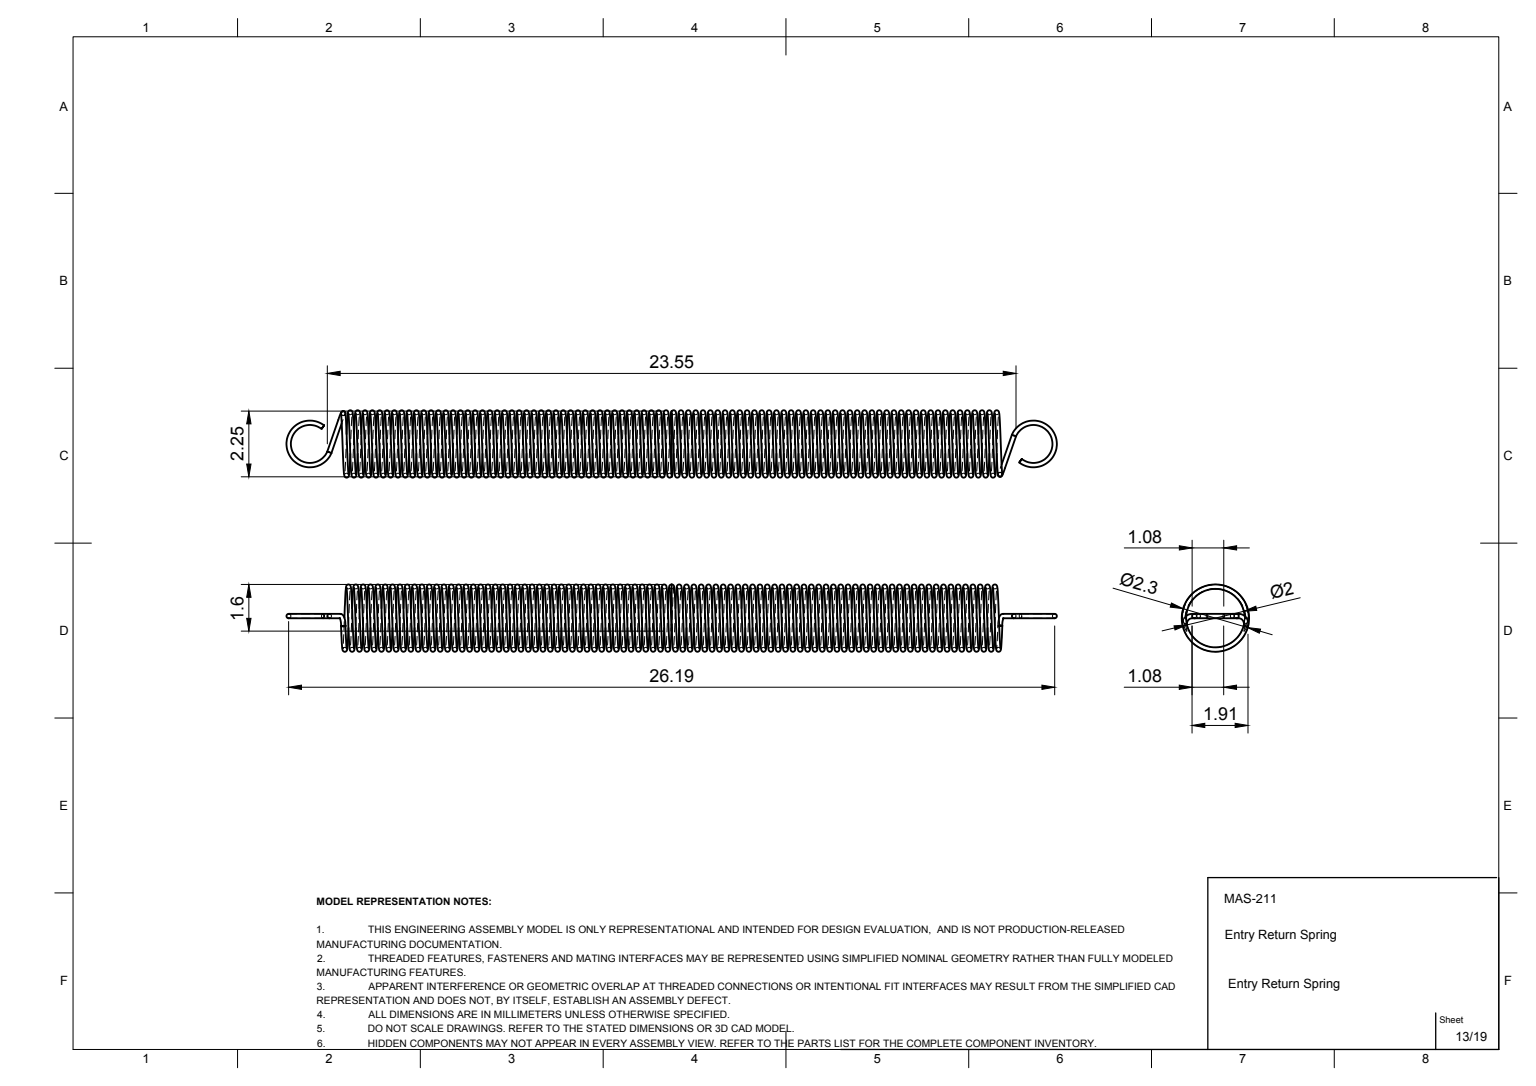
ISO-10303-21;
HEADER;
FILE_DESCRIPTION(
 (''),
 '2;1');
FILE_NAME ( 'Entry Return Spring.step', '2026-10-05T20:07:59+06:00', ( '' ), ( '' ), 'STEP AP214', 'Unspecified', '' );
FILE_SCHEMA (('AUTOMOTIVE_DESIGN { 1 0 10303 214 3 1 1 }'));
ENDSEC;
DATA;
#10=MECHANICAL_DESIGN_GEOMETRIC_PRESENTATION_REPRESENTATION('',(#331),#196741);
#19=(
BOUNDED_CURVE()
B_SPLINE_CURVE(3,(#132841,#132842,#132843,#132844,#132845,#132846,#132847,
#132848,#132849,#132850,#132851,#132852,#132853,#132854,#132855,#132856,
#132857,#132858,#132859,#132860,#132861,#132862,#132863,#132864,#132865,
#132866,#132867,#132868,#132869,#132870,#132871,#132872,#132873,#132874,
#132875,#132876,#132877,#132878,#132879,#132880,#132881,#132882,#132883,
#132884,#132885,#132886,#132887,#132888,#132889,#132890,#132891,#132892,
#132893,#132894,#132895,#132896,#132897,#132898,#132899,#132900,#132901,
#132902,#132903,#132904,#132905,#132906,#132907,#132908,#132909,#132910,
#132911,#132912,#132913,#132914,#132915,#132916,#132917,#132918,#132919,
#132920,#132921,#132922,#132923,#132924,#132925,#132926,#132927,#132928,
#132929,#132930,#132931,#132932,#132933,#132934,#132935,#132936,#132937,
#132938,#132939,#132940,#132941,#132942,#132943,#132944,#132945,#132946,
#132947,#132948,#132949,#132950,#132951,#132952,#132953,#132954,#132955,
#132956,#132957,#132958,#132959,#132960,#132961,#132962,#132963,#132964,
#132965,#132966,#132967,#132968,#132969,#132970,#132971,#132972,#132973,
#132974,#132975,#132976,#132977,#132978,#132979,#132980,#132981,#132982,
#132983,#132984,#132985,#132986,#132987,#132988,#132989,#132990,#132991,
#132992,#132993,#132994,#132995,#132996,#132997,#132998,#132999,#133000,
#133001,#133002,#133003,#133004,#133005,#133006,#133007,#133008,#133009,
#133010,#133011,#133012,#133013,#133014,#133015,#133016,#133017,#133018,
#133019,#133020,#133021,#133022,#133023,#133024,#133025,#133026,#133027,
#133028,#133029,#133030,#133031,#133032,#133033,#133034,#133035,#133036,
#133037,#133038,#133039,#133040,#133041,#133042,#133043,#133044,#133045,
#133046,#133047,#133048,#133049,#133050,#133051,#133052,#133053,#133054,
#133055,#133056,#133057,#133058,#133059,#133060,#133061,#133062,#133063,
#133064,#133065,#133066,#133067,#133068,#133069,#133070,#133071,#133072,
#133073,#133074,#133075,#133076,#133077,#133078,#133079,#133080,#133081,
#133082,#133083,#133084,#133085,#133086,#133087,#133088,#133089,#133090,
#133091,#133092,#133093,#133094,#133095,#133096,#133097,#133098,#133099,
#133100,#133101,#133102,#133103,#133104,#133105,#133106,#133107,#133108,
#133109,#133110,#133111,#133112,#133113,#133114,#133115,#133116,#133117,
#133118,#133119,#133120,#133121,#133122,#133123,#133124,#133125,#133126,
#133127,#133128,#133129,#133130,#133131,#133132,#133133,#133134,#133135,
#133136,#133137,#133138,#133139,#133140,#133141,#133142,#133143,#133144,
#133145,#133146,#133147,#133148,#133149,#133150,#133151,#133152,#133153,
#133154,#133155,#133156,#133157,#133158,#133159,#133160,#133161,#133162,
#133163,#133164,#133165,#133166,#133167,#133168,#133169,#133170,#133171,
#133172,#133173,#133174,#133175,#133176,#133177,#133178,#133179,#133180,
#133181,#133182,#133183,#133184,#133185,#133186,#133187,#133188,#133189,
#133190,#133191,#133192,#133193,#133194,#133195,#133196,#133197,#133198,
#133199,#133200,#133201,#133202,#133203,#133204,#133205,#133206,#133207,
#133208,#133209,#133210,#133211,#133212,#133213,#133214,#133215,#133216,
#133217,#133218,#133219,#133220,#133221,#133222,#133223,#133224,#133225,
#133226,#133227,#133228,#133229,#133230,#133231,#133232,#133233,#133234,
#133235,#133236,#133237,#133238,#133239,#133240,#133241,#133242,#133243,
#133244,#133245,#133246,#133247,#133248,#133249,#133250,#133251,#133252,
#133253,#133254,#133255,#133256,#133257,#133258,#133259,#133260,#133261,
#133262,#133263,#133264,#133265,#133266,#133267,#133268,#133269,#133270,
#133271,#133272,#133273,#133274,#133275,#133276,#133277,#133278,#133279,
#133280,#133281,#133282,#133283,#133284,#133285,#133286,#133287,#133288,
#133289,#133290,#133291,#133292,#133293,#133294,#133295,#133296,#133297,
#133298,#133299,#133300,#133301,#133302,#133303,#133304,#133305,#133306,
#133307,#133308,#133309,#133310,#133311,#133312,#133313,#133314,#133315,
#133316,#133317,#133318,#133319,#133320,#133321,#133322,#133323,#133324,
#133325,#133326,#133327,#133328,#133329,#133330,#133331,#133332,#133333,
#133334,#133335,#133336,#133337,#133338,#133339,#133340,#133341,#133342,
#133343,#133344,#133345,#133346,#133347,#133348,#133349,#133350,#133351,
#133352,#133353,#133354,#133355,#133356,#133357,#133358,#133359,#133360,
#133361,#133362,#133363,#133364,#133365,#133366,#133367,#133368,#133369,
#133370,#133371,#133372,#133373,#133374,#133375,#133376,#133377,#133378,
#133379,#133380,#133381,#133382,#133383,#133384,#133385,#133386,#133387,
#133388,#133389,#133390,#133391,#133392,#133393,#133394,#133395,#133396,
#133397,#133398,#133399,#133400,#133401,#133402,#133403,#133404,#133405,
#133406,#133407,#133408,#133409,#133410,#133411,#133412,#133413,#133414,
#133415,#133416,#133417,#133418,#133419,#133420,#133421,#133422,#133423,
#133424,#133425,#133426,#133427,#133428,#133429,#133430,#133431,#133432,
#133433,#133434,#133435,#133436,#133437,#133438,#133439,#133440,#133441,
#133442,#133443,#133444,#133445,#133446,#133447,#133448,#133449,#133450,
#133451,#133452,#133453,#133454,#133455,#133456,#133457,#133458,#133459,
#133460,#133461,#133462,#133463,#133464,#133465,#133466,#133467,#133468,
#133469,#133470,#133471,#133472,#133473,#133474,#133475,#133476,#133477,
#133478,#133479,#133480,#133481,#133482,#133483,#133484,#133485,#133486,
#133487,#133488,#133489,#133490,#133491,#133492,#133493,#133494,#133495,
#133496,#133497,#133498,#133499,#133500,#133501,#133502,#133503,#133504,
#133505,#133506,#133507,#133508,#133509,#133510,#133511,#133512,#133513,
#133514,#133515,#133516,#133517,#133518,#133519,#133520,#133521,#133522,
#133523,#133524,#133525,#133526,#133527,#133528,#133529,#133530,#133531,
#133532,#133533,#133534,#133535,#133536,#133537,#133538,#133539,#133540,
#133541,#133542,#133543,#133544,#133545,#133546,#133547,#133548,#133549,
#133550,#133551,#133552,#133553,#133554,#133555,#133556,#133557,#133558,
#133559,#133560,#133561,#133562,#133563,#133564,#133565,#133566,#133567,
#133568,#133569,#133570,#133571,#133572,#133573,#133574,#133575,#133576,
#133577,#133578,#133579,#133580,#133581,#133582,#133583,#133584,#133585,
#133586,#133587,#133588,#133589,#133590,#133591,#133592,#133593,#133594,
#133595,#133596,#133597,#133598,#133599,#133600,#133601,#133602,#133603,
#133604,#133605,#133606,#133607,#133608,#133609,#133610,#133611,#133612,
#133613,#133614,#133615,#133616,#133617,#133618,#133619,#133620,#133621,
#133622,#133623,#133624,#133625,#133626,#133627,#133628,#133629,#133630,
#133631,#133632,#133633,#133634,#133635,#133636,#133637,#133638,#133639,
#133640,#133641,#133642,#133643,#133644,#133645,#133646,#133647,#133648,
#133649,#133650,#133651,#133652,#133653,#133654,#133655,#133656,#133657,
#133658,#133659,#133660,#133661,#133662,#133663,#133664,#133665,#133666,
#133667,#133668,#133669,#133670,#133671,#133672,#133673,#133674,#133675,
#133676,#133677,#133678,#133679,#133680,#133681,#133682,#133683,#133684,
#133685,#133686,#133687,#133688,#133689,#133690,#133691,#133692,#133693,
#133694,#133695,#133696,#133697,#133698,#133699,#133700,#133701,#133702,
#133703,#133704,#133705,#133706,#133707,#133708,#133709,#133710,#133711,
#133712,#133713,#133714,#133715,#133716,#133717,#133718,#133719,#133720,
#133721,#133722,#133723,#133724,#133725,#133726,#133727,#133728,#133729,
#133730,#133731,#133732,#133733,#133734,#133735,#133736,#133737,#133738,
#133739,#133740,#133741,#133742,#133743,#133744,#133745,#133746,#133747,
#133748,#133749,#133750,#133751,#133752,#133753,#133754,#133755,#133756,
#133757,#133758,#133759,#133760,#133761,#133762,#133763,#133764,#133765,
#133766,#133767,#133768,#133769,#133770,#133771,#133772,#133773,#133774,
#133775,#133776,#133777,#133778,#133779,#133780,#133781,#133782,#133783,
#133784,#133785,#133786,#133787,#133788,#133789,#133790,#133791,#133792,
#133793,#133794,#133795,#133796,#133797,#133798,#133799,#133800,#133801,
#133802,#133803,#133804,#133805,#133806,#133807,#133808,#133809,#133810,
#133811,#133812,#133813,#133814,#133815,#133816,#133817,#133818,#133819,
#133820,#133821,#133822,#133823,#133824,#133825,#133826,#133827,#133828,
#133829,#133830,#133831,#133832,#133833,#133834,#133835,#133836,#133837,
#133838,#133839,#133840,#133841,#133842,#133843,#133844,#133845,#133846,
#133847,#133848,#133849,#133850,#133851,#133852,#133853,#133854,#133855,
#133856,#133857,#133858,#133859,#133860,#133861,#133862,#133863,#133864,
#133865,#133866,#133867,#133868,#133869,#133870,#133871,#133872,#133873,
#133874,#133875,#133876,#133877,#133878,#133879,#133880,#133881,#133882,
#133883,#133884,#133885,#133886,#133887,#133888,#133889,#133890,#133891,
#133892,#133893,#133894,#133895,#133896,#133897,#133898),.UNSPECIFIED.,
 .F.,.F.)
B_SPLINE_CURVE_WITH_KNOTS((4,1,1,1,1,1,1,1,1,1,1,1,1,1,1,1,1,1,1,1,1,1,
1,1,1,1,1,1,1,1,1,1,1,1,1,1,1,1,1,1,1,1,1,1,1,1,1,1,1,1,1,1,1,1,1,1,1,1,
1,1,1,1,1,1,1,1,1,1,1,1,1,1,1,1,1,1,1,1,1,1,1,1,1,1,1,1,1,1,1,1,1,1,1,1,
1,1,1,1,1,1,1,1,1,1,1,1,1,1,1,1,1,1,1,1,1,1,1,1,1,1,1,1,1,1,1,1,1,1,1,1,
1,1,1,1,1,1,1,1,1,1,1,1,1,1,1,1,1,1,1,1,1,1,1,1,1,1,1,1,1,1,1,1,1,1,1,1,
1,1,1,1,1,1,1,1,1,1,1,1,1,1,1,1,1,1,1,1,1,1,1,1,1,1,1,1,1,1,1,1,1,1,1,1,
1,1,1,1,1,1,1,1,1,1,1,1,1,1,1,1,1,1,1,1,1,1,1,1,1,1,1,1,1,1,1,1,1,1,1,1,
1,1,1,1,1,1,1,1,1,1,1,1,1,1,1,1,1,1,1,1,1,1,1,1,1,1,1,1,1,1,1,1,1,1,1,1,
1,1,1,1,1,1,1,1,1,1,1,1,1,1,1,1,1,1,1,1,1,1,1,1,1,1,1,1,1,1,1,1,1,1,1,1,
1,1,1,1,1,1,1,1,1,1,1,1,1,1,1,1,1,1,1,1,1,1,1,1,1,1,1,1,1,1,1,1,1,1,1,1,
1,1,1,1,1,1,1,1,1,1,1,1,1,1,1,1,1,1,1,1,1,1,1,1,1,1,1,1,1,1,1,1,1,1,1,1,
1,1,1,1,1,1,1,1,1,1,1,1,1,1,1,1,1,1,1,1,1,1,1,1,1,1,1,1,1,1,1,1,1,1,1,1,
1,1,1,1,1,1,1,1,1,1,1,1,1,1,1,1,1,1,1,1,1,1,1,1,1,1,1,1,1,1,1,1,1,1,1,1,
1,1,1,1,1,1,1,1,1,1,1,1,1,1,1,1,1,1,1,1,1,1,1,1,1,1,1,1,1,1,1,1,1,1,1,1,
1,1,1,1,1,1,1,1,1,1,1,1,1,1,1,1,1,1,1,1,1,1,1,1,1,1,1,1,1,1,1,1,1,1,1,1,
1,1,1,1,1,1,1,1,1,1,1,1,1,1,1,1,1,1,1,1,1,1,1,1,1,1,1,1,1,1,1,1,1,1,1,1,
1,1,1,1,1,1,1,1,1,1,1,1,1,1,1,1,1,1,1,1,1,1,1,1,1,1,1,1,1,1,1,1,1,1,1,1,
1,1,1,1,1,1,1,1,1,1,1,1,1,1,1,1,1,1,1,1,1,1,1,1,1,1,1,1,1,1,1,1,1,1,1,1,
1,1,1,1,1,1,1,1,1,1,1,1,1,1,1,1,1,1,1,1,1,1,1,1,1,1,1,1,1,1,1,1,1,1,1,1,
1,1,1,1,1,1,1,1,1,1,1,1,1,1,1,1,1,1,1,1,1,1,1,1,1,1,1,1,1,1,1,1,1,1,1,1,
1,1,1,1,1,1,1,1,1,1,1,1,1,1,1,1,1,1,1,1,1,1,1,1,1,1,1,1,1,1,1,1,1,1,1,1,
1,1,1,1,1,1,1,1,1,1,1,1,1,1,1,1,1,1,1,1,1,1,1,1,1,1,1,1,1,1,1,1,1,1,1,1,
1,1,1,1,1,1,1,1,1,1,1,1,1,1,1,1,1,1,1,1,1,1,1,1,1,1,1,1,1,1,1,1,1,1,1,1,
1,1,1,1,1,1,1,1,1,1,1,1,1,1,1,1,1,1,1,1,1,1,1,1,1,1,1,1,1,1,1,1,1,1,1,1,
1,1,1,1,1,1,1,1,1,1,1,1,1,1,1,1,1,1,1,1,1,1,1,1,1,1,1,1,1,1,1,1,1,1,1,1,
1,1,1,1,1,1,1,1,1,1,1,1,1,1,1,1,1,1,1,1,1,1,1,1,1,1,1,1,1,1,1,1,1,1,1,1,
1,1,1,1,1,1,1,1,1,1,1,1,1,1,1,1,1,1,1,1,1,1,1,1,1,1,1,1,1,1,1,1,1,1,1,1,
1,1,1,1,1,1,1,1,1,1,1,1,1,1,1,1,1,1,1,1,1,1,1,1,1,1,1,1,1,1,1,1,1,1,1,1,
1,1,1,1,1,1,1,1,1,1,1,1,1,1,1,1,1,1,1,1,1,1,1,1,1,1,1,1,1,1,1,1,1,1,1,1,
1,1,1,1,1,1,1,1,1,1,1,1,1,1,1,1,1,1,1,1,1,1,1,1,1,4),(0.,0.01797683372391,
0.286633051710584,0.555289278308216,0.823945516665782,1.09260176953922,
1.36125803873948,1.62991432588463,1.89857063164012,2.16722695661301,2.43588330050525,
2.70453966304674,2.9731960431531,3.24185243981471,3.51050885133453,3.77916527610465,
4.04782171198515,4.31647815691489,4.58513460847725,4.85379106430677,5.12244752187208,
5.39110397865606,5.65976043217153,5.92841687990537,6.19707331956994,6.46572974881596,
6.73438616570634,7.00304256821933,7.2716989549161,7.5403553242696,7.809011675483,
8.07766800769526,8.34632432089157,8.61498061505147,8.8836368910788,9.15229314997201,
9.4209493936865,9.68960562442157,9.95826184531348,10.226918059948,10.4955742727586,
10.7642304884925,11.0328867113173,11.3015429448574,11.5701991918227,11.8388554546081,
12.1075117346518,12.3761680332469,12.6448243507434,12.9134806874637,13.1821370428496,
13.450793416388,13.7194498067883,13.9881062128412,14.2567626326955,14.5254190645885,
14.7940755062772,15.0627319555912,15.3313884100611,15.6000448672586,15.8687013246492,
16.1373577797,16.4060142299691,16.6746706729765,16.9433271065265,17.2119835283531,
17.4806399366567,17.7492963295502,18.0179527057767,18.286609063996,18.555265403637,
18.8239217240786,19.0925780255742,19.3612343083975,19.6298905737625,19.898546823017,
20.1672030584666,20.4358592827168,20.7045154992928,20.973171712245,21.2418279262962,
21.5104841459723,21.7791403749736,22.0477966165324,22.316452872948,22.585109146262,
22.8537654375589,23.1224217478187,23.3910780770929,23.6597344254327,23.9283907920352,
24.197047176159,24.4657035763222,24.7343599911301,25.0030164185931,25.2716728568073,
25.5403293034427,25.8089857562333,26.0776422126729,26.3462986702843,26.6149551265448,
26.8836115789212,27.1522680250308,27.4209244624423,27.6895808890659,27.9582373027346,
28.2268937018004,28.4955500845261,28.7642064498512,29.0328627966379,29.3015191245544,
29.5701754332357,29.838831723217,30.1074879950829,30.3761442503694,30.6448004907916,
30.9134567190168,31.1821129380756,31.450769151893,31.7194253649682,31.9880815819663,
32.2567378070174,32.5253940433706,32.7940502938785,33.0627065604467,33.3313628447765,
33.6000191476151,33.8686754696427,34.1373318106287,34.405988170366,34.6746445478242,
34.9433009420458,35.2119573513747,35.480613774244,35.7492702085419,36.0179266522368,
36.2865831029275,36.5552395582669,36.8238960157264,37.0925524727952,37.3612089269773,
37.6298653757534,37.8985218168153,38.1671782477952,38.4358346667239,38.7044910715485,
38.9731474607866,39.2418038328672,39.5104601869391,39.7791165220837,40.0477728382212,
40.3164291352602,40.5850854140292,40.8537416754418,41.1223979213679,41.3910541539077,
41.6597103761025,41.9283665914244,42.1970228042084,42.4656790192,42.7343352406829,
43.0029914723808,43.2716477171096,43.540303977354,43.8089602546436,44.0776165503516,
44.3462728649052,44.614929198697,44.883585551232,45.1522419220568,45.4208983099307,
45.6895547136931,45.9582111315299,46.2268675617156,46.4955240020317,46.7641804503338,
47.0328369041642,47.3014933611089,47.5701498186329,47.8388062742058,48.107462725373,
48.3761191696448,48.6447756048012,48.9134320285537,49.1820884390673,49.4507448344197,
49.7194012133072,49.9880575743413,50.2567139168934,50.5253702402807,50.7940265446884,
51.0626828303152,51.3313390982961,51.5999953498901,51.8686515873141,52.1373078130706,
52.4059640305862,52.6746202437936,52.9432764573682,53.211932675918,53.480588903259,
53.7492451427202,54.0179013967021,54.2865576673334,54.5552139557853,54.823870263115,
55.0925265894471,55.3611829348992,55.6298392987282,55.8984956802486,56.1671520780245,
56.4358084907065,56.7044649163381,56.9731213530494,57.2417777985307,57.5104342505384,
57.7790907065743,58.0477471641719,58.3164036208043,58.5850600739368,58.8537165211707,
59.1223729600609,59.39102938849,59.6596858042645,59.9283422056975,60.1969985910129,
60.4656549590995,60.7343113087676,61.0029676396243,61.2716239512389,61.540280244075,
61.808936518638,62.0775927763821,62.3462490189291,62.6149052488546,62.8835614690812,
63.1522176834332,63.4208738963055,63.6895301124163,63.9581863359981,64.2268425704115,
64.4954988186027,64.7641550825741,65.0328113641112,65.3014676640435,65.5701239831253,
65.8387803211949,66.1074366781083,66.3760930528907,66.6447494446373,66.9134058517341,
67.1820622726558,67.4507187053199,67.7193751477252,67.988031597487,68.256688052277,
68.5253445095709,68.7940009668648,69.0626574216546,69.3313138714164,69.5999703138218,
69.8686267464858,70.1372831674076,70.4059395745042,70.6745959662509,70.9432523410334,
71.2119086979469,71.4805650360164,71.7492213550982,72.0178776550306,72.2865339365675,
72.5551902005389,72.8238464487301,73.0925026831433,73.3611589067251,73.6298151228357,
73.8984713357081,74.1671275500599,74.4357837702864,74.7044400002118,74.9730962427587,
75.2417525005027,75.5104087750655,75.7790650679015,76.047721379516,76.3163777103726,
76.5850340600405,76.853690428127,77.1223468134422,77.391003214875,77.6596596306495,
77.9283160590784,78.1969724979684,78.4656289452021,78.7342853983344,79.0029418549666,
79.2715983125641,79.5402547685998,79.8089112206075,80.0775676660886,80.3462241027997,
80.6148805284312,80.8835369411131,81.1521933388889,81.4208497204091,81.689506084238,
81.9581624296899,82.2268187560219,82.4954750633515,82.7641313518033,83.0327876224345,
83.3014438764161,83.5701001158772,83.838756343218,84.1074125617677,84.3760687753422,
84.6447249885494,84.913381206065,85.1820374318212,85.4506936692451,85.719349920839,
85.9880061888197,86.2566624744465,86.5253187788541,86.7939751022413,87.0626314447932,
87.3312878058273,87.5999441847146,87.8686005800667,88.1372569905802,88.4059134143327,
88.6745698494889,88.9432262937606,89.2118827449277,89.4805392005005,89.7491956580243,
90.0178521149689,90.2865085687992,90.5551650171012,90.8238214574172,91.0924778876028,
91.3611343054394,91.6297907092016,91.8984470970753,92.1671034679,92.4357598204347,
92.7044161542264,92.9730724687798,93.2417287644878,93.5103850417773,93.7790413020216,
94.0476975467502,94.3163537784479,94.5850099999307,94.8536662149221,95.1223224277061,
95.390978643028,95.6596348652226,95.9282910977624,96.1969473436883,96.4656036051009,
96.7342598838697,97.0029161809086,97.2715724970461,97.5402288321905,97.8088851862623,
98.0775415583427,98.3461979475807,98.6148543524051,98.8835107713336,99.1521672023136,
99.4208236433754,99.6894800921513,99.9581365463333,100.226793003402,100.495449460861,
100.7641059162,101.032762366891,101.301418810586,101.570075244884,101.838731667753,
102.107388077082,102.376044471303,102.644700848761,102.913357208498,103.182013549484,
103.450669871511,103.71932617435,103.98798245868,104.256638725248,104.525294975755,
104.793951212108,105.062607437159,105.331263654157,105.599919867233,105.86857608105,
106.137232300108,106.405888528334,106.674544768756,106.943201024042,107.211857295908,
107.480513585889,107.74916989457,108.017826222487,108.286482569273,108.555138934598,
108.823795317324,109.09245171639,109.361108130058,109.629764556682,109.898420994093,
110.167077440202,110.435733892579,110.704390348839,110.97304680645,111.24170326289,
111.51035971568,111.779016162316,112.04767260053,112.316329027993,112.5849854428,
112.853641842963,113.122298227087,113.39095459369,113.659610942029,113.928267271303,
114.196923581563,114.46557987286,114.734236146174,115.002892402589,115.271548644148,
115.540204873149,115.808861092825,116.077517306876,116.346173519828,116.614829736404,
116.883485960654,117.152142196103,117.420798445358,117.689454710722,117.958110993546,
118.226767295041,118.495423615483,118.764079955123,119.032736313343,119.301392689569,
119.570049082462,119.838705490766,120.107361912592,120.376018346142,120.644674789149,
120.913331239418,121.181987694469,121.45064415186,121.719300609057,121.987957063527,
122.256613512841,122.525269954529,122.793926386422,123.062582806276,123.331239212329,
123.599895602729,123.868551976268,124.137208331653,124.405864668374,124.67452098587,
124.943177284465,125.211833564508,125.480489827294,125.749146074259,126.017802307799,
126.286458530624,126.555114746357,126.823770959168,127.092427173802,127.361083394694,
127.629739625429,127.898395869143,128.167052128037,128.435708404064,128.704364698224,
128.97302101142,129.241677343633,129.510333694846,129.7789900642,130.047646450897,
130.31630285341,130.5849592703,130.853615699547,131.122272139211,131.390928586945,
131.659585040461,131.928241497245,132.19689795481,132.46555441064,132.734210862202,
133.002867307132,133.271523743013,133.540180167783,133.808836579303,134.077492975965,
134.346149356071,134.614805718613,134.883462062505,135.152118387478,135.420774693234,
135.689430980379,135.958087249579,136.226743502453,136.49539974081,136.76405596741,
137.032712185392,137.301368398783,137.570024612174,137.838680830155,138.107337056755,
138.375993295112,138.644649547986,138.913305817186,139.181962104332,139.450618410087,
139.71927473506,139.987931078952,140.256587441494,140.525243821601,140.793900218262,
141.062556629782,141.331213054552,141.599869490433,141.868525935363,142.137182386925,
142.405838842755,142.67449530032,142.943151757104,143.21180821062,143.480464658354,
143.749121098019,144.017777527265,144.286433944155,144.555090346668,144.823746733365,
145.092403102719,145.361059453932,145.629715786145,145.898372099341,146.167028393501,
146.435684669529,146.704340928422,146.972997172137,147.241653402872,147.510309623764,
147.778965838398,148.047622051209,148.316278266943,148.584934489768,148.853590723308,
149.122246970274,149.390903233059,149.659559513103,149.928215811698,150.196872129195,
150.465528465915,150.734184821301,151.00284119484,151.27149758524,151.540153991293,
151.808810411148,152.077466843041,152.34612328473,152.614779734044,152.883436188514,
153.152092645711,153.420749103102,153.689405558153,153.958062008422,154.22671845143,
154.49537488498,154.764031306806,155.03268771511,155.301344108004,155.57000048423,
155.838656842449,156.107313182091,156.375969502532,156.644625804028,156.913282086851,
157.181938352216,157.450594601471,157.719250836921,157.987907061171,158.256563277747,
158.525219490699,158.793875704751,159.062531924427,159.331188153428,159.599844394987,
159.868500651403,160.137156924717,160.405813216014,160.674469526274,160.943125855548,
161.211782203888,161.480438570491,161.749094954615,162.017751354778,162.286407769586,
162.555064197049,162.823720635263,163.092377081899,163.361033534689,163.629689991129,
163.898346448741,164.167002905001,164.435659357378,164.704315803488,164.972972240899,
165.241628667523,165.510285081192,165.778941480257,166.047597862983,166.316254228308,
166.584910575095,166.853566903012,167.122223211693,167.390879501675,167.659535773541,
167.928192028827,168.19684826925,168.465504497475,168.734160716534,169.002816930351,
169.271473143427,169.540129360425,169.808785585476,170.077441821829,170.346098072337,
170.614754338905,170.883410623235,171.152066926074,171.420723248102,171.689379589088,
171.958035948825,172.226692326284,172.495348720505,172.764005129834,173.032661552704,
173.301317987002,173.569974430697,173.838630881388,174.107287336727,174.375943794187,
174.644600251255,174.913256705437,175.181913154214,175.450569595276,175.719226026256,
175.987882445184,176.256538850009,176.525195239247,176.793851611328,177.0625079654,
177.331164300545,177.599820616682,177.868476913721,178.137133192491,178.405789453903,
178.674445699829,178.943101932369,179.211758154564,179.480414369886,179.74907058267,
180.017726797662,180.286383019145,180.555039250843,180.823695495572,181.092351755816,
181.361008033106,181.629664328814,181.898320643368,182.16697697716,182.435633329695,
182.70428970052,182.972946088394,183.241602492156,183.510258909993,183.778915340179,
184.047571780495,184.316228228797,184.584884682628,184.853541139572,185.122197597096,
185.39085405267,185.659510503837,185.928166948109,186.196823383265,186.465479807018,
186.734136217531,187.002792612884,187.271448991771,187.540105352806,187.808761695358,
188.077418018745,188.346074323153,188.61473060878,188.883386876761,189.152043128355,
189.420699365779,189.689355591536,189.958011809051,190.226668022259,190.495324235834,
190.763980454383,191.032636681725,191.301292921186,191.569949175168,191.838605445799,
192.107261734251,192.375918041581,192.644574367913,192.913230713365,193.181887077194,
193.450543458715,193.719199856491,193.987856269173,194.256512694805,194.525169131516,
194.793825576997,195.062482029005,195.331138485041,195.599794942639,195.868451399271,
196.137107852404,196.405764299638,196.674420738528,196.943077166957,197.211733582732,
197.480389984165,197.749046369481,198.017702737567,198.286359087236,198.555015418092,
198.823671729707,199.092328022543,199.360984297106,199.62964055485,199.898296797397,
200.166953027323,200.43560924755,200.704265461902,200.972921674774,201.241577890885,
201.510234114467,201.77889034888,202.047546597072,202.316202861043,202.584859142581,
202.853515442513,203.122171761595,203.390828099665,203.659484456579,203.928140831361,
204.196797223108,204.465453630205,204.734110051127,205.002766483791,205.271422926197,
205.540079375959,205.808735830749,206.077392288043,206.346048745337,206.614705200127,
206.883361649889,207.152018092295,207.420674524959,207.689330945881,207.957987352978,
208.226643744725,208.495300119508,208.763956476421,209.032612814491,209.301269133573,
209.569925433505,209.838581715043,210.107237979014,210.375894227206,210.644550461619,
210.913206685201,211.181862901312,211.450519114184,211.719175328536,211.987831548763,
212.256487778689,212.525144021236,212.79380027898,213.062456553543,213.331112846379,
213.599769157994,213.868425488851,214.137081838519,214.405738206606,214.674394591921,
214.943050993354,215.211707409129,215.480363837558,215.749020276448,216.017676723682,
216.286333176815,216.554989633447,216.823646091045,217.092302547081,217.360958999089,
217.62961544457,217.898271881281,218.166928306913,218.435584719595,218.704241117371,
218.972897498892,219.241553862721,219.510210208173,219.778866534505,220.047522841835,
220.316179130287,220.584835400918,220.8534916549,221.122147894361,221.390804121702,
221.659460340252,221.928116553827,222.196772767034,222.46542898455,222.734085210306,
223.00274144773,223.271397699324,223.540053967305,223.808710252932,224.07736655734,
224.346022880728,224.61467922328,224.883335584314,225.151991963201,225.420648358554,
225.689304769068,225.95796119282,226.226617627977,226.495274072249,226.763930523416,
227.032586978989,227.301243436513,227.569899893458,227.838556347288,228.10721279559,
228.375869235907,228.644525666093,228.913182083929,229.181838487692,229.450494875566,
229.719151246391,229.987807598926,230.256463932718,230.525120247271,230.79377654298,
231.062432820269,231.331089080514,231.599745325243,231.868401556941,232.137057778424,
232.405713993415,232.674370206199,232.943026421521,233.211682643716,233.480338876256,
233.748995122182,234.017651383595,234.286307662364,234.554963959403,234.823620275541,
235.092276610685,235.360932964757,235.629589336838,235.898245726076,236.166902130901,
236.43555854983,236.70421498081,236.972871421872,237.241527870648,237.51018432483,
237.778840781899,238.047497239359,238.316153694698,238.584810145389,238.853466589084,
239.122123023382,239.390779446251,239.65943585558,239.928092249802,240.19674862726,
240.465404986998,240.734061327984,241.002717650011,241.27137395285,241.54003023718,
241.808686503748,242.077342754256,242.345998990609,242.614655215661,242.883311432659,
243.151967645734,243.420623859552,243.68928007861,243.957936306836,244.226592547258,
244.495248802545,244.763905074411,245.032561364392,245.301217673074,245.56987400099,
245.838530347777,246.107186713102,246.375843095828,246.644499494894,246.913155908563,
247.181812335186,247.450468772598,247.719125218708,247.987781671084,248.256438127345,
248.525094584956,248.793751041396,249.062407494187,249.331063940822,249.599720379036,
249.8683768065,250.137033221308,250.405689621471,250.674346005595,250.943002372197,
251.211658720537,251.480315049812,251.748971360071,252.017627651368,252.286283924683,
252.554940181098,252.823596422657,253.092252651658,253.360908871335,253.629565085386,
253.898221298338,254.166877514914,254.435533739165,254.704189974614,254.972846223869,
255.241502489234,255.510158772057,255.778815073553,256.047471393995,256.316127733635,
256.584784091854,256.85344046808,257.122096860973,257.390753269276,257.659409691102,
257.928066124652,258.196722567659,258.465379017928,258.734035472978,259.002691930368,
259.271348387566,259.540004842035,259.808661291349,260.077317733037,260.345974164929,
260.614630584783,260.883286990836,261.151943381235,261.420599754774,261.689256110159,
261.957912446879,262.226568764375,262.49522506297,262.763881343014,263.032537605798,
263.301193852763,263.569850086303,263.838506309127,264.107162524861,264.375818737671,
264.644474952305,264.913131173196,265.181787403931,265.450443647645,265.719099906538,
265.987756182565,266.256412476724,266.52506878992,266.793725122132,267.062381473345,
267.331037842698,267.599694229394,267.868350631907,268.137007048797,268.405663478042,
268.674319917706,268.94297636544,269.211632818955,269.480289275739,269.748945733304,
270.017602189133,270.286258640695,270.554915085624,270.823571521504,271.092227946274,
271.360884357793,271.629540754454,271.89819713456,272.166853497101,272.435509840993,
272.704166165965,272.97282247172,273.241478758865,273.510135028065,273.778791280938,
274.047447519295,274.316103745894,274.584759963875,274.853416177266,275.122072390656,
275.390728608637,275.659384835237,275.928041073593,276.196697326466,276.465353595666,
276.734009882811,277.002666188566,277.271322513539,277.53997885743,277.808635219972,
278.077291600077,278.345947996739,278.614604408258,278.883260833028,279.151917268908,
279.420573713837,279.689230165399,279.957886621228,280.226543078793,280.495199535576,
280.763855989092,281.032512436825,281.301168876489,281.569825305735,281.838481722625,
282.107138125138,282.375794511834,282.644450881187,282.9131072324,283.140531716307),
 .UNSPECIFIED.)
CURVE()
GEOMETRIC_REPRESENTATION_ITEM()
RATIONAL_B_SPLINE_CURVE((1.,1.,1.,1.,1.,1.,1.,1.,1.,1.,1.,1.,1.,1.,1.,1.,
1.,1.,1.,1.,1.,1.,1.,1.,1.,1.,1.,1.,1.,1.,1.,1.,1.,1.,1.,1.,1.,1.,1.,1.,
1.,1.,1.,1.,1.,1.,1.,1.,1.,1.,1.,1.,1.,1.,1.,1.,1.,1.,1.,1.,1.,1.,1.,1.,
1.,1.,1.,1.,1.,1.,1.,1.,1.,1.,1.,1.,1.,1.,1.,1.,1.,1.,1.,1.,1.,1.,1.,1.,
1.,1.,1.,1.,1.,1.,1.,1.,1.,1.,1.,1.,1.,1.,1.,1.,1.,1.,1.,1.,1.,1.,1.,1.,
1.,1.,1.,1.,1.,1.,1.,1.,1.,1.,1.,1.,1.,1.,1.,1.,1.,1.,1.,1.,1.,1.,1.,1.,
1.,1.,1.,1.,1.,1.,1.,1.,1.,1.,1.,1.,1.,1.,1.,1.,1.,1.,1.,1.,1.,1.,1.,1.,
1.,1.,1.,1.,1.,1.,1.,1.,1.,1.,1.,1.,1.,1.,1.,1.,1.,1.,1.,1.,1.,1.,1.,1.,
1.,1.,1.,1.,1.,1.,1.,1.,1.,1.,1.,1.,1.,1.,1.,1.,1.,1.,1.,1.,1.,1.,1.,1.,
1.,1.,1.,1.,1.,1.,1.,1.,1.,1.,1.,1.,1.,1.,1.,1.,1.,1.,1.,1.,1.,1.,1.,1.,
1.,1.,1.,1.,1.,1.,1.,1.,1.,1.,1.,1.,1.,1.,1.,1.,1.,1.,1.,1.,1.,1.,1.,1.,
1.,1.,1.,1.,1.,1.,1.,1.,1.,1.,1.,1.,1.,1.,1.,1.,1.,1.,1.,1.,1.,1.,1.,1.,
1.,1.,1.,1.,1.,1.,1.,1.,1.,1.,1.,1.,1.,1.,1.,1.,1.,1.,1.,1.,1.,1.,1.,1.,
1.,1.,1.,1.,1.,1.,1.,1.,1.,1.,1.,1.,1.,1.,1.,1.,1.,1.,1.,1.,1.,1.,1.,1.,
1.,1.,1.,1.,1.,1.,1.,1.,1.,1.,1.,1.,1.,1.,1.,1.,1.,1.,1.,1.,1.,1.,1.,1.,
1.,1.,1.,1.,1.,1.,1.,1.,1.,1.,1.,1.,1.,1.,1.,1.,1.,1.,1.,1.,1.,1.,1.,1.,
1.,1.,1.,1.,1.,1.,1.,1.,1.,1.,1.,1.,1.,1.,1.,1.,1.,1.,1.,1.,1.,1.,1.,1.,
1.,1.,1.,1.,1.,1.,1.,1.,1.,1.,1.,1.,1.,1.,1.,1.,1.,1.,1.,1.,1.,1.,1.,1.,
1.,1.,1.,1.,1.,1.,1.,1.,1.,1.,1.,1.,1.,1.,1.,1.,1.,1.,1.,1.,1.,1.,1.,1.,
1.,1.,1.,1.,1.,1.,1.,1.,1.,1.,1.,1.,1.,1.,1.,1.,1.,1.,1.,1.,1.,1.,1.,1.,
1.,1.,1.,1.,1.,1.,1.,1.,1.,1.,1.,1.,1.,1.,1.,1.,1.,1.,1.,1.,1.,1.,1.,1.,
1.,1.,1.,1.,1.,1.,1.,1.,1.,1.,1.,1.,1.,1.,1.,1.,1.,1.,1.,1.,1.,1.,1.,1.,
1.,1.,1.,1.,1.,1.,1.,1.,1.,1.,1.,1.,1.,1.,1.,1.,1.,1.,1.,1.,1.,1.,1.,1.,
1.,1.,1.,1.,1.,1.,1.,1.,1.,1.,1.,1.,1.,1.,1.,1.,1.,1.,1.,1.,1.,1.,1.,1.,
1.,1.,1.,1.,1.,1.,1.,1.,1.,1.,1.,1.,1.,1.,1.,1.,1.,1.,1.,1.,1.,1.,1.,1.,
1.,1.,1.,1.,1.,1.,1.,1.,1.,1.,1.,1.,1.,1.,1.,1.,1.,1.,1.,1.,1.,1.,1.,1.,
1.,1.,1.,1.,1.,1.,1.,1.,1.,1.,1.,1.,1.,1.,1.,1.,1.,1.,1.,1.,1.,1.,1.,1.,
1.,1.,1.,1.,1.,1.,1.,1.,1.,1.,1.,1.,1.,1.,1.,1.,1.,1.,1.,1.,1.,1.,1.,1.,
1.,1.,1.,1.,1.,1.,1.,1.,1.,1.,1.,1.,1.,1.,1.,1.,1.,1.,1.,1.,1.,1.,1.,1.,
1.,1.,1.,1.,1.,1.,1.,1.,1.,1.,1.,1.,1.,1.,1.,1.,1.,1.,1.,1.,1.,1.,1.,1.,
1.,1.,1.,1.,1.,1.,1.,1.,1.,1.,1.,1.,1.,1.,1.,1.,1.,1.,1.,1.,1.,1.,1.,1.,
1.,1.,1.,1.,1.,1.,1.,1.,1.,1.,1.,1.,1.,1.,1.,1.,1.,1.,1.,1.,1.,1.,1.,1.,
1.,1.,1.,1.,1.,1.,1.,1.,1.,1.,1.,1.,1.,1.,1.,1.,1.,1.,1.,1.,1.,1.,1.,1.,
1.,1.,1.,1.,1.,1.,1.,1.,1.,1.,1.,1.,1.,1.,1.,1.,1.,1.,1.,1.,1.,1.,1.,1.,
1.,1.,1.,1.,1.,1.,1.,1.,1.,1.,1.,1.,1.,1.,1.,1.,1.,1.,1.,1.,1.,1.,1.,1.,
1.,1.,1.,1.,1.,1.,1.,1.,1.,1.,1.,1.,1.,1.,1.,1.,1.,1.,1.,1.,1.,1.,1.,1.,
1.,1.,1.,1.,1.,1.,1.,1.,1.,1.,1.,1.,1.,1.,1.,1.,1.,1.,1.,1.,1.,1.,1.,1.,
1.,1.,1.,1.,1.,1.,1.,1.,1.,1.,1.,1.,1.,1.,1.,1.,1.,1.,1.,1.,1.,1.,1.,1.,
1.,1.,1.,1.,1.,1.,1.,1.,1.,1.,1.,1.,1.,1.,1.,1.,1.,1.,1.,1.,1.,1.,1.,1.,
1.,1.,1.,1.,1.,1.,1.,1.,1.,1.,1.,1.,1.,1.,1.,1.,1.,1.,1.,1.,1.,1.,1.,1.,
1.,1.,1.,1.,1.,1.,1.,1.,1.,1.,1.,1.,1.,1.,1.,1.,1.,1.,1.,1.,1.,1.,1.,1.,
1.,1.,1.,1.,1.,1.,1.,1.,1.,1.,1.,1.,1.,1.,1.,1.,1.,1.,1.,1.,1.,1.,1.,1.,
1.,1.,1.,1.,1.,1.,1.,1.,1.,1.,1.,1.,1.,1.,1.,1.,1.,1.,1.,1.,1.,1.,1.,1.,
1.,1.,1.,1.,1.,1.,1.,1.,1.,1.,1.,1.,1.,1.,1.,1.,1.,1.,1.,1.,1.,1.,1.,1.,
1.,1.,1.,1.,1.,1.,1.,1.,1.,1.))
REPRESENTATION_ITEM('')
) ;
#20=(
BOUNDED_CURVE()
B_SPLINE_CURVE(3,(#134125,#134126,#134127,#134128,#134129,#134130,#134131),
 .UNSPECIFIED.,.F.,.F.)
B_SPLINE_CURVE_WITH_KNOTS((4,1,1,1,4),(0.,0.0911446219616379,0.182289243923276,
0.273433865884915,0.364578487846551),.UNSPECIFIED.)
CURVE()
GEOMETRIC_REPRESENTATION_ITEM()
RATIONAL_B_SPLINE_CURVE((1.,1.,1.,1.,1.,1.,1.))
REPRESENTATION_ITEM('')
) ;
#21=(
BOUNDED_CURVE()
B_SPLINE_CURVE(3,(#134347,#134348,#134349,#134350,#134351,#134352,#134353,
#134354,#134355,#134356,#134357,#134358,#134359,#134360,#134361,#134362,
#134363,#134364,#134365),.UNSPECIFIED.,.F.,.F.)
B_SPLINE_CURVE_WITH_KNOTS((4,1,1,1,1,1,1,1,1,1,1,1,1,1,1,1,4),(0.,0.226732296973331,
0.464902013928651,0.70307173088397,0.9298040278573,1.15653632483063,1.39470604178595,
1.63287575874127,1.8596080557146,2.08634035268793,2.32451006964325,2.56267978659857,
2.7894120835719,3.01614438054523,3.25431409750055,3.49248381445586,3.7192161114292),
 .UNSPECIFIED.)
CURVE()
GEOMETRIC_REPRESENTATION_ITEM()
RATIONAL_B_SPLINE_CURVE((1.,1.,1.,1.,1.,1.,1.,1.,1.,1.,1.,1.,1.,1.,1.,1.,
1.,1.,1.))
REPRESENTATION_ITEM('')
) ;
#22=(
BOUNDED_CURVE()
B_SPLINE_CURVE(3,(#152830,#152831,#152832,#152833,#152834,#152835,#152836,
#152837,#152838,#152839,#152840,#152841,#152842,#152843,#152844,#152845,
#152846,#152847,#152848,#152849,#152850,#152851,#152852,#152853,#152854,
#152855,#152856,#152857,#152858,#152859,#152860,#152861,#152862,#152863,
#152864,#152865,#152866,#152867,#152868,#152869,#152870,#152871,#152872,
#152873,#152874,#152875,#152876,#152877,#152878,#152879,#152880,#152881,
#152882,#152883,#152884,#152885,#152886,#152887,#152888,#152889,#152890,
#152891,#152892,#152893,#152894,#152895,#152896,#152897,#152898,#152899,
#152900,#152901,#152902,#152903,#152904,#152905,#152906,#152907,#152908,
#152909,#152910,#152911,#152912,#152913,#152914,#152915,#152916,#152917,
#152918,#152919,#152920,#152921,#152922,#152923,#152924,#152925,#152926,
#152927,#152928,#152929,#152930,#152931,#152932,#152933,#152934,#152935,
#152936,#152937,#152938,#152939,#152940,#152941,#152942,#152943,#152944,
#152945,#152946,#152947,#152948,#152949,#152950,#152951,#152952,#152953,
#152954,#152955,#152956,#152957,#152958,#152959,#152960,#152961,#152962,
#152963,#152964,#152965,#152966,#152967,#152968,#152969,#152970,#152971,
#152972,#152973,#152974,#152975,#152976,#152977,#152978,#152979,#152980,
#152981,#152982,#152983,#152984,#152985,#152986,#152987,#152988,#152989,
#152990,#152991,#152992,#152993,#152994,#152995,#152996,#152997,#152998,
#152999,#153000,#153001,#153002,#153003,#153004,#153005,#153006,#153007,
#153008,#153009,#153010,#153011,#153012,#153013,#153014,#153015,#153016,
#153017,#153018,#153019,#153020,#153021,#153022,#153023,#153024,#153025,
#153026,#153027,#153028,#153029,#153030,#153031,#153032,#153033,#153034,
#153035,#153036,#153037,#153038,#153039,#153040,#153041,#153042,#153043,
#153044,#153045,#153046,#153047,#153048,#153049,#153050,#153051,#153052,
#153053,#153054,#153055,#153056,#153057,#153058,#153059,#153060,#153061,
#153062,#153063,#153064,#153065,#153066,#153067,#153068,#153069,#153070,
#153071,#153072,#153073,#153074,#153075,#153076,#153077,#153078,#153079,
#153080,#153081,#153082,#153083,#153084,#153085,#153086,#153087,#153088,
#153089,#153090,#153091,#153092,#153093,#153094,#153095,#153096,#153097,
#153098,#153099,#153100,#153101,#153102,#153103,#153104,#153105,#153106,
#153107,#153108,#153109,#153110,#153111,#153112,#153113,#153114,#153115,
#153116,#153117,#153118,#153119,#153120,#153121,#153122,#153123,#153124,
#153125,#153126,#153127,#153128,#153129,#153130,#153131,#153132,#153133,
#153134,#153135,#153136,#153137,#153138,#153139,#153140,#153141,#153142,
#153143,#153144,#153145,#153146,#153147,#153148,#153149,#153150,#153151,
#153152,#153153,#153154,#153155,#153156,#153157,#153158,#153159,#153160,
#153161,#153162,#153163,#153164,#153165,#153166,#153167,#153168,#153169,
#153170,#153171,#153172,#153173,#153174,#153175,#153176,#153177,#153178,
#153179,#153180,#153181,#153182,#153183,#153184,#153185,#153186,#153187,
#153188,#153189,#153190,#153191,#153192,#153193,#153194,#153195,#153196,
#153197,#153198,#153199,#153200,#153201,#153202,#153203,#153204,#153205,
#153206,#153207,#153208,#153209,#153210,#153211,#153212,#153213,#153214,
#153215,#153216,#153217,#153218,#153219,#153220,#153221,#153222,#153223,
#153224,#153225,#153226,#153227,#153228,#153229,#153230,#153231,#153232,
#153233,#153234,#153235,#153236,#153237,#153238,#153239,#153240,#153241,
#153242,#153243,#153244,#153245,#153246,#153247,#153248,#153249,#153250,
#153251,#153252,#153253,#153254,#153255,#153256,#153257,#153258,#153259,
#153260,#153261,#153262,#153263,#153264,#153265,#153266,#153267,#153268,
#153269,#153270,#153271,#153272,#153273,#153274,#153275,#153276,#153277,
#153278,#153279,#153280,#153281,#153282,#153283,#153284,#153285,#153286,
#153287,#153288,#153289,#153290,#153291,#153292,#153293,#153294,#153295,
#153296,#153297,#153298,#153299,#153300,#153301,#153302,#153303,#153304,
#153305,#153306,#153307,#153308,#153309,#153310,#153311,#153312,#153313,
#153314,#153315,#153316,#153317,#153318,#153319,#153320,#153321,#153322,
#153323,#153324,#153325,#153326,#153327,#153328,#153329,#153330,#153331,
#153332,#153333,#153334,#153335,#153336,#153337,#153338,#153339,#153340,
#153341,#153342,#153343,#153344,#153345,#153346,#153347,#153348,#153349,
#153350,#153351,#153352,#153353,#153354,#153355,#153356,#153357,#153358,
#153359,#153360,#153361,#153362,#153363,#153364,#153365,#153366,#153367,
#153368,#153369,#153370,#153371,#153372,#153373,#153374,#153375,#153376,
#153377,#153378,#153379,#153380,#153381,#153382,#153383,#153384,#153385,
#153386,#153387,#153388,#153389,#153390,#153391,#153392,#153393,#153394,
#153395,#153396,#153397,#153398,#153399,#153400,#153401,#153402,#153403,
#153404,#153405,#153406,#153407,#153408,#153409,#153410,#153411,#153412,
#153413,#153414,#153415,#153416,#153417,#153418,#153419,#153420,#153421,
#153422,#153423,#153424,#153425,#153426,#153427,#153428,#153429,#153430,
#153431,#153432,#153433,#153434,#153435,#153436,#153437,#153438,#153439,
#153440,#153441,#153442,#153443,#153444,#153445,#153446,#153447,#153448,
#153449,#153450,#153451,#153452,#153453,#153454,#153455,#153456,#153457,
#153458,#153459,#153460,#153461,#153462,#153463,#153464,#153465,#153466,
#153467,#153468,#153469,#153470,#153471,#153472,#153473,#153474,#153475,
#153476,#153477,#153478,#153479,#153480,#153481,#153482,#153483,#153484,
#153485,#153486,#153487,#153488,#153489,#153490,#153491,#153492,#153493,
#153494,#153495,#153496,#153497,#153498,#153499,#153500,#153501,#153502,
#153503,#153504,#153505,#153506,#153507,#153508,#153509,#153510,#153511,
#153512,#153513,#153514,#153515,#153516,#153517,#153518,#153519,#153520,
#153521,#153522,#153523,#153524,#153525,#153526,#153527,#153528,#153529,
#153530,#153531,#153532,#153533,#153534,#153535,#153536,#153537,#153538,
#153539,#153540,#153541,#153542,#153543,#153544,#153545,#153546,#153547,
#153548,#153549,#153550,#153551,#153552,#153553,#153554,#153555,#153556,
#153557,#153558,#153559,#153560,#153561,#153562,#153563,#153564,#153565,
#153566,#153567,#153568,#153569,#153570,#153571,#153572,#153573,#153574,
#153575,#153576,#153577,#153578,#153579,#153580,#153581,#153582,#153583,
#153584,#153585,#153586,#153587,#153588,#153589,#153590,#153591,#153592,
#153593,#153594,#153595,#153596,#153597,#153598,#153599,#153600,#153601,
#153602,#153603,#153604,#153605,#153606,#153607,#153608,#153609,#153610,
#153611,#153612,#153613,#153614,#153615,#153616,#153617,#153618,#153619,
#153620,#153621,#153622,#153623,#153624,#153625,#153626,#153627,#153628,
#153629,#153630,#153631,#153632,#153633,#153634,#153635,#153636,#153637,
#153638,#153639,#153640,#153641,#153642,#153643,#153644,#153645,#153646,
#153647,#153648,#153649,#153650,#153651,#153652,#153653,#153654,#153655,
#153656,#153657,#153658,#153659,#153660,#153661,#153662,#153663,#153664,
#153665,#153666,#153667,#153668,#153669,#153670,#153671,#153672,#153673,
#153674,#153675,#153676,#153677,#153678,#153679,#153680,#153681,#153682,
#153683,#153684,#153685,#153686,#153687,#153688,#153689,#153690,#153691,
#153692,#153693,#153694,#153695,#153696,#153697,#153698,#153699,#153700,
#153701,#153702,#153703,#153704,#153705,#153706,#153707,#153708,#153709,
#153710,#153711,#153712,#153713,#153714,#153715,#153716,#153717,#153718,
#153719,#153720,#153721,#153722,#153723,#153724,#153725,#153726,#153727,
#153728,#153729,#153730,#153731,#153732,#153733,#153734,#153735,#153736,
#153737,#153738,#153739,#153740,#153741,#153742,#153743,#153744,#153745,
#153746,#153747,#153748,#153749,#153750,#153751,#153752,#153753,#153754,
#153755,#153756,#153757,#153758,#153759,#153760,#153761,#153762,#153763,
#153764,#153765,#153766,#153767,#153768,#153769,#153770,#153771,#153772,
#153773,#153774,#153775,#153776,#153777,#153778,#153779,#153780,#153781,
#153782,#153783,#153784,#153785,#153786,#153787,#153788,#153789,#153790,
#153791,#153792,#153793,#153794,#153795,#153796,#153797,#153798,#153799,
#153800,#153801,#153802,#153803,#153804,#153805,#153806,#153807,#153808,
#153809,#153810,#153811,#153812,#153813,#153814,#153815,#153816,#153817,
#153818,#153819,#153820,#153821,#153822,#153823,#153824,#153825,#153826,
#153827,#153828,#153829,#153830,#153831,#153832,#153833,#153834,#153835,
#153836,#153837,#153838,#153839,#153840,#153841,#153842,#153843,#153844,
#153845,#153846,#153847,#153848,#153849,#153850,#153851,#153852,#153853,
#153854,#153855,#153856,#153857,#153858,#153859,#153860,#153861,#153862,
#153863,#153864,#153865,#153866,#153867,#153868,#153869,#153870,#153871,
#153872,#153873,#153874,#153875,#153876,#153877,#153878,#153879,#153880,
#153881,#153882,#153883,#153884,#153885,#153886,#153887),.UNSPECIFIED.,
 .F.,.F.)
B_SPLINE_CURVE_WITH_KNOTS((4,1,1,1,1,1,1,1,1,1,1,1,1,1,1,1,1,1,1,1,1,1,
1,1,1,1,1,1,1,1,1,1,1,1,1,1,1,1,1,1,1,1,1,1,1,1,1,1,1,1,1,1,1,1,1,1,1,1,
1,1,1,1,1,1,1,1,1,1,1,1,1,1,1,1,1,1,1,1,1,1,1,1,1,1,1,1,1,1,1,1,1,1,1,1,
1,1,1,1,1,1,1,1,1,1,1,1,1,1,1,1,1,1,1,1,1,1,1,1,1,1,1,1,1,1,1,1,1,1,1,1,
1,1,1,1,1,1,1,1,1,1,1,1,1,1,1,1,1,1,1,1,1,1,1,1,1,1,1,1,1,1,1,1,1,1,1,1,
1,1,1,1,1,1,1,1,1,1,1,1,1,1,1,1,1,1,1,1,1,1,1,1,1,1,1,1,1,1,1,1,1,1,1,1,
1,1,1,1,1,1,1,1,1,1,1,1,1,1,1,1,1,1,1,1,1,1,1,1,1,1,1,1,1,1,1,1,1,1,1,1,
1,1,1,1,1,1,1,1,1,1,1,1,1,1,1,1,1,1,1,1,1,1,1,1,1,1,1,1,1,1,1,1,1,1,1,1,
1,1,1,1,1,1,1,1,1,1,1,1,1,1,1,1,1,1,1,1,1,1,1,1,1,1,1,1,1,1,1,1,1,1,1,1,
1,1,1,1,1,1,1,1,1,1,1,1,1,1,1,1,1,1,1,1,1,1,1,1,1,1,1,1,1,1,1,1,1,1,1,1,
1,1,1,1,1,1,1,1,1,1,1,1,1,1,1,1,1,1,1,1,1,1,1,1,1,1,1,1,1,1,1,1,1,1,1,1,
1,1,1,1,1,1,1,1,1,1,1,1,1,1,1,1,1,1,1,1,1,1,1,1,1,1,1,1,1,1,1,1,1,1,1,1,
1,1,1,1,1,1,1,1,1,1,1,1,1,1,1,1,1,1,1,1,1,1,1,1,1,1,1,1,1,1,1,1,1,1,1,1,
1,1,1,1,1,1,1,1,1,1,1,1,1,1,1,1,1,1,1,1,1,1,1,1,1,1,1,1,1,1,1,1,1,1,1,1,
1,1,1,1,1,1,1,1,1,1,1,1,1,1,1,1,1,1,1,1,1,1,1,1,1,1,1,1,1,1,1,1,1,1,1,1,
1,1,1,1,1,1,1,1,1,1,1,1,1,1,1,1,1,1,1,1,1,1,1,1,1,1,1,1,1,1,1,1,1,1,1,1,
1,1,1,1,1,1,1,1,1,1,1,1,1,1,1,1,1,1,1,1,1,1,1,1,1,1,1,1,1,1,1,1,1,1,1,1,
1,1,1,1,1,1,1,1,1,1,1,1,1,1,1,1,1,1,1,1,1,1,1,1,1,1,1,1,1,1,1,1,1,1,1,1,
1,1,1,1,1,1,1,1,1,1,1,1,1,1,1,1,1,1,1,1,1,1,1,1,1,1,1,1,1,1,1,1,1,1,1,1,
1,1,1,1,1,1,1,1,1,1,1,1,1,1,1,1,1,1,1,1,1,1,1,1,1,1,1,1,1,1,1,1,1,1,1,1,
1,1,1,1,1,1,1,1,1,1,1,1,1,1,1,1,1,1,1,1,1,1,1,1,1,1,1,1,1,1,1,1,1,1,1,1,
1,1,1,1,1,1,1,1,1,1,1,1,1,1,1,1,1,1,1,1,1,1,1,1,1,1,1,1,1,1,1,1,1,1,1,1,
1,1,1,1,1,1,1,1,1,1,1,1,1,1,1,1,1,1,1,1,1,1,1,1,1,1,1,1,1,1,1,1,1,1,1,1,
1,1,1,1,1,1,1,1,1,1,1,1,1,1,1,1,1,1,1,1,1,1,1,1,1,1,1,1,1,1,1,1,1,1,1,1,
1,1,1,1,1,1,1,1,1,1,1,1,1,1,1,1,1,1,1,1,1,1,1,1,1,1,1,1,1,1,1,1,1,1,1,1,
1,1,1,1,1,1,1,1,1,1,1,1,1,1,1,1,1,1,1,1,1,1,1,1,1,1,1,1,1,1,1,1,1,1,1,1,
1,1,1,1,1,1,1,1,1,1,1,1,1,1,1,1,1,1,1,1,1,1,1,1,1,1,1,1,1,1,1,1,1,1,1,1,
1,1,1,1,1,1,1,1,1,1,1,1,1,1,1,1,1,1,1,1,1,1,1,1,1,1,1,1,1,1,1,1,1,1,1,1,
1,1,1,1,1,1,1,1,1,1,1,1,1,1,1,1,1,1,1,1,1,1,1,1,1,1,1,1,1,1,1,1,1,1,1,1,
1,1,1,1,1,1,1,1,1,1,1,1,1,1,1,1,1,1,1,1,1,1,1,1,1,4),(0.,0.01797683372391,
0.286633051710584,0.555289278308216,0.823945516665782,1.09260176953922,
1.36125803873948,1.62991432588463,1.89857063164012,2.16722695661301,2.43588330050525,
2.70453966304674,2.9731960431531,3.24185243981471,3.51050885133453,3.77916527610465,
4.04782171198515,4.31647815691489,4.58513460847725,4.85379106430677,5.12244752187208,
5.39110397865606,5.65976043217153,5.92841687990537,6.19707331956994,6.46572974881596,
6.73438616570634,7.00304256821933,7.2716989549161,7.5403553242696,7.809011675483,
8.07766800769526,8.34632432089157,8.61498061505147,8.8836368910788,9.15229314997201,
9.4209493936865,9.68960562442157,9.95826184531348,10.226918059948,10.4955742727586,
10.7642304884925,11.0328867113173,11.3015429448574,11.5701991918227,11.8388554546081,
12.1075117346518,12.3761680332469,12.6448243507434,12.9134806874637,13.1821370428496,
13.450793416388,13.7194498067883,13.9881062128412,14.2567626326955,14.5254190645885,
14.7940755062772,15.0627319555912,15.3313884100611,15.6000448672586,15.8687013246492,
16.1373577797,16.4060142299691,16.6746706729765,16.9433271065265,17.2119835283531,
17.4806399366567,17.7492963295502,18.0179527057767,18.286609063996,18.555265403637,
18.8239217240786,19.0925780255742,19.3612343083975,19.6298905737625,19.898546823017,
20.1672030584666,20.4358592827168,20.7045154992928,20.973171712245,21.2418279262962,
21.5104841459723,21.7791403749736,22.0477966165324,22.316452872948,22.585109146262,
22.8537654375589,23.1224217478187,23.3910780770929,23.6597344254327,23.9283907920352,
24.197047176159,24.4657035763222,24.7343599911301,25.0030164185931,25.2716728568073,
25.5403293034427,25.8089857562333,26.0776422126729,26.3462986702843,26.6149551265448,
26.8836115789212,27.1522680250308,27.4209244624423,27.6895808890659,27.9582373027346,
28.2268937018004,28.4955500845261,28.7642064498512,29.0328627966379,29.3015191245544,
29.5701754332357,29.838831723217,30.1074879950829,30.3761442503694,30.6448004907916,
30.9134567190168,31.1821129380756,31.450769151893,31.7194253649682,31.9880815819663,
32.2567378070174,32.5253940433706,32.7940502938785,33.0627065604467,33.3313628447765,
33.6000191476151,33.8686754696427,34.1373318106287,34.405988170366,34.6746445478242,
34.9433009420458,35.2119573513747,35.480613774244,35.7492702085419,36.0179266522368,
36.2865831029275,36.5552395582669,36.8238960157264,37.0925524727952,37.3612089269773,
37.6298653757534,37.8985218168153,38.1671782477952,38.4358346667239,38.7044910715485,
38.9731474607866,39.2418038328672,39.5104601869391,39.7791165220837,40.0477728382212,
40.3164291352602,40.5850854140292,40.8537416754418,41.1223979213679,41.3910541539077,
41.6597103761025,41.9283665914244,42.1970228042084,42.4656790192,42.7343352406829,
43.0029914723808,43.2716477171096,43.540303977354,43.8089602546436,44.0776165503516,
44.3462728649052,44.614929198697,44.883585551232,45.1522419220568,45.4208983099307,
45.6895547136931,45.9582111315299,46.2268675617156,46.4955240020317,46.7641804503338,
47.0328369041642,47.3014933611089,47.5701498186329,47.8388062742058,48.107462725373,
48.3761191696448,48.6447756048012,48.9134320285537,49.1820884390673,49.4507448344197,
49.7194012133072,49.9880575743413,50.2567139168934,50.5253702402807,50.7940265446884,
51.0626828303152,51.3313390982961,51.5999953498901,51.8686515873141,52.1373078130706,
52.4059640305862,52.6746202437936,52.9432764573682,53.211932675918,53.480588903259,
53.7492451427202,54.0179013967021,54.2865576673334,54.5552139557853,54.823870263115,
55.0925265894471,55.3611829348992,55.6298392987282,55.8984956802486,56.1671520780245,
56.4358084907065,56.7044649163381,56.9731213530494,57.2417777985307,57.5104342505384,
57.7790907065743,58.0477471641719,58.3164036208043,58.5850600739368,58.8537165211707,
59.1223729600609,59.39102938849,59.6596858042645,59.9283422056975,60.1969985910129,
60.4656549590995,60.7343113087676,61.0029676396243,61.2716239512389,61.540280244075,
61.808936518638,62.0775927763821,62.3462490189291,62.6149052488546,62.8835614690812,
63.1522176834332,63.4208738963055,63.6895301124163,63.9581863359981,64.2268425704115,
64.4954988186027,64.7641550825741,65.0328113641112,65.3014676640435,65.5701239831253,
65.8387803211949,66.1074366781083,66.3760930528907,66.6447494446373,66.9134058517341,
67.1820622726558,67.4507187053199,67.7193751477252,67.988031597487,68.256688052277,
68.5253445095709,68.7940009668648,69.0626574216546,69.3313138714164,69.5999703138218,
69.8686267464858,70.1372831674076,70.4059395745042,70.6745959662509,70.9432523410334,
71.2119086979469,71.4805650360164,71.7492213550982,72.0178776550306,72.2865339365675,
72.5551902005389,72.8238464487301,73.0925026831433,73.3611589067251,73.6298151228357,
73.8984713357081,74.1671275500599,74.4357837702864,74.7044400002118,74.9730962427587,
75.2417525005027,75.5104087750655,75.7790650679015,76.047721379516,76.3163777103726,
76.5850340600405,76.853690428127,77.1223468134422,77.391003214875,77.6596596306495,
77.9283160590784,78.1969724979684,78.4656289452021,78.7342853983344,79.0029418549666,
79.2715983125641,79.5402547685998,79.8089112206075,80.0775676660886,80.3462241027997,
80.6148805284312,80.8835369411131,81.1521933388889,81.4208497204091,81.689506084238,
81.9581624296899,82.2268187560219,82.4954750633515,82.7641313518033,83.0327876224345,
83.3014438764161,83.5701001158772,83.838756343218,84.1074125617677,84.3760687753422,
84.6447249885494,84.913381206065,85.1820374318212,85.4506936692451,85.719349920839,
85.9880061888197,86.2566624744465,86.5253187788541,86.7939751022413,87.0626314447932,
87.3312878058273,87.5999441847146,87.8686005800667,88.1372569905802,88.4059134143327,
88.6745698494889,88.9432262937606,89.2118827449277,89.4805392005005,89.7491956580243,
90.0178521149689,90.2865085687992,90.5551650171012,90.8238214574172,91.0924778876028,
91.3611343054394,91.6297907092016,91.8984470970753,92.1671034679,92.4357598204347,
92.7044161542264,92.9730724687798,93.2417287644878,93.5103850417773,93.7790413020216,
94.0476975467502,94.3163537784479,94.5850099999307,94.8536662149221,95.1223224277061,
95.390978643028,95.6596348652226,95.9282910977624,96.1969473436883,96.4656036051009,
96.7342598838697,97.0029161809086,97.2715724970461,97.5402288321905,97.8088851862623,
98.0775415583427,98.3461979475807,98.6148543524051,98.8835107713336,99.1521672023136,
99.4208236433754,99.6894800921513,99.9581365463333,100.226793003402,100.495449460861,
100.7641059162,101.032762366891,101.301418810586,101.570075244884,101.838731667753,
102.107388077082,102.376044471303,102.644700848761,102.913357208498,103.182013549484,
103.450669871511,103.71932617435,103.98798245868,104.256638725248,104.525294975755,
104.793951212108,105.062607437159,105.331263654157,105.599919867233,105.86857608105,
106.137232300108,106.405888528334,106.674544768756,106.943201024042,107.211857295908,
107.480513585889,107.74916989457,108.017826222487,108.286482569273,108.555138934598,
108.823795317324,109.09245171639,109.361108130058,109.629764556682,109.898420994093,
110.167077440202,110.435733892579,110.704390348839,110.97304680645,111.24170326289,
111.51035971568,111.779016162316,112.04767260053,112.316329027993,112.5849854428,
112.853641842963,113.122298227087,113.39095459369,113.659610942029,113.928267271303,
114.196923581563,114.46557987286,114.734236146174,115.002892402589,115.271548644148,
115.540204873149,115.808861092825,116.077517306876,116.346173519828,116.614829736404,
116.883485960654,117.152142196103,117.420798445358,117.689454710722,117.958110993546,
118.226767295041,118.495423615483,118.764079955123,119.032736313343,119.301392689569,
119.570049082462,119.838705490766,120.107361912592,120.376018346142,120.644674789149,
120.913331239418,121.181987694469,121.45064415186,121.719300609057,121.987957063527,
122.256613512841,122.525269954529,122.793926386422,123.062582806276,123.331239212329,
123.599895602729,123.868551976268,124.137208331653,124.405864668374,124.67452098587,
124.943177284465,125.211833564508,125.480489827294,125.749146074259,126.017802307799,
126.286458530624,126.555114746357,126.823770959168,127.092427173802,127.361083394694,
127.629739625429,127.898395869143,128.167052128037,128.435708404064,128.704364698224,
128.97302101142,129.241677343633,129.510333694846,129.7789900642,130.047646450897,
130.31630285341,130.5849592703,130.853615699547,131.122272139211,131.390928586945,
131.659585040461,131.928241497245,132.19689795481,132.46555441064,132.734210862202,
133.002867307132,133.271523743013,133.540180167783,133.808836579303,134.077492975965,
134.346149356071,134.614805718613,134.883462062505,135.152118387478,135.420774693234,
135.689430980379,135.958087249579,136.226743502453,136.49539974081,136.76405596741,
137.032712185392,137.301368398783,137.570024612174,137.838680830155,138.107337056755,
138.375993295112,138.644649547986,138.913305817186,139.181962104332,139.450618410087,
139.71927473506,139.987931078952,140.256587441494,140.525243821601,140.793900218262,
141.062556629782,141.331213054552,141.599869490433,141.868525935363,142.137182386925,
142.405838842755,142.67449530032,142.943151757104,143.21180821062,143.480464658354,
143.749121098019,144.017777527265,144.286433944155,144.555090346668,144.823746733365,
145.092403102719,145.361059453932,145.629715786145,145.898372099341,146.167028393501,
146.435684669529,146.704340928422,146.972997172137,147.241653402872,147.510309623764,
147.778965838398,148.047622051209,148.316278266943,148.584934489768,148.853590723308,
149.122246970274,149.390903233059,149.659559513103,149.928215811698,150.196872129195,
150.465528465915,150.734184821301,151.00284119484,151.27149758524,151.540153991293,
151.808810411148,152.077466843041,152.34612328473,152.614779734044,152.883436188514,
153.152092645711,153.420749103102,153.689405558153,153.958062008422,154.22671845143,
154.49537488498,154.764031306806,155.03268771511,155.301344108004,155.57000048423,
155.838656842449,156.107313182091,156.375969502532,156.644625804028,156.913282086851,
157.181938352216,157.450594601471,157.719250836921,157.987907061171,158.256563277747,
158.525219490699,158.793875704751,159.062531924427,159.331188153428,159.599844394987,
159.868500651403,160.137156924717,160.405813216014,160.674469526274,160.943125855548,
161.211782203888,161.480438570491,161.749094954615,162.017751354778,162.286407769586,
162.555064197049,162.823720635263,163.092377081899,163.361033534689,163.629689991129,
163.898346448741,164.167002905001,164.435659357378,164.704315803488,164.972972240899,
165.241628667523,165.510285081192,165.778941480257,166.047597862983,166.316254228308,
166.584910575095,166.853566903012,167.122223211693,167.390879501675,167.659535773541,
167.928192028827,168.19684826925,168.465504497475,168.734160716534,169.002816930351,
169.271473143427,169.540129360425,169.808785585476,170.077441821829,170.346098072337,
170.614754338905,170.883410623235,171.152066926074,171.420723248102,171.689379589088,
171.958035948825,172.226692326284,172.495348720505,172.764005129834,173.032661552704,
173.301317987002,173.569974430697,173.838630881388,174.107287336727,174.375943794187,
174.644600251255,174.913256705437,175.181913154214,175.450569595276,175.719226026256,
175.987882445184,176.256538850009,176.525195239247,176.793851611328,177.0625079654,
177.331164300545,177.599820616682,177.868476913721,178.137133192491,178.405789453903,
178.674445699829,178.943101932369,179.211758154564,179.480414369886,179.74907058267,
180.017726797662,180.286383019145,180.555039250843,180.823695495572,181.092351755816,
181.361008033106,181.629664328814,181.898320643368,182.16697697716,182.435633329695,
182.70428970052,182.972946088394,183.241602492156,183.510258909993,183.778915340179,
184.047571780495,184.316228228797,184.584884682628,184.853541139572,185.122197597096,
185.39085405267,185.659510503837,185.928166948109,186.196823383265,186.465479807018,
186.734136217531,187.002792612884,187.271448991771,187.540105352806,187.808761695358,
188.077418018745,188.346074323153,188.61473060878,188.883386876761,189.152043128355,
189.420699365779,189.689355591536,189.958011809051,190.226668022259,190.495324235834,
190.763980454383,191.032636681725,191.301292921186,191.569949175168,191.838605445799,
192.107261734251,192.375918041581,192.644574367913,192.913230713365,193.181887077194,
193.450543458715,193.719199856491,193.987856269173,194.256512694805,194.525169131516,
194.793825576997,195.062482029005,195.331138485041,195.599794942639,195.868451399271,
196.137107852404,196.405764299638,196.674420738528,196.943077166957,197.211733582732,
197.480389984165,197.749046369481,198.017702737567,198.286359087236,198.555015418092,
198.823671729707,199.092328022543,199.360984297106,199.62964055485,199.898296797397,
200.166953027323,200.43560924755,200.704265461902,200.972921674774,201.241577890885,
201.510234114467,201.77889034888,202.047546597072,202.316202861043,202.584859142581,
202.853515442513,203.122171761595,203.390828099665,203.659484456579,203.928140831361,
204.196797223108,204.465453630205,204.734110051127,205.002766483791,205.271422926197,
205.540079375959,205.808735830749,206.077392288043,206.346048745337,206.614705200127,
206.883361649889,207.152018092295,207.420674524959,207.689330945881,207.957987352978,
208.226643744725,208.495300119508,208.763956476421,209.032612814491,209.301269133573,
209.569925433505,209.838581715043,210.107237979014,210.375894227206,210.644550461619,
210.913206685201,211.181862901312,211.450519114184,211.719175328536,211.987831548763,
212.256487778689,212.525144021236,212.79380027898,213.062456553543,213.331112846379,
213.599769157994,213.868425488851,214.137081838519,214.405738206606,214.674394591921,
214.943050993354,215.211707409129,215.480363837558,215.749020276448,216.017676723682,
216.286333176815,216.554989633447,216.823646091045,217.092302547081,217.360958999089,
217.62961544457,217.898271881281,218.166928306913,218.435584719595,218.704241117371,
218.972897498892,219.241553862721,219.510210208173,219.778866534505,220.047522841835,
220.316179130287,220.584835400918,220.8534916549,221.122147894361,221.390804121702,
221.659460340252,221.928116553827,222.196772767034,222.46542898455,222.734085210306,
223.00274144773,223.271397699324,223.540053967305,223.808710252932,224.07736655734,
224.346022880728,224.61467922328,224.883335584314,225.151991963201,225.420648358554,
225.689304769068,225.95796119282,226.226617627977,226.495274072249,226.763930523416,
227.032586978989,227.301243436513,227.569899893458,227.838556347288,228.10721279559,
228.375869235907,228.644525666093,228.913182083929,229.181838487692,229.450494875566,
229.719151246391,229.987807598926,230.256463932718,230.525120247271,230.79377654298,
231.062432820269,231.331089080514,231.599745325243,231.868401556941,232.137057778424,
232.405713993415,232.674370206199,232.943026421521,233.211682643716,233.480338876256,
233.748995122182,234.017651383595,234.286307662364,234.554963959403,234.823620275541,
235.092276610685,235.360932964757,235.629589336838,235.898245726076,236.166902130901,
236.43555854983,236.70421498081,236.972871421872,237.241527870648,237.51018432483,
237.778840781899,238.047497239359,238.316153694698,238.584810145389,238.853466589084,
239.122123023382,239.390779446251,239.65943585558,239.928092249802,240.19674862726,
240.465404986998,240.734061327984,241.002717650011,241.27137395285,241.54003023718,
241.808686503748,242.077342754256,242.345998990609,242.614655215661,242.883311432659,
243.151967645734,243.420623859552,243.68928007861,243.957936306836,244.226592547258,
244.495248802545,244.763905074411,245.032561364392,245.301217673074,245.56987400099,
245.838530347777,246.107186713102,246.375843095828,246.644499494894,246.913155908563,
247.181812335186,247.450468772598,247.719125218708,247.987781671084,248.256438127345,
248.525094584956,248.793751041396,249.062407494187,249.331063940822,249.599720379036,
249.8683768065,250.137033221308,250.405689621471,250.674346005595,250.943002372197,
251.211658720537,251.480315049812,251.748971360071,252.017627651368,252.286283924683,
252.554940181098,252.823596422657,253.092252651658,253.360908871335,253.629565085386,
253.898221298338,254.166877514914,254.435533739165,254.704189974614,254.972846223869,
255.241502489234,255.510158772057,255.778815073553,256.047471393995,256.316127733635,
256.584784091854,256.85344046808,257.122096860973,257.390753269276,257.659409691102,
257.928066124652,258.196722567659,258.465379017928,258.734035472978,259.002691930368,
259.271348387566,259.540004842035,259.808661291349,260.077317733037,260.345974164929,
260.614630584783,260.883286990836,261.151943381235,261.420599754774,261.689256110159,
261.957912446879,262.226568764375,262.49522506297,262.763881343014,263.032537605798,
263.301193852763,263.569850086303,263.838506309127,264.107162524861,264.375818737671,
264.644474952305,264.913131173196,265.181787403931,265.450443647645,265.719099906538,
265.987756182565,266.256412476724,266.52506878992,266.793725122132,267.062381473345,
267.331037842698,267.599694229394,267.868350631907,268.137007048797,268.405663478042,
268.674319917706,268.94297636544,269.211632818955,269.480289275739,269.748945733304,
270.017602189133,270.286258640695,270.554915085624,270.823571521504,271.092227946274,
271.360884357793,271.629540754454,271.89819713456,272.166853497101,272.435509840993,
272.704166165965,272.97282247172,273.241478758865,273.510135028065,273.778791280938,
274.047447519295,274.316103745894,274.584759963875,274.853416177266,275.122072390656,
275.390728608637,275.659384835237,275.928041073593,276.196697326466,276.465353595666,
276.734009882811,277.002666188566,277.271322513539,277.53997885743,277.808635219972,
278.077291600077,278.345947996739,278.614604408258,278.883260833028,279.151917268908,
279.420573713837,279.689230165399,279.957886621228,280.226543078793,280.495199535576,
280.763855989092,281.032512436825,281.301168876489,281.569825305735,281.838481722625,
282.107138125138,282.375794511834,282.644450881187,282.9131072324,283.140531716307),
 .UNSPECIFIED.)
CURVE()
GEOMETRIC_REPRESENTATION_ITEM()
RATIONAL_B_SPLINE_CURVE((1.,1.,1.,1.,1.,1.,1.,1.,1.,1.,1.,1.,1.,1.,1.,1.,
1.,1.,1.,1.,1.,1.,1.,1.,1.,1.,1.,1.,1.,1.,1.,1.,1.,1.,1.,1.,1.,1.,1.,1.,
1.,1.,1.,1.,1.,1.,1.,1.,1.,1.,1.,1.,1.,1.,1.,1.,1.,1.,1.,1.,1.,1.,1.,1.,
1.,1.,1.,1.,1.,1.,1.,1.,1.,1.,1.,1.,1.,1.,1.,1.,1.,1.,1.,1.,1.,1.,1.,1.,
1.,1.,1.,1.,1.,1.,1.,1.,1.,1.,1.,1.,1.,1.,1.,1.,1.,1.,1.,1.,1.,1.,1.,1.,
1.,1.,1.,1.,1.,1.,1.,1.,1.,1.,1.,1.,1.,1.,1.,1.,1.,1.,1.,1.,1.,1.,1.,1.,
1.,1.,1.,1.,1.,1.,1.,1.,1.,1.,1.,1.,1.,1.,1.,1.,1.,1.,1.,1.,1.,1.,1.,1.,
1.,1.,1.,1.,1.,1.,1.,1.,1.,1.,1.,1.,1.,1.,1.,1.,1.,1.,1.,1.,1.,1.,1.,1.,
1.,1.,1.,1.,1.,1.,1.,1.,1.,1.,1.,1.,1.,1.,1.,1.,1.,1.,1.,1.,1.,1.,1.,1.,
1.,1.,1.,1.,1.,1.,1.,1.,1.,1.,1.,1.,1.,1.,1.,1.,1.,1.,1.,1.,1.,1.,1.,1.,
1.,1.,1.,1.,1.,1.,1.,1.,1.,1.,1.,1.,1.,1.,1.,1.,1.,1.,1.,1.,1.,1.,1.,1.,
1.,1.,1.,1.,1.,1.,1.,1.,1.,1.,1.,1.,1.,1.,1.,1.,1.,1.,1.,1.,1.,1.,1.,1.,
1.,1.,1.,1.,1.,1.,1.,1.,1.,1.,1.,1.,1.,1.,1.,1.,1.,1.,1.,1.,1.,1.,1.,1.,
1.,1.,1.,1.,1.,1.,1.,1.,1.,1.,1.,1.,1.,1.,1.,1.,1.,1.,1.,1.,1.,1.,1.,1.,
1.,1.,1.,1.,1.,1.,1.,1.,1.,1.,1.,1.,1.,1.,1.,1.,1.,1.,1.,1.,1.,1.,1.,1.,
1.,1.,1.,1.,1.,1.,1.,1.,1.,1.,1.,1.,1.,1.,1.,1.,1.,1.,1.,1.,1.,1.,1.,1.,
1.,1.,1.,1.,1.,1.,1.,1.,1.,1.,1.,1.,1.,1.,1.,1.,1.,1.,1.,1.,1.,1.,1.,1.,
1.,1.,1.,1.,1.,1.,1.,1.,1.,1.,1.,1.,1.,1.,1.,1.,1.,1.,1.,1.,1.,1.,1.,1.,
1.,1.,1.,1.,1.,1.,1.,1.,1.,1.,1.,1.,1.,1.,1.,1.,1.,1.,1.,1.,1.,1.,1.,1.,
1.,1.,1.,1.,1.,1.,1.,1.,1.,1.,1.,1.,1.,1.,1.,1.,1.,1.,1.,1.,1.,1.,1.,1.,
1.,1.,1.,1.,1.,1.,1.,1.,1.,1.,1.,1.,1.,1.,1.,1.,1.,1.,1.,1.,1.,1.,1.,1.,
1.,1.,1.,1.,1.,1.,1.,1.,1.,1.,1.,1.,1.,1.,1.,1.,1.,1.,1.,1.,1.,1.,1.,1.,
1.,1.,1.,1.,1.,1.,1.,1.,1.,1.,1.,1.,1.,1.,1.,1.,1.,1.,1.,1.,1.,1.,1.,1.,
1.,1.,1.,1.,1.,1.,1.,1.,1.,1.,1.,1.,1.,1.,1.,1.,1.,1.,1.,1.,1.,1.,1.,1.,
1.,1.,1.,1.,1.,1.,1.,1.,1.,1.,1.,1.,1.,1.,1.,1.,1.,1.,1.,1.,1.,1.,1.,1.,
1.,1.,1.,1.,1.,1.,1.,1.,1.,1.,1.,1.,1.,1.,1.,1.,1.,1.,1.,1.,1.,1.,1.,1.,
1.,1.,1.,1.,1.,1.,1.,1.,1.,1.,1.,1.,1.,1.,1.,1.,1.,1.,1.,1.,1.,1.,1.,1.,
1.,1.,1.,1.,1.,1.,1.,1.,1.,1.,1.,1.,1.,1.,1.,1.,1.,1.,1.,1.,1.,1.,1.,1.,
1.,1.,1.,1.,1.,1.,1.,1.,1.,1.,1.,1.,1.,1.,1.,1.,1.,1.,1.,1.,1.,1.,1.,1.,
1.,1.,1.,1.,1.,1.,1.,1.,1.,1.,1.,1.,1.,1.,1.,1.,1.,1.,1.,1.,1.,1.,1.,1.,
1.,1.,1.,1.,1.,1.,1.,1.,1.,1.,1.,1.,1.,1.,1.,1.,1.,1.,1.,1.,1.,1.,1.,1.,
1.,1.,1.,1.,1.,1.,1.,1.,1.,1.,1.,1.,1.,1.,1.,1.,1.,1.,1.,1.,1.,1.,1.,1.,
1.,1.,1.,1.,1.,1.,1.,1.,1.,1.,1.,1.,1.,1.,1.,1.,1.,1.,1.,1.,1.,1.,1.,1.,
1.,1.,1.,1.,1.,1.,1.,1.,1.,1.,1.,1.,1.,1.,1.,1.,1.,1.,1.,1.,1.,1.,1.,1.,
1.,1.,1.,1.,1.,1.,1.,1.,1.,1.,1.,1.,1.,1.,1.,1.,1.,1.,1.,1.,1.,1.,1.,1.,
1.,1.,1.,1.,1.,1.,1.,1.,1.,1.,1.,1.,1.,1.,1.,1.,1.,1.,1.,1.,1.,1.,1.,1.,
1.,1.,1.,1.,1.,1.,1.,1.,1.,1.,1.,1.,1.,1.,1.,1.,1.,1.,1.,1.,1.,1.,1.,1.,
1.,1.,1.,1.,1.,1.,1.,1.,1.,1.,1.,1.,1.,1.,1.,1.,1.,1.,1.,1.,1.,1.,1.,1.,
1.,1.,1.,1.,1.,1.,1.,1.,1.,1.,1.,1.,1.,1.,1.,1.,1.,1.,1.,1.,1.,1.,1.,1.,
1.,1.,1.,1.,1.,1.,1.,1.,1.,1.,1.,1.,1.,1.,1.,1.,1.,1.,1.,1.,1.,1.,1.,1.,
1.,1.,1.,1.,1.,1.,1.,1.,1.,1.,1.,1.,1.,1.,1.,1.,1.,1.,1.,1.,1.,1.,1.,1.,
1.,1.,1.,1.,1.,1.,1.,1.,1.,1.,1.,1.,1.,1.,1.,1.,1.,1.,1.,1.,1.,1.,1.,1.,
1.,1.,1.,1.,1.,1.,1.,1.,1.,1.,1.,1.,1.,1.,1.,1.,1.,1.,1.,1.,1.,1.,1.,1.,
1.,1.,1.,1.,1.,1.,1.,1.,1.,1.,1.,1.,1.,1.,1.,1.,1.,1.,1.,1.,1.,1.,1.,1.,
1.,1.,1.,1.,1.,1.,1.,1.,1.,1.))
REPRESENTATION_ITEM('')
) ;
#23=(
BOUNDED_CURVE()
B_SPLINE_CURVE(3,(#154112,#154113,#154114,#154115,#154116,#154117,#154118),
 .UNSPECIFIED.,.F.,.F.)
B_SPLINE_CURVE_WITH_KNOTS((4,1,1,1,4),(0.,0.0911446219616379,0.182289243923276,
0.273433865884915,0.364578487846551),.UNSPECIFIED.)
CURVE()
GEOMETRIC_REPRESENTATION_ITEM()
RATIONAL_B_SPLINE_CURVE((1.,1.,1.,1.,1.,1.,1.))
REPRESENTATION_ITEM('')
) ;
#24=(
BOUNDED_CURVE()
B_SPLINE_CURVE(3,(#154334,#154335,#154336,#154337,#154338,#154339,#154340,
#154341,#154342,#154343,#154344,#154345,#154346,#154347,#154348,#154349,
#154350,#154351,#154352),.UNSPECIFIED.,.F.,.F.)
B_SPLINE_CURVE_WITH_KNOTS((4,1,1,1,1,1,1,1,1,1,1,1,1,1,1,1,4),(0.,0.226732296973331,
0.464902013928651,0.70307173088397,0.9298040278573,1.15653632483063,1.39470604178595,
1.63287575874127,1.8596080557146,2.08634035268793,2.32451006964325,2.56267978659857,
2.7894120835719,3.01614438054523,3.25431409750055,3.49248381445586,3.7192161114292),
 .UNSPECIFIED.)
CURVE()
GEOMETRIC_REPRESENTATION_ITEM()
RATIONAL_B_SPLINE_CURVE((1.,1.,1.,1.,1.,1.,1.,1.,1.,1.,1.,1.,1.,1.,1.,1.,
1.,1.,1.))
REPRESENTATION_ITEM('')
) ;
#43=(
BOUNDED_SURFACE()
B_SPLINE_SURFACE(2,3,((#114380,#114381,#114382,#114383,#114384,#114385,
#114386,#114387,#114388,#114389,#114390,#114391,#114392,#114393,#114394,
#114395,#114396,#114397,#114398,#114399,#114400,#114401,#114402,#114403,
#114404,#114405,#114406,#114407,#114408,#114409,#114410,#114411,#114412,
#114413,#114414,#114415,#114416,#114417,#114418,#114419,#114420,#114421,
#114422,#114423,#114424,#114425,#114426,#114427,#114428,#114429,#114430,
#114431,#114432,#114433,#114434,#114435,#114436,#114437,#114438,#114439,
#114440,#114441,#114442,#114443,#114444,#114445,#114446,#114447,#114448,
#114449,#114450,#114451,#114452,#114453,#114454,#114455,#114456,#114457,
#114458,#114459,#114460,#114461,#114462,#114463,#114464,#114465,#114466,
#114467,#114468,#114469,#114470,#114471,#114472,#114473,#114474,#114475,
#114476,#114477,#114478,#114479,#114480,#114481,#114482,#114483,#114484,
#114485,#114486,#114487,#114488,#114489,#114490,#114491,#114492,#114493,
#114494,#114495,#114496,#114497,#114498,#114499,#114500,#114501,#114502,
#114503,#114504,#114505,#114506,#114507,#114508,#114509,#114510,#114511,
#114512,#114513,#114514,#114515,#114516,#114517,#114518,#114519,#114520,
#114521,#114522,#114523,#114524,#114525,#114526,#114527,#114528,#114529,
#114530,#114531,#114532,#114533,#114534,#114535,#114536,#114537,#114538,
#114539,#114540,#114541,#114542,#114543,#114544,#114545,#114546,#114547,
#114548,#114549,#114550,#114551,#114552,#114553,#114554,#114555,#114556,
#114557,#114558,#114559,#114560,#114561,#114562,#114563,#114564,#114565,
#114566,#114567,#114568,#114569,#114570,#114571,#114572,#114573,#114574,
#114575,#114576,#114577,#114578,#114579,#114580,#114581,#114582,#114583,
#114584,#114585,#114586,#114587,#114588,#114589,#114590,#114591,#114592,
#114593,#114594,#114595,#114596,#114597,#114598,#114599,#114600,#114601,
#114602,#114603,#114604,#114605,#114606,#114607,#114608,#114609,#114610,
#114611,#114612,#114613,#114614,#114615,#114616,#114617,#114618,#114619,
#114620,#114621,#114622,#114623,#114624,#114625,#114626,#114627,#114628,
#114629,#114630,#114631,#114632,#114633,#114634,#114635,#114636,#114637,
#114638,#114639,#114640,#114641,#114642,#114643,#114644,#114645,#114646,
#114647,#114648,#114649,#114650,#114651,#114652,#114653,#114654,#114655,
#114656,#114657,#114658,#114659,#114660,#114661,#114662,#114663,#114664,
#114665,#114666,#114667,#114668,#114669,#114670,#114671,#114672,#114673,
#114674,#114675,#114676,#114677,#114678,#114679,#114680,#114681,#114682,
#114683,#114684,#114685,#114686,#114687,#114688,#114689,#114690,#114691,
#114692,#114693,#114694,#114695,#114696,#114697,#114698,#114699,#114700,
#114701,#114702,#114703,#114704,#114705,#114706,#114707,#114708,#114709,
#114710,#114711,#114712,#114713,#114714,#114715,#114716,#114717,#114718,
#114719,#114720,#114721,#114722,#114723,#114724,#114725,#114726,#114727,
#114728,#114729,#114730,#114731,#114732,#114733,#114734,#114735,#114736,
#114737,#114738,#114739,#114740,#114741,#114742,#114743,#114744,#114745,
#114746,#114747,#114748,#114749,#114750,#114751,#114752,#114753,#114754,
#114755,#114756,#114757,#114758,#114759,#114760,#114761,#114762,#114763,
#114764,#114765,#114766,#114767,#114768,#114769,#114770,#114771,#114772,
#114773,#114774,#114775,#114776,#114777,#114778,#114779,#114780,#114781,
#114782,#114783,#114784,#114785,#114786,#114787,#114788,#114789,#114790,
#114791,#114792,#114793,#114794,#114795,#114796,#114797,#114798,#114799,
#114800,#114801,#114802,#114803,#114804,#114805,#114806,#114807,#114808,
#114809,#114810,#114811,#114812,#114813,#114814,#114815,#114816,#114817,
#114818,#114819,#114820,#114821,#114822,#114823,#114824,#114825,#114826,
#114827,#114828,#114829,#114830,#114831,#114832,#114833,#114834,#114835,
#114836,#114837,#114838,#114839,#114840,#114841,#114842,#114843,#114844,
#114845,#114846,#114847,#114848,#114849,#114850,#114851,#114852,#114853,
#114854,#114855,#114856,#114857,#114858,#114859,#114860,#114861,#114862,
#114863,#114864,#114865,#114866,#114867,#114868,#114869,#114870,#114871,
#114872,#114873,#114874,#114875,#114876,#114877,#114878,#114879,#114880,
#114881,#114882,#114883,#114884,#114885,#114886,#114887,#114888,#114889,
#114890,#114891,#114892,#114893,#114894,#114895,#114896,#114897,#114898,
#114899,#114900,#114901,#114902,#114903,#114904,#114905,#114906,#114907,
#114908,#114909,#114910,#114911,#114912,#114913,#114914,#114915,#114916,
#114917,#114918,#114919,#114920,#114921,#114922,#114923,#114924,#114925,
#114926,#114927,#114928,#114929,#114930,#114931,#114932,#114933,#114934,
#114935,#114936,#114937,#114938,#114939,#114940,#114941,#114942,#114943,
#114944,#114945,#114946,#114947,#114948,#114949,#114950,#114951,#114952,
#114953,#114954,#114955,#114956,#114957,#114958,#114959,#114960,#114961,
#114962,#114963,#114964,#114965,#114966,#114967,#114968,#114969,#114970,
#114971,#114972,#114973,#114974,#114975,#114976,#114977,#114978,#114979,
#114980,#114981,#114982,#114983,#114984,#114985,#114986,#114987,#114988,
#114989,#114990,#114991,#114992,#114993,#114994,#114995,#114996,#114997,
#114998,#114999,#115000,#115001,#115002,#115003,#115004,#115005,#115006,
#115007,#115008,#115009,#115010,#115011,#115012,#115013,#115014,#115015,
#115016,#115017,#115018,#115019,#115020,#115021,#115022,#115023,#115024,
#115025,#115026,#115027,#115028,#115029,#115030,#115031,#115032,#115033,
#115034,#115035,#115036,#115037,#115038,#115039,#115040,#115041,#115042,
#115043,#115044,#115045,#115046,#115047,#115048,#115049,#115050,#115051,
#115052,#115053,#115054,#115055,#115056,#115057,#115058,#115059,#115060,
#115061,#115062,#115063,#115064,#115065,#115066,#115067,#115068,#115069,
#115070,#115071,#115072,#115073,#115074,#115075,#115076,#115077,#115078,
#115079,#115080,#115081,#115082,#115083,#115084,#115085,#115086,#115087,
#115088,#115089,#115090,#115091,#115092,#115093,#115094,#115095,#115096,
#115097,#115098,#115099,#115100,#115101,#115102,#115103,#115104,#115105,
#115106,#115107,#115108,#115109,#115110,#115111,#115112,#115113,#115114,
#115115,#115116,#115117,#115118,#115119,#115120,#115121,#115122,#115123,
#115124,#115125,#115126,#115127,#115128,#115129,#115130,#115131,#115132,
#115133,#115134,#115135,#115136,#115137,#115138,#115139,#115140,#115141,
#115142,#115143,#115144,#115145,#115146,#115147,#115148,#115149,#115150,
#115151,#115152,#115153,#115154,#115155,#115156,#115157,#115158,#115159,
#115160,#115161,#115162,#115163,#115164,#115165,#115166,#115167,#115168,
#115169,#115170,#115171,#115172,#115173,#115174,#115175,#115176,#115177,
#115178,#115179,#115180,#115181,#115182,#115183,#115184,#115185,#115186,
#115187,#115188,#115189,#115190,#115191,#115192,#115193,#115194,#115195,
#115196,#115197,#115198,#115199,#115200,#115201,#115202,#115203,#115204,
#115205,#115206,#115207,#115208,#115209,#115210,#115211,#115212,#115213,
#115214,#115215,#115216,#115217,#115218,#115219,#115220,#115221,#115222,
#115223,#115224,#115225,#115226,#115227,#115228,#115229,#115230,#115231,
#115232,#115233,#115234,#115235,#115236,#115237,#115238,#115239,#115240,
#115241,#115242,#115243,#115244,#115245,#115246,#115247,#115248,#115249,
#115250,#115251,#115252,#115253,#115254,#115255,#115256,#115257,#115258,
#115259,#115260,#115261,#115262,#115263,#115264,#115265,#115266,#115267,
#115268,#115269,#115270,#115271,#115272,#115273,#115274,#115275,#115276,
#115277,#115278,#115279,#115280,#115281,#115282,#115283,#115284,#115285,
#115286,#115287,#115288,#115289,#115290,#115291,#115292,#115293,#115294,
#115295,#115296,#115297,#115298,#115299,#115300,#115301,#115302,#115303,
#115304,#115305,#115306,#115307,#115308,#115309,#115310,#115311,#115312,
#115313,#115314,#115315,#115316,#115317,#115318,#115319,#115320,#115321,
#115322,#115323,#115324,#115325,#115326,#115327,#115328,#115329,#115330,
#115331,#115332,#115333,#115334,#115335,#115336,#115337,#115338,#115339,
#115340,#115341,#115342,#115343,#115344,#115345,#115346,#115347,#115348,
#115349,#115350,#115351,#115352,#115353,#115354,#115355,#115356,#115357,
#115358,#115359,#115360,#115361,#115362,#115363,#115364,#115365,#115366,
#115367,#115368,#115369,#115370,#115371,#115372,#115373,#115374,#115375,
#115376,#115377,#115378,#115379,#115380,#115381,#115382,#115383,#115384,
#115385,#115386,#115387,#115388,#115389,#115390,#115391,#115392,#115393,
#115394,#115395,#115396,#115397,#115398,#115399,#115400,#115401,#115402,
#115403,#115404,#115405,#115406,#115407,#115408,#115409,#115410,#115411,
#115412,#115413,#115414,#115415,#115416,#115417,#115418,#115419,#115420,
#115421,#115422,#115423,#115424,#115425,#115426,#115427,#115428,#115429,
#115430,#115431,#115432,#115433,#115434,#115435,#115436,#115437,#115438,
#115439,#115440,#115441,#115442,#115443,#115444,#115445,#115446,#115447,
#115448,#115449,#115450,#115451,#115452,#115453,#115454,#115455,#115456,
#115457,#115458,#115459,#115460,#115461,#115462,#115463,#115464,#115465,
#115466,#115467,#115468,#115469,#115470,#115471,#115472,#115473,#115474,
#115475,#115476,#115477,#115478,#115479,#115480,#115481,#115482,#115483,
#115484,#115485,#115486,#115487,#115488,#115489,#115490,#115491,#115492,
#115493,#115494,#115495,#115496,#115497,#115498,#115499,#115500,#115501,
#115502,#115503,#115504,#115505,#115506,#115507,#115508,#115509,#115510,
#115511,#115512,#115513,#115514,#115515,#115516,#115517,#115518,#115519,
#115520,#115521,#115522,#115523,#115524,#115525,#115526,#115527,#115528,
#115529,#115530,#115531,#115532,#115533,#115534,#115535,#115536,#115537,
#115538,#115539,#115540,#115541,#115542,#115543,#115544,#115545,#115546,
#115547,#115548,#115549,#115550,#115551,#115552,#115553,#115554,#115555,
#115556,#115557,#115558,#115559,#115560,#115561,#115562,#115563,#115564,
#115565,#115566,#115567,#115568,#115569,#115570,#115571,#115572,#115573,
#115574,#115575,#115576,#115577,#115578,#115579,#115580,#115581,#115582,
#115583,#115584,#115585,#115586,#115587,#115588,#115589,#115590,#115591,
#115592,#115593,#115594,#115595,#115596,#115597,#115598,#115599,#115600,
#115601,#115602,#115603,#115604,#115605,#115606,#115607,#115608,#115609,
#115610,#115611,#115612,#115613,#115614,#115615,#115616,#115617,#115618,
#115619,#115620,#115621,#115622,#115623,#115624,#115625,#115626,#115627,
#115628,#115629,#115630,#115631,#115632,#115633,#115634,#115635,#115636,
#115637,#115638,#115639,#115640,#115641,#115642,#115643,#115644,#115645,
#115646,#115647,#115648,#115649,#115650,#115651,#115652,#115653,#115654,
#115655,#115656,#115657,#115658,#115659,#115660,#115661,#115662,#115663,
#115664,#115665,#115666,#115667,#115668,#115669,#115670,#115671,#115672,
#115673,#115674,#115675,#115676,#115677,#115678,#115679,#115680,#115681,
#115682,#115683,#115684,#115685,#115686,#115687,#115688,#115689,#115690,
#115691,#115692,#115693,#115694,#115695,#115696,#115697,#115698,#115699,
#115700,#115701,#115702,#115703,#115704,#115705,#115706,#115707,#115708,
#115709,#115710,#115711,#115712,#115713,#115714,#115715,#115716,#115717,
#115718,#115719,#115720,#115721,#115722,#115723,#115724,#115725,#115726,
#115727,#115728,#115729,#115730,#115731,#115732,#115733,#115734,#115735,
#115736,#115737,#115738,#115739,#115740,#115741,#115742,#115743,#115744,
#115745,#115746,#115747,#115748,#115749,#115750,#115751,#115752,#115753,
#115754,#115755,#115756,#115757,#115758,#115759,#115760,#115761,#115762,
#115763,#115764,#115765,#115766,#115767,#115768,#115769,#115770,#115771,
#115772,#115773,#115774,#115775,#115776,#115777,#115778,#115779,#115780,
#115781,#115782,#115783,#115784,#115785,#115786,#115787,#115788,#115789,
#115790,#115791,#115792,#115793,#115794,#115795,#115796,#115797,#115798,
#115799,#115800,#115801,#115802,#115803,#115804,#115805,#115806,#115807,
#115808,#115809,#115810,#115811,#115812,#115813,#115814,#115815,#115816,
#115817,#115818,#115819,#115820,#115821,#115822,#115823,#115824,#115825,
#115826,#115827,#115828,#115829,#115830,#115831,#115832,#115833,#115834,
#115835,#115836,#115837,#115838,#115839,#115840,#115841,#115842,#115843,
#115844,#115845,#115846,#115847,#115848,#115849,#115850,#115851,#115852,
#115853,#115854,#115855,#115856,#115857,#115858,#115859,#115860,#115861,
#115862,#115863,#115864,#115865,#115866,#115867,#115868,#115869,#115870,
#115871,#115872,#115873,#115874,#115875,#115876,#115877,#115878,#115879,
#115880,#115881,#115882,#115883,#115884,#115885,#115886,#115887,#115888,
#115889,#115890,#115891,#115892,#115893,#115894,#115895,#115896,#115897,
#115898,#115899,#115900,#115901,#115902,#115903,#115904,#115905,#115906,
#115907,#115908,#115909,#115910,#115911,#115912,#115913,#115914,#115915,
#115916,#115917,#115918,#115919,#115920,#115921,#115922,#115923,#115924,
#115925,#115926,#115927,#115928,#115929,#115930,#115931,#115932,#115933,
#115934,#115935,#115936,#115937,#115938,#115939,#115940,#115941,#115942,
#115943,#115944,#115945,#115946,#115947,#115948,#115949,#115950,#115951,
#115952,#115953,#115954,#115955,#115956,#115957,#115958,#115959,#115960,
#115961,#115962,#115963,#115964,#115965,#115966,#115967,#115968,#115969,
#115970,#115971,#115972,#115973,#115974,#115975,#115976,#115977,#115978,
#115979,#115980,#115981,#115982,#115983,#115984,#115985,#115986,#115987,
#115988,#115989,#115990,#115991,#115992,#115993,#115994,#115995,#115996,
#115997,#115998,#115999,#116000,#116001,#116002,#116003,#116004,#116005,
#116006,#116007,#116008,#116009,#116010,#116011,#116012,#116013,#116014,
#116015,#116016,#116017,#116018,#116019,#116020,#116021,#116022,#116023,
#116024,#116025,#116026,#116027,#116028,#116029,#116030,#116031,#116032,
#116033,#116034,#116035,#116036,#116037,#116038,#116039,#116040,#116041,
#116042,#116043,#116044,#116045,#116046,#116047,#116048,#116049,#116050,
#116051,#116052,#116053,#116054,#116055,#116056,#116057,#116058,#116059,
#116060,#116061,#116062,#116063,#116064,#116065,#116066,#116067,#116068,
#116069,#116070,#116071,#116072,#116073,#116074,#116075,#116076,#116077,
#116078,#116079,#116080,#116081,#116082,#116083,#116084,#116085,#116086,
#116087,#116088,#116089,#116090,#116091,#116092,#116093,#116094,#116095,
#116096,#116097,#116098,#116099,#116100,#116101,#116102,#116103,#116104,
#116105,#116106,#116107,#116108,#116109,#116110,#116111,#116112,#116113,
#116114,#116115,#116116,#116117,#116118,#116119,#116120,#116121,#116122,
#116123,#116124,#116125,#116126,#116127,#116128,#116129,#116130,#116131,
#116132,#116133,#116134,#116135,#116136,#116137,#116138,#116139,#116140,
#116141,#116142,#116143,#116144,#116145,#116146,#116147,#116148,#116149,
#116150,#116151,#116152,#116153,#116154,#116155,#116156,#116157,#116158,
#116159,#116160,#116161,#116162,#116163,#116164,#116165,#116166,#116167,
#116168,#116169,#116170,#116171,#116172,#116173,#116174,#116175,#116176,
#116177,#116178,#116179,#116180,#116181,#116182,#116183,#116184,#116185,
#116186,#116187,#116188,#116189,#116190,#116191,#116192,#116193,#116194,
#116195,#116196,#116197,#116198,#116199,#116200,#116201,#116202,#116203,
#116204,#116205,#116206,#116207,#116208,#116209,#116210,#116211,#116212,
#116213,#116214,#116215,#116216,#116217,#116218,#116219,#116220,#116221,
#116222,#116223,#116224,#116225,#116226,#116227,#116228,#116229,#116230,
#116231,#116232,#116233,#116234,#116235,#116236,#116237,#116238,#116239,
#116240,#116241,#116242,#116243,#116244,#116245,#116246,#116247,#116248,
#116249,#116250,#116251,#116252,#116253,#116254,#116255,#116256,#116257,
#116258,#116259,#116260,#116261,#116262,#116263,#116264,#116265,#116266,
#116267,#116268,#116269,#116270,#116271,#116272,#116273,#116274,#116275,
#116276,#116277,#116278,#116279,#116280,#116281,#116282,#116283,#116284,
#116285,#116286,#116287,#116288,#116289,#116290,#116291,#116292,#116293,
#116294,#116295,#116296,#116297,#116298,#116299,#116300,#116301,#116302,
#116303,#116304,#116305,#116306,#116307,#116308,#116309,#116310,#116311,
#116312,#116313,#116314,#116315,#116316,#116317,#116318,#116319,#116320,
#116321,#116322,#116323,#116324,#116325,#116326,#116327,#116328,#116329,
#116330,#116331,#116332,#116333,#116334,#116335,#116336,#116337,#116338,
#116339,#116340,#116341,#116342,#116343,#116344,#116345,#116346,#116347,
#116348,#116349,#116350,#116351,#116352,#116353,#116354,#116355,#116356,
#116357,#116358,#116359,#116360,#116361,#116362,#116363,#116364,#116365,
#116366,#116367,#116368,#116369,#116370,#116371,#116372,#116373,#116374,
#116375,#116376,#116377,#116378,#116379,#116380,#116381,#116382,#116383,
#116384,#116385,#116386,#116387,#116388,#116389,#116390,#116391,#116392,
#116393,#116394,#116395,#116396,#116397,#116398,#116399,#116400,#116401,
#116402,#116403,#116404,#116405,#116406,#116407,#116408,#116409,#116410,
#116411,#116412,#116413,#116414,#116415,#116416,#116417,#116418,#116419,
#116420,#116421,#116422,#116423,#116424,#116425,#116426,#116427,#116428,
#116429,#116430),(#116431,#116432,#116433,#116434,#116435,#116436,#116437,
#116438,#116439,#116440,#116441,#116442,#116443,#116444,#116445,#116446,
#116447,#116448,#116449,#116450,#116451,#116452,#116453,#116454,#116455,
#116456,#116457,#116458,#116459,#116460,#116461,#116462,#116463,#116464,
#116465,#116466,#116467,#116468,#116469,#116470,#116471,#116472,#116473,
#116474,#116475,#116476,#116477,#116478,#116479,#116480,#116481,#116482,
#116483,#116484,#116485,#116486,#116487,#116488,#116489,#116490,#116491,
#116492,#116493,#116494,#116495,#116496,#116497,#116498,#116499,#116500,
#116501,#116502,#116503,#116504,#116505,#116506,#116507,#116508,#116509,
#116510,#116511,#116512,#116513,#116514,#116515,#116516,#116517,#116518,
#116519,#116520,#116521,#116522,#116523,#116524,#116525,#116526,#116527,
#116528,#116529,#116530,#116531,#116532,#116533,#116534,#116535,#116536,
#116537,#116538,#116539,#116540,#116541,#116542,#116543,#116544,#116545,
#116546,#116547,#116548,#116549,#116550,#116551,#116552,#116553,#116554,
#116555,#116556,#116557,#116558,#116559,#116560,#116561,#116562,#116563,
#116564,#116565,#116566,#116567,#116568,#116569,#116570,#116571,#116572,
#116573,#116574,#116575,#116576,#116577,#116578,#116579,#116580,#116581,
#116582,#116583,#116584,#116585,#116586,#116587,#116588,#116589,#116590,
#116591,#116592,#116593,#116594,#116595,#116596,#116597,#116598,#116599,
#116600,#116601,#116602,#116603,#116604,#116605,#116606,#116607,#116608,
#116609,#116610,#116611,#116612,#116613,#116614,#116615,#116616,#116617,
#116618,#116619,#116620,#116621,#116622,#116623,#116624,#116625,#116626,
#116627,#116628,#116629,#116630,#116631,#116632,#116633,#116634,#116635,
#116636,#116637,#116638,#116639,#116640,#116641,#116642,#116643,#116644,
#116645,#116646,#116647,#116648,#116649,#116650,#116651,#116652,#116653,
#116654,#116655,#116656,#116657,#116658,#116659,#116660,#116661,#116662,
#116663,#116664,#116665,#116666,#116667,#116668,#116669,#116670,#116671,
#116672,#116673,#116674,#116675,#116676,#116677,#116678,#116679,#116680,
#116681,#116682,#116683,#116684,#116685,#116686,#116687,#116688,#116689,
#116690,#116691,#116692,#116693,#116694,#116695,#116696,#116697,#116698,
#116699,#116700,#116701,#116702,#116703,#116704,#116705,#116706,#116707,
#116708,#116709,#116710,#116711,#116712,#116713,#116714,#116715,#116716,
#116717,#116718,#116719,#116720,#116721,#116722,#116723,#116724,#116725,
#116726,#116727,#116728,#116729,#116730,#116731,#116732,#116733,#116734,
#116735,#116736,#116737,#116738,#116739,#116740,#116741,#116742,#116743,
#116744,#116745,#116746,#116747,#116748,#116749,#116750,#116751,#116752,
#116753,#116754,#116755,#116756,#116757,#116758,#116759,#116760,#116761,
#116762,#116763,#116764,#116765,#116766,#116767,#116768,#116769,#116770,
#116771,#116772,#116773,#116774,#116775,#116776,#116777,#116778,#116779,
#116780,#116781,#116782,#116783,#116784,#116785,#116786,#116787,#116788,
#116789,#116790,#116791,#116792,#116793,#116794,#116795,#116796,#116797,
#116798,#116799,#116800,#116801,#116802,#116803,#116804,#116805,#116806,
#116807,#116808,#116809,#116810,#116811,#116812,#116813,#116814,#116815,
#116816,#116817,#116818,#116819,#116820,#116821,#116822,#116823,#116824,
#116825,#116826,#116827,#116828,#116829,#116830,#116831,#116832,#116833,
#116834,#116835,#116836,#116837,#116838,#116839,#116840,#116841,#116842,
#116843,#116844,#116845,#116846,#116847,#116848,#116849,#116850,#116851,
#116852,#116853,#116854,#116855,#116856,#116857,#116858,#116859,#116860,
#116861,#116862,#116863,#116864,#116865,#116866,#116867,#116868,#116869,
#116870,#116871,#116872,#116873,#116874,#116875,#116876,#116877,#116878,
#116879,#116880,#116881,#116882,#116883,#116884,#116885,#116886,#116887,
#116888,#116889,#116890,#116891,#116892,#116893,#116894,#116895,#116896,
#116897,#116898,#116899,#116900,#116901,#116902,#116903,#116904,#116905,
#116906,#116907,#116908,#116909,#116910,#116911,#116912,#116913,#116914,
#116915,#116916,#116917,#116918,#116919,#116920,#116921,#116922,#116923,
#116924,#116925,#116926,#116927,#116928,#116929,#116930,#116931,#116932,
#116933,#116934,#116935,#116936,#116937,#116938,#116939,#116940,#116941,
#116942,#116943,#116944,#116945,#116946,#116947,#116948,#116949,#116950,
#116951,#116952,#116953,#116954,#116955,#116956,#116957,#116958,#116959,
#116960,#116961,#116962,#116963,#116964,#116965,#116966,#116967,#116968,
#116969,#116970,#116971,#116972,#116973,#116974,#116975,#116976,#116977,
#116978,#116979,#116980,#116981,#116982,#116983,#116984,#116985,#116986,
#116987,#116988,#116989,#116990,#116991,#116992,#116993,#116994,#116995,
#116996,#116997,#116998,#116999,#117000,#117001,#117002,#117003,#117004,
#117005,#117006,#117007,#117008,#117009,#117010,#117011,#117012,#117013,
#117014,#117015,#117016,#117017,#117018,#117019,#117020,#117021,#117022,
#117023,#117024,#117025,#117026,#117027,#117028,#117029,#117030,#117031,
#117032,#117033,#117034,#117035,#117036,#117037,#117038,#117039,#117040,
#117041,#117042,#117043,#117044,#117045,#117046,#117047,#117048,#117049,
#117050,#117051,#117052,#117053,#117054,#117055,#117056,#117057,#117058,
#117059,#117060,#117061,#117062,#117063,#117064,#117065,#117066,#117067,
#117068,#117069,#117070,#117071,#117072,#117073,#117074,#117075,#117076,
#117077,#117078,#117079,#117080,#117081,#117082,#117083,#117084,#117085,
#117086,#117087,#117088,#117089,#117090,#117091,#117092,#117093,#117094,
#117095,#117096,#117097,#117098,#117099,#117100,#117101,#117102,#117103,
#117104,#117105,#117106,#117107,#117108,#117109,#117110,#117111,#117112,
#117113,#117114,#117115,#117116,#117117,#117118,#117119,#117120,#117121,
#117122,#117123,#117124,#117125,#117126,#117127,#117128,#117129,#117130,
#117131,#117132,#117133,#117134,#117135,#117136,#117137,#117138,#117139,
#117140,#117141,#117142,#117143,#117144,#117145,#117146,#117147,#117148,
#117149,#117150,#117151,#117152,#117153,#117154,#117155,#117156,#117157,
#117158,#117159,#117160,#117161,#117162,#117163,#117164,#117165,#117166,
#117167,#117168,#117169,#117170,#117171,#117172,#117173,#117174,#117175,
#117176,#117177,#117178,#117179,#117180,#117181,#117182,#117183,#117184,
#117185,#117186,#117187,#117188,#117189,#117190,#117191,#117192,#117193,
#117194,#117195,#117196,#117197,#117198,#117199,#117200,#117201,#117202,
#117203,#117204,#117205,#117206,#117207,#117208,#117209,#117210,#117211,
#117212,#117213,#117214,#117215,#117216,#117217,#117218,#117219,#117220,
#117221,#117222,#117223,#117224,#117225,#117226,#117227,#117228,#117229,
#117230,#117231,#117232,#117233,#117234,#117235,#117236,#117237,#117238,
#117239,#117240,#117241,#117242,#117243,#117244,#117245,#117246,#117247,
#117248,#117249,#117250,#117251,#117252,#117253,#117254,#117255,#117256,
#117257,#117258,#117259,#117260,#117261,#117262,#117263,#117264,#117265,
#117266,#117267,#117268,#117269,#117270,#117271,#117272,#117273,#117274,
#117275,#117276,#117277,#117278,#117279,#117280,#117281,#117282,#117283,
#117284,#117285,#117286,#117287,#117288,#117289,#117290,#117291,#117292,
#117293,#117294,#117295,#117296,#117297,#117298,#117299,#117300,#117301,
#117302,#117303,#117304,#117305,#117306,#117307,#117308,#117309,#117310,
#117311,#117312,#117313,#117314,#117315,#117316,#117317,#117318,#117319,
#117320,#117321,#117322,#117323,#117324,#117325,#117326,#117327,#117328,
#117329,#117330,#117331,#117332,#117333,#117334,#117335,#117336,#117337,
#117338,#117339,#117340,#117341,#117342,#117343,#117344,#117345,#117346,
#117347,#117348,#117349,#117350,#117351,#117352,#117353,#117354,#117355,
#117356,#117357,#117358,#117359,#117360,#117361,#117362,#117363,#117364,
#117365,#117366,#117367,#117368,#117369,#117370,#117371,#117372,#117373,
#117374,#117375,#117376,#117377,#117378,#117379,#117380,#117381,#117382,
#117383,#117384,#117385,#117386,#117387,#117388,#117389,#117390,#117391,
#117392,#117393,#117394,#117395,#117396,#117397,#117398,#117399,#117400,
#117401,#117402,#117403,#117404,#117405,#117406,#117407,#117408,#117409,
#117410,#117411,#117412,#117413,#117414,#117415,#117416,#117417,#117418,
#117419,#117420,#117421,#117422,#117423,#117424,#117425,#117426,#117427,
#117428,#117429,#117430,#117431,#117432,#117433,#117434,#117435,#117436,
#117437,#117438,#117439,#117440,#117441,#117442,#117443,#117444,#117445,
#117446,#117447,#117448,#117449,#117450,#117451,#117452,#117453,#117454,
#117455,#117456,#117457,#117458,#117459,#117460,#117461,#117462,#117463,
#117464,#117465,#117466,#117467,#117468,#117469,#117470,#117471,#117472,
#117473,#117474,#117475,#117476,#117477,#117478,#117479,#117480,#117481,
#117482,#117483,#117484,#117485,#117486,#117487,#117488,#117489,#117490,
#117491,#117492,#117493,#117494,#117495,#117496,#117497,#117498,#117499,
#117500,#117501,#117502,#117503,#117504,#117505,#117506,#117507,#117508,
#117509,#117510,#117511,#117512,#117513,#117514,#117515,#117516,#117517,
#117518,#117519,#117520,#117521,#117522,#117523,#117524,#117525,#117526,
#117527,#117528,#117529,#117530,#117531,#117532,#117533,#117534,#117535,
#117536,#117537,#117538,#117539,#117540,#117541,#117542,#117543,#117544,
#117545,#117546,#117547,#117548,#117549,#117550,#117551,#117552,#117553,
#117554,#117555,#117556,#117557,#117558,#117559,#117560,#117561,#117562,
#117563,#117564,#117565,#117566,#117567,#117568,#117569,#117570,#117571,
#117572,#117573,#117574,#117575,#117576,#117577,#117578,#117579,#117580,
#117581,#117582,#117583,#117584,#117585,#117586,#117587,#117588,#117589,
#117590,#117591,#117592,#117593,#117594,#117595,#117596,#117597,#117598,
#117599,#117600,#117601,#117602,#117603,#117604,#117605,#117606,#117607,
#117608,#117609,#117610,#117611,#117612,#117613,#117614,#117615,#117616,
#117617,#117618,#117619,#117620,#117621,#117622,#117623,#117624,#117625,
#117626,#117627,#117628,#117629,#117630,#117631,#117632,#117633,#117634,
#117635,#117636,#117637,#117638,#117639,#117640,#117641,#117642,#117643,
#117644,#117645,#117646,#117647,#117648,#117649,#117650,#117651,#117652,
#117653,#117654,#117655,#117656,#117657,#117658,#117659,#117660,#117661,
#117662,#117663,#117664,#117665,#117666,#117667,#117668,#117669,#117670,
#117671,#117672,#117673,#117674,#117675,#117676,#117677,#117678,#117679,
#117680,#117681,#117682,#117683,#117684,#117685,#117686,#117687,#117688,
#117689,#117690,#117691,#117692,#117693,#117694,#117695,#117696,#117697,
#117698,#117699,#117700,#117701,#117702,#117703,#117704,#117705,#117706,
#117707,#117708,#117709,#117710,#117711,#117712,#117713,#117714,#117715,
#117716,#117717,#117718,#117719,#117720,#117721,#117722,#117723,#117724,
#117725,#117726,#117727,#117728,#117729,#117730,#117731,#117732,#117733,
#117734,#117735,#117736,#117737,#117738,#117739,#117740,#117741,#117742,
#117743,#117744,#117745,#117746,#117747,#117748,#117749,#117750,#117751,
#117752,#117753,#117754,#117755,#117756,#117757,#117758,#117759,#117760,
#117761,#117762,#117763,#117764,#117765,#117766,#117767,#117768,#117769,
#117770,#117771,#117772,#117773,#117774,#117775,#117776,#117777,#117778,
#117779,#117780,#117781,#117782,#117783,#117784,#117785,#117786,#117787,
#117788,#117789,#117790,#117791,#117792,#117793,#117794,#117795,#117796,
#117797,#117798,#117799,#117800,#117801,#117802,#117803,#117804,#117805,
#117806,#117807,#117808,#117809,#117810,#117811,#117812,#117813,#117814,
#117815,#117816,#117817,#117818,#117819,#117820,#117821,#117822,#117823,
#117824,#117825,#117826,#117827,#117828,#117829,#117830,#117831,#117832,
#117833,#117834,#117835,#117836,#117837,#117838,#117839,#117840,#117841,
#117842,#117843,#117844,#117845,#117846,#117847,#117848,#117849,#117850,
#117851,#117852,#117853,#117854,#117855,#117856,#117857,#117858,#117859,
#117860,#117861,#117862,#117863,#117864,#117865,#117866,#117867,#117868,
#117869,#117870,#117871,#117872,#117873,#117874,#117875,#117876,#117877,
#117878,#117879,#117880,#117881,#117882,#117883,#117884,#117885,#117886,
#117887,#117888,#117889,#117890,#117891,#117892,#117893,#117894,#117895,
#117896,#117897,#117898,#117899,#117900,#117901,#117902,#117903,#117904,
#117905,#117906,#117907,#117908,#117909,#117910,#117911,#117912,#117913,
#117914,#117915,#117916,#117917,#117918,#117919,#117920,#117921,#117922,
#117923,#117924,#117925,#117926,#117927,#117928,#117929,#117930,#117931,
#117932,#117933,#117934,#117935,#117936,#117937,#117938,#117939,#117940,
#117941,#117942,#117943,#117944,#117945,#117946,#117947,#117948,#117949,
#117950,#117951,#117952,#117953,#117954,#117955,#117956,#117957,#117958,
#117959,#117960,#117961,#117962,#117963,#117964,#117965,#117966,#117967,
#117968,#117969,#117970,#117971,#117972,#117973,#117974,#117975,#117976,
#117977,#117978,#117979,#117980,#117981,#117982,#117983,#117984,#117985,
#117986,#117987,#117988,#117989,#117990,#117991,#117992,#117993,#117994,
#117995,#117996,#117997,#117998,#117999,#118000,#118001,#118002,#118003,
#118004,#118005,#118006,#118007,#118008,#118009,#118010,#118011,#118012,
#118013,#118014,#118015,#118016,#118017,#118018,#118019,#118020,#118021,
#118022,#118023,#118024,#118025,#118026,#118027,#118028,#118029,#118030,
#118031,#118032,#118033,#118034,#118035,#118036,#118037,#118038,#118039,
#118040,#118041,#118042,#118043,#118044,#118045,#118046,#118047,#118048,
#118049,#118050,#118051,#118052,#118053,#118054,#118055,#118056,#118057,
#118058,#118059,#118060,#118061,#118062,#118063,#118064,#118065,#118066,
#118067,#118068,#118069,#118070,#118071,#118072,#118073,#118074,#118075,
#118076,#118077,#118078,#118079,#118080,#118081,#118082,#118083,#118084,
#118085,#118086,#118087,#118088,#118089,#118090,#118091,#118092,#118093,
#118094,#118095,#118096,#118097,#118098,#118099,#118100,#118101,#118102,
#118103,#118104,#118105,#118106,#118107,#118108,#118109,#118110,#118111,
#118112,#118113,#118114,#118115,#118116,#118117,#118118,#118119,#118120,
#118121,#118122,#118123,#118124,#118125,#118126,#118127,#118128,#118129,
#118130,#118131,#118132,#118133,#118134,#118135,#118136,#118137,#118138,
#118139,#118140,#118141,#118142,#118143,#118144,#118145,#118146,#118147,
#118148,#118149,#118150,#118151,#118152,#118153,#118154,#118155,#118156,
#118157,#118158,#118159,#118160,#118161,#118162,#118163,#118164,#118165,
#118166,#118167,#118168,#118169,#118170,#118171,#118172,#118173,#118174,
#118175,#118176,#118177,#118178,#118179,#118180,#118181,#118182,#118183,
#118184,#118185,#118186,#118187,#118188,#118189,#118190,#118191,#118192,
#118193,#118194,#118195,#118196,#118197,#118198,#118199,#118200,#118201,
#118202,#118203,#118204,#118205,#118206,#118207,#118208,#118209,#118210,
#118211,#118212,#118213,#118214,#118215,#118216,#118217,#118218,#118219,
#118220,#118221,#118222,#118223,#118224,#118225,#118226,#118227,#118228,
#118229,#118230,#118231,#118232,#118233,#118234,#118235,#118236,#118237,
#118238,#118239,#118240,#118241,#118242,#118243,#118244,#118245,#118246,
#118247,#118248,#118249,#118250,#118251,#118252,#118253,#118254,#118255,
#118256,#118257,#118258,#118259,#118260,#118261,#118262,#118263,#118264,
#118265,#118266,#118267,#118268,#118269,#118270,#118271,#118272,#118273,
#118274,#118275,#118276,#118277,#118278,#118279,#118280,#118281,#118282,
#118283,#118284,#118285,#118286,#118287,#118288,#118289,#118290,#118291,
#118292,#118293,#118294,#118295,#118296,#118297,#118298,#118299,#118300,
#118301,#118302,#118303,#118304,#118305,#118306,#118307,#118308,#118309,
#118310,#118311,#118312,#118313,#118314,#118315,#118316,#118317,#118318,
#118319,#118320,#118321,#118322,#118323,#118324,#118325,#118326,#118327,
#118328,#118329,#118330,#118331,#118332,#118333,#118334,#118335,#118336,
#118337,#118338,#118339,#118340,#118341,#118342,#118343,#118344,#118345,
#118346,#118347,#118348,#118349,#118350,#118351,#118352,#118353,#118354,
#118355,#118356,#118357,#118358,#118359,#118360,#118361,#118362,#118363,
#118364,#118365,#118366,#118367,#118368,#118369,#118370,#118371,#118372,
#118373,#118374,#118375,#118376,#118377,#118378,#118379,#118380,#118381,
#118382,#118383,#118384,#118385,#118386,#118387,#118388,#118389,#118390,
#118391,#118392,#118393,#118394,#118395,#118396,#118397,#118398,#118399,
#118400,#118401,#118402,#118403,#118404,#118405,#118406,#118407,#118408,
#118409,#118410,#118411,#118412,#118413,#118414,#118415,#118416,#118417,
#118418,#118419,#118420,#118421,#118422,#118423,#118424,#118425,#118426,
#118427,#118428,#118429,#118430,#118431,#118432,#118433,#118434,#118435,
#118436,#118437,#118438,#118439,#118440,#118441,#118442,#118443,#118444,
#118445,#118446,#118447,#118448,#118449,#118450,#118451,#118452,#118453,
#118454,#118455,#118456,#118457,#118458,#118459,#118460,#118461,#118462,
#118463,#118464,#118465,#118466,#118467,#118468,#118469,#118470,#118471,
#118472,#118473,#118474,#118475,#118476,#118477,#118478,#118479,#118480,
#118481),(#118482,#118483,#118484,#118485,#118486,#118487,#118488,#118489,
#118490,#118491,#118492,#118493,#118494,#118495,#118496,#118497,#118498,
#118499,#118500,#118501,#118502,#118503,#118504,#118505,#118506,#118507,
#118508,#118509,#118510,#118511,#118512,#118513,#118514,#118515,#118516,
#118517,#118518,#118519,#118520,#118521,#118522,#118523,#118524,#118525,
#118526,#118527,#118528,#118529,#118530,#118531,#118532,#118533,#118534,
#118535,#118536,#118537,#118538,#118539,#118540,#118541,#118542,#118543,
#118544,#118545,#118546,#118547,#118548,#118549,#118550,#118551,#118552,
#118553,#118554,#118555,#118556,#118557,#118558,#118559,#118560,#118561,
#118562,#118563,#118564,#118565,#118566,#118567,#118568,#118569,#118570,
#118571,#118572,#118573,#118574,#118575,#118576,#118577,#118578,#118579,
#118580,#118581,#118582,#118583,#118584,#118585,#118586,#118587,#118588,
#118589,#118590,#118591,#118592,#118593,#118594,#118595,#118596,#118597,
#118598,#118599,#118600,#118601,#118602,#118603,#118604,#118605,#118606,
#118607,#118608,#118609,#118610,#118611,#118612,#118613,#118614,#118615,
#118616,#118617,#118618,#118619,#118620,#118621,#118622,#118623,#118624,
#118625,#118626,#118627,#118628,#118629,#118630,#118631,#118632,#118633,
#118634,#118635,#118636,#118637,#118638,#118639,#118640,#118641,#118642,
#118643,#118644,#118645,#118646,#118647,#118648,#118649,#118650,#118651,
#118652,#118653,#118654,#118655,#118656,#118657,#118658,#118659,#118660,
#118661,#118662,#118663,#118664,#118665,#118666,#118667,#118668,#118669,
#118670,#118671,#118672,#118673,#118674,#118675,#118676,#118677,#118678,
#118679,#118680,#118681,#118682,#118683,#118684,#118685,#118686,#118687,
#118688,#118689,#118690,#118691,#118692,#118693,#118694,#118695,#118696,
#118697,#118698,#118699,#118700,#118701,#118702,#118703,#118704,#118705,
#118706,#118707,#118708,#118709,#118710,#118711,#118712,#118713,#118714,
#118715,#118716,#118717,#118718,#118719,#118720,#118721,#118722,#118723,
#118724,#118725,#118726,#118727,#118728,#118729,#118730,#118731,#118732,
#118733,#118734,#118735,#118736,#118737,#118738,#118739,#118740,#118741,
#118742,#118743,#118744,#118745,#118746,#118747,#118748,#118749,#118750,
#118751,#118752,#118753,#118754,#118755,#118756,#118757,#118758,#118759,
#118760,#118761,#118762,#118763,#118764,#118765,#118766,#118767,#118768,
#118769,#118770,#118771,#118772,#118773,#118774,#118775,#118776,#118777,
#118778,#118779,#118780,#118781,#118782,#118783,#118784,#118785,#118786,
#118787,#118788,#118789,#118790,#118791,#118792,#118793,#118794,#118795,
#118796,#118797,#118798,#118799,#118800,#118801,#118802,#118803,#118804,
#118805,#118806,#118807,#118808,#118809,#118810,#118811,#118812,#118813,
#118814,#118815,#118816,#118817,#118818,#118819,#118820,#118821,#118822,
#118823,#118824,#118825,#118826,#118827,#118828,#118829,#118830,#118831,
#118832,#118833,#118834,#118835,#118836,#118837,#118838,#118839,#118840,
#118841,#118842,#118843,#118844,#118845,#118846,#118847,#118848,#118849,
#118850,#118851,#118852,#118853,#118854,#118855,#118856,#118857,#118858,
#118859,#118860,#118861,#118862,#118863,#118864,#118865,#118866,#118867,
#118868,#118869,#118870,#118871,#118872,#118873,#118874,#118875,#118876,
#118877,#118878,#118879,#118880,#118881,#118882,#118883,#118884,#118885,
#118886,#118887,#118888,#118889,#118890,#118891,#118892,#118893,#118894,
#118895,#118896,#118897,#118898,#118899,#118900,#118901,#118902,#118903,
#118904,#118905,#118906,#118907,#118908,#118909,#118910,#118911,#118912,
#118913,#118914,#118915,#118916,#118917,#118918,#118919,#118920,#118921,
#118922,#118923,#118924,#118925,#118926,#118927,#118928,#118929,#118930,
#118931,#118932,#118933,#118934,#118935,#118936,#118937,#118938,#118939,
#118940,#118941,#118942,#118943,#118944,#118945,#118946,#118947,#118948,
#118949,#118950,#118951,#118952,#118953,#118954,#118955,#118956,#118957,
#118958,#118959,#118960,#118961,#118962,#118963,#118964,#118965,#118966,
#118967,#118968,#118969,#118970,#118971,#118972,#118973,#118974,#118975,
#118976,#118977,#118978,#118979,#118980,#118981,#118982,#118983,#118984,
#118985,#118986,#118987,#118988,#118989,#118990,#118991,#118992,#118993,
#118994,#118995,#118996,#118997,#118998,#118999,#119000,#119001,#119002,
#119003,#119004,#119005,#119006,#119007,#119008,#119009,#119010,#119011,
#119012,#119013,#119014,#119015,#119016,#119017,#119018,#119019,#119020,
#119021,#119022,#119023,#119024,#119025,#119026,#119027,#119028,#119029,
#119030,#119031,#119032,#119033,#119034,#119035,#119036,#119037,#119038,
#119039,#119040,#119041,#119042,#119043,#119044,#119045,#119046,#119047,
#119048,#119049,#119050,#119051,#119052,#119053,#119054,#119055,#119056,
#119057,#119058,#119059,#119060,#119061,#119062,#119063,#119064,#119065,
#119066,#119067,#119068,#119069,#119070,#119071,#119072,#119073,#119074,
#119075,#119076,#119077,#119078,#119079,#119080,#119081,#119082,#119083,
#119084,#119085,#119086,#119087,#119088,#119089,#119090,#119091,#119092,
#119093,#119094,#119095,#119096,#119097,#119098,#119099,#119100,#119101,
#119102,#119103,#119104,#119105,#119106,#119107,#119108,#119109,#119110,
#119111,#119112,#119113,#119114,#119115,#119116,#119117,#119118,#119119,
#119120,#119121,#119122,#119123,#119124,#119125,#119126,#119127,#119128,
#119129,#119130,#119131,#119132,#119133,#119134,#119135,#119136,#119137,
#119138,#119139,#119140,#119141,#119142,#119143,#119144,#119145,#119146,
#119147,#119148,#119149,#119150,#119151,#119152,#119153,#119154,#119155,
#119156,#119157,#119158,#119159,#119160,#119161,#119162,#119163,#119164,
#119165,#119166,#119167,#119168,#119169,#119170,#119171,#119172,#119173,
#119174,#119175,#119176,#119177,#119178,#119179,#119180,#119181,#119182,
#119183,#119184,#119185,#119186,#119187,#119188,#119189,#119190,#119191,
#119192,#119193,#119194,#119195,#119196,#119197,#119198,#119199,#119200,
#119201,#119202,#119203,#119204,#119205,#119206,#119207,#119208,#119209,
#119210,#119211,#119212,#119213,#119214,#119215,#119216,#119217,#119218,
#119219,#119220,#119221,#119222,#119223,#119224,#119225,#119226,#119227,
#119228,#119229,#119230,#119231,#119232,#119233,#119234,#119235,#119236,
#119237,#119238,#119239,#119240,#119241,#119242,#119243,#119244,#119245,
#119246,#119247,#119248,#119249,#119250,#119251,#119252,#119253,#119254,
#119255,#119256,#119257,#119258,#119259,#119260,#119261,#119262,#119263,
#119264,#119265,#119266,#119267,#119268,#119269,#119270,#119271,#119272,
#119273,#119274,#119275,#119276,#119277,#119278,#119279,#119280,#119281,
#119282,#119283,#119284,#119285,#119286,#119287,#119288,#119289,#119290,
#119291,#119292,#119293,#119294,#119295,#119296,#119297,#119298,#119299,
#119300,#119301,#119302,#119303,#119304,#119305,#119306,#119307,#119308,
#119309,#119310,#119311,#119312,#119313,#119314,#119315,#119316,#119317,
#119318,#119319,#119320,#119321,#119322,#119323,#119324,#119325,#119326,
#119327,#119328,#119329,#119330,#119331,#119332,#119333,#119334,#119335,
#119336,#119337,#119338,#119339,#119340,#119341,#119342,#119343,#119344,
#119345,#119346,#119347,#119348,#119349,#119350,#119351,#119352,#119353,
#119354,#119355,#119356,#119357,#119358,#119359,#119360,#119361,#119362,
#119363,#119364,#119365,#119366,#119367,#119368,#119369,#119370,#119371,
#119372,#119373,#119374,#119375,#119376,#119377,#119378,#119379,#119380,
#119381,#119382,#119383,#119384,#119385,#119386,#119387,#119388,#119389,
#119390,#119391,#119392,#119393,#119394,#119395,#119396,#119397,#119398,
#119399,#119400,#119401,#119402,#119403,#119404,#119405,#119406,#119407,
#119408,#119409,#119410,#119411,#119412,#119413,#119414,#119415,#119416,
#119417,#119418,#119419,#119420,#119421,#119422,#119423,#119424,#119425,
#119426,#119427,#119428,#119429,#119430,#119431,#119432,#119433,#119434,
#119435,#119436,#119437,#119438,#119439,#119440,#119441,#119442,#119443,
#119444,#119445,#119446,#119447,#119448,#119449,#119450,#119451,#119452,
#119453,#119454,#119455,#119456,#119457,#119458,#119459,#119460,#119461,
#119462,#119463,#119464,#119465,#119466,#119467,#119468,#119469,#119470,
#119471,#119472,#119473,#119474,#119475,#119476,#119477,#119478,#119479,
#119480,#119481,#119482,#119483,#119484,#119485,#119486,#119487,#119488,
#119489,#119490,#119491,#119492,#119493,#119494,#119495,#119496,#119497,
#119498,#119499,#119500,#119501,#119502,#119503,#119504,#119505,#119506,
#119507,#119508,#119509,#119510,#119511,#119512,#119513,#119514,#119515,
#119516,#119517,#119518,#119519,#119520,#119521,#119522,#119523,#119524,
#119525,#119526,#119527,#119528,#119529,#119530,#119531,#119532,#119533,
#119534,#119535,#119536,#119537,#119538,#119539,#119540,#119541,#119542,
#119543,#119544,#119545,#119546,#119547,#119548,#119549,#119550,#119551,
#119552,#119553,#119554,#119555,#119556,#119557,#119558,#119559,#119560,
#119561,#119562,#119563,#119564,#119565,#119566,#119567,#119568,#119569,
#119570,#119571,#119572,#119573,#119574,#119575,#119576,#119577,#119578,
#119579,#119580,#119581,#119582,#119583,#119584,#119585,#119586,#119587,
#119588,#119589,#119590,#119591,#119592,#119593,#119594,#119595,#119596,
#119597,#119598,#119599,#119600,#119601,#119602,#119603,#119604,#119605,
#119606,#119607,#119608,#119609,#119610,#119611,#119612,#119613,#119614,
#119615,#119616,#119617,#119618,#119619,#119620,#119621,#119622,#119623,
#119624,#119625,#119626,#119627,#119628,#119629,#119630,#119631,#119632,
#119633,#119634,#119635,#119636,#119637,#119638,#119639,#119640,#119641,
#119642,#119643,#119644,#119645,#119646,#119647,#119648,#119649,#119650,
#119651,#119652,#119653,#119654,#119655,#119656,#119657,#119658,#119659,
#119660,#119661,#119662,#119663,#119664,#119665,#119666,#119667,#119668,
#119669,#119670,#119671,#119672,#119673,#119674,#119675,#119676,#119677,
#119678,#119679,#119680,#119681,#119682,#119683,#119684,#119685,#119686,
#119687,#119688,#119689,#119690,#119691,#119692,#119693,#119694,#119695,
#119696,#119697,#119698,#119699,#119700,#119701,#119702,#119703,#119704,
#119705,#119706,#119707,#119708,#119709,#119710,#119711,#119712,#119713,
#119714,#119715,#119716,#119717,#119718,#119719,#119720,#119721,#119722,
#119723,#119724,#119725,#119726,#119727,#119728,#119729,#119730,#119731,
#119732,#119733,#119734,#119735,#119736,#119737,#119738,#119739,#119740,
#119741,#119742,#119743,#119744,#119745,#119746,#119747,#119748,#119749,
#119750,#119751,#119752,#119753,#119754,#119755,#119756,#119757,#119758,
#119759,#119760,#119761,#119762,#119763,#119764,#119765,#119766,#119767,
#119768,#119769,#119770,#119771,#119772,#119773,#119774,#119775,#119776,
#119777,#119778,#119779,#119780,#119781,#119782,#119783,#119784,#119785,
#119786,#119787,#119788,#119789,#119790,#119791,#119792,#119793,#119794,
#119795,#119796,#119797,#119798,#119799,#119800,#119801,#119802,#119803,
#119804,#119805,#119806,#119807,#119808,#119809,#119810,#119811,#119812,
#119813,#119814,#119815,#119816,#119817,#119818,#119819,#119820,#119821,
#119822,#119823,#119824,#119825,#119826,#119827,#119828,#119829,#119830,
#119831,#119832,#119833,#119834,#119835,#119836,#119837,#119838,#119839,
#119840,#119841,#119842,#119843,#119844,#119845,#119846,#119847,#119848,
#119849,#119850,#119851,#119852,#119853,#119854,#119855,#119856,#119857,
#119858,#119859,#119860,#119861,#119862,#119863,#119864,#119865,#119866,
#119867,#119868,#119869,#119870,#119871,#119872,#119873,#119874,#119875,
#119876,#119877,#119878,#119879,#119880,#119881,#119882,#119883,#119884,
#119885,#119886,#119887,#119888,#119889,#119890,#119891,#119892,#119893,
#119894,#119895,#119896,#119897,#119898,#119899,#119900,#119901,#119902,
#119903,#119904,#119905,#119906,#119907,#119908,#119909,#119910,#119911,
#119912,#119913,#119914,#119915,#119916,#119917,#119918,#119919,#119920,
#119921,#119922,#119923,#119924,#119925,#119926,#119927,#119928,#119929,
#119930,#119931,#119932,#119933,#119934,#119935,#119936,#119937,#119938,
#119939,#119940,#119941,#119942,#119943,#119944,#119945,#119946,#119947,
#119948,#119949,#119950,#119951,#119952,#119953,#119954,#119955,#119956,
#119957,#119958,#119959,#119960,#119961,#119962,#119963,#119964,#119965,
#119966,#119967,#119968,#119969,#119970,#119971,#119972,#119973,#119974,
#119975,#119976,#119977,#119978,#119979,#119980,#119981,#119982,#119983,
#119984,#119985,#119986,#119987,#119988,#119989,#119990,#119991,#119992,
#119993,#119994,#119995,#119996,#119997,#119998,#119999,#120000,#120001,
#120002,#120003,#120004,#120005,#120006,#120007,#120008,#120009,#120010,
#120011,#120012,#120013,#120014,#120015,#120016,#120017,#120018,#120019,
#120020,#120021,#120022,#120023,#120024,#120025,#120026,#120027,#120028,
#120029,#120030,#120031,#120032,#120033,#120034,#120035,#120036,#120037,
#120038,#120039,#120040,#120041,#120042,#120043,#120044,#120045,#120046,
#120047,#120048,#120049,#120050,#120051,#120052,#120053,#120054,#120055,
#120056,#120057,#120058,#120059,#120060,#120061,#120062,#120063,#120064,
#120065,#120066,#120067,#120068,#120069,#120070,#120071,#120072,#120073,
#120074,#120075,#120076,#120077,#120078,#120079,#120080,#120081,#120082,
#120083,#120084,#120085,#120086,#120087,#120088,#120089,#120090,#120091,
#120092,#120093,#120094,#120095,#120096,#120097,#120098,#120099,#120100,
#120101,#120102,#120103,#120104,#120105,#120106,#120107,#120108,#120109,
#120110,#120111,#120112,#120113,#120114,#120115,#120116,#120117,#120118,
#120119,#120120,#120121,#120122,#120123,#120124,#120125,#120126,#120127,
#120128,#120129,#120130,#120131,#120132,#120133,#120134,#120135,#120136,
#120137,#120138,#120139,#120140,#120141,#120142,#120143,#120144,#120145,
#120146,#120147,#120148,#120149,#120150,#120151,#120152,#120153,#120154,
#120155,#120156,#120157,#120158,#120159,#120160,#120161,#120162,#120163,
#120164,#120165,#120166,#120167,#120168,#120169,#120170,#120171,#120172,
#120173,#120174,#120175,#120176,#120177,#120178,#120179,#120180,#120181,
#120182,#120183,#120184,#120185,#120186,#120187,#120188,#120189,#120190,
#120191,#120192,#120193,#120194,#120195,#120196,#120197,#120198,#120199,
#120200,#120201,#120202,#120203,#120204,#120205,#120206,#120207,#120208,
#120209,#120210,#120211,#120212,#120213,#120214,#120215,#120216,#120217,
#120218,#120219,#120220,#120221,#120222,#120223,#120224,#120225,#120226,
#120227,#120228,#120229,#120230,#120231,#120232,#120233,#120234,#120235,
#120236,#120237,#120238,#120239,#120240,#120241,#120242,#120243,#120244,
#120245,#120246,#120247,#120248,#120249,#120250,#120251,#120252,#120253,
#120254,#120255,#120256,#120257,#120258,#120259,#120260,#120261,#120262,
#120263,#120264,#120265,#120266,#120267,#120268,#120269,#120270,#120271,
#120272,#120273,#120274,#120275,#120276,#120277,#120278,#120279,#120280,
#120281,#120282,#120283,#120284,#120285,#120286,#120287,#120288,#120289,
#120290,#120291,#120292,#120293,#120294,#120295,#120296,#120297,#120298,
#120299,#120300,#120301,#120302,#120303,#120304,#120305,#120306,#120307,
#120308,#120309,#120310,#120311,#120312,#120313,#120314,#120315,#120316,
#120317,#120318,#120319,#120320,#120321,#120322,#120323,#120324,#120325,
#120326,#120327,#120328,#120329,#120330,#120331,#120332,#120333,#120334,
#120335,#120336,#120337,#120338,#120339,#120340,#120341,#120342,#120343,
#120344,#120345,#120346,#120347,#120348,#120349,#120350,#120351,#120352,
#120353,#120354,#120355,#120356,#120357,#120358,#120359,#120360,#120361,
#120362,#120363,#120364,#120365,#120366,#120367,#120368,#120369,#120370,
#120371,#120372,#120373,#120374,#120375,#120376,#120377,#120378,#120379,
#120380,#120381,#120382,#120383,#120384,#120385,#120386,#120387,#120388,
#120389,#120390,#120391,#120392,#120393,#120394,#120395,#120396,#120397,
#120398,#120399,#120400,#120401,#120402,#120403,#120404,#120405,#120406,
#120407,#120408,#120409,#120410,#120411,#120412,#120413,#120414,#120415,
#120416,#120417,#120418,#120419,#120420,#120421,#120422,#120423,#120424,
#120425,#120426,#120427,#120428,#120429,#120430,#120431,#120432,#120433,
#120434,#120435,#120436,#120437,#120438,#120439,#120440,#120441,#120442,
#120443,#120444,#120445,#120446,#120447,#120448,#120449,#120450,#120451,
#120452,#120453,#120454,#120455,#120456,#120457,#120458,#120459,#120460,
#120461,#120462,#120463,#120464,#120465,#120466,#120467,#120468,#120469,
#120470,#120471,#120472,#120473,#120474,#120475,#120476,#120477,#120478,
#120479,#120480,#120481,#120482,#120483,#120484,#120485,#120486,#120487,
#120488,#120489,#120490,#120491,#120492,#120493,#120494,#120495,#120496,
#120497,#120498,#120499,#120500,#120501,#120502,#120503,#120504,#120505,
#120506,#120507,#120508,#120509,#120510,#120511,#120512,#120513,#120514,
#120515,#120516,#120517,#120518,#120519,#120520,#120521,#120522,#120523,
#120524,#120525,#120526,#120527,#120528,#120529,#120530,#120531,#120532),
(#120533,#120534,#120535,#120536,#120537,#120538,#120539,#120540,#120541,
#120542,#120543,#120544,#120545,#120546,#120547,#120548,#120549,#120550,
#120551,#120552,#120553,#120554,#120555,#120556,#120557,#120558,#120559,
#120560,#120561,#120562,#120563,#120564,#120565,#120566,#120567,#120568,
#120569,#120570,#120571,#120572,#120573,#120574,#120575,#120576,#120577,
#120578,#120579,#120580,#120581,#120582,#120583,#120584,#120585,#120586,
#120587,#120588,#120589,#120590,#120591,#120592,#120593,#120594,#120595,
#120596,#120597,#120598,#120599,#120600,#120601,#120602,#120603,#120604,
#120605,#120606,#120607,#120608,#120609,#120610,#120611,#120612,#120613,
#120614,#120615,#120616,#120617,#120618,#120619,#120620,#120621,#120622,
#120623,#120624,#120625,#120626,#120627,#120628,#120629,#120630,#120631,
#120632,#120633,#120634,#120635,#120636,#120637,#120638,#120639,#120640,
#120641,#120642,#120643,#120644,#120645,#120646,#120647,#120648,#120649,
#120650,#120651,#120652,#120653,#120654,#120655,#120656,#120657,#120658,
#120659,#120660,#120661,#120662,#120663,#120664,#120665,#120666,#120667,
#120668,#120669,#120670,#120671,#120672,#120673,#120674,#120675,#120676,
#120677,#120678,#120679,#120680,#120681,#120682,#120683,#120684,#120685,
#120686,#120687,#120688,#120689,#120690,#120691,#120692,#120693,#120694,
#120695,#120696,#120697,#120698,#120699,#120700,#120701,#120702,#120703,
#120704,#120705,#120706,#120707,#120708,#120709,#120710,#120711,#120712,
#120713,#120714,#120715,#120716,#120717,#120718,#120719,#120720,#120721,
#120722,#120723,#120724,#120725,#120726,#120727,#120728,#120729,#120730,
#120731,#120732,#120733,#120734,#120735,#120736,#120737,#120738,#120739,
#120740,#120741,#120742,#120743,#120744,#120745,#120746,#120747,#120748,
#120749,#120750,#120751,#120752,#120753,#120754,#120755,#120756,#120757,
#120758,#120759,#120760,#120761,#120762,#120763,#120764,#120765,#120766,
#120767,#120768,#120769,#120770,#120771,#120772,#120773,#120774,#120775,
#120776,#120777,#120778,#120779,#120780,#120781,#120782,#120783,#120784,
#120785,#120786,#120787,#120788,#120789,#120790,#120791,#120792,#120793,
#120794,#120795,#120796,#120797,#120798,#120799,#120800,#120801,#120802,
#120803,#120804,#120805,#120806,#120807,#120808,#120809,#120810,#120811,
#120812,#120813,#120814,#120815,#120816,#120817,#120818,#120819,#120820,
#120821,#120822,#120823,#120824,#120825,#120826,#120827,#120828,#120829,
#120830,#120831,#120832,#120833,#120834,#120835,#120836,#120837,#120838,
#120839,#120840,#120841,#120842,#120843,#120844,#120845,#120846,#120847,
#120848,#120849,#120850,#120851,#120852,#120853,#120854,#120855,#120856,
#120857,#120858,#120859,#120860,#120861,#120862,#120863,#120864,#120865,
#120866,#120867,#120868,#120869,#120870,#120871,#120872,#120873,#120874,
#120875,#120876,#120877,#120878,#120879,#120880,#120881,#120882,#120883,
#120884,#120885,#120886,#120887,#120888,#120889,#120890,#120891,#120892,
#120893,#120894,#120895,#120896,#120897,#120898,#120899,#120900,#120901,
#120902,#120903,#120904,#120905,#120906,#120907,#120908,#120909,#120910,
#120911,#120912,#120913,#120914,#120915,#120916,#120917,#120918,#120919,
#120920,#120921,#120922,#120923,#120924,#120925,#120926,#120927,#120928,
#120929,#120930,#120931,#120932,#120933,#120934,#120935,#120936,#120937,
#120938,#120939,#120940,#120941,#120942,#120943,#120944,#120945,#120946,
#120947,#120948,#120949,#120950,#120951,#120952,#120953,#120954,#120955,
#120956,#120957,#120958,#120959,#120960,#120961,#120962,#120963,#120964,
#120965,#120966,#120967,#120968,#120969,#120970,#120971,#120972,#120973,
#120974,#120975,#120976,#120977,#120978,#120979,#120980,#120981,#120982,
#120983,#120984,#120985,#120986,#120987,#120988,#120989,#120990,#120991,
#120992,#120993,#120994,#120995,#120996,#120997,#120998,#120999,#121000,
#121001,#121002,#121003,#121004,#121005,#121006,#121007,#121008,#121009,
#121010,#121011,#121012,#121013,#121014,#121015,#121016,#121017,#121018,
#121019,#121020,#121021,#121022,#121023,#121024,#121025,#121026,#121027,
#121028,#121029,#121030,#121031,#121032,#121033,#121034,#121035,#121036,
#121037,#121038,#121039,#121040,#121041,#121042,#121043,#121044,#121045,
#121046,#121047,#121048,#121049,#121050,#121051,#121052,#121053,#121054,
#121055,#121056,#121057,#121058,#121059,#121060,#121061,#121062,#121063,
#121064,#121065,#121066,#121067,#121068,#121069,#121070,#121071,#121072,
#121073,#121074,#121075,#121076,#121077,#121078,#121079,#121080,#121081,
#121082,#121083,#121084,#121085,#121086,#121087,#121088,#121089,#121090,
#121091,#121092,#121093,#121094,#121095,#121096,#121097,#121098,#121099,
#121100,#121101,#121102,#121103,#121104,#121105,#121106,#121107,#121108,
#121109,#121110,#121111,#121112,#121113,#121114,#121115,#121116,#121117,
#121118,#121119,#121120,#121121,#121122,#121123,#121124,#121125,#121126,
#121127,#121128,#121129,#121130,#121131,#121132,#121133,#121134,#121135,
#121136,#121137,#121138,#121139,#121140,#121141,#121142,#121143,#121144,
#121145,#121146,#121147,#121148,#121149,#121150,#121151,#121152,#121153,
#121154,#121155,#121156,#121157,#121158,#121159,#121160,#121161,#121162,
#121163,#121164,#121165,#121166,#121167,#121168,#121169,#121170,#121171,
#121172,#121173,#121174,#121175,#121176,#121177,#121178,#121179,#121180,
#121181,#121182,#121183,#121184,#121185,#121186,#121187,#121188,#121189,
#121190,#121191,#121192,#121193,#121194,#121195,#121196,#121197,#121198,
#121199,#121200,#121201,#121202,#121203,#121204,#121205,#121206,#121207,
#121208,#121209,#121210,#121211,#121212,#121213,#121214,#121215,#121216,
#121217,#121218,#121219,#121220,#121221,#121222,#121223,#121224,#121225,
#121226,#121227,#121228,#121229,#121230,#121231,#121232,#121233,#121234,
#121235,#121236,#121237,#121238,#121239,#121240,#121241,#121242,#121243,
#121244,#121245,#121246,#121247,#121248,#121249,#121250,#121251,#121252,
#121253,#121254,#121255,#121256,#121257,#121258,#121259,#121260,#121261,
#121262,#121263,#121264,#121265,#121266,#121267,#121268,#121269,#121270,
#121271,#121272,#121273,#121274,#121275,#121276,#121277,#121278,#121279,
#121280,#121281,#121282,#121283,#121284,#121285,#121286,#121287,#121288,
#121289,#121290,#121291,#121292,#121293,#121294,#121295,#121296,#121297,
#121298,#121299,#121300,#121301,#121302,#121303,#121304,#121305,#121306,
#121307,#121308,#121309,#121310,#121311,#121312,#121313,#121314,#121315,
#121316,#121317,#121318,#121319,#121320,#121321,#121322,#121323,#121324,
#121325,#121326,#121327,#121328,#121329,#121330,#121331,#121332,#121333,
#121334,#121335,#121336,#121337,#121338,#121339,#121340,#121341,#121342,
#121343,#121344,#121345,#121346,#121347,#121348,#121349,#121350,#121351,
#121352,#121353,#121354,#121355,#121356,#121357,#121358,#121359,#121360,
#121361,#121362,#121363,#121364,#121365,#121366,#121367,#121368,#121369,
#121370,#121371,#121372,#121373,#121374,#121375,#121376,#121377,#121378,
#121379,#121380,#121381,#121382,#121383,#121384,#121385,#121386,#121387,
#121388,#121389,#121390,#121391,#121392,#121393,#121394,#121395,#121396,
#121397,#121398,#121399,#121400,#121401,#121402,#121403,#121404,#121405,
#121406,#121407,#121408,#121409,#121410,#121411,#121412,#121413,#121414,
#121415,#121416,#121417,#121418,#121419,#121420,#121421,#121422,#121423,
#121424,#121425,#121426,#121427,#121428,#121429,#121430,#121431,#121432,
#121433,#121434,#121435,#121436,#121437,#121438,#121439,#121440,#121441,
#121442,#121443,#121444,#121445,#121446,#121447,#121448,#121449,#121450,
#121451,#121452,#121453,#121454,#121455,#121456,#121457,#121458,#121459,
#121460,#121461,#121462,#121463,#121464,#121465,#121466,#121467,#121468,
#121469,#121470,#121471,#121472,#121473,#121474,#121475,#121476,#121477,
#121478,#121479,#121480,#121481,#121482,#121483,#121484,#121485,#121486,
#121487,#121488,#121489,#121490,#121491,#121492,#121493,#121494,#121495,
#121496,#121497,#121498,#121499,#121500,#121501,#121502,#121503,#121504,
#121505,#121506,#121507,#121508,#121509,#121510,#121511,#121512,#121513,
#121514,#121515,#121516,#121517,#121518,#121519,#121520,#121521,#121522,
#121523,#121524,#121525,#121526,#121527,#121528,#121529,#121530,#121531,
#121532,#121533,#121534,#121535,#121536,#121537,#121538,#121539,#121540,
#121541,#121542,#121543,#121544,#121545,#121546,#121547,#121548,#121549,
#121550,#121551,#121552,#121553,#121554,#121555,#121556,#121557,#121558,
#121559,#121560,#121561,#121562,#121563,#121564,#121565,#121566,#121567,
#121568,#121569,#121570,#121571,#121572,#121573,#121574,#121575,#121576,
#121577,#121578,#121579,#121580,#121581,#121582,#121583,#121584,#121585,
#121586,#121587,#121588,#121589,#121590,#121591,#121592,#121593,#121594,
#121595,#121596,#121597,#121598,#121599,#121600,#121601,#121602,#121603,
#121604,#121605,#121606,#121607,#121608,#121609,#121610,#121611,#121612,
#121613,#121614,#121615,#121616,#121617,#121618,#121619,#121620,#121621,
#121622,#121623,#121624,#121625,#121626,#121627,#121628,#121629,#121630,
#121631,#121632,#121633,#121634,#121635,#121636,#121637,#121638,#121639,
#121640,#121641,#121642,#121643,#121644,#121645,#121646,#121647,#121648,
#121649,#121650,#121651,#121652,#121653,#121654,#121655,#121656,#121657,
#121658,#121659,#121660,#121661,#121662,#121663,#121664,#121665,#121666,
#121667,#121668,#121669,#121670,#121671,#121672,#121673,#121674,#121675,
#121676,#121677,#121678,#121679,#121680,#121681,#121682,#121683,#121684,
#121685,#121686,#121687,#121688,#121689,#121690,#121691,#121692,#121693,
#121694,#121695,#121696,#121697,#121698,#121699,#121700,#121701,#121702,
#121703,#121704,#121705,#121706,#121707,#121708,#121709,#121710,#121711,
#121712,#121713,#121714,#121715,#121716,#121717,#121718,#121719,#121720,
#121721,#121722,#121723,#121724,#121725,#121726,#121727,#121728,#121729,
#121730,#121731,#121732,#121733,#121734,#121735,#121736,#121737,#121738,
#121739,#121740,#121741,#121742,#121743,#121744,#121745,#121746,#121747,
#121748,#121749,#121750,#121751,#121752,#121753,#121754,#121755,#121756,
#121757,#121758,#121759,#121760,#121761,#121762,#121763,#121764,#121765,
#121766,#121767,#121768,#121769,#121770,#121771,#121772,#121773,#121774,
#121775,#121776,#121777,#121778,#121779,#121780,#121781,#121782,#121783,
#121784,#121785,#121786,#121787,#121788,#121789,#121790,#121791,#121792,
#121793,#121794,#121795,#121796,#121797,#121798,#121799,#121800,#121801,
#121802,#121803,#121804,#121805,#121806,#121807,#121808,#121809,#121810,
#121811,#121812,#121813,#121814,#121815,#121816,#121817,#121818,#121819,
#121820,#121821,#121822,#121823,#121824,#121825,#121826,#121827,#121828,
#121829,#121830,#121831,#121832,#121833,#121834,#121835,#121836,#121837,
#121838,#121839,#121840,#121841,#121842,#121843,#121844,#121845,#121846,
#121847,#121848,#121849,#121850,#121851,#121852,#121853,#121854,#121855,
#121856,#121857,#121858,#121859,#121860,#121861,#121862,#121863,#121864,
#121865,#121866,#121867,#121868,#121869,#121870,#121871,#121872,#121873,
#121874,#121875,#121876,#121877,#121878,#121879,#121880,#121881,#121882,
#121883,#121884,#121885,#121886,#121887,#121888,#121889,#121890,#121891,
#121892,#121893,#121894,#121895,#121896,#121897,#121898,#121899,#121900,
#121901,#121902,#121903,#121904,#121905,#121906,#121907,#121908,#121909,
#121910,#121911,#121912,#121913,#121914,#121915,#121916,#121917,#121918,
#121919,#121920,#121921,#121922,#121923,#121924,#121925,#121926,#121927,
#121928,#121929,#121930,#121931,#121932,#121933,#121934,#121935,#121936,
#121937,#121938,#121939,#121940,#121941,#121942,#121943,#121944,#121945,
#121946,#121947,#121948,#121949,#121950,#121951,#121952,#121953,#121954,
#121955,#121956,#121957,#121958,#121959,#121960,#121961,#121962,#121963,
#121964,#121965,#121966,#121967,#121968,#121969,#121970,#121971,#121972,
#121973,#121974,#121975,#121976,#121977,#121978,#121979,#121980,#121981,
#121982,#121983,#121984,#121985,#121986,#121987,#121988,#121989,#121990,
#121991,#121992,#121993,#121994,#121995,#121996,#121997,#121998,#121999,
#122000,#122001,#122002,#122003,#122004,#122005,#122006,#122007,#122008,
#122009,#122010,#122011,#122012,#122013,#122014,#122015,#122016,#122017,
#122018,#122019,#122020,#122021,#122022,#122023,#122024,#122025,#122026,
#122027,#122028,#122029,#122030,#122031,#122032,#122033,#122034,#122035,
#122036,#122037,#122038,#122039,#122040,#122041,#122042,#122043,#122044,
#122045,#122046,#122047,#122048,#122049,#122050,#122051,#122052,#122053,
#122054,#122055,#122056,#122057,#122058,#122059,#122060,#122061,#122062,
#122063,#122064,#122065,#122066,#122067,#122068,#122069,#122070,#122071,
#122072,#122073,#122074,#122075,#122076,#122077,#122078,#122079,#122080,
#122081,#122082,#122083,#122084,#122085,#122086,#122087,#122088,#122089,
#122090,#122091,#122092,#122093,#122094,#122095,#122096,#122097,#122098,
#122099,#122100,#122101,#122102,#122103,#122104,#122105,#122106,#122107,
#122108,#122109,#122110,#122111,#122112,#122113,#122114,#122115,#122116,
#122117,#122118,#122119,#122120,#122121,#122122,#122123,#122124,#122125,
#122126,#122127,#122128,#122129,#122130,#122131,#122132,#122133,#122134,
#122135,#122136,#122137,#122138,#122139,#122140,#122141,#122142,#122143,
#122144,#122145,#122146,#122147,#122148,#122149,#122150,#122151,#122152,
#122153,#122154,#122155,#122156,#122157,#122158,#122159,#122160,#122161,
#122162,#122163,#122164,#122165,#122166,#122167,#122168,#122169,#122170,
#122171,#122172,#122173,#122174,#122175,#122176,#122177,#122178,#122179,
#122180,#122181,#122182,#122183,#122184,#122185,#122186,#122187,#122188,
#122189,#122190,#122191,#122192,#122193,#122194,#122195,#122196,#122197,
#122198,#122199,#122200,#122201,#122202,#122203,#122204,#122205,#122206,
#122207,#122208,#122209,#122210,#122211,#122212,#122213,#122214,#122215,
#122216,#122217,#122218,#122219,#122220,#122221,#122222,#122223,#122224,
#122225,#122226,#122227,#122228,#122229,#122230,#122231,#122232,#122233,
#122234,#122235,#122236,#122237,#122238,#122239,#122240,#122241,#122242,
#122243,#122244,#122245,#122246,#122247,#122248,#122249,#122250,#122251,
#122252,#122253,#122254,#122255,#122256,#122257,#122258,#122259,#122260,
#122261,#122262,#122263,#122264,#122265,#122266,#122267,#122268,#122269,
#122270,#122271,#122272,#122273,#122274,#122275,#122276,#122277,#122278,
#122279,#122280,#122281,#122282,#122283,#122284,#122285,#122286,#122287,
#122288,#122289,#122290,#122291,#122292,#122293,#122294,#122295,#122296,
#122297,#122298,#122299,#122300,#122301,#122302,#122303,#122304,#122305,
#122306,#122307,#122308,#122309,#122310,#122311,#122312,#122313,#122314,
#122315,#122316,#122317,#122318,#122319,#122320,#122321,#122322,#122323,
#122324,#122325,#122326,#122327,#122328,#122329,#122330,#122331,#122332,
#122333,#122334,#122335,#122336,#122337,#122338,#122339,#122340,#122341,
#122342,#122343,#122344,#122345,#122346,#122347,#122348,#122349,#122350,
#122351,#122352,#122353,#122354,#122355,#122356,#122357,#122358,#122359,
#122360,#122361,#122362,#122363,#122364,#122365,#122366,#122367,#122368,
#122369,#122370,#122371,#122372,#122373,#122374,#122375,#122376,#122377,
#122378,#122379,#122380,#122381,#122382,#122383,#122384,#122385,#122386,
#122387,#122388,#122389,#122390,#122391,#122392,#122393,#122394,#122395,
#122396,#122397,#122398,#122399,#122400,#122401,#122402,#122403,#122404,
#122405,#122406,#122407,#122408,#122409,#122410,#122411,#122412,#122413,
#122414,#122415,#122416,#122417,#122418,#122419,#122420,#122421,#122422,
#122423,#122424,#122425,#122426,#122427,#122428,#122429,#122430,#122431,
#122432,#122433,#122434,#122435,#122436,#122437,#122438,#122439,#122440,
#122441,#122442,#122443,#122444,#122445,#122446,#122447,#122448,#122449,
#122450,#122451,#122452,#122453,#122454,#122455,#122456,#122457,#122458,
#122459,#122460,#122461,#122462,#122463,#122464,#122465,#122466,#122467,
#122468,#122469,#122470,#122471,#122472,#122473,#122474,#122475,#122476,
#122477,#122478,#122479,#122480,#122481,#122482,#122483,#122484,#122485,
#122486,#122487,#122488,#122489,#122490,#122491,#122492,#122493,#122494,
#122495,#122496,#122497,#122498,#122499,#122500,#122501,#122502,#122503,
#122504,#122505,#122506,#122507,#122508,#122509,#122510,#122511,#122512,
#122513,#122514,#122515,#122516,#122517,#122518,#122519,#122520,#122521,
#122522,#122523,#122524,#122525,#122526,#122527,#122528,#122529,#122530,
#122531,#122532,#122533,#122534,#122535,#122536,#122537,#122538,#122539,
#122540,#122541,#122542,#122543,#122544,#122545,#122546,#122547,#122548,
#122549,#122550,#122551,#122552,#122553,#122554,#122555,#122556,#122557,
#122558,#122559,#122560,#122561,#122562,#122563,#122564,#122565,#122566,
#122567,#122568,#122569,#122570,#122571,#122572,#122573,#122574,#122575,
#122576,#122577,#122578,#122579,#122580,#122581,#122582,#122583),(#122584,
#122585,#122586,#122587,#122588,#122589,#122590,#122591,#122592,#122593,
#122594,#122595,#122596,#122597,#122598,#122599,#122600,#122601,#122602,
#122603,#122604,#122605,#122606,#122607,#122608,#122609,#122610,#122611,
#122612,#122613,#122614,#122615,#122616,#122617,#122618,#122619,#122620,
#122621,#122622,#122623,#122624,#122625,#122626,#122627,#122628,#122629,
#122630,#122631,#122632,#122633,#122634,#122635,#122636,#122637,#122638,
#122639,#122640,#122641,#122642,#122643,#122644,#122645,#122646,#122647,
#122648,#122649,#122650,#122651,#122652,#122653,#122654,#122655,#122656,
#122657,#122658,#122659,#122660,#122661,#122662,#122663,#122664,#122665,
#122666,#122667,#122668,#122669,#122670,#122671,#122672,#122673,#122674,
#122675,#122676,#122677,#122678,#122679,#122680,#122681,#122682,#122683,
#122684,#122685,#122686,#122687,#122688,#122689,#122690,#122691,#122692,
#122693,#122694,#122695,#122696,#122697,#122698,#122699,#122700,#122701,
#122702,#122703,#122704,#122705,#122706,#122707,#122708,#122709,#122710,
#122711,#122712,#122713,#122714,#122715,#122716,#122717,#122718,#122719,
#122720,#122721,#122722,#122723,#122724,#122725,#122726,#122727,#122728,
#122729,#122730,#122731,#122732,#122733,#122734,#122735,#122736,#122737,
#122738,#122739,#122740,#122741,#122742,#122743,#122744,#122745,#122746,
#122747,#122748,#122749,#122750,#122751,#122752,#122753,#122754,#122755,
#122756,#122757,#122758,#122759,#122760,#122761,#122762,#122763,#122764,
#122765,#122766,#122767,#122768,#122769,#122770,#122771,#122772,#122773,
#122774,#122775,#122776,#122777,#122778,#122779,#122780,#122781,#122782,
#122783,#122784,#122785,#122786,#122787,#122788,#122789,#122790,#122791,
#122792,#122793,#122794,#122795,#122796,#122797,#122798,#122799,#122800,
#122801,#122802,#122803,#122804,#122805,#122806,#122807,#122808,#122809,
#122810,#122811,#122812,#122813,#122814,#122815,#122816,#122817,#122818,
#122819,#122820,#122821,#122822,#122823,#122824,#122825,#122826,#122827,
#122828,#122829,#122830,#122831,#122832,#122833,#122834,#122835,#122836,
#122837,#122838,#122839,#122840,#122841,#122842,#122843,#122844,#122845,
#122846,#122847,#122848,#122849,#122850,#122851,#122852,#122853,#122854,
#122855,#122856,#122857,#122858,#122859,#122860,#122861,#122862,#122863,
#122864,#122865,#122866,#122867,#122868,#122869,#122870,#122871,#122872,
#122873,#122874,#122875,#122876,#122877,#122878,#122879,#122880,#122881,
#122882,#122883,#122884,#122885,#122886,#122887,#122888,#122889,#122890,
#122891,#122892,#122893,#122894,#122895,#122896,#122897,#122898,#122899,
#122900,#122901,#122902,#122903,#122904,#122905,#122906,#122907,#122908,
#122909,#122910,#122911,#122912,#122913,#122914,#122915,#122916,#122917,
#122918,#122919,#122920,#122921,#122922,#122923,#122924,#122925,#122926,
#122927,#122928,#122929,#122930,#122931,#122932,#122933,#122934,#122935,
#122936,#122937,#122938,#122939,#122940,#122941,#122942,#122943,#122944,
#122945,#122946,#122947,#122948,#122949,#122950,#122951,#122952,#122953,
#122954,#122955,#122956,#122957,#122958,#122959,#122960,#122961,#122962,
#122963,#122964,#122965,#122966,#122967,#122968,#122969,#122970,#122971,
#122972,#122973,#122974,#122975,#122976,#122977,#122978,#122979,#122980,
#122981,#122982,#122983,#122984,#122985,#122986,#122987,#122988,#122989,
#122990,#122991,#122992,#122993,#122994,#122995,#122996,#122997,#122998,
#122999,#123000,#123001,#123002,#123003,#123004,#123005,#123006,#123007,
#123008,#123009,#123010,#123011,#123012,#123013,#123014,#123015,#123016,
#123017,#123018,#123019,#123020,#123021,#123022,#123023,#123024,#123025,
#123026,#123027,#123028,#123029,#123030,#123031,#123032,#123033,#123034,
#123035,#123036,#123037,#123038,#123039,#123040,#123041,#123042,#123043,
#123044,#123045,#123046,#123047,#123048,#123049,#123050,#123051,#123052,
#123053,#123054,#123055,#123056,#123057,#123058,#123059,#123060,#123061,
#123062,#123063,#123064,#123065,#123066,#123067,#123068,#123069,#123070,
#123071,#123072,#123073,#123074,#123075,#123076,#123077,#123078,#123079,
#123080,#123081,#123082,#123083,#123084,#123085,#123086,#123087,#123088,
#123089,#123090,#123091,#123092,#123093,#123094,#123095,#123096,#123097,
#123098,#123099,#123100,#123101,#123102,#123103,#123104,#123105,#123106,
#123107,#123108,#123109,#123110,#123111,#123112,#123113,#123114,#123115,
#123116,#123117,#123118,#123119,#123120,#123121,#123122,#123123,#123124,
#123125,#123126,#123127,#123128,#123129,#123130,#123131,#123132,#123133,
#123134,#123135,#123136,#123137,#123138,#123139,#123140,#123141,#123142,
#123143,#123144,#123145,#123146,#123147,#123148,#123149,#123150,#123151,
#123152,#123153,#123154,#123155,#123156,#123157,#123158,#123159,#123160,
#123161,#123162,#123163,#123164,#123165,#123166,#123167,#123168,#123169,
#123170,#123171,#123172,#123173,#123174,#123175,#123176,#123177,#123178,
#123179,#123180,#123181,#123182,#123183,#123184,#123185,#123186,#123187,
#123188,#123189,#123190,#123191,#123192,#123193,#123194,#123195,#123196,
#123197,#123198,#123199,#123200,#123201,#123202,#123203,#123204,#123205,
#123206,#123207,#123208,#123209,#123210,#123211,#123212,#123213,#123214,
#123215,#123216,#123217,#123218,#123219,#123220,#123221,#123222,#123223,
#123224,#123225,#123226,#123227,#123228,#123229,#123230,#123231,#123232,
#123233,#123234,#123235,#123236,#123237,#123238,#123239,#123240,#123241,
#123242,#123243,#123244,#123245,#123246,#123247,#123248,#123249,#123250,
#123251,#123252,#123253,#123254,#123255,#123256,#123257,#123258,#123259,
#123260,#123261,#123262,#123263,#123264,#123265,#123266,#123267,#123268,
#123269,#123270,#123271,#123272,#123273,#123274,#123275,#123276,#123277,
#123278,#123279,#123280,#123281,#123282,#123283,#123284,#123285,#123286,
#123287,#123288,#123289,#123290,#123291,#123292,#123293,#123294,#123295,
#123296,#123297,#123298,#123299,#123300,#123301,#123302,#123303,#123304,
#123305,#123306,#123307,#123308,#123309,#123310,#123311,#123312,#123313,
#123314,#123315,#123316,#123317,#123318,#123319,#123320,#123321,#123322,
#123323,#123324,#123325,#123326,#123327,#123328,#123329,#123330,#123331,
#123332,#123333,#123334,#123335,#123336,#123337,#123338,#123339,#123340,
#123341,#123342,#123343,#123344,#123345,#123346,#123347,#123348,#123349,
#123350,#123351,#123352,#123353,#123354,#123355,#123356,#123357,#123358,
#123359,#123360,#123361,#123362,#123363,#123364,#123365,#123366,#123367,
#123368,#123369,#123370,#123371,#123372,#123373,#123374,#123375,#123376,
#123377,#123378,#123379,#123380,#123381,#123382,#123383,#123384,#123385,
#123386,#123387,#123388,#123389,#123390,#123391,#123392,#123393,#123394,
#123395,#123396,#123397,#123398,#123399,#123400,#123401,#123402,#123403,
#123404,#123405,#123406,#123407,#123408,#123409,#123410,#123411,#123412,
#123413,#123414,#123415,#123416,#123417,#123418,#123419,#123420,#123421,
#123422,#123423,#123424,#123425,#123426,#123427,#123428,#123429,#123430,
#123431,#123432,#123433,#123434,#123435,#123436,#123437,#123438,#123439,
#123440,#123441,#123442,#123443,#123444,#123445,#123446,#123447,#123448,
#123449,#123450,#123451,#123452,#123453,#123454,#123455,#123456,#123457,
#123458,#123459,#123460,#123461,#123462,#123463,#123464,#123465,#123466,
#123467,#123468,#123469,#123470,#123471,#123472,#123473,#123474,#123475,
#123476,#123477,#123478,#123479,#123480,#123481,#123482,#123483,#123484,
#123485,#123486,#123487,#123488,#123489,#123490,#123491,#123492,#123493,
#123494,#123495,#123496,#123497,#123498,#123499,#123500,#123501,#123502,
#123503,#123504,#123505,#123506,#123507,#123508,#123509,#123510,#123511,
#123512,#123513,#123514,#123515,#123516,#123517,#123518,#123519,#123520,
#123521,#123522,#123523,#123524,#123525,#123526,#123527,#123528,#123529,
#123530,#123531,#123532,#123533,#123534,#123535,#123536,#123537,#123538,
#123539,#123540,#123541,#123542,#123543,#123544,#123545,#123546,#123547,
#123548,#123549,#123550,#123551,#123552,#123553,#123554,#123555,#123556,
#123557,#123558,#123559,#123560,#123561,#123562,#123563,#123564,#123565,
#123566,#123567,#123568,#123569,#123570,#123571,#123572,#123573,#123574,
#123575,#123576,#123577,#123578,#123579,#123580,#123581,#123582,#123583,
#123584,#123585,#123586,#123587,#123588,#123589,#123590,#123591,#123592,
#123593,#123594,#123595,#123596,#123597,#123598,#123599,#123600,#123601,
#123602,#123603,#123604,#123605,#123606,#123607,#123608,#123609,#123610,
#123611,#123612,#123613,#123614,#123615,#123616,#123617,#123618,#123619,
#123620,#123621,#123622,#123623,#123624,#123625,#123626,#123627,#123628,
#123629,#123630,#123631,#123632,#123633,#123634,#123635,#123636,#123637,
#123638,#123639,#123640,#123641,#123642,#123643,#123644,#123645,#123646,
#123647,#123648,#123649,#123650,#123651,#123652,#123653,#123654,#123655,
#123656,#123657,#123658,#123659,#123660,#123661,#123662,#123663,#123664,
#123665,#123666,#123667,#123668,#123669,#123670,#123671,#123672,#123673,
#123674,#123675,#123676,#123677,#123678,#123679,#123680,#123681,#123682,
#123683,#123684,#123685,#123686,#123687,#123688,#123689,#123690,#123691,
#123692,#123693,#123694,#123695,#123696,#123697,#123698,#123699,#123700,
#123701,#123702,#123703,#123704,#123705,#123706,#123707,#123708,#123709,
#123710,#123711,#123712,#123713,#123714,#123715,#123716,#123717,#123718,
#123719,#123720,#123721,#123722,#123723,#123724,#123725,#123726,#123727,
#123728,#123729,#123730,#123731,#123732,#123733,#123734,#123735,#123736,
#123737,#123738,#123739,#123740,#123741,#123742,#123743,#123744,#123745,
#123746,#123747,#123748,#123749,#123750,#123751,#123752,#123753,#123754,
#123755,#123756,#123757,#123758,#123759,#123760,#123761,#123762,#123763,
#123764,#123765,#123766,#123767,#123768,#123769,#123770,#123771,#123772,
#123773,#123774,#123775,#123776,#123777,#123778,#123779,#123780,#123781,
#123782,#123783,#123784,#123785,#123786,#123787,#123788,#123789,#123790,
#123791,#123792,#123793,#123794,#123795,#123796,#123797,#123798,#123799,
#123800,#123801,#123802,#123803,#123804,#123805,#123806,#123807,#123808,
#123809,#123810,#123811,#123812,#123813,#123814,#123815,#123816,#123817,
#123818,#123819,#123820,#123821,#123822,#123823,#123824,#123825,#123826,
#123827,#123828,#123829,#123830,#123831,#123832,#123833,#123834,#123835,
#123836,#123837,#123838,#123839,#123840,#123841,#123842,#123843,#123844,
#123845,#123846,#123847,#123848,#123849,#123850,#123851,#123852,#123853,
#123854,#123855,#123856,#123857,#123858,#123859,#123860,#123861,#123862,
#123863,#123864,#123865,#123866,#123867,#123868,#123869,#123870,#123871,
#123872,#123873,#123874,#123875,#123876,#123877,#123878,#123879,#123880,
#123881,#123882,#123883,#123884,#123885,#123886,#123887,#123888,#123889,
#123890,#123891,#123892,#123893,#123894,#123895,#123896,#123897,#123898,
#123899,#123900,#123901,#123902,#123903,#123904,#123905,#123906,#123907,
#123908,#123909,#123910,#123911,#123912,#123913,#123914,#123915,#123916,
#123917,#123918,#123919,#123920,#123921,#123922,#123923,#123924,#123925,
#123926,#123927,#123928,#123929,#123930,#123931,#123932,#123933,#123934,
#123935,#123936,#123937,#123938,#123939,#123940,#123941,#123942,#123943,
#123944,#123945,#123946,#123947,#123948,#123949,#123950,#123951,#123952,
#123953,#123954,#123955,#123956,#123957,#123958,#123959,#123960,#123961,
#123962,#123963,#123964,#123965,#123966,#123967,#123968,#123969,#123970,
#123971,#123972,#123973,#123974,#123975,#123976,#123977,#123978,#123979,
#123980,#123981,#123982,#123983,#123984,#123985,#123986,#123987,#123988,
#123989,#123990,#123991,#123992,#123993,#123994,#123995,#123996,#123997,
#123998,#123999,#124000,#124001,#124002,#124003,#124004,#124005,#124006,
#124007,#124008,#124009,#124010,#124011,#124012,#124013,#124014,#124015,
#124016,#124017,#124018,#124019,#124020,#124021,#124022,#124023,#124024,
#124025,#124026,#124027,#124028,#124029,#124030,#124031,#124032,#124033,
#124034,#124035,#124036,#124037,#124038,#124039,#124040,#124041,#124042,
#124043,#124044,#124045,#124046,#124047,#124048,#124049,#124050,#124051,
#124052,#124053,#124054,#124055,#124056,#124057,#124058,#124059,#124060,
#124061,#124062,#124063,#124064,#124065,#124066,#124067,#124068,#124069,
#124070,#124071,#124072,#124073,#124074,#124075,#124076,#124077,#124078,
#124079,#124080,#124081,#124082,#124083,#124084,#124085,#124086,#124087,
#124088,#124089,#124090,#124091,#124092,#124093,#124094,#124095,#124096,
#124097,#124098,#124099,#124100,#124101,#124102,#124103,#124104,#124105,
#124106,#124107,#124108,#124109,#124110,#124111,#124112,#124113,#124114,
#124115,#124116,#124117,#124118,#124119,#124120,#124121,#124122,#124123,
#124124,#124125,#124126,#124127,#124128,#124129,#124130,#124131,#124132,
#124133,#124134,#124135,#124136,#124137,#124138,#124139,#124140,#124141,
#124142,#124143,#124144,#124145,#124146,#124147,#124148,#124149,#124150,
#124151,#124152,#124153,#124154,#124155,#124156,#124157,#124158,#124159,
#124160,#124161,#124162,#124163,#124164,#124165,#124166,#124167,#124168,
#124169,#124170,#124171,#124172,#124173,#124174,#124175,#124176,#124177,
#124178,#124179,#124180,#124181,#124182,#124183,#124184,#124185,#124186,
#124187,#124188,#124189,#124190,#124191,#124192,#124193,#124194,#124195,
#124196,#124197,#124198,#124199,#124200,#124201,#124202,#124203,#124204,
#124205,#124206,#124207,#124208,#124209,#124210,#124211,#124212,#124213,
#124214,#124215,#124216,#124217,#124218,#124219,#124220,#124221,#124222,
#124223,#124224,#124225,#124226,#124227,#124228,#124229,#124230,#124231,
#124232,#124233,#124234,#124235,#124236,#124237,#124238,#124239,#124240,
#124241,#124242,#124243,#124244,#124245,#124246,#124247,#124248,#124249,
#124250,#124251,#124252,#124253,#124254,#124255,#124256,#124257,#124258,
#124259,#124260,#124261,#124262,#124263,#124264,#124265,#124266,#124267,
#124268,#124269,#124270,#124271,#124272,#124273,#124274,#124275,#124276,
#124277,#124278,#124279,#124280,#124281,#124282,#124283,#124284,#124285,
#124286,#124287,#124288,#124289,#124290,#124291,#124292,#124293,#124294,
#124295,#124296,#124297,#124298,#124299,#124300,#124301,#124302,#124303,
#124304,#124305,#124306,#124307,#124308,#124309,#124310,#124311,#124312,
#124313,#124314,#124315,#124316,#124317,#124318,#124319,#124320,#124321,
#124322,#124323,#124324,#124325,#124326,#124327,#124328,#124329,#124330,
#124331,#124332,#124333,#124334,#124335,#124336,#124337,#124338,#124339,
#124340,#124341,#124342,#124343,#124344,#124345,#124346,#124347,#124348,
#124349,#124350,#124351,#124352,#124353,#124354,#124355,#124356,#124357,
#124358,#124359,#124360,#124361,#124362,#124363,#124364,#124365,#124366,
#124367,#124368,#124369,#124370,#124371,#124372,#124373,#124374,#124375,
#124376,#124377,#124378,#124379,#124380,#124381,#124382,#124383,#124384,
#124385,#124386,#124387,#124388,#124389,#124390,#124391,#124392,#124393,
#124394,#124395,#124396,#124397,#124398,#124399,#124400,#124401,#124402,
#124403,#124404,#124405,#124406,#124407,#124408,#124409,#124410,#124411,
#124412,#124413,#124414,#124415,#124416,#124417,#124418,#124419,#124420,
#124421,#124422,#124423,#124424,#124425,#124426,#124427,#124428,#124429,
#124430,#124431,#124432,#124433,#124434,#124435,#124436,#124437,#124438,
#124439,#124440,#124441,#124442,#124443,#124444,#124445,#124446,#124447,
#124448,#124449,#124450,#124451,#124452,#124453,#124454,#124455,#124456,
#124457,#124458,#124459,#124460,#124461,#124462,#124463,#124464,#124465,
#124466,#124467,#124468,#124469,#124470,#124471,#124472,#124473,#124474,
#124475,#124476,#124477,#124478,#124479,#124480,#124481,#124482,#124483,
#124484,#124485,#124486,#124487,#124488,#124489,#124490,#124491,#124492,
#124493,#124494,#124495,#124496,#124497,#124498,#124499,#124500,#124501,
#124502,#124503,#124504,#124505,#124506,#124507,#124508,#124509,#124510,
#124511,#124512,#124513,#124514,#124515,#124516,#124517,#124518,#124519,
#124520,#124521,#124522,#124523,#124524,#124525,#124526,#124527,#124528,
#124529,#124530,#124531,#124532,#124533,#124534,#124535,#124536,#124537,
#124538,#124539,#124540,#124541,#124542,#124543,#124544,#124545,#124546,
#124547,#124548,#124549,#124550,#124551,#124552,#124553,#124554,#124555,
#124556,#124557,#124558,#124559,#124560,#124561,#124562,#124563,#124564,
#124565,#124566,#124567,#124568,#124569,#124570,#124571,#124572,#124573,
#124574,#124575,#124576,#124577,#124578,#124579,#124580,#124581,#124582,
#124583,#124584,#124585,#124586,#124587,#124588,#124589,#124590,#124591,
#124592,#124593,#124594,#124595,#124596,#124597,#124598,#124599,#124600,
#124601,#124602,#124603,#124604,#124605,#124606,#124607,#124608,#124609,
#124610,#124611,#124612,#124613,#124614,#124615,#124616,#124617,#124618,
#124619,#124620,#124621,#124622,#124623,#124624,#124625,#124626,#124627,
#124628,#124629,#124630,#124631,#124632,#124633,#124634),(#124635,#124636,
#124637,#124638,#124639,#124640,#124641,#124642,#124643,#124644,#124645,
#124646,#124647,#124648,#124649,#124650,#124651,#124652,#124653,#124654,
#124655,#124656,#124657,#124658,#124659,#124660,#124661,#124662,#124663,
#124664,#124665,#124666,#124667,#124668,#124669,#124670,#124671,#124672,
#124673,#124674,#124675,#124676,#124677,#124678,#124679,#124680,#124681,
#124682,#124683,#124684,#124685,#124686,#124687,#124688,#124689,#124690,
#124691,#124692,#124693,#124694,#124695,#124696,#124697,#124698,#124699,
#124700,#124701,#124702,#124703,#124704,#124705,#124706,#124707,#124708,
#124709,#124710,#124711,#124712,#124713,#124714,#124715,#124716,#124717,
#124718,#124719,#124720,#124721,#124722,#124723,#124724,#124725,#124726,
#124727,#124728,#124729,#124730,#124731,#124732,#124733,#124734,#124735,
#124736,#124737,#124738,#124739,#124740,#124741,#124742,#124743,#124744,
#124745,#124746,#124747,#124748,#124749,#124750,#124751,#124752,#124753,
#124754,#124755,#124756,#124757,#124758,#124759,#124760,#124761,#124762,
#124763,#124764,#124765,#124766,#124767,#124768,#124769,#124770,#124771,
#124772,#124773,#124774,#124775,#124776,#124777,#124778,#124779,#124780,
#124781,#124782,#124783,#124784,#124785,#124786,#124787,#124788,#124789,
#124790,#124791,#124792,#124793,#124794,#124795,#124796,#124797,#124798,
#124799,#124800,#124801,#124802,#124803,#124804,#124805,#124806,#124807,
#124808,#124809,#124810,#124811,#124812,#124813,#124814,#124815,#124816,
#124817,#124818,#124819,#124820,#124821,#124822,#124823,#124824,#124825,
#124826,#124827,#124828,#124829,#124830,#124831,#124832,#124833,#124834,
#124835,#124836,#124837,#124838,#124839,#124840,#124841,#124842,#124843,
#124844,#124845,#124846,#124847,#124848,#124849,#124850,#124851,#124852,
#124853,#124854,#124855,#124856,#124857,#124858,#124859,#124860,#124861,
#124862,#124863,#124864,#124865,#124866,#124867,#124868,#124869,#124870,
#124871,#124872,#124873,#124874,#124875,#124876,#124877,#124878,#124879,
#124880,#124881,#124882,#124883,#124884,#124885,#124886,#124887,#124888,
#124889,#124890,#124891,#124892,#124893,#124894,#124895,#124896,#124897,
#124898,#124899,#124900,#124901,#124902,#124903,#124904,#124905,#124906,
#124907,#124908,#124909,#124910,#124911,#124912,#124913,#124914,#124915,
#124916,#124917,#124918,#124919,#124920,#124921,#124922,#124923,#124924,
#124925,#124926,#124927,#124928,#124929,#124930,#124931,#124932,#124933,
#124934,#124935,#124936,#124937,#124938,#124939,#124940,#124941,#124942,
#124943,#124944,#124945,#124946,#124947,#124948,#124949,#124950,#124951,
#124952,#124953,#124954,#124955,#124956,#124957,#124958,#124959,#124960,
#124961,#124962,#124963,#124964,#124965,#124966,#124967,#124968,#124969,
#124970,#124971,#124972,#124973,#124974,#124975,#124976,#124977,#124978,
#124979,#124980,#124981,#124982,#124983,#124984,#124985,#124986,#124987,
#124988,#124989,#124990,#124991,#124992,#124993,#124994,#124995,#124996,
#124997,#124998,#124999,#125000,#125001,#125002,#125003,#125004,#125005,
#125006,#125007,#125008,#125009,#125010,#125011,#125012,#125013,#125014,
#125015,#125016,#125017,#125018,#125019,#125020,#125021,#125022,#125023,
#125024,#125025,#125026,#125027,#125028,#125029,#125030,#125031,#125032,
#125033,#125034,#125035,#125036,#125037,#125038,#125039,#125040,#125041,
#125042,#125043,#125044,#125045,#125046,#125047,#125048,#125049,#125050,
#125051,#125052,#125053,#125054,#125055,#125056,#125057,#125058,#125059,
#125060,#125061,#125062,#125063,#125064,#125065,#125066,#125067,#125068,
#125069,#125070,#125071,#125072,#125073,#125074,#125075,#125076,#125077,
#125078,#125079,#125080,#125081,#125082,#125083,#125084,#125085,#125086,
#125087,#125088,#125089,#125090,#125091,#125092,#125093,#125094,#125095,
#125096,#125097,#125098,#125099,#125100,#125101,#125102,#125103,#125104,
#125105,#125106,#125107,#125108,#125109,#125110,#125111,#125112,#125113,
#125114,#125115,#125116,#125117,#125118,#125119,#125120,#125121,#125122,
#125123,#125124,#125125,#125126,#125127,#125128,#125129,#125130,#125131,
#125132,#125133,#125134,#125135,#125136,#125137,#125138,#125139,#125140,
#125141,#125142,#125143,#125144,#125145,#125146,#125147,#125148,#125149,
#125150,#125151,#125152,#125153,#125154,#125155,#125156,#125157,#125158,
#125159,#125160,#125161,#125162,#125163,#125164,#125165,#125166,#125167,
#125168,#125169,#125170,#125171,#125172,#125173,#125174,#125175,#125176,
#125177,#125178,#125179,#125180,#125181,#125182,#125183,#125184,#125185,
#125186,#125187,#125188,#125189,#125190,#125191,#125192,#125193,#125194,
#125195,#125196,#125197,#125198,#125199,#125200,#125201,#125202,#125203,
#125204,#125205,#125206,#125207,#125208,#125209,#125210,#125211,#125212,
#125213,#125214,#125215,#125216,#125217,#125218,#125219,#125220,#125221,
#125222,#125223,#125224,#125225,#125226,#125227,#125228,#125229,#125230,
#125231,#125232,#125233,#125234,#125235,#125236,#125237,#125238,#125239,
#125240,#125241,#125242,#125243,#125244,#125245,#125246,#125247,#125248,
#125249,#125250,#125251,#125252,#125253,#125254,#125255,#125256,#125257,
#125258,#125259,#125260,#125261,#125262,#125263,#125264,#125265,#125266,
#125267,#125268,#125269,#125270,#125271,#125272,#125273,#125274,#125275,
#125276,#125277,#125278,#125279,#125280,#125281,#125282,#125283,#125284,
#125285,#125286,#125287,#125288,#125289,#125290,#125291,#125292,#125293,
#125294,#125295,#125296,#125297,#125298,#125299,#125300,#125301,#125302,
#125303,#125304,#125305,#125306,#125307,#125308,#125309,#125310,#125311,
#125312,#125313,#125314,#125315,#125316,#125317,#125318,#125319,#125320,
#125321,#125322,#125323,#125324,#125325,#125326,#125327,#125328,#125329,
#125330,#125331,#125332,#125333,#125334,#125335,#125336,#125337,#125338,
#125339,#125340,#125341,#125342,#125343,#125344,#125345,#125346,#125347,
#125348,#125349,#125350,#125351,#125352,#125353,#125354,#125355,#125356,
#125357,#125358,#125359,#125360,#125361,#125362,#125363,#125364,#125365,
#125366,#125367,#125368,#125369,#125370,#125371,#125372,#125373,#125374,
#125375,#125376,#125377,#125378,#125379,#125380,#125381,#125382,#125383,
#125384,#125385,#125386,#125387,#125388,#125389,#125390,#125391,#125392,
#125393,#125394,#125395,#125396,#125397,#125398,#125399,#125400,#125401,
#125402,#125403,#125404,#125405,#125406,#125407,#125408,#125409,#125410,
#125411,#125412,#125413,#125414,#125415,#125416,#125417,#125418,#125419,
#125420,#125421,#125422,#125423,#125424,#125425,#125426,#125427,#125428,
#125429,#125430,#125431,#125432,#125433,#125434,#125435,#125436,#125437,
#125438,#125439,#125440,#125441,#125442,#125443,#125444,#125445,#125446,
#125447,#125448,#125449,#125450,#125451,#125452,#125453,#125454,#125455,
#125456,#125457,#125458,#125459,#125460,#125461,#125462,#125463,#125464,
#125465,#125466,#125467,#125468,#125469,#125470,#125471,#125472,#125473,
#125474,#125475,#125476,#125477,#125478,#125479,#125480,#125481,#125482,
#125483,#125484,#125485,#125486,#125487,#125488,#125489,#125490,#125491,
#125492,#125493,#125494,#125495,#125496,#125497,#125498,#125499,#125500,
#125501,#125502,#125503,#125504,#125505,#125506,#125507,#125508,#125509,
#125510,#125511,#125512,#125513,#125514,#125515,#125516,#125517,#125518,
#125519,#125520,#125521,#125522,#125523,#125524,#125525,#125526,#125527,
#125528,#125529,#125530,#125531,#125532,#125533,#125534,#125535,#125536,
#125537,#125538,#125539,#125540,#125541,#125542,#125543,#125544,#125545,
#125546,#125547,#125548,#125549,#125550,#125551,#125552,#125553,#125554,
#125555,#125556,#125557,#125558,#125559,#125560,#125561,#125562,#125563,
#125564,#125565,#125566,#125567,#125568,#125569,#125570,#125571,#125572,
#125573,#125574,#125575,#125576,#125577,#125578,#125579,#125580,#125581,
#125582,#125583,#125584,#125585,#125586,#125587,#125588,#125589,#125590,
#125591,#125592,#125593,#125594,#125595,#125596,#125597,#125598,#125599,
#125600,#125601,#125602,#125603,#125604,#125605,#125606,#125607,#125608,
#125609,#125610,#125611,#125612,#125613,#125614,#125615,#125616,#125617,
#125618,#125619,#125620,#125621,#125622,#125623,#125624,#125625,#125626,
#125627,#125628,#125629,#125630,#125631,#125632,#125633,#125634,#125635,
#125636,#125637,#125638,#125639,#125640,#125641,#125642,#125643,#125644,
#125645,#125646,#125647,#125648,#125649,#125650,#125651,#125652,#125653,
#125654,#125655,#125656,#125657,#125658,#125659,#125660,#125661,#125662,
#125663,#125664,#125665,#125666,#125667,#125668,#125669,#125670,#125671,
#125672,#125673,#125674,#125675,#125676,#125677,#125678,#125679,#125680,
#125681,#125682,#125683,#125684,#125685,#125686,#125687,#125688,#125689,
#125690,#125691,#125692,#125693,#125694,#125695,#125696,#125697,#125698,
#125699,#125700,#125701,#125702,#125703,#125704,#125705,#125706,#125707,
#125708,#125709,#125710,#125711,#125712,#125713,#125714,#125715,#125716,
#125717,#125718,#125719,#125720,#125721,#125722,#125723,#125724,#125725,
#125726,#125727,#125728,#125729,#125730,#125731,#125732,#125733,#125734,
#125735,#125736,#125737,#125738,#125739,#125740,#125741,#125742,#125743,
#125744,#125745,#125746,#125747,#125748,#125749,#125750,#125751,#125752,
#125753,#125754,#125755,#125756,#125757,#125758,#125759,#125760,#125761,
#125762,#125763,#125764,#125765,#125766,#125767,#125768,#125769,#125770,
#125771,#125772,#125773,#125774,#125775,#125776,#125777,#125778,#125779,
#125780,#125781,#125782,#125783,#125784,#125785,#125786,#125787,#125788,
#125789,#125790,#125791,#125792,#125793,#125794,#125795,#125796,#125797,
#125798,#125799,#125800,#125801,#125802,#125803,#125804,#125805,#125806,
#125807,#125808,#125809,#125810,#125811,#125812,#125813,#125814,#125815,
#125816,#125817,#125818,#125819,#125820,#125821,#125822,#125823,#125824,
#125825,#125826,#125827,#125828,#125829,#125830,#125831,#125832,#125833,
#125834,#125835,#125836,#125837,#125838,#125839,#125840,#125841,#125842,
#125843,#125844,#125845,#125846,#125847,#125848,#125849,#125850,#125851,
#125852,#125853,#125854,#125855,#125856,#125857,#125858,#125859,#125860,
#125861,#125862,#125863,#125864,#125865,#125866,#125867,#125868,#125869,
#125870,#125871,#125872,#125873,#125874,#125875,#125876,#125877,#125878,
#125879,#125880,#125881,#125882,#125883,#125884,#125885,#125886,#125887,
#125888,#125889,#125890,#125891,#125892,#125893,#125894,#125895,#125896,
#125897,#125898,#125899,#125900,#125901,#125902,#125903,#125904,#125905,
#125906,#125907,#125908,#125909,#125910,#125911,#125912,#125913,#125914,
#125915,#125916,#125917,#125918,#125919,#125920,#125921,#125922,#125923,
#125924,#125925,#125926,#125927,#125928,#125929,#125930,#125931,#125932,
#125933,#125934,#125935,#125936,#125937,#125938,#125939,#125940,#125941,
#125942,#125943,#125944,#125945,#125946,#125947,#125948,#125949,#125950,
#125951,#125952,#125953,#125954,#125955,#125956,#125957,#125958,#125959,
#125960,#125961,#125962,#125963,#125964,#125965,#125966,#125967,#125968,
#125969,#125970,#125971,#125972,#125973,#125974,#125975,#125976,#125977,
#125978,#125979,#125980,#125981,#125982,#125983,#125984,#125985,#125986,
#125987,#125988,#125989,#125990,#125991,#125992,#125993,#125994,#125995,
#125996,#125997,#125998,#125999,#126000,#126001,#126002,#126003,#126004,
#126005,#126006,#126007,#126008,#126009,#126010,#126011,#126012,#126013,
#126014,#126015,#126016,#126017,#126018,#126019,#126020,#126021,#126022,
#126023,#126024,#126025,#126026,#126027,#126028,#126029,#126030,#126031,
#126032,#126033,#126034,#126035,#126036,#126037,#126038,#126039,#126040,
#126041,#126042,#126043,#126044,#126045,#126046,#126047,#126048,#126049,
#126050,#126051,#126052,#126053,#126054,#126055,#126056,#126057,#126058,
#126059,#126060,#126061,#126062,#126063,#126064,#126065,#126066,#126067,
#126068,#126069,#126070,#126071,#126072,#126073,#126074,#126075,#126076,
#126077,#126078,#126079,#126080,#126081,#126082,#126083,#126084,#126085,
#126086,#126087,#126088,#126089,#126090,#126091,#126092,#126093,#126094,
#126095,#126096,#126097,#126098,#126099,#126100,#126101,#126102,#126103,
#126104,#126105,#126106,#126107,#126108,#126109,#126110,#126111,#126112,
#126113,#126114,#126115,#126116,#126117,#126118,#126119,#126120,#126121,
#126122,#126123,#126124,#126125,#126126,#126127,#126128,#126129,#126130,
#126131,#126132,#126133,#126134,#126135,#126136,#126137,#126138,#126139,
#126140,#126141,#126142,#126143,#126144,#126145,#126146,#126147,#126148,
#126149,#126150,#126151,#126152,#126153,#126154,#126155,#126156,#126157,
#126158,#126159,#126160,#126161,#126162,#126163,#126164,#126165,#126166,
#126167,#126168,#126169,#126170,#126171,#126172,#126173,#126174,#126175,
#126176,#126177,#126178,#126179,#126180,#126181,#126182,#126183,#126184,
#126185,#126186,#126187,#126188,#126189,#126190,#126191,#126192,#126193,
#126194,#126195,#126196,#126197,#126198,#126199,#126200,#126201,#126202,
#126203,#126204,#126205,#126206,#126207,#126208,#126209,#126210,#126211,
#126212,#126213,#126214,#126215,#126216,#126217,#126218,#126219,#126220,
#126221,#126222,#126223,#126224,#126225,#126226,#126227,#126228,#126229,
#126230,#126231,#126232,#126233,#126234,#126235,#126236,#126237,#126238,
#126239,#126240,#126241,#126242,#126243,#126244,#126245,#126246,#126247,
#126248,#126249,#126250,#126251,#126252,#126253,#126254,#126255,#126256,
#126257,#126258,#126259,#126260,#126261,#126262,#126263,#126264,#126265,
#126266,#126267,#126268,#126269,#126270,#126271,#126272,#126273,#126274,
#126275,#126276,#126277,#126278,#126279,#126280,#126281,#126282,#126283,
#126284,#126285,#126286,#126287,#126288,#126289,#126290,#126291,#126292,
#126293,#126294,#126295,#126296,#126297,#126298,#126299,#126300,#126301,
#126302,#126303,#126304,#126305,#126306,#126307,#126308,#126309,#126310,
#126311,#126312,#126313,#126314,#126315,#126316,#126317,#126318,#126319,
#126320,#126321,#126322,#126323,#126324,#126325,#126326,#126327,#126328,
#126329,#126330,#126331,#126332,#126333,#126334,#126335,#126336,#126337,
#126338,#126339,#126340,#126341,#126342,#126343,#126344,#126345,#126346,
#126347,#126348,#126349,#126350,#126351,#126352,#126353,#126354,#126355,
#126356,#126357,#126358,#126359,#126360,#126361,#126362,#126363,#126364,
#126365,#126366,#126367,#126368,#126369,#126370,#126371,#126372,#126373,
#126374,#126375,#126376,#126377,#126378,#126379,#126380,#126381,#126382,
#126383,#126384,#126385,#126386,#126387,#126388,#126389,#126390,#126391,
#126392,#126393,#126394,#126395,#126396,#126397,#126398,#126399,#126400,
#126401,#126402,#126403,#126404,#126405,#126406,#126407,#126408,#126409,
#126410,#126411,#126412,#126413,#126414,#126415,#126416,#126417,#126418,
#126419,#126420,#126421,#126422,#126423,#126424,#126425,#126426,#126427,
#126428,#126429,#126430,#126431,#126432,#126433,#126434,#126435,#126436,
#126437,#126438,#126439,#126440,#126441,#126442,#126443,#126444,#126445,
#126446,#126447,#126448,#126449,#126450,#126451,#126452,#126453,#126454,
#126455,#126456,#126457,#126458,#126459,#126460,#126461,#126462,#126463,
#126464,#126465,#126466,#126467,#126468,#126469,#126470,#126471,#126472,
#126473,#126474,#126475,#126476,#126477,#126478,#126479,#126480,#126481,
#126482,#126483,#126484,#126485,#126486,#126487,#126488,#126489,#126490,
#126491,#126492,#126493,#126494,#126495,#126496,#126497,#126498,#126499,
#126500,#126501,#126502,#126503,#126504,#126505,#126506,#126507,#126508,
#126509,#126510,#126511,#126512,#126513,#126514,#126515,#126516,#126517,
#126518,#126519,#126520,#126521,#126522,#126523,#126524,#126525,#126526,
#126527,#126528,#126529,#126530,#126531,#126532,#126533,#126534,#126535,
#126536,#126537,#126538,#126539,#126540,#126541,#126542,#126543,#126544,
#126545,#126546,#126547,#126548,#126549,#126550,#126551,#126552,#126553,
#126554,#126555,#126556,#126557,#126558,#126559,#126560,#126561,#126562,
#126563,#126564,#126565,#126566,#126567,#126568,#126569,#126570,#126571,
#126572,#126573,#126574,#126575,#126576,#126577,#126578,#126579,#126580,
#126581,#126582,#126583,#126584,#126585,#126586,#126587,#126588,#126589,
#126590,#126591,#126592,#126593,#126594,#126595,#126596,#126597,#126598,
#126599,#126600,#126601,#126602,#126603,#126604,#126605,#126606,#126607,
#126608,#126609,#126610,#126611,#126612,#126613,#126614,#126615,#126616,
#126617,#126618,#126619,#126620,#126621,#126622,#126623,#126624,#126625,
#126626,#126627,#126628,#126629,#126630,#126631,#126632,#126633,#126634,
#126635,#126636,#126637,#126638,#126639,#126640,#126641,#126642,#126643,
#126644,#126645,#126646,#126647,#126648,#126649,#126650,#126651,#126652,
#126653,#126654,#126655,#126656,#126657,#126658,#126659,#126660,#126661,
#126662,#126663,#126664,#126665,#126666,#126667,#126668,#126669,#126670,
#126671,#126672,#126673,#126674,#126675,#126676,#126677,#126678,#126679,
#126680,#126681,#126682,#126683,#126684,#126685),(#126686,#126687,#126688,
#126689,#126690,#126691,#126692,#126693,#126694,#126695,#126696,#126697,
#126698,#126699,#126700,#126701,#126702,#126703,#126704,#126705,#126706,
#126707,#126708,#126709,#126710,#126711,#126712,#126713,#126714,#126715,
#126716,#126717,#126718,#126719,#126720,#126721,#126722,#126723,#126724,
#126725,#126726,#126727,#126728,#126729,#126730,#126731,#126732,#126733,
#126734,#126735,#126736,#126737,#126738,#126739,#126740,#126741,#126742,
#126743,#126744,#126745,#126746,#126747,#126748,#126749,#126750,#126751,
#126752,#126753,#126754,#126755,#126756,#126757,#126758,#126759,#126760,
#126761,#126762,#126763,#126764,#126765,#126766,#126767,#126768,#126769,
#126770,#126771,#126772,#126773,#126774,#126775,#126776,#126777,#126778,
#126779,#126780,#126781,#126782,#126783,#126784,#126785,#126786,#126787,
#126788,#126789,#126790,#126791,#126792,#126793,#126794,#126795,#126796,
#126797,#126798,#126799,#126800,#126801,#126802,#126803,#126804,#126805,
#126806,#126807,#126808,#126809,#126810,#126811,#126812,#126813,#126814,
#126815,#126816,#126817,#126818,#126819,#126820,#126821,#126822,#126823,
#126824,#126825,#126826,#126827,#126828,#126829,#126830,#126831,#126832,
#126833,#126834,#126835,#126836,#126837,#126838,#126839,#126840,#126841,
#126842,#126843,#126844,#126845,#126846,#126847,#126848,#126849,#126850,
#126851,#126852,#126853,#126854,#126855,#126856,#126857,#126858,#126859,
#126860,#126861,#126862,#126863,#126864,#126865,#126866,#126867,#126868,
#126869,#126870,#126871,#126872,#126873,#126874,#126875,#126876,#126877,
#126878,#126879,#126880,#126881,#126882,#126883,#126884,#126885,#126886,
#126887,#126888,#126889,#126890,#126891,#126892,#126893,#126894,#126895,
#126896,#126897,#126898,#126899,#126900,#126901,#126902,#126903,#126904,
#126905,#126906,#126907,#126908,#126909,#126910,#126911,#126912,#126913,
#126914,#126915,#126916,#126917,#126918,#126919,#126920,#126921,#126922,
#126923,#126924,#126925,#126926,#126927,#126928,#126929,#126930,#126931,
#126932,#126933,#126934,#126935,#126936,#126937,#126938,#126939,#126940,
#126941,#126942,#126943,#126944,#126945,#126946,#126947,#126948,#126949,
#126950,#126951,#126952,#126953,#126954,#126955,#126956,#126957,#126958,
#126959,#126960,#126961,#126962,#126963,#126964,#126965,#126966,#126967,
#126968,#126969,#126970,#126971,#126972,#126973,#126974,#126975,#126976,
#126977,#126978,#126979,#126980,#126981,#126982,#126983,#126984,#126985,
#126986,#126987,#126988,#126989,#126990,#126991,#126992,#126993,#126994,
#126995,#126996,#126997,#126998,#126999,#127000,#127001,#127002,#127003,
#127004,#127005,#127006,#127007,#127008,#127009,#127010,#127011,#127012,
#127013,#127014,#127015,#127016,#127017,#127018,#127019,#127020,#127021,
#127022,#127023,#127024,#127025,#127026,#127027,#127028,#127029,#127030,
#127031,#127032,#127033,#127034,#127035,#127036,#127037,#127038,#127039,
#127040,#127041,#127042,#127043,#127044,#127045,#127046,#127047,#127048,
#127049,#127050,#127051,#127052,#127053,#127054,#127055,#127056,#127057,
#127058,#127059,#127060,#127061,#127062,#127063,#127064,#127065,#127066,
#127067,#127068,#127069,#127070,#127071,#127072,#127073,#127074,#127075,
#127076,#127077,#127078,#127079,#127080,#127081,#127082,#127083,#127084,
#127085,#127086,#127087,#127088,#127089,#127090,#127091,#127092,#127093,
#127094,#127095,#127096,#127097,#127098,#127099,#127100,#127101,#127102,
#127103,#127104,#127105,#127106,#127107,#127108,#127109,#127110,#127111,
#127112,#127113,#127114,#127115,#127116,#127117,#127118,#127119,#127120,
#127121,#127122,#127123,#127124,#127125,#127126,#127127,#127128,#127129,
#127130,#127131,#127132,#127133,#127134,#127135,#127136,#127137,#127138,
#127139,#127140,#127141,#127142,#127143,#127144,#127145,#127146,#127147,
#127148,#127149,#127150,#127151,#127152,#127153,#127154,#127155,#127156,
#127157,#127158,#127159,#127160,#127161,#127162,#127163,#127164,#127165,
#127166,#127167,#127168,#127169,#127170,#127171,#127172,#127173,#127174,
#127175,#127176,#127177,#127178,#127179,#127180,#127181,#127182,#127183,
#127184,#127185,#127186,#127187,#127188,#127189,#127190,#127191,#127192,
#127193,#127194,#127195,#127196,#127197,#127198,#127199,#127200,#127201,
#127202,#127203,#127204,#127205,#127206,#127207,#127208,#127209,#127210,
#127211,#127212,#127213,#127214,#127215,#127216,#127217,#127218,#127219,
#127220,#127221,#127222,#127223,#127224,#127225,#127226,#127227,#127228,
#127229,#127230,#127231,#127232,#127233,#127234,#127235,#127236,#127237,
#127238,#127239,#127240,#127241,#127242,#127243,#127244,#127245,#127246,
#127247,#127248,#127249,#127250,#127251,#127252,#127253,#127254,#127255,
#127256,#127257,#127258,#127259,#127260,#127261,#127262,#127263,#127264,
#127265,#127266,#127267,#127268,#127269,#127270,#127271,#127272,#127273,
#127274,#127275,#127276,#127277,#127278,#127279,#127280,#127281,#127282,
#127283,#127284,#127285,#127286,#127287,#127288,#127289,#127290,#127291,
#127292,#127293,#127294,#127295,#127296,#127297,#127298,#127299,#127300,
#127301,#127302,#127303,#127304,#127305,#127306,#127307,#127308,#127309,
#127310,#127311,#127312,#127313,#127314,#127315,#127316,#127317,#127318,
#127319,#127320,#127321,#127322,#127323,#127324,#127325,#127326,#127327,
#127328,#127329,#127330,#127331,#127332,#127333,#127334,#127335,#127336,
#127337,#127338,#127339,#127340,#127341,#127342,#127343,#127344,#127345,
#127346,#127347,#127348,#127349,#127350,#127351,#127352,#127353,#127354,
#127355,#127356,#127357,#127358,#127359,#127360,#127361,#127362,#127363,
#127364,#127365,#127366,#127367,#127368,#127369,#127370,#127371,#127372,
#127373,#127374,#127375,#127376,#127377,#127378,#127379,#127380,#127381,
#127382,#127383,#127384,#127385,#127386,#127387,#127388,#127389,#127390,
#127391,#127392,#127393,#127394,#127395,#127396,#127397,#127398,#127399,
#127400,#127401,#127402,#127403,#127404,#127405,#127406,#127407,#127408,
#127409,#127410,#127411,#127412,#127413,#127414,#127415,#127416,#127417,
#127418,#127419,#127420,#127421,#127422,#127423,#127424,#127425,#127426,
#127427,#127428,#127429,#127430,#127431,#127432,#127433,#127434,#127435,
#127436,#127437,#127438,#127439,#127440,#127441,#127442,#127443,#127444,
#127445,#127446,#127447,#127448,#127449,#127450,#127451,#127452,#127453,
#127454,#127455,#127456,#127457,#127458,#127459,#127460,#127461,#127462,
#127463,#127464,#127465,#127466,#127467,#127468,#127469,#127470,#127471,
#127472,#127473,#127474,#127475,#127476,#127477,#127478,#127479,#127480,
#127481,#127482,#127483,#127484,#127485,#127486,#127487,#127488,#127489,
#127490,#127491,#127492,#127493,#127494,#127495,#127496,#127497,#127498,
#127499,#127500,#127501,#127502,#127503,#127504,#127505,#127506,#127507,
#127508,#127509,#127510,#127511,#127512,#127513,#127514,#127515,#127516,
#127517,#127518,#127519,#127520,#127521,#127522,#127523,#127524,#127525,
#127526,#127527,#127528,#127529,#127530,#127531,#127532,#127533,#127534,
#127535,#127536,#127537,#127538,#127539,#127540,#127541,#127542,#127543,
#127544,#127545,#127546,#127547,#127548,#127549,#127550,#127551,#127552,
#127553,#127554,#127555,#127556,#127557,#127558,#127559,#127560,#127561,
#127562,#127563,#127564,#127565,#127566,#127567,#127568,#127569,#127570,
#127571,#127572,#127573,#127574,#127575,#127576,#127577,#127578,#127579,
#127580,#127581,#127582,#127583,#127584,#127585,#127586,#127587,#127588,
#127589,#127590,#127591,#127592,#127593,#127594,#127595,#127596,#127597,
#127598,#127599,#127600,#127601,#127602,#127603,#127604,#127605,#127606,
#127607,#127608,#127609,#127610,#127611,#127612,#127613,#127614,#127615,
#127616,#127617,#127618,#127619,#127620,#127621,#127622,#127623,#127624,
#127625,#127626,#127627,#127628,#127629,#127630,#127631,#127632,#127633,
#127634,#127635,#127636,#127637,#127638,#127639,#127640,#127641,#127642,
#127643,#127644,#127645,#127646,#127647,#127648,#127649,#127650,#127651,
#127652,#127653,#127654,#127655,#127656,#127657,#127658,#127659,#127660,
#127661,#127662,#127663,#127664,#127665,#127666,#127667,#127668,#127669,
#127670,#127671,#127672,#127673,#127674,#127675,#127676,#127677,#127678,
#127679,#127680,#127681,#127682,#127683,#127684,#127685,#127686,#127687,
#127688,#127689,#127690,#127691,#127692,#127693,#127694,#127695,#127696,
#127697,#127698,#127699,#127700,#127701,#127702,#127703,#127704,#127705,
#127706,#127707,#127708,#127709,#127710,#127711,#127712,#127713,#127714,
#127715,#127716,#127717,#127718,#127719,#127720,#127721,#127722,#127723,
#127724,#127725,#127726,#127727,#127728,#127729,#127730,#127731,#127732,
#127733,#127734,#127735,#127736,#127737,#127738,#127739,#127740,#127741,
#127742,#127743,#127744,#127745,#127746,#127747,#127748,#127749,#127750,
#127751,#127752,#127753,#127754,#127755,#127756,#127757,#127758,#127759,
#127760,#127761,#127762,#127763,#127764,#127765,#127766,#127767,#127768,
#127769,#127770,#127771,#127772,#127773,#127774,#127775,#127776,#127777,
#127778,#127779,#127780,#127781,#127782,#127783,#127784,#127785,#127786,
#127787,#127788,#127789,#127790,#127791,#127792,#127793,#127794,#127795,
#127796,#127797,#127798,#127799,#127800,#127801,#127802,#127803,#127804,
#127805,#127806,#127807,#127808,#127809,#127810,#127811,#127812,#127813,
#127814,#127815,#127816,#127817,#127818,#127819,#127820,#127821,#127822,
#127823,#127824,#127825,#127826,#127827,#127828,#127829,#127830,#127831,
#127832,#127833,#127834,#127835,#127836,#127837,#127838,#127839,#127840,
#127841,#127842,#127843,#127844,#127845,#127846,#127847,#127848,#127849,
#127850,#127851,#127852,#127853,#127854,#127855,#127856,#127857,#127858,
#127859,#127860,#127861,#127862,#127863,#127864,#127865,#127866,#127867,
#127868,#127869,#127870,#127871,#127872,#127873,#127874,#127875,#127876,
#127877,#127878,#127879,#127880,#127881,#127882,#127883,#127884,#127885,
#127886,#127887,#127888,#127889,#127890,#127891,#127892,#127893,#127894,
#127895,#127896,#127897,#127898,#127899,#127900,#127901,#127902,#127903,
#127904,#127905,#127906,#127907,#127908,#127909,#127910,#127911,#127912,
#127913,#127914,#127915,#127916,#127917,#127918,#127919,#127920,#127921,
#127922,#127923,#127924,#127925,#127926,#127927,#127928,#127929,#127930,
#127931,#127932,#127933,#127934,#127935,#127936,#127937,#127938,#127939,
#127940,#127941,#127942,#127943,#127944,#127945,#127946,#127947,#127948,
#127949,#127950,#127951,#127952,#127953,#127954,#127955,#127956,#127957,
#127958,#127959,#127960,#127961,#127962,#127963,#127964,#127965,#127966,
#127967,#127968,#127969,#127970,#127971,#127972,#127973,#127974,#127975,
#127976,#127977,#127978,#127979,#127980,#127981,#127982,#127983,#127984,
#127985,#127986,#127987,#127988,#127989,#127990,#127991,#127992,#127993,
#127994,#127995,#127996,#127997,#127998,#127999,#128000,#128001,#128002,
#128003,#128004,#128005,#128006,#128007,#128008,#128009,#128010,#128011,
#128012,#128013,#128014,#128015,#128016,#128017,#128018,#128019,#128020,
#128021,#128022,#128023,#128024,#128025,#128026,#128027,#128028,#128029,
#128030,#128031,#128032,#128033,#128034,#128035,#128036,#128037,#128038,
#128039,#128040,#128041,#128042,#128043,#128044,#128045,#128046,#128047,
#128048,#128049,#128050,#128051,#128052,#128053,#128054,#128055,#128056,
#128057,#128058,#128059,#128060,#128061,#128062,#128063,#128064,#128065,
#128066,#128067,#128068,#128069,#128070,#128071,#128072,#128073,#128074,
#128075,#128076,#128077,#128078,#128079,#128080,#128081,#128082,#128083,
#128084,#128085,#128086,#128087,#128088,#128089,#128090,#128091,#128092,
#128093,#128094,#128095,#128096,#128097,#128098,#128099,#128100,#128101,
#128102,#128103,#128104,#128105,#128106,#128107,#128108,#128109,#128110,
#128111,#128112,#128113,#128114,#128115,#128116,#128117,#128118,#128119,
#128120,#128121,#128122,#128123,#128124,#128125,#128126,#128127,#128128,
#128129,#128130,#128131,#128132,#128133,#128134,#128135,#128136,#128137,
#128138,#128139,#128140,#128141,#128142,#128143,#128144,#128145,#128146,
#128147,#128148,#128149,#128150,#128151,#128152,#128153,#128154,#128155,
#128156,#128157,#128158,#128159,#128160,#128161,#128162,#128163,#128164,
#128165,#128166,#128167,#128168,#128169,#128170,#128171,#128172,#128173,
#128174,#128175,#128176,#128177,#128178,#128179,#128180,#128181,#128182,
#128183,#128184,#128185,#128186,#128187,#128188,#128189,#128190,#128191,
#128192,#128193,#128194,#128195,#128196,#128197,#128198,#128199,#128200,
#128201,#128202,#128203,#128204,#128205,#128206,#128207,#128208,#128209,
#128210,#128211,#128212,#128213,#128214,#128215,#128216,#128217,#128218,
#128219,#128220,#128221,#128222,#128223,#128224,#128225,#128226,#128227,
#128228,#128229,#128230,#128231,#128232,#128233,#128234,#128235,#128236,
#128237,#128238,#128239,#128240,#128241,#128242,#128243,#128244,#128245,
#128246,#128247,#128248,#128249,#128250,#128251,#128252,#128253,#128254,
#128255,#128256,#128257,#128258,#128259,#128260,#128261,#128262,#128263,
#128264,#128265,#128266,#128267,#128268,#128269,#128270,#128271,#128272,
#128273,#128274,#128275,#128276,#128277,#128278,#128279,#128280,#128281,
#128282,#128283,#128284,#128285,#128286,#128287,#128288,#128289,#128290,
#128291,#128292,#128293,#128294,#128295,#128296,#128297,#128298,#128299,
#128300,#128301,#128302,#128303,#128304,#128305,#128306,#128307,#128308,
#128309,#128310,#128311,#128312,#128313,#128314,#128315,#128316,#128317,
#128318,#128319,#128320,#128321,#128322,#128323,#128324,#128325,#128326,
#128327,#128328,#128329,#128330,#128331,#128332,#128333,#128334,#128335,
#128336,#128337,#128338,#128339,#128340,#128341,#128342,#128343,#128344,
#128345,#128346,#128347,#128348,#128349,#128350,#128351,#128352,#128353,
#128354,#128355,#128356,#128357,#128358,#128359,#128360,#128361,#128362,
#128363,#128364,#128365,#128366,#128367,#128368,#128369,#128370,#128371,
#128372,#128373,#128374,#128375,#128376,#128377,#128378,#128379,#128380,
#128381,#128382,#128383,#128384,#128385,#128386,#128387,#128388,#128389,
#128390,#128391,#128392,#128393,#128394,#128395,#128396,#128397,#128398,
#128399,#128400,#128401,#128402,#128403,#128404,#128405,#128406,#128407,
#128408,#128409,#128410,#128411,#128412,#128413,#128414,#128415,#128416,
#128417,#128418,#128419,#128420,#128421,#128422,#128423,#128424,#128425,
#128426,#128427,#128428,#128429,#128430,#128431,#128432,#128433,#128434,
#128435,#128436,#128437,#128438,#128439,#128440,#128441,#128442,#128443,
#128444,#128445,#128446,#128447,#128448,#128449,#128450,#128451,#128452,
#128453,#128454,#128455,#128456,#128457,#128458,#128459,#128460,#128461,
#128462,#128463,#128464,#128465,#128466,#128467,#128468,#128469,#128470,
#128471,#128472,#128473,#128474,#128475,#128476,#128477,#128478,#128479,
#128480,#128481,#128482,#128483,#128484,#128485,#128486,#128487,#128488,
#128489,#128490,#128491,#128492,#128493,#128494,#128495,#128496,#128497,
#128498,#128499,#128500,#128501,#128502,#128503,#128504,#128505,#128506,
#128507,#128508,#128509,#128510,#128511,#128512,#128513,#128514,#128515,
#128516,#128517,#128518,#128519,#128520,#128521,#128522,#128523,#128524,
#128525,#128526,#128527,#128528,#128529,#128530,#128531,#128532,#128533,
#128534,#128535,#128536,#128537,#128538,#128539,#128540,#128541,#128542,
#128543,#128544,#128545,#128546,#128547,#128548,#128549,#128550,#128551,
#128552,#128553,#128554,#128555,#128556,#128557,#128558,#128559,#128560,
#128561,#128562,#128563,#128564,#128565,#128566,#128567,#128568,#128569,
#128570,#128571,#128572,#128573,#128574,#128575,#128576,#128577,#128578,
#128579,#128580,#128581,#128582,#128583,#128584,#128585,#128586,#128587,
#128588,#128589,#128590,#128591,#128592,#128593,#128594,#128595,#128596,
#128597,#128598,#128599,#128600,#128601,#128602,#128603,#128604,#128605,
#128606,#128607,#128608,#128609,#128610,#128611,#128612,#128613,#128614,
#128615,#128616,#128617,#128618,#128619,#128620,#128621,#128622,#128623,
#128624,#128625,#128626,#128627,#128628,#128629,#128630,#128631,#128632,
#128633,#128634,#128635,#128636,#128637,#128638,#128639,#128640,#128641,
#128642,#128643,#128644,#128645,#128646,#128647,#128648,#128649,#128650,
#128651,#128652,#128653,#128654,#128655,#128656,#128657,#128658,#128659,
#128660,#128661,#128662,#128663,#128664,#128665,#128666,#128667,#128668,
#128669,#128670,#128671,#128672,#128673,#128674,#128675,#128676,#128677,
#128678,#128679,#128680,#128681,#128682,#128683,#128684,#128685,#128686,
#128687,#128688,#128689,#128690,#128691,#128692,#128693,#128694,#128695,
#128696,#128697,#128698,#128699,#128700,#128701,#128702,#128703,#128704,
#128705,#128706,#128707,#128708,#128709,#128710,#128711,#128712,#128713,
#128714,#128715,#128716,#128717,#128718,#128719,#128720,#128721,#128722,
#128723,#128724,#128725,#128726,#128727,#128728,#128729,#128730,#128731,
#128732,#128733,#128734,#128735,#128736),(#128737,#128738,#128739,#128740,
#128741,#128742,#128743,#128744,#128745,#128746,#128747,#128748,#128749,
#128750,#128751,#128752,#128753,#128754,#128755,#128756,#128757,#128758,
#128759,#128760,#128761,#128762,#128763,#128764,#128765,#128766,#128767,
#128768,#128769,#128770,#128771,#128772,#128773,#128774,#128775,#128776,
#128777,#128778,#128779,#128780,#128781,#128782,#128783,#128784,#128785,
#128786,#128787,#128788,#128789,#128790,#128791,#128792,#128793,#128794,
#128795,#128796,#128797,#128798,#128799,#128800,#128801,#128802,#128803,
#128804,#128805,#128806,#128807,#128808,#128809,#128810,#128811,#128812,
#128813,#128814,#128815,#128816,#128817,#128818,#128819,#128820,#128821,
#128822,#128823,#128824,#128825,#128826,#128827,#128828,#128829,#128830,
#128831,#128832,#128833,#128834,#128835,#128836,#128837,#128838,#128839,
#128840,#128841,#128842,#128843,#128844,#128845,#128846,#128847,#128848,
#128849,#128850,#128851,#128852,#128853,#128854,#128855,#128856,#128857,
#128858,#128859,#128860,#128861,#128862,#128863,#128864,#128865,#128866,
#128867,#128868,#128869,#128870,#128871,#128872,#128873,#128874,#128875,
#128876,#128877,#128878,#128879,#128880,#128881,#128882,#128883,#128884,
#128885,#128886,#128887,#128888,#128889,#128890,#128891,#128892,#128893,
#128894,#128895,#128896,#128897,#128898,#128899,#128900,#128901,#128902,
#128903,#128904,#128905,#128906,#128907,#128908,#128909,#128910,#128911,
#128912,#128913,#128914,#128915,#128916,#128917,#128918,#128919,#128920,
#128921,#128922,#128923,#128924,#128925,#128926,#128927,#128928,#128929,
#128930,#128931,#128932,#128933,#128934,#128935,#128936,#128937,#128938,
#128939,#128940,#128941,#128942,#128943,#128944,#128945,#128946,#128947,
#128948,#128949,#128950,#128951,#128952,#128953,#128954,#128955,#128956,
#128957,#128958,#128959,#128960,#128961,#128962,#128963,#128964,#128965,
#128966,#128967,#128968,#128969,#128970,#128971,#128972,#128973,#128974,
#128975,#128976,#128977,#128978,#128979,#128980,#128981,#128982,#128983,
#128984,#128985,#128986,#128987,#128988,#128989,#128990,#128991,#128992,
#128993,#128994,#128995,#128996,#128997,#128998,#128999,#129000,#129001,
#129002,#129003,#129004,#129005,#129006,#129007,#129008,#129009,#129010,
#129011,#129012,#129013,#129014,#129015,#129016,#129017,#129018,#129019,
#129020,#129021,#129022,#129023,#129024,#129025,#129026,#129027,#129028,
#129029,#129030,#129031,#129032,#129033,#129034,#129035,#129036,#129037,
#129038,#129039,#129040,#129041,#129042,#129043,#129044,#129045,#129046,
#129047,#129048,#129049,#129050,#129051,#129052,#129053,#129054,#129055,
#129056,#129057,#129058,#129059,#129060,#129061,#129062,#129063,#129064,
#129065,#129066,#129067,#129068,#129069,#129070,#129071,#129072,#129073,
#129074,#129075,#129076,#129077,#129078,#129079,#129080,#129081,#129082,
#129083,#129084,#129085,#129086,#129087,#129088,#129089,#129090,#129091,
#129092,#129093,#129094,#129095,#129096,#129097,#129098,#129099,#129100,
#129101,#129102,#129103,#129104,#129105,#129106,#129107,#129108,#129109,
#129110,#129111,#129112,#129113,#129114,#129115,#129116,#129117,#129118,
#129119,#129120,#129121,#129122,#129123,#129124,#129125,#129126,#129127,
#129128,#129129,#129130,#129131,#129132,#129133,#129134,#129135,#129136,
#129137,#129138,#129139,#129140,#129141,#129142,#129143,#129144,#129145,
#129146,#129147,#129148,#129149,#129150,#129151,#129152,#129153,#129154,
#129155,#129156,#129157,#129158,#129159,#129160,#129161,#129162,#129163,
#129164,#129165,#129166,#129167,#129168,#129169,#129170,#129171,#129172,
#129173,#129174,#129175,#129176,#129177,#129178,#129179,#129180,#129181,
#129182,#129183,#129184,#129185,#129186,#129187,#129188,#129189,#129190,
#129191,#129192,#129193,#129194,#129195,#129196,#129197,#129198,#129199,
#129200,#129201,#129202,#129203,#129204,#129205,#129206,#129207,#129208,
#129209,#129210,#129211,#129212,#129213,#129214,#129215,#129216,#129217,
#129218,#129219,#129220,#129221,#129222,#129223,#129224,#129225,#129226,
#129227,#129228,#129229,#129230,#129231,#129232,#129233,#129234,#129235,
#129236,#129237,#129238,#129239,#129240,#129241,#129242,#129243,#129244,
#129245,#129246,#129247,#129248,#129249,#129250,#129251,#129252,#129253,
#129254,#129255,#129256,#129257,#129258,#129259,#129260,#129261,#129262,
#129263,#129264,#129265,#129266,#129267,#129268,#129269,#129270,#129271,
#129272,#129273,#129274,#129275,#129276,#129277,#129278,#129279,#129280,
#129281,#129282,#129283,#129284,#129285,#129286,#129287,#129288,#129289,
#129290,#129291,#129292,#129293,#129294,#129295,#129296,#129297,#129298,
#129299,#129300,#129301,#129302,#129303,#129304,#129305,#129306,#129307,
#129308,#129309,#129310,#129311,#129312,#129313,#129314,#129315,#129316,
#129317,#129318,#129319,#129320,#129321,#129322,#129323,#129324,#129325,
#129326,#129327,#129328,#129329,#129330,#129331,#129332,#129333,#129334,
#129335,#129336,#129337,#129338,#129339,#129340,#129341,#129342,#129343,
#129344,#129345,#129346,#129347,#129348,#129349,#129350,#129351,#129352,
#129353,#129354,#129355,#129356,#129357,#129358,#129359,#129360,#129361,
#129362,#129363,#129364,#129365,#129366,#129367,#129368,#129369,#129370,
#129371,#129372,#129373,#129374,#129375,#129376,#129377,#129378,#129379,
#129380,#129381,#129382,#129383,#129384,#129385,#129386,#129387,#129388,
#129389,#129390,#129391,#129392,#129393,#129394,#129395,#129396,#129397,
#129398,#129399,#129400,#129401,#129402,#129403,#129404,#129405,#129406,
#129407,#129408,#129409,#129410,#129411,#129412,#129413,#129414,#129415,
#129416,#129417,#129418,#129419,#129420,#129421,#129422,#129423,#129424,
#129425,#129426,#129427,#129428,#129429,#129430,#129431,#129432,#129433,
#129434,#129435,#129436,#129437,#129438,#129439,#129440,#129441,#129442,
#129443,#129444,#129445,#129446,#129447,#129448,#129449,#129450,#129451,
#129452,#129453,#129454,#129455,#129456,#129457,#129458,#129459,#129460,
#129461,#129462,#129463,#129464,#129465,#129466,#129467,#129468,#129469,
#129470,#129471,#129472,#129473,#129474,#129475,#129476,#129477,#129478,
#129479,#129480,#129481,#129482,#129483,#129484,#129485,#129486,#129487,
#129488,#129489,#129490,#129491,#129492,#129493,#129494,#129495,#129496,
#129497,#129498,#129499,#129500,#129501,#129502,#129503,#129504,#129505,
#129506,#129507,#129508,#129509,#129510,#129511,#129512,#129513,#129514,
#129515,#129516,#129517,#129518,#129519,#129520,#129521,#129522,#129523,
#129524,#129525,#129526,#129527,#129528,#129529,#129530,#129531,#129532,
#129533,#129534,#129535,#129536,#129537,#129538,#129539,#129540,#129541,
#129542,#129543,#129544,#129545,#129546,#129547,#129548,#129549,#129550,
#129551,#129552,#129553,#129554,#129555,#129556,#129557,#129558,#129559,
#129560,#129561,#129562,#129563,#129564,#129565,#129566,#129567,#129568,
#129569,#129570,#129571,#129572,#129573,#129574,#129575,#129576,#129577,
#129578,#129579,#129580,#129581,#129582,#129583,#129584,#129585,#129586,
#129587,#129588,#129589,#129590,#129591,#129592,#129593,#129594,#129595,
#129596,#129597,#129598,#129599,#129600,#129601,#129602,#129603,#129604,
#129605,#129606,#129607,#129608,#129609,#129610,#129611,#129612,#129613,
#129614,#129615,#129616,#129617,#129618,#129619,#129620,#129621,#129622,
#129623,#129624,#129625,#129626,#129627,#129628,#129629,#129630,#129631,
#129632,#129633,#129634,#129635,#129636,#129637,#129638,#129639,#129640,
#129641,#129642,#129643,#129644,#129645,#129646,#129647,#129648,#129649,
#129650,#129651,#129652,#129653,#129654,#129655,#129656,#129657,#129658,
#129659,#129660,#129661,#129662,#129663,#129664,#129665,#129666,#129667,
#129668,#129669,#129670,#129671,#129672,#129673,#129674,#129675,#129676,
#129677,#129678,#129679,#129680,#129681,#129682,#129683,#129684,#129685,
#129686,#129687,#129688,#129689,#129690,#129691,#129692,#129693,#129694,
#129695,#129696,#129697,#129698,#129699,#129700,#129701,#129702,#129703,
#129704,#129705,#129706,#129707,#129708,#129709,#129710,#129711,#129712,
#129713,#129714,#129715,#129716,#129717,#129718,#129719,#129720,#129721,
#129722,#129723,#129724,#129725,#129726,#129727,#129728,#129729,#129730,
#129731,#129732,#129733,#129734,#129735,#129736,#129737,#129738,#129739,
#129740,#129741,#129742,#129743,#129744,#129745,#129746,#129747,#129748,
#129749,#129750,#129751,#129752,#129753,#129754,#129755,#129756,#129757,
#129758,#129759,#129760,#129761,#129762,#129763,#129764,#129765,#129766,
#129767,#129768,#129769,#129770,#129771,#129772,#129773,#129774,#129775,
#129776,#129777,#129778,#129779,#129780,#129781,#129782,#129783,#129784,
#129785,#129786,#129787,#129788,#129789,#129790,#129791,#129792,#129793,
#129794,#129795,#129796,#129797,#129798,#129799,#129800,#129801,#129802,
#129803,#129804,#129805,#129806,#129807,#129808,#129809,#129810,#129811,
#129812,#129813,#129814,#129815,#129816,#129817,#129818,#129819,#129820,
#129821,#129822,#129823,#129824,#129825,#129826,#129827,#129828,#129829,
#129830,#129831,#129832,#129833,#129834,#129835,#129836,#129837,#129838,
#129839,#129840,#129841,#129842,#129843,#129844,#129845,#129846,#129847,
#129848,#129849,#129850,#129851,#129852,#129853,#129854,#129855,#129856,
#129857,#129858,#129859,#129860,#129861,#129862,#129863,#129864,#129865,
#129866,#129867,#129868,#129869,#129870,#129871,#129872,#129873,#129874,
#129875,#129876,#129877,#129878,#129879,#129880,#129881,#129882,#129883,
#129884,#129885,#129886,#129887,#129888,#129889,#129890,#129891,#129892,
#129893,#129894,#129895,#129896,#129897,#129898,#129899,#129900,#129901,
#129902,#129903,#129904,#129905,#129906,#129907,#129908,#129909,#129910,
#129911,#129912,#129913,#129914,#129915,#129916,#129917,#129918,#129919,
#129920,#129921,#129922,#129923,#129924,#129925,#129926,#129927,#129928,
#129929,#129930,#129931,#129932,#129933,#129934,#129935,#129936,#129937,
#129938,#129939,#129940,#129941,#129942,#129943,#129944,#129945,#129946,
#129947,#129948,#129949,#129950,#129951,#129952,#129953,#129954,#129955,
#129956,#129957,#129958,#129959,#129960,#129961,#129962,#129963,#129964,
#129965,#129966,#129967,#129968,#129969,#129970,#129971,#129972,#129973,
#129974,#129975,#129976,#129977,#129978,#129979,#129980,#129981,#129982,
#129983,#129984,#129985,#129986,#129987,#129988,#129989,#129990,#129991,
#129992,#129993,#129994,#129995,#129996,#129997,#129998,#129999,#130000,
#130001,#130002,#130003,#130004,#130005,#130006,#130007,#130008,#130009,
#130010,#130011,#130012,#130013,#130014,#130015,#130016,#130017,#130018,
#130019,#130020,#130021,#130022,#130023,#130024,#130025,#130026,#130027,
#130028,#130029,#130030,#130031,#130032,#130033,#130034,#130035,#130036,
#130037,#130038,#130039,#130040,#130041,#130042,#130043,#130044,#130045,
#130046,#130047,#130048,#130049,#130050,#130051,#130052,#130053,#130054,
#130055,#130056,#130057,#130058,#130059,#130060,#130061,#130062,#130063,
#130064,#130065,#130066,#130067,#130068,#130069,#130070,#130071,#130072,
#130073,#130074,#130075,#130076,#130077,#130078,#130079,#130080,#130081,
#130082,#130083,#130084,#130085,#130086,#130087,#130088,#130089,#130090,
#130091,#130092,#130093,#130094,#130095,#130096,#130097,#130098,#130099,
#130100,#130101,#130102,#130103,#130104,#130105,#130106,#130107,#130108,
#130109,#130110,#130111,#130112,#130113,#130114,#130115,#130116,#130117,
#130118,#130119,#130120,#130121,#130122,#130123,#130124,#130125,#130126,
#130127,#130128,#130129,#130130,#130131,#130132,#130133,#130134,#130135,
#130136,#130137,#130138,#130139,#130140,#130141,#130142,#130143,#130144,
#130145,#130146,#130147,#130148,#130149,#130150,#130151,#130152,#130153,
#130154,#130155,#130156,#130157,#130158,#130159,#130160,#130161,#130162,
#130163,#130164,#130165,#130166,#130167,#130168,#130169,#130170,#130171,
#130172,#130173,#130174,#130175,#130176,#130177,#130178,#130179,#130180,
#130181,#130182,#130183,#130184,#130185,#130186,#130187,#130188,#130189,
#130190,#130191,#130192,#130193,#130194,#130195,#130196,#130197,#130198,
#130199,#130200,#130201,#130202,#130203,#130204,#130205,#130206,#130207,
#130208,#130209,#130210,#130211,#130212,#130213,#130214,#130215,#130216,
#130217,#130218,#130219,#130220,#130221,#130222,#130223,#130224,#130225,
#130226,#130227,#130228,#130229,#130230,#130231,#130232,#130233,#130234,
#130235,#130236,#130237,#130238,#130239,#130240,#130241,#130242,#130243,
#130244,#130245,#130246,#130247,#130248,#130249,#130250,#130251,#130252,
#130253,#130254,#130255,#130256,#130257,#130258,#130259,#130260,#130261,
#130262,#130263,#130264,#130265,#130266,#130267,#130268,#130269,#130270,
#130271,#130272,#130273,#130274,#130275,#130276,#130277,#130278,#130279,
#130280,#130281,#130282,#130283,#130284,#130285,#130286,#130287,#130288,
#130289,#130290,#130291,#130292,#130293,#130294,#130295,#130296,#130297,
#130298,#130299,#130300,#130301,#130302,#130303,#130304,#130305,#130306,
#130307,#130308,#130309,#130310,#130311,#130312,#130313,#130314,#130315,
#130316,#130317,#130318,#130319,#130320,#130321,#130322,#130323,#130324,
#130325,#130326,#130327,#130328,#130329,#130330,#130331,#130332,#130333,
#130334,#130335,#130336,#130337,#130338,#130339,#130340,#130341,#130342,
#130343,#130344,#130345,#130346,#130347,#130348,#130349,#130350,#130351,
#130352,#130353,#130354,#130355,#130356,#130357,#130358,#130359,#130360,
#130361,#130362,#130363,#130364,#130365,#130366,#130367,#130368,#130369,
#130370,#130371,#130372,#130373,#130374,#130375,#130376,#130377,#130378,
#130379,#130380,#130381,#130382,#130383,#130384,#130385,#130386,#130387,
#130388,#130389,#130390,#130391,#130392,#130393,#130394,#130395,#130396,
#130397,#130398,#130399,#130400,#130401,#130402,#130403,#130404,#130405,
#130406,#130407,#130408,#130409,#130410,#130411,#130412,#130413,#130414,
#130415,#130416,#130417,#130418,#130419,#130420,#130421,#130422,#130423,
#130424,#130425,#130426,#130427,#130428,#130429,#130430,#130431,#130432,
#130433,#130434,#130435,#130436,#130437,#130438,#130439,#130440,#130441,
#130442,#130443,#130444,#130445,#130446,#130447,#130448,#130449,#130450,
#130451,#130452,#130453,#130454,#130455,#130456,#130457,#130458,#130459,
#130460,#130461,#130462,#130463,#130464,#130465,#130466,#130467,#130468,
#130469,#130470,#130471,#130472,#130473,#130474,#130475,#130476,#130477,
#130478,#130479,#130480,#130481,#130482,#130483,#130484,#130485,#130486,
#130487,#130488,#130489,#130490,#130491,#130492,#130493,#130494,#130495,
#130496,#130497,#130498,#130499,#130500,#130501,#130502,#130503,#130504,
#130505,#130506,#130507,#130508,#130509,#130510,#130511,#130512,#130513,
#130514,#130515,#130516,#130517,#130518,#130519,#130520,#130521,#130522,
#130523,#130524,#130525,#130526,#130527,#130528,#130529,#130530,#130531,
#130532,#130533,#130534,#130535,#130536,#130537,#130538,#130539,#130540,
#130541,#130542,#130543,#130544,#130545,#130546,#130547,#130548,#130549,
#130550,#130551,#130552,#130553,#130554,#130555,#130556,#130557,#130558,
#130559,#130560,#130561,#130562,#130563,#130564,#130565,#130566,#130567,
#130568,#130569,#130570,#130571,#130572,#130573,#130574,#130575,#130576,
#130577,#130578,#130579,#130580,#130581,#130582,#130583,#130584,#130585,
#130586,#130587,#130588,#130589,#130590,#130591,#130592,#130593,#130594,
#130595,#130596,#130597,#130598,#130599,#130600,#130601,#130602,#130603,
#130604,#130605,#130606,#130607,#130608,#130609,#130610,#130611,#130612,
#130613,#130614,#130615,#130616,#130617,#130618,#130619,#130620,#130621,
#130622,#130623,#130624,#130625,#130626,#130627,#130628,#130629,#130630,
#130631,#130632,#130633,#130634,#130635,#130636,#130637,#130638,#130639,
#130640,#130641,#130642,#130643,#130644,#130645,#130646,#130647,#130648,
#130649,#130650,#130651,#130652,#130653,#130654,#130655,#130656,#130657,
#130658,#130659,#130660,#130661,#130662,#130663,#130664,#130665,#130666,
#130667,#130668,#130669,#130670,#130671,#130672,#130673,#130674,#130675,
#130676,#130677,#130678,#130679,#130680,#130681,#130682,#130683,#130684,
#130685,#130686,#130687,#130688,#130689,#130690,#130691,#130692,#130693,
#130694,#130695,#130696,#130697,#130698,#130699,#130700,#130701,#130702,
#130703,#130704,#130705,#130706,#130707,#130708,#130709,#130710,#130711,
#130712,#130713,#130714,#130715,#130716,#130717,#130718,#130719,#130720,
#130721,#130722,#130723,#130724,#130725,#130726,#130727,#130728,#130729,
#130730,#130731,#130732,#130733,#130734,#130735,#130736,#130737,#130738,
#130739,#130740,#130741,#130742,#130743,#130744,#130745,#130746,#130747,
#130748,#130749,#130750,#130751,#130752,#130753,#130754,#130755,#130756,
#130757,#130758,#130759,#130760,#130761,#130762,#130763,#130764,#130765,
#130766,#130767,#130768,#130769,#130770,#130771,#130772,#130773,#130774,
#130775,#130776,#130777,#130778,#130779,#130780,#130781,#130782,#130783,
#130784,#130785,#130786,#130787),(#130788,#130789,#130790,#130791,#130792,
#130793,#130794,#130795,#130796,#130797,#130798,#130799,#130800,#130801,
#130802,#130803,#130804,#130805,#130806,#130807,#130808,#130809,#130810,
#130811,#130812,#130813,#130814,#130815,#130816,#130817,#130818,#130819,
#130820,#130821,#130822,#130823,#130824,#130825,#130826,#130827,#130828,
#130829,#130830,#130831,#130832,#130833,#130834,#130835,#130836,#130837,
#130838,#130839,#130840,#130841,#130842,#130843,#130844,#130845,#130846,
#130847,#130848,#130849,#130850,#130851,#130852,#130853,#130854,#130855,
#130856,#130857,#130858,#130859,#130860,#130861,#130862,#130863,#130864,
#130865,#130866,#130867,#130868,#130869,#130870,#130871,#130872,#130873,
#130874,#130875,#130876,#130877,#130878,#130879,#130880,#130881,#130882,
#130883,#130884,#130885,#130886,#130887,#130888,#130889,#130890,#130891,
#130892,#130893,#130894,#130895,#130896,#130897,#130898,#130899,#130900,
#130901,#130902,#130903,#130904,#130905,#130906,#130907,#130908,#130909,
#130910,#130911,#130912,#130913,#130914,#130915,#130916,#130917,#130918,
#130919,#130920,#130921,#130922,#130923,#130924,#130925,#130926,#130927,
#130928,#130929,#130930,#130931,#130932,#130933,#130934,#130935,#130936,
#130937,#130938,#130939,#130940,#130941,#130942,#130943,#130944,#130945,
#130946,#130947,#130948,#130949,#130950,#130951,#130952,#130953,#130954,
#130955,#130956,#130957,#130958,#130959,#130960,#130961,#130962,#130963,
#130964,#130965,#130966,#130967,#130968,#130969,#130970,#130971,#130972,
#130973,#130974,#130975,#130976,#130977,#130978,#130979,#130980,#130981,
#130982,#130983,#130984,#130985,#130986,#130987,#130988,#130989,#130990,
#130991,#130992,#130993,#130994,#130995,#130996,#130997,#130998,#130999,
#131000,#131001,#131002,#131003,#131004,#131005,#131006,#131007,#131008,
#131009,#131010,#131011,#131012,#131013,#131014,#131015,#131016,#131017,
#131018,#131019,#131020,#131021,#131022,#131023,#131024,#131025,#131026,
#131027,#131028,#131029,#131030,#131031,#131032,#131033,#131034,#131035,
#131036,#131037,#131038,#131039,#131040,#131041,#131042,#131043,#131044,
#131045,#131046,#131047,#131048,#131049,#131050,#131051,#131052,#131053,
#131054,#131055,#131056,#131057,#131058,#131059,#131060,#131061,#131062,
#131063,#131064,#131065,#131066,#131067,#131068,#131069,#131070,#131071,
#131072,#131073,#131074,#131075,#131076,#131077,#131078,#131079,#131080,
#131081,#131082,#131083,#131084,#131085,#131086,#131087,#131088,#131089,
#131090,#131091,#131092,#131093,#131094,#131095,#131096,#131097,#131098,
#131099,#131100,#131101,#131102,#131103,#131104,#131105,#131106,#131107,
#131108,#131109,#131110,#131111,#131112,#131113,#131114,#131115,#131116,
#131117,#131118,#131119,#131120,#131121,#131122,#131123,#131124,#131125,
#131126,#131127,#131128,#131129,#131130,#131131,#131132,#131133,#131134,
#131135,#131136,#131137,#131138,#131139,#131140,#131141,#131142,#131143,
#131144,#131145,#131146,#131147,#131148,#131149,#131150,#131151,#131152,
#131153,#131154,#131155,#131156,#131157,#131158,#131159,#131160,#131161,
#131162,#131163,#131164,#131165,#131166,#131167,#131168,#131169,#131170,
#131171,#131172,#131173,#131174,#131175,#131176,#131177,#131178,#131179,
#131180,#131181,#131182,#131183,#131184,#131185,#131186,#131187,#131188,
#131189,#131190,#131191,#131192,#131193,#131194,#131195,#131196,#131197,
#131198,#131199,#131200,#131201,#131202,#131203,#131204,#131205,#131206,
#131207,#131208,#131209,#131210,#131211,#131212,#131213,#131214,#131215,
#131216,#131217,#131218,#131219,#131220,#131221,#131222,#131223,#131224,
#131225,#131226,#131227,#131228,#131229,#131230,#131231,#131232,#131233,
#131234,#131235,#131236,#131237,#131238,#131239,#131240,#131241,#131242,
#131243,#131244,#131245,#131246,#131247,#131248,#131249,#131250,#131251,
#131252,#131253,#131254,#131255,#131256,#131257,#131258,#131259,#131260,
#131261,#131262,#131263,#131264,#131265,#131266,#131267,#131268,#131269,
#131270,#131271,#131272,#131273,#131274,#131275,#131276,#131277,#131278,
#131279,#131280,#131281,#131282,#131283,#131284,#131285,#131286,#131287,
#131288,#131289,#131290,#131291,#131292,#131293,#131294,#131295,#131296,
#131297,#131298,#131299,#131300,#131301,#131302,#131303,#131304,#131305,
#131306,#131307,#131308,#131309,#131310,#131311,#131312,#131313,#131314,
#131315,#131316,#131317,#131318,#131319,#131320,#131321,#131322,#131323,
#131324,#131325,#131326,#131327,#131328,#131329,#131330,#131331,#131332,
#131333,#131334,#131335,#131336,#131337,#131338,#131339,#131340,#131341,
#131342,#131343,#131344,#131345,#131346,#131347,#131348,#131349,#131350,
#131351,#131352,#131353,#131354,#131355,#131356,#131357,#131358,#131359,
#131360,#131361,#131362,#131363,#131364,#131365,#131366,#131367,#131368,
#131369,#131370,#131371,#131372,#131373,#131374,#131375,#131376,#131377,
#131378,#131379,#131380,#131381,#131382,#131383,#131384,#131385,#131386,
#131387,#131388,#131389,#131390,#131391,#131392,#131393,#131394,#131395,
#131396,#131397,#131398,#131399,#131400,#131401,#131402,#131403,#131404,
#131405,#131406,#131407,#131408,#131409,#131410,#131411,#131412,#131413,
#131414,#131415,#131416,#131417,#131418,#131419,#131420,#131421,#131422,
#131423,#131424,#131425,#131426,#131427,#131428,#131429,#131430,#131431,
#131432,#131433,#131434,#131435,#131436,#131437,#131438,#131439,#131440,
#131441,#131442,#131443,#131444,#131445,#131446,#131447,#131448,#131449,
#131450,#131451,#131452,#131453,#131454,#131455,#131456,#131457,#131458,
#131459,#131460,#131461,#131462,#131463,#131464,#131465,#131466,#131467,
#131468,#131469,#131470,#131471,#131472,#131473,#131474,#131475,#131476,
#131477,#131478,#131479,#131480,#131481,#131482,#131483,#131484,#131485,
#131486,#131487,#131488,#131489,#131490,#131491,#131492,#131493,#131494,
#131495,#131496,#131497,#131498,#131499,#131500,#131501,#131502,#131503,
#131504,#131505,#131506,#131507,#131508,#131509,#131510,#131511,#131512,
#131513,#131514,#131515,#131516,#131517,#131518,#131519,#131520,#131521,
#131522,#131523,#131524,#131525,#131526,#131527,#131528,#131529,#131530,
#131531,#131532,#131533,#131534,#131535,#131536,#131537,#131538,#131539,
#131540,#131541,#131542,#131543,#131544,#131545,#131546,#131547,#131548,
#131549,#131550,#131551,#131552,#131553,#131554,#131555,#131556,#131557,
#131558,#131559,#131560,#131561,#131562,#131563,#131564,#131565,#131566,
#131567,#131568,#131569,#131570,#131571,#131572,#131573,#131574,#131575,
#131576,#131577,#131578,#131579,#131580,#131581,#131582,#131583,#131584,
#131585,#131586,#131587,#131588,#131589,#131590,#131591,#131592,#131593,
#131594,#131595,#131596,#131597,#131598,#131599,#131600,#131601,#131602,
#131603,#131604,#131605,#131606,#131607,#131608,#131609,#131610,#131611,
#131612,#131613,#131614,#131615,#131616,#131617,#131618,#131619,#131620,
#131621,#131622,#131623,#131624,#131625,#131626,#131627,#131628,#131629,
#131630,#131631,#131632,#131633,#131634,#131635,#131636,#131637,#131638,
#131639,#131640,#131641,#131642,#131643,#131644,#131645,#131646,#131647,
#131648,#131649,#131650,#131651,#131652,#131653,#131654,#131655,#131656,
#131657,#131658,#131659,#131660,#131661,#131662,#131663,#131664,#131665,
#131666,#131667,#131668,#131669,#131670,#131671,#131672,#131673,#131674,
#131675,#131676,#131677,#131678,#131679,#131680,#131681,#131682,#131683,
#131684,#131685,#131686,#131687,#131688,#131689,#131690,#131691,#131692,
#131693,#131694,#131695,#131696,#131697,#131698,#131699,#131700,#131701,
#131702,#131703,#131704,#131705,#131706,#131707,#131708,#131709,#131710,
#131711,#131712,#131713,#131714,#131715,#131716,#131717,#131718,#131719,
#131720,#131721,#131722,#131723,#131724,#131725,#131726,#131727,#131728,
#131729,#131730,#131731,#131732,#131733,#131734,#131735,#131736,#131737,
#131738,#131739,#131740,#131741,#131742,#131743,#131744,#131745,#131746,
#131747,#131748,#131749,#131750,#131751,#131752,#131753,#131754,#131755,
#131756,#131757,#131758,#131759,#131760,#131761,#131762,#131763,#131764,
#131765,#131766,#131767,#131768,#131769,#131770,#131771,#131772,#131773,
#131774,#131775,#131776,#131777,#131778,#131779,#131780,#131781,#131782,
#131783,#131784,#131785,#131786,#131787,#131788,#131789,#131790,#131791,
#131792,#131793,#131794,#131795,#131796,#131797,#131798,#131799,#131800,
#131801,#131802,#131803,#131804,#131805,#131806,#131807,#131808,#131809,
#131810,#131811,#131812,#131813,#131814,#131815,#131816,#131817,#131818,
#131819,#131820,#131821,#131822,#131823,#131824,#131825,#131826,#131827,
#131828,#131829,#131830,#131831,#131832,#131833,#131834,#131835,#131836,
#131837,#131838,#131839,#131840,#131841,#131842,#131843,#131844,#131845,
#131846,#131847,#131848,#131849,#131850,#131851,#131852,#131853,#131854,
#131855,#131856,#131857,#131858,#131859,#131860,#131861,#131862,#131863,
#131864,#131865,#131866,#131867,#131868,#131869,#131870,#131871,#131872,
#131873,#131874,#131875,#131876,#131877,#131878,#131879,#131880,#131881,
#131882,#131883,#131884,#131885,#131886,#131887,#131888,#131889,#131890,
#131891,#131892,#131893,#131894,#131895,#131896,#131897,#131898,#131899,
#131900,#131901,#131902,#131903,#131904,#131905,#131906,#131907,#131908,
#131909,#131910,#131911,#131912,#131913,#131914,#131915,#131916,#131917,
#131918,#131919,#131920,#131921,#131922,#131923,#131924,#131925,#131926,
#131927,#131928,#131929,#131930,#131931,#131932,#131933,#131934,#131935,
#131936,#131937,#131938,#131939,#131940,#131941,#131942,#131943,#131944,
#131945,#131946,#131947,#131948,#131949,#131950,#131951,#131952,#131953,
#131954,#131955,#131956,#131957,#131958,#131959,#131960,#131961,#131962,
#131963,#131964,#131965,#131966,#131967,#131968,#131969,#131970,#131971,
#131972,#131973,#131974,#131975,#131976,#131977,#131978,#131979,#131980,
#131981,#131982,#131983,#131984,#131985,#131986,#131987,#131988,#131989,
#131990,#131991,#131992,#131993,#131994,#131995,#131996,#131997,#131998,
#131999,#132000,#132001,#132002,#132003,#132004,#132005,#132006,#132007,
#132008,#132009,#132010,#132011,#132012,#132013,#132014,#132015,#132016,
#132017,#132018,#132019,#132020,#132021,#132022,#132023,#132024,#132025,
#132026,#132027,#132028,#132029,#132030,#132031,#132032,#132033,#132034,
#132035,#132036,#132037,#132038,#132039,#132040,#132041,#132042,#132043,
#132044,#132045,#132046,#132047,#132048,#132049,#132050,#132051,#132052,
#132053,#132054,#132055,#132056,#132057,#132058,#132059,#132060,#132061,
#132062,#132063,#132064,#132065,#132066,#132067,#132068,#132069,#132070,
#132071,#132072,#132073,#132074,#132075,#132076,#132077,#132078,#132079,
#132080,#132081,#132082,#132083,#132084,#132085,#132086,#132087,#132088,
#132089,#132090,#132091,#132092,#132093,#132094,#132095,#132096,#132097,
#132098,#132099,#132100,#132101,#132102,#132103,#132104,#132105,#132106,
#132107,#132108,#132109,#132110,#132111,#132112,#132113,#132114,#132115,
#132116,#132117,#132118,#132119,#132120,#132121,#132122,#132123,#132124,
#132125,#132126,#132127,#132128,#132129,#132130,#132131,#132132,#132133,
#132134,#132135,#132136,#132137,#132138,#132139,#132140,#132141,#132142,
#132143,#132144,#132145,#132146,#132147,#132148,#132149,#132150,#132151,
#132152,#132153,#132154,#132155,#132156,#132157,#132158,#132159,#132160,
#132161,#132162,#132163,#132164,#132165,#132166,#132167,#132168,#132169,
#132170,#132171,#132172,#132173,#132174,#132175,#132176,#132177,#132178,
#132179,#132180,#132181,#132182,#132183,#132184,#132185,#132186,#132187,
#132188,#132189,#132190,#132191,#132192,#132193,#132194,#132195,#132196,
#132197,#132198,#132199,#132200,#132201,#132202,#132203,#132204,#132205,
#132206,#132207,#132208,#132209,#132210,#132211,#132212,#132213,#132214,
#132215,#132216,#132217,#132218,#132219,#132220,#132221,#132222,#132223,
#132224,#132225,#132226,#132227,#132228,#132229,#132230,#132231,#132232,
#132233,#132234,#132235,#132236,#132237,#132238,#132239,#132240,#132241,
#132242,#132243,#132244,#132245,#132246,#132247,#132248,#132249,#132250,
#132251,#132252,#132253,#132254,#132255,#132256,#132257,#132258,#132259,
#132260,#132261,#132262,#132263,#132264,#132265,#132266,#132267,#132268,
#132269,#132270,#132271,#132272,#132273,#132274,#132275,#132276,#132277,
#132278,#132279,#132280,#132281,#132282,#132283,#132284,#132285,#132286,
#132287,#132288,#132289,#132290,#132291,#132292,#132293,#132294,#132295,
#132296,#132297,#132298,#132299,#132300,#132301,#132302,#132303,#132304,
#132305,#132306,#132307,#132308,#132309,#132310,#132311,#132312,#132313,
#132314,#132315,#132316,#132317,#132318,#132319,#132320,#132321,#132322,
#132323,#132324,#132325,#132326,#132327,#132328,#132329,#132330,#132331,
#132332,#132333,#132334,#132335,#132336,#132337,#132338,#132339,#132340,
#132341,#132342,#132343,#132344,#132345,#132346,#132347,#132348,#132349,
#132350,#132351,#132352,#132353,#132354,#132355,#132356,#132357,#132358,
#132359,#132360,#132361,#132362,#132363,#132364,#132365,#132366,#132367,
#132368,#132369,#132370,#132371,#132372,#132373,#132374,#132375,#132376,
#132377,#132378,#132379,#132380,#132381,#132382,#132383,#132384,#132385,
#132386,#132387,#132388,#132389,#132390,#132391,#132392,#132393,#132394,
#132395,#132396,#132397,#132398,#132399,#132400,#132401,#132402,#132403,
#132404,#132405,#132406,#132407,#132408,#132409,#132410,#132411,#132412,
#132413,#132414,#132415,#132416,#132417,#132418,#132419,#132420,#132421,
#132422,#132423,#132424,#132425,#132426,#132427,#132428,#132429,#132430,
#132431,#132432,#132433,#132434,#132435,#132436,#132437,#132438,#132439,
#132440,#132441,#132442,#132443,#132444,#132445,#132446,#132447,#132448,
#132449,#132450,#132451,#132452,#132453,#132454,#132455,#132456,#132457,
#132458,#132459,#132460,#132461,#132462,#132463,#132464,#132465,#132466,
#132467,#132468,#132469,#132470,#132471,#132472,#132473,#132474,#132475,
#132476,#132477,#132478,#132479,#132480,#132481,#132482,#132483,#132484,
#132485,#132486,#132487,#132488,#132489,#132490,#132491,#132492,#132493,
#132494,#132495,#132496,#132497,#132498,#132499,#132500,#132501,#132502,
#132503,#132504,#132505,#132506,#132507,#132508,#132509,#132510,#132511,
#132512,#132513,#132514,#132515,#132516,#132517,#132518,#132519,#132520,
#132521,#132522,#132523,#132524,#132525,#132526,#132527,#132528,#132529,
#132530,#132531,#132532,#132533,#132534,#132535,#132536,#132537,#132538,
#132539,#132540,#132541,#132542,#132543,#132544,#132545,#132546,#132547,
#132548,#132549,#132550,#132551,#132552,#132553,#132554,#132555,#132556,
#132557,#132558,#132559,#132560,#132561,#132562,#132563,#132564,#132565,
#132566,#132567,#132568,#132569,#132570,#132571,#132572,#132573,#132574,
#132575,#132576,#132577,#132578,#132579,#132580,#132581,#132582,#132583,
#132584,#132585,#132586,#132587,#132588,#132589,#132590,#132591,#132592,
#132593,#132594,#132595,#132596,#132597,#132598,#132599,#132600,#132601,
#132602,#132603,#132604,#132605,#132606,#132607,#132608,#132609,#132610,
#132611,#132612,#132613,#132614,#132615,#132616,#132617,#132618,#132619,
#132620,#132621,#132622,#132623,#132624,#132625,#132626,#132627,#132628,
#132629,#132630,#132631,#132632,#132633,#132634,#132635,#132636,#132637,
#132638,#132639,#132640,#132641,#132642,#132643,#132644,#132645,#132646,
#132647,#132648,#132649,#132650,#132651,#132652,#132653,#132654,#132655,
#132656,#132657,#132658,#132659,#132660,#132661,#132662,#132663,#132664,
#132665,#132666,#132667,#132668,#132669,#132670,#132671,#132672,#132673,
#132674,#132675,#132676,#132677,#132678,#132679,#132680,#132681,#132682,
#132683,#132684,#132685,#132686,#132687,#132688,#132689,#132690,#132691,
#132692,#132693,#132694,#132695,#132696,#132697,#132698,#132699,#132700,
#132701,#132702,#132703,#132704,#132705,#132706,#132707,#132708,#132709,
#132710,#132711,#132712,#132713,#132714,#132715,#132716,#132717,#132718,
#132719,#132720,#132721,#132722,#132723,#132724,#132725,#132726,#132727,
#132728,#132729,#132730,#132731,#132732,#132733,#132734,#132735,#132736,
#132737,#132738,#132739,#132740,#132741,#132742,#132743,#132744,#132745,
#132746,#132747,#132748,#132749,#132750,#132751,#132752,#132753,#132754,
#132755,#132756,#132757,#132758,#132759,#132760,#132761,#132762,#132763,
#132764,#132765,#132766,#132767,#132768,#132769,#132770,#132771,#132772,
#132773,#132774,#132775,#132776,#132777,#132778,#132779,#132780,#132781,
#132782,#132783,#132784,#132785,#132786,#132787,#132788,#132789,#132790,
#132791,#132792,#132793,#132794,#132795,#132796,#132797,#132798,#132799,
#132800,#132801,#132802,#132803,#132804,#132805,#132806,#132807,#132808,
#132809,#132810,#132811,#132812,#132813,#132814,#132815,#132816,#132817,
#132818,#132819,#132820,#132821,#132822,#132823,#132824,#132825,#132826,
#132827,#132828,#132829,#132830,#132831,#132832,#132833,#132834,#132835,
#132836,#132837,#132838)),.UNSPECIFIED.,.T.,.F.,.F.)
B_SPLINE_SURFACE_WITH_KNOTS((3,2,2,2,3),(4,1,1,1,1,1,1,1,1,1,1,1,1,1,1,
1,1,1,1,1,1,1,1,1,1,1,1,1,1,1,1,1,1,1,1,1,1,1,1,1,1,1,1,1,1,1,1,1,1,1,1,
1,1,1,1,1,1,1,1,1,1,1,1,1,1,1,1,1,1,1,1,1,1,1,1,1,1,1,1,1,1,1,1,1,1,1,1,
1,1,1,1,1,1,1,1,1,1,1,1,1,1,1,1,1,1,1,1,1,1,1,1,1,1,1,1,1,1,1,1,1,1,1,1,
1,1,1,1,1,1,1,1,1,1,1,1,1,1,1,1,1,1,1,1,1,1,1,1,1,1,1,1,1,1,1,1,1,1,1,1,
1,1,1,1,1,1,1,1,1,1,1,1,1,1,1,1,1,1,1,1,1,1,1,1,1,1,1,1,1,1,1,1,1,1,1,1,
1,1,1,1,1,1,1,1,1,1,1,1,1,1,1,1,1,1,1,1,1,1,1,1,1,1,1,1,1,1,1,1,1,1,1,1,
1,1,1,1,1,1,1,1,1,1,1,1,1,1,1,1,1,1,1,1,1,1,1,1,1,1,1,1,1,1,1,1,1,1,1,1,
1,1,1,1,1,1,1,1,1,1,1,1,1,1,1,1,1,1,1,1,1,1,1,1,1,1,1,1,1,1,1,1,1,1,1,1,
1,1,1,1,1,1,1,1,1,1,1,1,1,1,1,1,1,1,1,1,1,1,1,1,1,1,1,1,1,1,1,1,1,1,1,1,
1,1,1,1,1,1,1,1,1,1,1,1,1,1,1,1,1,1,1,1,1,1,1,1,1,1,1,1,1,1,1,1,1,1,1,1,
1,1,1,1,1,1,1,1,1,1,1,1,1,1,1,1,1,1,1,1,1,1,1,1,1,1,1,1,1,1,1,1,1,1,1,1,
1,1,1,1,1,1,1,1,1,1,1,1,1,1,1,1,1,1,1,1,1,1,1,1,1,1,1,1,1,1,1,1,1,1,1,1,
1,1,1,1,1,1,1,1,1,1,1,1,1,1,1,1,1,1,1,1,1,1,1,1,1,1,1,1,1,1,1,1,1,1,1,1,
1,1,1,1,1,1,1,1,1,1,1,1,1,1,1,1,1,1,1,1,1,1,1,1,1,1,1,1,1,1,1,1,1,1,1,1,
1,1,1,1,1,1,1,1,1,1,1,1,1,1,1,1,1,1,1,1,1,1,1,1,1,1,1,1,1,1,1,1,1,1,1,1,
1,1,1,1,1,1,1,1,1,1,1,1,1,1,1,1,1,1,1,1,1,1,1,1,1,1,1,1,1,1,1,1,1,1,1,1,
1,1,1,1,1,1,1,1,1,1,1,1,1,1,1,1,1,1,1,1,1,1,1,1,1,1,1,1,1,1,1,1,1,1,1,1,
1,1,1,1,1,1,1,1,1,1,1,1,1,1,1,1,1,1,1,1,1,1,1,1,1,1,1,1,1,1,1,1,1,1,1,1,
1,1,1,1,1,1,1,1,1,1,1,1,1,1,1,1,1,1,1,1,1,1,1,1,1,1,1,1,1,1,1,1,1,1,1,1,
1,1,1,1,1,1,1,1,1,1,1,1,1,1,1,1,1,1,1,1,1,1,1,1,1,1,1,1,1,1,1,1,1,1,1,1,
1,1,1,1,1,1,1,1,1,1,1,1,1,1,1,1,1,1,1,1,1,1,1,1,1,1,1,1,1,1,1,1,1,1,1,1,
1,1,1,1,1,1,1,1,1,1,1,1,1,1,1,1,1,1,1,1,1,1,1,1,1,1,1,1,1,1,1,1,1,1,1,1,
1,1,1,1,1,1,1,1,1,1,1,1,1,1,1,1,1,1,1,1,1,1,1,1,1,1,1,1,1,1,1,1,1,1,1,1,
1,1,1,1,1,1,1,1,1,1,1,1,1,1,1,1,1,1,1,1,1,1,1,1,1,1,1,1,1,1,1,1,1,1,1,1,
1,1,1,1,1,1,1,1,1,1,1,1,1,1,1,1,1,1,1,1,1,1,1,1,1,1,1,1,1,1,1,1,1,1,1,1,
1,1,1,1,1,1,1,1,1,1,1,1,1,1,1,1,1,1,1,1,1,1,1,1,1,1,1,1,1,1,1,1,1,1,1,1,
1,1,1,1,1,1,1,1,1,1,1,1,1,1,1,1,1,1,1,1,1,1,1,1,1,1,1,1,1,1,1,1,1,1,1,1,
1,1,1,1,1,1,1,1,1,1,1,1,1,1,1,1,1,1,1,1,1,1,1,1,1,1,1,1,1,1,1,1,1,1,1,1,
1,1,1,1,1,1,1,1,1,1,1,1,1,1,1,1,1,1,1,1,1,1,1,1,1,1,1,1,1,1,1,1,1,1,1,1,
1,1,1,1,1,1,1,1,1,1,1,1,1,1,1,1,1,1,1,1,1,1,1,1,1,1,1,1,1,1,1,1,1,1,1,1,
1,1,1,1,1,1,1,1,1,1,1,1,1,1,1,1,1,1,1,1,1,1,1,1,1,1,1,1,1,1,1,1,1,1,1,1,
1,1,1,1,1,1,1,1,1,1,1,1,1,1,1,1,1,1,1,1,1,1,1,1,1,1,1,1,1,1,1,1,1,1,1,1,
1,1,1,1,1,1,1,1,1,1,1,1,1,1,1,1,1,1,1,1,1,1,1,1,1,1,1,1,1,1,1,1,1,1,1,1,
1,1,1,1,1,1,1,1,1,1,1,1,1,1,1,1,1,1,1,1,1,1,1,1,1,1,1,1,1,1,1,1,1,1,1,1,
1,1,1,1,1,1,1,1,1,1,1,1,1,1,1,1,1,1,1,1,1,1,1,1,1,1,1,1,1,1,1,1,1,1,1,1,
1,1,1,1,1,1,1,1,1,1,1,1,1,1,1,1,1,1,1,1,1,1,1,1,1,1,1,1,1,1,1,1,1,1,1,1,
1,1,1,1,1,1,1,1,1,1,1,1,1,1,1,1,1,1,1,1,1,1,1,1,1,1,1,1,1,1,1,1,1,1,1,1,
1,1,1,1,1,1,1,1,1,1,1,1,1,1,1,1,1,1,1,1,1,1,1,1,1,1,1,1,1,1,1,1,1,1,1,1,
1,1,1,1,1,1,1,1,1,1,1,1,1,1,1,1,1,1,1,1,1,1,1,1,1,1,1,1,1,1,1,1,1,1,1,1,
1,1,1,1,1,1,1,1,1,1,1,1,1,1,1,1,1,1,1,1,1,1,1,1,1,1,1,1,1,1,1,1,1,1,1,1,
1,1,1,1,1,1,1,1,1,1,1,1,1,1,1,1,1,1,1,1,1,1,1,1,1,1,1,1,1,1,1,1,1,1,1,1,
1,1,1,1,1,1,1,1,1,1,1,1,1,1,1,1,1,1,1,1,1,1,1,1,1,1,1,1,1,1,1,1,1,1,1,1,
1,1,1,1,1,1,1,1,1,1,1,1,1,1,1,1,1,1,1,1,1,1,1,1,1,1,1,1,1,1,1,1,1,1,1,1,
1,1,1,1,1,1,1,1,1,1,1,1,1,1,1,1,1,1,1,1,1,1,1,1,1,1,1,1,1,1,1,1,1,1,1,1,
1,1,1,1,1,1,1,1,1,1,1,1,1,1,1,1,1,1,1,1,1,1,1,1,1,1,1,1,1,1,1,1,1,1,1,1,
1,1,1,1,1,1,1,1,1,1,1,1,1,1,1,1,1,1,1,1,1,1,1,1,1,1,1,1,1,1,1,1,1,1,1,1,
1,1,1,1,1,1,1,1,1,1,1,1,1,1,1,1,1,1,1,1,1,1,1,1,1,1,1,1,1,1,1,1,1,1,1,1,
1,1,1,1,1,1,1,1,1,1,1,1,1,1,1,1,1,1,1,1,1,1,1,1,1,1,1,1,1,1,1,1,1,1,1,1,
1,1,1,1,1,1,1,1,1,1,1,1,1,1,1,1,1,1,1,1,1,1,1,1,1,1,1,1,1,1,1,1,1,1,1,1,
1,1,1,1,1,1,1,1,1,1,1,1,1,1,1,1,1,1,1,1,1,1,1,1,1,1,1,1,1,1,1,1,1,1,1,1,
1,1,1,1,1,1,1,1,1,1,1,1,1,1,1,1,1,1,1,1,1,1,1,1,1,1,1,1,1,1,1,1,1,1,1,1,
1,1,1,1,1,1,1,1,1,1,1,1,1,1,1,1,1,1,1,1,1,1,1,1,1,1,1,1,1,1,1,1,1,1,1,1,
1,1,1,1,1,1,1,1,1,1,1,1,1,1,1,1,1,1,1,1,1,1,1,1,1,1,1,1,1,1,1,1,1,1,1,1,
1,1,1,1,1,1,1,1,1,1,1,1,1,1,1,1,1,1,1,1,1,1,1,1,1,1,1,1,1,1,1,1,1,1,1,1,
1,1,1,1,1,1,1,1,1,1,1,1,1,1,1,1,1,1,1,1,1,1,1,1,1,1,1,1,1,1,1,1,1,1,1,1,
1,1,1,1,1,1,1,1,1,1,1,1,1,1,1,1,1,1,1,1,1,1,1,1,1,1,1,1,1,1,1,1,1,1,1,1,
1,1,1,1,1,1,1,1,1,1,1,1,1,1,1,1,1,4),(0.,0.117809724509617,0.235619449019234,
0.353429173528852,0.471238898038469),(0.,0.01797683372391,0.286633051710584,
0.555289278308216,0.823945516665782,1.09260176953922,1.36125803873948,1.62991432588463,
1.89857063164012,2.16722695661301,2.43588330050525,2.70453966304674,2.9731960431531,
3.24185243981471,3.51050885133453,3.77916527610465,4.04782171198515,4.31647815691489,
4.58513460847725,4.85379106430677,5.12244752187208,5.39110397865606,5.65976043217153,
5.92841687990537,6.19707331956994,6.46572974881596,6.73438616570634,7.00304256821933,
7.2716989549161,7.5403553242696,7.809011675483,8.07766800769526,8.34632432089157,
8.61498061505147,8.8836368910788,9.15229314997201,9.4209493936865,9.68960562442157,
9.95826184531348,10.226918059948,10.4955742727586,10.7642304884925,11.0328867113173,
11.3015429448574,11.5701991918227,11.8388554546081,12.1075117346518,12.3761680332469,
12.6448243507434,12.9134806874637,13.1821370428496,13.450793416388,13.7194498067883,
13.9881062128412,14.2567626326955,14.5254190645885,14.7940755062772,15.0627319555912,
15.3313884100611,15.6000448672586,15.8687013246492,16.1373577797,16.4060142299691,
16.6746706729765,16.9433271065265,17.2119835283531,17.4806399366567,17.7492963295502,
18.0179527057767,18.286609063996,18.555265403637,18.8239217240786,19.0925780255742,
19.3612343083975,19.6298905737625,19.898546823017,20.1672030584666,20.4358592827168,
20.7045154992928,20.973171712245,21.2418279262962,21.5104841459723,21.7791403749736,
22.0477966165324,22.316452872948,22.585109146262,22.8537654375589,23.1224217478187,
23.3910780770929,23.6597344254327,23.9283907920352,24.197047176159,24.4657035763222,
24.7343599911301,25.0030164185931,25.2716728568073,25.5403293034427,25.8089857562333,
26.0776422126729,26.3462986702843,26.6149551265448,26.8836115789212,27.1522680250308,
27.4209244624423,27.6895808890659,27.9582373027346,28.2268937018004,28.4955500845261,
28.7642064498512,29.0328627966379,29.3015191245544,29.5701754332357,29.838831723217,
30.1074879950829,30.3761442503694,30.6448004907916,30.9134567190168,31.1821129380756,
31.450769151893,31.7194253649682,31.9880815819663,32.2567378070174,32.5253940433706,
32.7940502938785,33.0627065604467,33.3313628447765,33.6000191476151,33.8686754696427,
34.1373318106287,34.405988170366,34.6746445478242,34.9433009420458,35.2119573513747,
35.480613774244,35.7492702085419,36.0179266522368,36.2865831029275,36.5552395582669,
36.8238960157264,37.0925524727952,37.3612089269773,37.6298653757534,37.8985218168153,
38.1671782477952,38.4358346667239,38.7044910715485,38.9731474607866,39.2418038328672,
39.5104601869391,39.7791165220837,40.0477728382212,40.3164291352602,40.5850854140292,
40.8537416754418,41.1223979213679,41.3910541539077,41.6597103761025,41.9283665914244,
42.1970228042084,42.4656790192,42.7343352406829,43.0029914723808,43.2716477171096,
43.540303977354,43.8089602546436,44.0776165503516,44.3462728649052,44.614929198697,
44.883585551232,45.1522419220568,45.4208983099307,45.6895547136931,45.9582111315299,
46.2268675617156,46.4955240020317,46.7641804503338,47.0328369041642,47.3014933611089,
47.5701498186329,47.8388062742058,48.107462725373,48.3761191696448,48.6447756048012,
48.9134320285537,49.1820884390673,49.4507448344197,49.7194012133072,49.9880575743413,
50.2567139168934,50.5253702402807,50.7940265446884,51.0626828303152,51.3313390982961,
51.5999953498901,51.8686515873141,52.1373078130706,52.4059640305862,52.6746202437936,
52.9432764573682,53.211932675918,53.480588903259,53.7492451427202,54.0179013967021,
54.2865576673334,54.5552139557853,54.823870263115,55.0925265894471,55.3611829348992,
55.6298392987282,55.8984956802486,56.1671520780245,56.4358084907065,56.7044649163381,
56.9731213530494,57.2417777985307,57.5104342505384,57.7790907065743,58.0477471641719,
58.3164036208043,58.5850600739368,58.8537165211707,59.1223729600609,59.39102938849,
59.6596858042645,59.9283422056975,60.1969985910129,60.4656549590995,60.7343113087676,
61.0029676396243,61.2716239512389,61.540280244075,61.808936518638,62.0775927763821,
62.3462490189291,62.6149052488546,62.8835614690812,63.1522176834332,63.4208738963055,
63.6895301124163,63.9581863359981,64.2268425704115,64.4954988186027,64.7641550825741,
65.0328113641112,65.3014676640435,65.5701239831253,65.8387803211949,66.1074366781083,
66.3760930528907,66.6447494446373,66.9134058517341,67.1820622726558,67.4507187053199,
67.7193751477252,67.988031597487,68.256688052277,68.5253445095709,68.7940009668648,
69.0626574216546,69.3313138714164,69.5999703138218,69.8686267464858,70.1372831674076,
70.4059395745042,70.6745959662509,70.9432523410334,71.2119086979469,71.4805650360164,
71.7492213550982,72.0178776550306,72.2865339365675,72.5551902005389,72.8238464487301,
73.0925026831433,73.3611589067251,73.6298151228357,73.8984713357081,74.1671275500599,
74.4357837702864,74.7044400002118,74.9730962427587,75.2417525005027,75.5104087750655,
75.7790650679015,76.047721379516,76.3163777103726,76.5850340600405,76.853690428127,
77.1223468134422,77.391003214875,77.6596596306495,77.9283160590784,78.1969724979684,
78.4656289452021,78.7342853983344,79.0029418549666,79.2715983125641,79.5402547685998,
79.8089112206075,80.0775676660886,80.3462241027997,80.6148805284312,80.8835369411131,
81.1521933388889,81.4208497204091,81.689506084238,81.9581624296899,82.2268187560219,
82.4954750633515,82.7641313518033,83.0327876224345,83.3014438764161,83.5701001158772,
83.838756343218,84.1074125617677,84.3760687753422,84.6447249885494,84.913381206065,
85.1820374318212,85.4506936692451,85.719349920839,85.9880061888197,86.2566624744465,
86.5253187788541,86.7939751022413,87.0626314447932,87.3312878058273,87.5999441847146,
87.8686005800667,88.1372569905802,88.4059134143327,88.6745698494889,88.9432262937606,
89.2118827449277,89.4805392005005,89.7491956580243,90.0178521149689,90.2865085687992,
90.5551650171012,90.8238214574172,91.0924778876028,91.3611343054394,91.6297907092016,
91.8984470970753,92.1671034679,92.4357598204347,92.7044161542264,92.9730724687798,
93.2417287644878,93.5103850417773,93.7790413020216,94.0476975467502,94.3163537784479,
94.5850099999307,94.8536662149221,95.1223224277061,95.390978643028,95.6596348652226,
95.9282910977624,96.1969473436883,96.4656036051009,96.7342598838697,97.0029161809086,
97.2715724970461,97.5402288321905,97.8088851862623,98.0775415583427,98.3461979475807,
98.6148543524051,98.8835107713336,99.1521672023136,99.4208236433754,99.6894800921513,
99.9581365463333,100.226793003402,100.495449460861,100.7641059162,101.032762366891,
101.301418810586,101.570075244884,101.838731667753,102.107388077082,102.376044471303,
102.644700848761,102.913357208498,103.182013549484,103.450669871511,103.71932617435,
103.98798245868,104.256638725248,104.525294975755,104.793951212108,105.062607437159,
105.331263654157,105.599919867233,105.86857608105,106.137232300108,106.405888528334,
106.674544768756,106.943201024042,107.211857295908,107.480513585889,107.74916989457,
108.017826222487,108.286482569273,108.555138934598,108.823795317324,109.09245171639,
109.361108130058,109.629764556682,109.898420994093,110.167077440202,110.435733892579,
110.704390348839,110.97304680645,111.24170326289,111.51035971568,111.779016162316,
112.04767260053,112.316329027993,112.5849854428,112.853641842963,113.122298227087,
113.39095459369,113.659610942029,113.928267271303,114.196923581563,114.46557987286,
114.734236146174,115.002892402589,115.271548644148,115.540204873149,115.808861092825,
116.077517306876,116.346173519828,116.614829736404,116.883485960654,117.152142196103,
117.420798445358,117.689454710722,117.958110993546,118.226767295041,118.495423615483,
118.764079955123,119.032736313343,119.301392689569,119.570049082462,119.838705490766,
120.107361912592,120.376018346142,120.644674789149,120.913331239418,121.181987694469,
121.45064415186,121.719300609057,121.987957063527,122.256613512841,122.525269954529,
122.793926386422,123.062582806276,123.331239212329,123.599895602729,123.868551976268,
124.137208331653,124.405864668374,124.67452098587,124.943177284465,125.211833564508,
125.480489827294,125.749146074259,126.017802307799,126.286458530624,126.555114746357,
126.823770959168,127.092427173802,127.361083394694,127.629739625429,127.898395869143,
128.167052128037,128.435708404064,128.704364698224,128.97302101142,129.241677343633,
129.510333694846,129.7789900642,130.047646450897,130.31630285341,130.5849592703,
130.853615699547,131.122272139211,131.390928586945,131.659585040461,131.928241497245,
132.19689795481,132.46555441064,132.734210862202,133.002867307132,133.271523743013,
133.540180167783,133.808836579303,134.077492975965,134.346149356071,134.614805718613,
134.883462062505,135.152118387478,135.420774693234,135.689430980379,135.958087249579,
136.226743502453,136.49539974081,136.76405596741,137.032712185392,137.301368398783,
137.570024612174,137.838680830155,138.107337056755,138.375993295112,138.644649547986,
138.913305817186,139.181962104332,139.450618410087,139.71927473506,139.987931078952,
140.256587441494,140.525243821601,140.793900218262,141.062556629782,141.331213054552,
141.599869490433,141.868525935363,142.137182386925,142.405838842755,142.67449530032,
142.943151757104,143.21180821062,143.480464658354,143.749121098019,144.017777527265,
144.286433944155,144.555090346668,144.823746733365,145.092403102719,145.361059453932,
145.629715786145,145.898372099341,146.167028393501,146.435684669529,146.704340928422,
146.972997172137,147.241653402872,147.510309623764,147.778965838398,148.047622051209,
148.316278266943,148.584934489768,148.853590723308,149.122246970274,149.390903233059,
149.659559513103,149.928215811698,150.196872129195,150.465528465915,150.734184821301,
151.00284119484,151.27149758524,151.540153991293,151.808810411148,152.077466843041,
152.34612328473,152.614779734044,152.883436188514,153.152092645711,153.420749103102,
153.689405558153,153.958062008422,154.22671845143,154.49537488498,154.764031306806,
155.03268771511,155.301344108004,155.57000048423,155.838656842449,156.107313182091,
156.375969502532,156.644625804028,156.913282086851,157.181938352216,157.450594601471,
157.719250836921,157.987907061171,158.256563277747,158.525219490699,158.793875704751,
159.062531924427,159.331188153428,159.599844394987,159.868500651403,160.137156924717,
160.405813216014,160.674469526274,160.943125855548,161.211782203888,161.480438570491,
161.749094954615,162.017751354778,162.286407769586,162.555064197049,162.823720635263,
163.092377081899,163.361033534689,163.629689991129,163.898346448741,164.167002905001,
164.435659357378,164.704315803488,164.972972240899,165.241628667523,165.510285081192,
165.778941480257,166.047597862983,166.316254228308,166.584910575095,166.853566903012,
167.122223211693,167.390879501675,167.659535773541,167.928192028827,168.19684826925,
168.465504497475,168.734160716534,169.002816930351,169.271473143427,169.540129360425,
169.808785585476,170.077441821829,170.346098072337,170.614754338905,170.883410623235,
171.152066926074,171.420723248102,171.689379589088,171.958035948825,172.226692326284,
172.495348720505,172.764005129834,173.032661552704,173.301317987002,173.569974430697,
173.838630881388,174.107287336727,174.375943794187,174.644600251255,174.913256705437,
175.181913154214,175.450569595276,175.719226026256,175.987882445184,176.256538850009,
176.525195239247,176.793851611328,177.0625079654,177.331164300545,177.599820616682,
177.868476913721,178.137133192491,178.405789453903,178.674445699829,178.943101932369,
179.211758154564,179.480414369886,179.74907058267,180.017726797662,180.286383019145,
180.555039250843,180.823695495572,181.092351755816,181.361008033106,181.629664328814,
181.898320643368,182.16697697716,182.435633329695,182.70428970052,182.972946088394,
183.241602492156,183.510258909993,183.778915340179,184.047571780495,184.316228228797,
184.584884682628,184.853541139572,185.122197597096,185.39085405267,185.659510503837,
185.928166948109,186.196823383265,186.465479807018,186.734136217531,187.002792612884,
187.271448991771,187.540105352806,187.808761695358,188.077418018745,188.346074323153,
188.61473060878,188.883386876761,189.152043128355,189.420699365779,189.689355591536,
189.958011809051,190.226668022259,190.495324235834,190.763980454383,191.032636681725,
191.301292921186,191.569949175168,191.838605445799,192.107261734251,192.375918041581,
192.644574367913,192.913230713365,193.181887077194,193.450543458715,193.719199856491,
193.987856269173,194.256512694805,194.525169131516,194.793825576997,195.062482029005,
195.331138485041,195.599794942639,195.868451399271,196.137107852404,196.405764299638,
196.674420738528,196.943077166957,197.211733582732,197.480389984165,197.749046369481,
198.017702737567,198.286359087236,198.555015418092,198.823671729707,199.092328022543,
199.360984297106,199.62964055485,199.898296797397,200.166953027323,200.43560924755,
200.704265461902,200.972921674774,201.241577890885,201.510234114467,201.77889034888,
202.047546597072,202.316202861043,202.584859142581,202.853515442513,203.122171761595,
203.390828099665,203.659484456579,203.928140831361,204.196797223108,204.465453630205,
204.734110051127,205.002766483791,205.271422926197,205.540079375959,205.808735830749,
206.077392288043,206.346048745337,206.614705200127,206.883361649889,207.152018092295,
207.420674524959,207.689330945881,207.957987352978,208.226643744725,208.495300119508,
208.763956476421,209.032612814491,209.301269133573,209.569925433505,209.838581715043,
210.107237979014,210.375894227206,210.644550461619,210.913206685201,211.181862901312,
211.450519114184,211.719175328536,211.987831548763,212.256487778689,212.525144021236,
212.79380027898,213.062456553543,213.331112846379,213.599769157994,213.868425488851,
214.137081838519,214.405738206606,214.674394591921,214.943050993354,215.211707409129,
215.480363837558,215.749020276448,216.017676723682,216.286333176815,216.554989633447,
216.823646091045,217.092302547081,217.360958999089,217.62961544457,217.898271881281,
218.166928306913,218.435584719595,218.704241117371,218.972897498892,219.241553862721,
219.510210208173,219.778866534505,220.047522841835,220.316179130287,220.584835400918,
220.8534916549,221.122147894361,221.390804121702,221.659460340252,221.928116553827,
222.196772767034,222.46542898455,222.734085210306,223.00274144773,223.271397699324,
223.540053967305,223.808710252932,224.07736655734,224.346022880728,224.61467922328,
224.883335584314,225.151991963201,225.420648358554,225.689304769068,225.95796119282,
226.226617627977,226.495274072249,226.763930523416,227.032586978989,227.301243436513,
227.569899893458,227.838556347288,228.10721279559,228.375869235907,228.644525666093,
228.913182083929,229.181838487692,229.450494875566,229.719151246391,229.987807598926,
230.256463932718,230.525120247271,230.79377654298,231.062432820269,231.331089080514,
231.599745325243,231.868401556941,232.137057778424,232.405713993415,232.674370206199,
232.943026421521,233.211682643716,233.480338876256,233.748995122182,234.017651383595,
234.286307662364,234.554963959403,234.823620275541,235.092276610685,235.360932964757,
235.629589336838,235.898245726076,236.166902130901,236.43555854983,236.70421498081,
236.972871421872,237.241527870648,237.51018432483,237.778840781899,238.047497239359,
238.316153694698,238.584810145389,238.853466589084,239.122123023382,239.390779446251,
239.65943585558,239.928092249802,240.19674862726,240.465404986998,240.734061327984,
241.002717650011,241.27137395285,241.54003023718,241.808686503748,242.077342754256,
242.345998990609,242.614655215661,242.883311432659,243.151967645734,243.420623859552,
243.68928007861,243.957936306836,244.226592547258,244.495248802545,244.763905074411,
245.032561364392,245.301217673074,245.56987400099,245.838530347777,246.107186713102,
246.375843095828,246.644499494894,246.913155908563,247.181812335186,247.450468772598,
247.719125218708,247.987781671084,248.256438127345,248.525094584956,248.793751041396,
249.062407494187,249.331063940822,249.599720379036,249.8683768065,250.137033221308,
250.405689621471,250.674346005595,250.943002372197,251.211658720537,251.480315049812,
251.748971360071,252.017627651368,252.286283924683,252.554940181098,252.823596422657,
253.092252651658,253.360908871335,253.629565085386,253.898221298338,254.166877514914,
254.435533739165,254.704189974614,254.972846223869,255.241502489234,255.510158772057,
255.778815073553,256.047471393995,256.316127733635,256.584784091854,256.85344046808,
257.122096860973,257.390753269276,257.659409691102,257.928066124652,258.196722567659,
258.465379017928,258.734035472978,259.002691930368,259.271348387566,259.540004842035,
259.808661291349,260.077317733037,260.345974164929,260.614630584783,260.883286990836,
261.151943381235,261.420599754774,261.689256110159,261.957912446879,262.226568764375,
262.49522506297,262.763881343014,263.032537605798,263.301193852763,263.569850086303,
263.838506309127,264.107162524861,264.375818737671,264.644474952305,264.913131173196,
265.181787403931,265.450443647645,265.719099906538,265.987756182565,266.256412476724,
266.52506878992,266.793725122132,267.062381473345,267.331037842698,267.599694229394,
267.868350631907,268.137007048797,268.405663478042,268.674319917706,268.94297636544,
269.211632818955,269.480289275739,269.748945733304,270.017602189133,270.286258640695,
270.554915085624,270.823571521504,271.092227946274,271.360884357793,271.629540754454,
271.89819713456,272.166853497101,272.435509840993,272.704166165965,272.97282247172,
273.241478758865,273.510135028065,273.778791280938,274.047447519295,274.316103745894,
274.584759963875,274.853416177266,275.122072390656,275.390728608637,275.659384835237,
275.928041073593,276.196697326466,276.465353595666,276.734009882811,277.002666188566,
277.271322513539,277.53997885743,277.808635219972,278.077291600077,278.345947996739,
278.614604408258,278.883260833028,279.151917268908,279.420573713837,279.689230165399,
279.957886621228,280.226543078793,280.495199535576,280.763855989092,281.032512436825,
281.301168876489,281.569825305735,281.838481722625,282.107138125138,282.375794511834,
282.644450881187,282.9131072324,283.181763564612,283.450419877808,283.719076171967,
283.987732447994,284.256388706887,284.525044950601,284.793701181336,285.062357402228,
285.331013616862,285.599669829672,285.868326045405,286.136982268229,286.405638501769,
286.674294748734,286.942951011519,287.211607291562,287.480263590157,287.748919907653,
288.017576244373,288.286232599758,288.554888973296,288.823545363696,289.092201769749,
289.360858189603,289.629514621495,289.898171063183,290.166827512497,290.435483966966,
290.704140424163,290.972796881554,291.241453336604,291.510109786873,291.77876622988,
292.047422663429,292.316079085255,292.584735493559,292.853391886452,293.122048262678,
293.390704620897,293.659360960537,293.928017280978,294.196673582474,294.465329865297,
294.733986130661,295.002642379915,295.271298615364,295.539954839614,295.808611056189,
296.077267269141,296.345923483192,296.614579702867,296.883235931868,297.151892173427,
297.420548429842,297.689204703155,297.957860994452,298.226517304711,298.495173633985,
298.763829982324,299.032486348927,299.30114273305,299.569799133212,299.83845554802,
300.107111975482,300.375768413696,300.644424860331,300.913081313121,301.181737769561,
301.450394227172,301.719050683432,301.987707135808,302.256363581917,302.525020019328,
302.793676445951,303.062332859619,303.330989258684,303.59964564141,303.868302006734,
304.136958353521,304.405614681437,304.674270990118,304.942927280098,305.211583551964,
305.48023980725,305.748896047671,306.017552275896,306.286208494954,306.554864708772,
306.823520921846,307.092177138844,307.360833363895,307.629489600247,307.898145850755,
308.166802117323,308.435458401652,308.70411470449,308.972771026517,309.241427367503,
309.51008372724,309.778740104698,310.047396498919,310.316052908247,310.584709331116,
310.853365765414,311.122022209108,311.390678659798,311.659335115137,311.927991572596,
312.196648029665,312.465304483846,312.733960932622,313.002617373684,313.271273804663,
313.539930223591,313.808586628416,314.077243017653,314.345899389733,314.614555743805,
314.883212078949,315.151868395086,315.420524692125,315.689180970894,315.957837232306,
316.226493478231,316.495149710771,316.763805932965,317.032462148286,317.30111836107,
317.569774576061,317.838430797543,318.107087029241,318.375743273969,318.644399534213,
318.913055811502,319.18171210721,319.450368421763,319.719024755555,319.987681108089,
320.256337478914,320.524993866787,320.793650270549,321.062306688385,321.33096311857,
321.599619558886,321.868276007188,322.136932461018,322.405588917962,322.674245375486,
322.942901831059,323.211558282225,323.480214726497,323.748871161653,324.017527585405,
324.286183995918,324.55484039127,324.823496770157,325.09215313119,325.360809473742,
325.629465797129,325.898122101536,326.166778387163,326.435434655143,326.704090906737,
326.97274714416,327.241403369916,327.510059587432,327.778715800638,328.047372014213,
328.316028232762,328.584684460102,328.853340699563,329.121996953545,329.390653224175,
329.659309512627,329.927965819956,330.196622146288,330.46527849174,330.733934855568,
331.002591237088,331.271247634863,331.539904047545,331.808560473176,332.077216909887,
332.345873355368,332.614529807375,332.883186263411,333.151842721008,333.42049917764,
333.689155630772,333.957812078005,334.226468516895,334.495124945324,334.763781361098,
335.03243776253,335.301094147845,335.569750515931,335.838406865599,336.107063196455,
336.375719508069,336.644375800905,336.913032075468,337.181688333211,337.450344575758,
337.719000805683,337.987657025909,338.256313240261,338.524969453133,338.793625669243,
339.062281892824,339.330938127237,339.599594375428,339.868250639399,340.136906920936,
340.405563220868,340.674219539949,340.942875878019,341.211532234932,341.480188609714,
341.74884500146,342.017501408557,342.286157829478,342.554814262142,342.823470704547,
343.092127154308,343.360783609098,343.629440066391,343.898096523685,344.166752978475,
344.435409428236,344.704065870641,344.972722303305,345.241378724226,345.510035131323,
345.778691523069,346.047347897851,346.316004254764,346.584660592834,346.853316911915,
347.121973211847,347.390629493384,347.659285757355,347.927942005546,348.196598239959,
348.46525446354,348.733910679651,349.002566892523,349.271223106874,349.5398793271,
349.808535557025,350.077191799572,350.345848057315,350.614504331878,350.883160624714,
351.151816936328,351.420473267184,351.689129616852,351.957785984938,352.226442370253,
352.495098771685,352.76375518746,353.032411615888,353.301068054778,353.569724502012,
353.838380955144,354.107037411776,354.375693869373,354.644350325408,354.913006777416,
355.181663222896,355.450319659607,355.718976085238,355.98763249792,356.256288895695,
356.524945277215,356.793601641044,357.062257986496,357.330914312827,357.599570620156,
357.868226908608,358.136883179239,358.40553943322,358.674195672681,358.942851900021,
359.211508118571,359.480164332145,359.748820545352,360.017476762867,360.286132988623,
360.554789226047,360.82344547764,361.09210174562,361.360758031247,361.629414335654,
361.898070659041,362.166727001593,362.435383362626,362.704039741513,362.972696136865,
363.241352547378,363.510008971131,363.778665406287,364.047321850558,364.315978301725,
364.584634757297,364.853291214821,365.121947671765,365.390604125595,365.659260573897,
365.927917014213,366.196573444398,366.465229862234,366.733886265996,367.002542653869,
367.271199024694,367.539855377228,367.808511711019,368.077168025573,368.34582432128,
368.614480598569,368.883136858813,369.151793103542,369.420449335239,369.689105556722,
369.957761771713,370.226417984496,370.495074199818,370.763730422012,371.032386654551,
371.301042900477,371.569699161889,371.838355440658,372.107011737697,372.375668053834,
372.644324388978,372.912980743049,373.18163711513,373.450293504367,373.718949909191,
373.98760632812,374.256262759099,374.524919200161,374.793575648936,375.062232103118,
375.330888560186,375.599545017646,375.868201472985,376.136857923675,376.40551436737,
376.674170801667,376.942827224536,377.211483633864,377.480140028085,377.748796405543,
378.01745276528,378.286109106266,378.554765428293,378.823421731131,379.092078015461,
379.360734282028,379.629390532536,379.898046768888,380.166702993939,380.435359210937,
380.704015424011,380.972671637828,381.241327856887,381.509984085112,381.778640325533,
382.047296580819,382.315952852685,382.584609142666,382.853265451347,383.121921779263,
383.390578126049,383.659234491374,383.927890874099,384.196547273165,384.465203686833,
384.733860113456,385.002516550867,385.271172996977,385.539829449352,385.808485905613,
386.077142363224,386.345798819663,386.614455272453,386.883111719088,387.151768157302,
387.420424584764,387.689080999572,387.957737399735,388.226393783858,388.49505015046,
388.7637064988,389.032362828074,389.301019138333,389.56967542963,389.838331702943,
390.106987959358,390.375644200917,390.644300429918,390.912956649593,391.181612863644,
391.450269076596,391.718925293171,391.987581517421,392.25623775287,392.524894002124,
392.793550267489,393.062206550312,393.330862851807,393.599519172248,393.868175511888,
394.136831870107,394.405488246334,394.674144639227,394.94280104753,395.211457469356,
395.480113902905,395.748770345913,396.017426796181,396.286083251232,396.554739708622,
396.823396165819,397.092052620289,397.360709069602,397.629365511291,397.898021943183,
398.166678363037,398.43533476909,398.703991159489,398.972647533028,399.241303888413,
399.509960225133,399.778616542629,400.047272841224,400.315929121267,400.584585384052,
400.853241631017,401.121897864557,401.390554087381,401.659210303115,401.927866515925,
402.196522730559,402.465178951451,402.733835182185,403.002491425899,403.271147684792,
403.539803960819,403.808460254978,404.077116568174,404.345772900386,404.614429251599,
404.883085620952,405.151742007649,405.420398410161,405.689054827051,405.957711256297,
406.226367695961,406.495024143695,406.76368059721,407.032337053993,407.300993511558,
407.569649967387,407.838306418949,408.106962863879,408.375619299759,408.644275724528,
408.912932136048,409.181588532709,409.450244912815,409.718901275356,409.987557619248,
410.25621394422,410.524870249975,410.79352653712,411.06218280632,411.330839059193,
411.599495297549,411.868151524149,412.13680774213,412.40546395552,412.674120168911,
412.942776386892,413.211432613491,413.480088851848,413.748745104721,414.017401373921,
414.286057661065,414.55471396682,414.823370291793,415.092026635685,415.360682998226,
415.629339378332,415.897995774993,416.166652186512,416.435308611282,416.703965047162,
416.972621492092,417.241277943654,417.509934399483,417.778590857048,418.047247313831,
418.315903767346,418.58456021508,418.853216654744,419.121873083989,419.390529500879,
419.659185903392,419.927842290088,420.196498659441,420.465155010654,420.733811342866,
421.002467656062,421.271123950222,421.539780226249,421.808436485141,422.077092728855,
422.34574895959,422.614405180482,422.883061395116,423.151717607926,423.42037382366,
423.689030046484,423.957686280024,424.226342526988,424.494998789773,424.763655069817,
425.032311368411,425.300967685907,425.569624022627,425.838280378013,426.106936751551,
426.375593141951,426.644249548003,426.912905967857,427.18156239975,427.450218841438,
427.718875290752,427.987531745221,428.256188202418,428.524844659809,428.793501114859,
429.062157565128,429.330814008135,429.599470441684,429.868126863511,430.136783271814,
430.405439664707,430.674096040933,430.942752399152,431.211408738792,431.480065059233,
431.748721360729,432.017377643552,432.286033908916,432.554690158171,432.823346393619,
433.092002617869,433.360658834445,433.629315047397,433.897971261447,434.166627481123,
434.435283710124,434.703939951682,434.972596208097,435.241252481411,435.509908772707,
435.778565082967,436.047221412241,436.31587776058,436.584534127182,436.853190511305,
437.121846911468,437.390503326275,437.659159753738,437.927816191952,438.196472638587,
438.465129091377,438.733785547816,439.002442005427,439.271098461688,439.539754914064,
439.808411360173,440.077067797584,440.345724224207,440.614380637875,440.883037036941,
441.151693419666,441.420349784991,441.689006131777,441.957662459693,442.226318768374,
442.494975058355,442.763631330221,443.032287585506,443.300943825928,443.569600054153,
443.838256273211,444.106912487028,444.375568700103,444.644224917101,444.912881142151,
445.181537378504,445.450193629011,445.718849895579,445.987506179909,446.256162482747,
446.524818804774,446.79347514576,447.062131505496,447.330787882954,447.599444277176,
447.868100686504,448.136757109373,448.40541354367,448.674069987365,448.942726438055,
449.211382893394,449.480039350853,449.748695807921,450.017352262103,450.286008710879,
450.55466515194,450.82332158292,451.091978001848,451.360634406672,451.62929079591,
451.89794716799,452.166603522061,452.435259857205,452.703916173343,452.972572470381,
453.24122874915,453.509885010562,453.778541256488,454.047197489028,454.315853711222,
454.584509926543,454.853166139327,455.121822354318,455.3904785758,455.659134807498,
455.927791052226,456.19644731247,456.465103589759,456.733759885467,457.00241620002,
457.271072533811,457.539728886346,457.80838525717,458.077041645044,458.345698048806,
458.614354466642,458.883010896827,459.151667337143,459.420323785445,459.688980239275,
459.957636696219,460.226293153743,460.494949609316,460.763606060482,461.032262504754,
461.300918939909,461.569575363662,461.838231774175,462.106888169527,462.375544548414,
462.644200909447,462.912857251999,463.181513575386,463.450169879794,463.71882616542,
463.987482433401,464.256138684994,464.524794922418,464.793451148174,465.062107365689,
465.330763578896,465.59941979247,465.86807601102,466.13673223836,466.405388477821,
466.674044731802,466.942701002433,467.211357290885,467.480013598214,467.748669924546,
468.017326269997,468.285982633826,468.554639015346,468.823295413121,469.091951825803,
469.360608251434,469.629264688145,469.897921133626,470.166577585633,470.435234041669,
470.703890499266,470.972546955898,471.24120340903,471.509859856263,471.778516295153,
472.047172723582,472.315829139356,472.584485540789,472.853141926103,473.12179829419,
473.390454643857,473.659110974714,473.927767286328,474.196423579164,474.465079853726,
474.73373611147,475.002392354016,475.271048583941,475.539704804167,475.808361018519,
476.077017231391,476.345673447501,476.614329671083,476.882985905496,477.151642153686,
477.420298417658,477.688954699194,477.957610999126,478.226267318208,478.494923656277,
478.76358001319,479.032236387973,479.300892779719,479.569549186815,479.838205607737,
480.106862040401,480.375518482806,480.644174932567,480.912831387357,481.18148784465,
481.450144301944,481.718800756733,481.987457206495,482.2561136489,482.524770081563,
482.793426502485,483.062082909582,483.330739301328,483.59939567611,483.868052033023,
484.136708371092,484.405364690174,484.674020990106,484.942677271643,485.211333535614,
485.479989783805,485.748646018218,486.017302241799,486.28595845791,486.554614670781,
486.823270885133,487.091927105359,487.360583335284,487.629239577831,487.897895835574,
488.166552110137,488.435208402973,488.703864714587,488.972521045443,489.241177395111,
489.509833763197,489.778490148512,490.047146549945,490.315802965719,490.584459394147,
490.853115833037,491.12177228027,491.390428733402,491.659085190034,491.927741647632,
492.196398103667,492.465054555674,492.733711001155,493.002367437866,493.271023863497,
493.539680276179,493.808336673954,494.076993055474,494.345649419303,494.614305764754,
494.882962091086,495.151618398416,495.420274686867,495.688930957498,495.95758721148,
496.22624345094,496.494899678281,496.76355589683,497.032212110404,497.300868323611,
497.569524541126,497.838180766882,498.106837004306,498.3754932559,498.64414952388,
498.912805809507,499.181462113914,499.450118437301,499.718774779852,499.987431140886,
500.256087519773,500.524743915125,500.793400325638,501.06205674939,501.330713184546,
501.599369628818,501.868026079984,502.136682535557,502.40533899308,502.673995450025,
502.942651903855,503.211308352156,503.479964792472,503.748621222657,504.017277640494,
504.285934044256,504.554590432129,504.823246802954,505.091903155488,505.360559489279,
505.629215803832,505.89787209954,506.166528376829,506.435184637073,506.703840881801,
506.972497113499,507.241153334981,507.509809549972,507.778465762756,508.047121978078,
508.315778200272,508.584434432811,508.853090678737,509.121746940149,509.390403218918,
509.659059515956,509.927715832093,510.196372167238,510.465028521309,510.733684893389,
511.002341282627,511.270997687451,511.53965410638,511.808310537359,512.076966978421,
512.345623427198,512.614279881382,512.882936338452,513.151592795914,513.420249251254,
513.688905701946,513.957562145643,514.226218579942,514.494875002812,514.763531412143,
515.032187806366,515.300844183826,515.569500543564,515.838156884552,516.106813206581,
516.375469509421,516.644125793752,516.912782060321,517.181438310831,517.450094547186,
517.718750772238,517.987406989238,518.256063202315,518.524719416134,518.793375635194,
519.062031863421,519.330688103845,519.599344359133,519.868000631,520.136656920983,
520.405313229665,520.673969557583,520.942625904371,521.211282269698,521.479938652425,
521.748595051492,522.017251465163,522.285907891788,522.554564329201,522.823220775312,
523.091877227689,523.360533683951,523.629190141564,523.897846598005,524.166503050797,
524.435159497434,524.70381593565,524.972472363114,525.241128777924,525.509785178088,
525.778441562214,526.047097928818,526.315754277159,526.584410606435,526.853066916696,
527.121723207994,527.390379481309,527.659035737726,527.927691979287,528.19634820829,
528.465004427967,528.73366064202,529.002316854973,529.270973071551,529.539629295803,
529.808285531254,530.07694178051,530.345598045876,530.614254328701,530.882910630198,
531.151566950641,531.420223290284,531.688879648504,531.957536024733,532.226192417628,
532.494848825933,532.76350524776,533.032161681312,533.30081812432,533.569474574591,
533.838131029643,534.106787487035,534.375443944235,534.644100398706,534.912756848021,
535.181413289711,535.450069721605,535.718726141461,535.987382547516,536.256038937917,
536.524695311458,536.793351666845,537.062008003567,537.330664321065,537.599320619661,
537.867976899706,538.136633162493,538.40528940946,538.673945643001,538.942601865828,
539.211258081563,539.479914294375,539.748570509011,540.017226729904,540.285882960641,
540.554539204357,540.823195463252,541.09185173928,541.360508033441,541.629164346639,
541.897820678853,542.166477030068,542.435133399423,542.703789786121,542.972446188636,
543.241102605527,543.509759034775,543.778415474441,544.047071922176,544.315728375693,
544.584384832479,544.853041290046,545.121697745877,545.390354197441,545.659010642372,
545.927667078254,546.196323503025,546.464979914547,546.733636311202,547.002292691334,
547.270949053789,547.539605397955,547.808261722147,548.076918029812,548.345574313508,
548.614230583738,548.882886864851,549.151542935882,549.420199787641,549.68885445376,
549.957511414581),.UNSPECIFIED.)
GEOMETRIC_REPRESENTATION_ITEM()
RATIONAL_B_SPLINE_SURFACE(((1.,1.,1.,1.,1.,1.,1.,1.,1.,1.,1.,1.,1.,1.,1.,
1.,1.,1.,1.,1.,1.,1.,1.,1.,1.,1.,1.,1.,1.,1.,1.,1.,1.,1.,1.,1.,1.,1.,1.,
1.,1.,1.,1.,1.,1.,1.,1.,1.,1.,1.,1.,1.,1.,1.,1.,1.,1.,1.,1.,1.,1.,1.,1.,
1.,1.,1.,1.,1.,1.,1.,1.,1.,1.,1.,1.,1.,1.,1.,1.,1.,1.,1.,1.,1.,1.,1.,1.,
1.,1.,1.,1.,1.,1.,1.,1.,1.,1.,1.,1.,1.,1.,1.,1.,1.,1.,1.,1.,1.,1.,1.,1.,
1.,1.,1.,1.,1.,1.,1.,1.,1.,1.,1.,1.,1.,1.,1.,1.,1.,1.,1.,1.,1.,1.,1.,1.,
1.,1.,1.,1.,1.,1.,1.,1.,1.,1.,1.,1.,1.,1.,1.,1.,1.,1.,1.,1.,1.,1.,1.,1.,
1.,1.,1.,1.,1.,1.,1.,1.,1.,1.,1.,1.,1.,1.,1.,1.,1.,1.,1.,1.,1.,1.,1.,1.,
1.,1.,1.,1.,1.,1.,1.,1.,1.,1.,1.,1.,1.,1.,1.,1.,1.,1.,1.,1.,1.,1.,1.,1.,
1.,1.,1.,1.,1.,1.,1.,1.,1.,1.,1.,1.,1.,1.,1.,1.,1.,1.,1.,1.,1.,1.,1.,1.,
1.,1.,1.,1.,1.,1.,1.,1.,1.,1.,1.,1.,1.,1.,1.,1.,1.,1.,1.,1.,1.,1.,1.,1.,
1.,1.,1.,1.,1.,1.,1.,1.,1.,1.,1.,1.,1.,1.,1.,1.,1.,1.,1.,1.,1.,1.,1.,1.,
1.,1.,1.,1.,1.,1.,1.,1.,1.,1.,1.,1.,1.,1.,1.,1.,1.,1.,1.,1.,1.,1.,1.,1.,
1.,1.,1.,1.,1.,1.,1.,1.,1.,1.,1.,1.,1.,1.,1.,1.,1.,1.,1.,1.,1.,1.,1.,1.,
1.,1.,1.,1.,1.,1.,1.,1.,1.,1.,1.,1.,1.,1.,1.,1.,1.,1.,1.,1.,1.,1.,1.,1.,
1.,1.,1.,1.,1.,1.,1.,1.,1.,1.,1.,1.,1.,1.,1.,1.,1.,1.,1.,1.,1.,1.,1.,1.,
1.,1.,1.,1.,1.,1.,1.,1.,1.,1.,1.,1.,1.,1.,1.,1.,1.,1.,1.,1.,1.,1.,1.,1.,
1.,1.,1.,1.,1.,1.,1.,1.,1.,1.,1.,1.,1.,1.,1.,1.,1.,1.,1.,1.,1.,1.,1.,1.,
1.,1.,1.,1.,1.,1.,1.,1.,1.,1.,1.,1.,1.,1.,1.,1.,1.,1.,1.,1.,1.,1.,1.,1.,
1.,1.,1.,1.,1.,1.,1.,1.,1.,1.,1.,1.,1.,1.,1.,1.,1.,1.,1.,1.,1.,1.,1.,1.,
1.,1.,1.,1.,1.,1.,1.,1.,1.,1.,1.,1.,1.,1.,1.,1.,1.,1.,1.,1.,1.,1.,1.,1.,
1.,1.,1.,1.,1.,1.,1.,1.,1.,1.,1.,1.,1.,1.,1.,1.,1.,1.,1.,1.,1.,1.,1.,1.,
1.,1.,1.,1.,1.,1.,1.,1.,1.,1.,1.,1.,1.,1.,1.,1.,1.,1.,1.,1.,1.,1.,1.,1.,
1.,1.,1.,1.,1.,1.,1.,1.,1.,1.,1.,1.,1.,1.,1.,1.,1.,1.,1.,1.,1.,1.,1.,1.,
1.,1.,1.,1.,1.,1.,1.,1.,1.,1.,1.,1.,1.,1.,1.,1.,1.,1.,1.,1.,1.,1.,1.,1.,
1.,1.,1.,1.,1.,1.,1.,1.,1.,1.,1.,1.,1.,1.,1.,1.,1.,1.,1.,1.,1.,1.,1.,1.,
1.,1.,1.,1.,1.,1.,1.,1.,1.,1.,1.,1.,1.,1.,1.,1.,1.,1.,1.,1.,1.,1.,1.,1.,
1.,1.,1.,1.,1.,1.,1.,1.,1.,1.,1.,1.,1.,1.,1.,1.,1.,1.,1.,1.,1.,1.,1.,1.,
1.,1.,1.,1.,1.,1.,1.,1.,1.,1.,1.,1.,1.,1.,1.,1.,1.,1.,1.,1.,1.,1.,1.,1.,
1.,1.,1.,1.,1.,1.,1.,1.,1.,1.,1.,1.,1.,1.,1.,1.,1.,1.,1.,1.,1.,1.,1.,1.,
1.,1.,1.,1.,1.,1.,1.,1.,1.,1.,1.,1.,1.,1.,1.,1.,1.,1.,1.,1.,1.,1.,1.,1.,
1.,1.,1.,1.,1.,1.,1.,1.,1.,1.,1.,1.,1.,1.,1.,1.,1.,1.,1.,1.,1.,1.,1.,1.,
1.,1.,1.,1.,1.,1.,1.,1.,1.,1.,1.,1.,1.,1.,1.,1.,1.,1.,1.,1.,1.,1.,1.,1.,
1.,1.,1.,1.,1.,1.,1.,1.,1.,1.,1.,1.,1.,1.,1.,1.,1.,1.,1.,1.,1.,1.,1.,1.,
1.,1.,1.,1.,1.,1.,1.,1.,1.,1.,1.,1.,1.,1.,1.,1.,1.,1.,1.,1.,1.,1.,1.,1.,
1.,1.,1.,1.,1.,1.,1.,1.,1.,1.,1.,1.,1.,1.,1.,1.,1.,1.,1.,1.,1.,1.,1.,1.,
1.,1.,1.,1.,1.,1.,1.,1.,1.,1.,1.,1.,1.,1.,1.,1.,1.,1.,1.,1.,1.,1.,1.,1.,
1.,1.,1.,1.,1.,1.,1.,1.,1.,1.,1.,1.,1.,1.,1.,1.,1.,1.,1.,1.,1.,1.,1.,1.,
1.,1.,1.,1.,1.,1.,1.,1.,1.,1.,1.,1.,1.,1.,1.,1.,1.,1.,1.,1.,1.,1.,1.,1.,
1.,1.,1.,1.,1.,1.,1.,1.,1.,1.,1.,1.,1.,1.,1.,1.,1.,1.,1.,1.,1.,1.,1.,1.,
1.,1.,1.,1.,1.,1.,1.,1.,1.,1.,1.,1.,1.,1.,1.,1.,1.,1.,1.,1.,1.,1.,1.,1.,
1.,1.,1.,1.,1.,1.,1.,1.,1.,1.,1.,1.,1.,1.,1.,1.,1.,1.,1.,1.,1.,1.,1.,1.,
1.,1.,1.,1.,1.,1.,1.,1.,1.,1.,1.,1.,1.,1.,1.,1.,1.,1.,1.,1.,1.,1.,1.,1.,
1.,1.,1.,1.,1.,1.,1.,1.,1.,1.,1.,1.,1.,1.,1.,1.,1.,1.,1.,1.,1.,1.,1.,1.,
1.,1.,1.,1.,1.,1.,1.,1.,1.,1.,1.,1.,1.,1.,1.,1.,1.,1.,1.,1.,1.,1.,1.,1.,
1.,1.,1.,1.,1.,1.,1.,1.,1.,1.,1.,1.,1.,1.,1.,1.,1.,1.,1.,1.,1.,1.,1.,1.,
1.,1.,1.,1.,1.,1.,1.,1.,1.,1.,1.,1.,1.,1.,1.,1.,1.,1.,1.,1.,1.,1.,1.,1.,
1.,1.,1.,1.,1.,1.,1.,1.,1.,1.,1.,1.,1.,1.,1.,1.,1.,1.,1.,1.,1.,1.,1.,1.,
1.,1.,1.,1.,1.,1.,1.,1.,1.,1.,1.,1.,1.,1.,1.,1.,1.,1.,1.,1.,1.,1.,1.,1.,
1.,1.,1.,1.,1.,1.,1.,1.,1.,1.,1.,1.,1.,1.,1.,1.,1.,1.,1.,1.,1.,1.,1.,1.,
1.,1.,1.,1.,1.,1.,1.,1.,1.,1.,1.,1.,1.,1.,1.,1.,1.,1.,1.,1.,1.,1.,1.,1.,
1.,1.,1.,1.,1.,1.,1.,1.,1.,1.,1.,1.,1.,1.,1.,1.,1.,1.,1.,1.,1.,1.,1.,1.,
1.,1.,1.,1.,1.,1.,1.,1.,1.,1.,1.,1.,1.,1.,1.,1.,1.,1.,1.,1.,1.,1.,1.,1.,
1.,1.,1.,1.,1.,1.,1.,1.,1.,1.,1.,1.,1.,1.,1.,1.,1.,1.,1.,1.,1.,1.,1.,1.,
1.,1.,1.,1.,1.,1.,1.,1.,1.,1.,1.,1.,1.,1.,1.,1.,1.,1.,1.,1.,1.,1.,1.,1.,
1.,1.,1.,1.,1.,1.,1.,1.,1.,1.,1.,1.,1.,1.,1.,1.,1.,1.,1.,1.,1.,1.,1.,1.,
1.,1.,1.,1.,1.,1.,1.,1.,1.,1.,1.,1.,1.,1.,1.,1.,1.,1.,1.,1.,1.,1.,1.,1.,
1.,1.,1.,1.,1.,1.,1.,1.,1.,1.,1.,1.,1.,1.,1.,1.,1.,1.,1.,1.,1.,1.,1.,1.,
1.,1.,1.,1.,1.,1.,1.,1.,1.,1.,1.,1.,1.,1.,1.,1.,1.,1.,1.,1.,1.,1.,1.,1.,
1.,1.,1.,1.,1.,1.,1.,1.,1.,1.,1.,1.,1.,1.,1.,1.,1.,1.,1.,1.,1.,1.,1.,1.,
1.,1.,1.,1.,1.,1.,1.,1.,1.,1.,1.,1.,1.,1.,1.,1.,1.,1.,1.,1.,1.,1.,1.,1.,
1.,1.,1.,1.,1.,1.,1.,1.,1.,1.,1.,1.,1.,1.,1.,1.,1.,1.,1.,1.,1.,1.,1.,1.,
1.,1.,1.,1.,1.,1.,1.,1.,1.,1.,1.,1.,1.,1.,1.,1.,1.,1.,1.,1.,1.,1.,1.,1.,
1.,1.,1.,1.,1.,1.,1.,1.,1.,1.,1.,1.,1.,1.,1.,1.,1.,1.,1.,1.,1.,1.,1.,1.,
1.,1.,1.,1.,1.,1.,1.,1.,1.,1.,1.,1.,1.,1.,1.,1.,1.,1.,1.,1.,1.,1.,1.,1.,
1.,1.,1.,1.,1.,1.,1.,1.,1.,1.,1.,1.,1.,1.,1.,1.,1.,1.,1.,1.,1.,1.,1.,1.,
1.,1.,1.,1.,1.,1.,1.,1.,1.,1.,1.,1.,1.,1.,1.,1.,1.,1.,1.,1.,1.,1.,1.,1.,
1.,1.,1.,1.,1.,1.,1.,1.,1.,1.,1.,1.,1.,1.,1.,1.,1.,1.,1.,1.,1.,1.,1.,1.,
1.,1.,1.,1.,1.,1.,1.,1.,1.,1.,1.,1.,1.,1.,1.,1.,1.,1.,1.,1.,1.,1.,1.,1.,
1.,1.,1.,1.,1.,1.,1.,1.,1.,1.,1.,1.,1.,1.,1.,1.,1.,1.,1.,1.,1.,1.,1.,1.,
1.,1.,1.,1.,1.,1.,1.,1.,1.,1.,1.,1.,1.,1.,1.,1.,1.,1.,1.,1.,1.,1.,1.,1.,
1.,1.,1.,1.,1.,1.,1.,1.,1.,1.,1.,1.,1.,1.,1.,1.,1.,1.,1.,1.,1.,1.,1.,1.,
1.,1.,1.,1.,1.,1.,1.,1.,1.,1.,1.,1.,1.,1.,1.,1.,1.,1.,1.,1.,1.,1.,1.,1.,
1.,1.,1.,1.,1.,1.,1.,1.,1.,1.,1.,1.,1.,1.,1.,1.,1.,1.,1.,1.,1.,1.,1.,1.,
1.,1.,1.,1.,1.,1.,1.,1.,1.,1.,1.,1.,1.,1.,1.,1.,1.,1.,1.,1.,1.,1.,1.,1.,
1.,1.,1.,1.,1.,1.,1.,1.,1.,1.,1.,1.,1.,1.,1.,1.,1.,1.,1.,1.,1.,1.,1.,1.,
1.,1.,1.,1.,1.,1.,1.,1.,1.,1.,1.,1.,1.,1.,1.,1.,1.,1.,1.,1.,1.,1.,1.,1.,
1.,1.,1.,1.,1.,1.,1.,1.,1.,1.,1.,1.,1.,1.,1.,1.,1.,1.,1.,1.,1.,1.,1.,1.,
1.,1.,1.,1.,1.,1.,1.,1.,1.,1.,1.,1.,1.,1.,1.,1.,1.,1.,1.,1.,1.,1.,1.,1.,
1.,1.,1.,1.,1.,1.,1.,1.,1.,1.,1.,1.,1.,1.,1.,1.,1.,1.,1.,1.,1.,1.,1.,1.,
1.,1.,1.,1.,1.,1.,1.,1.,1.,1.,1.,1.,1.,1.,1.,1.,1.,1.,1.,1.,1.,1.,1.,1.,
1.,1.,1.,1.,1.,1.,1.,1.,1.,1.,1.,1.,1.,1.,1.,1.,1.,1.,1.,1.,1.,1.,1.,1.,
1.,1.,1.,1.,1.,1.,1.,1.,1.,1.,1.,1.,1.,1.,1.,1.,1.,1.,1.,1.,1.,1.,1.,1.,
1.,1.,1.,1.,1.,1.,1.,1.,1.,1.,1.,1.,1.,1.,1.,1.,1.,1.,1.,1.,1.,1.,1.,1.,
1.,1.,1.,1.,1.,1.,1.,1.,1.,1.,1.,1.,1.,1.,1.,1.,1.,1.,1.,1.,1.,1.,1.,1.,
1.,1.,1.,1.,1.,1.,1.,1.,1.,1.,1.,1.,1.,1.,1.,1.,1.,1.,1.,1.),(0.707106781186548,
0.707106781186548,0.707106781186548,0.707106781186547,0.707106781186547,
0.707106781186548,0.707106781186547,0.707106781186547,0.707106781186547,
0.707106781186547,0.707106781186547,0.707106781186548,0.707106781186548,
0.707106781186548,0.707106781186547,0.707106781186548,0.707106781186547,
0.707106781186547,0.707106781186548,0.707106781186547,0.707106781186548,
0.707106781186547,0.707106781186548,0.707106781186547,0.707106781186548,
0.707106781186547,0.707106781186547,0.707106781186547,0.707106781186547,
0.707106781186547,0.707106781186548,0.707106781186547,0.707106781186547,
0.707106781186548,0.707106781186547,0.707106781186547,0.707106781186548,
0.707106781186547,0.707106781186547,0.707106781186548,0.707106781186548,
0.707106781186547,0.707106781186548,0.707106781186547,0.707106781186547,
0.707106781186547,0.707106781186548,0.707106781186548,0.707106781186547,
0.707106781186547,0.707106781186548,0.707106781186547,0.707106781186548,
0.707106781186547,0.707106781186547,0.707106781186547,0.707106781186547,
0.707106781186547,0.707106781186548,0.707106781186547,0.707106781186548,
0.707106781186547,0.707106781186548,0.707106781186547,0.707106781186548,
0.707106781186547,0.707106781186547,0.707106781186548,0.707106781186547,
0.707106781186547,0.707106781186548,0.707106781186547,0.707106781186548,
0.707106781186547,0.707106781186548,0.707106781186548,0.707106781186547,
0.707106781186548,0.707106781186547,0.707106781186547,0.707106781186548,
0.707106781186547,0.707106781186547,0.707106781186547,0.707106781186548,
0.707106781186547,0.707106781186547,0.707106781186547,0.707106781186547,
0.707106781186547,0.707106781186547,0.707106781186548,0.707106781186548,
0.707106781186547,0.707106781186548,0.707106781186547,0.707106781186548,
0.707106781186548,0.707106781186547,0.707106781186548,0.707106781186548,
0.707106781186548,0.707106781186547,0.707106781186548,0.707106781186547,
0.707106781186548,0.707106781186548,0.707106781186548,0.707106781186547,
0.707106781186547,0.707106781186547,0.707106781186548,0.707106781186548,
0.707106781186548,0.707106781186547,0.707106781186547,0.707106781186547,
0.707106781186548,0.707106781186548,0.707106781186547,0.707106781186547,
0.707106781186548,0.707106781186547,0.707106781186547,0.707106781186547,
0.707106781186547,0.707106781186548,0.707106781186547,0.707106781186548,
0.707106781186547,0.707106781186547,0.707106781186547,0.707106781186548,
0.707106781186548,0.707106781186547,0.707106781186548,0.707106781186548,
0.707106781186547,0.707106781186548,0.707106781186547,0.707106781186548,
0.707106781186547,0.707106781186548,0.707106781186547,0.707106781186547,
0.707106781186548,0.707106781186547,0.707106781186547,0.707106781186548,
0.707106781186547,0.707106781186547,0.707106781186548,0.707106781186547,
0.707106781186548,0.707106781186547,0.707106781186547,0.707106781186548,
0.707106781186548,0.707106781186547,0.707106781186548,0.707106781186547,
0.707106781186548,0.707106781186547,0.707106781186548,0.707106781186547,
0.707106781186548,0.707106781186547,0.707106781186548,0.707106781186547,
0.707106781186548,0.707106781186547,0.707106781186548,0.707106781186547,
0.707106781186547,0.707106781186548,0.707106781186547,0.707106781186548,
0.707106781186547,0.707106781186548,0.707106781186547,0.707106781186548,
0.707106781186547,0.707106781186547,0.707106781186548,0.707106781186547,
0.707106781186548,0.707106781186548,0.707106781186548,0.707106781186547,
0.707106781186547,0.707106781186547,0.707106781186547,0.707106781186548,
0.707106781186547,0.707106781186548,0.707106781186548,0.707106781186547,
0.707106781186547,0.707106781186548,0.707106781186548,0.707106781186547,
0.707106781186547,0.707106781186548,0.707106781186547,0.707106781186548,
0.707106781186547,0.707106781186547,0.707106781186547,0.707106781186547,
0.707106781186547,0.707106781186547,0.707106781186547,0.707106781186548,
0.707106781186547,0.707106781186548,0.707106781186547,0.707106781186548,
0.707106781186548,0.707106781186547,0.707106781186548,0.707106781186548,
0.707106781186548,0.707106781186548,0.707106781186547,0.707106781186548,
0.707106781186547,0.707106781186548,0.707106781186547,0.707106781186547,
0.707106781186548,0.707106781186548,0.707106781186547,0.707106781186547,
0.707106781186547,0.707106781186547,0.707106781186547,0.707106781186548,
0.707106781186548,0.707106781186547,0.707106781186547,0.707106781186548,
0.707106781186548,0.707106781186547,0.707106781186548,0.707106781186547,
0.707106781186548,0.707106781186548,0.707106781186547,0.707106781186547,
0.707106781186548,0.707106781186547,0.707106781186547,0.707106781186548,
0.707106781186547,0.707106781186548,0.707106781186547,0.707106781186548,
0.707106781186547,0.707106781186547,0.707106781186548,0.707106781186548,
0.707106781186547,0.707106781186547,0.707106781186548,0.707106781186547,
0.707106781186547,0.707106781186548,0.707106781186547,0.707106781186548,
0.707106781186547,0.707106781186548,0.707106781186547,0.707106781186548,
0.707106781186547,0.707106781186547,0.707106781186547,0.707106781186547,
0.707106781186547,0.707106781186547,0.707106781186548,0.707106781186547,
0.707106781186548,0.707106781186547,0.707106781186548,0.707106781186548,
0.707106781186547,0.707106781186548,0.707106781186548,0.707106781186547,
0.707106781186548,0.707106781186547,0.707106781186547,0.707106781186547,
0.707106781186548,0.707106781186547,0.707106781186547,0.707106781186548,
0.707106781186547,0.707106781186548,0.707106781186547,0.707106781186547,
0.707106781186547,0.707106781186548,0.707106781186548,0.707106781186547,
0.707106781186548,0.707106781186548,0.707106781186547,0.707106781186548,
0.707106781186547,0.707106781186548,0.707106781186548,0.707106781186547,
0.707106781186548,0.707106781186548,0.707106781186548,0.707106781186547,
0.707106781186547,0.707106781186548,0.707106781186547,0.707106781186548,
0.707106781186547,0.707106781186547,0.707106781186548,0.707106781186548,
0.707106781186548,0.707106781186547,0.707106781186547,0.707106781186548,
0.707106781186548,0.707106781186547,0.707106781186547,0.707106781186548,
0.707106781186547,0.707106781186547,0.707106781186548,0.707106781186548,
0.707106781186547,0.707106781186547,0.707106781186547,0.707106781186548,
0.707106781186547,0.707106781186547,0.707106781186547,0.707106781186548,
0.707106781186548,0.707106781186547,0.707106781186548,0.707106781186547,
0.707106781186548,0.707106781186547,0.707106781186548,0.707106781186548,
0.707106781186547,0.707106781186547,0.707106781186548,0.707106781186547,
0.707106781186547,0.707106781186548,0.707106781186547,0.707106781186548,
0.707106781186548,0.707106781186547,0.707106781186548,0.707106781186547,
0.707106781186547,0.707106781186547,0.707106781186548,0.707106781186548,
0.707106781186548,0.707106781186547,0.707106781186548,0.707106781186547,
0.707106781186548,0.707106781186547,0.707106781186547,0.707106781186547,
0.707106781186547,0.707106781186548,0.707106781186548,0.707106781186547,
0.707106781186547,0.707106781186548,0.707106781186547,0.707106781186548,
0.707106781186547,0.707106781186548,0.707106781186547,0.707106781186547,
0.707106781186548,0.707106781186547,0.707106781186548,0.707106781186547,
0.707106781186548,0.707106781186548,0.707106781186547,0.707106781186548,
0.707106781186547,0.707106781186548,0.707106781186548,0.707106781186547,
0.707106781186548,0.707106781186547,0.707106781186547,0.707106781186548,
0.707106781186547,0.707106781186548,0.707106781186547,0.707106781186548,
0.707106781186547,0.707106781186547,0.707106781186548,0.707106781186548,
0.707106781186548,0.707106781186548,0.707106781186547,0.707106781186548,
0.707106781186548,0.707106781186548,0.707106781186547,0.707106781186548,
0.707106781186548,0.707106781186548,0.707106781186547,0.707106781186547,
0.707106781186548,0.707106781186547,0.707106781186548,0.707106781186547,
0.707106781186548,0.707106781186548,0.707106781186547,0.707106781186547,
0.707106781186548,0.707106781186547,0.707106781186548,0.707106781186547,
0.707106781186548,0.707106781186548,0.707106781186547,0.707106781186547,
0.707106781186547,0.707106781186548,0.707106781186548,0.707106781186547,
0.707106781186547,0.707106781186548,0.707106781186548,0.707106781186548,
0.707106781186548,0.707106781186547,0.707106781186547,0.707106781186548,
0.707106781186548,0.707106781186547,0.707106781186548,0.707106781186547,
0.707106781186548,0.707106781186547,0.707106781186548,0.707106781186547,
0.707106781186547,0.707106781186548,0.707106781186547,0.707106781186547,
0.707106781186548,0.707106781186547,0.707106781186548,0.707106781186547,
0.707106781186548,0.707106781186547,0.707106781186548,0.707106781186547,
0.707106781186548,0.707106781186547,0.707106781186548,0.707106781186547,
0.707106781186547,0.707106781186548,0.707106781186548,0.707106781186547,
0.707106781186547,0.707106781186547,0.707106781186548,0.707106781186547,
0.707106781186548,0.707106781186547,0.707106781186548,0.707106781186547,
0.707106781186548,0.707106781186547,0.707106781186547,0.707106781186547,
0.707106781186548,0.707106781186547,0.707106781186548,0.707106781186548,
0.707106781186547,0.707106781186548,0.707106781186547,0.707106781186547,
0.707106781186548,0.707106781186547,0.707106781186547,0.707106781186548,
0.707106781186547,0.707106781186547,0.707106781186547,0.707106781186547,
0.707106781186548,0.707106781186547,0.707106781186547,0.707106781186547,
0.707106781186548,0.707106781186547,0.707106781186547,0.707106781186548,
0.707106781186548,0.707106781186547,0.707106781186548,0.707106781186548,
0.707106781186547,0.707106781186547,0.707106781186548,0.707106781186547,
0.707106781186547,0.707106781186548,0.707106781186547,0.707106781186547,
0.707106781186547,0.707106781186548,0.707106781186547,0.707106781186548,
0.707106781186547,0.707106781186548,0.707106781186547,0.707106781186548,
0.707106781186547,0.707106781186548,0.707106781186547,0.707106781186548,
0.707106781186548,0.707106781186547,0.707106781186547,0.707106781186548,
0.707106781186547,0.707106781186548,0.707106781186547,0.707106781186548,
0.707106781186548,0.707106781186547,0.707106781186548,0.707106781186547,
0.707106781186548,0.707106781186548,0.707106781186547,0.707106781186547,
0.707106781186548,0.707106781186547,0.707106781186548,0.707106781186547,
0.707106781186548,0.707106781186547,0.707106781186548,0.707106781186547,
0.707106781186547,0.707106781186547,0.707106781186547,0.707106781186547,
0.707106781186547,0.707106781186547,0.707106781186547,0.707106781186548,
0.707106781186547,0.707106781186548,0.707106781186547,0.707106781186547,
0.707106781186548,0.707106781186547,0.707106781186548,0.707106781186547,
0.707106781186547,0.707106781186548,0.707106781186547,0.707106781186548,
0.707106781186547,0.707106781186548,0.707106781186547,0.707106781186548,
0.707106781186547,0.707106781186548,0.707106781186547,0.707106781186548,
0.707106781186547,0.707106781186548,0.707106781186548,0.707106781186547,
0.707106781186548,0.707106781186547,0.707106781186547,0.707106781186547,
0.707106781186548,0.707106781186547,0.707106781186547,0.707106781186547,
0.707106781186548,0.707106781186547,0.707106781186547,0.707106781186548,
0.707106781186547,0.707106781186547,0.707106781186547,0.707106781186547,
0.707106781186548,0.707106781186547,0.707106781186547,0.707106781186547,
0.707106781186548,0.707106781186548,0.707106781186548,0.707106781186548,
0.707106781186547,0.707106781186548,0.707106781186547,0.707106781186547,
0.707106781186548,0.707106781186547,0.707106781186548,0.707106781186547,
0.707106781186547,0.707106781186548,0.707106781186547,0.707106781186547,
0.707106781186547,0.707106781186547,0.707106781186548,0.707106781186548,
0.707106781186547,0.707106781186547,0.707106781186548,0.707106781186547,
0.707106781186548,0.707106781186547,0.707106781186548,0.707106781186548,
0.707106781186547,0.707106781186547,0.707106781186548,0.707106781186548,
0.707106781186547,0.707106781186548,0.707106781186548,0.707106781186547,
0.707106781186548,0.707106781186548,0.707106781186548,0.707106781186547,
0.707106781186548,0.707106781186547,0.707106781186548,0.707106781186547,
0.707106781186548,0.707106781186547,0.707106781186548,0.707106781186547,
0.707106781186548,0.707106781186548,0.707106781186547,0.707106781186547,
0.707106781186548,0.707106781186547,0.707106781186548,0.707106781186547,
0.707106781186548,0.707106781186548,0.707106781186548,0.707106781186548,
0.707106781186548,0.707106781186547,0.707106781186547,0.707106781186547,
0.707106781186547,0.707106781186548,0.707106781186547,0.707106781186548,
0.707106781186547,0.707106781186547,0.707106781186548,0.707106781186548,
0.707106781186547,0.707106781186548,0.707106781186547,0.707106781186548,
0.707106781186548,0.707106781186547,0.707106781186547,0.707106781186548,
0.707106781186547,0.707106781186548,0.707106781186547,0.707106781186548,
0.707106781186547,0.707106781186548,0.707106781186547,0.707106781186548,
0.707106781186547,0.707106781186548,0.707106781186547,0.707106781186548,
0.707106781186548,0.707106781186547,0.707106781186548,0.707106781186547,
0.707106781186548,0.707106781186547,0.707106781186548,0.707106781186548,
0.707106781186548,0.707106781186547,0.707106781186547,0.707106781186548,
0.707106781186548,0.707106781186547,0.707106781186547,0.707106781186547,
0.707106781186548,0.707106781186547,0.707106781186548,0.707106781186547,
0.707106781186548,0.707106781186547,0.707106781186547,0.707106781186547,
0.707106781186548,0.707106781186547,0.707106781186548,0.707106781186547,
0.707106781186548,0.707106781186547,0.707106781186548,0.707106781186547,
0.707106781186547,0.707106781186548,0.707106781186547,0.707106781186547,
0.707106781186548,0.707106781186547,0.707106781186547,0.707106781186548,
0.707106781186547,0.707106781186547,0.707106781186547,0.707106781186548,
0.707106781186547,0.707106781186548,0.707106781186547,0.707106781186547,
0.707106781186547,0.707106781186548,0.707106781186548,0.707106781186547,
0.707106781186547,0.707106781186548,0.707106781186548,0.707106781186548,
0.707106781186547,0.707106781186548,0.707106781186547,0.707106781186548,
0.707106781186547,0.707106781186548,0.707106781186547,0.707106781186547,
0.707106781186547,0.707106781186547,0.707106781186548,0.707106781186547,
0.707106781186548,0.707106781186548,0.707106781186547,0.707106781186548,
0.707106781186547,0.707106781186547,0.707106781186547,0.707106781186547,
0.707106781186548,0.707106781186547,0.707106781186548,0.707106781186547,
0.707106781186548,0.707106781186548,0.707106781186547,0.707106781186548,
0.707106781186547,0.707106781186547,0.707106781186547,0.707106781186547,
0.707106781186548,0.707106781186547,0.707106781186548,0.707106781186548,
0.707106781186547,0.707106781186548,0.707106781186547,0.707106781186548,
0.707106781186547,0.707106781186547,0.707106781186548,0.707106781186547,
0.707106781186548,0.707106781186548,0.707106781186547,0.707106781186547,
0.707106781186548,0.707106781186548,0.707106781186547,0.707106781186547,
0.707106781186548,0.707106781186547,0.707106781186547,0.707106781186548,
0.707106781186547,0.707106781186547,0.707106781186548,0.707106781186547,
0.707106781186548,0.707106781186547,0.707106781186547,0.707106781186548,
0.707106781186547,0.707106781186548,0.707106781186547,0.707106781186548,
0.707106781186547,0.707106781186547,0.707106781186547,0.707106781186548,
0.707106781186547,0.707106781186548,0.707106781186547,0.707106781186548,
0.707106781186548,0.707106781186548,0.707106781186548,0.707106781186547,
0.707106781186547,0.707106781186547,0.707106781186548,0.707106781186547,
0.707106781186548,0.707106781186547,0.707106781186547,0.707106781186548,
0.707106781186547,0.707106781186547,0.707106781186548,0.707106781186547,
0.707106781186547,0.707106781186548,0.707106781186548,0.707106781186547,
0.707106781186548,0.707106781186547,0.707106781186547,0.707106781186548,
0.707106781186547,0.707106781186548,0.707106781186547,0.707106781186548,
0.707106781186547,0.707106781186547,0.707106781186547,0.707106781186548,
0.707106781186547,0.707106781186548,0.707106781186547,0.707106781186548,
0.707106781186547,0.707106781186547,0.707106781186548,0.707106781186548,
0.707106781186548,0.707106781186547,0.707106781186548,0.707106781186547,
0.707106781186548,0.707106781186547,0.707106781186548,0.707106781186547,
0.707106781186548,0.707106781186548,0.707106781186547,0.707106781186547,
0.707106781186547,0.707106781186548,0.707106781186547,0.707106781186547,
0.707106781186548,0.707106781186547,0.707106781186547,0.707106781186548,
0.707106781186547,0.707106781186548,0.707106781186548,0.707106781186548,
0.707106781186547,0.707106781186548,0.707106781186547,0.707106781186548,
0.707106781186547,0.707106781186548,0.707106781186547,0.707106781186548,
0.707106781186547,0.707106781186548,0.707106781186547,0.707106781186548,
0.707106781186548,0.707106781186547,0.707106781186548,0.707106781186547,
0.707106781186548,0.707106781186548,0.707106781186547,0.707106781186547,
0.707106781186548,0.707106781186547,0.707106781186547,0.707106781186548,
0.707106781186547,0.707106781186548,0.707106781186548,0.707106781186547,
0.707106781186548,0.707106781186548,0.707106781186548,0.707106781186548,
0.707106781186548,0.707106781186547,0.707106781186548,0.707106781186548,
0.707106781186548,0.707106781186547,0.707106781186548,0.707106781186547,
0.707106781186548,0.707106781186547,0.707106781186548,0.707106781186547,
0.707106781186548,0.707106781186547,0.707106781186548,0.707106781186547,
0.707106781186547,0.707106781186548,0.707106781186547,0.707106781186547,
0.707106781186548,0.707106781186547,0.707106781186548,0.707106781186547,
0.707106781186548,0.707106781186547,0.707106781186548,0.707106781186547,
0.707106781186547,0.707106781186548,0.707106781186547,0.707106781186547,
0.707106781186548,0.707106781186547,0.707106781186548,0.707106781186547,
0.707106781186547,0.707106781186548,0.707106781186548,0.707106781186547,
0.707106781186548,0.707106781186547,0.707106781186547,0.707106781186547,
0.707106781186548,0.707106781186547,0.707106781186547,0.707106781186548,
0.707106781186547,0.707106781186547,0.707106781186547,0.707106781186548,
0.707106781186548,0.707106781186547,0.707106781186548,0.707106781186547,
0.707106781186548,0.707106781186547,0.707106781186547,0.707106781186548,
0.707106781186547,0.707106781186548,0.707106781186547,0.707106781186547,
0.707106781186547,0.707106781186547,0.707106781186548,0.707106781186547,
0.707106781186547,0.707106781186547,0.707106781186547,0.707106781186547,
0.707106781186548,0.707106781186547,0.707106781186547,0.707106781186547,
0.707106781186547,0.707106781186548,0.707106781186547,0.707106781186548,
0.707106781186547,0.707106781186547,0.707106781186548,0.707106781186547,
0.707106781186548,0.707106781186547,0.707106781186547,0.707106781186548,
0.707106781186547,0.707106781186547,0.707106781186548,0.707106781186547,
0.707106781186547,0.707106781186547,0.707106781186547,0.707106781186548,
0.707106781186547,0.707106781186548,0.707106781186548,0.707106781186547,
0.707106781186548,0.707106781186548,0.707106781186547,0.707106781186547,
0.707106781186548,0.707106781186547,0.707106781186547,0.707106781186547,
0.707106781186548,0.707106781186547,0.707106781186547,0.707106781186548,
0.707106781186547,0.707106781186548,0.707106781186547,0.707106781186548,
0.707106781186547,0.707106781186547,0.707106781186548,0.707106781186547,
0.707106781186548,0.707106781186547,0.707106781186548,0.707106781186547,
0.707106781186548,0.707106781186547,0.707106781186548,0.707106781186547,
0.707106781186547,0.707106781186547,0.707106781186547,0.707106781186548,
0.707106781186548,0.707106781186547,0.707106781186548,0.707106781186548,
0.707106781186547,0.707106781186548,0.707106781186547,0.707106781186547,
0.707106781186548,0.707106781186547,0.707106781186547,0.707106781186547,
0.707106781186547,0.707106781186548,0.707106781186547,0.707106781186547,
0.707106781186547,0.707106781186548,0.707106781186547,0.707106781186547,
0.707106781186548,0.707106781186547,0.707106781186548,0.707106781186548,
0.707106781186547,0.707106781186548,0.707106781186547,0.707106781186548,
0.707106781186547,0.707106781186548,0.707106781186547,0.707106781186547,
0.707106781186548,0.707106781186547,0.707106781186548,0.707106781186548,
0.707106781186547,0.707106781186547,0.707106781186548,0.707106781186547,
0.707106781186548,0.707106781186547,0.707106781186548,0.707106781186547,
0.707106781186547,0.707106781186548,0.707106781186548,0.707106781186547,
0.707106781186548,0.707106781186548,0.707106781186547,0.707106781186548,
0.707106781186548,0.707106781186547,0.707106781186548,0.707106781186547,
0.707106781186548,0.707106781186547,0.707106781186548,0.707106781186547,
0.707106781186548,0.707106781186547,0.707106781186547,0.707106781186548,
0.707106781186547,0.707106781186547,0.707106781186548,0.707106781186547,
0.707106781186548,0.707106781186548,0.707106781186547,0.707106781186547,
0.707106781186547,0.707106781186548,0.707106781186547,0.707106781186548,
0.707106781186548,0.707106781186547,0.707106781186548,0.707106781186547,
0.707106781186548,0.707106781186547,0.707106781186548,0.707106781186547,
0.707106781186547,0.707106781186548,0.707106781186548,0.707106781186548,
0.707106781186547,0.707106781186548,0.707106781186548,0.707106781186547,
0.707106781186548,0.707106781186547,0.707106781186548,0.707106781186548,
0.707106781186548,0.707106781186548,0.707106781186548,0.707106781186548,
0.707106781186547,0.707106781186547,0.707106781186548,0.707106781186547,
0.707106781186547,0.707106781186548,0.707106781186547,0.707106781186547,
0.707106781186548,0.707106781186547,0.707106781186548,0.707106781186547,
0.707106781186548,0.707106781186547,0.707106781186547,0.707106781186547,
0.707106781186548,0.707106781186547,0.707106781186547,0.707106781186548,
0.707106781186547,0.707106781186548,0.707106781186547,0.707106781186548,
0.707106781186547,0.707106781186547,0.707106781186547,0.707106781186547,
0.707106781186548,0.707106781186547,0.707106781186547,0.707106781186548,
0.707106781186548,0.707106781186547,0.707106781186548,0.707106781186547,
0.707106781186548,0.707106781186547,0.707106781186547,0.707106781186548,
0.707106781186547,0.707106781186548,0.707106781186547,0.707106781186548,
0.707106781186547,0.707106781186548,0.707106781186548,0.707106781186547,
0.707106781186548,0.707106781186547,0.707106781186547,0.707106781186548,
0.707106781186547,0.707106781186547,0.707106781186548,0.707106781186548,
0.707106781186548,0.707106781186547,0.707106781186548,0.707106781186547,
0.707106781186547,0.707106781186547,0.707106781186548,0.707106781186547,
0.707106781186548,0.707106781186548,0.707106781186548,0.707106781186547,
0.707106781186547,0.707106781186547,0.707106781186547,0.707106781186548,
0.707106781186547,0.707106781186547,0.707106781186548,0.707106781186547,
0.707106781186548,0.707106781186547,0.707106781186547,0.707106781186548,
0.707106781186547,0.707106781186548,0.707106781186547,0.707106781186548,
0.707106781186547,0.707106781186547,0.707106781186547,0.707106781186547,
0.707106781186547,0.707106781186547,0.707106781186548,0.707106781186547,
0.707106781186547,0.707106781186548,0.707106781186548,0.707106781186547,
0.707106781186548,0.707106781186548,0.707106781186547,0.707106781186547,
0.707106781186548,0.707106781186547,0.707106781186547,0.707106781186548,
0.707106781186547,0.707106781186548,0.707106781186548,0.707106781186548,
0.707106781186547,0.707106781186547,0.707106781186547,0.707106781186547,
0.707106781186548,0.707106781186548,0.707106781186548,0.707106781186547,
0.707106781186548,0.707106781186547,0.707106781186548,0.707106781186548,
0.707106781186547,0.707106781186548,0.707106781186547,0.707106781186548,
0.707106781186548,0.707106781186547,0.707106781186547,0.707106781186548,
0.707106781186547,0.707106781186548,0.707106781186547,0.707106781186548,
0.707106781186548,0.707106781186548,0.707106781186547,0.707106781186548,
0.707106781186547,0.707106781186547,0.707106781186547,0.707106781186547,
0.707106781186548,0.707106781186548,0.707106781186547,0.707106781186547,
0.707106781186547,0.707106781186548,0.707106781186547,0.707106781186547,
0.707106781186548,0.707106781186547,0.707106781186548,0.707106781186548,
0.707106781186548,0.707106781186547,0.707106781186547,0.707106781186547,
0.707106781186547,0.707106781186548,0.707106781186548,0.707106781186547,
0.707106781186548,0.707106781186547,0.707106781186548,0.707106781186548,
0.707106781186547,0.707106781186548,0.707106781186547,0.707106781186548,
0.707106781186547,0.707106781186547,0.707106781186547,0.707106781186548,
0.707106781186547,0.707106781186548,0.707106781186547,0.707106781186548,
0.707106781186547,0.707106781186548,0.707106781186547,0.707106781186548,
0.707106781186547,0.707106781186547,0.707106781186548,0.707106781186547,
0.707106781186548,0.707106781186547,0.707106781186547,0.707106781186548,
0.707106781186548,0.707106781186547,0.707106781186548,0.707106781186548,
0.707106781186547,0.707106781186548,0.707106781186547,0.707106781186548,
0.707106781186547,0.707106781186547,0.707106781186547,0.707106781186548,
0.707106781186547,0.707106781186547,0.707106781186548,0.707106781186547,
0.707106781186548,0.707106781186547,0.707106781186548,0.707106781186548,
0.707106781186547,0.707106781186548,0.707106781186547,0.707106781186548,
0.707106781186548,0.707106781186548,0.707106781186548,0.707106781186547,
0.707106781186547,0.707106781186548,0.707106781186547,0.707106781186547,
0.707106781186548,0.707106781186548,0.707106781186547,0.707106781186547,
0.707106781186548,0.707106781186547,0.707106781186547,0.707106781186548,
0.707106781186547,0.707106781186548,0.707106781186547,0.707106781186548,
0.707106781186547,0.707106781186547,0.707106781186547,0.707106781186548,
0.707106781186547,0.707106781186547,0.707106781186548,0.707106781186547,
0.707106781186548,0.707106781186548,0.707106781186548,0.707106781186547,
0.707106781186547,0.707106781186547,0.707106781186548,0.707106781186548,
0.707106781186547,0.707106781186547,0.707106781186547,0.707106781186547,
0.707106781186548,0.707106781186548,0.707106781186547,0.707106781186547,
0.707106781186547,0.707106781186548,0.707106781186548,0.707106781186547,
0.707106781186548,0.707106781186547,0.707106781186548,0.707106781186547,
0.707106781186548,0.707106781186548,0.707106781186547,0.707106781186548,
0.707106781186548,0.707106781186548,0.707106781186547,0.707106781186547,
0.707106781186547,0.707106781186548,0.707106781186548,0.707106781186548,
0.707106781186547,0.707106781186547,0.707106781186548,0.707106781186548,
0.707106781186547,0.707106781186548,0.707106781186547,0.707106781186547,
0.707106781186548,0.707106781186547,0.707106781186548,0.707106781186547,
0.707106781186547,0.707106781186548,0.707106781186547,0.707106781186548,
0.707106781186548,0.707106781186547,0.707106781186547,0.707106781186548,
0.707106781186547,0.707106781186548,0.707106781186547,0.707106781186547,
0.707106781186548,0.707106781186547,0.707106781186548,0.707106781186547,
0.707106781186548,0.707106781186547,0.707106781186547,0.707106781186548,
0.707106781186547,0.707106781186547,0.707106781186547,0.707106781186547,
0.707106781186547,0.707106781186547,0.707106781186548,0.707106781186547,
0.707106781186548,0.707106781186548,0.707106781186548,0.707106781186547,
0.707106781186547,0.707106781186547,0.707106781186548,0.707106781186547,
0.707106781186548,0.707106781186547,0.707106781186547,0.707106781186548,
0.707106781186547,0.707106781186547,0.707106781186547,0.707106781186547,
0.707106781186547,0.707106781186548,0.707106781186547,0.707106781186548,
0.707106781186547,0.707106781186547,0.707106781186548,0.707106781186548,
0.707106781186547,0.707106781186547,0.707106781186547,0.707106781186548,
0.707106781186547,0.707106781186547,0.707106781186548,0.707106781186548,
0.707106781186547,0.707106781186548,0.707106781186547,0.707106781186548,
0.707106781186548,0.707106781186547,0.707106781186547,0.707106781186547,
0.707106781186548,0.707106781186548,0.707106781186547,0.707106781186548,
0.707106781186547,0.707106781186548,0.707106781186548,0.707106781186547,
0.707106781186548,0.707106781186547,0.707106781186547,0.707106781186547,
0.707106781186548,0.707106781186547,0.707106781186548,0.707106781186547,
0.707106781186548,0.707106781186547,0.707106781186547,0.707106781186547,
0.707106781186547,0.707106781186547,0.707106781186548,0.707106781186547,
0.707106781186548,0.707106781186547,0.707106781186548,0.707106781186547,
0.707106781186548,0.707106781186547,0.707106781186547,0.707106781186547,
0.707106781186547,0.707106781186547,0.707106781186548,0.707106781186548,
0.707106781186548,0.707106781186547,0.707106781186548,0.707106781186547,
0.707106781186548,0.707106781186547,0.707106781186547,0.707106781186548,
0.707106781186547,0.707106781186548,0.707106781186547,0.707106781186547,
0.707106781186547,0.707106781186548,0.707106781186548,0.707106781186547,
0.707106781186548,0.707106781186547,0.707106781186548,0.707106781186548,
0.707106781186547,0.707106781186548,0.707106781186547,0.707106781186548,
0.707106781186548,0.707106781186547,0.707106781186547,0.707106781186547,
0.707106781186547,0.707106781186547,0.707106781186547,0.707106781186548,
0.707106781186548,0.707106781186547,0.707106781186548,0.707106781186547,
0.707106781186547,0.707106781186548,0.707106781186547,0.707106781186547,
0.707106781186548,0.707106781186547,0.707106781186547,0.707106781186547,
0.707106781186548,0.707106781186547,0.707106781186547,0.707106781186548,
0.707106781186547,0.707106781186548,0.707106781186548,0.707106781186547,
0.707106781186547,0.707106781186547,0.707106781186548,0.707106781186547,
0.707106781186547,0.707106781186548,0.707106781186548,0.707106781186548,
0.707106781186548,0.707106781186547,0.707106781186548,0.707106781186548,
0.707106781186547,0.707106781186547,0.707106781186548,0.707106781186547,
0.707106781186548,0.707106781186547,0.707106781186547,0.707106781186548,
0.707106781186547,0.707106781186547,0.707106781186548,0.707106781186547,
0.707106781186548,0.707106781186547,0.707106781186548,0.707106781186547,
0.707106781186548,0.707106781186547,0.707106781186548,0.707106781186547,
0.707106781186548,0.707106781186548,0.707106781186547,0.707106781186547,
0.707106781186548,0.707106781186548,0.707106781186547,0.707106781186547,
0.707106781186547,0.707106781186547,0.707106781186547,0.707106781186548,
0.707106781186547,0.707106781186547,0.707106781186548,0.707106781186547,
0.707106781186548,0.707106781186548,0.707106781186547,0.707106781186548,
0.707106781186547,0.707106781186548,0.707106781186547,0.707106781186548,
0.707106781186547,0.707106781186547,0.707106781186547,0.707106781186547,
0.707106781186547,0.707106781186547,0.707106781186548,0.707106781186547,
0.707106781186548,0.707106781186547,0.707106781186547,0.707106781186547,
0.707106781186548,0.707106781186547,0.707106781186548,0.707106781186548,
0.707106781186547,0.707106781186547,0.707106781186548,0.707106781186547,
0.707106781186548,0.707106781186547,0.707106781186548,0.707106781186547,
0.707106781186548,0.707106781186547,0.707106781186547,0.707106781186548,
0.707106781186547,0.707106781186548,0.707106781186547,0.707106781186548,
0.707106781186548,0.707106781186548,0.707106781186548,0.707106781186547,
0.707106781186548,0.707106781186548,0.707106781186548,0.707106781186547,
0.707106781186548,0.707106781186548,0.707106781186547,0.707106781186548,
0.707106781186547,0.707106781186548,0.707106781186547,0.707106781186547,
0.707106781186547,0.707106781186548,0.707106781186548,0.707106781186547,
0.707106781186548,0.707106781186547,0.707106781186548,0.707106781186547,
0.707106781186548,0.707106781186548,0.707106781186547,0.707106781186548,
0.707106781186547,0.707106781186547,0.707106781186548,0.707106781186547,
0.707106781186547,0.707106781186547,0.707106781186548,0.707106781186547,
0.707106781186548,0.707106781186548,0.707106781186547,0.707106781186548,
0.707106781186547,0.707106781186548,0.707106781186548,0.707106781186548,
0.707106781186548,0.707106781186547,0.707106781186548,0.707106781186547,
0.707106781186548,0.707106781186547,0.707106781186548,0.707106781186547,
0.707106781186547,0.707106781186547,0.707106781186547,0.707106781186548,
0.707106781186547,0.707106781186548,0.707106781186547,0.707106781186547,
0.707106781186548,0.707106781186547,0.707106781186548,0.707106781186547,
0.707106781186548,0.707106781186547,0.707106781186548,0.707106781186548,
0.707106781186548,0.707106781186548,0.707106781186547,0.707106781186548,
0.707106781186548,0.707106781186547,0.707106781186548,0.707106781186547,
0.707106781186548,0.707106781186547,0.707106781186548,0.707106781186547,
0.707106781186547,0.707106781186548,0.707106781186547,0.707106781186548,
0.707106781186547,0.707106781186547,0.707106781186548,0.707106781186547,
0.707106781186548,0.707106781186547,0.707106781186547,0.707106781186548,
0.707106781186548,0.707106781186548,0.707106781186548,0.707106781186548,
0.707106781186548,0.707106781186548,0.707106781186548,0.707106781186548,
0.707106781186547,0.707106781186548,0.707106781186547,0.707106781186547,
0.707106781186548,0.707106781186547,0.707106781186548,0.707106781186548,
0.707106781186547,0.707106781186547,0.707106781186548,0.707106781186548,
0.707106781186547,0.707106781186547,0.707106781186547,0.707106781186547,
0.707106781186547,0.707106781186548,0.707106781186547,0.707106781186548,
0.707106781186548,0.707106781186548,0.707106781186547,0.707106781186548,
0.707106781186547,0.707106781186548,0.707106781186547,0.707106781186548,
0.707106781186547,0.707106781186548,0.707106781186548,0.707106781186547,
0.707106781186547,0.707106781186548,0.707106781186548,0.707106781186548,
0.707106781186547,0.707106781186547,0.707106781186548,0.707106781186547,
0.707106781186547,0.707106781186548,0.707106781186547,0.707106781186548,
0.707106781186547,0.707106781186547,0.707106781186548,0.707106781186548,
0.707106781186548,0.707106781186547,0.707106781186547,0.707106781186548,
0.707106781186547,0.707106781186548,0.707106781186547,0.707106781186548,
0.707106781186547,0.707106781186548,0.707106781186548,0.707106781186547,
0.707106781186548,0.707106781186547,0.707106781186548,0.707106781186547,
0.707106781186547,0.707106781186547,0.707106781186548,0.707106781186547,
0.707106781186548,0.707106781186547,0.707106781186547,0.707106781186547,
0.707106781186548,0.707106781186547,0.707106781186547,0.707106781186548,
0.707106781186548,0.707106781186547,0.707106781186548,0.707106781186547,
0.707106781186548,0.707106781186548,0.707106781186547,0.707106781186548,
0.707106781186547,0.707106781186547,0.707106781186548,0.707106781186547,
0.707106781186547,0.707106781186547,0.707106781186548,0.707106781186547,
0.707106781186548,0.707106781186547,0.707106781186548,0.707106781186548,
0.707106781186548,0.707106781186547,0.707106781186548,0.707106781186548,
0.707106781186548,0.707106781186547,0.707106781186548,0.707106781186547,
0.707106781186547,0.707106781186548,0.707106781186547,0.707106781186547,
0.707106781186548,0.707106781186548,0.707106781186547,0.707106781186548,
0.707106781186547,0.707106781186548,0.707106781186548,0.707106781186547,
0.707106781186548,0.707106781186547,0.707106781186548,0.707106781186547,
0.707106781186548,0.707106781186547,0.707106781186548,0.707106781186548,
0.707106781186548,0.707106781186547,0.707106781186548,0.707106781186548,
0.707106781186547,0.707106781186547,0.707106781186548,0.707106781186547,
0.707106781186548,0.707106781186548,0.707106781186547,0.707106781186548,
0.707106781186548,0.707106781186547,0.707106781186548,0.707106781186548,
0.707106781186547,0.707106781186547,0.707106781186548,0.707106781186547,
0.707106781186548,0.707106781186547,0.707106781186548,0.707106781186547,
0.707106781186548,0.707106781186548,0.707106781186548,0.707106781186547,
0.707106781186548,0.707106781186547,0.707106781186548,0.707106781186547,
0.707106781186548,0.707106781186547,0.707106781186548,0.707106781186547,
0.707106781186548,0.707106781186547,0.707106781186548,0.707106781186547,
0.707106781186547,0.707106781186547,0.707106781186548,0.707106781186547,
0.707106781186548,0.707106781186547,0.707106781186548,0.707106781186547,
0.707106781186548,0.707106781186547,0.707106781186548,0.707106781186548,
0.707106781186548,0.707106781186547,0.707106781186548,0.707106781186547,
0.707106781186548,0.707106781186548,0.707106781186547,0.707106781186548,
0.707106781186547,0.707106781186548,0.707106781186547,0.707106781186548,
0.707106781186547,0.707106781186548,0.707106781186547,0.707106781186547,
0.707106781186547,0.707106781186548,0.707106781186547,0.707106781186547,
0.707106781186548,0.707106781186547,0.707106781186548,0.707106781186547,
0.707106781186547,0.707106781186548,0.707106781186547,0.707106781186548,
0.707106781186547,0.707106781186548,0.707106781186548,0.707106781186548,
0.707106781186547,0.707106781186547,0.707106781186548,0.707106781186548,
0.707106781186547,0.707106781186548,0.707106781186547,0.707106781186547,
0.707106781186547,0.707106781186548,0.707106781186547,0.707106781186548,
0.707106781186547,0.707106781186548,0.707106781186548,0.707106781186548,
0.707106781186547,0.707106781186547,0.707106781186547,0.707106781186547,
0.707106781186547,0.707106781186547,0.707106781186548,0.707106781186547,
0.707106781186548,0.707106781186547,0.707106781186548,0.707106781186547,
0.707106781186547,0.707106781186548,0.707106781186547,0.707106781186547,
0.707106781186548,0.707106781186548,0.707106781186547,0.707106781186547,
0.707106781186547,0.707106781186548,0.707106781186547,0.707106781186547,
0.707106781186548,0.707106781186548),(1.,1.,1.,1.,1.,1.,1.,1.,1.,1.,1.,
1.,1.,1.,1.,1.,1.,1.,1.,1.,1.,1.,1.,1.,1.,1.,1.,1.,1.,1.,1.,1.,1.,1.,1.,
1.,1.,1.,1.,1.,1.,1.,1.,1.,1.,1.,1.,1.,1.,1.,1.,1.,1.,1.,1.,1.,1.,1.,1.,
1.,1.,1.,1.,1.,1.,1.,1.,1.,1.,1.,1.,1.,1.,1.,1.,1.,1.,1.,1.,1.,1.,1.,1.,
1.,1.,1.,1.,1.,1.,1.,1.,1.,1.,1.,1.,1.,1.,1.,1.,1.,1.,1.,1.,1.,1.,1.,1.,
1.,1.,1.,1.,1.,1.,1.,1.,1.,1.,1.,1.,1.,1.,1.,1.,1.,1.,1.,1.,1.,1.,1.,1.,
1.,1.,1.,1.,1.,1.,1.,1.,1.,1.,1.,1.,1.,1.,1.,1.,1.,1.,1.,1.,1.,1.,1.,1.,
1.,1.,1.,1.,1.,1.,1.,1.,1.,1.,1.,1.,1.,1.,1.,1.,1.,1.,1.,1.,1.,1.,1.,1.,
1.,1.,1.,1.,1.,1.,1.,1.,1.,1.,1.,1.,1.,1.,1.,1.,1.,1.,1.,1.,1.,1.,1.,1.,
1.,1.,1.,1.,1.,1.,1.,1.,1.,1.,1.,1.,1.,1.,1.,1.,1.,1.,1.,1.,1.,1.,1.,1.,
1.,1.,1.,1.,1.,1.,1.,1.,1.,1.,1.,1.,1.,1.,1.,1.,1.,1.,1.,1.,1.,1.,1.,1.,
1.,1.,1.,1.,1.,1.,1.,1.,1.,1.,1.,1.,1.,1.,1.,1.,1.,1.,1.,1.,1.,1.,1.,1.,
1.,1.,1.,1.,1.,1.,1.,1.,1.,1.,1.,1.,1.,1.,1.,1.,1.,1.,1.,1.,1.,1.,1.,1.,
1.,1.,1.,1.,1.,1.,1.,1.,1.,1.,1.,1.,1.,1.,1.,1.,1.,1.,1.,1.,1.,1.,1.,1.,
1.,1.,1.,1.,1.,1.,1.,1.,1.,1.,1.,1.,1.,1.,1.,1.,1.,1.,1.,1.,1.,1.,1.,1.,
1.,1.,1.,1.,1.,1.,1.,1.,1.,1.,1.,1.,1.,1.,1.,1.,1.,1.,1.,1.,1.,1.,1.,1.,
1.,1.,1.,1.,1.,1.,1.,1.,1.,1.,1.,1.,1.,1.,1.,1.,1.,1.,1.,1.,1.,1.,1.,1.,
1.,1.,1.,1.,1.,1.,1.,1.,1.,1.,1.,1.,1.,1.,1.,1.,1.,1.,1.,1.,1.,1.,1.,1.,
1.,1.,1.,1.,1.,1.,1.,1.,1.,1.,1.,1.,1.,1.,1.,1.,1.,1.,1.,1.,1.,1.,1.,1.,
1.,1.,1.,1.,1.,1.,1.,1.,1.,1.,1.,1.,1.,1.,1.,1.,1.,1.,1.,1.,1.,1.,1.,1.,
1.,1.,1.,1.,1.,1.,1.,1.,1.,1.,1.,1.,1.,1.,1.,1.,1.,1.,1.,1.,1.,1.,1.,1.,
1.,1.,1.,1.,1.,1.,1.,1.,1.,1.,1.,1.,1.,1.,1.,1.,1.,1.,1.,1.,1.,1.,1.,1.,
1.,1.,1.,1.,1.,1.,1.,1.,1.,1.,1.,1.,1.,1.,1.,1.,1.,1.,1.,1.,1.,1.,1.,1.,
1.,1.,1.,1.,1.,1.,1.,1.,1.,1.,1.,1.,1.,1.,1.,1.,1.,1.,1.,1.,1.,1.,1.,1.,
1.,1.,1.,1.,1.,1.,1.,1.,1.,1.,1.,1.,1.,1.,1.,1.,1.,1.,1.,1.,1.,1.,1.,1.,
1.,1.,1.,1.,1.,1.,1.,1.,1.,1.,1.,1.,1.,1.,1.,1.,1.,1.,1.,1.,1.,1.,1.,1.,
1.,1.,1.,1.,1.,1.,1.,1.,1.,1.,1.,1.,1.,1.,1.,1.,1.,1.,1.,1.,1.,1.,1.,1.,
1.,1.,1.,1.,1.,1.,1.,1.,1.,1.,1.,1.,1.,1.,1.,1.,1.,1.,1.,1.,1.,1.,1.,1.,
1.,1.,1.,1.,1.,1.,1.,1.,1.,1.,1.,1.,1.,1.,1.,1.,1.,1.,1.,1.,1.,1.,1.,1.,
1.,1.,1.,1.,1.,1.,1.,1.,1.,1.,1.,1.,1.,1.,1.,1.,1.,1.,1.,1.,1.,1.,1.,1.,
1.,1.,1.,1.,1.,1.,1.,1.,1.,1.,1.,1.,1.,1.,1.,1.,1.,1.,1.,1.,1.,1.,1.,1.,
1.,1.,1.,1.,1.,1.,1.,1.,1.,1.,1.,1.,1.,1.,1.,1.,1.,1.,1.,1.,1.,1.,1.,1.,
1.,1.,1.,1.,1.,1.,1.,1.,1.,1.,1.,1.,1.,1.,1.,1.,1.,1.,1.,1.,1.,1.,1.,1.,
1.,1.,1.,1.,1.,1.,1.,1.,1.,1.,1.,1.,1.,1.,1.,1.,1.,1.,1.,1.,1.,1.,1.,1.,
1.,1.,1.,1.,1.,1.,1.,1.,1.,1.,1.,1.,1.,1.,1.,1.,1.,1.,1.,1.,1.,1.,1.,1.,
1.,1.,1.,1.,1.,1.,1.,1.,1.,1.,1.,1.,1.,1.,1.,1.,1.,1.,1.,1.,1.,1.,1.,1.,
1.,1.,1.,1.,1.,1.,1.,1.,1.,1.,1.,1.,1.,1.,1.,1.,1.,1.,1.,1.,1.,1.,1.,1.,
1.,1.,1.,1.,1.,1.,1.,1.,1.,1.,1.,1.,1.,1.,1.,1.,1.,1.,1.,1.,1.,1.,1.,1.,
1.,1.,1.,1.,1.,1.,1.,1.,1.,1.,1.,1.,1.,1.,1.,1.,1.,1.,1.,1.,1.,1.,1.,1.,
1.,1.,1.,1.,1.,1.,1.,1.,1.,1.,1.,1.,1.,1.,1.,1.,1.,1.,1.,1.,1.,1.,1.,1.,
1.,1.,1.,1.,1.,1.,1.,1.,1.,1.,1.,1.,1.,1.,1.,1.,1.,1.,1.,1.,1.,1.,1.,1.,
1.,1.,1.,1.,1.,1.,1.,1.,1.,1.,1.,1.,1.,1.,1.,1.,1.,1.,1.,1.,1.,1.,1.,1.,
1.,1.,1.,1.,1.,1.,1.,1.,1.,1.,1.,1.,1.,1.,1.,1.,1.,1.,1.,1.,1.,1.,1.,1.,
1.,1.,1.,1.,1.,1.,1.,1.,1.,1.,1.,1.,1.,1.,1.,1.,1.,1.,1.,1.,1.,1.,1.,1.,
1.,1.,1.,1.,1.,1.,1.,1.,1.,1.,1.,1.,1.,1.,1.,1.,1.,1.,1.,1.,1.,1.,1.,1.,
1.,1.,1.,1.,1.,1.,1.,1.,1.,1.,1.,1.,1.,1.,1.,1.,1.,1.,1.,1.,1.,1.,1.,1.,
1.,1.,1.,1.,1.,1.,1.,1.,1.,1.,1.,1.,1.,1.,1.,1.,1.,1.,1.,1.,1.,1.,1.,1.,
1.,1.,1.,1.,1.,1.,1.,1.,1.,1.,1.,1.,1.,1.,1.,1.,1.,1.,1.,1.,1.,1.,1.,1.,
1.,1.,1.,1.,1.,1.,1.,1.,1.,1.,1.,1.,1.,1.,1.,1.,1.,1.,1.,1.,1.,1.,1.,1.,
1.,1.,1.,1.,1.,1.,1.,1.,1.,1.,1.,1.,1.,1.,1.,1.,1.,1.,1.,1.,1.,1.,1.,1.,
1.,1.,1.,1.,1.,1.,1.,1.,1.,1.,1.,1.,1.,1.,1.,1.,1.,1.,1.,1.,1.,1.,1.,1.,
1.,1.,1.,1.,1.,1.,1.,1.,1.,1.,1.,1.,1.,1.,1.,1.,1.,1.,1.,1.,1.,1.,1.,1.,
1.,1.,1.,1.,1.,1.,1.,1.,1.,1.,1.,1.,1.,1.,1.,1.,1.,1.,1.,1.,1.,1.,1.,1.,
1.,1.,1.,1.,1.,1.,1.,1.,1.,1.,1.,1.,1.,1.,1.,1.,1.,1.,1.,1.,1.,1.,1.,1.,
1.,1.,1.,1.,1.,1.,1.,1.,1.,1.,1.,1.,1.,1.,1.,1.,1.,1.,1.,1.,1.,1.,1.,1.,
1.,1.,1.,1.,1.,1.,1.,1.,1.,1.,1.,1.,1.,1.,1.,1.,1.,1.,1.,1.,1.,1.,1.,1.,
1.,1.,1.,1.,1.,1.,1.,1.,1.,1.,1.,1.,1.,1.,1.,1.,1.,1.,1.,1.,1.,1.,1.,1.,
1.,1.,1.,1.,1.,1.,1.,1.,1.,1.,1.,1.,1.,1.,1.,1.,1.,1.,1.,1.,1.,1.,1.,1.,
1.,1.,1.,1.,1.,1.,1.,1.,1.,1.,1.,1.,1.,1.,1.,1.,1.,1.,1.,1.,1.,1.,1.,1.,
1.,1.,1.,1.,1.,1.,1.,1.,1.,1.,1.,1.,1.,1.,1.,1.,1.,1.,1.,1.,1.,1.,1.,1.,
1.,1.,1.,1.,1.,1.,1.,1.,1.,1.,1.,1.,1.,1.,1.,1.,1.,1.,1.,1.,1.,1.,1.,1.,
1.,1.,1.,1.,1.,1.,1.,1.,1.,1.,1.,1.,1.,1.,1.,1.,1.,1.,1.,1.,1.,1.,1.,1.,
1.,1.,1.,1.,1.,1.,1.,1.,1.,1.,1.,1.,1.,1.,1.,1.,1.,1.,1.,1.,1.,1.,1.,1.,
1.,1.,1.,1.,1.,1.,1.,1.,1.,1.,1.,1.,1.,1.,1.,1.,1.,1.,1.,1.,1.,1.,1.,1.,
1.,1.,1.,1.,1.,1.,1.,1.,1.,1.,1.,1.,1.,1.,1.,1.,1.,1.,1.,1.,1.,1.,1.,1.,
1.,1.,1.,1.,1.,1.,1.,1.,1.,1.,1.,1.,1.,1.,1.,1.,1.,1.,1.,1.,1.,1.,1.,1.,
1.,1.,1.,1.,1.,1.,1.,1.,1.,1.,1.,1.,1.,1.,1.,1.,1.,1.,1.,1.,1.,1.,1.,1.,
1.,1.,1.,1.,1.,1.,1.,1.,1.,1.,1.,1.,1.,1.,1.,1.,1.,1.,1.,1.,1.,1.,1.,1.,
1.,1.,1.,1.,1.,1.,1.,1.,1.,1.,1.,1.,1.,1.,1.,1.,1.,1.,1.,1.,1.,1.,1.,1.,
1.,1.,1.,1.,1.,1.,1.,1.,1.,1.,1.,1.,1.,1.,1.,1.,1.,1.,1.,1.,1.,1.,1.,1.,
1.,1.,1.,1.,1.,1.,1.,1.,1.,1.,1.,1.,1.,1.,1.,1.,1.,1.,1.,1.,1.,1.,1.,1.,
1.,1.,1.,1.,1.,1.,1.,1.,1.,1.,1.,1.,1.,1.,1.,1.,1.,1.,1.,1.,1.,1.,1.,1.,
1.,1.,1.,1.,1.,1.,1.,1.,1.,1.,1.,1.,1.,1.,1.,1.,1.,1.,1.,1.,1.,1.,1.,1.,
1.,1.,1.,1.,1.,1.,1.,1.,1.,1.,1.,1.,1.,1.,1.,1.,1.,1.,1.,1.,1.,1.,1.,1.,
1.,1.,1.,1.,1.,1.,1.,1.,1.,1.,1.,1.,1.,1.,1.,1.,1.,1.,1.,1.,1.,1.,1.,1.,
1.,1.,1.,1.,1.,1.,1.,1.,1.,1.,1.,1.,1.,1.,1.,1.,1.,1.,1.,1.,1.,1.,1.,1.,
1.,1.,1.,1.,1.,1.,1.,1.,1.,1.,1.,1.,1.,1.,1.,1.,1.,1.,1.,1.,1.,1.,1.,1.,
1.,1.,1.,1.,1.,1.,1.,1.,1.,1.,1.,1.,1.,1.,1.,1.,1.,1.,1.,1.,1.,1.,1.,1.,
1.,1.,1.,1.,1.,1.,1.,1.,1.,1.,1.,1.,1.,1.,1.,1.,1.,1.,1.,1.,1.,1.,1.,1.,
1.,1.,1.,1.,1.,1.,1.,1.,1.,1.,1.,1.,1.,1.,1.,1.,1.,1.,1.,1.,1.,1.,1.,1.,
1.,1.,1.,1.,1.,1.,1.,1.,1.,1.,1.,1.,1.,1.,1.,1.,1.,1.,1.,1.,1.,1.,1.,1.,
1.,1.,1.,1.,1.,1.,1.,1.,1.,1.,1.,1.,1.,1.,1.,1.,1.,1.,1.,1.,1.,1.,1.,1.,
1.,1.,1.,1.,1.,1.,1.,1.,1.,1.,1.,1.,1.,1.,1.,1.,1.,1.,1.,1.,1.,1.,1.,1.,
1.,1.,1.,1.,1.,1.,1.,1.,1.,1.,1.,1.,1.,1.,1.,1.,1.,1.,1.,1.,1.,1.,1.,1.,
1.,1.,1.,1.,1.,1.,1.,1.,1.,1.,1.,1.,1.,1.,1.,1.,1.,1.,1.,1.,1.,1.,1.,1.,
1.,1.,1.,1.,1.,1.,1.,1.,1.,1.,1.,1.,1.,1.,1.,1.,1.,1.,1.,1.,1.,1.,1.,1.),
(0.707106781186548,0.707106781186548,0.707106781186548,0.707106781186547,
0.707106781186547,0.707106781186548,0.707106781186547,0.707106781186547,
0.707106781186547,0.707106781186547,0.707106781186547,0.707106781186548,
0.707106781186548,0.707106781186548,0.707106781186547,0.707106781186548,
0.707106781186547,0.707106781186547,0.707106781186548,0.707106781186547,
0.707106781186548,0.707106781186547,0.707106781186548,0.707106781186547,
0.707106781186548,0.707106781186547,0.707106781186547,0.707106781186547,
0.707106781186547,0.707106781186547,0.707106781186548,0.707106781186547,
0.707106781186547,0.707106781186548,0.707106781186547,0.707106781186547,
0.707106781186548,0.707106781186547,0.707106781186547,0.707106781186548,
0.707106781186548,0.707106781186547,0.707106781186548,0.707106781186547,
0.707106781186547,0.707106781186547,0.707106781186548,0.707106781186548,
0.707106781186547,0.707106781186547,0.707106781186548,0.707106781186547,
0.707106781186548,0.707106781186547,0.707106781186547,0.707106781186547,
0.707106781186547,0.707106781186547,0.707106781186548,0.707106781186547,
0.707106781186548,0.707106781186547,0.707106781186548,0.707106781186547,
0.707106781186548,0.707106781186547,0.707106781186547,0.707106781186548,
0.707106781186547,0.707106781186547,0.707106781186548,0.707106781186547,
0.707106781186548,0.707106781186547,0.707106781186548,0.707106781186548,
0.707106781186547,0.707106781186548,0.707106781186547,0.707106781186547,
0.707106781186548,0.707106781186547,0.707106781186547,0.707106781186547,
0.707106781186548,0.707106781186547,0.707106781186547,0.707106781186547,
0.707106781186547,0.707106781186547,0.707106781186547,0.707106781186548,
0.707106781186548,0.707106781186547,0.707106781186548,0.707106781186547,
0.707106781186548,0.707106781186548,0.707106781186547,0.707106781186548,
0.707106781186548,0.707106781186548,0.707106781186547,0.707106781186548,
0.707106781186547,0.707106781186548,0.707106781186548,0.707106781186548,
0.707106781186547,0.707106781186547,0.707106781186547,0.707106781186548,
0.707106781186548,0.707106781186548,0.707106781186547,0.707106781186547,
0.707106781186547,0.707106781186548,0.707106781186548,0.707106781186547,
0.707106781186547,0.707106781186548,0.707106781186547,0.707106781186547,
0.707106781186547,0.707106781186547,0.707106781186548,0.707106781186547,
0.707106781186548,0.707106781186547,0.707106781186547,0.707106781186547,
0.707106781186548,0.707106781186548,0.707106781186547,0.707106781186548,
0.707106781186548,0.707106781186547,0.707106781186548,0.707106781186547,
0.707106781186548,0.707106781186547,0.707106781186548,0.707106781186547,
0.707106781186547,0.707106781186548,0.707106781186547,0.707106781186547,
0.707106781186548,0.707106781186547,0.707106781186547,0.707106781186548,
0.707106781186547,0.707106781186548,0.707106781186547,0.707106781186547,
0.707106781186548,0.707106781186548,0.707106781186547,0.707106781186548,
0.707106781186547,0.707106781186548,0.707106781186547,0.707106781186548,
0.707106781186547,0.707106781186548,0.707106781186547,0.707106781186548,
0.707106781186547,0.707106781186548,0.707106781186547,0.707106781186548,
0.707106781186547,0.707106781186547,0.707106781186548,0.707106781186547,
0.707106781186548,0.707106781186547,0.707106781186548,0.707106781186547,
0.707106781186548,0.707106781186547,0.707106781186547,0.707106781186548,
0.707106781186547,0.707106781186548,0.707106781186548,0.707106781186548,
0.707106781186547,0.707106781186547,0.707106781186547,0.707106781186547,
0.707106781186548,0.707106781186547,0.707106781186548,0.707106781186548,
0.707106781186547,0.707106781186547,0.707106781186548,0.707106781186548,
0.707106781186547,0.707106781186547,0.707106781186548,0.707106781186547,
0.707106781186548,0.707106781186547,0.707106781186547,0.707106781186547,
0.707106781186547,0.707106781186547,0.707106781186547,0.707106781186547,
0.707106781186548,0.707106781186547,0.707106781186548,0.707106781186547,
0.707106781186548,0.707106781186548,0.707106781186547,0.707106781186548,
0.707106781186548,0.707106781186548,0.707106781186548,0.707106781186547,
0.707106781186548,0.707106781186547,0.707106781186548,0.707106781186547,
0.707106781186547,0.707106781186548,0.707106781186548,0.707106781186547,
0.707106781186547,0.707106781186547,0.707106781186547,0.707106781186547,
0.707106781186548,0.707106781186548,0.707106781186547,0.707106781186547,
0.707106781186548,0.707106781186548,0.707106781186547,0.707106781186548,
0.707106781186547,0.707106781186548,0.707106781186548,0.707106781186547,
0.707106781186547,0.707106781186548,0.707106781186547,0.707106781186547,
0.707106781186548,0.707106781186547,0.707106781186548,0.707106781186547,
0.707106781186548,0.707106781186547,0.707106781186547,0.707106781186548,
0.707106781186548,0.707106781186547,0.707106781186547,0.707106781186548,
0.707106781186547,0.707106781186547,0.707106781186548,0.707106781186547,
0.707106781186548,0.707106781186547,0.707106781186548,0.707106781186547,
0.707106781186548,0.707106781186547,0.707106781186547,0.707106781186547,
0.707106781186547,0.707106781186547,0.707106781186547,0.707106781186548,
0.707106781186547,0.707106781186548,0.707106781186547,0.707106781186548,
0.707106781186548,0.707106781186547,0.707106781186548,0.707106781186548,
0.707106781186547,0.707106781186548,0.707106781186547,0.707106781186547,
0.707106781186547,0.707106781186548,0.707106781186547,0.707106781186547,
0.707106781186548,0.707106781186547,0.707106781186548,0.707106781186547,
0.707106781186547,0.707106781186547,0.707106781186548,0.707106781186548,
0.707106781186547,0.707106781186548,0.707106781186548,0.707106781186547,
0.707106781186548,0.707106781186547,0.707106781186548,0.707106781186548,
0.707106781186547,0.707106781186548,0.707106781186548,0.707106781186548,
0.707106781186547,0.707106781186547,0.707106781186548,0.707106781186547,
0.707106781186548,0.707106781186547,0.707106781186547,0.707106781186548,
0.707106781186548,0.707106781186548,0.707106781186547,0.707106781186547,
0.707106781186548,0.707106781186548,0.707106781186547,0.707106781186547,
0.707106781186548,0.707106781186547,0.707106781186547,0.707106781186548,
0.707106781186548,0.707106781186547,0.707106781186547,0.707106781186547,
0.707106781186548,0.707106781186547,0.707106781186547,0.707106781186547,
0.707106781186548,0.707106781186548,0.707106781186547,0.707106781186548,
0.707106781186547,0.707106781186548,0.707106781186547,0.707106781186548,
0.707106781186548,0.707106781186547,0.707106781186547,0.707106781186548,
0.707106781186547,0.707106781186547,0.707106781186548,0.707106781186547,
0.707106781186548,0.707106781186548,0.707106781186547,0.707106781186548,
0.707106781186547,0.707106781186547,0.707106781186547,0.707106781186548,
0.707106781186548,0.707106781186548,0.707106781186547,0.707106781186548,
0.707106781186547,0.707106781186548,0.707106781186547,0.707106781186547,
0.707106781186547,0.707106781186547,0.707106781186548,0.707106781186548,
0.707106781186547,0.707106781186547,0.707106781186548,0.707106781186547,
0.707106781186548,0.707106781186547,0.707106781186548,0.707106781186547,
0.707106781186547,0.707106781186548,0.707106781186547,0.707106781186548,
0.707106781186547,0.707106781186548,0.707106781186548,0.707106781186547,
0.707106781186548,0.707106781186547,0.707106781186548,0.707106781186548,
0.707106781186547,0.707106781186548,0.707106781186547,0.707106781186547,
0.707106781186548,0.707106781186547,0.707106781186548,0.707106781186547,
0.707106781186548,0.707106781186547,0.707106781186547,0.707106781186548,
0.707106781186548,0.707106781186548,0.707106781186548,0.707106781186547,
0.707106781186548,0.707106781186548,0.707106781186548,0.707106781186547,
0.707106781186548,0.707106781186548,0.707106781186548,0.707106781186547,
0.707106781186547,0.707106781186548,0.707106781186547,0.707106781186548,
0.707106781186547,0.707106781186548,0.707106781186548,0.707106781186547,
0.707106781186547,0.707106781186548,0.707106781186547,0.707106781186548,
0.707106781186547,0.707106781186548,0.707106781186548,0.707106781186547,
0.707106781186547,0.707106781186547,0.707106781186548,0.707106781186548,
0.707106781186547,0.707106781186547,0.707106781186548,0.707106781186548,
0.707106781186548,0.707106781186548,0.707106781186547,0.707106781186547,
0.707106781186548,0.707106781186548,0.707106781186547,0.707106781186548,
0.707106781186547,0.707106781186548,0.707106781186547,0.707106781186548,
0.707106781186547,0.707106781186547,0.707106781186548,0.707106781186547,
0.707106781186547,0.707106781186548,0.707106781186547,0.707106781186548,
0.707106781186547,0.707106781186548,0.707106781186547,0.707106781186548,
0.707106781186547,0.707106781186548,0.707106781186547,0.707106781186548,
0.707106781186547,0.707106781186547,0.707106781186548,0.707106781186548,
0.707106781186547,0.707106781186547,0.707106781186547,0.707106781186548,
0.707106781186547,0.707106781186548,0.707106781186547,0.707106781186548,
0.707106781186547,0.707106781186548,0.707106781186547,0.707106781186547,
0.707106781186547,0.707106781186548,0.707106781186547,0.707106781186548,
0.707106781186548,0.707106781186547,0.707106781186548,0.707106781186547,
0.707106781186547,0.707106781186548,0.707106781186547,0.707106781186547,
0.707106781186548,0.707106781186547,0.707106781186547,0.707106781186547,
0.707106781186547,0.707106781186548,0.707106781186547,0.707106781186547,
0.707106781186547,0.707106781186548,0.707106781186547,0.707106781186547,
0.707106781186548,0.707106781186548,0.707106781186547,0.707106781186548,
0.707106781186548,0.707106781186547,0.707106781186547,0.707106781186548,
0.707106781186547,0.707106781186547,0.707106781186548,0.707106781186547,
0.707106781186547,0.707106781186547,0.707106781186548,0.707106781186547,
0.707106781186548,0.707106781186547,0.707106781186548,0.707106781186547,
0.707106781186548,0.707106781186547,0.707106781186548,0.707106781186547,
0.707106781186548,0.707106781186548,0.707106781186547,0.707106781186547,
0.707106781186548,0.707106781186547,0.707106781186548,0.707106781186547,
0.707106781186548,0.707106781186548,0.707106781186547,0.707106781186548,
0.707106781186547,0.707106781186548,0.707106781186548,0.707106781186547,
0.707106781186547,0.707106781186548,0.707106781186547,0.707106781186548,
0.707106781186547,0.707106781186548,0.707106781186547,0.707106781186548,
0.707106781186547,0.707106781186547,0.707106781186547,0.707106781186547,
0.707106781186547,0.707106781186547,0.707106781186547,0.707106781186547,
0.707106781186548,0.707106781186547,0.707106781186548,0.707106781186547,
0.707106781186547,0.707106781186548,0.707106781186547,0.707106781186548,
0.707106781186547,0.707106781186547,0.707106781186548,0.707106781186547,
0.707106781186548,0.707106781186547,0.707106781186548,0.707106781186547,
0.707106781186548,0.707106781186547,0.707106781186548,0.707106781186547,
0.707106781186548,0.707106781186547,0.707106781186548,0.707106781186548,
0.707106781186547,0.707106781186548,0.707106781186547,0.707106781186547,
0.707106781186547,0.707106781186548,0.707106781186547,0.707106781186547,
0.707106781186547,0.707106781186548,0.707106781186547,0.707106781186547,
0.707106781186548,0.707106781186547,0.707106781186547,0.707106781186547,
0.707106781186547,0.707106781186548,0.707106781186547,0.707106781186547,
0.707106781186547,0.707106781186548,0.707106781186548,0.707106781186548,
0.707106781186548,0.707106781186547,0.707106781186548,0.707106781186547,
0.707106781186547,0.707106781186548,0.707106781186547,0.707106781186548,
0.707106781186547,0.707106781186547,0.707106781186548,0.707106781186547,
0.707106781186547,0.707106781186547,0.707106781186547,0.707106781186548,
0.707106781186548,0.707106781186547,0.707106781186547,0.707106781186548,
0.707106781186547,0.707106781186548,0.707106781186547,0.707106781186548,
0.707106781186548,0.707106781186547,0.707106781186547,0.707106781186548,
0.707106781186548,0.707106781186547,0.707106781186548,0.707106781186548,
0.707106781186547,0.707106781186548,0.707106781186548,0.707106781186548,
0.707106781186547,0.707106781186548,0.707106781186547,0.707106781186548,
0.707106781186547,0.707106781186548,0.707106781186547,0.707106781186548,
0.707106781186547,0.707106781186548,0.707106781186548,0.707106781186547,
0.707106781186547,0.707106781186548,0.707106781186547,0.707106781186548,
0.707106781186547,0.707106781186548,0.707106781186548,0.707106781186548,
0.707106781186548,0.707106781186548,0.707106781186547,0.707106781186547,
0.707106781186547,0.707106781186547,0.707106781186548,0.707106781186547,
0.707106781186548,0.707106781186547,0.707106781186547,0.707106781186548,
0.707106781186548,0.707106781186547,0.707106781186548,0.707106781186547,
0.707106781186548,0.707106781186548,0.707106781186547,0.707106781186547,
0.707106781186548,0.707106781186547,0.707106781186548,0.707106781186547,
0.707106781186548,0.707106781186547,0.707106781186548,0.707106781186547,
0.707106781186548,0.707106781186547,0.707106781186548,0.707106781186547,
0.707106781186548,0.707106781186548,0.707106781186547,0.707106781186548,
0.707106781186547,0.707106781186548,0.707106781186547,0.707106781186548,
0.707106781186548,0.707106781186548,0.707106781186547,0.707106781186547,
0.707106781186548,0.707106781186548,0.707106781186547,0.707106781186547,
0.707106781186547,0.707106781186548,0.707106781186547,0.707106781186548,
0.707106781186547,0.707106781186548,0.707106781186547,0.707106781186547,
0.707106781186547,0.707106781186548,0.707106781186547,0.707106781186548,
0.707106781186547,0.707106781186548,0.707106781186547,0.707106781186548,
0.707106781186547,0.707106781186547,0.707106781186548,0.707106781186547,
0.707106781186547,0.707106781186548,0.707106781186547,0.707106781186547,
0.707106781186548,0.707106781186547,0.707106781186547,0.707106781186547,
0.707106781186548,0.707106781186547,0.707106781186548,0.707106781186547,
0.707106781186547,0.707106781186547,0.707106781186548,0.707106781186548,
0.707106781186547,0.707106781186547,0.707106781186548,0.707106781186548,
0.707106781186548,0.707106781186547,0.707106781186548,0.707106781186547,
0.707106781186548,0.707106781186547,0.707106781186548,0.707106781186547,
0.707106781186547,0.707106781186547,0.707106781186547,0.707106781186548,
0.707106781186547,0.707106781186548,0.707106781186548,0.707106781186547,
0.707106781186548,0.707106781186547,0.707106781186547,0.707106781186547,
0.707106781186547,0.707106781186548,0.707106781186547,0.707106781186548,
0.707106781186547,0.707106781186548,0.707106781186548,0.707106781186547,
0.707106781186548,0.707106781186547,0.707106781186547,0.707106781186547,
0.707106781186547,0.707106781186548,0.707106781186547,0.707106781186548,
0.707106781186548,0.707106781186547,0.707106781186548,0.707106781186547,
0.707106781186548,0.707106781186547,0.707106781186547,0.707106781186548,
0.707106781186547,0.707106781186548,0.707106781186548,0.707106781186547,
0.707106781186547,0.707106781186548,0.707106781186548,0.707106781186547,
0.707106781186547,0.707106781186548,0.707106781186547,0.707106781186547,
0.707106781186548,0.707106781186547,0.707106781186547,0.707106781186548,
0.707106781186547,0.707106781186548,0.707106781186547,0.707106781186547,
0.707106781186548,0.707106781186547,0.707106781186548,0.707106781186547,
0.707106781186548,0.707106781186547,0.707106781186547,0.707106781186547,
0.707106781186548,0.707106781186547,0.707106781186548,0.707106781186547,
0.707106781186548,0.707106781186548,0.707106781186548,0.707106781186548,
0.707106781186547,0.707106781186547,0.707106781186547,0.707106781186548,
0.707106781186547,0.707106781186548,0.707106781186547,0.707106781186547,
0.707106781186548,0.707106781186547,0.707106781186547,0.707106781186548,
0.707106781186547,0.707106781186547,0.707106781186548,0.707106781186548,
0.707106781186547,0.707106781186548,0.707106781186547,0.707106781186547,
0.707106781186548,0.707106781186547,0.707106781186548,0.707106781186547,
0.707106781186548,0.707106781186547,0.707106781186547,0.707106781186547,
0.707106781186548,0.707106781186547,0.707106781186548,0.707106781186547,
0.707106781186548,0.707106781186547,0.707106781186547,0.707106781186548,
0.707106781186548,0.707106781186548,0.707106781186547,0.707106781186548,
0.707106781186547,0.707106781186548,0.707106781186547,0.707106781186548,
0.707106781186547,0.707106781186548,0.707106781186548,0.707106781186547,
0.707106781186547,0.707106781186547,0.707106781186548,0.707106781186547,
0.707106781186547,0.707106781186548,0.707106781186547,0.707106781186547,
0.707106781186548,0.707106781186547,0.707106781186548,0.707106781186548,
0.707106781186548,0.707106781186547,0.707106781186548,0.707106781186547,
0.707106781186548,0.707106781186547,0.707106781186548,0.707106781186547,
0.707106781186548,0.707106781186547,0.707106781186548,0.707106781186547,
0.707106781186548,0.707106781186548,0.707106781186547,0.707106781186548,
0.707106781186547,0.707106781186548,0.707106781186548,0.707106781186547,
0.707106781186547,0.707106781186548,0.707106781186547,0.707106781186547,
0.707106781186548,0.707106781186547,0.707106781186548,0.707106781186548,
0.707106781186547,0.707106781186548,0.707106781186548,0.707106781186548,
0.707106781186548,0.707106781186548,0.707106781186547,0.707106781186548,
0.707106781186548,0.707106781186548,0.707106781186547,0.707106781186548,
0.707106781186547,0.707106781186548,0.707106781186547,0.707106781186548,
0.707106781186547,0.707106781186548,0.707106781186547,0.707106781186548,
0.707106781186547,0.707106781186547,0.707106781186548,0.707106781186547,
0.707106781186547,0.707106781186548,0.707106781186547,0.707106781186548,
0.707106781186547,0.707106781186548,0.707106781186547,0.707106781186548,
0.707106781186547,0.707106781186547,0.707106781186548,0.707106781186547,
0.707106781186547,0.707106781186548,0.707106781186547,0.707106781186548,
0.707106781186547,0.707106781186547,0.707106781186548,0.707106781186548,
0.707106781186547,0.707106781186548,0.707106781186547,0.707106781186547,
0.707106781186547,0.707106781186548,0.707106781186547,0.707106781186547,
0.707106781186548,0.707106781186547,0.707106781186547,0.707106781186547,
0.707106781186548,0.707106781186548,0.707106781186547,0.707106781186548,
0.707106781186547,0.707106781186548,0.707106781186547,0.707106781186547,
0.707106781186548,0.707106781186547,0.707106781186548,0.707106781186547,
0.707106781186547,0.707106781186547,0.707106781186547,0.707106781186548,
0.707106781186547,0.707106781186547,0.707106781186547,0.707106781186547,
0.707106781186547,0.707106781186548,0.707106781186547,0.707106781186547,
0.707106781186547,0.707106781186547,0.707106781186548,0.707106781186547,
0.707106781186548,0.707106781186547,0.707106781186547,0.707106781186548,
0.707106781186547,0.707106781186548,0.707106781186547,0.707106781186547,
0.707106781186548,0.707106781186547,0.707106781186547,0.707106781186548,
0.707106781186547,0.707106781186547,0.707106781186547,0.707106781186547,
0.707106781186548,0.707106781186547,0.707106781186548,0.707106781186548,
0.707106781186547,0.707106781186548,0.707106781186548,0.707106781186547,
0.707106781186547,0.707106781186548,0.707106781186547,0.707106781186547,
0.707106781186547,0.707106781186548,0.707106781186547,0.707106781186547,
0.707106781186548,0.707106781186547,0.707106781186548,0.707106781186547,
0.707106781186548,0.707106781186547,0.707106781186547,0.707106781186548,
0.707106781186547,0.707106781186548,0.707106781186547,0.707106781186548,
0.707106781186547,0.707106781186548,0.707106781186547,0.707106781186548,
0.707106781186547,0.707106781186547,0.707106781186547,0.707106781186547,
0.707106781186548,0.707106781186548,0.707106781186547,0.707106781186548,
0.707106781186548,0.707106781186547,0.707106781186548,0.707106781186547,
0.707106781186547,0.707106781186548,0.707106781186547,0.707106781186547,
0.707106781186547,0.707106781186547,0.707106781186548,0.707106781186547,
0.707106781186547,0.707106781186547,0.707106781186548,0.707106781186547,
0.707106781186547,0.707106781186548,0.707106781186547,0.707106781186548,
0.707106781186548,0.707106781186547,0.707106781186548,0.707106781186547,
0.707106781186548,0.707106781186547,0.707106781186548,0.707106781186547,
0.707106781186547,0.707106781186548,0.707106781186547,0.707106781186548,
0.707106781186548,0.707106781186547,0.707106781186547,0.707106781186548,
0.707106781186547,0.707106781186548,0.707106781186547,0.707106781186548,
0.707106781186547,0.707106781186547,0.707106781186548,0.707106781186548,
0.707106781186547,0.707106781186548,0.707106781186548,0.707106781186547,
0.707106781186548,0.707106781186548,0.707106781186547,0.707106781186548,
0.707106781186547,0.707106781186548,0.707106781186547,0.707106781186548,
0.707106781186547,0.707106781186548,0.707106781186547,0.707106781186547,
0.707106781186548,0.707106781186547,0.707106781186547,0.707106781186548,
0.707106781186547,0.707106781186548,0.707106781186548,0.707106781186547,
0.707106781186547,0.707106781186547,0.707106781186548,0.707106781186547,
0.707106781186548,0.707106781186548,0.707106781186547,0.707106781186548,
0.707106781186547,0.707106781186548,0.707106781186547,0.707106781186548,
0.707106781186547,0.707106781186547,0.707106781186548,0.707106781186548,
0.707106781186548,0.707106781186547,0.707106781186548,0.707106781186548,
0.707106781186547,0.707106781186548,0.707106781186547,0.707106781186548,
0.707106781186548,0.707106781186548,0.707106781186548,0.707106781186548,
0.707106781186548,0.707106781186547,0.707106781186547,0.707106781186548,
0.707106781186547,0.707106781186547,0.707106781186548,0.707106781186547,
0.707106781186547,0.707106781186548,0.707106781186547,0.707106781186548,
0.707106781186547,0.707106781186548,0.707106781186547,0.707106781186547,
0.707106781186547,0.707106781186548,0.707106781186547,0.707106781186547,
0.707106781186548,0.707106781186547,0.707106781186548,0.707106781186547,
0.707106781186548,0.707106781186547,0.707106781186547,0.707106781186547,
0.707106781186547,0.707106781186548,0.707106781186547,0.707106781186547,
0.707106781186548,0.707106781186548,0.707106781186547,0.707106781186548,
0.707106781186547,0.707106781186548,0.707106781186547,0.707106781186547,
0.707106781186548,0.707106781186547,0.707106781186548,0.707106781186547,
0.707106781186548,0.707106781186547,0.707106781186548,0.707106781186548,
0.707106781186547,0.707106781186548,0.707106781186547,0.707106781186547,
0.707106781186548,0.707106781186547,0.707106781186547,0.707106781186548,
0.707106781186548,0.707106781186548,0.707106781186547,0.707106781186548,
0.707106781186547,0.707106781186547,0.707106781186547,0.707106781186548,
0.707106781186547,0.707106781186548,0.707106781186548,0.707106781186548,
0.707106781186547,0.707106781186547,0.707106781186547,0.707106781186547,
0.707106781186548,0.707106781186547,0.707106781186547,0.707106781186548,
0.707106781186547,0.707106781186548,0.707106781186547,0.707106781186547,
0.707106781186548,0.707106781186547,0.707106781186548,0.707106781186547,
0.707106781186548,0.707106781186547,0.707106781186547,0.707106781186547,
0.707106781186547,0.707106781186547,0.707106781186547,0.707106781186548,
0.707106781186547,0.707106781186547,0.707106781186548,0.707106781186548,
0.707106781186547,0.707106781186548,0.707106781186548,0.707106781186547,
0.707106781186547,0.707106781186548,0.707106781186547,0.707106781186547,
0.707106781186548,0.707106781186547,0.707106781186548,0.707106781186548,
0.707106781186548,0.707106781186547,0.707106781186547,0.707106781186547,
0.707106781186547,0.707106781186548,0.707106781186548,0.707106781186548,
0.707106781186547,0.707106781186548,0.707106781186547,0.707106781186548,
0.707106781186548,0.707106781186547,0.707106781186548,0.707106781186547,
0.707106781186548,0.707106781186548,0.707106781186547,0.707106781186547,
0.707106781186548,0.707106781186547,0.707106781186548,0.707106781186547,
0.707106781186548,0.707106781186548,0.707106781186548,0.707106781186547,
0.707106781186548,0.707106781186547,0.707106781186547,0.707106781186547,
0.707106781186547,0.707106781186548,0.707106781186548,0.707106781186547,
0.707106781186547,0.707106781186547,0.707106781186548,0.707106781186547,
0.707106781186547,0.707106781186548,0.707106781186547,0.707106781186548,
0.707106781186548,0.707106781186548,0.707106781186547,0.707106781186547,
0.707106781186547,0.707106781186547,0.707106781186548,0.707106781186548,
0.707106781186547,0.707106781186548,0.707106781186547,0.707106781186548,
0.707106781186548,0.707106781186547,0.707106781186548,0.707106781186547,
0.707106781186548,0.707106781186547,0.707106781186547,0.707106781186547,
0.707106781186548,0.707106781186547,0.707106781186548,0.707106781186547,
0.707106781186548,0.707106781186547,0.707106781186548,0.707106781186547,
0.707106781186548,0.707106781186547,0.707106781186547,0.707106781186548,
0.707106781186547,0.707106781186548,0.707106781186547,0.707106781186547,
0.707106781186548,0.707106781186548,0.707106781186547,0.707106781186548,
0.707106781186548,0.707106781186547,0.707106781186548,0.707106781186547,
0.707106781186548,0.707106781186547,0.707106781186547,0.707106781186547,
0.707106781186548,0.707106781186547,0.707106781186547,0.707106781186548,
0.707106781186547,0.707106781186548,0.707106781186547,0.707106781186548,
0.707106781186548,0.707106781186547,0.707106781186548,0.707106781186547,
0.707106781186548,0.707106781186548,0.707106781186548,0.707106781186548,
0.707106781186547,0.707106781186547,0.707106781186548,0.707106781186547,
0.707106781186547,0.707106781186548,0.707106781186548,0.707106781186547,
0.707106781186547,0.707106781186548,0.707106781186547,0.707106781186547,
0.707106781186548,0.707106781186547,0.707106781186548,0.707106781186547,
0.707106781186548,0.707106781186547,0.707106781186547,0.707106781186547,
0.707106781186548,0.707106781186547,0.707106781186547,0.707106781186548,
0.707106781186547,0.707106781186548,0.707106781186548,0.707106781186548,
0.707106781186547,0.707106781186547,0.707106781186547,0.707106781186548,
0.707106781186548,0.707106781186547,0.707106781186547,0.707106781186547,
0.707106781186547,0.707106781186548,0.707106781186548,0.707106781186547,
0.707106781186547,0.707106781186547,0.707106781186548,0.707106781186548,
0.707106781186547,0.707106781186548,0.707106781186547,0.707106781186548,
0.707106781186547,0.707106781186548,0.707106781186548,0.707106781186547,
0.707106781186548,0.707106781186548,0.707106781186548,0.707106781186547,
0.707106781186547,0.707106781186547,0.707106781186548,0.707106781186548,
0.707106781186548,0.707106781186547,0.707106781186547,0.707106781186548,
0.707106781186548,0.707106781186547,0.707106781186548,0.707106781186547,
0.707106781186547,0.707106781186548,0.707106781186547,0.707106781186548,
0.707106781186547,0.707106781186547,0.707106781186548,0.707106781186547,
0.707106781186548,0.707106781186548,0.707106781186547,0.707106781186547,
0.707106781186548,0.707106781186547,0.707106781186548,0.707106781186547,
0.707106781186547,0.707106781186548,0.707106781186547,0.707106781186548,
0.707106781186547,0.707106781186548,0.707106781186547,0.707106781186547,
0.707106781186548,0.707106781186547,0.707106781186547,0.707106781186547,
0.707106781186547,0.707106781186547,0.707106781186547,0.707106781186548,
0.707106781186547,0.707106781186548,0.707106781186548,0.707106781186548,
0.707106781186547,0.707106781186547,0.707106781186547,0.707106781186548,
0.707106781186547,0.707106781186548,0.707106781186547,0.707106781186547,
0.707106781186548,0.707106781186547,0.707106781186547,0.707106781186547,
0.707106781186547,0.707106781186547,0.707106781186548,0.707106781186547,
0.707106781186548,0.707106781186547,0.707106781186547,0.707106781186548,
0.707106781186548,0.707106781186547,0.707106781186547,0.707106781186547,
0.707106781186548,0.707106781186547,0.707106781186547,0.707106781186548,
0.707106781186548,0.707106781186547,0.707106781186548,0.707106781186547,
0.707106781186548,0.707106781186548,0.707106781186547,0.707106781186547,
0.707106781186547,0.707106781186548,0.707106781186548,0.707106781186547,
0.707106781186548,0.707106781186547,0.707106781186548,0.707106781186548,
0.707106781186547,0.707106781186548,0.707106781186547,0.707106781186547,
0.707106781186547,0.707106781186548,0.707106781186547,0.707106781186548,
0.707106781186547,0.707106781186548,0.707106781186547,0.707106781186547,
0.707106781186547,0.707106781186547,0.707106781186547,0.707106781186548,
0.707106781186547,0.707106781186548,0.707106781186547,0.707106781186548,
0.707106781186547,0.707106781186548,0.707106781186547,0.707106781186547,
0.707106781186547,0.707106781186547,0.707106781186547,0.707106781186548,
0.707106781186548,0.707106781186548,0.707106781186547,0.707106781186548,
0.707106781186547,0.707106781186548,0.707106781186547,0.707106781186547,
0.707106781186548,0.707106781186547,0.707106781186548,0.707106781186547,
0.707106781186547,0.707106781186547,0.707106781186548,0.707106781186548,
0.707106781186547,0.707106781186548,0.707106781186547,0.707106781186548,
0.707106781186548,0.707106781186547,0.707106781186548,0.707106781186547,
0.707106781186548,0.707106781186548,0.707106781186547,0.707106781186547,
0.707106781186547,0.707106781186547,0.707106781186547,0.707106781186547,
0.707106781186548,0.707106781186548,0.707106781186547,0.707106781186548,
0.707106781186547,0.707106781186547,0.707106781186548,0.707106781186547,
0.707106781186547,0.707106781186548,0.707106781186547,0.707106781186547,
0.707106781186547,0.707106781186548,0.707106781186547,0.707106781186547,
0.707106781186548,0.707106781186547,0.707106781186548,0.707106781186548,
0.707106781186547,0.707106781186547,0.707106781186547,0.707106781186548,
0.707106781186547,0.707106781186547,0.707106781186548,0.707106781186548,
0.707106781186548,0.707106781186548,0.707106781186547,0.707106781186548,
0.707106781186548,0.707106781186547,0.707106781186547,0.707106781186548,
0.707106781186547,0.707106781186548,0.707106781186547,0.707106781186547,
0.707106781186548,0.707106781186547,0.707106781186547,0.707106781186548,
0.707106781186547,0.707106781186548,0.707106781186547,0.707106781186548,
0.707106781186547,0.707106781186548,0.707106781186547,0.707106781186548,
0.707106781186547,0.707106781186548,0.707106781186548,0.707106781186547,
0.707106781186547,0.707106781186548,0.707106781186548,0.707106781186547,
0.707106781186547,0.707106781186547,0.707106781186547,0.707106781186547,
0.707106781186548,0.707106781186547,0.707106781186547,0.707106781186548,
0.707106781186547,0.707106781186548,0.707106781186548,0.707106781186547,
0.707106781186548,0.707106781186547,0.707106781186548,0.707106781186547,
0.707106781186548,0.707106781186547,0.707106781186547,0.707106781186547,
0.707106781186547,0.707106781186547,0.707106781186547,0.707106781186548,
0.707106781186547,0.707106781186548,0.707106781186547,0.707106781186547,
0.707106781186547,0.707106781186548,0.707106781186547,0.707106781186548,
0.707106781186548,0.707106781186547,0.707106781186547,0.707106781186548,
0.707106781186547,0.707106781186548,0.707106781186547,0.707106781186548,
0.707106781186547,0.707106781186548,0.707106781186547,0.707106781186547,
0.707106781186548,0.707106781186547,0.707106781186548,0.707106781186547,
0.707106781186548,0.707106781186548,0.707106781186548,0.707106781186548,
0.707106781186547,0.707106781186548,0.707106781186548,0.707106781186548,
0.707106781186547,0.707106781186548,0.707106781186548,0.707106781186547,
0.707106781186548,0.707106781186547,0.707106781186548,0.707106781186547,
0.707106781186547,0.707106781186547,0.707106781186548,0.707106781186548,
0.707106781186547,0.707106781186548,0.707106781186547,0.707106781186548,
0.707106781186547,0.707106781186548,0.707106781186548,0.707106781186547,
0.707106781186548,0.707106781186547,0.707106781186547,0.707106781186548,
0.707106781186547,0.707106781186547,0.707106781186547,0.707106781186548,
0.707106781186547,0.707106781186548,0.707106781186548,0.707106781186547,
0.707106781186548,0.707106781186547,0.707106781186548,0.707106781186548,
0.707106781186548,0.707106781186548,0.707106781186547,0.707106781186548,
0.707106781186547,0.707106781186548,0.707106781186547,0.707106781186548,
0.707106781186547,0.707106781186547,0.707106781186547,0.707106781186547,
0.707106781186548,0.707106781186547,0.707106781186548,0.707106781186547,
0.707106781186547,0.707106781186548,0.707106781186547,0.707106781186548,
0.707106781186547,0.707106781186548,0.707106781186547,0.707106781186548,
0.707106781186548,0.707106781186548,0.707106781186548,0.707106781186547,
0.707106781186548,0.707106781186548,0.707106781186547,0.707106781186548,
0.707106781186547,0.707106781186548,0.707106781186547,0.707106781186548,
0.707106781186547,0.707106781186547,0.707106781186548,0.707106781186547,
0.707106781186548,0.707106781186547,0.707106781186547,0.707106781186548,
0.707106781186547,0.707106781186548,0.707106781186547,0.707106781186547,
0.707106781186548,0.707106781186548,0.707106781186548,0.707106781186548,
0.707106781186548,0.707106781186548,0.707106781186548,0.707106781186548,
0.707106781186548,0.707106781186547,0.707106781186548,0.707106781186547,
0.707106781186547,0.707106781186548,0.707106781186547,0.707106781186548,
0.707106781186548,0.707106781186547,0.707106781186547,0.707106781186548,
0.707106781186548,0.707106781186547,0.707106781186547,0.707106781186547,
0.707106781186547,0.707106781186547,0.707106781186548,0.707106781186547,
0.707106781186548,0.707106781186548,0.707106781186548,0.707106781186547,
0.707106781186548,0.707106781186547,0.707106781186548,0.707106781186547,
0.707106781186548,0.707106781186547,0.707106781186548,0.707106781186548,
0.707106781186547,0.707106781186547,0.707106781186548,0.707106781186548,
0.707106781186548,0.707106781186547,0.707106781186547,0.707106781186548,
0.707106781186547,0.707106781186547,0.707106781186548,0.707106781186547,
0.707106781186548,0.707106781186547,0.707106781186547,0.707106781186548,
0.707106781186548,0.707106781186548,0.707106781186547,0.707106781186547,
0.707106781186548,0.707106781186547,0.707106781186548,0.707106781186547,
0.707106781186548,0.707106781186547,0.707106781186548,0.707106781186548,
0.707106781186547,0.707106781186548,0.707106781186547,0.707106781186548,
0.707106781186547,0.707106781186547,0.707106781186547,0.707106781186548,
0.707106781186547,0.707106781186548,0.707106781186547,0.707106781186547,
0.707106781186547,0.707106781186548,0.707106781186547,0.707106781186547,
0.707106781186548,0.707106781186548,0.707106781186547,0.707106781186548,
0.707106781186547,0.707106781186548,0.707106781186548,0.707106781186547,
0.707106781186548,0.707106781186547,0.707106781186547,0.707106781186548,
0.707106781186547,0.707106781186547,0.707106781186547,0.707106781186548,
0.707106781186547,0.707106781186548,0.707106781186547,0.707106781186548,
0.707106781186548,0.707106781186548,0.707106781186547,0.707106781186548,
0.707106781186548,0.707106781186548,0.707106781186547,0.707106781186548,
0.707106781186547,0.707106781186547,0.707106781186548,0.707106781186547,
0.707106781186547,0.707106781186548,0.707106781186548,0.707106781186547,
0.707106781186548,0.707106781186547,0.707106781186548,0.707106781186548,
0.707106781186547,0.707106781186548,0.707106781186547,0.707106781186548,
0.707106781186547,0.707106781186548,0.707106781186547,0.707106781186548,
0.707106781186548,0.707106781186548,0.707106781186547,0.707106781186548,
0.707106781186548,0.707106781186547,0.707106781186547,0.707106781186548,
0.707106781186547,0.707106781186548,0.707106781186548,0.707106781186547,
0.707106781186548,0.707106781186548,0.707106781186547,0.707106781186548,
0.707106781186548,0.707106781186547,0.707106781186547,0.707106781186548,
0.707106781186547,0.707106781186548,0.707106781186547,0.707106781186548,
0.707106781186547,0.707106781186548,0.707106781186548,0.707106781186548,
0.707106781186547,0.707106781186548,0.707106781186547,0.707106781186548,
0.707106781186547,0.707106781186548,0.707106781186547,0.707106781186548,
0.707106781186547,0.707106781186548,0.707106781186547,0.707106781186548,
0.707106781186547,0.707106781186547,0.707106781186547,0.707106781186548,
0.707106781186547,0.707106781186548,0.707106781186547,0.707106781186548,
0.707106781186547,0.707106781186548,0.707106781186547,0.707106781186548,
0.707106781186548,0.707106781186548,0.707106781186547,0.707106781186548,
0.707106781186547,0.707106781186548,0.707106781186548,0.707106781186547,
0.707106781186548,0.707106781186547,0.707106781186548,0.707106781186547,
0.707106781186548,0.707106781186547,0.707106781186548,0.707106781186547,
0.707106781186547,0.707106781186547,0.707106781186548,0.707106781186547,
0.707106781186547,0.707106781186548,0.707106781186547,0.707106781186548,
0.707106781186547,0.707106781186547,0.707106781186548,0.707106781186547,
0.707106781186548,0.707106781186547,0.707106781186548,0.707106781186548,
0.707106781186548,0.707106781186547,0.707106781186547,0.707106781186548,
0.707106781186548,0.707106781186547,0.707106781186548,0.707106781186547,
0.707106781186547,0.707106781186547,0.707106781186548,0.707106781186547,
0.707106781186548,0.707106781186547,0.707106781186548,0.707106781186548,
0.707106781186548,0.707106781186547,0.707106781186547,0.707106781186547,
0.707106781186547,0.707106781186547,0.707106781186547,0.707106781186548,
0.707106781186547,0.707106781186548,0.707106781186547,0.707106781186548,
0.707106781186547,0.707106781186547,0.707106781186548,0.707106781186547,
0.707106781186547,0.707106781186548,0.707106781186548,0.707106781186547,
0.707106781186547,0.707106781186547,0.707106781186548,0.707106781186547,
0.707106781186547,0.707106781186548,0.707106781186548),(1.,1.,1.,1.,1.,
1.,1.,1.,1.,1.,1.,1.,1.,1.,1.,1.,1.,1.,1.,1.,1.,1.,1.,1.,1.,1.,1.,1.,1.,
1.,1.,1.,1.,1.,1.,1.,1.,1.,1.,1.,1.,1.,1.,1.,1.,1.,1.,1.,1.,1.,1.,1.,1.,
1.,1.,1.,1.,1.,1.,1.,1.,1.,1.,1.,1.,1.,1.,1.,1.,1.,1.,1.,1.,1.,1.,1.,1.,
1.,1.,1.,1.,1.,1.,1.,1.,1.,1.,1.,1.,1.,1.,1.,1.,1.,1.,1.,1.,1.,1.,1.,1.,
1.,1.,1.,1.,1.,1.,1.,1.,1.,1.,1.,1.,1.,1.,1.,1.,1.,1.,1.,1.,1.,1.,1.,1.,
1.,1.,1.,1.,1.,1.,1.,1.,1.,1.,1.,1.,1.,1.,1.,1.,1.,1.,1.,1.,1.,1.,1.,1.,
1.,1.,1.,1.,1.,1.,1.,1.,1.,1.,1.,1.,1.,1.,1.,1.,1.,1.,1.,1.,1.,1.,1.,1.,
1.,1.,1.,1.,1.,1.,1.,1.,1.,1.,1.,1.,1.,1.,1.,1.,1.,1.,1.,1.,1.,1.,1.,1.,
1.,1.,1.,1.,1.,1.,1.,1.,1.,1.,1.,1.,1.,1.,1.,1.,1.,1.,1.,1.,1.,1.,1.,1.,
1.,1.,1.,1.,1.,1.,1.,1.,1.,1.,1.,1.,1.,1.,1.,1.,1.,1.,1.,1.,1.,1.,1.,1.,
1.,1.,1.,1.,1.,1.,1.,1.,1.,1.,1.,1.,1.,1.,1.,1.,1.,1.,1.,1.,1.,1.,1.,1.,
1.,1.,1.,1.,1.,1.,1.,1.,1.,1.,1.,1.,1.,1.,1.,1.,1.,1.,1.,1.,1.,1.,1.,1.,
1.,1.,1.,1.,1.,1.,1.,1.,1.,1.,1.,1.,1.,1.,1.,1.,1.,1.,1.,1.,1.,1.,1.,1.,
1.,1.,1.,1.,1.,1.,1.,1.,1.,1.,1.,1.,1.,1.,1.,1.,1.,1.,1.,1.,1.,1.,1.,1.,
1.,1.,1.,1.,1.,1.,1.,1.,1.,1.,1.,1.,1.,1.,1.,1.,1.,1.,1.,1.,1.,1.,1.,1.,
1.,1.,1.,1.,1.,1.,1.,1.,1.,1.,1.,1.,1.,1.,1.,1.,1.,1.,1.,1.,1.,1.,1.,1.,
1.,1.,1.,1.,1.,1.,1.,1.,1.,1.,1.,1.,1.,1.,1.,1.,1.,1.,1.,1.,1.,1.,1.,1.,
1.,1.,1.,1.,1.,1.,1.,1.,1.,1.,1.,1.,1.,1.,1.,1.,1.,1.,1.,1.,1.,1.,1.,1.,
1.,1.,1.,1.,1.,1.,1.,1.,1.,1.,1.,1.,1.,1.,1.,1.,1.,1.,1.,1.,1.,1.,1.,1.,
1.,1.,1.,1.,1.,1.,1.,1.,1.,1.,1.,1.,1.,1.,1.,1.,1.,1.,1.,1.,1.,1.,1.,1.,
1.,1.,1.,1.,1.,1.,1.,1.,1.,1.,1.,1.,1.,1.,1.,1.,1.,1.,1.,1.,1.,1.,1.,1.,
1.,1.,1.,1.,1.,1.,1.,1.,1.,1.,1.,1.,1.,1.,1.,1.,1.,1.,1.,1.,1.,1.,1.,1.,
1.,1.,1.,1.,1.,1.,1.,1.,1.,1.,1.,1.,1.,1.,1.,1.,1.,1.,1.,1.,1.,1.,1.,1.,
1.,1.,1.,1.,1.,1.,1.,1.,1.,1.,1.,1.,1.,1.,1.,1.,1.,1.,1.,1.,1.,1.,1.,1.,
1.,1.,1.,1.,1.,1.,1.,1.,1.,1.,1.,1.,1.,1.,1.,1.,1.,1.,1.,1.,1.,1.,1.,1.,
1.,1.,1.,1.,1.,1.,1.,1.,1.,1.,1.,1.,1.,1.,1.,1.,1.,1.,1.,1.,1.,1.,1.,1.,
1.,1.,1.,1.,1.,1.,1.,1.,1.,1.,1.,1.,1.,1.,1.,1.,1.,1.,1.,1.,1.,1.,1.,1.,
1.,1.,1.,1.,1.,1.,1.,1.,1.,1.,1.,1.,1.,1.,1.,1.,1.,1.,1.,1.,1.,1.,1.,1.,
1.,1.,1.,1.,1.,1.,1.,1.,1.,1.,1.,1.,1.,1.,1.,1.,1.,1.,1.,1.,1.,1.,1.,1.,
1.,1.,1.,1.,1.,1.,1.,1.,1.,1.,1.,1.,1.,1.,1.,1.,1.,1.,1.,1.,1.,1.,1.,1.,
1.,1.,1.,1.,1.,1.,1.,1.,1.,1.,1.,1.,1.,1.,1.,1.,1.,1.,1.,1.,1.,1.,1.,1.,
1.,1.,1.,1.,1.,1.,1.,1.,1.,1.,1.,1.,1.,1.,1.,1.,1.,1.,1.,1.,1.,1.,1.,1.,
1.,1.,1.,1.,1.,1.,1.,1.,1.,1.,1.,1.,1.,1.,1.,1.,1.,1.,1.,1.,1.,1.,1.,1.,
1.,1.,1.,1.,1.,1.,1.,1.,1.,1.,1.,1.,1.,1.,1.,1.,1.,1.,1.,1.,1.,1.,1.,1.,
1.,1.,1.,1.,1.,1.,1.,1.,1.,1.,1.,1.,1.,1.,1.,1.,1.,1.,1.,1.,1.,1.,1.,1.,
1.,1.,1.,1.,1.,1.,1.,1.,1.,1.,1.,1.,1.,1.,1.,1.,1.,1.,1.,1.,1.,1.,1.,1.,
1.,1.,1.,1.,1.,1.,1.,1.,1.,1.,1.,1.,1.,1.,1.,1.,1.,1.,1.,1.,1.,1.,1.,1.,
1.,1.,1.,1.,1.,1.,1.,1.,1.,1.,1.,1.,1.,1.,1.,1.,1.,1.,1.,1.,1.,1.,1.,1.,
1.,1.,1.,1.,1.,1.,1.,1.,1.,1.,1.,1.,1.,1.,1.,1.,1.,1.,1.,1.,1.,1.,1.,1.,
1.,1.,1.,1.,1.,1.,1.,1.,1.,1.,1.,1.,1.,1.,1.,1.,1.,1.,1.,1.,1.,1.,1.,1.,
1.,1.,1.,1.,1.,1.,1.,1.,1.,1.,1.,1.,1.,1.,1.,1.,1.,1.,1.,1.,1.,1.,1.,1.,
1.,1.,1.,1.,1.,1.,1.,1.,1.,1.,1.,1.,1.,1.,1.,1.,1.,1.,1.,1.,1.,1.,1.,1.,
1.,1.,1.,1.,1.,1.,1.,1.,1.,1.,1.,1.,1.,1.,1.,1.,1.,1.,1.,1.,1.,1.,1.,1.,
1.,1.,1.,1.,1.,1.,1.,1.,1.,1.,1.,1.,1.,1.,1.,1.,1.,1.,1.,1.,1.,1.,1.,1.,
1.,1.,1.,1.,1.,1.,1.,1.,1.,1.,1.,1.,1.,1.,1.,1.,1.,1.,1.,1.,1.,1.,1.,1.,
1.,1.,1.,1.,1.,1.,1.,1.,1.,1.,1.,1.,1.,1.,1.,1.,1.,1.,1.,1.,1.,1.,1.,1.,
1.,1.,1.,1.,1.,1.,1.,1.,1.,1.,1.,1.,1.,1.,1.,1.,1.,1.,1.,1.,1.,1.,1.,1.,
1.,1.,1.,1.,1.,1.,1.,1.,1.,1.,1.,1.,1.,1.,1.,1.,1.,1.,1.,1.,1.,1.,1.,1.,
1.,1.,1.,1.,1.,1.,1.,1.,1.,1.,1.,1.,1.,1.,1.,1.,1.,1.,1.,1.,1.,1.,1.,1.,
1.,1.,1.,1.,1.,1.,1.,1.,1.,1.,1.,1.,1.,1.,1.,1.,1.,1.,1.,1.,1.,1.,1.,1.,
1.,1.,1.,1.,1.,1.,1.,1.,1.,1.,1.,1.,1.,1.,1.,1.,1.,1.,1.,1.,1.,1.,1.,1.,
1.,1.,1.,1.,1.,1.,1.,1.,1.,1.,1.,1.,1.,1.,1.,1.,1.,1.,1.,1.,1.,1.,1.,1.,
1.,1.,1.,1.,1.,1.,1.,1.,1.,1.,1.,1.,1.,1.,1.,1.,1.,1.,1.,1.,1.,1.,1.,1.,
1.,1.,1.,1.,1.,1.,1.,1.,1.,1.,1.,1.,1.,1.,1.,1.,1.,1.,1.,1.,1.,1.,1.,1.,
1.,1.,1.,1.,1.,1.,1.,1.,1.,1.,1.,1.,1.,1.,1.,1.,1.,1.,1.,1.,1.,1.,1.,1.,
1.,1.,1.,1.,1.,1.,1.,1.,1.,1.,1.,1.,1.,1.,1.,1.,1.,1.,1.,1.,1.,1.,1.,1.,
1.,1.,1.,1.,1.,1.,1.,1.,1.,1.,1.,1.,1.,1.,1.,1.,1.,1.,1.,1.,1.,1.,1.,1.,
1.,1.,1.,1.,1.,1.,1.,1.,1.,1.,1.,1.,1.,1.,1.,1.,1.,1.,1.,1.,1.,1.,1.,1.,
1.,1.,1.,1.,1.,1.,1.,1.,1.,1.,1.,1.,1.,1.,1.,1.,1.,1.,1.,1.,1.,1.,1.,1.,
1.,1.,1.,1.,1.,1.,1.,1.,1.,1.,1.,1.,1.,1.,1.,1.,1.,1.,1.,1.,1.,1.,1.,1.,
1.,1.,1.,1.,1.,1.,1.,1.,1.,1.,1.,1.,1.,1.,1.,1.,1.,1.,1.,1.,1.,1.,1.,1.,
1.,1.,1.,1.,1.,1.,1.,1.,1.,1.,1.,1.,1.,1.,1.,1.,1.,1.,1.,1.,1.,1.,1.,1.,
1.,1.,1.,1.,1.,1.,1.,1.,1.,1.,1.,1.,1.,1.,1.,1.,1.,1.,1.,1.,1.,1.,1.,1.,
1.,1.,1.,1.,1.,1.,1.,1.,1.,1.,1.,1.,1.,1.,1.,1.,1.,1.,1.,1.,1.,1.,1.,1.,
1.,1.,1.,1.,1.,1.,1.,1.,1.,1.,1.,1.,1.,1.,1.,1.,1.,1.,1.,1.,1.,1.,1.,1.,
1.,1.,1.,1.,1.,1.,1.,1.,1.,1.,1.,1.,1.,1.,1.,1.,1.,1.,1.,1.,1.,1.,1.,1.,
1.,1.,1.,1.,1.,1.,1.,1.,1.,1.,1.,1.,1.,1.,1.,1.,1.,1.,1.,1.,1.,1.,1.,1.,
1.,1.,1.,1.,1.,1.,1.,1.,1.,1.,1.,1.,1.,1.,1.,1.,1.,1.,1.,1.,1.,1.,1.,1.,
1.,1.,1.,1.,1.,1.,1.,1.,1.,1.,1.,1.,1.,1.,1.,1.,1.,1.,1.,1.,1.,1.,1.,1.,
1.,1.,1.,1.,1.,1.,1.,1.,1.,1.,1.,1.,1.,1.,1.,1.,1.,1.,1.,1.,1.,1.,1.,1.,
1.,1.,1.,1.,1.,1.,1.,1.,1.,1.,1.,1.,1.,1.,1.,1.,1.,1.,1.,1.,1.,1.,1.,1.,
1.,1.,1.,1.,1.,1.,1.,1.,1.,1.,1.,1.,1.,1.,1.,1.,1.,1.,1.,1.,1.,1.,1.,1.,
1.,1.,1.,1.,1.,1.,1.,1.,1.,1.,1.,1.,1.,1.,1.,1.,1.,1.,1.,1.,1.,1.,1.,1.,
1.,1.,1.,1.,1.,1.,1.,1.,1.,1.,1.,1.,1.,1.,1.,1.,1.,1.,1.,1.,1.,1.,1.,1.,
1.,1.,1.,1.,1.,1.,1.,1.,1.,1.,1.,1.,1.,1.,1.,1.,1.,1.,1.,1.,1.,1.,1.,1.,
1.,1.,1.,1.,1.,1.,1.,1.,1.,1.,1.,1.,1.,1.,1.,1.,1.,1.,1.,1.,1.,1.,1.,1.,
1.,1.,1.,1.,1.,1.,1.,1.,1.,1.,1.,1.,1.,1.,1.,1.,1.,1.,1.,1.,1.,1.,1.,1.,
1.,1.,1.,1.,1.,1.,1.,1.,1.,1.,1.,1.,1.,1.,1.,1.,1.,1.,1.,1.,1.,1.,1.,1.,
1.,1.,1.,1.,1.,1.,1.,1.,1.,1.,1.,1.,1.,1.,1.,1.,1.,1.,1.,1.,1.,1.,1.,1.,
1.,1.,1.,1.,1.,1.,1.,1.,1.,1.,1.,1.,1.,1.,1.,1.,1.,1.,1.,1.,1.,1.,1.,1.,
1.,1.,1.,1.,1.,1.,1.,1.,1.,1.,1.,1.,1.,1.,1.,1.,1.,1.,1.,1.,1.,1.,1.,1.,
1.,1.,1.,1.,1.,1.,1.,1.,1.,1.,1.,1.,1.,1.,1.,1.,1.,1.,1.,1.,1.,1.,1.,1.,
1.,1.,1.,1.,1.,1.,1.,1.,1.,1.,1.,1.,1.,1.,1.,1.,1.,1.,1.,1.,1.,1.,1.,1.,
1.,1.,1.,1.,1.,1.,1.,1.,1.,1.,1.,1.,1.,1.,1.,1.,1.,1.,1.,1.,1.,1.,1.,1.,
1.,1.,1.,1.,1.,1.,1.,1.,1.,1.,1.,1.,1.,1.,1.,1.,1.,1.,1.,1.,1.,1.,1.,1.,
1.,1.,1.,1.,1.,1.),(0.707106781186548,0.707106781186548,0.707106781186548,
0.707106781186547,0.707106781186547,0.707106781186548,0.707106781186547,
0.707106781186547,0.707106781186547,0.707106781186547,0.707106781186547,
0.707106781186548,0.707106781186548,0.707106781186548,0.707106781186547,
0.707106781186548,0.707106781186547,0.707106781186547,0.707106781186548,
0.707106781186547,0.707106781186548,0.707106781186547,0.707106781186548,
0.707106781186547,0.707106781186548,0.707106781186547,0.707106781186547,
0.707106781186547,0.707106781186547,0.707106781186547,0.707106781186548,
0.707106781186547,0.707106781186547,0.707106781186548,0.707106781186547,
0.707106781186547,0.707106781186548,0.707106781186547,0.707106781186547,
0.707106781186548,0.707106781186548,0.707106781186547,0.707106781186548,
0.707106781186547,0.707106781186547,0.707106781186547,0.707106781186548,
0.707106781186548,0.707106781186547,0.707106781186547,0.707106781186548,
0.707106781186547,0.707106781186548,0.707106781186547,0.707106781186547,
0.707106781186547,0.707106781186547,0.707106781186547,0.707106781186548,
0.707106781186547,0.707106781186548,0.707106781186547,0.707106781186548,
0.707106781186547,0.707106781186548,0.707106781186547,0.707106781186547,
0.707106781186548,0.707106781186547,0.707106781186547,0.707106781186548,
0.707106781186547,0.707106781186548,0.707106781186547,0.707106781186548,
0.707106781186548,0.707106781186547,0.707106781186548,0.707106781186547,
0.707106781186547,0.707106781186548,0.707106781186547,0.707106781186547,
0.707106781186547,0.707106781186548,0.707106781186547,0.707106781186547,
0.707106781186547,0.707106781186547,0.707106781186547,0.707106781186547,
0.707106781186548,0.707106781186548,0.707106781186547,0.707106781186548,
0.707106781186547,0.707106781186548,0.707106781186548,0.707106781186547,
0.707106781186548,0.707106781186548,0.707106781186548,0.707106781186547,
0.707106781186548,0.707106781186547,0.707106781186548,0.707106781186548,
0.707106781186548,0.707106781186547,0.707106781186547,0.707106781186547,
0.707106781186548,0.707106781186548,0.707106781186548,0.707106781186547,
0.707106781186547,0.707106781186547,0.707106781186548,0.707106781186548,
0.707106781186547,0.707106781186547,0.707106781186548,0.707106781186547,
0.707106781186547,0.707106781186547,0.707106781186547,0.707106781186548,
0.707106781186547,0.707106781186548,0.707106781186547,0.707106781186547,
0.707106781186547,0.707106781186548,0.707106781186548,0.707106781186547,
0.707106781186548,0.707106781186548,0.707106781186547,0.707106781186548,
0.707106781186547,0.707106781186548,0.707106781186547,0.707106781186548,
0.707106781186547,0.707106781186547,0.707106781186548,0.707106781186547,
0.707106781186547,0.707106781186548,0.707106781186547,0.707106781186547,
0.707106781186548,0.707106781186547,0.707106781186548,0.707106781186547,
0.707106781186547,0.707106781186548,0.707106781186548,0.707106781186547,
0.707106781186548,0.707106781186547,0.707106781186548,0.707106781186547,
0.707106781186548,0.707106781186547,0.707106781186548,0.707106781186547,
0.707106781186548,0.707106781186547,0.707106781186548,0.707106781186547,
0.707106781186548,0.707106781186547,0.707106781186547,0.707106781186548,
0.707106781186547,0.707106781186548,0.707106781186547,0.707106781186548,
0.707106781186547,0.707106781186548,0.707106781186547,0.707106781186547,
0.707106781186548,0.707106781186547,0.707106781186548,0.707106781186548,
0.707106781186548,0.707106781186547,0.707106781186547,0.707106781186547,
0.707106781186547,0.707106781186548,0.707106781186547,0.707106781186548,
0.707106781186548,0.707106781186547,0.707106781186547,0.707106781186548,
0.707106781186548,0.707106781186547,0.707106781186547,0.707106781186548,
0.707106781186547,0.707106781186548,0.707106781186547,0.707106781186547,
0.707106781186547,0.707106781186547,0.707106781186547,0.707106781186547,
0.707106781186547,0.707106781186548,0.707106781186547,0.707106781186548,
0.707106781186547,0.707106781186548,0.707106781186548,0.707106781186547,
0.707106781186548,0.707106781186548,0.707106781186548,0.707106781186548,
0.707106781186547,0.707106781186548,0.707106781186547,0.707106781186548,
0.707106781186547,0.707106781186547,0.707106781186548,0.707106781186548,
0.707106781186547,0.707106781186547,0.707106781186547,0.707106781186547,
0.707106781186547,0.707106781186548,0.707106781186548,0.707106781186547,
0.707106781186547,0.707106781186548,0.707106781186548,0.707106781186547,
0.707106781186548,0.707106781186547,0.707106781186548,0.707106781186548,
0.707106781186547,0.707106781186547,0.707106781186548,0.707106781186547,
0.707106781186547,0.707106781186548,0.707106781186547,0.707106781186548,
0.707106781186547,0.707106781186548,0.707106781186547,0.707106781186547,
0.707106781186548,0.707106781186548,0.707106781186547,0.707106781186547,
0.707106781186548,0.707106781186547,0.707106781186547,0.707106781186548,
0.707106781186547,0.707106781186548,0.707106781186547,0.707106781186548,
0.707106781186547,0.707106781186548,0.707106781186547,0.707106781186547,
0.707106781186547,0.707106781186547,0.707106781186547,0.707106781186547,
0.707106781186548,0.707106781186547,0.707106781186548,0.707106781186547,
0.707106781186548,0.707106781186548,0.707106781186547,0.707106781186548,
0.707106781186548,0.707106781186547,0.707106781186548,0.707106781186547,
0.707106781186547,0.707106781186547,0.707106781186548,0.707106781186547,
0.707106781186547,0.707106781186548,0.707106781186547,0.707106781186548,
0.707106781186547,0.707106781186547,0.707106781186547,0.707106781186548,
0.707106781186548,0.707106781186547,0.707106781186548,0.707106781186548,
0.707106781186547,0.707106781186548,0.707106781186547,0.707106781186548,
0.707106781186548,0.707106781186547,0.707106781186548,0.707106781186548,
0.707106781186548,0.707106781186547,0.707106781186547,0.707106781186548,
0.707106781186547,0.707106781186548,0.707106781186547,0.707106781186547,
0.707106781186548,0.707106781186548,0.707106781186548,0.707106781186547,
0.707106781186547,0.707106781186548,0.707106781186548,0.707106781186547,
0.707106781186547,0.707106781186548,0.707106781186547,0.707106781186547,
0.707106781186548,0.707106781186548,0.707106781186547,0.707106781186547,
0.707106781186547,0.707106781186548,0.707106781186547,0.707106781186547,
0.707106781186547,0.707106781186548,0.707106781186548,0.707106781186547,
0.707106781186548,0.707106781186547,0.707106781186548,0.707106781186547,
0.707106781186548,0.707106781186548,0.707106781186547,0.707106781186547,
0.707106781186548,0.707106781186547,0.707106781186547,0.707106781186548,
0.707106781186547,0.707106781186548,0.707106781186548,0.707106781186547,
0.707106781186548,0.707106781186547,0.707106781186547,0.707106781186547,
0.707106781186548,0.707106781186548,0.707106781186548,0.707106781186547,
0.707106781186548,0.707106781186547,0.707106781186548,0.707106781186547,
0.707106781186547,0.707106781186547,0.707106781186547,0.707106781186548,
0.707106781186548,0.707106781186547,0.707106781186547,0.707106781186548,
0.707106781186547,0.707106781186548,0.707106781186547,0.707106781186548,
0.707106781186547,0.707106781186547,0.707106781186548,0.707106781186547,
0.707106781186548,0.707106781186547,0.707106781186548,0.707106781186548,
0.707106781186547,0.707106781186548,0.707106781186547,0.707106781186548,
0.707106781186548,0.707106781186547,0.707106781186548,0.707106781186547,
0.707106781186547,0.707106781186548,0.707106781186547,0.707106781186548,
0.707106781186547,0.707106781186548,0.707106781186547,0.707106781186547,
0.707106781186548,0.707106781186548,0.707106781186548,0.707106781186548,
0.707106781186547,0.707106781186548,0.707106781186548,0.707106781186548,
0.707106781186547,0.707106781186548,0.707106781186548,0.707106781186548,
0.707106781186547,0.707106781186547,0.707106781186548,0.707106781186547,
0.707106781186548,0.707106781186547,0.707106781186548,0.707106781186548,
0.707106781186547,0.707106781186547,0.707106781186548,0.707106781186547,
0.707106781186548,0.707106781186547,0.707106781186548,0.707106781186548,
0.707106781186547,0.707106781186547,0.707106781186547,0.707106781186548,
0.707106781186548,0.707106781186547,0.707106781186547,0.707106781186548,
0.707106781186548,0.707106781186548,0.707106781186548,0.707106781186547,
0.707106781186547,0.707106781186548,0.707106781186548,0.707106781186547,
0.707106781186548,0.707106781186547,0.707106781186548,0.707106781186547,
0.707106781186548,0.707106781186547,0.707106781186547,0.707106781186548,
0.707106781186547,0.707106781186547,0.707106781186548,0.707106781186547,
0.707106781186548,0.707106781186547,0.707106781186548,0.707106781186547,
0.707106781186548,0.707106781186547,0.707106781186548,0.707106781186547,
0.707106781186548,0.707106781186547,0.707106781186547,0.707106781186548,
0.707106781186548,0.707106781186547,0.707106781186547,0.707106781186547,
0.707106781186548,0.707106781186547,0.707106781186548,0.707106781186547,
0.707106781186548,0.707106781186547,0.707106781186548,0.707106781186547,
0.707106781186547,0.707106781186547,0.707106781186548,0.707106781186547,
0.707106781186548,0.707106781186548,0.707106781186547,0.707106781186548,
0.707106781186547,0.707106781186547,0.707106781186548,0.707106781186547,
0.707106781186547,0.707106781186548,0.707106781186547,0.707106781186547,
0.707106781186547,0.707106781186547,0.707106781186548,0.707106781186547,
0.707106781186547,0.707106781186547,0.707106781186548,0.707106781186547,
0.707106781186547,0.707106781186548,0.707106781186548,0.707106781186547,
0.707106781186548,0.707106781186548,0.707106781186547,0.707106781186547,
0.707106781186548,0.707106781186547,0.707106781186547,0.707106781186548,
0.707106781186547,0.707106781186547,0.707106781186547,0.707106781186548,
0.707106781186547,0.707106781186548,0.707106781186547,0.707106781186548,
0.707106781186547,0.707106781186548,0.707106781186547,0.707106781186548,
0.707106781186547,0.707106781186548,0.707106781186548,0.707106781186547,
0.707106781186547,0.707106781186548,0.707106781186547,0.707106781186548,
0.707106781186547,0.707106781186548,0.707106781186548,0.707106781186547,
0.707106781186548,0.707106781186547,0.707106781186548,0.707106781186548,
0.707106781186547,0.707106781186547,0.707106781186548,0.707106781186547,
0.707106781186548,0.707106781186547,0.707106781186548,0.707106781186547,
0.707106781186548,0.707106781186547,0.707106781186547,0.707106781186547,
0.707106781186547,0.707106781186547,0.707106781186547,0.707106781186547,
0.707106781186547,0.707106781186548,0.707106781186547,0.707106781186548,
0.707106781186547,0.707106781186547,0.707106781186548,0.707106781186547,
0.707106781186548,0.707106781186547,0.707106781186547,0.707106781186548,
0.707106781186547,0.707106781186548,0.707106781186547,0.707106781186548,
0.707106781186547,0.707106781186548,0.707106781186547,0.707106781186548,
0.707106781186547,0.707106781186548,0.707106781186547,0.707106781186548,
0.707106781186548,0.707106781186547,0.707106781186548,0.707106781186547,
0.707106781186547,0.707106781186547,0.707106781186548,0.707106781186547,
0.707106781186547,0.707106781186547,0.707106781186548,0.707106781186547,
0.707106781186547,0.707106781186548,0.707106781186547,0.707106781186547,
0.707106781186547,0.707106781186547,0.707106781186548,0.707106781186547,
0.707106781186547,0.707106781186547,0.707106781186548,0.707106781186548,
0.707106781186548,0.707106781186548,0.707106781186547,0.707106781186548,
0.707106781186547,0.707106781186547,0.707106781186548,0.707106781186547,
0.707106781186548,0.707106781186547,0.707106781186547,0.707106781186548,
0.707106781186547,0.707106781186547,0.707106781186547,0.707106781186547,
0.707106781186548,0.707106781186548,0.707106781186547,0.707106781186547,
0.707106781186548,0.707106781186547,0.707106781186548,0.707106781186547,
0.707106781186548,0.707106781186548,0.707106781186547,0.707106781186547,
0.707106781186548,0.707106781186548,0.707106781186547,0.707106781186548,
0.707106781186548,0.707106781186547,0.707106781186548,0.707106781186548,
0.707106781186548,0.707106781186547,0.707106781186548,0.707106781186547,
0.707106781186548,0.707106781186547,0.707106781186548,0.707106781186547,
0.707106781186548,0.707106781186547,0.707106781186548,0.707106781186548,
0.707106781186547,0.707106781186547,0.707106781186548,0.707106781186547,
0.707106781186548,0.707106781186547,0.707106781186548,0.707106781186548,
0.707106781186548,0.707106781186548,0.707106781186548,0.707106781186547,
0.707106781186547,0.707106781186547,0.707106781186547,0.707106781186548,
0.707106781186547,0.707106781186548,0.707106781186547,0.707106781186547,
0.707106781186548,0.707106781186548,0.707106781186547,0.707106781186548,
0.707106781186547,0.707106781186548,0.707106781186548,0.707106781186547,
0.707106781186547,0.707106781186548,0.707106781186547,0.707106781186548,
0.707106781186547,0.707106781186548,0.707106781186547,0.707106781186548,
0.707106781186547,0.707106781186548,0.707106781186547,0.707106781186548,
0.707106781186547,0.707106781186548,0.707106781186548,0.707106781186547,
0.707106781186548,0.707106781186547,0.707106781186548,0.707106781186547,
0.707106781186548,0.707106781186548,0.707106781186548,0.707106781186547,
0.707106781186547,0.707106781186548,0.707106781186548,0.707106781186547,
0.707106781186547,0.707106781186547,0.707106781186548,0.707106781186547,
0.707106781186548,0.707106781186547,0.707106781186548,0.707106781186547,
0.707106781186547,0.707106781186547,0.707106781186548,0.707106781186547,
0.707106781186548,0.707106781186547,0.707106781186548,0.707106781186547,
0.707106781186548,0.707106781186547,0.707106781186547,0.707106781186548,
0.707106781186547,0.707106781186547,0.707106781186548,0.707106781186547,
0.707106781186547,0.707106781186548,0.707106781186547,0.707106781186547,
0.707106781186547,0.707106781186548,0.707106781186547,0.707106781186548,
0.707106781186547,0.707106781186547,0.707106781186547,0.707106781186548,
0.707106781186548,0.707106781186547,0.707106781186547,0.707106781186548,
0.707106781186548,0.707106781186548,0.707106781186547,0.707106781186548,
0.707106781186547,0.707106781186548,0.707106781186547,0.707106781186548,
0.707106781186547,0.707106781186547,0.707106781186547,0.707106781186547,
0.707106781186548,0.707106781186547,0.707106781186548,0.707106781186548,
0.707106781186547,0.707106781186548,0.707106781186547,0.707106781186547,
0.707106781186547,0.707106781186547,0.707106781186548,0.707106781186547,
0.707106781186548,0.707106781186547,0.707106781186548,0.707106781186548,
0.707106781186547,0.707106781186548,0.707106781186547,0.707106781186547,
0.707106781186547,0.707106781186547,0.707106781186548,0.707106781186547,
0.707106781186548,0.707106781186548,0.707106781186547,0.707106781186548,
0.707106781186547,0.707106781186548,0.707106781186547,0.707106781186547,
0.707106781186548,0.707106781186547,0.707106781186548,0.707106781186548,
0.707106781186547,0.707106781186547,0.707106781186548,0.707106781186548,
0.707106781186547,0.707106781186547,0.707106781186548,0.707106781186547,
0.707106781186547,0.707106781186548,0.707106781186547,0.707106781186547,
0.707106781186548,0.707106781186547,0.707106781186548,0.707106781186547,
0.707106781186547,0.707106781186548,0.707106781186547,0.707106781186548,
0.707106781186547,0.707106781186548,0.707106781186547,0.707106781186547,
0.707106781186547,0.707106781186548,0.707106781186547,0.707106781186548,
0.707106781186547,0.707106781186548,0.707106781186548,0.707106781186548,
0.707106781186548,0.707106781186547,0.707106781186547,0.707106781186547,
0.707106781186548,0.707106781186547,0.707106781186548,0.707106781186547,
0.707106781186547,0.707106781186548,0.707106781186547,0.707106781186547,
0.707106781186548,0.707106781186547,0.707106781186547,0.707106781186548,
0.707106781186548,0.707106781186547,0.707106781186548,0.707106781186547,
0.707106781186547,0.707106781186548,0.707106781186547,0.707106781186548,
0.707106781186547,0.707106781186548,0.707106781186547,0.707106781186547,
0.707106781186547,0.707106781186548,0.707106781186547,0.707106781186548,
0.707106781186547,0.707106781186548,0.707106781186547,0.707106781186547,
0.707106781186548,0.707106781186548,0.707106781186548,0.707106781186547,
0.707106781186548,0.707106781186547,0.707106781186548,0.707106781186547,
0.707106781186548,0.707106781186547,0.707106781186548,0.707106781186548,
0.707106781186547,0.707106781186547,0.707106781186547,0.707106781186548,
0.707106781186547,0.707106781186547,0.707106781186548,0.707106781186547,
0.707106781186547,0.707106781186548,0.707106781186547,0.707106781186548,
0.707106781186548,0.707106781186548,0.707106781186547,0.707106781186548,
0.707106781186547,0.707106781186548,0.707106781186547,0.707106781186548,
0.707106781186547,0.707106781186548,0.707106781186547,0.707106781186548,
0.707106781186547,0.707106781186548,0.707106781186548,0.707106781186547,
0.707106781186548,0.707106781186547,0.707106781186548,0.707106781186548,
0.707106781186547,0.707106781186547,0.707106781186548,0.707106781186547,
0.707106781186547,0.707106781186548,0.707106781186547,0.707106781186548,
0.707106781186548,0.707106781186547,0.707106781186548,0.707106781186548,
0.707106781186548,0.707106781186548,0.707106781186548,0.707106781186547,
0.707106781186548,0.707106781186548,0.707106781186548,0.707106781186547,
0.707106781186548,0.707106781186547,0.707106781186548,0.707106781186547,
0.707106781186548,0.707106781186547,0.707106781186548,0.707106781186547,
0.707106781186548,0.707106781186547,0.707106781186547,0.707106781186548,
0.707106781186547,0.707106781186547,0.707106781186548,0.707106781186547,
0.707106781186548,0.707106781186547,0.707106781186548,0.707106781186547,
0.707106781186548,0.707106781186547,0.707106781186547,0.707106781186548,
0.707106781186547,0.707106781186547,0.707106781186548,0.707106781186547,
0.707106781186548,0.707106781186547,0.707106781186547,0.707106781186548,
0.707106781186548,0.707106781186547,0.707106781186548,0.707106781186547,
0.707106781186547,0.707106781186547,0.707106781186548,0.707106781186547,
0.707106781186547,0.707106781186548,0.707106781186547,0.707106781186547,
0.707106781186547,0.707106781186548,0.707106781186548,0.707106781186547,
0.707106781186548,0.707106781186547,0.707106781186548,0.707106781186547,
0.707106781186547,0.707106781186548,0.707106781186547,0.707106781186548,
0.707106781186547,0.707106781186547,0.707106781186547,0.707106781186547,
0.707106781186548,0.707106781186547,0.707106781186547,0.707106781186547,
0.707106781186547,0.707106781186547,0.707106781186548,0.707106781186547,
0.707106781186547,0.707106781186547,0.707106781186547,0.707106781186548,
0.707106781186547,0.707106781186548,0.707106781186547,0.707106781186547,
0.707106781186548,0.707106781186547,0.707106781186548,0.707106781186547,
0.707106781186547,0.707106781186548,0.707106781186547,0.707106781186547,
0.707106781186548,0.707106781186547,0.707106781186547,0.707106781186547,
0.707106781186547,0.707106781186548,0.707106781186547,0.707106781186548,
0.707106781186548,0.707106781186547,0.707106781186548,0.707106781186548,
0.707106781186547,0.707106781186547,0.707106781186548,0.707106781186547,
0.707106781186547,0.707106781186547,0.707106781186548,0.707106781186547,
0.707106781186547,0.707106781186548,0.707106781186547,0.707106781186548,
0.707106781186547,0.707106781186548,0.707106781186547,0.707106781186547,
0.707106781186548,0.707106781186547,0.707106781186548,0.707106781186547,
0.707106781186548,0.707106781186547,0.707106781186548,0.707106781186547,
0.707106781186548,0.707106781186547,0.707106781186547,0.707106781186547,
0.707106781186547,0.707106781186548,0.707106781186548,0.707106781186547,
0.707106781186548,0.707106781186548,0.707106781186547,0.707106781186548,
0.707106781186547,0.707106781186547,0.707106781186548,0.707106781186547,
0.707106781186547,0.707106781186547,0.707106781186547,0.707106781186548,
0.707106781186547,0.707106781186547,0.707106781186547,0.707106781186548,
0.707106781186547,0.707106781186547,0.707106781186548,0.707106781186547,
0.707106781186548,0.707106781186548,0.707106781186547,0.707106781186548,
0.707106781186547,0.707106781186548,0.707106781186547,0.707106781186548,
0.707106781186547,0.707106781186547,0.707106781186548,0.707106781186547,
0.707106781186548,0.707106781186548,0.707106781186547,0.707106781186547,
0.707106781186548,0.707106781186547,0.707106781186548,0.707106781186547,
0.707106781186548,0.707106781186547,0.707106781186547,0.707106781186548,
0.707106781186548,0.707106781186547,0.707106781186548,0.707106781186548,
0.707106781186547,0.707106781186548,0.707106781186548,0.707106781186547,
0.707106781186548,0.707106781186547,0.707106781186548,0.707106781186547,
0.707106781186548,0.707106781186547,0.707106781186548,0.707106781186547,
0.707106781186547,0.707106781186548,0.707106781186547,0.707106781186547,
0.707106781186548,0.707106781186547,0.707106781186548,0.707106781186548,
0.707106781186547,0.707106781186547,0.707106781186547,0.707106781186548,
0.707106781186547,0.707106781186548,0.707106781186548,0.707106781186547,
0.707106781186548,0.707106781186547,0.707106781186548,0.707106781186547,
0.707106781186548,0.707106781186547,0.707106781186547,0.707106781186548,
0.707106781186548,0.707106781186548,0.707106781186547,0.707106781186548,
0.707106781186548,0.707106781186547,0.707106781186548,0.707106781186547,
0.707106781186548,0.707106781186548,0.707106781186548,0.707106781186548,
0.707106781186548,0.707106781186548,0.707106781186547,0.707106781186547,
0.707106781186548,0.707106781186547,0.707106781186547,0.707106781186548,
0.707106781186547,0.707106781186547,0.707106781186548,0.707106781186547,
0.707106781186548,0.707106781186547,0.707106781186548,0.707106781186547,
0.707106781186547,0.707106781186547,0.707106781186548,0.707106781186547,
0.707106781186547,0.707106781186548,0.707106781186547,0.707106781186548,
0.707106781186547,0.707106781186548,0.707106781186547,0.707106781186547,
0.707106781186547,0.707106781186547,0.707106781186548,0.707106781186547,
0.707106781186547,0.707106781186548,0.707106781186548,0.707106781186547,
0.707106781186548,0.707106781186547,0.707106781186548,0.707106781186547,
0.707106781186547,0.707106781186548,0.707106781186547,0.707106781186548,
0.707106781186547,0.707106781186548,0.707106781186547,0.707106781186548,
0.707106781186548,0.707106781186547,0.707106781186548,0.707106781186547,
0.707106781186547,0.707106781186548,0.707106781186547,0.707106781186547,
0.707106781186548,0.707106781186548,0.707106781186548,0.707106781186547,
0.707106781186548,0.707106781186547,0.707106781186547,0.707106781186547,
0.707106781186548,0.707106781186547,0.707106781186548,0.707106781186548,
0.707106781186548,0.707106781186547,0.707106781186547,0.707106781186547,
0.707106781186547,0.707106781186548,0.707106781186547,0.707106781186547,
0.707106781186548,0.707106781186547,0.707106781186548,0.707106781186547,
0.707106781186547,0.707106781186548,0.707106781186547,0.707106781186548,
0.707106781186547,0.707106781186548,0.707106781186547,0.707106781186547,
0.707106781186547,0.707106781186547,0.707106781186547,0.707106781186547,
0.707106781186548,0.707106781186547,0.707106781186547,0.707106781186548,
0.707106781186548,0.707106781186547,0.707106781186548,0.707106781186548,
0.707106781186547,0.707106781186547,0.707106781186548,0.707106781186547,
0.707106781186547,0.707106781186548,0.707106781186547,0.707106781186548,
0.707106781186548,0.707106781186548,0.707106781186547,0.707106781186547,
0.707106781186547,0.707106781186547,0.707106781186548,0.707106781186548,
0.707106781186548,0.707106781186547,0.707106781186548,0.707106781186547,
0.707106781186548,0.707106781186548,0.707106781186547,0.707106781186548,
0.707106781186547,0.707106781186548,0.707106781186548,0.707106781186547,
0.707106781186547,0.707106781186548,0.707106781186547,0.707106781186548,
0.707106781186547,0.707106781186548,0.707106781186548,0.707106781186548,
0.707106781186547,0.707106781186548,0.707106781186547,0.707106781186547,
0.707106781186547,0.707106781186547,0.707106781186548,0.707106781186548,
0.707106781186547,0.707106781186547,0.707106781186547,0.707106781186548,
0.707106781186547,0.707106781186547,0.707106781186548,0.707106781186547,
0.707106781186548,0.707106781186548,0.707106781186548,0.707106781186547,
0.707106781186547,0.707106781186547,0.707106781186547,0.707106781186548,
0.707106781186548,0.707106781186547,0.707106781186548,0.707106781186547,
0.707106781186548,0.707106781186548,0.707106781186547,0.707106781186548,
0.707106781186547,0.707106781186548,0.707106781186547,0.707106781186547,
0.707106781186547,0.707106781186548,0.707106781186547,0.707106781186548,
0.707106781186547,0.707106781186548,0.707106781186547,0.707106781186548,
0.707106781186547,0.707106781186548,0.707106781186547,0.707106781186547,
0.707106781186548,0.707106781186547,0.707106781186548,0.707106781186547,
0.707106781186547,0.707106781186548,0.707106781186548,0.707106781186547,
0.707106781186548,0.707106781186548,0.707106781186547,0.707106781186548,
0.707106781186547,0.707106781186548,0.707106781186547,0.707106781186547,
0.707106781186547,0.707106781186548,0.707106781186547,0.707106781186547,
0.707106781186548,0.707106781186547,0.707106781186548,0.707106781186547,
0.707106781186548,0.707106781186548,0.707106781186547,0.707106781186548,
0.707106781186547,0.707106781186548,0.707106781186548,0.707106781186548,
0.707106781186548,0.707106781186547,0.707106781186547,0.707106781186548,
0.707106781186547,0.707106781186547,0.707106781186548,0.707106781186548,
0.707106781186547,0.707106781186547,0.707106781186548,0.707106781186547,
0.707106781186547,0.707106781186548,0.707106781186547,0.707106781186548,
0.707106781186547,0.707106781186548,0.707106781186547,0.707106781186547,
0.707106781186547,0.707106781186548,0.707106781186547,0.707106781186547,
0.707106781186548,0.707106781186547,0.707106781186548,0.707106781186548,
0.707106781186548,0.707106781186547,0.707106781186547,0.707106781186547,
0.707106781186548,0.707106781186548,0.707106781186547,0.707106781186547,
0.707106781186547,0.707106781186547,0.707106781186548,0.707106781186548,
0.707106781186547,0.707106781186547,0.707106781186547,0.707106781186548,
0.707106781186548,0.707106781186547,0.707106781186548,0.707106781186547,
0.707106781186548,0.707106781186547,0.707106781186548,0.707106781186548,
0.707106781186547,0.707106781186548,0.707106781186548,0.707106781186548,
0.707106781186547,0.707106781186547,0.707106781186547,0.707106781186548,
0.707106781186548,0.707106781186548,0.707106781186547,0.707106781186547,
0.707106781186548,0.707106781186548,0.707106781186547,0.707106781186548,
0.707106781186547,0.707106781186547,0.707106781186548,0.707106781186547,
0.707106781186548,0.707106781186547,0.707106781186547,0.707106781186548,
0.707106781186547,0.707106781186548,0.707106781186548,0.707106781186547,
0.707106781186547,0.707106781186548,0.707106781186547,0.707106781186548,
0.707106781186547,0.707106781186547,0.707106781186548,0.707106781186547,
0.707106781186548,0.707106781186547,0.707106781186548,0.707106781186547,
0.707106781186547,0.707106781186548,0.707106781186547,0.707106781186547,
0.707106781186547,0.707106781186547,0.707106781186547,0.707106781186547,
0.707106781186548,0.707106781186547,0.707106781186548,0.707106781186548,
0.707106781186548,0.707106781186547,0.707106781186547,0.707106781186547,
0.707106781186548,0.707106781186547,0.707106781186548,0.707106781186547,
0.707106781186547,0.707106781186548,0.707106781186547,0.707106781186547,
0.707106781186547,0.707106781186547,0.707106781186547,0.707106781186548,
0.707106781186547,0.707106781186548,0.707106781186547,0.707106781186547,
0.707106781186548,0.707106781186548,0.707106781186547,0.707106781186547,
0.707106781186547,0.707106781186548,0.707106781186547,0.707106781186547,
0.707106781186548,0.707106781186548,0.707106781186547,0.707106781186548,
0.707106781186547,0.707106781186548,0.707106781186548,0.707106781186547,
0.707106781186547,0.707106781186547,0.707106781186548,0.707106781186548,
0.707106781186547,0.707106781186548,0.707106781186547,0.707106781186548,
0.707106781186548,0.707106781186547,0.707106781186548,0.707106781186547,
0.707106781186547,0.707106781186547,0.707106781186548,0.707106781186547,
0.707106781186548,0.707106781186547,0.707106781186548,0.707106781186547,
0.707106781186547,0.707106781186547,0.707106781186547,0.707106781186547,
0.707106781186548,0.707106781186547,0.707106781186548,0.707106781186547,
0.707106781186548,0.707106781186547,0.707106781186548,0.707106781186547,
0.707106781186547,0.707106781186547,0.707106781186547,0.707106781186547,
0.707106781186548,0.707106781186548,0.707106781186548,0.707106781186547,
0.707106781186548,0.707106781186547,0.707106781186548,0.707106781186547,
0.707106781186547,0.707106781186548,0.707106781186547,0.707106781186548,
0.707106781186547,0.707106781186547,0.707106781186547,0.707106781186548,
0.707106781186548,0.707106781186547,0.707106781186548,0.707106781186547,
0.707106781186548,0.707106781186548,0.707106781186547,0.707106781186548,
0.707106781186547,0.707106781186548,0.707106781186548,0.707106781186547,
0.707106781186547,0.707106781186547,0.707106781186547,0.707106781186547,
0.707106781186547,0.707106781186548,0.707106781186548,0.707106781186547,
0.707106781186548,0.707106781186547,0.707106781186547,0.707106781186548,
0.707106781186547,0.707106781186547,0.707106781186548,0.707106781186547,
0.707106781186547,0.707106781186547,0.707106781186548,0.707106781186547,
0.707106781186547,0.707106781186548,0.707106781186547,0.707106781186548,
0.707106781186548,0.707106781186547,0.707106781186547,0.707106781186547,
0.707106781186548,0.707106781186547,0.707106781186547,0.707106781186548,
0.707106781186548,0.707106781186548,0.707106781186548,0.707106781186547,
0.707106781186548,0.707106781186548,0.707106781186547,0.707106781186547,
0.707106781186548,0.707106781186547,0.707106781186548,0.707106781186547,
0.707106781186547,0.707106781186548,0.707106781186547,0.707106781186547,
0.707106781186548,0.707106781186547,0.707106781186548,0.707106781186547,
0.707106781186548,0.707106781186547,0.707106781186548,0.707106781186547,
0.707106781186548,0.707106781186547,0.707106781186548,0.707106781186548,
0.707106781186547,0.707106781186547,0.707106781186548,0.707106781186548,
0.707106781186547,0.707106781186547,0.707106781186547,0.707106781186547,
0.707106781186547,0.707106781186548,0.707106781186547,0.707106781186547,
0.707106781186548,0.707106781186547,0.707106781186548,0.707106781186548,
0.707106781186547,0.707106781186548,0.707106781186547,0.707106781186548,
0.707106781186547,0.707106781186548,0.707106781186547,0.707106781186547,
0.707106781186547,0.707106781186547,0.707106781186547,0.707106781186547,
0.707106781186548,0.707106781186547,0.707106781186548,0.707106781186547,
0.707106781186547,0.707106781186547,0.707106781186548,0.707106781186547,
0.707106781186548,0.707106781186548,0.707106781186547,0.707106781186547,
0.707106781186548,0.707106781186547,0.707106781186548,0.707106781186547,
0.707106781186548,0.707106781186547,0.707106781186548,0.707106781186547,
0.707106781186547,0.707106781186548,0.707106781186547,0.707106781186548,
0.707106781186547,0.707106781186548,0.707106781186548,0.707106781186548,
0.707106781186548,0.707106781186547,0.707106781186548,0.707106781186548,
0.707106781186548,0.707106781186547,0.707106781186548,0.707106781186548,
0.707106781186547,0.707106781186548,0.707106781186547,0.707106781186548,
0.707106781186547,0.707106781186547,0.707106781186547,0.707106781186548,
0.707106781186548,0.707106781186547,0.707106781186548,0.707106781186547,
0.707106781186548,0.707106781186547,0.707106781186548,0.707106781186548,
0.707106781186547,0.707106781186548,0.707106781186547,0.707106781186547,
0.707106781186548,0.707106781186547,0.707106781186547,0.707106781186547,
0.707106781186548,0.707106781186547,0.707106781186548,0.707106781186548,
0.707106781186547,0.707106781186548,0.707106781186547,0.707106781186548,
0.707106781186548,0.707106781186548,0.707106781186548,0.707106781186547,
0.707106781186548,0.707106781186547,0.707106781186548,0.707106781186547,
0.707106781186548,0.707106781186547,0.707106781186547,0.707106781186547,
0.707106781186547,0.707106781186548,0.707106781186547,0.707106781186548,
0.707106781186547,0.707106781186547,0.707106781186548,0.707106781186547,
0.707106781186548,0.707106781186547,0.707106781186548,0.707106781186547,
0.707106781186548,0.707106781186548,0.707106781186548,0.707106781186548,
0.707106781186547,0.707106781186548,0.707106781186548,0.707106781186547,
0.707106781186548,0.707106781186547,0.707106781186548,0.707106781186547,
0.707106781186548,0.707106781186547,0.707106781186547,0.707106781186548,
0.707106781186547,0.707106781186548,0.707106781186547,0.707106781186547,
0.707106781186548,0.707106781186547,0.707106781186548,0.707106781186547,
0.707106781186547,0.707106781186548,0.707106781186548,0.707106781186548,
0.707106781186548,0.707106781186548,0.707106781186548,0.707106781186548,
0.707106781186548,0.707106781186548,0.707106781186547,0.707106781186548,
0.707106781186547,0.707106781186547,0.707106781186548,0.707106781186547,
0.707106781186548,0.707106781186548,0.707106781186547,0.707106781186547,
0.707106781186548,0.707106781186548,0.707106781186547,0.707106781186547,
0.707106781186547,0.707106781186547,0.707106781186547,0.707106781186548,
0.707106781186547,0.707106781186548,0.707106781186548,0.707106781186548,
0.707106781186547,0.707106781186548,0.707106781186547,0.707106781186548,
0.707106781186547,0.707106781186548,0.707106781186547,0.707106781186548,
0.707106781186548,0.707106781186547,0.707106781186547,0.707106781186548,
0.707106781186548,0.707106781186548,0.707106781186547,0.707106781186547,
0.707106781186548,0.707106781186547,0.707106781186547,0.707106781186548,
0.707106781186547,0.707106781186548,0.707106781186547,0.707106781186547,
0.707106781186548,0.707106781186548,0.707106781186548,0.707106781186547,
0.707106781186547,0.707106781186548,0.707106781186547,0.707106781186548,
0.707106781186547,0.707106781186548,0.707106781186547,0.707106781186548,
0.707106781186548,0.707106781186547,0.707106781186548,0.707106781186547,
0.707106781186548,0.707106781186547,0.707106781186547,0.707106781186547,
0.707106781186548,0.707106781186547,0.707106781186548,0.707106781186547,
0.707106781186547,0.707106781186547,0.707106781186548,0.707106781186547,
0.707106781186547,0.707106781186548,0.707106781186548,0.707106781186547,
0.707106781186548,0.707106781186547,0.707106781186548,0.707106781186548,
0.707106781186547,0.707106781186548,0.707106781186547,0.707106781186547,
0.707106781186548,0.707106781186547,0.707106781186547,0.707106781186547,
0.707106781186548,0.707106781186547,0.707106781186548,0.707106781186547,
0.707106781186548,0.707106781186548,0.707106781186548,0.707106781186547,
0.707106781186548,0.707106781186548,0.707106781186548,0.707106781186547,
0.707106781186548,0.707106781186547,0.707106781186547,0.707106781186548,
0.707106781186547,0.707106781186547,0.707106781186548,0.707106781186548,
0.707106781186547,0.707106781186548,0.707106781186547,0.707106781186548,
0.707106781186548,0.707106781186547,0.707106781186548,0.707106781186547,
0.707106781186548,0.707106781186547,0.707106781186548,0.707106781186547,
0.707106781186548,0.707106781186548,0.707106781186548,0.707106781186547,
0.707106781186548,0.707106781186548,0.707106781186547,0.707106781186547,
0.707106781186548,0.707106781186547,0.707106781186548,0.707106781186548,
0.707106781186547,0.707106781186548,0.707106781186548,0.707106781186547,
0.707106781186548,0.707106781186548,0.707106781186547,0.707106781186547,
0.707106781186548,0.707106781186547,0.707106781186548,0.707106781186547,
0.707106781186548,0.707106781186547,0.707106781186548,0.707106781186548,
0.707106781186548,0.707106781186547,0.707106781186548,0.707106781186547,
0.707106781186548,0.707106781186547,0.707106781186548,0.707106781186547,
0.707106781186548,0.707106781186547,0.707106781186548,0.707106781186547,
0.707106781186548,0.707106781186547,0.707106781186547,0.707106781186547,
0.707106781186548,0.707106781186547,0.707106781186548,0.707106781186547,
0.707106781186548,0.707106781186547,0.707106781186548,0.707106781186547,
0.707106781186548,0.707106781186548,0.707106781186548,0.707106781186547,
0.707106781186548,0.707106781186547,0.707106781186548,0.707106781186548,
0.707106781186547,0.707106781186548,0.707106781186547,0.707106781186548,
0.707106781186547,0.707106781186548,0.707106781186547,0.707106781186548,
0.707106781186547,0.707106781186547,0.707106781186547,0.707106781186548,
0.707106781186547,0.707106781186547,0.707106781186548,0.707106781186547,
0.707106781186548,0.707106781186547,0.707106781186547,0.707106781186548,
0.707106781186547,0.707106781186548,0.707106781186547,0.707106781186548,
0.707106781186548,0.707106781186548,0.707106781186547,0.707106781186547,
0.707106781186548,0.707106781186548,0.707106781186547,0.707106781186548,
0.707106781186547,0.707106781186547,0.707106781186547,0.707106781186548,
0.707106781186547,0.707106781186548,0.707106781186547,0.707106781186548,
0.707106781186548,0.707106781186548,0.707106781186547,0.707106781186547,
0.707106781186547,0.707106781186547,0.707106781186547,0.707106781186547,
0.707106781186548,0.707106781186547,0.707106781186548,0.707106781186547,
0.707106781186548,0.707106781186547,0.707106781186547,0.707106781186548,
0.707106781186547,0.707106781186547,0.707106781186548,0.707106781186548,
0.707106781186547,0.707106781186547,0.707106781186547,0.707106781186548,
0.707106781186547,0.707106781186547,0.707106781186548,0.707106781186548),
(1.,1.,1.,1.,1.,1.,1.,1.,1.,1.,1.,1.,1.,1.,1.,1.,1.,1.,1.,1.,1.,1.,1.,1.,
1.,1.,1.,1.,1.,1.,1.,1.,1.,1.,1.,1.,1.,1.,1.,1.,1.,1.,1.,1.,1.,1.,1.,1.,
1.,1.,1.,1.,1.,1.,1.,1.,1.,1.,1.,1.,1.,1.,1.,1.,1.,1.,1.,1.,1.,1.,1.,1.,
1.,1.,1.,1.,1.,1.,1.,1.,1.,1.,1.,1.,1.,1.,1.,1.,1.,1.,1.,1.,1.,1.,1.,1.,
1.,1.,1.,1.,1.,1.,1.,1.,1.,1.,1.,1.,1.,1.,1.,1.,1.,1.,1.,1.,1.,1.,1.,1.,
1.,1.,1.,1.,1.,1.,1.,1.,1.,1.,1.,1.,1.,1.,1.,1.,1.,1.,1.,1.,1.,1.,1.,1.,
1.,1.,1.,1.,1.,1.,1.,1.,1.,1.,1.,1.,1.,1.,1.,1.,1.,1.,1.,1.,1.,1.,1.,1.,
1.,1.,1.,1.,1.,1.,1.,1.,1.,1.,1.,1.,1.,1.,1.,1.,1.,1.,1.,1.,1.,1.,1.,1.,
1.,1.,1.,1.,1.,1.,1.,1.,1.,1.,1.,1.,1.,1.,1.,1.,1.,1.,1.,1.,1.,1.,1.,1.,
1.,1.,1.,1.,1.,1.,1.,1.,1.,1.,1.,1.,1.,1.,1.,1.,1.,1.,1.,1.,1.,1.,1.,1.,
1.,1.,1.,1.,1.,1.,1.,1.,1.,1.,1.,1.,1.,1.,1.,1.,1.,1.,1.,1.,1.,1.,1.,1.,
1.,1.,1.,1.,1.,1.,1.,1.,1.,1.,1.,1.,1.,1.,1.,1.,1.,1.,1.,1.,1.,1.,1.,1.,
1.,1.,1.,1.,1.,1.,1.,1.,1.,1.,1.,1.,1.,1.,1.,1.,1.,1.,1.,1.,1.,1.,1.,1.,
1.,1.,1.,1.,1.,1.,1.,1.,1.,1.,1.,1.,1.,1.,1.,1.,1.,1.,1.,1.,1.,1.,1.,1.,
1.,1.,1.,1.,1.,1.,1.,1.,1.,1.,1.,1.,1.,1.,1.,1.,1.,1.,1.,1.,1.,1.,1.,1.,
1.,1.,1.,1.,1.,1.,1.,1.,1.,1.,1.,1.,1.,1.,1.,1.,1.,1.,1.,1.,1.,1.,1.,1.,
1.,1.,1.,1.,1.,1.,1.,1.,1.,1.,1.,1.,1.,1.,1.,1.,1.,1.,1.,1.,1.,1.,1.,1.,
1.,1.,1.,1.,1.,1.,1.,1.,1.,1.,1.,1.,1.,1.,1.,1.,1.,1.,1.,1.,1.,1.,1.,1.,
1.,1.,1.,1.,1.,1.,1.,1.,1.,1.,1.,1.,1.,1.,1.,1.,1.,1.,1.,1.,1.,1.,1.,1.,
1.,1.,1.,1.,1.,1.,1.,1.,1.,1.,1.,1.,1.,1.,1.,1.,1.,1.,1.,1.,1.,1.,1.,1.,
1.,1.,1.,1.,1.,1.,1.,1.,1.,1.,1.,1.,1.,1.,1.,1.,1.,1.,1.,1.,1.,1.,1.,1.,
1.,1.,1.,1.,1.,1.,1.,1.,1.,1.,1.,1.,1.,1.,1.,1.,1.,1.,1.,1.,1.,1.,1.,1.,
1.,1.,1.,1.,1.,1.,1.,1.,1.,1.,1.,1.,1.,1.,1.,1.,1.,1.,1.,1.,1.,1.,1.,1.,
1.,1.,1.,1.,1.,1.,1.,1.,1.,1.,1.,1.,1.,1.,1.,1.,1.,1.,1.,1.,1.,1.,1.,1.,
1.,1.,1.,1.,1.,1.,1.,1.,1.,1.,1.,1.,1.,1.,1.,1.,1.,1.,1.,1.,1.,1.,1.,1.,
1.,1.,1.,1.,1.,1.,1.,1.,1.,1.,1.,1.,1.,1.,1.,1.,1.,1.,1.,1.,1.,1.,1.,1.,
1.,1.,1.,1.,1.,1.,1.,1.,1.,1.,1.,1.,1.,1.,1.,1.,1.,1.,1.,1.,1.,1.,1.,1.,
1.,1.,1.,1.,1.,1.,1.,1.,1.,1.,1.,1.,1.,1.,1.,1.,1.,1.,1.,1.,1.,1.,1.,1.,
1.,1.,1.,1.,1.,1.,1.,1.,1.,1.,1.,1.,1.,1.,1.,1.,1.,1.,1.,1.,1.,1.,1.,1.,
1.,1.,1.,1.,1.,1.,1.,1.,1.,1.,1.,1.,1.,1.,1.,1.,1.,1.,1.,1.,1.,1.,1.,1.,
1.,1.,1.,1.,1.,1.,1.,1.,1.,1.,1.,1.,1.,1.,1.,1.,1.,1.,1.,1.,1.,1.,1.,1.,
1.,1.,1.,1.,1.,1.,1.,1.,1.,1.,1.,1.,1.,1.,1.,1.,1.,1.,1.,1.,1.,1.,1.,1.,
1.,1.,1.,1.,1.,1.,1.,1.,1.,1.,1.,1.,1.,1.,1.,1.,1.,1.,1.,1.,1.,1.,1.,1.,
1.,1.,1.,1.,1.,1.,1.,1.,1.,1.,1.,1.,1.,1.,1.,1.,1.,1.,1.,1.,1.,1.,1.,1.,
1.,1.,1.,1.,1.,1.,1.,1.,1.,1.,1.,1.,1.,1.,1.,1.,1.,1.,1.,1.,1.,1.,1.,1.,
1.,1.,1.,1.,1.,1.,1.,1.,1.,1.,1.,1.,1.,1.,1.,1.,1.,1.,1.,1.,1.,1.,1.,1.,
1.,1.,1.,1.,1.,1.,1.,1.,1.,1.,1.,1.,1.,1.,1.,1.,1.,1.,1.,1.,1.,1.,1.,1.,
1.,1.,1.,1.,1.,1.,1.,1.,1.,1.,1.,1.,1.,1.,1.,1.,1.,1.,1.,1.,1.,1.,1.,1.,
1.,1.,1.,1.,1.,1.,1.,1.,1.,1.,1.,1.,1.,1.,1.,1.,1.,1.,1.,1.,1.,1.,1.,1.,
1.,1.,1.,1.,1.,1.,1.,1.,1.,1.,1.,1.,1.,1.,1.,1.,1.,1.,1.,1.,1.,1.,1.,1.,
1.,1.,1.,1.,1.,1.,1.,1.,1.,1.,1.,1.,1.,1.,1.,1.,1.,1.,1.,1.,1.,1.,1.,1.,
1.,1.,1.,1.,1.,1.,1.,1.,1.,1.,1.,1.,1.,1.,1.,1.,1.,1.,1.,1.,1.,1.,1.,1.,
1.,1.,1.,1.,1.,1.,1.,1.,1.,1.,1.,1.,1.,1.,1.,1.,1.,1.,1.,1.,1.,1.,1.,1.,
1.,1.,1.,1.,1.,1.,1.,1.,1.,1.,1.,1.,1.,1.,1.,1.,1.,1.,1.,1.,1.,1.,1.,1.,
1.,1.,1.,1.,1.,1.,1.,1.,1.,1.,1.,1.,1.,1.,1.,1.,1.,1.,1.,1.,1.,1.,1.,1.,
1.,1.,1.,1.,1.,1.,1.,1.,1.,1.,1.,1.,1.,1.,1.,1.,1.,1.,1.,1.,1.,1.,1.,1.,
1.,1.,1.,1.,1.,1.,1.,1.,1.,1.,1.,1.,1.,1.,1.,1.,1.,1.,1.,1.,1.,1.,1.,1.,
1.,1.,1.,1.,1.,1.,1.,1.,1.,1.,1.,1.,1.,1.,1.,1.,1.,1.,1.,1.,1.,1.,1.,1.,
1.,1.,1.,1.,1.,1.,1.,1.,1.,1.,1.,1.,1.,1.,1.,1.,1.,1.,1.,1.,1.,1.,1.,1.,
1.,1.,1.,1.,1.,1.,1.,1.,1.,1.,1.,1.,1.,1.,1.,1.,1.,1.,1.,1.,1.,1.,1.,1.,
1.,1.,1.,1.,1.,1.,1.,1.,1.,1.,1.,1.,1.,1.,1.,1.,1.,1.,1.,1.,1.,1.,1.,1.,
1.,1.,1.,1.,1.,1.,1.,1.,1.,1.,1.,1.,1.,1.,1.,1.,1.,1.,1.,1.,1.,1.,1.,1.,
1.,1.,1.,1.,1.,1.,1.,1.,1.,1.,1.,1.,1.,1.,1.,1.,1.,1.,1.,1.,1.,1.,1.,1.,
1.,1.,1.,1.,1.,1.,1.,1.,1.,1.,1.,1.,1.,1.,1.,1.,1.,1.,1.,1.,1.,1.,1.,1.,
1.,1.,1.,1.,1.,1.,1.,1.,1.,1.,1.,1.,1.,1.,1.,1.,1.,1.,1.,1.,1.,1.,1.,1.,
1.,1.,1.,1.,1.,1.,1.,1.,1.,1.,1.,1.,1.,1.,1.,1.,1.,1.,1.,1.,1.,1.,1.,1.,
1.,1.,1.,1.,1.,1.,1.,1.,1.,1.,1.,1.,1.,1.,1.,1.,1.,1.,1.,1.,1.,1.,1.,1.,
1.,1.,1.,1.,1.,1.,1.,1.,1.,1.,1.,1.,1.,1.,1.,1.,1.,1.,1.,1.,1.,1.,1.,1.,
1.,1.,1.,1.,1.,1.,1.,1.,1.,1.,1.,1.,1.,1.,1.,1.,1.,1.,1.,1.,1.,1.,1.,1.,
1.,1.,1.,1.,1.,1.,1.,1.,1.,1.,1.,1.,1.,1.,1.,1.,1.,1.,1.,1.,1.,1.,1.,1.,
1.,1.,1.,1.,1.,1.,1.,1.,1.,1.,1.,1.,1.,1.,1.,1.,1.,1.,1.,1.,1.,1.,1.,1.,
1.,1.,1.,1.,1.,1.,1.,1.,1.,1.,1.,1.,1.,1.,1.,1.,1.,1.,1.,1.,1.,1.,1.,1.,
1.,1.,1.,1.,1.,1.,1.,1.,1.,1.,1.,1.,1.,1.,1.,1.,1.,1.,1.,1.,1.,1.,1.,1.,
1.,1.,1.,1.,1.,1.,1.,1.,1.,1.,1.,1.,1.,1.,1.,1.,1.,1.,1.,1.,1.,1.,1.,1.,
1.,1.,1.,1.,1.,1.,1.,1.,1.,1.,1.,1.,1.,1.,1.,1.,1.,1.,1.,1.,1.,1.,1.,1.,
1.,1.,1.,1.,1.,1.,1.,1.,1.,1.,1.,1.,1.,1.,1.,1.,1.,1.,1.,1.,1.,1.,1.,1.,
1.,1.,1.,1.,1.,1.,1.,1.,1.,1.,1.,1.,1.,1.,1.,1.,1.,1.,1.,1.,1.,1.,1.,1.,
1.,1.,1.,1.,1.,1.,1.,1.,1.,1.,1.,1.,1.,1.,1.,1.,1.,1.,1.,1.,1.,1.,1.,1.,
1.,1.,1.,1.,1.,1.,1.,1.,1.,1.,1.,1.,1.,1.,1.,1.,1.,1.,1.,1.,1.,1.,1.,1.,
1.,1.,1.,1.,1.,1.,1.,1.,1.,1.,1.,1.,1.,1.,1.,1.,1.,1.,1.,1.,1.,1.,1.,1.,
1.,1.,1.,1.,1.,1.,1.,1.,1.,1.,1.,1.,1.,1.,1.,1.,1.,1.,1.,1.,1.,1.,1.,1.,
1.,1.,1.,1.,1.,1.,1.,1.,1.,1.,1.,1.,1.,1.,1.,1.,1.,1.,1.,1.,1.,1.,1.,1.,
1.,1.,1.,1.,1.,1.,1.,1.,1.,1.,1.,1.,1.,1.,1.,1.,1.,1.,1.,1.,1.,1.,1.,1.,
1.,1.,1.,1.,1.,1.,1.,1.,1.,1.,1.,1.,1.,1.,1.,1.,1.,1.,1.,1.,1.,1.,1.,1.,
1.,1.,1.,1.,1.,1.,1.,1.,1.,1.,1.,1.,1.,1.,1.,1.,1.,1.,1.,1.,1.,1.,1.,1.,
1.,1.,1.,1.,1.,1.,1.,1.,1.,1.,1.,1.,1.,1.,1.,1.,1.,1.,1.,1.,1.,1.,1.,1.,
1.,1.,1.,1.,1.,1.,1.,1.,1.,1.,1.,1.,1.,1.,1.,1.,1.,1.,1.,1.,1.,1.,1.,1.,
1.,1.,1.,1.,1.,1.,1.,1.,1.,1.,1.,1.,1.,1.,1.,1.,1.,1.,1.,1.,1.,1.,1.,1.,
1.,1.,1.,1.,1.,1.,1.,1.,1.,1.,1.,1.,1.,1.,1.,1.,1.,1.,1.,1.,1.,1.,1.,1.,
1.,1.,1.,1.,1.,1.,1.,1.,1.,1.,1.,1.,1.,1.,1.,1.,1.,1.,1.,1.,1.,1.,1.,1.,
1.,1.,1.,1.,1.,1.,1.,1.,1.,1.,1.,1.,1.,1.,1.,1.,1.,1.,1.,1.,1.,1.,1.,1.,
1.,1.,1.,1.,1.,1.,1.,1.,1.,1.,1.,1.,1.,1.,1.,1.,1.,1.,1.,1.,1.,1.,1.,1.,
1.,1.,1.,1.,1.,1.,1.,1.,1.,1.,1.,1.,1.,1.,1.,1.,1.,1.,1.,1.,1.,1.,1.,1.,
1.,1.,1.,1.,1.,1.,1.,1.,1.,1.,1.,1.,1.,1.,1.,1.,1.,1.,1.,1.,1.,1.,1.,1.,
1.,1.,1.,1.,1.,1.,1.,1.,1.,1.,1.,1.,1.,1.,1.,1.,1.,1.,1.,1.,1.,1.,1.,1.,
1.,1.,1.,1.,1.,1.,1.,1.,1.,1.,1.),(0.707106781186548,0.707106781186548,
0.707106781186548,0.707106781186547,0.707106781186547,0.707106781186548,
0.707106781186547,0.707106781186547,0.707106781186547,0.707106781186547,
0.707106781186547,0.707106781186548,0.707106781186548,0.707106781186548,
0.707106781186547,0.707106781186548,0.707106781186547,0.707106781186547,
0.707106781186548,0.707106781186547,0.707106781186548,0.707106781186547,
0.707106781186548,0.707106781186547,0.707106781186548,0.707106781186547,
0.707106781186547,0.707106781186547,0.707106781186547,0.707106781186547,
0.707106781186548,0.707106781186547,0.707106781186547,0.707106781186548,
0.707106781186547,0.707106781186547,0.707106781186548,0.707106781186547,
0.707106781186547,0.707106781186548,0.707106781186548,0.707106781186547,
0.707106781186548,0.707106781186547,0.707106781186547,0.707106781186547,
0.707106781186548,0.707106781186548,0.707106781186547,0.707106781186547,
0.707106781186548,0.707106781186547,0.707106781186548,0.707106781186547,
0.707106781186547,0.707106781186547,0.707106781186547,0.707106781186547,
0.707106781186548,0.707106781186547,0.707106781186548,0.707106781186547,
0.707106781186548,0.707106781186547,0.707106781186548,0.707106781186547,
0.707106781186547,0.707106781186548,0.707106781186547,0.707106781186547,
0.707106781186548,0.707106781186547,0.707106781186548,0.707106781186547,
0.707106781186548,0.707106781186548,0.707106781186547,0.707106781186548,
0.707106781186547,0.707106781186547,0.707106781186548,0.707106781186547,
0.707106781186547,0.707106781186547,0.707106781186548,0.707106781186547,
0.707106781186547,0.707106781186547,0.707106781186547,0.707106781186547,
0.707106781186547,0.707106781186548,0.707106781186548,0.707106781186547,
0.707106781186548,0.707106781186547,0.707106781186548,0.707106781186548,
0.707106781186547,0.707106781186548,0.707106781186548,0.707106781186548,
0.707106781186547,0.707106781186548,0.707106781186547,0.707106781186548,
0.707106781186548,0.707106781186548,0.707106781186547,0.707106781186547,
0.707106781186547,0.707106781186548,0.707106781186548,0.707106781186548,
0.707106781186547,0.707106781186547,0.707106781186547,0.707106781186548,
0.707106781186548,0.707106781186547,0.707106781186547,0.707106781186548,
0.707106781186547,0.707106781186547,0.707106781186547,0.707106781186547,
0.707106781186548,0.707106781186547,0.707106781186548,0.707106781186547,
0.707106781186547,0.707106781186547,0.707106781186548,0.707106781186548,
0.707106781186547,0.707106781186548,0.707106781186548,0.707106781186547,
0.707106781186548,0.707106781186547,0.707106781186548,0.707106781186547,
0.707106781186548,0.707106781186547,0.707106781186547,0.707106781186548,
0.707106781186547,0.707106781186547,0.707106781186548,0.707106781186547,
0.707106781186547,0.707106781186548,0.707106781186547,0.707106781186548,
0.707106781186547,0.707106781186547,0.707106781186548,0.707106781186548,
0.707106781186547,0.707106781186548,0.707106781186547,0.707106781186548,
0.707106781186547,0.707106781186548,0.707106781186547,0.707106781186548,
0.707106781186547,0.707106781186548,0.707106781186547,0.707106781186548,
0.707106781186547,0.707106781186548,0.707106781186547,0.707106781186547,
0.707106781186548,0.707106781186547,0.707106781186548,0.707106781186547,
0.707106781186548,0.707106781186547,0.707106781186548,0.707106781186547,
0.707106781186547,0.707106781186548,0.707106781186547,0.707106781186548,
0.707106781186548,0.707106781186548,0.707106781186547,0.707106781186547,
0.707106781186547,0.707106781186547,0.707106781186548,0.707106781186547,
0.707106781186548,0.707106781186548,0.707106781186547,0.707106781186547,
0.707106781186548,0.707106781186548,0.707106781186547,0.707106781186547,
0.707106781186548,0.707106781186547,0.707106781186548,0.707106781186547,
0.707106781186547,0.707106781186547,0.707106781186547,0.707106781186547,
0.707106781186547,0.707106781186547,0.707106781186548,0.707106781186547,
0.707106781186548,0.707106781186547,0.707106781186548,0.707106781186548,
0.707106781186547,0.707106781186548,0.707106781186548,0.707106781186548,
0.707106781186548,0.707106781186547,0.707106781186548,0.707106781186547,
0.707106781186548,0.707106781186547,0.707106781186547,0.707106781186548,
0.707106781186548,0.707106781186547,0.707106781186547,0.707106781186547,
0.707106781186547,0.707106781186547,0.707106781186548,0.707106781186548,
0.707106781186547,0.707106781186547,0.707106781186548,0.707106781186548,
0.707106781186547,0.707106781186548,0.707106781186547,0.707106781186548,
0.707106781186548,0.707106781186547,0.707106781186547,0.707106781186548,
0.707106781186547,0.707106781186547,0.707106781186548,0.707106781186547,
0.707106781186548,0.707106781186547,0.707106781186548,0.707106781186547,
0.707106781186547,0.707106781186548,0.707106781186548,0.707106781186547,
0.707106781186547,0.707106781186548,0.707106781186547,0.707106781186547,
0.707106781186548,0.707106781186547,0.707106781186548,0.707106781186547,
0.707106781186548,0.707106781186547,0.707106781186548,0.707106781186547,
0.707106781186547,0.707106781186547,0.707106781186547,0.707106781186547,
0.707106781186547,0.707106781186548,0.707106781186547,0.707106781186548,
0.707106781186547,0.707106781186548,0.707106781186548,0.707106781186547,
0.707106781186548,0.707106781186548,0.707106781186547,0.707106781186548,
0.707106781186547,0.707106781186547,0.707106781186547,0.707106781186548,
0.707106781186547,0.707106781186547,0.707106781186548,0.707106781186547,
0.707106781186548,0.707106781186547,0.707106781186547,0.707106781186547,
0.707106781186548,0.707106781186548,0.707106781186547,0.707106781186548,
0.707106781186548,0.707106781186547,0.707106781186548,0.707106781186547,
0.707106781186548,0.707106781186548,0.707106781186547,0.707106781186548,
0.707106781186548,0.707106781186548,0.707106781186547,0.707106781186547,
0.707106781186548,0.707106781186547,0.707106781186548,0.707106781186547,
0.707106781186547,0.707106781186548,0.707106781186548,0.707106781186548,
0.707106781186547,0.707106781186547,0.707106781186548,0.707106781186548,
0.707106781186547,0.707106781186547,0.707106781186548,0.707106781186547,
0.707106781186547,0.707106781186548,0.707106781186548,0.707106781186547,
0.707106781186547,0.707106781186547,0.707106781186548,0.707106781186547,
0.707106781186547,0.707106781186547,0.707106781186548,0.707106781186548,
0.707106781186547,0.707106781186548,0.707106781186547,0.707106781186548,
0.707106781186547,0.707106781186548,0.707106781186548,0.707106781186547,
0.707106781186547,0.707106781186548,0.707106781186547,0.707106781186547,
0.707106781186548,0.707106781186547,0.707106781186548,0.707106781186548,
0.707106781186547,0.707106781186548,0.707106781186547,0.707106781186547,
0.707106781186547,0.707106781186548,0.707106781186548,0.707106781186548,
0.707106781186547,0.707106781186548,0.707106781186547,0.707106781186548,
0.707106781186547,0.707106781186547,0.707106781186547,0.707106781186547,
0.707106781186548,0.707106781186548,0.707106781186547,0.707106781186547,
0.707106781186548,0.707106781186547,0.707106781186548,0.707106781186547,
0.707106781186548,0.707106781186547,0.707106781186547,0.707106781186548,
0.707106781186547,0.707106781186548,0.707106781186547,0.707106781186548,
0.707106781186548,0.707106781186547,0.707106781186548,0.707106781186547,
0.707106781186548,0.707106781186548,0.707106781186547,0.707106781186548,
0.707106781186547,0.707106781186547,0.707106781186548,0.707106781186547,
0.707106781186548,0.707106781186547,0.707106781186548,0.707106781186547,
0.707106781186547,0.707106781186548,0.707106781186548,0.707106781186548,
0.707106781186548,0.707106781186547,0.707106781186548,0.707106781186548,
0.707106781186548,0.707106781186547,0.707106781186548,0.707106781186548,
0.707106781186548,0.707106781186547,0.707106781186547,0.707106781186548,
0.707106781186547,0.707106781186548,0.707106781186547,0.707106781186548,
0.707106781186548,0.707106781186547,0.707106781186547,0.707106781186548,
0.707106781186547,0.707106781186548,0.707106781186547,0.707106781186548,
0.707106781186548,0.707106781186547,0.707106781186547,0.707106781186547,
0.707106781186548,0.707106781186548,0.707106781186547,0.707106781186547,
0.707106781186548,0.707106781186548,0.707106781186548,0.707106781186548,
0.707106781186547,0.707106781186547,0.707106781186548,0.707106781186548,
0.707106781186547,0.707106781186548,0.707106781186547,0.707106781186548,
0.707106781186547,0.707106781186548,0.707106781186547,0.707106781186547,
0.707106781186548,0.707106781186547,0.707106781186547,0.707106781186548,
0.707106781186547,0.707106781186548,0.707106781186547,0.707106781186548,
0.707106781186547,0.707106781186548,0.707106781186547,0.707106781186548,
0.707106781186547,0.707106781186548,0.707106781186547,0.707106781186547,
0.707106781186548,0.707106781186548,0.707106781186547,0.707106781186547,
0.707106781186547,0.707106781186548,0.707106781186547,0.707106781186548,
0.707106781186547,0.707106781186548,0.707106781186547,0.707106781186548,
0.707106781186547,0.707106781186547,0.707106781186547,0.707106781186548,
0.707106781186547,0.707106781186548,0.707106781186548,0.707106781186547,
0.707106781186548,0.707106781186547,0.707106781186547,0.707106781186548,
0.707106781186547,0.707106781186547,0.707106781186548,0.707106781186547,
0.707106781186547,0.707106781186547,0.707106781186547,0.707106781186548,
0.707106781186547,0.707106781186547,0.707106781186547,0.707106781186548,
0.707106781186547,0.707106781186547,0.707106781186548,0.707106781186548,
0.707106781186547,0.707106781186548,0.707106781186548,0.707106781186547,
0.707106781186547,0.707106781186548,0.707106781186547,0.707106781186547,
0.707106781186548,0.707106781186547,0.707106781186547,0.707106781186547,
0.707106781186548,0.707106781186547,0.707106781186548,0.707106781186547,
0.707106781186548,0.707106781186547,0.707106781186548,0.707106781186547,
0.707106781186548,0.707106781186547,0.707106781186548,0.707106781186548,
0.707106781186547,0.707106781186547,0.707106781186548,0.707106781186547,
0.707106781186548,0.707106781186547,0.707106781186548,0.707106781186548,
0.707106781186547,0.707106781186548,0.707106781186547,0.707106781186548,
0.707106781186548,0.707106781186547,0.707106781186547,0.707106781186548,
0.707106781186547,0.707106781186548,0.707106781186547,0.707106781186548,
0.707106781186547,0.707106781186548,0.707106781186547,0.707106781186547,
0.707106781186547,0.707106781186547,0.707106781186547,0.707106781186547,
0.707106781186547,0.707106781186547,0.707106781186548,0.707106781186547,
0.707106781186548,0.707106781186547,0.707106781186547,0.707106781186548,
0.707106781186547,0.707106781186548,0.707106781186547,0.707106781186547,
0.707106781186548,0.707106781186547,0.707106781186548,0.707106781186547,
0.707106781186548,0.707106781186547,0.707106781186548,0.707106781186547,
0.707106781186548,0.707106781186547,0.707106781186548,0.707106781186547,
0.707106781186548,0.707106781186548,0.707106781186547,0.707106781186548,
0.707106781186547,0.707106781186547,0.707106781186547,0.707106781186548,
0.707106781186547,0.707106781186547,0.707106781186547,0.707106781186548,
0.707106781186547,0.707106781186547,0.707106781186548,0.707106781186547,
0.707106781186547,0.707106781186547,0.707106781186547,0.707106781186548,
0.707106781186547,0.707106781186547,0.707106781186547,0.707106781186548,
0.707106781186548,0.707106781186548,0.707106781186548,0.707106781186547,
0.707106781186548,0.707106781186547,0.707106781186547,0.707106781186548,
0.707106781186547,0.707106781186548,0.707106781186547,0.707106781186547,
0.707106781186548,0.707106781186547,0.707106781186547,0.707106781186547,
0.707106781186547,0.707106781186548,0.707106781186548,0.707106781186547,
0.707106781186547,0.707106781186548,0.707106781186547,0.707106781186548,
0.707106781186547,0.707106781186548,0.707106781186548,0.707106781186547,
0.707106781186547,0.707106781186548,0.707106781186548,0.707106781186547,
0.707106781186548,0.707106781186548,0.707106781186547,0.707106781186548,
0.707106781186548,0.707106781186548,0.707106781186547,0.707106781186548,
0.707106781186547,0.707106781186548,0.707106781186547,0.707106781186548,
0.707106781186547,0.707106781186548,0.707106781186547,0.707106781186548,
0.707106781186548,0.707106781186547,0.707106781186547,0.707106781186548,
0.707106781186547,0.707106781186548,0.707106781186547,0.707106781186548,
0.707106781186548,0.707106781186548,0.707106781186548,0.707106781186548,
0.707106781186547,0.707106781186547,0.707106781186547,0.707106781186547,
0.707106781186548,0.707106781186547,0.707106781186548,0.707106781186547,
0.707106781186547,0.707106781186548,0.707106781186548,0.707106781186547,
0.707106781186548,0.707106781186547,0.707106781186548,0.707106781186548,
0.707106781186547,0.707106781186547,0.707106781186548,0.707106781186547,
0.707106781186548,0.707106781186547,0.707106781186548,0.707106781186547,
0.707106781186548,0.707106781186547,0.707106781186548,0.707106781186547,
0.707106781186548,0.707106781186547,0.707106781186548,0.707106781186548,
0.707106781186547,0.707106781186548,0.707106781186547,0.707106781186548,
0.707106781186547,0.707106781186548,0.707106781186548,0.707106781186548,
0.707106781186547,0.707106781186547,0.707106781186548,0.707106781186548,
0.707106781186547,0.707106781186547,0.707106781186547,0.707106781186548,
0.707106781186547,0.707106781186548,0.707106781186547,0.707106781186548,
0.707106781186547,0.707106781186547,0.707106781186547,0.707106781186548,
0.707106781186547,0.707106781186548,0.707106781186547,0.707106781186548,
0.707106781186547,0.707106781186548,0.707106781186547,0.707106781186547,
0.707106781186548,0.707106781186547,0.707106781186547,0.707106781186548,
0.707106781186547,0.707106781186547,0.707106781186548,0.707106781186547,
0.707106781186547,0.707106781186547,0.707106781186548,0.707106781186547,
0.707106781186548,0.707106781186547,0.707106781186547,0.707106781186547,
0.707106781186548,0.707106781186548,0.707106781186547,0.707106781186547,
0.707106781186548,0.707106781186548,0.707106781186548,0.707106781186547,
0.707106781186548,0.707106781186547,0.707106781186548,0.707106781186547,
0.707106781186548,0.707106781186547,0.707106781186547,0.707106781186547,
0.707106781186547,0.707106781186548,0.707106781186547,0.707106781186548,
0.707106781186548,0.707106781186547,0.707106781186548,0.707106781186547,
0.707106781186547,0.707106781186547,0.707106781186547,0.707106781186548,
0.707106781186547,0.707106781186548,0.707106781186547,0.707106781186548,
0.707106781186548,0.707106781186547,0.707106781186548,0.707106781186547,
0.707106781186547,0.707106781186547,0.707106781186547,0.707106781186548,
0.707106781186547,0.707106781186548,0.707106781186548,0.707106781186547,
0.707106781186548,0.707106781186547,0.707106781186548,0.707106781186547,
0.707106781186547,0.707106781186548,0.707106781186547,0.707106781186548,
0.707106781186548,0.707106781186547,0.707106781186547,0.707106781186548,
0.707106781186548,0.707106781186547,0.707106781186547,0.707106781186548,
0.707106781186547,0.707106781186547,0.707106781186548,0.707106781186547,
0.707106781186547,0.707106781186548,0.707106781186547,0.707106781186548,
0.707106781186547,0.707106781186547,0.707106781186548,0.707106781186547,
0.707106781186548,0.707106781186547,0.707106781186548,0.707106781186547,
0.707106781186547,0.707106781186547,0.707106781186548,0.707106781186547,
0.707106781186548,0.707106781186547,0.707106781186548,0.707106781186548,
0.707106781186548,0.707106781186548,0.707106781186547,0.707106781186547,
0.707106781186547,0.707106781186548,0.707106781186547,0.707106781186548,
0.707106781186547,0.707106781186547,0.707106781186548,0.707106781186547,
0.707106781186547,0.707106781186548,0.707106781186547,0.707106781186547,
0.707106781186548,0.707106781186548,0.707106781186547,0.707106781186548,
0.707106781186547,0.707106781186547,0.707106781186548,0.707106781186547,
0.707106781186548,0.707106781186547,0.707106781186548,0.707106781186547,
0.707106781186547,0.707106781186547,0.707106781186548,0.707106781186547,
0.707106781186548,0.707106781186547,0.707106781186548,0.707106781186547,
0.707106781186547,0.707106781186548,0.707106781186548,0.707106781186548,
0.707106781186547,0.707106781186548,0.707106781186547,0.707106781186548,
0.707106781186547,0.707106781186548,0.707106781186547,0.707106781186548,
0.707106781186548,0.707106781186547,0.707106781186547,0.707106781186547,
0.707106781186548,0.707106781186547,0.707106781186547,0.707106781186548,
0.707106781186547,0.707106781186547,0.707106781186548,0.707106781186547,
0.707106781186548,0.707106781186548,0.707106781186548,0.707106781186547,
0.707106781186548,0.707106781186547,0.707106781186548,0.707106781186547,
0.707106781186548,0.707106781186547,0.707106781186548,0.707106781186547,
0.707106781186548,0.707106781186547,0.707106781186548,0.707106781186548,
0.707106781186547,0.707106781186548,0.707106781186547,0.707106781186548,
0.707106781186548,0.707106781186547,0.707106781186547,0.707106781186548,
0.707106781186547,0.707106781186547,0.707106781186548,0.707106781186547,
0.707106781186548,0.707106781186548,0.707106781186547,0.707106781186548,
0.707106781186548,0.707106781186548,0.707106781186548,0.707106781186548,
0.707106781186547,0.707106781186548,0.707106781186548,0.707106781186548,
0.707106781186547,0.707106781186548,0.707106781186547,0.707106781186548,
0.707106781186547,0.707106781186548,0.707106781186547,0.707106781186548,
0.707106781186547,0.707106781186548,0.707106781186547,0.707106781186547,
0.707106781186548,0.707106781186547,0.707106781186547,0.707106781186548,
0.707106781186547,0.707106781186548,0.707106781186547,0.707106781186548,
0.707106781186547,0.707106781186548,0.707106781186547,0.707106781186547,
0.707106781186548,0.707106781186547,0.707106781186547,0.707106781186548,
0.707106781186547,0.707106781186548,0.707106781186547,0.707106781186547,
0.707106781186548,0.707106781186548,0.707106781186547,0.707106781186548,
0.707106781186547,0.707106781186547,0.707106781186547,0.707106781186548,
0.707106781186547,0.707106781186547,0.707106781186548,0.707106781186547,
0.707106781186547,0.707106781186547,0.707106781186548,0.707106781186548,
0.707106781186547,0.707106781186548,0.707106781186547,0.707106781186548,
0.707106781186547,0.707106781186547,0.707106781186548,0.707106781186547,
0.707106781186548,0.707106781186547,0.707106781186547,0.707106781186547,
0.707106781186547,0.707106781186548,0.707106781186547,0.707106781186547,
0.707106781186547,0.707106781186547,0.707106781186547,0.707106781186548,
0.707106781186547,0.707106781186547,0.707106781186547,0.707106781186547,
0.707106781186548,0.707106781186547,0.707106781186548,0.707106781186547,
0.707106781186547,0.707106781186548,0.707106781186547,0.707106781186548,
0.707106781186547,0.707106781186547,0.707106781186548,0.707106781186547,
0.707106781186547,0.707106781186548,0.707106781186547,0.707106781186547,
0.707106781186547,0.707106781186547,0.707106781186548,0.707106781186547,
0.707106781186548,0.707106781186548,0.707106781186547,0.707106781186548,
0.707106781186548,0.707106781186547,0.707106781186547,0.707106781186548,
0.707106781186547,0.707106781186547,0.707106781186547,0.707106781186548,
0.707106781186547,0.707106781186547,0.707106781186548,0.707106781186547,
0.707106781186548,0.707106781186547,0.707106781186548,0.707106781186547,
0.707106781186547,0.707106781186548,0.707106781186547,0.707106781186548,
0.707106781186547,0.707106781186548,0.707106781186547,0.707106781186548,
0.707106781186547,0.707106781186548,0.707106781186547,0.707106781186547,
0.707106781186547,0.707106781186547,0.707106781186548,0.707106781186548,
0.707106781186547,0.707106781186548,0.707106781186548,0.707106781186547,
0.707106781186548,0.707106781186547,0.707106781186547,0.707106781186548,
0.707106781186547,0.707106781186547,0.707106781186547,0.707106781186547,
0.707106781186548,0.707106781186547,0.707106781186547,0.707106781186547,
0.707106781186548,0.707106781186547,0.707106781186547,0.707106781186548,
0.707106781186547,0.707106781186548,0.707106781186548,0.707106781186547,
0.707106781186548,0.707106781186547,0.707106781186548,0.707106781186547,
0.707106781186548,0.707106781186547,0.707106781186547,0.707106781186548,
0.707106781186547,0.707106781186548,0.707106781186548,0.707106781186547,
0.707106781186547,0.707106781186548,0.707106781186547,0.707106781186548,
0.707106781186547,0.707106781186548,0.707106781186547,0.707106781186547,
0.707106781186548,0.707106781186548,0.707106781186547,0.707106781186548,
0.707106781186548,0.707106781186547,0.707106781186548,0.707106781186548,
0.707106781186547,0.707106781186548,0.707106781186547,0.707106781186548,
0.707106781186547,0.707106781186548,0.707106781186547,0.707106781186548,
0.707106781186547,0.707106781186547,0.707106781186548,0.707106781186547,
0.707106781186547,0.707106781186548,0.707106781186547,0.707106781186548,
0.707106781186548,0.707106781186547,0.707106781186547,0.707106781186547,
0.707106781186548,0.707106781186547,0.707106781186548,0.707106781186548,
0.707106781186547,0.707106781186548,0.707106781186547,0.707106781186548,
0.707106781186547,0.707106781186548,0.707106781186547,0.707106781186547,
0.707106781186548,0.707106781186548,0.707106781186548,0.707106781186547,
0.707106781186548,0.707106781186548,0.707106781186547,0.707106781186548,
0.707106781186547,0.707106781186548,0.707106781186548,0.707106781186548,
0.707106781186548,0.707106781186548,0.707106781186548,0.707106781186547,
0.707106781186547,0.707106781186548,0.707106781186547,0.707106781186547,
0.707106781186548,0.707106781186547,0.707106781186547,0.707106781186548,
0.707106781186547,0.707106781186548,0.707106781186547,0.707106781186548,
0.707106781186547,0.707106781186547,0.707106781186547,0.707106781186548,
0.707106781186547,0.707106781186547,0.707106781186548,0.707106781186547,
0.707106781186548,0.707106781186547,0.707106781186548,0.707106781186547,
0.707106781186547,0.707106781186547,0.707106781186547,0.707106781186548,
0.707106781186547,0.707106781186547,0.707106781186548,0.707106781186548,
0.707106781186547,0.707106781186548,0.707106781186547,0.707106781186548,
0.707106781186547,0.707106781186547,0.707106781186548,0.707106781186547,
0.707106781186548,0.707106781186547,0.707106781186548,0.707106781186547,
0.707106781186548,0.707106781186548,0.707106781186547,0.707106781186548,
0.707106781186547,0.707106781186547,0.707106781186548,0.707106781186547,
0.707106781186547,0.707106781186548,0.707106781186548,0.707106781186548,
0.707106781186547,0.707106781186548,0.707106781186547,0.707106781186547,
0.707106781186547,0.707106781186548,0.707106781186547,0.707106781186548,
0.707106781186548,0.707106781186548,0.707106781186547,0.707106781186547,
0.707106781186547,0.707106781186547,0.707106781186548,0.707106781186547,
0.707106781186547,0.707106781186548,0.707106781186547,0.707106781186548,
0.707106781186547,0.707106781186547,0.707106781186548,0.707106781186547,
0.707106781186548,0.707106781186547,0.707106781186548,0.707106781186547,
0.707106781186547,0.707106781186547,0.707106781186547,0.707106781186547,
0.707106781186547,0.707106781186548,0.707106781186547,0.707106781186547,
0.707106781186548,0.707106781186548,0.707106781186547,0.707106781186548,
0.707106781186548,0.707106781186547,0.707106781186547,0.707106781186548,
0.707106781186547,0.707106781186547,0.707106781186548,0.707106781186547,
0.707106781186548,0.707106781186548,0.707106781186548,0.707106781186547,
0.707106781186547,0.707106781186547,0.707106781186547,0.707106781186548,
0.707106781186548,0.707106781186548,0.707106781186547,0.707106781186548,
0.707106781186547,0.707106781186548,0.707106781186548,0.707106781186547,
0.707106781186548,0.707106781186547,0.707106781186548,0.707106781186548,
0.707106781186547,0.707106781186547,0.707106781186548,0.707106781186547,
0.707106781186548,0.707106781186547,0.707106781186548,0.707106781186548,
0.707106781186548,0.707106781186547,0.707106781186548,0.707106781186547,
0.707106781186547,0.707106781186547,0.707106781186547,0.707106781186548,
0.707106781186548,0.707106781186547,0.707106781186547,0.707106781186547,
0.707106781186548,0.707106781186547,0.707106781186547,0.707106781186548,
0.707106781186547,0.707106781186548,0.707106781186548,0.707106781186548,
0.707106781186547,0.707106781186547,0.707106781186547,0.707106781186547,
0.707106781186548,0.707106781186548,0.707106781186547,0.707106781186548,
0.707106781186547,0.707106781186548,0.707106781186548,0.707106781186547,
0.707106781186548,0.707106781186547,0.707106781186548,0.707106781186547,
0.707106781186547,0.707106781186547,0.707106781186548,0.707106781186547,
0.707106781186548,0.707106781186547,0.707106781186548,0.707106781186547,
0.707106781186548,0.707106781186547,0.707106781186548,0.707106781186547,
0.707106781186547,0.707106781186548,0.707106781186547,0.707106781186548,
0.707106781186547,0.707106781186547,0.707106781186548,0.707106781186548,
0.707106781186547,0.707106781186548,0.707106781186548,0.707106781186547,
0.707106781186548,0.707106781186547,0.707106781186548,0.707106781186547,
0.707106781186547,0.707106781186547,0.707106781186548,0.707106781186547,
0.707106781186547,0.707106781186548,0.707106781186547,0.707106781186548,
0.707106781186547,0.707106781186548,0.707106781186548,0.707106781186547,
0.707106781186548,0.707106781186547,0.707106781186548,0.707106781186548,
0.707106781186548,0.707106781186548,0.707106781186547,0.707106781186547,
0.707106781186548,0.707106781186547,0.707106781186547,0.707106781186548,
0.707106781186548,0.707106781186547,0.707106781186547,0.707106781186548,
0.707106781186547,0.707106781186547,0.707106781186548,0.707106781186547,
0.707106781186548,0.707106781186547,0.707106781186548,0.707106781186547,
0.707106781186547,0.707106781186547,0.707106781186548,0.707106781186547,
0.707106781186547,0.707106781186548,0.707106781186547,0.707106781186548,
0.707106781186548,0.707106781186548,0.707106781186547,0.707106781186547,
0.707106781186547,0.707106781186548,0.707106781186548,0.707106781186547,
0.707106781186547,0.707106781186547,0.707106781186547,0.707106781186548,
0.707106781186548,0.707106781186547,0.707106781186547,0.707106781186547,
0.707106781186548,0.707106781186548,0.707106781186547,0.707106781186548,
0.707106781186547,0.707106781186548,0.707106781186547,0.707106781186548,
0.707106781186548,0.707106781186547,0.707106781186548,0.707106781186548,
0.707106781186548,0.707106781186547,0.707106781186547,0.707106781186547,
0.707106781186548,0.707106781186548,0.707106781186548,0.707106781186547,
0.707106781186547,0.707106781186548,0.707106781186548,0.707106781186547,
0.707106781186548,0.707106781186547,0.707106781186547,0.707106781186548,
0.707106781186547,0.707106781186548,0.707106781186547,0.707106781186547,
0.707106781186548,0.707106781186547,0.707106781186548,0.707106781186548,
0.707106781186547,0.707106781186547,0.707106781186548,0.707106781186547,
0.707106781186548,0.707106781186547,0.707106781186547,0.707106781186548,
0.707106781186547,0.707106781186548,0.707106781186547,0.707106781186548,
0.707106781186547,0.707106781186547,0.707106781186548,0.707106781186547,
0.707106781186547,0.707106781186547,0.707106781186547,0.707106781186547,
0.707106781186547,0.707106781186548,0.707106781186547,0.707106781186548,
0.707106781186548,0.707106781186548,0.707106781186547,0.707106781186547,
0.707106781186547,0.707106781186548,0.707106781186547,0.707106781186548,
0.707106781186547,0.707106781186547,0.707106781186548,0.707106781186547,
0.707106781186547,0.707106781186547,0.707106781186547,0.707106781186547,
0.707106781186548,0.707106781186547,0.707106781186548,0.707106781186547,
0.707106781186547,0.707106781186548,0.707106781186548,0.707106781186547,
0.707106781186547,0.707106781186547,0.707106781186548,0.707106781186547,
0.707106781186547,0.707106781186548,0.707106781186548,0.707106781186547,
0.707106781186548,0.707106781186547,0.707106781186548,0.707106781186548,
0.707106781186547,0.707106781186547,0.707106781186547,0.707106781186548,
0.707106781186548,0.707106781186547,0.707106781186548,0.707106781186547,
0.707106781186548,0.707106781186548,0.707106781186547,0.707106781186548,
0.707106781186547,0.707106781186547,0.707106781186547,0.707106781186548,
0.707106781186547,0.707106781186548,0.707106781186547,0.707106781186548,
0.707106781186547,0.707106781186547,0.707106781186547,0.707106781186547,
0.707106781186547,0.707106781186548,0.707106781186547,0.707106781186548,
0.707106781186547,0.707106781186548,0.707106781186547,0.707106781186548,
0.707106781186547,0.707106781186547,0.707106781186547,0.707106781186547,
0.707106781186547,0.707106781186548,0.707106781186548,0.707106781186548,
0.707106781186547,0.707106781186548,0.707106781186547,0.707106781186548,
0.707106781186547,0.707106781186547,0.707106781186548,0.707106781186547,
0.707106781186548,0.707106781186547,0.707106781186547,0.707106781186547,
0.707106781186548,0.707106781186548,0.707106781186547,0.707106781186548,
0.707106781186547,0.707106781186548,0.707106781186548,0.707106781186547,
0.707106781186548,0.707106781186547,0.707106781186548,0.707106781186548,
0.707106781186547,0.707106781186547,0.707106781186547,0.707106781186547,
0.707106781186547,0.707106781186547,0.707106781186548,0.707106781186548,
0.707106781186547,0.707106781186548,0.707106781186547,0.707106781186547,
0.707106781186548,0.707106781186547,0.707106781186547,0.707106781186548,
0.707106781186547,0.707106781186547,0.707106781186547,0.707106781186548,
0.707106781186547,0.707106781186547,0.707106781186548,0.707106781186547,
0.707106781186548,0.707106781186548,0.707106781186547,0.707106781186547,
0.707106781186547,0.707106781186548,0.707106781186547,0.707106781186547,
0.707106781186548,0.707106781186548,0.707106781186548,0.707106781186548,
0.707106781186547,0.707106781186548,0.707106781186548,0.707106781186547,
0.707106781186547,0.707106781186548,0.707106781186547,0.707106781186548,
0.707106781186547,0.707106781186547,0.707106781186548,0.707106781186547,
0.707106781186547,0.707106781186548,0.707106781186547,0.707106781186548,
0.707106781186547,0.707106781186548,0.707106781186547,0.707106781186548,
0.707106781186547,0.707106781186548,0.707106781186547,0.707106781186548,
0.707106781186548,0.707106781186547,0.707106781186547,0.707106781186548,
0.707106781186548,0.707106781186547,0.707106781186547,0.707106781186547,
0.707106781186547,0.707106781186547,0.707106781186548,0.707106781186547,
0.707106781186547,0.707106781186548,0.707106781186547,0.707106781186548,
0.707106781186548,0.707106781186547,0.707106781186548,0.707106781186547,
0.707106781186548,0.707106781186547,0.707106781186548,0.707106781186547,
0.707106781186547,0.707106781186547,0.707106781186547,0.707106781186547,
0.707106781186547,0.707106781186548,0.707106781186547,0.707106781186548,
0.707106781186547,0.707106781186547,0.707106781186547,0.707106781186548,
0.707106781186547,0.707106781186548,0.707106781186548,0.707106781186547,
0.707106781186547,0.707106781186548,0.707106781186547,0.707106781186548,
0.707106781186547,0.707106781186548,0.707106781186547,0.707106781186548,
0.707106781186547,0.707106781186547,0.707106781186548,0.707106781186547,
0.707106781186548,0.707106781186547,0.707106781186548,0.707106781186548,
0.707106781186548,0.707106781186548,0.707106781186547,0.707106781186548,
0.707106781186548,0.707106781186548,0.707106781186547,0.707106781186548,
0.707106781186548,0.707106781186547,0.707106781186548,0.707106781186547,
0.707106781186548,0.707106781186547,0.707106781186547,0.707106781186547,
0.707106781186548,0.707106781186548,0.707106781186547,0.707106781186548,
0.707106781186547,0.707106781186548,0.707106781186547,0.707106781186548,
0.707106781186548,0.707106781186547,0.707106781186548,0.707106781186547,
0.707106781186547,0.707106781186548,0.707106781186547,0.707106781186547,
0.707106781186547,0.707106781186548,0.707106781186547,0.707106781186548,
0.707106781186548,0.707106781186547,0.707106781186548,0.707106781186547,
0.707106781186548,0.707106781186548,0.707106781186548,0.707106781186548,
0.707106781186547,0.707106781186548,0.707106781186547,0.707106781186548,
0.707106781186547,0.707106781186548,0.707106781186547,0.707106781186547,
0.707106781186547,0.707106781186547,0.707106781186548,0.707106781186547,
0.707106781186548,0.707106781186547,0.707106781186547,0.707106781186548,
0.707106781186547,0.707106781186548,0.707106781186547,0.707106781186548,
0.707106781186547,0.707106781186548,0.707106781186548,0.707106781186548,
0.707106781186548,0.707106781186547,0.707106781186548,0.707106781186548,
0.707106781186547,0.707106781186548,0.707106781186547,0.707106781186548,
0.707106781186547,0.707106781186548,0.707106781186547,0.707106781186547,
0.707106781186548,0.707106781186547,0.707106781186548,0.707106781186547,
0.707106781186547,0.707106781186548,0.707106781186547,0.707106781186548,
0.707106781186547,0.707106781186547,0.707106781186548,0.707106781186548,
0.707106781186548,0.707106781186548,0.707106781186548,0.707106781186548,
0.707106781186548,0.707106781186548,0.707106781186548,0.707106781186547,
0.707106781186548,0.707106781186547,0.707106781186547,0.707106781186548,
0.707106781186547,0.707106781186548,0.707106781186548,0.707106781186547,
0.707106781186547,0.707106781186548,0.707106781186548,0.707106781186547,
0.707106781186547,0.707106781186547,0.707106781186547,0.707106781186547,
0.707106781186548,0.707106781186547,0.707106781186548,0.707106781186548,
0.707106781186548,0.707106781186547,0.707106781186548,0.707106781186547,
0.707106781186548,0.707106781186547,0.707106781186548,0.707106781186547,
0.707106781186548,0.707106781186548,0.707106781186547,0.707106781186547,
0.707106781186548,0.707106781186548,0.707106781186548,0.707106781186547,
0.707106781186547,0.707106781186548,0.707106781186547,0.707106781186547,
0.707106781186548,0.707106781186547,0.707106781186548,0.707106781186547,
0.707106781186547,0.707106781186548,0.707106781186548,0.707106781186548,
0.707106781186547,0.707106781186547,0.707106781186548,0.707106781186547,
0.707106781186548,0.707106781186547,0.707106781186548,0.707106781186547,
0.707106781186548,0.707106781186548,0.707106781186547,0.707106781186548,
0.707106781186547,0.707106781186548,0.707106781186547,0.707106781186547,
0.707106781186547,0.707106781186548,0.707106781186547,0.707106781186548,
0.707106781186547,0.707106781186547,0.707106781186547,0.707106781186548,
0.707106781186547,0.707106781186547,0.707106781186548,0.707106781186548,
0.707106781186547,0.707106781186548,0.707106781186547,0.707106781186548,
0.707106781186548,0.707106781186547,0.707106781186548,0.707106781186547,
0.707106781186547,0.707106781186548,0.707106781186547,0.707106781186547,
0.707106781186547,0.707106781186548,0.707106781186547,0.707106781186548,
0.707106781186547,0.707106781186548,0.707106781186548,0.707106781186548,
0.707106781186547,0.707106781186548,0.707106781186548,0.707106781186548,
0.707106781186547,0.707106781186548,0.707106781186547,0.707106781186547,
0.707106781186548,0.707106781186547,0.707106781186547,0.707106781186548,
0.707106781186548,0.707106781186547,0.707106781186548,0.707106781186547,
0.707106781186548,0.707106781186548,0.707106781186547,0.707106781186548,
0.707106781186547,0.707106781186548,0.707106781186547,0.707106781186548,
0.707106781186547,0.707106781186548,0.707106781186548,0.707106781186548,
0.707106781186547,0.707106781186548,0.707106781186548,0.707106781186547,
0.707106781186547,0.707106781186548,0.707106781186547,0.707106781186548,
0.707106781186548,0.707106781186547,0.707106781186548,0.707106781186548,
0.707106781186547,0.707106781186548,0.707106781186548,0.707106781186547,
0.707106781186547,0.707106781186548,0.707106781186547,0.707106781186548,
0.707106781186547,0.707106781186548,0.707106781186547,0.707106781186548,
0.707106781186548,0.707106781186548,0.707106781186547,0.707106781186548,
0.707106781186547,0.707106781186548,0.707106781186547,0.707106781186548,
0.707106781186547,0.707106781186548,0.707106781186547,0.707106781186548,
0.707106781186547,0.707106781186548,0.707106781186547,0.707106781186547,
0.707106781186547,0.707106781186548,0.707106781186547,0.707106781186548,
0.707106781186547,0.707106781186548,0.707106781186547,0.707106781186548,
0.707106781186547,0.707106781186548,0.707106781186548,0.707106781186548,
0.707106781186547,0.707106781186548,0.707106781186547,0.707106781186548,
0.707106781186548,0.707106781186547,0.707106781186548,0.707106781186547,
0.707106781186548,0.707106781186547,0.707106781186548,0.707106781186547,
0.707106781186548,0.707106781186547,0.707106781186547,0.707106781186547,
0.707106781186548,0.707106781186547,0.707106781186547,0.707106781186548,
0.707106781186547,0.707106781186548,0.707106781186547,0.707106781186547,
0.707106781186548,0.707106781186547,0.707106781186548,0.707106781186547,
0.707106781186548,0.707106781186548,0.707106781186548,0.707106781186547,
0.707106781186547,0.707106781186548,0.707106781186548,0.707106781186547,
0.707106781186548,0.707106781186547,0.707106781186547,0.707106781186547,
0.707106781186548,0.707106781186547,0.707106781186548,0.707106781186547,
0.707106781186548,0.707106781186548,0.707106781186548,0.707106781186547,
0.707106781186547,0.707106781186547,0.707106781186547,0.707106781186547,
0.707106781186547,0.707106781186548,0.707106781186547,0.707106781186548,
0.707106781186547,0.707106781186548,0.707106781186547,0.707106781186547,
0.707106781186548,0.707106781186547,0.707106781186547,0.707106781186548,
0.707106781186548,0.707106781186547,0.707106781186547,0.707106781186547,
0.707106781186548,0.707106781186547,0.707106781186547,0.707106781186548,
0.707106781186548),(1.,1.,1.,1.,1.,1.,1.,1.,1.,1.,1.,1.,1.,1.,1.,1.,1.,
1.,1.,1.,1.,1.,1.,1.,1.,1.,1.,1.,1.,1.,1.,1.,1.,1.,1.,1.,1.,1.,1.,1.,1.,
1.,1.,1.,1.,1.,1.,1.,1.,1.,1.,1.,1.,1.,1.,1.,1.,1.,1.,1.,1.,1.,1.,1.,1.,
1.,1.,1.,1.,1.,1.,1.,1.,1.,1.,1.,1.,1.,1.,1.,1.,1.,1.,1.,1.,1.,1.,1.,1.,
1.,1.,1.,1.,1.,1.,1.,1.,1.,1.,1.,1.,1.,1.,1.,1.,1.,1.,1.,1.,1.,1.,1.,1.,
1.,1.,1.,1.,1.,1.,1.,1.,1.,1.,1.,1.,1.,1.,1.,1.,1.,1.,1.,1.,1.,1.,1.,1.,
1.,1.,1.,1.,1.,1.,1.,1.,1.,1.,1.,1.,1.,1.,1.,1.,1.,1.,1.,1.,1.,1.,1.,1.,
1.,1.,1.,1.,1.,1.,1.,1.,1.,1.,1.,1.,1.,1.,1.,1.,1.,1.,1.,1.,1.,1.,1.,1.,
1.,1.,1.,1.,1.,1.,1.,1.,1.,1.,1.,1.,1.,1.,1.,1.,1.,1.,1.,1.,1.,1.,1.,1.,
1.,1.,1.,1.,1.,1.,1.,1.,1.,1.,1.,1.,1.,1.,1.,1.,1.,1.,1.,1.,1.,1.,1.,1.,
1.,1.,1.,1.,1.,1.,1.,1.,1.,1.,1.,1.,1.,1.,1.,1.,1.,1.,1.,1.,1.,1.,1.,1.,
1.,1.,1.,1.,1.,1.,1.,1.,1.,1.,1.,1.,1.,1.,1.,1.,1.,1.,1.,1.,1.,1.,1.,1.,
1.,1.,1.,1.,1.,1.,1.,1.,1.,1.,1.,1.,1.,1.,1.,1.,1.,1.,1.,1.,1.,1.,1.,1.,
1.,1.,1.,1.,1.,1.,1.,1.,1.,1.,1.,1.,1.,1.,1.,1.,1.,1.,1.,1.,1.,1.,1.,1.,
1.,1.,1.,1.,1.,1.,1.,1.,1.,1.,1.,1.,1.,1.,1.,1.,1.,1.,1.,1.,1.,1.,1.,1.,
1.,1.,1.,1.,1.,1.,1.,1.,1.,1.,1.,1.,1.,1.,1.,1.,1.,1.,1.,1.,1.,1.,1.,1.,
1.,1.,1.,1.,1.,1.,1.,1.,1.,1.,1.,1.,1.,1.,1.,1.,1.,1.,1.,1.,1.,1.,1.,1.,
1.,1.,1.,1.,1.,1.,1.,1.,1.,1.,1.,1.,1.,1.,1.,1.,1.,1.,1.,1.,1.,1.,1.,1.,
1.,1.,1.,1.,1.,1.,1.,1.,1.,1.,1.,1.,1.,1.,1.,1.,1.,1.,1.,1.,1.,1.,1.,1.,
1.,1.,1.,1.,1.,1.,1.,1.,1.,1.,1.,1.,1.,1.,1.,1.,1.,1.,1.,1.,1.,1.,1.,1.,
1.,1.,1.,1.,1.,1.,1.,1.,1.,1.,1.,1.,1.,1.,1.,1.,1.,1.,1.,1.,1.,1.,1.,1.,
1.,1.,1.,1.,1.,1.,1.,1.,1.,1.,1.,1.,1.,1.,1.,1.,1.,1.,1.,1.,1.,1.,1.,1.,
1.,1.,1.,1.,1.,1.,1.,1.,1.,1.,1.,1.,1.,1.,1.,1.,1.,1.,1.,1.,1.,1.,1.,1.,
1.,1.,1.,1.,1.,1.,1.,1.,1.,1.,1.,1.,1.,1.,1.,1.,1.,1.,1.,1.,1.,1.,1.,1.,
1.,1.,1.,1.,1.,1.,1.,1.,1.,1.,1.,1.,1.,1.,1.,1.,1.,1.,1.,1.,1.,1.,1.,1.,
1.,1.,1.,1.,1.,1.,1.,1.,1.,1.,1.,1.,1.,1.,1.,1.,1.,1.,1.,1.,1.,1.,1.,1.,
1.,1.,1.,1.,1.,1.,1.,1.,1.,1.,1.,1.,1.,1.,1.,1.,1.,1.,1.,1.,1.,1.,1.,1.,
1.,1.,1.,1.,1.,1.,1.,1.,1.,1.,1.,1.,1.,1.,1.,1.,1.,1.,1.,1.,1.,1.,1.,1.,
1.,1.,1.,1.,1.,1.,1.,1.,1.,1.,1.,1.,1.,1.,1.,1.,1.,1.,1.,1.,1.,1.,1.,1.,
1.,1.,1.,1.,1.,1.,1.,1.,1.,1.,1.,1.,1.,1.,1.,1.,1.,1.,1.,1.,1.,1.,1.,1.,
1.,1.,1.,1.,1.,1.,1.,1.,1.,1.,1.,1.,1.,1.,1.,1.,1.,1.,1.,1.,1.,1.,1.,1.,
1.,1.,1.,1.,1.,1.,1.,1.,1.,1.,1.,1.,1.,1.,1.,1.,1.,1.,1.,1.,1.,1.,1.,1.,
1.,1.,1.,1.,1.,1.,1.,1.,1.,1.,1.,1.,1.,1.,1.,1.,1.,1.,1.,1.,1.,1.,1.,1.,
1.,1.,1.,1.,1.,1.,1.,1.,1.,1.,1.,1.,1.,1.,1.,1.,1.,1.,1.,1.,1.,1.,1.,1.,
1.,1.,1.,1.,1.,1.,1.,1.,1.,1.,1.,1.,1.,1.,1.,1.,1.,1.,1.,1.,1.,1.,1.,1.,
1.,1.,1.,1.,1.,1.,1.,1.,1.,1.,1.,1.,1.,1.,1.,1.,1.,1.,1.,1.,1.,1.,1.,1.,
1.,1.,1.,1.,1.,1.,1.,1.,1.,1.,1.,1.,1.,1.,1.,1.,1.,1.,1.,1.,1.,1.,1.,1.,
1.,1.,1.,1.,1.,1.,1.,1.,1.,1.,1.,1.,1.,1.,1.,1.,1.,1.,1.,1.,1.,1.,1.,1.,
1.,1.,1.,1.,1.,1.,1.,1.,1.,1.,1.,1.,1.,1.,1.,1.,1.,1.,1.,1.,1.,1.,1.,1.,
1.,1.,1.,1.,1.,1.,1.,1.,1.,1.,1.,1.,1.,1.,1.,1.,1.,1.,1.,1.,1.,1.,1.,1.,
1.,1.,1.,1.,1.,1.,1.,1.,1.,1.,1.,1.,1.,1.,1.,1.,1.,1.,1.,1.,1.,1.,1.,1.,
1.,1.,1.,1.,1.,1.,1.,1.,1.,1.,1.,1.,1.,1.,1.,1.,1.,1.,1.,1.,1.,1.,1.,1.,
1.,1.,1.,1.,1.,1.,1.,1.,1.,1.,1.,1.,1.,1.,1.,1.,1.,1.,1.,1.,1.,1.,1.,1.,
1.,1.,1.,1.,1.,1.,1.,1.,1.,1.,1.,1.,1.,1.,1.,1.,1.,1.,1.,1.,1.,1.,1.,1.,
1.,1.,1.,1.,1.,1.,1.,1.,1.,1.,1.,1.,1.,1.,1.,1.,1.,1.,1.,1.,1.,1.,1.,1.,
1.,1.,1.,1.,1.,1.,1.,1.,1.,1.,1.,1.,1.,1.,1.,1.,1.,1.,1.,1.,1.,1.,1.,1.,
1.,1.,1.,1.,1.,1.,1.,1.,1.,1.,1.,1.,1.,1.,1.,1.,1.,1.,1.,1.,1.,1.,1.,1.,
1.,1.,1.,1.,1.,1.,1.,1.,1.,1.,1.,1.,1.,1.,1.,1.,1.,1.,1.,1.,1.,1.,1.,1.,
1.,1.,1.,1.,1.,1.,1.,1.,1.,1.,1.,1.,1.,1.,1.,1.,1.,1.,1.,1.,1.,1.,1.,1.,
1.,1.,1.,1.,1.,1.,1.,1.,1.,1.,1.,1.,1.,1.,1.,1.,1.,1.,1.,1.,1.,1.,1.,1.,
1.,1.,1.,1.,1.,1.,1.,1.,1.,1.,1.,1.,1.,1.,1.,1.,1.,1.,1.,1.,1.,1.,1.,1.,
1.,1.,1.,1.,1.,1.,1.,1.,1.,1.,1.,1.,1.,1.,1.,1.,1.,1.,1.,1.,1.,1.,1.,1.,
1.,1.,1.,1.,1.,1.,1.,1.,1.,1.,1.,1.,1.,1.,1.,1.,1.,1.,1.,1.,1.,1.,1.,1.,
1.,1.,1.,1.,1.,1.,1.,1.,1.,1.,1.,1.,1.,1.,1.,1.,1.,1.,1.,1.,1.,1.,1.,1.,
1.,1.,1.,1.,1.,1.,1.,1.,1.,1.,1.,1.,1.,1.,1.,1.,1.,1.,1.,1.,1.,1.,1.,1.,
1.,1.,1.,1.,1.,1.,1.,1.,1.,1.,1.,1.,1.,1.,1.,1.,1.,1.,1.,1.,1.,1.,1.,1.,
1.,1.,1.,1.,1.,1.,1.,1.,1.,1.,1.,1.,1.,1.,1.,1.,1.,1.,1.,1.,1.,1.,1.,1.,
1.,1.,1.,1.,1.,1.,1.,1.,1.,1.,1.,1.,1.,1.,1.,1.,1.,1.,1.,1.,1.,1.,1.,1.,
1.,1.,1.,1.,1.,1.,1.,1.,1.,1.,1.,1.,1.,1.,1.,1.,1.,1.,1.,1.,1.,1.,1.,1.,
1.,1.,1.,1.,1.,1.,1.,1.,1.,1.,1.,1.,1.,1.,1.,1.,1.,1.,1.,1.,1.,1.,1.,1.,
1.,1.,1.,1.,1.,1.,1.,1.,1.,1.,1.,1.,1.,1.,1.,1.,1.,1.,1.,1.,1.,1.,1.,1.,
1.,1.,1.,1.,1.,1.,1.,1.,1.,1.,1.,1.,1.,1.,1.,1.,1.,1.,1.,1.,1.,1.,1.,1.,
1.,1.,1.,1.,1.,1.,1.,1.,1.,1.,1.,1.,1.,1.,1.,1.,1.,1.,1.,1.,1.,1.,1.,1.,
1.,1.,1.,1.,1.,1.,1.,1.,1.,1.,1.,1.,1.,1.,1.,1.,1.,1.,1.,1.,1.,1.,1.,1.,
1.,1.,1.,1.,1.,1.,1.,1.,1.,1.,1.,1.,1.,1.,1.,1.,1.,1.,1.,1.,1.,1.,1.,1.,
1.,1.,1.,1.,1.,1.,1.,1.,1.,1.,1.,1.,1.,1.,1.,1.,1.,1.,1.,1.,1.,1.,1.,1.,
1.,1.,1.,1.,1.,1.,1.,1.,1.,1.,1.,1.,1.,1.,1.,1.,1.,1.,1.,1.,1.,1.,1.,1.,
1.,1.,1.,1.,1.,1.,1.,1.,1.,1.,1.,1.,1.,1.,1.,1.,1.,1.,1.,1.,1.,1.,1.,1.,
1.,1.,1.,1.,1.,1.,1.,1.,1.,1.,1.,1.,1.,1.,1.,1.,1.,1.,1.,1.,1.,1.,1.,1.,
1.,1.,1.,1.,1.,1.,1.,1.,1.,1.,1.,1.,1.,1.,1.,1.,1.,1.,1.,1.,1.,1.,1.,1.,
1.,1.,1.,1.,1.,1.,1.,1.,1.,1.,1.,1.,1.,1.,1.,1.,1.,1.,1.,1.,1.,1.,1.,1.,
1.,1.,1.,1.,1.,1.,1.,1.,1.,1.,1.,1.,1.,1.,1.,1.,1.,1.,1.,1.,1.,1.,1.,1.,
1.,1.,1.,1.,1.,1.,1.,1.,1.,1.,1.,1.,1.,1.,1.,1.,1.,1.,1.,1.,1.,1.,1.,1.,
1.,1.,1.,1.,1.,1.,1.,1.,1.,1.,1.,1.,1.,1.,1.,1.,1.,1.,1.,1.,1.,1.,1.,1.,
1.,1.,1.,1.,1.,1.,1.,1.,1.,1.,1.,1.,1.,1.,1.,1.,1.,1.,1.,1.,1.,1.,1.,1.,
1.,1.,1.,1.,1.,1.,1.,1.,1.,1.,1.,1.,1.,1.,1.,1.,1.,1.,1.,1.,1.,1.,1.,1.,
1.,1.,1.,1.,1.,1.,1.,1.,1.,1.,1.,1.,1.,1.,1.,1.,1.,1.,1.,1.,1.,1.,1.,1.,
1.,1.,1.,1.,1.,1.,1.,1.,1.,1.,1.,1.,1.,1.,1.,1.,1.,1.,1.,1.,1.,1.,1.,1.,
1.,1.,1.,1.,1.,1.,1.,1.,1.,1.,1.,1.,1.,1.,1.,1.,1.,1.,1.,1.,1.,1.,1.,1.,
1.,1.,1.,1.,1.,1.,1.,1.,1.,1.,1.,1.,1.,1.,1.,1.,1.,1.,1.,1.,1.,1.,1.,1.,
1.,1.,1.,1.,1.,1.,1.,1.,1.,1.,1.,1.,1.,1.,1.,1.,1.,1.,1.,1.,1.,1.,1.,1.,
1.,1.,1.,1.,1.,1.,1.,1.,1.,1.,1.,1.,1.,1.,1.,1.,1.,1.,1.,1.,1.,1.,1.,1.,
1.,1.,1.,1.,1.,1.,1.,1.,1.,1.,1.,1.,1.,1.,1.,1.,1.,1.,1.,1.,1.,1.,1.,1.,
1.,1.,1.,1.,1.,1.,1.,1.,1.,1.,1.,1.,1.,1.,1.,1.,1.,1.,1.,1.,1.,1.,1.,1.,
1.,1.,1.,1.,1.,1.,1.,1.,1.,1.,1.,1.,1.,1.,1.,1.,1.,1.,1.,1.,1.,1.,1.,1.,
1.,1.,1.,1.,1.,1.,1.,1.,1.,1.,1.,1.,1.,1.,1.,1.,1.,1.)))
REPRESENTATION_ITEM('')
SURFACE()
) ;
#44=(
BOUNDED_SURFACE()
B_SPLINE_SURFACE(3,2,((#134061,#134062,#134063,#134064,#134065,#134066,
#134067,#134068,#134069),(#134070,#134071,#134072,#134073,#134074,#134075,
#134076,#134077,#134078),(#134079,#134080,#134081,#134082,#134083,#134084,
#134085,#134086,#134087),(#134088,#134089,#134090,#134091,#134092,#134093,
#134094,#134095,#134096),(#134097,#134098,#134099,#134100,#134101,#134102,
#134103,#134104,#134105),(#134106,#134107,#134108,#134109,#134110,#134111,
#134112,#134113,#134114),(#134115,#134116,#134117,#134118,#134119,#134120,
#134121,#134122,#134123)),.UNSPECIFIED.,.F.,.T.,.F.)
B_SPLINE_SURFACE_WITH_KNOTS((4,1,1,1,4),(3,2,2,2,3),(0.,0.0911446219616379,
0.182289243923276,0.273433865884915,0.364578487846551),(0.,0.117809724509617,
0.235619449019234,0.353429173528852,0.471238898038469),.UNSPECIFIED.)
GEOMETRIC_REPRESENTATION_ITEM()
RATIONAL_B_SPLINE_SURFACE(((1.,0.707106781186548,1.,0.707106781186548,1.,
0.707106781186548,1.,0.707106781186548,1.),(1.,0.707106781186548,1.,0.707106781186548,
1.,0.707106781186548,1.,0.707106781186548,1.),(1.,0.707106781186547,1.,
0.707106781186547,1.,0.707106781186547,1.,0.707106781186547,1.),(1.,0.707106781186548,
1.,0.707106781186548,1.,0.707106781186548,1.,0.707106781186548,1.),(1.,
0.707106781186547,1.,0.707106781186547,1.,0.707106781186547,1.,0.707106781186547,
1.),(1.,0.707106781186548,1.,0.707106781186548,1.,0.707106781186548,1.,
0.707106781186548,1.),(1.,0.707106781186548,1.,0.707106781186548,1.,0.707106781186548,
1.,0.707106781186548,1.)))
REPRESENTATION_ITEM('')
SURFACE()
) ;
#45=(
BOUNDED_SURFACE()
B_SPLINE_SURFACE(3,2,((#134133,#134134,#134135,#134136,#134137,#134138,
#134139,#134140,#134141),(#134142,#134143,#134144,#134145,#134146,#134147,
#134148,#134149,#134150),(#134151,#134152,#134153,#134154,#134155,#134156,
#134157,#134158,#134159),(#134160,#134161,#134162,#134163,#134164,#134165,
#134166,#134167,#134168)),.UNSPECIFIED.,.F.,.T.,.F.)
B_SPLINE_SURFACE_WITH_KNOTS((4,4),(3,2,2,2,3),(0.,1.1454147408364),(0.,
0.117809724509617,0.235619449019234,0.353429173528852,0.471238898038469),
 .UNSPECIFIED.)
GEOMETRIC_REPRESENTATION_ITEM()
RATIONAL_B_SPLINE_SURFACE(((1.,0.707106781186548,1.,0.707106781186548,1.,
0.707106781186548,1.,0.707106781186548,1.),(1.,0.707106781186548,1.,0.707106781186548,
1.,0.707106781186548,1.,0.707106781186548,1.),(1.,0.707106781186547,1.,
0.707106781186547,1.,0.707106781186547,1.,0.707106781186547,1.),(1.,0.707106781186548,
1.,0.707106781186548,1.,0.707106781186548,1.,0.707106781186548,1.)))
REPRESENTATION_ITEM('')
SURFACE()
) ;
#46=(
BOUNDED_SURFACE()
B_SPLINE_SURFACE(3,2,((#134176,#134177,#134178,#134179,#134180,#134181,
#134182,#134183,#134184),(#134185,#134186,#134187,#134188,#134189,#134190,
#134191,#134192,#134193),(#134194,#134195,#134196,#134197,#134198,#134199,
#134200,#134201,#134202),(#134203,#134204,#134205,#134206,#134207,#134208,
#134209,#134210,#134211),(#134212,#134213,#134214,#134215,#134216,#134217,
#134218,#134219,#134220),(#134221,#134222,#134223,#134224,#134225,#134226,
#134227,#134228,#134229),(#134230,#134231,#134232,#134233,#134234,#134235,
#134236,#134237,#134238),(#134239,#134240,#134241,#134242,#134243,#134244,
#134245,#134246,#134247),(#134248,#134249,#134250,#134251,#134252,#134253,
#134254,#134255,#134256),(#134257,#134258,#134259,#134260,#134261,#134262,
#134263,#134264,#134265),(#134266,#134267,#134268,#134269,#134270,#134271,
#134272,#134273,#134274),(#134275,#134276,#134277,#134278,#134279,#134280,
#134281,#134282,#134283),(#134284,#134285,#134286,#134287,#134288,#134289,
#134290,#134291,#134292),(#134293,#134294,#134295,#134296,#134297,#134298,
#134299,#134300,#134301),(#134302,#134303,#134304,#134305,#134306,#134307,
#134308,#134309,#134310),(#134311,#134312,#134313,#134314,#134315,#134316,
#134317,#134318,#134319),(#134320,#134321,#134322,#134323,#134324,#134325,
#134326,#134327,#134328),(#134329,#134330,#134331,#134332,#134333,#134334,
#134335,#134336,#134337),(#134338,#134339,#134340,#134341,#134342,#134343,
#134344,#134345,#134346)),.UNSPECIFIED.,.F.,.T.,.F.)
B_SPLINE_SURFACE_WITH_KNOTS((4,1,1,1,1,1,1,1,1,1,1,1,1,1,1,1,4),(3,2,2,
2,3),(0.,0.226732296973331,0.464902013928651,0.70307173088397,0.9298040278573,
1.15653632483063,1.39470604178595,1.63287575874127,1.8596080557146,2.08634035268793,
2.32451006964325,2.56267978659857,2.7894120835719,3.01614438054523,3.25431409750055,
3.49248381445586,3.7192161114292),(0.,0.117809724509617,0.235619449019234,
0.353429173528852,0.471238898038469),.UNSPECIFIED.)
GEOMETRIC_REPRESENTATION_ITEM()
RATIONAL_B_SPLINE_SURFACE(((1.,0.707106781186548,1.,0.707106781186548,1.,
0.707106781186548,1.,0.707106781186548,1.),(1.,0.707106781186547,1.,0.707106781186547,
1.,0.707106781186547,1.,0.707106781186547,1.),(1.,0.707106781186548,1.,
0.707106781186548,1.,0.707106781186548,1.,0.707106781186548,1.),(1.,0.707106781186547,
1.,0.707106781186547,1.,0.707106781186547,1.,0.707106781186547,1.),(1.,
0.707106781186548,1.,0.707106781186548,1.,0.707106781186548,1.,0.707106781186548,
1.),(1.,0.707106781186547,1.,0.707106781186547,1.,0.707106781186547,1.,
0.707106781186547,1.),(1.,0.707106781186548,1.,0.707106781186548,1.,0.707106781186548,
1.,0.707106781186548,1.),(1.,0.707106781186547,1.,0.707106781186547,1.,
0.707106781186547,1.,0.707106781186547,1.),(1.,0.707106781186547,1.,0.707106781186547,
1.,0.707106781186547,1.,0.707106781186547,1.),(1.,0.707106781186547,1.,
0.707106781186547,1.,0.707106781186547,1.,0.707106781186547,1.),(1.,0.707106781186548,
1.,0.707106781186548,1.,0.707106781186548,1.,0.707106781186548,1.),(1.,
0.707106781186547,1.,0.707106781186547,1.,0.707106781186547,1.,0.707106781186547,
1.),(1.,0.707106781186547,1.,0.707106781186547,1.,0.707106781186547,1.,
0.707106781186547,1.),(1.,0.707106781186547,1.,0.707106781186547,1.,0.707106781186547,
1.,0.707106781186547,1.),(1.,0.707106781186547,1.,0.707106781186547,1.,
0.707106781186547,1.,0.707106781186547,1.),(1.,0.707106781186547,1.,0.707106781186547,
1.,0.707106781186547,1.,0.707106781186547,1.),(1.,0.707106781186548,1.,
0.707106781186548,1.,0.707106781186548,1.,0.707106781186548,1.),(1.,0.707106781186547,
1.,0.707106781186547,1.,0.707106781186547,1.,0.707106781186547,1.),(1.,
0.707106781186548,1.,0.707106781186548,1.,0.707106781186548,1.,0.707106781186548,
1.)))
REPRESENTATION_ITEM('')
SURFACE()
) ;
#47=(
BOUNDED_SURFACE()
B_SPLINE_SURFACE(2,3,((#134369,#134370,#134371,#134372,#134373,#134374,
#134375,#134376,#134377,#134378,#134379,#134380,#134381,#134382,#134383,
#134384,#134385,#134386,#134387,#134388,#134389,#134390,#134391,#134392,
#134393,#134394,#134395,#134396,#134397,#134398,#134399,#134400,#134401,
#134402,#134403,#134404,#134405,#134406,#134407,#134408,#134409,#134410,
#134411,#134412,#134413,#134414,#134415,#134416,#134417,#134418,#134419,
#134420,#134421,#134422,#134423,#134424,#134425,#134426,#134427,#134428,
#134429,#134430,#134431,#134432,#134433,#134434,#134435,#134436,#134437,
#134438,#134439,#134440,#134441,#134442,#134443,#134444,#134445,#134446,
#134447,#134448,#134449,#134450,#134451,#134452,#134453,#134454,#134455,
#134456,#134457,#134458,#134459,#134460,#134461,#134462,#134463,#134464,
#134465,#134466,#134467,#134468,#134469,#134470,#134471,#134472,#134473,
#134474,#134475,#134476,#134477,#134478,#134479,#134480,#134481,#134482,
#134483,#134484,#134485,#134486,#134487,#134488,#134489,#134490,#134491,
#134492,#134493,#134494,#134495,#134496,#134497,#134498,#134499,#134500,
#134501,#134502,#134503,#134504,#134505,#134506,#134507,#134508,#134509,
#134510,#134511,#134512,#134513,#134514,#134515,#134516,#134517,#134518,
#134519,#134520,#134521,#134522,#134523,#134524,#134525,#134526,#134527,
#134528,#134529,#134530,#134531,#134532,#134533,#134534,#134535,#134536,
#134537,#134538,#134539,#134540,#134541,#134542,#134543,#134544,#134545,
#134546,#134547,#134548,#134549,#134550,#134551,#134552,#134553,#134554,
#134555,#134556,#134557,#134558,#134559,#134560,#134561,#134562,#134563,
#134564,#134565,#134566,#134567,#134568,#134569,#134570,#134571,#134572,
#134573,#134574,#134575,#134576,#134577,#134578,#134579,#134580,#134581,
#134582,#134583,#134584,#134585,#134586,#134587,#134588,#134589,#134590,
#134591,#134592,#134593,#134594,#134595,#134596,#134597,#134598,#134599,
#134600,#134601,#134602,#134603,#134604,#134605,#134606,#134607,#134608,
#134609,#134610,#134611,#134612,#134613,#134614,#134615,#134616,#134617,
#134618,#134619,#134620,#134621,#134622,#134623,#134624,#134625,#134626,
#134627,#134628,#134629,#134630,#134631,#134632,#134633,#134634,#134635,
#134636,#134637,#134638,#134639,#134640,#134641,#134642,#134643,#134644,
#134645,#134646,#134647,#134648,#134649,#134650,#134651,#134652,#134653,
#134654,#134655,#134656,#134657,#134658,#134659,#134660,#134661,#134662,
#134663,#134664,#134665,#134666,#134667,#134668,#134669,#134670,#134671,
#134672,#134673,#134674,#134675,#134676,#134677,#134678,#134679,#134680,
#134681,#134682,#134683,#134684,#134685,#134686,#134687,#134688,#134689,
#134690,#134691,#134692,#134693,#134694,#134695,#134696,#134697,#134698,
#134699,#134700,#134701,#134702,#134703,#134704,#134705,#134706,#134707,
#134708,#134709,#134710,#134711,#134712,#134713,#134714,#134715,#134716,
#134717,#134718,#134719,#134720,#134721,#134722,#134723,#134724,#134725,
#134726,#134727,#134728,#134729,#134730,#134731,#134732,#134733,#134734,
#134735,#134736,#134737,#134738,#134739,#134740,#134741,#134742,#134743,
#134744,#134745,#134746,#134747,#134748,#134749,#134750,#134751,#134752,
#134753,#134754,#134755,#134756,#134757,#134758,#134759,#134760,#134761,
#134762,#134763,#134764,#134765,#134766,#134767,#134768,#134769,#134770,
#134771,#134772,#134773,#134774,#134775,#134776,#134777,#134778,#134779,
#134780,#134781,#134782,#134783,#134784,#134785,#134786,#134787,#134788,
#134789,#134790,#134791,#134792,#134793,#134794,#134795,#134796,#134797,
#134798,#134799,#134800,#134801,#134802,#134803,#134804,#134805,#134806,
#134807,#134808,#134809,#134810,#134811,#134812,#134813,#134814,#134815,
#134816,#134817,#134818,#134819,#134820,#134821,#134822,#134823,#134824,
#134825,#134826,#134827,#134828,#134829,#134830,#134831,#134832,#134833,
#134834,#134835,#134836,#134837,#134838,#134839,#134840,#134841,#134842,
#134843,#134844,#134845,#134846,#134847,#134848,#134849,#134850,#134851,
#134852,#134853,#134854,#134855,#134856,#134857,#134858,#134859,#134860,
#134861,#134862,#134863,#134864,#134865,#134866,#134867,#134868,#134869,
#134870,#134871,#134872,#134873,#134874,#134875,#134876,#134877,#134878,
#134879,#134880,#134881,#134882,#134883,#134884,#134885,#134886,#134887,
#134888,#134889,#134890,#134891,#134892,#134893,#134894,#134895,#134896,
#134897,#134898,#134899,#134900,#134901,#134902,#134903,#134904,#134905,
#134906,#134907,#134908,#134909,#134910,#134911,#134912,#134913,#134914,
#134915,#134916,#134917,#134918,#134919,#134920,#134921,#134922,#134923,
#134924,#134925,#134926,#134927,#134928,#134929,#134930,#134931,#134932,
#134933,#134934,#134935,#134936,#134937,#134938,#134939,#134940,#134941,
#134942,#134943,#134944,#134945,#134946,#134947,#134948,#134949,#134950,
#134951,#134952,#134953,#134954,#134955,#134956,#134957,#134958,#134959,
#134960,#134961,#134962,#134963,#134964,#134965,#134966,#134967,#134968,
#134969,#134970,#134971,#134972,#134973,#134974,#134975,#134976,#134977,
#134978,#134979,#134980,#134981,#134982,#134983,#134984,#134985,#134986,
#134987,#134988,#134989,#134990,#134991,#134992,#134993,#134994,#134995,
#134996,#134997,#134998,#134999,#135000,#135001,#135002,#135003,#135004,
#135005,#135006,#135007,#135008,#135009,#135010,#135011,#135012,#135013,
#135014,#135015,#135016,#135017,#135018,#135019,#135020,#135021,#135022,
#135023,#135024,#135025,#135026,#135027,#135028,#135029,#135030,#135031,
#135032,#135033,#135034,#135035,#135036,#135037,#135038,#135039,#135040,
#135041,#135042,#135043,#135044,#135045,#135046,#135047,#135048,#135049,
#135050,#135051,#135052,#135053,#135054,#135055,#135056,#135057,#135058,
#135059,#135060,#135061,#135062,#135063,#135064,#135065,#135066,#135067,
#135068,#135069,#135070,#135071,#135072,#135073,#135074,#135075,#135076,
#135077,#135078,#135079,#135080,#135081,#135082,#135083,#135084,#135085,
#135086,#135087,#135088,#135089,#135090,#135091,#135092,#135093,#135094,
#135095,#135096,#135097,#135098,#135099,#135100,#135101,#135102,#135103,
#135104,#135105,#135106,#135107,#135108,#135109,#135110,#135111,#135112,
#135113,#135114,#135115,#135116,#135117,#135118,#135119,#135120,#135121,
#135122,#135123,#135124,#135125,#135126,#135127,#135128,#135129,#135130,
#135131,#135132,#135133,#135134,#135135,#135136,#135137,#135138,#135139,
#135140,#135141,#135142,#135143,#135144,#135145,#135146,#135147,#135148,
#135149,#135150,#135151,#135152,#135153,#135154,#135155,#135156,#135157,
#135158,#135159,#135160,#135161,#135162,#135163,#135164,#135165,#135166,
#135167,#135168,#135169,#135170,#135171,#135172,#135173,#135174,#135175,
#135176,#135177,#135178,#135179,#135180,#135181,#135182,#135183,#135184,
#135185,#135186,#135187,#135188,#135189,#135190,#135191,#135192,#135193,
#135194,#135195,#135196,#135197,#135198,#135199,#135200,#135201,#135202,
#135203,#135204,#135205,#135206,#135207,#135208,#135209,#135210,#135211,
#135212,#135213,#135214,#135215,#135216,#135217,#135218,#135219,#135220,
#135221,#135222,#135223,#135224,#135225,#135226,#135227,#135228,#135229,
#135230,#135231,#135232,#135233,#135234,#135235,#135236,#135237,#135238,
#135239,#135240,#135241,#135242,#135243,#135244,#135245,#135246,#135247,
#135248,#135249,#135250,#135251,#135252,#135253,#135254,#135255,#135256,
#135257,#135258,#135259,#135260,#135261,#135262,#135263,#135264,#135265,
#135266,#135267,#135268,#135269,#135270,#135271,#135272,#135273,#135274,
#135275,#135276,#135277,#135278,#135279,#135280,#135281,#135282,#135283,
#135284,#135285,#135286,#135287,#135288,#135289,#135290,#135291,#135292,
#135293,#135294,#135295,#135296,#135297,#135298,#135299,#135300,#135301,
#135302,#135303,#135304,#135305,#135306,#135307,#135308,#135309,#135310,
#135311,#135312,#135313,#135314,#135315,#135316,#135317,#135318,#135319,
#135320,#135321,#135322,#135323,#135324,#135325,#135326,#135327,#135328,
#135329,#135330,#135331,#135332,#135333,#135334,#135335,#135336,#135337,
#135338,#135339,#135340,#135341,#135342,#135343,#135344,#135345,#135346,
#135347,#135348,#135349,#135350,#135351,#135352,#135353,#135354,#135355,
#135356,#135357,#135358,#135359,#135360,#135361,#135362,#135363,#135364,
#135365,#135366,#135367,#135368,#135369,#135370,#135371,#135372,#135373,
#135374,#135375,#135376,#135377,#135378,#135379,#135380,#135381,#135382,
#135383,#135384,#135385,#135386,#135387,#135388,#135389,#135390,#135391,
#135392,#135393,#135394,#135395,#135396,#135397,#135398,#135399,#135400,
#135401,#135402,#135403,#135404,#135405,#135406,#135407,#135408,#135409,
#135410,#135411,#135412,#135413,#135414,#135415,#135416,#135417,#135418,
#135419,#135420,#135421,#135422,#135423,#135424,#135425,#135426,#135427,
#135428,#135429,#135430,#135431,#135432,#135433,#135434,#135435,#135436,
#135437,#135438,#135439,#135440,#135441,#135442,#135443,#135444,#135445,
#135446,#135447,#135448,#135449,#135450,#135451,#135452,#135453,#135454,
#135455,#135456,#135457,#135458,#135459,#135460,#135461,#135462,#135463,
#135464,#135465,#135466,#135467,#135468,#135469,#135470,#135471,#135472,
#135473,#135474,#135475,#135476,#135477,#135478,#135479,#135480,#135481,
#135482,#135483,#135484,#135485,#135486,#135487,#135488,#135489,#135490,
#135491,#135492,#135493,#135494,#135495,#135496,#135497,#135498,#135499,
#135500,#135501,#135502,#135503,#135504,#135505,#135506,#135507,#135508,
#135509,#135510,#135511,#135512,#135513,#135514,#135515,#135516,#135517,
#135518,#135519,#135520,#135521,#135522,#135523,#135524,#135525,#135526,
#135527,#135528,#135529,#135530,#135531,#135532,#135533,#135534,#135535,
#135536,#135537,#135538,#135539,#135540,#135541,#135542,#135543,#135544,
#135545,#135546,#135547,#135548,#135549,#135550,#135551,#135552,#135553,
#135554,#135555,#135556,#135557,#135558,#135559,#135560,#135561,#135562,
#135563,#135564,#135565,#135566,#135567,#135568,#135569,#135570,#135571,
#135572,#135573,#135574,#135575,#135576,#135577,#135578,#135579,#135580,
#135581,#135582,#135583,#135584,#135585,#135586,#135587,#135588,#135589,
#135590,#135591,#135592,#135593,#135594,#135595,#135596,#135597,#135598,
#135599,#135600,#135601,#135602,#135603,#135604,#135605,#135606,#135607,
#135608,#135609,#135610,#135611,#135612,#135613,#135614,#135615,#135616,
#135617,#135618,#135619,#135620,#135621,#135622,#135623,#135624,#135625,
#135626,#135627,#135628,#135629,#135630,#135631,#135632,#135633,#135634,
#135635,#135636,#135637,#135638,#135639,#135640,#135641,#135642,#135643,
#135644,#135645,#135646,#135647,#135648,#135649,#135650,#135651,#135652,
#135653,#135654,#135655,#135656,#135657,#135658,#135659,#135660,#135661,
#135662,#135663,#135664,#135665,#135666,#135667,#135668,#135669,#135670,
#135671,#135672,#135673,#135674,#135675,#135676,#135677,#135678,#135679,
#135680,#135681,#135682,#135683,#135684,#135685,#135686,#135687,#135688,
#135689,#135690,#135691,#135692,#135693,#135694,#135695,#135696,#135697,
#135698,#135699,#135700,#135701,#135702,#135703,#135704,#135705,#135706,
#135707,#135708,#135709,#135710,#135711,#135712,#135713,#135714,#135715,
#135716,#135717,#135718,#135719,#135720,#135721,#135722,#135723,#135724,
#135725,#135726,#135727,#135728,#135729,#135730,#135731,#135732,#135733,
#135734,#135735,#135736,#135737,#135738,#135739,#135740,#135741,#135742,
#135743,#135744,#135745,#135746,#135747,#135748,#135749,#135750,#135751,
#135752,#135753,#135754,#135755,#135756,#135757,#135758,#135759,#135760,
#135761,#135762,#135763,#135764,#135765,#135766,#135767,#135768,#135769,
#135770,#135771,#135772,#135773,#135774,#135775,#135776,#135777,#135778,
#135779,#135780,#135781,#135782,#135783,#135784,#135785,#135786,#135787,
#135788,#135789,#135790,#135791,#135792,#135793,#135794,#135795,#135796,
#135797,#135798,#135799,#135800,#135801,#135802,#135803,#135804,#135805,
#135806,#135807,#135808,#135809,#135810,#135811,#135812,#135813,#135814,
#135815,#135816,#135817,#135818,#135819,#135820,#135821,#135822,#135823,
#135824,#135825,#135826,#135827,#135828,#135829,#135830,#135831,#135832,
#135833,#135834,#135835,#135836,#135837,#135838,#135839,#135840,#135841,
#135842,#135843,#135844,#135845,#135846,#135847,#135848,#135849,#135850,
#135851,#135852,#135853,#135854,#135855,#135856,#135857,#135858,#135859,
#135860,#135861,#135862,#135863,#135864,#135865,#135866,#135867,#135868,
#135869,#135870,#135871,#135872,#135873,#135874,#135875,#135876,#135877,
#135878,#135879,#135880,#135881,#135882,#135883,#135884,#135885,#135886,
#135887,#135888,#135889,#135890,#135891,#135892,#135893,#135894,#135895,
#135896,#135897,#135898,#135899,#135900,#135901,#135902,#135903,#135904,
#135905,#135906,#135907,#135908,#135909,#135910,#135911,#135912,#135913,
#135914,#135915,#135916,#135917,#135918,#135919,#135920,#135921,#135922,
#135923,#135924,#135925,#135926,#135927,#135928,#135929,#135930,#135931,
#135932,#135933,#135934,#135935,#135936,#135937,#135938,#135939,#135940,
#135941,#135942,#135943,#135944,#135945,#135946,#135947,#135948,#135949,
#135950,#135951,#135952,#135953,#135954,#135955,#135956,#135957,#135958,
#135959,#135960,#135961,#135962,#135963,#135964,#135965,#135966,#135967,
#135968,#135969,#135970,#135971,#135972,#135973,#135974,#135975,#135976,
#135977,#135978,#135979,#135980,#135981,#135982,#135983,#135984,#135985,
#135986,#135987,#135988,#135989,#135990,#135991,#135992,#135993,#135994,
#135995,#135996,#135997,#135998,#135999,#136000,#136001,#136002,#136003,
#136004,#136005,#136006,#136007,#136008,#136009,#136010,#136011,#136012,
#136013,#136014,#136015,#136016,#136017,#136018,#136019,#136020,#136021,
#136022,#136023,#136024,#136025,#136026,#136027,#136028,#136029,#136030,
#136031,#136032,#136033,#136034,#136035,#136036,#136037,#136038,#136039,
#136040,#136041,#136042,#136043,#136044,#136045,#136046,#136047,#136048,
#136049,#136050,#136051,#136052,#136053,#136054,#136055,#136056,#136057,
#136058,#136059,#136060,#136061,#136062,#136063,#136064,#136065,#136066,
#136067,#136068,#136069,#136070,#136071,#136072,#136073,#136074,#136075,
#136076,#136077,#136078,#136079,#136080,#136081,#136082,#136083,#136084,
#136085,#136086,#136087,#136088,#136089,#136090,#136091,#136092,#136093,
#136094,#136095,#136096,#136097,#136098,#136099,#136100,#136101,#136102,
#136103,#136104,#136105,#136106,#136107,#136108,#136109,#136110,#136111,
#136112,#136113,#136114,#136115,#136116,#136117,#136118,#136119,#136120,
#136121,#136122,#136123,#136124,#136125,#136126,#136127,#136128,#136129,
#136130,#136131,#136132,#136133,#136134,#136135,#136136,#136137,#136138,
#136139,#136140,#136141,#136142,#136143,#136144,#136145,#136146,#136147,
#136148,#136149,#136150,#136151,#136152,#136153,#136154,#136155,#136156,
#136157,#136158,#136159,#136160,#136161,#136162,#136163,#136164,#136165,
#136166,#136167,#136168,#136169,#136170,#136171,#136172,#136173,#136174,
#136175,#136176,#136177,#136178,#136179,#136180,#136181,#136182,#136183,
#136184,#136185,#136186,#136187,#136188,#136189,#136190,#136191,#136192,
#136193,#136194,#136195,#136196,#136197,#136198,#136199,#136200,#136201,
#136202,#136203,#136204,#136205,#136206,#136207,#136208,#136209,#136210,
#136211,#136212,#136213,#136214,#136215,#136216,#136217,#136218,#136219,
#136220,#136221,#136222,#136223,#136224,#136225,#136226,#136227,#136228,
#136229,#136230,#136231,#136232,#136233,#136234,#136235,#136236,#136237,
#136238,#136239,#136240,#136241,#136242,#136243,#136244,#136245,#136246,
#136247,#136248,#136249,#136250,#136251,#136252,#136253,#136254,#136255,
#136256,#136257,#136258,#136259,#136260,#136261,#136262,#136263,#136264,
#136265,#136266,#136267,#136268,#136269,#136270,#136271,#136272,#136273,
#136274,#136275,#136276,#136277,#136278,#136279,#136280,#136281,#136282,
#136283,#136284,#136285,#136286,#136287,#136288,#136289,#136290,#136291,
#136292,#136293,#136294,#136295,#136296,#136297,#136298,#136299,#136300,
#136301,#136302,#136303,#136304,#136305,#136306,#136307,#136308,#136309,
#136310,#136311,#136312,#136313,#136314,#136315,#136316,#136317,#136318,
#136319,#136320,#136321,#136322,#136323,#136324,#136325,#136326,#136327,
#136328,#136329,#136330,#136331,#136332,#136333,#136334,#136335,#136336,
#136337,#136338,#136339,#136340,#136341,#136342,#136343,#136344,#136345,
#136346,#136347,#136348,#136349,#136350,#136351,#136352,#136353,#136354,
#136355,#136356,#136357,#136358,#136359,#136360,#136361,#136362,#136363,
#136364,#136365,#136366,#136367,#136368,#136369,#136370,#136371,#136372,
#136373,#136374,#136375,#136376,#136377,#136378,#136379,#136380,#136381,
#136382,#136383,#136384,#136385,#136386,#136387,#136388,#136389,#136390,
#136391,#136392,#136393,#136394,#136395,#136396,#136397,#136398,#136399,
#136400,#136401,#136402,#136403,#136404,#136405,#136406,#136407,#136408,
#136409,#136410,#136411,#136412,#136413,#136414,#136415,#136416,#136417,
#136418,#136419),(#136420,#136421,#136422,#136423,#136424,#136425,#136426,
#136427,#136428,#136429,#136430,#136431,#136432,#136433,#136434,#136435,
#136436,#136437,#136438,#136439,#136440,#136441,#136442,#136443,#136444,
#136445,#136446,#136447,#136448,#136449,#136450,#136451,#136452,#136453,
#136454,#136455,#136456,#136457,#136458,#136459,#136460,#136461,#136462,
#136463,#136464,#136465,#136466,#136467,#136468,#136469,#136470,#136471,
#136472,#136473,#136474,#136475,#136476,#136477,#136478,#136479,#136480,
#136481,#136482,#136483,#136484,#136485,#136486,#136487,#136488,#136489,
#136490,#136491,#136492,#136493,#136494,#136495,#136496,#136497,#136498,
#136499,#136500,#136501,#136502,#136503,#136504,#136505,#136506,#136507,
#136508,#136509,#136510,#136511,#136512,#136513,#136514,#136515,#136516,
#136517,#136518,#136519,#136520,#136521,#136522,#136523,#136524,#136525,
#136526,#136527,#136528,#136529,#136530,#136531,#136532,#136533,#136534,
#136535,#136536,#136537,#136538,#136539,#136540,#136541,#136542,#136543,
#136544,#136545,#136546,#136547,#136548,#136549,#136550,#136551,#136552,
#136553,#136554,#136555,#136556,#136557,#136558,#136559,#136560,#136561,
#136562,#136563,#136564,#136565,#136566,#136567,#136568,#136569,#136570,
#136571,#136572,#136573,#136574,#136575,#136576,#136577,#136578,#136579,
#136580,#136581,#136582,#136583,#136584,#136585,#136586,#136587,#136588,
#136589,#136590,#136591,#136592,#136593,#136594,#136595,#136596,#136597,
#136598,#136599,#136600,#136601,#136602,#136603,#136604,#136605,#136606,
#136607,#136608,#136609,#136610,#136611,#136612,#136613,#136614,#136615,
#136616,#136617,#136618,#136619,#136620,#136621,#136622,#136623,#136624,
#136625,#136626,#136627,#136628,#136629,#136630,#136631,#136632,#136633,
#136634,#136635,#136636,#136637,#136638,#136639,#136640,#136641,#136642,
#136643,#136644,#136645,#136646,#136647,#136648,#136649,#136650,#136651,
#136652,#136653,#136654,#136655,#136656,#136657,#136658,#136659,#136660,
#136661,#136662,#136663,#136664,#136665,#136666,#136667,#136668,#136669,
#136670,#136671,#136672,#136673,#136674,#136675,#136676,#136677,#136678,
#136679,#136680,#136681,#136682,#136683,#136684,#136685,#136686,#136687,
#136688,#136689,#136690,#136691,#136692,#136693,#136694,#136695,#136696,
#136697,#136698,#136699,#136700,#136701,#136702,#136703,#136704,#136705,
#136706,#136707,#136708,#136709,#136710,#136711,#136712,#136713,#136714,
#136715,#136716,#136717,#136718,#136719,#136720,#136721,#136722,#136723,
#136724,#136725,#136726,#136727,#136728,#136729,#136730,#136731,#136732,
#136733,#136734,#136735,#136736,#136737,#136738,#136739,#136740,#136741,
#136742,#136743,#136744,#136745,#136746,#136747,#136748,#136749,#136750,
#136751,#136752,#136753,#136754,#136755,#136756,#136757,#136758,#136759,
#136760,#136761,#136762,#136763,#136764,#136765,#136766,#136767,#136768,
#136769,#136770,#136771,#136772,#136773,#136774,#136775,#136776,#136777,
#136778,#136779,#136780,#136781,#136782,#136783,#136784,#136785,#136786,
#136787,#136788,#136789,#136790,#136791,#136792,#136793,#136794,#136795,
#136796,#136797,#136798,#136799,#136800,#136801,#136802,#136803,#136804,
#136805,#136806,#136807,#136808,#136809,#136810,#136811,#136812,#136813,
#136814,#136815,#136816,#136817,#136818,#136819,#136820,#136821,#136822,
#136823,#136824,#136825,#136826,#136827,#136828,#136829,#136830,#136831,
#136832,#136833,#136834,#136835,#136836,#136837,#136838,#136839,#136840,
#136841,#136842,#136843,#136844,#136845,#136846,#136847,#136848,#136849,
#136850,#136851,#136852,#136853,#136854,#136855,#136856,#136857,#136858,
#136859,#136860,#136861,#136862,#136863,#136864,#136865,#136866,#136867,
#136868,#136869,#136870,#136871,#136872,#136873,#136874,#136875,#136876,
#136877,#136878,#136879,#136880,#136881,#136882,#136883,#136884,#136885,
#136886,#136887,#136888,#136889,#136890,#136891,#136892,#136893,#136894,
#136895,#136896,#136897,#136898,#136899,#136900,#136901,#136902,#136903,
#136904,#136905,#136906,#136907,#136908,#136909,#136910,#136911,#136912,
#136913,#136914,#136915,#136916,#136917,#136918,#136919,#136920,#136921,
#136922,#136923,#136924,#136925,#136926,#136927,#136928,#136929,#136930,
#136931,#136932,#136933,#136934,#136935,#136936,#136937,#136938,#136939,
#136940,#136941,#136942,#136943,#136944,#136945,#136946,#136947,#136948,
#136949,#136950,#136951,#136952,#136953,#136954,#136955,#136956,#136957,
#136958,#136959,#136960,#136961,#136962,#136963,#136964,#136965,#136966,
#136967,#136968,#136969,#136970,#136971,#136972,#136973,#136974,#136975,
#136976,#136977,#136978,#136979,#136980,#136981,#136982,#136983,#136984,
#136985,#136986,#136987,#136988,#136989,#136990,#136991,#136992,#136993,
#136994,#136995,#136996,#136997,#136998,#136999,#137000,#137001,#137002,
#137003,#137004,#137005,#137006,#137007,#137008,#137009,#137010,#137011,
#137012,#137013,#137014,#137015,#137016,#137017,#137018,#137019,#137020,
#137021,#137022,#137023,#137024,#137025,#137026,#137027,#137028,#137029,
#137030,#137031,#137032,#137033,#137034,#137035,#137036,#137037,#137038,
#137039,#137040,#137041,#137042,#137043,#137044,#137045,#137046,#137047,
#137048,#137049,#137050,#137051,#137052,#137053,#137054,#137055,#137056,
#137057,#137058,#137059,#137060,#137061,#137062,#137063,#137064,#137065,
#137066,#137067,#137068,#137069,#137070,#137071,#137072,#137073,#137074,
#137075,#137076,#137077,#137078,#137079,#137080,#137081,#137082,#137083,
#137084,#137085,#137086,#137087,#137088,#137089,#137090,#137091,#137092,
#137093,#137094,#137095,#137096,#137097,#137098,#137099,#137100,#137101,
#137102,#137103,#137104,#137105,#137106,#137107,#137108,#137109,#137110,
#137111,#137112,#137113,#137114,#137115,#137116,#137117,#137118,#137119,
#137120,#137121,#137122,#137123,#137124,#137125,#137126,#137127,#137128,
#137129,#137130,#137131,#137132,#137133,#137134,#137135,#137136,#137137,
#137138,#137139,#137140,#137141,#137142,#137143,#137144,#137145,#137146,
#137147,#137148,#137149,#137150,#137151,#137152,#137153,#137154,#137155,
#137156,#137157,#137158,#137159,#137160,#137161,#137162,#137163,#137164,
#137165,#137166,#137167,#137168,#137169,#137170,#137171,#137172,#137173,
#137174,#137175,#137176,#137177,#137178,#137179,#137180,#137181,#137182,
#137183,#137184,#137185,#137186,#137187,#137188,#137189,#137190,#137191,
#137192,#137193,#137194,#137195,#137196,#137197,#137198,#137199,#137200,
#137201,#137202,#137203,#137204,#137205,#137206,#137207,#137208,#137209,
#137210,#137211,#137212,#137213,#137214,#137215,#137216,#137217,#137218,
#137219,#137220,#137221,#137222,#137223,#137224,#137225,#137226,#137227,
#137228,#137229,#137230,#137231,#137232,#137233,#137234,#137235,#137236,
#137237,#137238,#137239,#137240,#137241,#137242,#137243,#137244,#137245,
#137246,#137247,#137248,#137249,#137250,#137251,#137252,#137253,#137254,
#137255,#137256,#137257,#137258,#137259,#137260,#137261,#137262,#137263,
#137264,#137265,#137266,#137267,#137268,#137269,#137270,#137271,#137272,
#137273,#137274,#137275,#137276,#137277,#137278,#137279,#137280,#137281,
#137282,#137283,#137284,#137285,#137286,#137287,#137288,#137289,#137290,
#137291,#137292,#137293,#137294,#137295,#137296,#137297,#137298,#137299,
#137300,#137301,#137302,#137303,#137304,#137305,#137306,#137307,#137308,
#137309,#137310,#137311,#137312,#137313,#137314,#137315,#137316,#137317,
#137318,#137319,#137320,#137321,#137322,#137323,#137324,#137325,#137326,
#137327,#137328,#137329,#137330,#137331,#137332,#137333,#137334,#137335,
#137336,#137337,#137338,#137339,#137340,#137341,#137342,#137343,#137344,
#137345,#137346,#137347,#137348,#137349,#137350,#137351,#137352,#137353,
#137354,#137355,#137356,#137357,#137358,#137359,#137360,#137361,#137362,
#137363,#137364,#137365,#137366,#137367,#137368,#137369,#137370,#137371,
#137372,#137373,#137374,#137375,#137376,#137377,#137378,#137379,#137380,
#137381,#137382,#137383,#137384,#137385,#137386,#137387,#137388,#137389,
#137390,#137391,#137392,#137393,#137394,#137395,#137396,#137397,#137398,
#137399,#137400,#137401,#137402,#137403,#137404,#137405,#137406,#137407,
#137408,#137409,#137410,#137411,#137412,#137413,#137414,#137415,#137416,
#137417,#137418,#137419,#137420,#137421,#137422,#137423,#137424,#137425,
#137426,#137427,#137428,#137429,#137430,#137431,#137432,#137433,#137434,
#137435,#137436,#137437,#137438,#137439,#137440,#137441,#137442,#137443,
#137444,#137445,#137446,#137447,#137448,#137449,#137450,#137451,#137452,
#137453,#137454,#137455,#137456,#137457,#137458,#137459,#137460,#137461,
#137462,#137463,#137464,#137465,#137466,#137467,#137468,#137469,#137470,
#137471,#137472,#137473,#137474,#137475,#137476,#137477,#137478,#137479,
#137480,#137481,#137482,#137483,#137484,#137485,#137486,#137487,#137488,
#137489,#137490,#137491,#137492,#137493,#137494,#137495,#137496,#137497,
#137498,#137499,#137500,#137501,#137502,#137503,#137504,#137505,#137506,
#137507,#137508,#137509,#137510,#137511,#137512,#137513,#137514,#137515,
#137516,#137517,#137518,#137519,#137520,#137521,#137522,#137523,#137524,
#137525,#137526,#137527,#137528,#137529,#137530,#137531,#137532,#137533,
#137534,#137535,#137536,#137537,#137538,#137539,#137540,#137541,#137542,
#137543,#137544,#137545,#137546,#137547,#137548,#137549,#137550,#137551,
#137552,#137553,#137554,#137555,#137556,#137557,#137558,#137559,#137560,
#137561,#137562,#137563,#137564,#137565,#137566,#137567,#137568,#137569,
#137570,#137571,#137572,#137573,#137574,#137575,#137576,#137577,#137578,
#137579,#137580,#137581,#137582,#137583,#137584,#137585,#137586,#137587,
#137588,#137589,#137590,#137591,#137592,#137593,#137594,#137595,#137596,
#137597,#137598,#137599,#137600,#137601,#137602,#137603,#137604,#137605,
#137606,#137607,#137608,#137609,#137610,#137611,#137612,#137613,#137614,
#137615,#137616,#137617,#137618,#137619,#137620,#137621,#137622,#137623,
#137624,#137625,#137626,#137627,#137628,#137629,#137630,#137631,#137632,
#137633,#137634,#137635,#137636,#137637,#137638,#137639,#137640,#137641,
#137642,#137643,#137644,#137645,#137646,#137647,#137648,#137649,#137650,
#137651,#137652,#137653,#137654,#137655,#137656,#137657,#137658,#137659,
#137660,#137661,#137662,#137663,#137664,#137665,#137666,#137667,#137668,
#137669,#137670,#137671,#137672,#137673,#137674,#137675,#137676,#137677,
#137678,#137679,#137680,#137681,#137682,#137683,#137684,#137685,#137686,
#137687,#137688,#137689,#137690,#137691,#137692,#137693,#137694,#137695,
#137696,#137697,#137698,#137699,#137700,#137701,#137702,#137703,#137704,
#137705,#137706,#137707,#137708,#137709,#137710,#137711,#137712,#137713,
#137714,#137715,#137716,#137717,#137718,#137719,#137720,#137721,#137722,
#137723,#137724,#137725,#137726,#137727,#137728,#137729,#137730,#137731,
#137732,#137733,#137734,#137735,#137736,#137737,#137738,#137739,#137740,
#137741,#137742,#137743,#137744,#137745,#137746,#137747,#137748,#137749,
#137750,#137751,#137752,#137753,#137754,#137755,#137756,#137757,#137758,
#137759,#137760,#137761,#137762,#137763,#137764,#137765,#137766,#137767,
#137768,#137769,#137770,#137771,#137772,#137773,#137774,#137775,#137776,
#137777,#137778,#137779,#137780,#137781,#137782,#137783,#137784,#137785,
#137786,#137787,#137788,#137789,#137790,#137791,#137792,#137793,#137794,
#137795,#137796,#137797,#137798,#137799,#137800,#137801,#137802,#137803,
#137804,#137805,#137806,#137807,#137808,#137809,#137810,#137811,#137812,
#137813,#137814,#137815,#137816,#137817,#137818,#137819,#137820,#137821,
#137822,#137823,#137824,#137825,#137826,#137827,#137828,#137829,#137830,
#137831,#137832,#137833,#137834,#137835,#137836,#137837,#137838,#137839,
#137840,#137841,#137842,#137843,#137844,#137845,#137846,#137847,#137848,
#137849,#137850,#137851,#137852,#137853,#137854,#137855,#137856,#137857,
#137858,#137859,#137860,#137861,#137862,#137863,#137864,#137865,#137866,
#137867,#137868,#137869,#137870,#137871,#137872,#137873,#137874,#137875,
#137876,#137877,#137878,#137879,#137880,#137881,#137882,#137883,#137884,
#137885,#137886,#137887,#137888,#137889,#137890,#137891,#137892,#137893,
#137894,#137895,#137896,#137897,#137898,#137899,#137900,#137901,#137902,
#137903,#137904,#137905,#137906,#137907,#137908,#137909,#137910,#137911,
#137912,#137913,#137914,#137915,#137916,#137917,#137918,#137919,#137920,
#137921,#137922,#137923,#137924,#137925,#137926,#137927,#137928,#137929,
#137930,#137931,#137932,#137933,#137934,#137935,#137936,#137937,#137938,
#137939,#137940,#137941,#137942,#137943,#137944,#137945,#137946,#137947,
#137948,#137949,#137950,#137951,#137952,#137953,#137954,#137955,#137956,
#137957,#137958,#137959,#137960,#137961,#137962,#137963,#137964,#137965,
#137966,#137967,#137968,#137969,#137970,#137971,#137972,#137973,#137974,
#137975,#137976,#137977,#137978,#137979,#137980,#137981,#137982,#137983,
#137984,#137985,#137986,#137987,#137988,#137989,#137990,#137991,#137992,
#137993,#137994,#137995,#137996,#137997,#137998,#137999,#138000,#138001,
#138002,#138003,#138004,#138005,#138006,#138007,#138008,#138009,#138010,
#138011,#138012,#138013,#138014,#138015,#138016,#138017,#138018,#138019,
#138020,#138021,#138022,#138023,#138024,#138025,#138026,#138027,#138028,
#138029,#138030,#138031,#138032,#138033,#138034,#138035,#138036,#138037,
#138038,#138039,#138040,#138041,#138042,#138043,#138044,#138045,#138046,
#138047,#138048,#138049,#138050,#138051,#138052,#138053,#138054,#138055,
#138056,#138057,#138058,#138059,#138060,#138061,#138062,#138063,#138064,
#138065,#138066,#138067,#138068,#138069,#138070,#138071,#138072,#138073,
#138074,#138075,#138076,#138077,#138078,#138079,#138080,#138081,#138082,
#138083,#138084,#138085,#138086,#138087,#138088,#138089,#138090,#138091,
#138092,#138093,#138094,#138095,#138096,#138097,#138098,#138099,#138100,
#138101,#138102,#138103,#138104,#138105,#138106,#138107,#138108,#138109,
#138110,#138111,#138112,#138113,#138114,#138115,#138116,#138117,#138118,
#138119,#138120,#138121,#138122,#138123,#138124,#138125,#138126,#138127,
#138128,#138129,#138130,#138131,#138132,#138133,#138134,#138135,#138136,
#138137,#138138,#138139,#138140,#138141,#138142,#138143,#138144,#138145,
#138146,#138147,#138148,#138149,#138150,#138151,#138152,#138153,#138154,
#138155,#138156,#138157,#138158,#138159,#138160,#138161,#138162,#138163,
#138164,#138165,#138166,#138167,#138168,#138169,#138170,#138171,#138172,
#138173,#138174,#138175,#138176,#138177,#138178,#138179,#138180,#138181,
#138182,#138183,#138184,#138185,#138186,#138187,#138188,#138189,#138190,
#138191,#138192,#138193,#138194,#138195,#138196,#138197,#138198,#138199,
#138200,#138201,#138202,#138203,#138204,#138205,#138206,#138207,#138208,
#138209,#138210,#138211,#138212,#138213,#138214,#138215,#138216,#138217,
#138218,#138219,#138220,#138221,#138222,#138223,#138224,#138225,#138226,
#138227,#138228,#138229,#138230,#138231,#138232,#138233,#138234,#138235,
#138236,#138237,#138238,#138239,#138240,#138241,#138242,#138243,#138244,
#138245,#138246,#138247,#138248,#138249,#138250,#138251,#138252,#138253,
#138254,#138255,#138256,#138257,#138258,#138259,#138260,#138261,#138262,
#138263,#138264,#138265,#138266,#138267,#138268,#138269,#138270,#138271,
#138272,#138273,#138274,#138275,#138276,#138277,#138278,#138279,#138280,
#138281,#138282,#138283,#138284,#138285,#138286,#138287,#138288,#138289,
#138290,#138291,#138292,#138293,#138294,#138295,#138296,#138297,#138298,
#138299,#138300,#138301,#138302,#138303,#138304,#138305,#138306,#138307,
#138308,#138309,#138310,#138311,#138312,#138313,#138314,#138315,#138316,
#138317,#138318,#138319,#138320,#138321,#138322,#138323,#138324,#138325,
#138326,#138327,#138328,#138329,#138330,#138331,#138332,#138333,#138334,
#138335,#138336,#138337,#138338,#138339,#138340,#138341,#138342,#138343,
#138344,#138345,#138346,#138347,#138348,#138349,#138350,#138351,#138352,
#138353,#138354,#138355,#138356,#138357,#138358,#138359,#138360,#138361,
#138362,#138363,#138364,#138365,#138366,#138367,#138368,#138369,#138370,
#138371,#138372,#138373,#138374,#138375,#138376,#138377,#138378,#138379,
#138380,#138381,#138382,#138383,#138384,#138385,#138386,#138387,#138388,
#138389,#138390,#138391,#138392,#138393,#138394,#138395,#138396,#138397,
#138398,#138399,#138400,#138401,#138402,#138403,#138404,#138405,#138406,
#138407,#138408,#138409,#138410,#138411,#138412,#138413,#138414,#138415,
#138416,#138417,#138418,#138419,#138420,#138421,#138422,#138423,#138424,
#138425,#138426,#138427,#138428,#138429,#138430,#138431,#138432,#138433,
#138434,#138435,#138436,#138437,#138438,#138439,#138440,#138441,#138442,
#138443,#138444,#138445,#138446,#138447,#138448,#138449,#138450,#138451,
#138452,#138453,#138454,#138455,#138456,#138457,#138458,#138459,#138460,
#138461,#138462,#138463,#138464,#138465,#138466,#138467,#138468,#138469,
#138470),(#138471,#138472,#138473,#138474,#138475,#138476,#138477,#138478,
#138479,#138480,#138481,#138482,#138483,#138484,#138485,#138486,#138487,
#138488,#138489,#138490,#138491,#138492,#138493,#138494,#138495,#138496,
#138497,#138498,#138499,#138500,#138501,#138502,#138503,#138504,#138505,
#138506,#138507,#138508,#138509,#138510,#138511,#138512,#138513,#138514,
#138515,#138516,#138517,#138518,#138519,#138520,#138521,#138522,#138523,
#138524,#138525,#138526,#138527,#138528,#138529,#138530,#138531,#138532,
#138533,#138534,#138535,#138536,#138537,#138538,#138539,#138540,#138541,
#138542,#138543,#138544,#138545,#138546,#138547,#138548,#138549,#138550,
#138551,#138552,#138553,#138554,#138555,#138556,#138557,#138558,#138559,
#138560,#138561,#138562,#138563,#138564,#138565,#138566,#138567,#138568,
#138569,#138570,#138571,#138572,#138573,#138574,#138575,#138576,#138577,
#138578,#138579,#138580,#138581,#138582,#138583,#138584,#138585,#138586,
#138587,#138588,#138589,#138590,#138591,#138592,#138593,#138594,#138595,
#138596,#138597,#138598,#138599,#138600,#138601,#138602,#138603,#138604,
#138605,#138606,#138607,#138608,#138609,#138610,#138611,#138612,#138613,
#138614,#138615,#138616,#138617,#138618,#138619,#138620,#138621,#138622,
#138623,#138624,#138625,#138626,#138627,#138628,#138629,#138630,#138631,
#138632,#138633,#138634,#138635,#138636,#138637,#138638,#138639,#138640,
#138641,#138642,#138643,#138644,#138645,#138646,#138647,#138648,#138649,
#138650,#138651,#138652,#138653,#138654,#138655,#138656,#138657,#138658,
#138659,#138660,#138661,#138662,#138663,#138664,#138665,#138666,#138667,
#138668,#138669,#138670,#138671,#138672,#138673,#138674,#138675,#138676,
#138677,#138678,#138679,#138680,#138681,#138682,#138683,#138684,#138685,
#138686,#138687,#138688,#138689,#138690,#138691,#138692,#138693,#138694,
#138695,#138696,#138697,#138698,#138699,#138700,#138701,#138702,#138703,
#138704,#138705,#138706,#138707,#138708,#138709,#138710,#138711,#138712,
#138713,#138714,#138715,#138716,#138717,#138718,#138719,#138720,#138721,
#138722,#138723,#138724,#138725,#138726,#138727,#138728,#138729,#138730,
#138731,#138732,#138733,#138734,#138735,#138736,#138737,#138738,#138739,
#138740,#138741,#138742,#138743,#138744,#138745,#138746,#138747,#138748,
#138749,#138750,#138751,#138752,#138753,#138754,#138755,#138756,#138757,
#138758,#138759,#138760,#138761,#138762,#138763,#138764,#138765,#138766,
#138767,#138768,#138769,#138770,#138771,#138772,#138773,#138774,#138775,
#138776,#138777,#138778,#138779,#138780,#138781,#138782,#138783,#138784,
#138785,#138786,#138787,#138788,#138789,#138790,#138791,#138792,#138793,
#138794,#138795,#138796,#138797,#138798,#138799,#138800,#138801,#138802,
#138803,#138804,#138805,#138806,#138807,#138808,#138809,#138810,#138811,
#138812,#138813,#138814,#138815,#138816,#138817,#138818,#138819,#138820,
#138821,#138822,#138823,#138824,#138825,#138826,#138827,#138828,#138829,
#138830,#138831,#138832,#138833,#138834,#138835,#138836,#138837,#138838,
#138839,#138840,#138841,#138842,#138843,#138844,#138845,#138846,#138847,
#138848,#138849,#138850,#138851,#138852,#138853,#138854,#138855,#138856,
#138857,#138858,#138859,#138860,#138861,#138862,#138863,#138864,#138865,
#138866,#138867,#138868,#138869,#138870,#138871,#138872,#138873,#138874,
#138875,#138876,#138877,#138878,#138879,#138880,#138881,#138882,#138883,
#138884,#138885,#138886,#138887,#138888,#138889,#138890,#138891,#138892,
#138893,#138894,#138895,#138896,#138897,#138898,#138899,#138900,#138901,
#138902,#138903,#138904,#138905,#138906,#138907,#138908,#138909,#138910,
#138911,#138912,#138913,#138914,#138915,#138916,#138917,#138918,#138919,
#138920,#138921,#138922,#138923,#138924,#138925,#138926,#138927,#138928,
#138929,#138930,#138931,#138932,#138933,#138934,#138935,#138936,#138937,
#138938,#138939,#138940,#138941,#138942,#138943,#138944,#138945,#138946,
#138947,#138948,#138949,#138950,#138951,#138952,#138953,#138954,#138955,
#138956,#138957,#138958,#138959,#138960,#138961,#138962,#138963,#138964,
#138965,#138966,#138967,#138968,#138969,#138970,#138971,#138972,#138973,
#138974,#138975,#138976,#138977,#138978,#138979,#138980,#138981,#138982,
#138983,#138984,#138985,#138986,#138987,#138988,#138989,#138990,#138991,
#138992,#138993,#138994,#138995,#138996,#138997,#138998,#138999,#139000,
#139001,#139002,#139003,#139004,#139005,#139006,#139007,#139008,#139009,
#139010,#139011,#139012,#139013,#139014,#139015,#139016,#139017,#139018,
#139019,#139020,#139021,#139022,#139023,#139024,#139025,#139026,#139027,
#139028,#139029,#139030,#139031,#139032,#139033,#139034,#139035,#139036,
#139037,#139038,#139039,#139040,#139041,#139042,#139043,#139044,#139045,
#139046,#139047,#139048,#139049,#139050,#139051,#139052,#139053,#139054,
#139055,#139056,#139057,#139058,#139059,#139060,#139061,#139062,#139063,
#139064,#139065,#139066,#139067,#139068,#139069,#139070,#139071,#139072,
#139073,#139074,#139075,#139076,#139077,#139078,#139079,#139080,#139081,
#139082,#139083,#139084,#139085,#139086,#139087,#139088,#139089,#139090,
#139091,#139092,#139093,#139094,#139095,#139096,#139097,#139098,#139099,
#139100,#139101,#139102,#139103,#139104,#139105,#139106,#139107,#139108,
#139109,#139110,#139111,#139112,#139113,#139114,#139115,#139116,#139117,
#139118,#139119,#139120,#139121,#139122,#139123,#139124,#139125,#139126,
#139127,#139128,#139129,#139130,#139131,#139132,#139133,#139134,#139135,
#139136,#139137,#139138,#139139,#139140,#139141,#139142,#139143,#139144,
#139145,#139146,#139147,#139148,#139149,#139150,#139151,#139152,#139153,
#139154,#139155,#139156,#139157,#139158,#139159,#139160,#139161,#139162,
#139163,#139164,#139165,#139166,#139167,#139168,#139169,#139170,#139171,
#139172,#139173,#139174,#139175,#139176,#139177,#139178,#139179,#139180,
#139181,#139182,#139183,#139184,#139185,#139186,#139187,#139188,#139189,
#139190,#139191,#139192,#139193,#139194,#139195,#139196,#139197,#139198,
#139199,#139200,#139201,#139202,#139203,#139204,#139205,#139206,#139207,
#139208,#139209,#139210,#139211,#139212,#139213,#139214,#139215,#139216,
#139217,#139218,#139219,#139220,#139221,#139222,#139223,#139224,#139225,
#139226,#139227,#139228,#139229,#139230,#139231,#139232,#139233,#139234,
#139235,#139236,#139237,#139238,#139239,#139240,#139241,#139242,#139243,
#139244,#139245,#139246,#139247,#139248,#139249,#139250,#139251,#139252,
#139253,#139254,#139255,#139256,#139257,#139258,#139259,#139260,#139261,
#139262,#139263,#139264,#139265,#139266,#139267,#139268,#139269,#139270,
#139271,#139272,#139273,#139274,#139275,#139276,#139277,#139278,#139279,
#139280,#139281,#139282,#139283,#139284,#139285,#139286,#139287,#139288,
#139289,#139290,#139291,#139292,#139293,#139294,#139295,#139296,#139297,
#139298,#139299,#139300,#139301,#139302,#139303,#139304,#139305,#139306,
#139307,#139308,#139309,#139310,#139311,#139312,#139313,#139314,#139315,
#139316,#139317,#139318,#139319,#139320,#139321,#139322,#139323,#139324,
#139325,#139326,#139327,#139328,#139329,#139330,#139331,#139332,#139333,
#139334,#139335,#139336,#139337,#139338,#139339,#139340,#139341,#139342,
#139343,#139344,#139345,#139346,#139347,#139348,#139349,#139350,#139351,
#139352,#139353,#139354,#139355,#139356,#139357,#139358,#139359,#139360,
#139361,#139362,#139363,#139364,#139365,#139366,#139367,#139368,#139369,
#139370,#139371,#139372,#139373,#139374,#139375,#139376,#139377,#139378,
#139379,#139380,#139381,#139382,#139383,#139384,#139385,#139386,#139387,
#139388,#139389,#139390,#139391,#139392,#139393,#139394,#139395,#139396,
#139397,#139398,#139399,#139400,#139401,#139402,#139403,#139404,#139405,
#139406,#139407,#139408,#139409,#139410,#139411,#139412,#139413,#139414,
#139415,#139416,#139417,#139418,#139419,#139420,#139421,#139422,#139423,
#139424,#139425,#139426,#139427,#139428,#139429,#139430,#139431,#139432,
#139433,#139434,#139435,#139436,#139437,#139438,#139439,#139440,#139441,
#139442,#139443,#139444,#139445,#139446,#139447,#139448,#139449,#139450,
#139451,#139452,#139453,#139454,#139455,#139456,#139457,#139458,#139459,
#139460,#139461,#139462,#139463,#139464,#139465,#139466,#139467,#139468,
#139469,#139470,#139471,#139472,#139473,#139474,#139475,#139476,#139477,
#139478,#139479,#139480,#139481,#139482,#139483,#139484,#139485,#139486,
#139487,#139488,#139489,#139490,#139491,#139492,#139493,#139494,#139495,
#139496,#139497,#139498,#139499,#139500,#139501,#139502,#139503,#139504,
#139505,#139506,#139507,#139508,#139509,#139510,#139511,#139512,#139513,
#139514,#139515,#139516,#139517,#139518,#139519,#139520,#139521,#139522,
#139523,#139524,#139525,#139526,#139527,#139528,#139529,#139530,#139531,
#139532,#139533,#139534,#139535,#139536,#139537,#139538,#139539,#139540,
#139541,#139542,#139543,#139544,#139545,#139546,#139547,#139548,#139549,
#139550,#139551,#139552,#139553,#139554,#139555,#139556,#139557,#139558,
#139559,#139560,#139561,#139562,#139563,#139564,#139565,#139566,#139567,
#139568,#139569,#139570,#139571,#139572,#139573,#139574,#139575,#139576,
#139577,#139578,#139579,#139580,#139581,#139582,#139583,#139584,#139585,
#139586,#139587,#139588,#139589,#139590,#139591,#139592,#139593,#139594,
#139595,#139596,#139597,#139598,#139599,#139600,#139601,#139602,#139603,
#139604,#139605,#139606,#139607,#139608,#139609,#139610,#139611,#139612,
#139613,#139614,#139615,#139616,#139617,#139618,#139619,#139620,#139621,
#139622,#139623,#139624,#139625,#139626,#139627,#139628,#139629,#139630,
#139631,#139632,#139633,#139634,#139635,#139636,#139637,#139638,#139639,
#139640,#139641,#139642,#139643,#139644,#139645,#139646,#139647,#139648,
#139649,#139650,#139651,#139652,#139653,#139654,#139655,#139656,#139657,
#139658,#139659,#139660,#139661,#139662,#139663,#139664,#139665,#139666,
#139667,#139668,#139669,#139670,#139671,#139672,#139673,#139674,#139675,
#139676,#139677,#139678,#139679,#139680,#139681,#139682,#139683,#139684,
#139685,#139686,#139687,#139688,#139689,#139690,#139691,#139692,#139693,
#139694,#139695,#139696,#139697,#139698,#139699,#139700,#139701,#139702,
#139703,#139704,#139705,#139706,#139707,#139708,#139709,#139710,#139711,
#139712,#139713,#139714,#139715,#139716,#139717,#139718,#139719,#139720,
#139721,#139722,#139723,#139724,#139725,#139726,#139727,#139728,#139729,
#139730,#139731,#139732,#139733,#139734,#139735,#139736,#139737,#139738,
#139739,#139740,#139741,#139742,#139743,#139744,#139745,#139746,#139747,
#139748,#139749,#139750,#139751,#139752,#139753,#139754,#139755,#139756,
#139757,#139758,#139759,#139760,#139761,#139762,#139763,#139764,#139765,
#139766,#139767,#139768,#139769,#139770,#139771,#139772,#139773,#139774,
#139775,#139776,#139777,#139778,#139779,#139780,#139781,#139782,#139783,
#139784,#139785,#139786,#139787,#139788,#139789,#139790,#139791,#139792,
#139793,#139794,#139795,#139796,#139797,#139798,#139799,#139800,#139801,
#139802,#139803,#139804,#139805,#139806,#139807,#139808,#139809,#139810,
#139811,#139812,#139813,#139814,#139815,#139816,#139817,#139818,#139819,
#139820,#139821,#139822,#139823,#139824,#139825,#139826,#139827,#139828,
#139829,#139830,#139831,#139832,#139833,#139834,#139835,#139836,#139837,
#139838,#139839,#139840,#139841,#139842,#139843,#139844,#139845,#139846,
#139847,#139848,#139849,#139850,#139851,#139852,#139853,#139854,#139855,
#139856,#139857,#139858,#139859,#139860,#139861,#139862,#139863,#139864,
#139865,#139866,#139867,#139868,#139869,#139870,#139871,#139872,#139873,
#139874,#139875,#139876,#139877,#139878,#139879,#139880,#139881,#139882,
#139883,#139884,#139885,#139886,#139887,#139888,#139889,#139890,#139891,
#139892,#139893,#139894,#139895,#139896,#139897,#139898,#139899,#139900,
#139901,#139902,#139903,#139904,#139905,#139906,#139907,#139908,#139909,
#139910,#139911,#139912,#139913,#139914,#139915,#139916,#139917,#139918,
#139919,#139920,#139921,#139922,#139923,#139924,#139925,#139926,#139927,
#139928,#139929,#139930,#139931,#139932,#139933,#139934,#139935,#139936,
#139937,#139938,#139939,#139940,#139941,#139942,#139943,#139944,#139945,
#139946,#139947,#139948,#139949,#139950,#139951,#139952,#139953,#139954,
#139955,#139956,#139957,#139958,#139959,#139960,#139961,#139962,#139963,
#139964,#139965,#139966,#139967,#139968,#139969,#139970,#139971,#139972,
#139973,#139974,#139975,#139976,#139977,#139978,#139979,#139980,#139981,
#139982,#139983,#139984,#139985,#139986,#139987,#139988,#139989,#139990,
#139991,#139992,#139993,#139994,#139995,#139996,#139997,#139998,#139999,
#140000,#140001,#140002,#140003,#140004,#140005,#140006,#140007,#140008,
#140009,#140010,#140011,#140012,#140013,#140014,#140015,#140016,#140017,
#140018,#140019,#140020,#140021,#140022,#140023,#140024,#140025,#140026,
#140027,#140028,#140029,#140030,#140031,#140032,#140033,#140034,#140035,
#140036,#140037,#140038,#140039,#140040,#140041,#140042,#140043,#140044,
#140045,#140046,#140047,#140048,#140049,#140050,#140051,#140052,#140053,
#140054,#140055,#140056,#140057,#140058,#140059,#140060,#140061,#140062,
#140063,#140064,#140065,#140066,#140067,#140068,#140069,#140070,#140071,
#140072,#140073,#140074,#140075,#140076,#140077,#140078,#140079,#140080,
#140081,#140082,#140083,#140084,#140085,#140086,#140087,#140088,#140089,
#140090,#140091,#140092,#140093,#140094,#140095,#140096,#140097,#140098,
#140099,#140100,#140101,#140102,#140103,#140104,#140105,#140106,#140107,
#140108,#140109,#140110,#140111,#140112,#140113,#140114,#140115,#140116,
#140117,#140118,#140119,#140120,#140121,#140122,#140123,#140124,#140125,
#140126,#140127,#140128,#140129,#140130,#140131,#140132,#140133,#140134,
#140135,#140136,#140137,#140138,#140139,#140140,#140141,#140142,#140143,
#140144,#140145,#140146,#140147,#140148,#140149,#140150,#140151,#140152,
#140153,#140154,#140155,#140156,#140157,#140158,#140159,#140160,#140161,
#140162,#140163,#140164,#140165,#140166,#140167,#140168,#140169,#140170,
#140171,#140172,#140173,#140174,#140175,#140176,#140177,#140178,#140179,
#140180,#140181,#140182,#140183,#140184,#140185,#140186,#140187,#140188,
#140189,#140190,#140191,#140192,#140193,#140194,#140195,#140196,#140197,
#140198,#140199,#140200,#140201,#140202,#140203,#140204,#140205,#140206,
#140207,#140208,#140209,#140210,#140211,#140212,#140213,#140214,#140215,
#140216,#140217,#140218,#140219,#140220,#140221,#140222,#140223,#140224,
#140225,#140226,#140227,#140228,#140229,#140230,#140231,#140232,#140233,
#140234,#140235,#140236,#140237,#140238,#140239,#140240,#140241,#140242,
#140243,#140244,#140245,#140246,#140247,#140248,#140249,#140250,#140251,
#140252,#140253,#140254,#140255,#140256,#140257,#140258,#140259,#140260,
#140261,#140262,#140263,#140264,#140265,#140266,#140267,#140268,#140269,
#140270,#140271,#140272,#140273,#140274,#140275,#140276,#140277,#140278,
#140279,#140280,#140281,#140282,#140283,#140284,#140285,#140286,#140287,
#140288,#140289,#140290,#140291,#140292,#140293,#140294,#140295,#140296,
#140297,#140298,#140299,#140300,#140301,#140302,#140303,#140304,#140305,
#140306,#140307,#140308,#140309,#140310,#140311,#140312,#140313,#140314,
#140315,#140316,#140317,#140318,#140319,#140320,#140321,#140322,#140323,
#140324,#140325,#140326,#140327,#140328,#140329,#140330,#140331,#140332,
#140333,#140334,#140335,#140336,#140337,#140338,#140339,#140340,#140341,
#140342,#140343,#140344,#140345,#140346,#140347,#140348,#140349,#140350,
#140351,#140352,#140353,#140354,#140355,#140356,#140357,#140358,#140359,
#140360,#140361,#140362,#140363,#140364,#140365,#140366,#140367,#140368,
#140369,#140370,#140371,#140372,#140373,#140374,#140375,#140376,#140377,
#140378,#140379,#140380,#140381,#140382,#140383,#140384,#140385,#140386,
#140387,#140388,#140389,#140390,#140391,#140392,#140393,#140394,#140395,
#140396,#140397,#140398,#140399,#140400,#140401,#140402,#140403,#140404,
#140405,#140406,#140407,#140408,#140409,#140410,#140411,#140412,#140413,
#140414,#140415,#140416,#140417,#140418,#140419,#140420,#140421,#140422,
#140423,#140424,#140425,#140426,#140427,#140428,#140429,#140430,#140431,
#140432,#140433,#140434,#140435,#140436,#140437,#140438,#140439,#140440,
#140441,#140442,#140443,#140444,#140445,#140446,#140447,#140448,#140449,
#140450,#140451,#140452,#140453,#140454,#140455,#140456,#140457,#140458,
#140459,#140460,#140461,#140462,#140463,#140464,#140465,#140466,#140467,
#140468,#140469,#140470,#140471,#140472,#140473,#140474,#140475,#140476,
#140477,#140478,#140479,#140480,#140481,#140482,#140483,#140484,#140485,
#140486,#140487,#140488,#140489,#140490,#140491,#140492,#140493,#140494,
#140495,#140496,#140497,#140498,#140499,#140500,#140501,#140502,#140503,
#140504,#140505,#140506,#140507,#140508,#140509,#140510,#140511,#140512,
#140513,#140514,#140515,#140516,#140517,#140518,#140519,#140520,#140521),
(#140522,#140523,#140524,#140525,#140526,#140527,#140528,#140529,#140530,
#140531,#140532,#140533,#140534,#140535,#140536,#140537,#140538,#140539,
#140540,#140541,#140542,#140543,#140544,#140545,#140546,#140547,#140548,
#140549,#140550,#140551,#140552,#140553,#140554,#140555,#140556,#140557,
#140558,#140559,#140560,#140561,#140562,#140563,#140564,#140565,#140566,
#140567,#140568,#140569,#140570,#140571,#140572,#140573,#140574,#140575,
#140576,#140577,#140578,#140579,#140580,#140581,#140582,#140583,#140584,
#140585,#140586,#140587,#140588,#140589,#140590,#140591,#140592,#140593,
#140594,#140595,#140596,#140597,#140598,#140599,#140600,#140601,#140602,
#140603,#140604,#140605,#140606,#140607,#140608,#140609,#140610,#140611,
#140612,#140613,#140614,#140615,#140616,#140617,#140618,#140619,#140620,
#140621,#140622,#140623,#140624,#140625,#140626,#140627,#140628,#140629,
#140630,#140631,#140632,#140633,#140634,#140635,#140636,#140637,#140638,
#140639,#140640,#140641,#140642,#140643,#140644,#140645,#140646,#140647,
#140648,#140649,#140650,#140651,#140652,#140653,#140654,#140655,#140656,
#140657,#140658,#140659,#140660,#140661,#140662,#140663,#140664,#140665,
#140666,#140667,#140668,#140669,#140670,#140671,#140672,#140673,#140674,
#140675,#140676,#140677,#140678,#140679,#140680,#140681,#140682,#140683,
#140684,#140685,#140686,#140687,#140688,#140689,#140690,#140691,#140692,
#140693,#140694,#140695,#140696,#140697,#140698,#140699,#140700,#140701,
#140702,#140703,#140704,#140705,#140706,#140707,#140708,#140709,#140710,
#140711,#140712,#140713,#140714,#140715,#140716,#140717,#140718,#140719,
#140720,#140721,#140722,#140723,#140724,#140725,#140726,#140727,#140728,
#140729,#140730,#140731,#140732,#140733,#140734,#140735,#140736,#140737,
#140738,#140739,#140740,#140741,#140742,#140743,#140744,#140745,#140746,
#140747,#140748,#140749,#140750,#140751,#140752,#140753,#140754,#140755,
#140756,#140757,#140758,#140759,#140760,#140761,#140762,#140763,#140764,
#140765,#140766,#140767,#140768,#140769,#140770,#140771,#140772,#140773,
#140774,#140775,#140776,#140777,#140778,#140779,#140780,#140781,#140782,
#140783,#140784,#140785,#140786,#140787,#140788,#140789,#140790,#140791,
#140792,#140793,#140794,#140795,#140796,#140797,#140798,#140799,#140800,
#140801,#140802,#140803,#140804,#140805,#140806,#140807,#140808,#140809,
#140810,#140811,#140812,#140813,#140814,#140815,#140816,#140817,#140818,
#140819,#140820,#140821,#140822,#140823,#140824,#140825,#140826,#140827,
#140828,#140829,#140830,#140831,#140832,#140833,#140834,#140835,#140836,
#140837,#140838,#140839,#140840,#140841,#140842,#140843,#140844,#140845,
#140846,#140847,#140848,#140849,#140850,#140851,#140852,#140853,#140854,
#140855,#140856,#140857,#140858,#140859,#140860,#140861,#140862,#140863,
#140864,#140865,#140866,#140867,#140868,#140869,#140870,#140871,#140872,
#140873,#140874,#140875,#140876,#140877,#140878,#140879,#140880,#140881,
#140882,#140883,#140884,#140885,#140886,#140887,#140888,#140889,#140890,
#140891,#140892,#140893,#140894,#140895,#140896,#140897,#140898,#140899,
#140900,#140901,#140902,#140903,#140904,#140905,#140906,#140907,#140908,
#140909,#140910,#140911,#140912,#140913,#140914,#140915,#140916,#140917,
#140918,#140919,#140920,#140921,#140922,#140923,#140924,#140925,#140926,
#140927,#140928,#140929,#140930,#140931,#140932,#140933,#140934,#140935,
#140936,#140937,#140938,#140939,#140940,#140941,#140942,#140943,#140944,
#140945,#140946,#140947,#140948,#140949,#140950,#140951,#140952,#140953,
#140954,#140955,#140956,#140957,#140958,#140959,#140960,#140961,#140962,
#140963,#140964,#140965,#140966,#140967,#140968,#140969,#140970,#140971,
#140972,#140973,#140974,#140975,#140976,#140977,#140978,#140979,#140980,
#140981,#140982,#140983,#140984,#140985,#140986,#140987,#140988,#140989,
#140990,#140991,#140992,#140993,#140994,#140995,#140996,#140997,#140998,
#140999,#141000,#141001,#141002,#141003,#141004,#141005,#141006,#141007,
#141008,#141009,#141010,#141011,#141012,#141013,#141014,#141015,#141016,
#141017,#141018,#141019,#141020,#141021,#141022,#141023,#141024,#141025,
#141026,#141027,#141028,#141029,#141030,#141031,#141032,#141033,#141034,
#141035,#141036,#141037,#141038,#141039,#141040,#141041,#141042,#141043,
#141044,#141045,#141046,#141047,#141048,#141049,#141050,#141051,#141052,
#141053,#141054,#141055,#141056,#141057,#141058,#141059,#141060,#141061,
#141062,#141063,#141064,#141065,#141066,#141067,#141068,#141069,#141070,
#141071,#141072,#141073,#141074,#141075,#141076,#141077,#141078,#141079,
#141080,#141081,#141082,#141083,#141084,#141085,#141086,#141087,#141088,
#141089,#141090,#141091,#141092,#141093,#141094,#141095,#141096,#141097,
#141098,#141099,#141100,#141101,#141102,#141103,#141104,#141105,#141106,
#141107,#141108,#141109,#141110,#141111,#141112,#141113,#141114,#141115,
#141116,#141117,#141118,#141119,#141120,#141121,#141122,#141123,#141124,
#141125,#141126,#141127,#141128,#141129,#141130,#141131,#141132,#141133,
#141134,#141135,#141136,#141137,#141138,#141139,#141140,#141141,#141142,
#141143,#141144,#141145,#141146,#141147,#141148,#141149,#141150,#141151,
#141152,#141153,#141154,#141155,#141156,#141157,#141158,#141159,#141160,
#141161,#141162,#141163,#141164,#141165,#141166,#141167,#141168,#141169,
#141170,#141171,#141172,#141173,#141174,#141175,#141176,#141177,#141178,
#141179,#141180,#141181,#141182,#141183,#141184,#141185,#141186,#141187,
#141188,#141189,#141190,#141191,#141192,#141193,#141194,#141195,#141196,
#141197,#141198,#141199,#141200,#141201,#141202,#141203,#141204,#141205,
#141206,#141207,#141208,#141209,#141210,#141211,#141212,#141213,#141214,
#141215,#141216,#141217,#141218,#141219,#141220,#141221,#141222,#141223,
#141224,#141225,#141226,#141227,#141228,#141229,#141230,#141231,#141232,
#141233,#141234,#141235,#141236,#141237,#141238,#141239,#141240,#141241,
#141242,#141243,#141244,#141245,#141246,#141247,#141248,#141249,#141250,
#141251,#141252,#141253,#141254,#141255,#141256,#141257,#141258,#141259,
#141260,#141261,#141262,#141263,#141264,#141265,#141266,#141267,#141268,
#141269,#141270,#141271,#141272,#141273,#141274,#141275,#141276,#141277,
#141278,#141279,#141280,#141281,#141282,#141283,#141284,#141285,#141286,
#141287,#141288,#141289,#141290,#141291,#141292,#141293,#141294,#141295,
#141296,#141297,#141298,#141299,#141300,#141301,#141302,#141303,#141304,
#141305,#141306,#141307,#141308,#141309,#141310,#141311,#141312,#141313,
#141314,#141315,#141316,#141317,#141318,#141319,#141320,#141321,#141322,
#141323,#141324,#141325,#141326,#141327,#141328,#141329,#141330,#141331,
#141332,#141333,#141334,#141335,#141336,#141337,#141338,#141339,#141340,
#141341,#141342,#141343,#141344,#141345,#141346,#141347,#141348,#141349,
#141350,#141351,#141352,#141353,#141354,#141355,#141356,#141357,#141358,
#141359,#141360,#141361,#141362,#141363,#141364,#141365,#141366,#141367,
#141368,#141369,#141370,#141371,#141372,#141373,#141374,#141375,#141376,
#141377,#141378,#141379,#141380,#141381,#141382,#141383,#141384,#141385,
#141386,#141387,#141388,#141389,#141390,#141391,#141392,#141393,#141394,
#141395,#141396,#141397,#141398,#141399,#141400,#141401,#141402,#141403,
#141404,#141405,#141406,#141407,#141408,#141409,#141410,#141411,#141412,
#141413,#141414,#141415,#141416,#141417,#141418,#141419,#141420,#141421,
#141422,#141423,#141424,#141425,#141426,#141427,#141428,#141429,#141430,
#141431,#141432,#141433,#141434,#141435,#141436,#141437,#141438,#141439,
#141440,#141441,#141442,#141443,#141444,#141445,#141446,#141447,#141448,
#141449,#141450,#141451,#141452,#141453,#141454,#141455,#141456,#141457,
#141458,#141459,#141460,#141461,#141462,#141463,#141464,#141465,#141466,
#141467,#141468,#141469,#141470,#141471,#141472,#141473,#141474,#141475,
#141476,#141477,#141478,#141479,#141480,#141481,#141482,#141483,#141484,
#141485,#141486,#141487,#141488,#141489,#141490,#141491,#141492,#141493,
#141494,#141495,#141496,#141497,#141498,#141499,#141500,#141501,#141502,
#141503,#141504,#141505,#141506,#141507,#141508,#141509,#141510,#141511,
#141512,#141513,#141514,#141515,#141516,#141517,#141518,#141519,#141520,
#141521,#141522,#141523,#141524,#141525,#141526,#141527,#141528,#141529,
#141530,#141531,#141532,#141533,#141534,#141535,#141536,#141537,#141538,
#141539,#141540,#141541,#141542,#141543,#141544,#141545,#141546,#141547,
#141548,#141549,#141550,#141551,#141552,#141553,#141554,#141555,#141556,
#141557,#141558,#141559,#141560,#141561,#141562,#141563,#141564,#141565,
#141566,#141567,#141568,#141569,#141570,#141571,#141572,#141573,#141574,
#141575,#141576,#141577,#141578,#141579,#141580,#141581,#141582,#141583,
#141584,#141585,#141586,#141587,#141588,#141589,#141590,#141591,#141592,
#141593,#141594,#141595,#141596,#141597,#141598,#141599,#141600,#141601,
#141602,#141603,#141604,#141605,#141606,#141607,#141608,#141609,#141610,
#141611,#141612,#141613,#141614,#141615,#141616,#141617,#141618,#141619,
#141620,#141621,#141622,#141623,#141624,#141625,#141626,#141627,#141628,
#141629,#141630,#141631,#141632,#141633,#141634,#141635,#141636,#141637,
#141638,#141639,#141640,#141641,#141642,#141643,#141644,#141645,#141646,
#141647,#141648,#141649,#141650,#141651,#141652,#141653,#141654,#141655,
#141656,#141657,#141658,#141659,#141660,#141661,#141662,#141663,#141664,
#141665,#141666,#141667,#141668,#141669,#141670,#141671,#141672,#141673,
#141674,#141675,#141676,#141677,#141678,#141679,#141680,#141681,#141682,
#141683,#141684,#141685,#141686,#141687,#141688,#141689,#141690,#141691,
#141692,#141693,#141694,#141695,#141696,#141697,#141698,#141699,#141700,
#141701,#141702,#141703,#141704,#141705,#141706,#141707,#141708,#141709,
#141710,#141711,#141712,#141713,#141714,#141715,#141716,#141717,#141718,
#141719,#141720,#141721,#141722,#141723,#141724,#141725,#141726,#141727,
#141728,#141729,#141730,#141731,#141732,#141733,#141734,#141735,#141736,
#141737,#141738,#141739,#141740,#141741,#141742,#141743,#141744,#141745,
#141746,#141747,#141748,#141749,#141750,#141751,#141752,#141753,#141754,
#141755,#141756,#141757,#141758,#141759,#141760,#141761,#141762,#141763,
#141764,#141765,#141766,#141767,#141768,#141769,#141770,#141771,#141772,
#141773,#141774,#141775,#141776,#141777,#141778,#141779,#141780,#141781,
#141782,#141783,#141784,#141785,#141786,#141787,#141788,#141789,#141790,
#141791,#141792,#141793,#141794,#141795,#141796,#141797,#141798,#141799,
#141800,#141801,#141802,#141803,#141804,#141805,#141806,#141807,#141808,
#141809,#141810,#141811,#141812,#141813,#141814,#141815,#141816,#141817,
#141818,#141819,#141820,#141821,#141822,#141823,#141824,#141825,#141826,
#141827,#141828,#141829,#141830,#141831,#141832,#141833,#141834,#141835,
#141836,#141837,#141838,#141839,#141840,#141841,#141842,#141843,#141844,
#141845,#141846,#141847,#141848,#141849,#141850,#141851,#141852,#141853,
#141854,#141855,#141856,#141857,#141858,#141859,#141860,#141861,#141862,
#141863,#141864,#141865,#141866,#141867,#141868,#141869,#141870,#141871,
#141872,#141873,#141874,#141875,#141876,#141877,#141878,#141879,#141880,
#141881,#141882,#141883,#141884,#141885,#141886,#141887,#141888,#141889,
#141890,#141891,#141892,#141893,#141894,#141895,#141896,#141897,#141898,
#141899,#141900,#141901,#141902,#141903,#141904,#141905,#141906,#141907,
#141908,#141909,#141910,#141911,#141912,#141913,#141914,#141915,#141916,
#141917,#141918,#141919,#141920,#141921,#141922,#141923,#141924,#141925,
#141926,#141927,#141928,#141929,#141930,#141931,#141932,#141933,#141934,
#141935,#141936,#141937,#141938,#141939,#141940,#141941,#141942,#141943,
#141944,#141945,#141946,#141947,#141948,#141949,#141950,#141951,#141952,
#141953,#141954,#141955,#141956,#141957,#141958,#141959,#141960,#141961,
#141962,#141963,#141964,#141965,#141966,#141967,#141968,#141969,#141970,
#141971,#141972,#141973,#141974,#141975,#141976,#141977,#141978,#141979,
#141980,#141981,#141982,#141983,#141984,#141985,#141986,#141987,#141988,
#141989,#141990,#141991,#141992,#141993,#141994,#141995,#141996,#141997,
#141998,#141999,#142000,#142001,#142002,#142003,#142004,#142005,#142006,
#142007,#142008,#142009,#142010,#142011,#142012,#142013,#142014,#142015,
#142016,#142017,#142018,#142019,#142020,#142021,#142022,#142023,#142024,
#142025,#142026,#142027,#142028,#142029,#142030,#142031,#142032,#142033,
#142034,#142035,#142036,#142037,#142038,#142039,#142040,#142041,#142042,
#142043,#142044,#142045,#142046,#142047,#142048,#142049,#142050,#142051,
#142052,#142053,#142054,#142055,#142056,#142057,#142058,#142059,#142060,
#142061,#142062,#142063,#142064,#142065,#142066,#142067,#142068,#142069,
#142070,#142071,#142072,#142073,#142074,#142075,#142076,#142077,#142078,
#142079,#142080,#142081,#142082,#142083,#142084,#142085,#142086,#142087,
#142088,#142089,#142090,#142091,#142092,#142093,#142094,#142095,#142096,
#142097,#142098,#142099,#142100,#142101,#142102,#142103,#142104,#142105,
#142106,#142107,#142108,#142109,#142110,#142111,#142112,#142113,#142114,
#142115,#142116,#142117,#142118,#142119,#142120,#142121,#142122,#142123,
#142124,#142125,#142126,#142127,#142128,#142129,#142130,#142131,#142132,
#142133,#142134,#142135,#142136,#142137,#142138,#142139,#142140,#142141,
#142142,#142143,#142144,#142145,#142146,#142147,#142148,#142149,#142150,
#142151,#142152,#142153,#142154,#142155,#142156,#142157,#142158,#142159,
#142160,#142161,#142162,#142163,#142164,#142165,#142166,#142167,#142168,
#142169,#142170,#142171,#142172,#142173,#142174,#142175,#142176,#142177,
#142178,#142179,#142180,#142181,#142182,#142183,#142184,#142185,#142186,
#142187,#142188,#142189,#142190,#142191,#142192,#142193,#142194,#142195,
#142196,#142197,#142198,#142199,#142200,#142201,#142202,#142203,#142204,
#142205,#142206,#142207,#142208,#142209,#142210,#142211,#142212,#142213,
#142214,#142215,#142216,#142217,#142218,#142219,#142220,#142221,#142222,
#142223,#142224,#142225,#142226,#142227,#142228,#142229,#142230,#142231,
#142232,#142233,#142234,#142235,#142236,#142237,#142238,#142239,#142240,
#142241,#142242,#142243,#142244,#142245,#142246,#142247,#142248,#142249,
#142250,#142251,#142252,#142253,#142254,#142255,#142256,#142257,#142258,
#142259,#142260,#142261,#142262,#142263,#142264,#142265,#142266,#142267,
#142268,#142269,#142270,#142271,#142272,#142273,#142274,#142275,#142276,
#142277,#142278,#142279,#142280,#142281,#142282,#142283,#142284,#142285,
#142286,#142287,#142288,#142289,#142290,#142291,#142292,#142293,#142294,
#142295,#142296,#142297,#142298,#142299,#142300,#142301,#142302,#142303,
#142304,#142305,#142306,#142307,#142308,#142309,#142310,#142311,#142312,
#142313,#142314,#142315,#142316,#142317,#142318,#142319,#142320,#142321,
#142322,#142323,#142324,#142325,#142326,#142327,#142328,#142329,#142330,
#142331,#142332,#142333,#142334,#142335,#142336,#142337,#142338,#142339,
#142340,#142341,#142342,#142343,#142344,#142345,#142346,#142347,#142348,
#142349,#142350,#142351,#142352,#142353,#142354,#142355,#142356,#142357,
#142358,#142359,#142360,#142361,#142362,#142363,#142364,#142365,#142366,
#142367,#142368,#142369,#142370,#142371,#142372,#142373,#142374,#142375,
#142376,#142377,#142378,#142379,#142380,#142381,#142382,#142383,#142384,
#142385,#142386,#142387,#142388,#142389,#142390,#142391,#142392,#142393,
#142394,#142395,#142396,#142397,#142398,#142399,#142400,#142401,#142402,
#142403,#142404,#142405,#142406,#142407,#142408,#142409,#142410,#142411,
#142412,#142413,#142414,#142415,#142416,#142417,#142418,#142419,#142420,
#142421,#142422,#142423,#142424,#142425,#142426,#142427,#142428,#142429,
#142430,#142431,#142432,#142433,#142434,#142435,#142436,#142437,#142438,
#142439,#142440,#142441,#142442,#142443,#142444,#142445,#142446,#142447,
#142448,#142449,#142450,#142451,#142452,#142453,#142454,#142455,#142456,
#142457,#142458,#142459,#142460,#142461,#142462,#142463,#142464,#142465,
#142466,#142467,#142468,#142469,#142470,#142471,#142472,#142473,#142474,
#142475,#142476,#142477,#142478,#142479,#142480,#142481,#142482,#142483,
#142484,#142485,#142486,#142487,#142488,#142489,#142490,#142491,#142492,
#142493,#142494,#142495,#142496,#142497,#142498,#142499,#142500,#142501,
#142502,#142503,#142504,#142505,#142506,#142507,#142508,#142509,#142510,
#142511,#142512,#142513,#142514,#142515,#142516,#142517,#142518,#142519,
#142520,#142521,#142522,#142523,#142524,#142525,#142526,#142527,#142528,
#142529,#142530,#142531,#142532,#142533,#142534,#142535,#142536,#142537,
#142538,#142539,#142540,#142541,#142542,#142543,#142544,#142545,#142546,
#142547,#142548,#142549,#142550,#142551,#142552,#142553,#142554,#142555,
#142556,#142557,#142558,#142559,#142560,#142561,#142562,#142563,#142564,
#142565,#142566,#142567,#142568,#142569,#142570,#142571,#142572),(#142573,
#142574,#142575,#142576,#142577,#142578,#142579,#142580,#142581,#142582,
#142583,#142584,#142585,#142586,#142587,#142588,#142589,#142590,#142591,
#142592,#142593,#142594,#142595,#142596,#142597,#142598,#142599,#142600,
#142601,#142602,#142603,#142604,#142605,#142606,#142607,#142608,#142609,
#142610,#142611,#142612,#142613,#142614,#142615,#142616,#142617,#142618,
#142619,#142620,#142621,#142622,#142623,#142624,#142625,#142626,#142627,
#142628,#142629,#142630,#142631,#142632,#142633,#142634,#142635,#142636,
#142637,#142638,#142639,#142640,#142641,#142642,#142643,#142644,#142645,
#142646,#142647,#142648,#142649,#142650,#142651,#142652,#142653,#142654,
#142655,#142656,#142657,#142658,#142659,#142660,#142661,#142662,#142663,
#142664,#142665,#142666,#142667,#142668,#142669,#142670,#142671,#142672,
#142673,#142674,#142675,#142676,#142677,#142678,#142679,#142680,#142681,
#142682,#142683,#142684,#142685,#142686,#142687,#142688,#142689,#142690,
#142691,#142692,#142693,#142694,#142695,#142696,#142697,#142698,#142699,
#142700,#142701,#142702,#142703,#142704,#142705,#142706,#142707,#142708,
#142709,#142710,#142711,#142712,#142713,#142714,#142715,#142716,#142717,
#142718,#142719,#142720,#142721,#142722,#142723,#142724,#142725,#142726,
#142727,#142728,#142729,#142730,#142731,#142732,#142733,#142734,#142735,
#142736,#142737,#142738,#142739,#142740,#142741,#142742,#142743,#142744,
#142745,#142746,#142747,#142748,#142749,#142750,#142751,#142752,#142753,
#142754,#142755,#142756,#142757,#142758,#142759,#142760,#142761,#142762,
#142763,#142764,#142765,#142766,#142767,#142768,#142769,#142770,#142771,
#142772,#142773,#142774,#142775,#142776,#142777,#142778,#142779,#142780,
#142781,#142782,#142783,#142784,#142785,#142786,#142787,#142788,#142789,
#142790,#142791,#142792,#142793,#142794,#142795,#142796,#142797,#142798,
#142799,#142800,#142801,#142802,#142803,#142804,#142805,#142806,#142807,
#142808,#142809,#142810,#142811,#142812,#142813,#142814,#142815,#142816,
#142817,#142818,#142819,#142820,#142821,#142822,#142823,#142824,#142825,
#142826,#142827,#142828,#142829,#142830,#142831,#142832,#142833,#142834,
#142835,#142836,#142837,#142838,#142839,#142840,#142841,#142842,#142843,
#142844,#142845,#142846,#142847,#142848,#142849,#142850,#142851,#142852,
#142853,#142854,#142855,#142856,#142857,#142858,#142859,#142860,#142861,
#142862,#142863,#142864,#142865,#142866,#142867,#142868,#142869,#142870,
#142871,#142872,#142873,#142874,#142875,#142876,#142877,#142878,#142879,
#142880,#142881,#142882,#142883,#142884,#142885,#142886,#142887,#142888,
#142889,#142890,#142891,#142892,#142893,#142894,#142895,#142896,#142897,
#142898,#142899,#142900,#142901,#142902,#142903,#142904,#142905,#142906,
#142907,#142908,#142909,#142910,#142911,#142912,#142913,#142914,#142915,
#142916,#142917,#142918,#142919,#142920,#142921,#142922,#142923,#142924,
#142925,#142926,#142927,#142928,#142929,#142930,#142931,#142932,#142933,
#142934,#142935,#142936,#142937,#142938,#142939,#142940,#142941,#142942,
#142943,#142944,#142945,#142946,#142947,#142948,#142949,#142950,#142951,
#142952,#142953,#142954,#142955,#142956,#142957,#142958,#142959,#142960,
#142961,#142962,#142963,#142964,#142965,#142966,#142967,#142968,#142969,
#142970,#142971,#142972,#142973,#142974,#142975,#142976,#142977,#142978,
#142979,#142980,#142981,#142982,#142983,#142984,#142985,#142986,#142987,
#142988,#142989,#142990,#142991,#142992,#142993,#142994,#142995,#142996,
#142997,#142998,#142999,#143000,#143001,#143002,#143003,#143004,#143005,
#143006,#143007,#143008,#143009,#143010,#143011,#143012,#143013,#143014,
#143015,#143016,#143017,#143018,#143019,#143020,#143021,#143022,#143023,
#143024,#143025,#143026,#143027,#143028,#143029,#143030,#143031,#143032,
#143033,#143034,#143035,#143036,#143037,#143038,#143039,#143040,#143041,
#143042,#143043,#143044,#143045,#143046,#143047,#143048,#143049,#143050,
#143051,#143052,#143053,#143054,#143055,#143056,#143057,#143058,#143059,
#143060,#143061,#143062,#143063,#143064,#143065,#143066,#143067,#143068,
#143069,#143070,#143071,#143072,#143073,#143074,#143075,#143076,#143077,
#143078,#143079,#143080,#143081,#143082,#143083,#143084,#143085,#143086,
#143087,#143088,#143089,#143090,#143091,#143092,#143093,#143094,#143095,
#143096,#143097,#143098,#143099,#143100,#143101,#143102,#143103,#143104,
#143105,#143106,#143107,#143108,#143109,#143110,#143111,#143112,#143113,
#143114,#143115,#143116,#143117,#143118,#143119,#143120,#143121,#143122,
#143123,#143124,#143125,#143126,#143127,#143128,#143129,#143130,#143131,
#143132,#143133,#143134,#143135,#143136,#143137,#143138,#143139,#143140,
#143141,#143142,#143143,#143144,#143145,#143146,#143147,#143148,#143149,
#143150,#143151,#143152,#143153,#143154,#143155,#143156,#143157,#143158,
#143159,#143160,#143161,#143162,#143163,#143164,#143165,#143166,#143167,
#143168,#143169,#143170,#143171,#143172,#143173,#143174,#143175,#143176,
#143177,#143178,#143179,#143180,#143181,#143182,#143183,#143184,#143185,
#143186,#143187,#143188,#143189,#143190,#143191,#143192,#143193,#143194,
#143195,#143196,#143197,#143198,#143199,#143200,#143201,#143202,#143203,
#143204,#143205,#143206,#143207,#143208,#143209,#143210,#143211,#143212,
#143213,#143214,#143215,#143216,#143217,#143218,#143219,#143220,#143221,
#143222,#143223,#143224,#143225,#143226,#143227,#143228,#143229,#143230,
#143231,#143232,#143233,#143234,#143235,#143236,#143237,#143238,#143239,
#143240,#143241,#143242,#143243,#143244,#143245,#143246,#143247,#143248,
#143249,#143250,#143251,#143252,#143253,#143254,#143255,#143256,#143257,
#143258,#143259,#143260,#143261,#143262,#143263,#143264,#143265,#143266,
#143267,#143268,#143269,#143270,#143271,#143272,#143273,#143274,#143275,
#143276,#143277,#143278,#143279,#143280,#143281,#143282,#143283,#143284,
#143285,#143286,#143287,#143288,#143289,#143290,#143291,#143292,#143293,
#143294,#143295,#143296,#143297,#143298,#143299,#143300,#143301,#143302,
#143303,#143304,#143305,#143306,#143307,#143308,#143309,#143310,#143311,
#143312,#143313,#143314,#143315,#143316,#143317,#143318,#143319,#143320,
#143321,#143322,#143323,#143324,#143325,#143326,#143327,#143328,#143329,
#143330,#143331,#143332,#143333,#143334,#143335,#143336,#143337,#143338,
#143339,#143340,#143341,#143342,#143343,#143344,#143345,#143346,#143347,
#143348,#143349,#143350,#143351,#143352,#143353,#143354,#143355,#143356,
#143357,#143358,#143359,#143360,#143361,#143362,#143363,#143364,#143365,
#143366,#143367,#143368,#143369,#143370,#143371,#143372,#143373,#143374,
#143375,#143376,#143377,#143378,#143379,#143380,#143381,#143382,#143383,
#143384,#143385,#143386,#143387,#143388,#143389,#143390,#143391,#143392,
#143393,#143394,#143395,#143396,#143397,#143398,#143399,#143400,#143401,
#143402,#143403,#143404,#143405,#143406,#143407,#143408,#143409,#143410,
#143411,#143412,#143413,#143414,#143415,#143416,#143417,#143418,#143419,
#143420,#143421,#143422,#143423,#143424,#143425,#143426,#143427,#143428,
#143429,#143430,#143431,#143432,#143433,#143434,#143435,#143436,#143437,
#143438,#143439,#143440,#143441,#143442,#143443,#143444,#143445,#143446,
#143447,#143448,#143449,#143450,#143451,#143452,#143453,#143454,#143455,
#143456,#143457,#143458,#143459,#143460,#143461,#143462,#143463,#143464,
#143465,#143466,#143467,#143468,#143469,#143470,#143471,#143472,#143473,
#143474,#143475,#143476,#143477,#143478,#143479,#143480,#143481,#143482,
#143483,#143484,#143485,#143486,#143487,#143488,#143489,#143490,#143491,
#143492,#143493,#143494,#143495,#143496,#143497,#143498,#143499,#143500,
#143501,#143502,#143503,#143504,#143505,#143506,#143507,#143508,#143509,
#143510,#143511,#143512,#143513,#143514,#143515,#143516,#143517,#143518,
#143519,#143520,#143521,#143522,#143523,#143524,#143525,#143526,#143527,
#143528,#143529,#143530,#143531,#143532,#143533,#143534,#143535,#143536,
#143537,#143538,#143539,#143540,#143541,#143542,#143543,#143544,#143545,
#143546,#143547,#143548,#143549,#143550,#143551,#143552,#143553,#143554,
#143555,#143556,#143557,#143558,#143559,#143560,#143561,#143562,#143563,
#143564,#143565,#143566,#143567,#143568,#143569,#143570,#143571,#143572,
#143573,#143574,#143575,#143576,#143577,#143578,#143579,#143580,#143581,
#143582,#143583,#143584,#143585,#143586,#143587,#143588,#143589,#143590,
#143591,#143592,#143593,#143594,#143595,#143596,#143597,#143598,#143599,
#143600,#143601,#143602,#143603,#143604,#143605,#143606,#143607,#143608,
#143609,#143610,#143611,#143612,#143613,#143614,#143615,#143616,#143617,
#143618,#143619,#143620,#143621,#143622,#143623,#143624,#143625,#143626,
#143627,#143628,#143629,#143630,#143631,#143632,#143633,#143634,#143635,
#143636,#143637,#143638,#143639,#143640,#143641,#143642,#143643,#143644,
#143645,#143646,#143647,#143648,#143649,#143650,#143651,#143652,#143653,
#143654,#143655,#143656,#143657,#143658,#143659,#143660,#143661,#143662,
#143663,#143664,#143665,#143666,#143667,#143668,#143669,#143670,#143671,
#143672,#143673,#143674,#143675,#143676,#143677,#143678,#143679,#143680,
#143681,#143682,#143683,#143684,#143685,#143686,#143687,#143688,#143689,
#143690,#143691,#143692,#143693,#143694,#143695,#143696,#143697,#143698,
#143699,#143700,#143701,#143702,#143703,#143704,#143705,#143706,#143707,
#143708,#143709,#143710,#143711,#143712,#143713,#143714,#143715,#143716,
#143717,#143718,#143719,#143720,#143721,#143722,#143723,#143724,#143725,
#143726,#143727,#143728,#143729,#143730,#143731,#143732,#143733,#143734,
#143735,#143736,#143737,#143738,#143739,#143740,#143741,#143742,#143743,
#143744,#143745,#143746,#143747,#143748,#143749,#143750,#143751,#143752,
#143753,#143754,#143755,#143756,#143757,#143758,#143759,#143760,#143761,
#143762,#143763,#143764,#143765,#143766,#143767,#143768,#143769,#143770,
#143771,#143772,#143773,#143774,#143775,#143776,#143777,#143778,#143779,
#143780,#143781,#143782,#143783,#143784,#143785,#143786,#143787,#143788,
#143789,#143790,#143791,#143792,#143793,#143794,#143795,#143796,#143797,
#143798,#143799,#143800,#143801,#143802,#143803,#143804,#143805,#143806,
#143807,#143808,#143809,#143810,#143811,#143812,#143813,#143814,#143815,
#143816,#143817,#143818,#143819,#143820,#143821,#143822,#143823,#143824,
#143825,#143826,#143827,#143828,#143829,#143830,#143831,#143832,#143833,
#143834,#143835,#143836,#143837,#143838,#143839,#143840,#143841,#143842,
#143843,#143844,#143845,#143846,#143847,#143848,#143849,#143850,#143851,
#143852,#143853,#143854,#143855,#143856,#143857,#143858,#143859,#143860,
#143861,#143862,#143863,#143864,#143865,#143866,#143867,#143868,#143869,
#143870,#143871,#143872,#143873,#143874,#143875,#143876,#143877,#143878,
#143879,#143880,#143881,#143882,#143883,#143884,#143885,#143886,#143887,
#143888,#143889,#143890,#143891,#143892,#143893,#143894,#143895,#143896,
#143897,#143898,#143899,#143900,#143901,#143902,#143903,#143904,#143905,
#143906,#143907,#143908,#143909,#143910,#143911,#143912,#143913,#143914,
#143915,#143916,#143917,#143918,#143919,#143920,#143921,#143922,#143923,
#143924,#143925,#143926,#143927,#143928,#143929,#143930,#143931,#143932,
#143933,#143934,#143935,#143936,#143937,#143938,#143939,#143940,#143941,
#143942,#143943,#143944,#143945,#143946,#143947,#143948,#143949,#143950,
#143951,#143952,#143953,#143954,#143955,#143956,#143957,#143958,#143959,
#143960,#143961,#143962,#143963,#143964,#143965,#143966,#143967,#143968,
#143969,#143970,#143971,#143972,#143973,#143974,#143975,#143976,#143977,
#143978,#143979,#143980,#143981,#143982,#143983,#143984,#143985,#143986,
#143987,#143988,#143989,#143990,#143991,#143992,#143993,#143994,#143995,
#143996,#143997,#143998,#143999,#144000,#144001,#144002,#144003,#144004,
#144005,#144006,#144007,#144008,#144009,#144010,#144011,#144012,#144013,
#144014,#144015,#144016,#144017,#144018,#144019,#144020,#144021,#144022,
#144023,#144024,#144025,#144026,#144027,#144028,#144029,#144030,#144031,
#144032,#144033,#144034,#144035,#144036,#144037,#144038,#144039,#144040,
#144041,#144042,#144043,#144044,#144045,#144046,#144047,#144048,#144049,
#144050,#144051,#144052,#144053,#144054,#144055,#144056,#144057,#144058,
#144059,#144060,#144061,#144062,#144063,#144064,#144065,#144066,#144067,
#144068,#144069,#144070,#144071,#144072,#144073,#144074,#144075,#144076,
#144077,#144078,#144079,#144080,#144081,#144082,#144083,#144084,#144085,
#144086,#144087,#144088,#144089,#144090,#144091,#144092,#144093,#144094,
#144095,#144096,#144097,#144098,#144099,#144100,#144101,#144102,#144103,
#144104,#144105,#144106,#144107,#144108,#144109,#144110,#144111,#144112,
#144113,#144114,#144115,#144116,#144117,#144118,#144119,#144120,#144121,
#144122,#144123,#144124,#144125,#144126,#144127,#144128,#144129,#144130,
#144131,#144132,#144133,#144134,#144135,#144136,#144137,#144138,#144139,
#144140,#144141,#144142,#144143,#144144,#144145,#144146,#144147,#144148,
#144149,#144150,#144151,#144152,#144153,#144154,#144155,#144156,#144157,
#144158,#144159,#144160,#144161,#144162,#144163,#144164,#144165,#144166,
#144167,#144168,#144169,#144170,#144171,#144172,#144173,#144174,#144175,
#144176,#144177,#144178,#144179,#144180,#144181,#144182,#144183,#144184,
#144185,#144186,#144187,#144188,#144189,#144190,#144191,#144192,#144193,
#144194,#144195,#144196,#144197,#144198,#144199,#144200,#144201,#144202,
#144203,#144204,#144205,#144206,#144207,#144208,#144209,#144210,#144211,
#144212,#144213,#144214,#144215,#144216,#144217,#144218,#144219,#144220,
#144221,#144222,#144223,#144224,#144225,#144226,#144227,#144228,#144229,
#144230,#144231,#144232,#144233,#144234,#144235,#144236,#144237,#144238,
#144239,#144240,#144241,#144242,#144243,#144244,#144245,#144246,#144247,
#144248,#144249,#144250,#144251,#144252,#144253,#144254,#144255,#144256,
#144257,#144258,#144259,#144260,#144261,#144262,#144263,#144264,#144265,
#144266,#144267,#144268,#144269,#144270,#144271,#144272,#144273,#144274,
#144275,#144276,#144277,#144278,#144279,#144280,#144281,#144282,#144283,
#144284,#144285,#144286,#144287,#144288,#144289,#144290,#144291,#144292,
#144293,#144294,#144295,#144296,#144297,#144298,#144299,#144300,#144301,
#144302,#144303,#144304,#144305,#144306,#144307,#144308,#144309,#144310,
#144311,#144312,#144313,#144314,#144315,#144316,#144317,#144318,#144319,
#144320,#144321,#144322,#144323,#144324,#144325,#144326,#144327,#144328,
#144329,#144330,#144331,#144332,#144333,#144334,#144335,#144336,#144337,
#144338,#144339,#144340,#144341,#144342,#144343,#144344,#144345,#144346,
#144347,#144348,#144349,#144350,#144351,#144352,#144353,#144354,#144355,
#144356,#144357,#144358,#144359,#144360,#144361,#144362,#144363,#144364,
#144365,#144366,#144367,#144368,#144369,#144370,#144371,#144372,#144373,
#144374,#144375,#144376,#144377,#144378,#144379,#144380,#144381,#144382,
#144383,#144384,#144385,#144386,#144387,#144388,#144389,#144390,#144391,
#144392,#144393,#144394,#144395,#144396,#144397,#144398,#144399,#144400,
#144401,#144402,#144403,#144404,#144405,#144406,#144407,#144408,#144409,
#144410,#144411,#144412,#144413,#144414,#144415,#144416,#144417,#144418,
#144419,#144420,#144421,#144422,#144423,#144424,#144425,#144426,#144427,
#144428,#144429,#144430,#144431,#144432,#144433,#144434,#144435,#144436,
#144437,#144438,#144439,#144440,#144441,#144442,#144443,#144444,#144445,
#144446,#144447,#144448,#144449,#144450,#144451,#144452,#144453,#144454,
#144455,#144456,#144457,#144458,#144459,#144460,#144461,#144462,#144463,
#144464,#144465,#144466,#144467,#144468,#144469,#144470,#144471,#144472,
#144473,#144474,#144475,#144476,#144477,#144478,#144479,#144480,#144481,
#144482,#144483,#144484,#144485,#144486,#144487,#144488,#144489,#144490,
#144491,#144492,#144493,#144494,#144495,#144496,#144497,#144498,#144499,
#144500,#144501,#144502,#144503,#144504,#144505,#144506,#144507,#144508,
#144509,#144510,#144511,#144512,#144513,#144514,#144515,#144516,#144517,
#144518,#144519,#144520,#144521,#144522,#144523,#144524,#144525,#144526,
#144527,#144528,#144529,#144530,#144531,#144532,#144533,#144534,#144535,
#144536,#144537,#144538,#144539,#144540,#144541,#144542,#144543,#144544,
#144545,#144546,#144547,#144548,#144549,#144550,#144551,#144552,#144553,
#144554,#144555,#144556,#144557,#144558,#144559,#144560,#144561,#144562,
#144563,#144564,#144565,#144566,#144567,#144568,#144569,#144570,#144571,
#144572,#144573,#144574,#144575,#144576,#144577,#144578,#144579,#144580,
#144581,#144582,#144583,#144584,#144585,#144586,#144587,#144588,#144589,
#144590,#144591,#144592,#144593,#144594,#144595,#144596,#144597,#144598,
#144599,#144600,#144601,#144602,#144603,#144604,#144605,#144606,#144607,
#144608,#144609,#144610,#144611,#144612,#144613,#144614,#144615,#144616,
#144617,#144618,#144619,#144620,#144621,#144622,#144623),(#144624,#144625,
#144626,#144627,#144628,#144629,#144630,#144631,#144632,#144633,#144634,
#144635,#144636,#144637,#144638,#144639,#144640,#144641,#144642,#144643,
#144644,#144645,#144646,#144647,#144648,#144649,#144650,#144651,#144652,
#144653,#144654,#144655,#144656,#144657,#144658,#144659,#144660,#144661,
#144662,#144663,#144664,#144665,#144666,#144667,#144668,#144669,#144670,
#144671,#144672,#144673,#144674,#144675,#144676,#144677,#144678,#144679,
#144680,#144681,#144682,#144683,#144684,#144685,#144686,#144687,#144688,
#144689,#144690,#144691,#144692,#144693,#144694,#144695,#144696,#144697,
#144698,#144699,#144700,#144701,#144702,#144703,#144704,#144705,#144706,
#144707,#144708,#144709,#144710,#144711,#144712,#144713,#144714,#144715,
#144716,#144717,#144718,#144719,#144720,#144721,#144722,#144723,#144724,
#144725,#144726,#144727,#144728,#144729,#144730,#144731,#144732,#144733,
#144734,#144735,#144736,#144737,#144738,#144739,#144740,#144741,#144742,
#144743,#144744,#144745,#144746,#144747,#144748,#144749,#144750,#144751,
#144752,#144753,#144754,#144755,#144756,#144757,#144758,#144759,#144760,
#144761,#144762,#144763,#144764,#144765,#144766,#144767,#144768,#144769,
#144770,#144771,#144772,#144773,#144774,#144775,#144776,#144777,#144778,
#144779,#144780,#144781,#144782,#144783,#144784,#144785,#144786,#144787,
#144788,#144789,#144790,#144791,#144792,#144793,#144794,#144795,#144796,
#144797,#144798,#144799,#144800,#144801,#144802,#144803,#144804,#144805,
#144806,#144807,#144808,#144809,#144810,#144811,#144812,#144813,#144814,
#144815,#144816,#144817,#144818,#144819,#144820,#144821,#144822,#144823,
#144824,#144825,#144826,#144827,#144828,#144829,#144830,#144831,#144832,
#144833,#144834,#144835,#144836,#144837,#144838,#144839,#144840,#144841,
#144842,#144843,#144844,#144845,#144846,#144847,#144848,#144849,#144850,
#144851,#144852,#144853,#144854,#144855,#144856,#144857,#144858,#144859,
#144860,#144861,#144862,#144863,#144864,#144865,#144866,#144867,#144868,
#144869,#144870,#144871,#144872,#144873,#144874,#144875,#144876,#144877,
#144878,#144879,#144880,#144881,#144882,#144883,#144884,#144885,#144886,
#144887,#144888,#144889,#144890,#144891,#144892,#144893,#144894,#144895,
#144896,#144897,#144898,#144899,#144900,#144901,#144902,#144903,#144904,
#144905,#144906,#144907,#144908,#144909,#144910,#144911,#144912,#144913,
#144914,#144915,#144916,#144917,#144918,#144919,#144920,#144921,#144922,
#144923,#144924,#144925,#144926,#144927,#144928,#144929,#144930,#144931,
#144932,#144933,#144934,#144935,#144936,#144937,#144938,#144939,#144940,
#144941,#144942,#144943,#144944,#144945,#144946,#144947,#144948,#144949,
#144950,#144951,#144952,#144953,#144954,#144955,#144956,#144957,#144958,
#144959,#144960,#144961,#144962,#144963,#144964,#144965,#144966,#144967,
#144968,#144969,#144970,#144971,#144972,#144973,#144974,#144975,#144976,
#144977,#144978,#144979,#144980,#144981,#144982,#144983,#144984,#144985,
#144986,#144987,#144988,#144989,#144990,#144991,#144992,#144993,#144994,
#144995,#144996,#144997,#144998,#144999,#145000,#145001,#145002,#145003,
#145004,#145005,#145006,#145007,#145008,#145009,#145010,#145011,#145012,
#145013,#145014,#145015,#145016,#145017,#145018,#145019,#145020,#145021,
#145022,#145023,#145024,#145025,#145026,#145027,#145028,#145029,#145030,
#145031,#145032,#145033,#145034,#145035,#145036,#145037,#145038,#145039,
#145040,#145041,#145042,#145043,#145044,#145045,#145046,#145047,#145048,
#145049,#145050,#145051,#145052,#145053,#145054,#145055,#145056,#145057,
#145058,#145059,#145060,#145061,#145062,#145063,#145064,#145065,#145066,
#145067,#145068,#145069,#145070,#145071,#145072,#145073,#145074,#145075,
#145076,#145077,#145078,#145079,#145080,#145081,#145082,#145083,#145084,
#145085,#145086,#145087,#145088,#145089,#145090,#145091,#145092,#145093,
#145094,#145095,#145096,#145097,#145098,#145099,#145100,#145101,#145102,
#145103,#145104,#145105,#145106,#145107,#145108,#145109,#145110,#145111,
#145112,#145113,#145114,#145115,#145116,#145117,#145118,#145119,#145120,
#145121,#145122,#145123,#145124,#145125,#145126,#145127,#145128,#145129,
#145130,#145131,#145132,#145133,#145134,#145135,#145136,#145137,#145138,
#145139,#145140,#145141,#145142,#145143,#145144,#145145,#145146,#145147,
#145148,#145149,#145150,#145151,#145152,#145153,#145154,#145155,#145156,
#145157,#145158,#145159,#145160,#145161,#145162,#145163,#145164,#145165,
#145166,#145167,#145168,#145169,#145170,#145171,#145172,#145173,#145174,
#145175,#145176,#145177,#145178,#145179,#145180,#145181,#145182,#145183,
#145184,#145185,#145186,#145187,#145188,#145189,#145190,#145191,#145192,
#145193,#145194,#145195,#145196,#145197,#145198,#145199,#145200,#145201,
#145202,#145203,#145204,#145205,#145206,#145207,#145208,#145209,#145210,
#145211,#145212,#145213,#145214,#145215,#145216,#145217,#145218,#145219,
#145220,#145221,#145222,#145223,#145224,#145225,#145226,#145227,#145228,
#145229,#145230,#145231,#145232,#145233,#145234,#145235,#145236,#145237,
#145238,#145239,#145240,#145241,#145242,#145243,#145244,#145245,#145246,
#145247,#145248,#145249,#145250,#145251,#145252,#145253,#145254,#145255,
#145256,#145257,#145258,#145259,#145260,#145261,#145262,#145263,#145264,
#145265,#145266,#145267,#145268,#145269,#145270,#145271,#145272,#145273,
#145274,#145275,#145276,#145277,#145278,#145279,#145280,#145281,#145282,
#145283,#145284,#145285,#145286,#145287,#145288,#145289,#145290,#145291,
#145292,#145293,#145294,#145295,#145296,#145297,#145298,#145299,#145300,
#145301,#145302,#145303,#145304,#145305,#145306,#145307,#145308,#145309,
#145310,#145311,#145312,#145313,#145314,#145315,#145316,#145317,#145318,
#145319,#145320,#145321,#145322,#145323,#145324,#145325,#145326,#145327,
#145328,#145329,#145330,#145331,#145332,#145333,#145334,#145335,#145336,
#145337,#145338,#145339,#145340,#145341,#145342,#145343,#145344,#145345,
#145346,#145347,#145348,#145349,#145350,#145351,#145352,#145353,#145354,
#145355,#145356,#145357,#145358,#145359,#145360,#145361,#145362,#145363,
#145364,#145365,#145366,#145367,#145368,#145369,#145370,#145371,#145372,
#145373,#145374,#145375,#145376,#145377,#145378,#145379,#145380,#145381,
#145382,#145383,#145384,#145385,#145386,#145387,#145388,#145389,#145390,
#145391,#145392,#145393,#145394,#145395,#145396,#145397,#145398,#145399,
#145400,#145401,#145402,#145403,#145404,#145405,#145406,#145407,#145408,
#145409,#145410,#145411,#145412,#145413,#145414,#145415,#145416,#145417,
#145418,#145419,#145420,#145421,#145422,#145423,#145424,#145425,#145426,
#145427,#145428,#145429,#145430,#145431,#145432,#145433,#145434,#145435,
#145436,#145437,#145438,#145439,#145440,#145441,#145442,#145443,#145444,
#145445,#145446,#145447,#145448,#145449,#145450,#145451,#145452,#145453,
#145454,#145455,#145456,#145457,#145458,#145459,#145460,#145461,#145462,
#145463,#145464,#145465,#145466,#145467,#145468,#145469,#145470,#145471,
#145472,#145473,#145474,#145475,#145476,#145477,#145478,#145479,#145480,
#145481,#145482,#145483,#145484,#145485,#145486,#145487,#145488,#145489,
#145490,#145491,#145492,#145493,#145494,#145495,#145496,#145497,#145498,
#145499,#145500,#145501,#145502,#145503,#145504,#145505,#145506,#145507,
#145508,#145509,#145510,#145511,#145512,#145513,#145514,#145515,#145516,
#145517,#145518,#145519,#145520,#145521,#145522,#145523,#145524,#145525,
#145526,#145527,#145528,#145529,#145530,#145531,#145532,#145533,#145534,
#145535,#145536,#145537,#145538,#145539,#145540,#145541,#145542,#145543,
#145544,#145545,#145546,#145547,#145548,#145549,#145550,#145551,#145552,
#145553,#145554,#145555,#145556,#145557,#145558,#145559,#145560,#145561,
#145562,#145563,#145564,#145565,#145566,#145567,#145568,#145569,#145570,
#145571,#145572,#145573,#145574,#145575,#145576,#145577,#145578,#145579,
#145580,#145581,#145582,#145583,#145584,#145585,#145586,#145587,#145588,
#145589,#145590,#145591,#145592,#145593,#145594,#145595,#145596,#145597,
#145598,#145599,#145600,#145601,#145602,#145603,#145604,#145605,#145606,
#145607,#145608,#145609,#145610,#145611,#145612,#145613,#145614,#145615,
#145616,#145617,#145618,#145619,#145620,#145621,#145622,#145623,#145624,
#145625,#145626,#145627,#145628,#145629,#145630,#145631,#145632,#145633,
#145634,#145635,#145636,#145637,#145638,#145639,#145640,#145641,#145642,
#145643,#145644,#145645,#145646,#145647,#145648,#145649,#145650,#145651,
#145652,#145653,#145654,#145655,#145656,#145657,#145658,#145659,#145660,
#145661,#145662,#145663,#145664,#145665,#145666,#145667,#145668,#145669,
#145670,#145671,#145672,#145673,#145674,#145675,#145676,#145677,#145678,
#145679,#145680,#145681,#145682,#145683,#145684,#145685,#145686,#145687,
#145688,#145689,#145690,#145691,#145692,#145693,#145694,#145695,#145696,
#145697,#145698,#145699,#145700,#145701,#145702,#145703,#145704,#145705,
#145706,#145707,#145708,#145709,#145710,#145711,#145712,#145713,#145714,
#145715,#145716,#145717,#145718,#145719,#145720,#145721,#145722,#145723,
#145724,#145725,#145726,#145727,#145728,#145729,#145730,#145731,#145732,
#145733,#145734,#145735,#145736,#145737,#145738,#145739,#145740,#145741,
#145742,#145743,#145744,#145745,#145746,#145747,#145748,#145749,#145750,
#145751,#145752,#145753,#145754,#145755,#145756,#145757,#145758,#145759,
#145760,#145761,#145762,#145763,#145764,#145765,#145766,#145767,#145768,
#145769,#145770,#145771,#145772,#145773,#145774,#145775,#145776,#145777,
#145778,#145779,#145780,#145781,#145782,#145783,#145784,#145785,#145786,
#145787,#145788,#145789,#145790,#145791,#145792,#145793,#145794,#145795,
#145796,#145797,#145798,#145799,#145800,#145801,#145802,#145803,#145804,
#145805,#145806,#145807,#145808,#145809,#145810,#145811,#145812,#145813,
#145814,#145815,#145816,#145817,#145818,#145819,#145820,#145821,#145822,
#145823,#145824,#145825,#145826,#145827,#145828,#145829,#145830,#145831,
#145832,#145833,#145834,#145835,#145836,#145837,#145838,#145839,#145840,
#145841,#145842,#145843,#145844,#145845,#145846,#145847,#145848,#145849,
#145850,#145851,#145852,#145853,#145854,#145855,#145856,#145857,#145858,
#145859,#145860,#145861,#145862,#145863,#145864,#145865,#145866,#145867,
#145868,#145869,#145870,#145871,#145872,#145873,#145874,#145875,#145876,
#145877,#145878,#145879,#145880,#145881,#145882,#145883,#145884,#145885,
#145886,#145887,#145888,#145889,#145890,#145891,#145892,#145893,#145894,
#145895,#145896,#145897,#145898,#145899,#145900,#145901,#145902,#145903,
#145904,#145905,#145906,#145907,#145908,#145909,#145910,#145911,#145912,
#145913,#145914,#145915,#145916,#145917,#145918,#145919,#145920,#145921,
#145922,#145923,#145924,#145925,#145926,#145927,#145928,#145929,#145930,
#145931,#145932,#145933,#145934,#145935,#145936,#145937,#145938,#145939,
#145940,#145941,#145942,#145943,#145944,#145945,#145946,#145947,#145948,
#145949,#145950,#145951,#145952,#145953,#145954,#145955,#145956,#145957,
#145958,#145959,#145960,#145961,#145962,#145963,#145964,#145965,#145966,
#145967,#145968,#145969,#145970,#145971,#145972,#145973,#145974,#145975,
#145976,#145977,#145978,#145979,#145980,#145981,#145982,#145983,#145984,
#145985,#145986,#145987,#145988,#145989,#145990,#145991,#145992,#145993,
#145994,#145995,#145996,#145997,#145998,#145999,#146000,#146001,#146002,
#146003,#146004,#146005,#146006,#146007,#146008,#146009,#146010,#146011,
#146012,#146013,#146014,#146015,#146016,#146017,#146018,#146019,#146020,
#146021,#146022,#146023,#146024,#146025,#146026,#146027,#146028,#146029,
#146030,#146031,#146032,#146033,#146034,#146035,#146036,#146037,#146038,
#146039,#146040,#146041,#146042,#146043,#146044,#146045,#146046,#146047,
#146048,#146049,#146050,#146051,#146052,#146053,#146054,#146055,#146056,
#146057,#146058,#146059,#146060,#146061,#146062,#146063,#146064,#146065,
#146066,#146067,#146068,#146069,#146070,#146071,#146072,#146073,#146074,
#146075,#146076,#146077,#146078,#146079,#146080,#146081,#146082,#146083,
#146084,#146085,#146086,#146087,#146088,#146089,#146090,#146091,#146092,
#146093,#146094,#146095,#146096,#146097,#146098,#146099,#146100,#146101,
#146102,#146103,#146104,#146105,#146106,#146107,#146108,#146109,#146110,
#146111,#146112,#146113,#146114,#146115,#146116,#146117,#146118,#146119,
#146120,#146121,#146122,#146123,#146124,#146125,#146126,#146127,#146128,
#146129,#146130,#146131,#146132,#146133,#146134,#146135,#146136,#146137,
#146138,#146139,#146140,#146141,#146142,#146143,#146144,#146145,#146146,
#146147,#146148,#146149,#146150,#146151,#146152,#146153,#146154,#146155,
#146156,#146157,#146158,#146159,#146160,#146161,#146162,#146163,#146164,
#146165,#146166,#146167,#146168,#146169,#146170,#146171,#146172,#146173,
#146174,#146175,#146176,#146177,#146178,#146179,#146180,#146181,#146182,
#146183,#146184,#146185,#146186,#146187,#146188,#146189,#146190,#146191,
#146192,#146193,#146194,#146195,#146196,#146197,#146198,#146199,#146200,
#146201,#146202,#146203,#146204,#146205,#146206,#146207,#146208,#146209,
#146210,#146211,#146212,#146213,#146214,#146215,#146216,#146217,#146218,
#146219,#146220,#146221,#146222,#146223,#146224,#146225,#146226,#146227,
#146228,#146229,#146230,#146231,#146232,#146233,#146234,#146235,#146236,
#146237,#146238,#146239,#146240,#146241,#146242,#146243,#146244,#146245,
#146246,#146247,#146248,#146249,#146250,#146251,#146252,#146253,#146254,
#146255,#146256,#146257,#146258,#146259,#146260,#146261,#146262,#146263,
#146264,#146265,#146266,#146267,#146268,#146269,#146270,#146271,#146272,
#146273,#146274,#146275,#146276,#146277,#146278,#146279,#146280,#146281,
#146282,#146283,#146284,#146285,#146286,#146287,#146288,#146289,#146290,
#146291,#146292,#146293,#146294,#146295,#146296,#146297,#146298,#146299,
#146300,#146301,#146302,#146303,#146304,#146305,#146306,#146307,#146308,
#146309,#146310,#146311,#146312,#146313,#146314,#146315,#146316,#146317,
#146318,#146319,#146320,#146321,#146322,#146323,#146324,#146325,#146326,
#146327,#146328,#146329,#146330,#146331,#146332,#146333,#146334,#146335,
#146336,#146337,#146338,#146339,#146340,#146341,#146342,#146343,#146344,
#146345,#146346,#146347,#146348,#146349,#146350,#146351,#146352,#146353,
#146354,#146355,#146356,#146357,#146358,#146359,#146360,#146361,#146362,
#146363,#146364,#146365,#146366,#146367,#146368,#146369,#146370,#146371,
#146372,#146373,#146374,#146375,#146376,#146377,#146378,#146379,#146380,
#146381,#146382,#146383,#146384,#146385,#146386,#146387,#146388,#146389,
#146390,#146391,#146392,#146393,#146394,#146395,#146396,#146397,#146398,
#146399,#146400,#146401,#146402,#146403,#146404,#146405,#146406,#146407,
#146408,#146409,#146410,#146411,#146412,#146413,#146414,#146415,#146416,
#146417,#146418,#146419,#146420,#146421,#146422,#146423,#146424,#146425,
#146426,#146427,#146428,#146429,#146430,#146431,#146432,#146433,#146434,
#146435,#146436,#146437,#146438,#146439,#146440,#146441,#146442,#146443,
#146444,#146445,#146446,#146447,#146448,#146449,#146450,#146451,#146452,
#146453,#146454,#146455,#146456,#146457,#146458,#146459,#146460,#146461,
#146462,#146463,#146464,#146465,#146466,#146467,#146468,#146469,#146470,
#146471,#146472,#146473,#146474,#146475,#146476,#146477,#146478,#146479,
#146480,#146481,#146482,#146483,#146484,#146485,#146486,#146487,#146488,
#146489,#146490,#146491,#146492,#146493,#146494,#146495,#146496,#146497,
#146498,#146499,#146500,#146501,#146502,#146503,#146504,#146505,#146506,
#146507,#146508,#146509,#146510,#146511,#146512,#146513,#146514,#146515,
#146516,#146517,#146518,#146519,#146520,#146521,#146522,#146523,#146524,
#146525,#146526,#146527,#146528,#146529,#146530,#146531,#146532,#146533,
#146534,#146535,#146536,#146537,#146538,#146539,#146540,#146541,#146542,
#146543,#146544,#146545,#146546,#146547,#146548,#146549,#146550,#146551,
#146552,#146553,#146554,#146555,#146556,#146557,#146558,#146559,#146560,
#146561,#146562,#146563,#146564,#146565,#146566,#146567,#146568,#146569,
#146570,#146571,#146572,#146573,#146574,#146575,#146576,#146577,#146578,
#146579,#146580,#146581,#146582,#146583,#146584,#146585,#146586,#146587,
#146588,#146589,#146590,#146591,#146592,#146593,#146594,#146595,#146596,
#146597,#146598,#146599,#146600,#146601,#146602,#146603,#146604,#146605,
#146606,#146607,#146608,#146609,#146610,#146611,#146612,#146613,#146614,
#146615,#146616,#146617,#146618,#146619,#146620,#146621,#146622,#146623,
#146624,#146625,#146626,#146627,#146628,#146629,#146630,#146631,#146632,
#146633,#146634,#146635,#146636,#146637,#146638,#146639,#146640,#146641,
#146642,#146643,#146644,#146645,#146646,#146647,#146648,#146649,#146650,
#146651,#146652,#146653,#146654,#146655,#146656,#146657,#146658,#146659,
#146660,#146661,#146662,#146663,#146664,#146665,#146666,#146667,#146668,
#146669,#146670,#146671,#146672,#146673,#146674),(#146675,#146676,#146677,
#146678,#146679,#146680,#146681,#146682,#146683,#146684,#146685,#146686,
#146687,#146688,#146689,#146690,#146691,#146692,#146693,#146694,#146695,
#146696,#146697,#146698,#146699,#146700,#146701,#146702,#146703,#146704,
#146705,#146706,#146707,#146708,#146709,#146710,#146711,#146712,#146713,
#146714,#146715,#146716,#146717,#146718,#146719,#146720,#146721,#146722,
#146723,#146724,#146725,#146726,#146727,#146728,#146729,#146730,#146731,
#146732,#146733,#146734,#146735,#146736,#146737,#146738,#146739,#146740,
#146741,#146742,#146743,#146744,#146745,#146746,#146747,#146748,#146749,
#146750,#146751,#146752,#146753,#146754,#146755,#146756,#146757,#146758,
#146759,#146760,#146761,#146762,#146763,#146764,#146765,#146766,#146767,
#146768,#146769,#146770,#146771,#146772,#146773,#146774,#146775,#146776,
#146777,#146778,#146779,#146780,#146781,#146782,#146783,#146784,#146785,
#146786,#146787,#146788,#146789,#146790,#146791,#146792,#146793,#146794,
#146795,#146796,#146797,#146798,#146799,#146800,#146801,#146802,#146803,
#146804,#146805,#146806,#146807,#146808,#146809,#146810,#146811,#146812,
#146813,#146814,#146815,#146816,#146817,#146818,#146819,#146820,#146821,
#146822,#146823,#146824,#146825,#146826,#146827,#146828,#146829,#146830,
#146831,#146832,#146833,#146834,#146835,#146836,#146837,#146838,#146839,
#146840,#146841,#146842,#146843,#146844,#146845,#146846,#146847,#146848,
#146849,#146850,#146851,#146852,#146853,#146854,#146855,#146856,#146857,
#146858,#146859,#146860,#146861,#146862,#146863,#146864,#146865,#146866,
#146867,#146868,#146869,#146870,#146871,#146872,#146873,#146874,#146875,
#146876,#146877,#146878,#146879,#146880,#146881,#146882,#146883,#146884,
#146885,#146886,#146887,#146888,#146889,#146890,#146891,#146892,#146893,
#146894,#146895,#146896,#146897,#146898,#146899,#146900,#146901,#146902,
#146903,#146904,#146905,#146906,#146907,#146908,#146909,#146910,#146911,
#146912,#146913,#146914,#146915,#146916,#146917,#146918,#146919,#146920,
#146921,#146922,#146923,#146924,#146925,#146926,#146927,#146928,#146929,
#146930,#146931,#146932,#146933,#146934,#146935,#146936,#146937,#146938,
#146939,#146940,#146941,#146942,#146943,#146944,#146945,#146946,#146947,
#146948,#146949,#146950,#146951,#146952,#146953,#146954,#146955,#146956,
#146957,#146958,#146959,#146960,#146961,#146962,#146963,#146964,#146965,
#146966,#146967,#146968,#146969,#146970,#146971,#146972,#146973,#146974,
#146975,#146976,#146977,#146978,#146979,#146980,#146981,#146982,#146983,
#146984,#146985,#146986,#146987,#146988,#146989,#146990,#146991,#146992,
#146993,#146994,#146995,#146996,#146997,#146998,#146999,#147000,#147001,
#147002,#147003,#147004,#147005,#147006,#147007,#147008,#147009,#147010,
#147011,#147012,#147013,#147014,#147015,#147016,#147017,#147018,#147019,
#147020,#147021,#147022,#147023,#147024,#147025,#147026,#147027,#147028,
#147029,#147030,#147031,#147032,#147033,#147034,#147035,#147036,#147037,
#147038,#147039,#147040,#147041,#147042,#147043,#147044,#147045,#147046,
#147047,#147048,#147049,#147050,#147051,#147052,#147053,#147054,#147055,
#147056,#147057,#147058,#147059,#147060,#147061,#147062,#147063,#147064,
#147065,#147066,#147067,#147068,#147069,#147070,#147071,#147072,#147073,
#147074,#147075,#147076,#147077,#147078,#147079,#147080,#147081,#147082,
#147083,#147084,#147085,#147086,#147087,#147088,#147089,#147090,#147091,
#147092,#147093,#147094,#147095,#147096,#147097,#147098,#147099,#147100,
#147101,#147102,#147103,#147104,#147105,#147106,#147107,#147108,#147109,
#147110,#147111,#147112,#147113,#147114,#147115,#147116,#147117,#147118,
#147119,#147120,#147121,#147122,#147123,#147124,#147125,#147126,#147127,
#147128,#147129,#147130,#147131,#147132,#147133,#147134,#147135,#147136,
#147137,#147138,#147139,#147140,#147141,#147142,#147143,#147144,#147145,
#147146,#147147,#147148,#147149,#147150,#147151,#147152,#147153,#147154,
#147155,#147156,#147157,#147158,#147159,#147160,#147161,#147162,#147163,
#147164,#147165,#147166,#147167,#147168,#147169,#147170,#147171,#147172,
#147173,#147174,#147175,#147176,#147177,#147178,#147179,#147180,#147181,
#147182,#147183,#147184,#147185,#147186,#147187,#147188,#147189,#147190,
#147191,#147192,#147193,#147194,#147195,#147196,#147197,#147198,#147199,
#147200,#147201,#147202,#147203,#147204,#147205,#147206,#147207,#147208,
#147209,#147210,#147211,#147212,#147213,#147214,#147215,#147216,#147217,
#147218,#147219,#147220,#147221,#147222,#147223,#147224,#147225,#147226,
#147227,#147228,#147229,#147230,#147231,#147232,#147233,#147234,#147235,
#147236,#147237,#147238,#147239,#147240,#147241,#147242,#147243,#147244,
#147245,#147246,#147247,#147248,#147249,#147250,#147251,#147252,#147253,
#147254,#147255,#147256,#147257,#147258,#147259,#147260,#147261,#147262,
#147263,#147264,#147265,#147266,#147267,#147268,#147269,#147270,#147271,
#147272,#147273,#147274,#147275,#147276,#147277,#147278,#147279,#147280,
#147281,#147282,#147283,#147284,#147285,#147286,#147287,#147288,#147289,
#147290,#147291,#147292,#147293,#147294,#147295,#147296,#147297,#147298,
#147299,#147300,#147301,#147302,#147303,#147304,#147305,#147306,#147307,
#147308,#147309,#147310,#147311,#147312,#147313,#147314,#147315,#147316,
#147317,#147318,#147319,#147320,#147321,#147322,#147323,#147324,#147325,
#147326,#147327,#147328,#147329,#147330,#147331,#147332,#147333,#147334,
#147335,#147336,#147337,#147338,#147339,#147340,#147341,#147342,#147343,
#147344,#147345,#147346,#147347,#147348,#147349,#147350,#147351,#147352,
#147353,#147354,#147355,#147356,#147357,#147358,#147359,#147360,#147361,
#147362,#147363,#147364,#147365,#147366,#147367,#147368,#147369,#147370,
#147371,#147372,#147373,#147374,#147375,#147376,#147377,#147378,#147379,
#147380,#147381,#147382,#147383,#147384,#147385,#147386,#147387,#147388,
#147389,#147390,#147391,#147392,#147393,#147394,#147395,#147396,#147397,
#147398,#147399,#147400,#147401,#147402,#147403,#147404,#147405,#147406,
#147407,#147408,#147409,#147410,#147411,#147412,#147413,#147414,#147415,
#147416,#147417,#147418,#147419,#147420,#147421,#147422,#147423,#147424,
#147425,#147426,#147427,#147428,#147429,#147430,#147431,#147432,#147433,
#147434,#147435,#147436,#147437,#147438,#147439,#147440,#147441,#147442,
#147443,#147444,#147445,#147446,#147447,#147448,#147449,#147450,#147451,
#147452,#147453,#147454,#147455,#147456,#147457,#147458,#147459,#147460,
#147461,#147462,#147463,#147464,#147465,#147466,#147467,#147468,#147469,
#147470,#147471,#147472,#147473,#147474,#147475,#147476,#147477,#147478,
#147479,#147480,#147481,#147482,#147483,#147484,#147485,#147486,#147487,
#147488,#147489,#147490,#147491,#147492,#147493,#147494,#147495,#147496,
#147497,#147498,#147499,#147500,#147501,#147502,#147503,#147504,#147505,
#147506,#147507,#147508,#147509,#147510,#147511,#147512,#147513,#147514,
#147515,#147516,#147517,#147518,#147519,#147520,#147521,#147522,#147523,
#147524,#147525,#147526,#147527,#147528,#147529,#147530,#147531,#147532,
#147533,#147534,#147535,#147536,#147537,#147538,#147539,#147540,#147541,
#147542,#147543,#147544,#147545,#147546,#147547,#147548,#147549,#147550,
#147551,#147552,#147553,#147554,#147555,#147556,#147557,#147558,#147559,
#147560,#147561,#147562,#147563,#147564,#147565,#147566,#147567,#147568,
#147569,#147570,#147571,#147572,#147573,#147574,#147575,#147576,#147577,
#147578,#147579,#147580,#147581,#147582,#147583,#147584,#147585,#147586,
#147587,#147588,#147589,#147590,#147591,#147592,#147593,#147594,#147595,
#147596,#147597,#147598,#147599,#147600,#147601,#147602,#147603,#147604,
#147605,#147606,#147607,#147608,#147609,#147610,#147611,#147612,#147613,
#147614,#147615,#147616,#147617,#147618,#147619,#147620,#147621,#147622,
#147623,#147624,#147625,#147626,#147627,#147628,#147629,#147630,#147631,
#147632,#147633,#147634,#147635,#147636,#147637,#147638,#147639,#147640,
#147641,#147642,#147643,#147644,#147645,#147646,#147647,#147648,#147649,
#147650,#147651,#147652,#147653,#147654,#147655,#147656,#147657,#147658,
#147659,#147660,#147661,#147662,#147663,#147664,#147665,#147666,#147667,
#147668,#147669,#147670,#147671,#147672,#147673,#147674,#147675,#147676,
#147677,#147678,#147679,#147680,#147681,#147682,#147683,#147684,#147685,
#147686,#147687,#147688,#147689,#147690,#147691,#147692,#147693,#147694,
#147695,#147696,#147697,#147698,#147699,#147700,#147701,#147702,#147703,
#147704,#147705,#147706,#147707,#147708,#147709,#147710,#147711,#147712,
#147713,#147714,#147715,#147716,#147717,#147718,#147719,#147720,#147721,
#147722,#147723,#147724,#147725,#147726,#147727,#147728,#147729,#147730,
#147731,#147732,#147733,#147734,#147735,#147736,#147737,#147738,#147739,
#147740,#147741,#147742,#147743,#147744,#147745,#147746,#147747,#147748,
#147749,#147750,#147751,#147752,#147753,#147754,#147755,#147756,#147757,
#147758,#147759,#147760,#147761,#147762,#147763,#147764,#147765,#147766,
#147767,#147768,#147769,#147770,#147771,#147772,#147773,#147774,#147775,
#147776,#147777,#147778,#147779,#147780,#147781,#147782,#147783,#147784,
#147785,#147786,#147787,#147788,#147789,#147790,#147791,#147792,#147793,
#147794,#147795,#147796,#147797,#147798,#147799,#147800,#147801,#147802,
#147803,#147804,#147805,#147806,#147807,#147808,#147809,#147810,#147811,
#147812,#147813,#147814,#147815,#147816,#147817,#147818,#147819,#147820,
#147821,#147822,#147823,#147824,#147825,#147826,#147827,#147828,#147829,
#147830,#147831,#147832,#147833,#147834,#147835,#147836,#147837,#147838,
#147839,#147840,#147841,#147842,#147843,#147844,#147845,#147846,#147847,
#147848,#147849,#147850,#147851,#147852,#147853,#147854,#147855,#147856,
#147857,#147858,#147859,#147860,#147861,#147862,#147863,#147864,#147865,
#147866,#147867,#147868,#147869,#147870,#147871,#147872,#147873,#147874,
#147875,#147876,#147877,#147878,#147879,#147880,#147881,#147882,#147883,
#147884,#147885,#147886,#147887,#147888,#147889,#147890,#147891,#147892,
#147893,#147894,#147895,#147896,#147897,#147898,#147899,#147900,#147901,
#147902,#147903,#147904,#147905,#147906,#147907,#147908,#147909,#147910,
#147911,#147912,#147913,#147914,#147915,#147916,#147917,#147918,#147919,
#147920,#147921,#147922,#147923,#147924,#147925,#147926,#147927,#147928,
#147929,#147930,#147931,#147932,#147933,#147934,#147935,#147936,#147937,
#147938,#147939,#147940,#147941,#147942,#147943,#147944,#147945,#147946,
#147947,#147948,#147949,#147950,#147951,#147952,#147953,#147954,#147955,
#147956,#147957,#147958,#147959,#147960,#147961,#147962,#147963,#147964,
#147965,#147966,#147967,#147968,#147969,#147970,#147971,#147972,#147973,
#147974,#147975,#147976,#147977,#147978,#147979,#147980,#147981,#147982,
#147983,#147984,#147985,#147986,#147987,#147988,#147989,#147990,#147991,
#147992,#147993,#147994,#147995,#147996,#147997,#147998,#147999,#148000,
#148001,#148002,#148003,#148004,#148005,#148006,#148007,#148008,#148009,
#148010,#148011,#148012,#148013,#148014,#148015,#148016,#148017,#148018,
#148019,#148020,#148021,#148022,#148023,#148024,#148025,#148026,#148027,
#148028,#148029,#148030,#148031,#148032,#148033,#148034,#148035,#148036,
#148037,#148038,#148039,#148040,#148041,#148042,#148043,#148044,#148045,
#148046,#148047,#148048,#148049,#148050,#148051,#148052,#148053,#148054,
#148055,#148056,#148057,#148058,#148059,#148060,#148061,#148062,#148063,
#148064,#148065,#148066,#148067,#148068,#148069,#148070,#148071,#148072,
#148073,#148074,#148075,#148076,#148077,#148078,#148079,#148080,#148081,
#148082,#148083,#148084,#148085,#148086,#148087,#148088,#148089,#148090,
#148091,#148092,#148093,#148094,#148095,#148096,#148097,#148098,#148099,
#148100,#148101,#148102,#148103,#148104,#148105,#148106,#148107,#148108,
#148109,#148110,#148111,#148112,#148113,#148114,#148115,#148116,#148117,
#148118,#148119,#148120,#148121,#148122,#148123,#148124,#148125,#148126,
#148127,#148128,#148129,#148130,#148131,#148132,#148133,#148134,#148135,
#148136,#148137,#148138,#148139,#148140,#148141,#148142,#148143,#148144,
#148145,#148146,#148147,#148148,#148149,#148150,#148151,#148152,#148153,
#148154,#148155,#148156,#148157,#148158,#148159,#148160,#148161,#148162,
#148163,#148164,#148165,#148166,#148167,#148168,#148169,#148170,#148171,
#148172,#148173,#148174,#148175,#148176,#148177,#148178,#148179,#148180,
#148181,#148182,#148183,#148184,#148185,#148186,#148187,#148188,#148189,
#148190,#148191,#148192,#148193,#148194,#148195,#148196,#148197,#148198,
#148199,#148200,#148201,#148202,#148203,#148204,#148205,#148206,#148207,
#148208,#148209,#148210,#148211,#148212,#148213,#148214,#148215,#148216,
#148217,#148218,#148219,#148220,#148221,#148222,#148223,#148224,#148225,
#148226,#148227,#148228,#148229,#148230,#148231,#148232,#148233,#148234,
#148235,#148236,#148237,#148238,#148239,#148240,#148241,#148242,#148243,
#148244,#148245,#148246,#148247,#148248,#148249,#148250,#148251,#148252,
#148253,#148254,#148255,#148256,#148257,#148258,#148259,#148260,#148261,
#148262,#148263,#148264,#148265,#148266,#148267,#148268,#148269,#148270,
#148271,#148272,#148273,#148274,#148275,#148276,#148277,#148278,#148279,
#148280,#148281,#148282,#148283,#148284,#148285,#148286,#148287,#148288,
#148289,#148290,#148291,#148292,#148293,#148294,#148295,#148296,#148297,
#148298,#148299,#148300,#148301,#148302,#148303,#148304,#148305,#148306,
#148307,#148308,#148309,#148310,#148311,#148312,#148313,#148314,#148315,
#148316,#148317,#148318,#148319,#148320,#148321,#148322,#148323,#148324,
#148325,#148326,#148327,#148328,#148329,#148330,#148331,#148332,#148333,
#148334,#148335,#148336,#148337,#148338,#148339,#148340,#148341,#148342,
#148343,#148344,#148345,#148346,#148347,#148348,#148349,#148350,#148351,
#148352,#148353,#148354,#148355,#148356,#148357,#148358,#148359,#148360,
#148361,#148362,#148363,#148364,#148365,#148366,#148367,#148368,#148369,
#148370,#148371,#148372,#148373,#148374,#148375,#148376,#148377,#148378,
#148379,#148380,#148381,#148382,#148383,#148384,#148385,#148386,#148387,
#148388,#148389,#148390,#148391,#148392,#148393,#148394,#148395,#148396,
#148397,#148398,#148399,#148400,#148401,#148402,#148403,#148404,#148405,
#148406,#148407,#148408,#148409,#148410,#148411,#148412,#148413,#148414,
#148415,#148416,#148417,#148418,#148419,#148420,#148421,#148422,#148423,
#148424,#148425,#148426,#148427,#148428,#148429,#148430,#148431,#148432,
#148433,#148434,#148435,#148436,#148437,#148438,#148439,#148440,#148441,
#148442,#148443,#148444,#148445,#148446,#148447,#148448,#148449,#148450,
#148451,#148452,#148453,#148454,#148455,#148456,#148457,#148458,#148459,
#148460,#148461,#148462,#148463,#148464,#148465,#148466,#148467,#148468,
#148469,#148470,#148471,#148472,#148473,#148474,#148475,#148476,#148477,
#148478,#148479,#148480,#148481,#148482,#148483,#148484,#148485,#148486,
#148487,#148488,#148489,#148490,#148491,#148492,#148493,#148494,#148495,
#148496,#148497,#148498,#148499,#148500,#148501,#148502,#148503,#148504,
#148505,#148506,#148507,#148508,#148509,#148510,#148511,#148512,#148513,
#148514,#148515,#148516,#148517,#148518,#148519,#148520,#148521,#148522,
#148523,#148524,#148525,#148526,#148527,#148528,#148529,#148530,#148531,
#148532,#148533,#148534,#148535,#148536,#148537,#148538,#148539,#148540,
#148541,#148542,#148543,#148544,#148545,#148546,#148547,#148548,#148549,
#148550,#148551,#148552,#148553,#148554,#148555,#148556,#148557,#148558,
#148559,#148560,#148561,#148562,#148563,#148564,#148565,#148566,#148567,
#148568,#148569,#148570,#148571,#148572,#148573,#148574,#148575,#148576,
#148577,#148578,#148579,#148580,#148581,#148582,#148583,#148584,#148585,
#148586,#148587,#148588,#148589,#148590,#148591,#148592,#148593,#148594,
#148595,#148596,#148597,#148598,#148599,#148600,#148601,#148602,#148603,
#148604,#148605,#148606,#148607,#148608,#148609,#148610,#148611,#148612,
#148613,#148614,#148615,#148616,#148617,#148618,#148619,#148620,#148621,
#148622,#148623,#148624,#148625,#148626,#148627,#148628,#148629,#148630,
#148631,#148632,#148633,#148634,#148635,#148636,#148637,#148638,#148639,
#148640,#148641,#148642,#148643,#148644,#148645,#148646,#148647,#148648,
#148649,#148650,#148651,#148652,#148653,#148654,#148655,#148656,#148657,
#148658,#148659,#148660,#148661,#148662,#148663,#148664,#148665,#148666,
#148667,#148668,#148669,#148670,#148671,#148672,#148673,#148674,#148675,
#148676,#148677,#148678,#148679,#148680,#148681,#148682,#148683,#148684,
#148685,#148686,#148687,#148688,#148689,#148690,#148691,#148692,#148693,
#148694,#148695,#148696,#148697,#148698,#148699,#148700,#148701,#148702,
#148703,#148704,#148705,#148706,#148707,#148708,#148709,#148710,#148711,
#148712,#148713,#148714,#148715,#148716,#148717,#148718,#148719,#148720,
#148721,#148722,#148723,#148724,#148725),(#148726,#148727,#148728,#148729,
#148730,#148731,#148732,#148733,#148734,#148735,#148736,#148737,#148738,
#148739,#148740,#148741,#148742,#148743,#148744,#148745,#148746,#148747,
#148748,#148749,#148750,#148751,#148752,#148753,#148754,#148755,#148756,
#148757,#148758,#148759,#148760,#148761,#148762,#148763,#148764,#148765,
#148766,#148767,#148768,#148769,#148770,#148771,#148772,#148773,#148774,
#148775,#148776,#148777,#148778,#148779,#148780,#148781,#148782,#148783,
#148784,#148785,#148786,#148787,#148788,#148789,#148790,#148791,#148792,
#148793,#148794,#148795,#148796,#148797,#148798,#148799,#148800,#148801,
#148802,#148803,#148804,#148805,#148806,#148807,#148808,#148809,#148810,
#148811,#148812,#148813,#148814,#148815,#148816,#148817,#148818,#148819,
#148820,#148821,#148822,#148823,#148824,#148825,#148826,#148827,#148828,
#148829,#148830,#148831,#148832,#148833,#148834,#148835,#148836,#148837,
#148838,#148839,#148840,#148841,#148842,#148843,#148844,#148845,#148846,
#148847,#148848,#148849,#148850,#148851,#148852,#148853,#148854,#148855,
#148856,#148857,#148858,#148859,#148860,#148861,#148862,#148863,#148864,
#148865,#148866,#148867,#148868,#148869,#148870,#148871,#148872,#148873,
#148874,#148875,#148876,#148877,#148878,#148879,#148880,#148881,#148882,
#148883,#148884,#148885,#148886,#148887,#148888,#148889,#148890,#148891,
#148892,#148893,#148894,#148895,#148896,#148897,#148898,#148899,#148900,
#148901,#148902,#148903,#148904,#148905,#148906,#148907,#148908,#148909,
#148910,#148911,#148912,#148913,#148914,#148915,#148916,#148917,#148918,
#148919,#148920,#148921,#148922,#148923,#148924,#148925,#148926,#148927,
#148928,#148929,#148930,#148931,#148932,#148933,#148934,#148935,#148936,
#148937,#148938,#148939,#148940,#148941,#148942,#148943,#148944,#148945,
#148946,#148947,#148948,#148949,#148950,#148951,#148952,#148953,#148954,
#148955,#148956,#148957,#148958,#148959,#148960,#148961,#148962,#148963,
#148964,#148965,#148966,#148967,#148968,#148969,#148970,#148971,#148972,
#148973,#148974,#148975,#148976,#148977,#148978,#148979,#148980,#148981,
#148982,#148983,#148984,#148985,#148986,#148987,#148988,#148989,#148990,
#148991,#148992,#148993,#148994,#148995,#148996,#148997,#148998,#148999,
#149000,#149001,#149002,#149003,#149004,#149005,#149006,#149007,#149008,
#149009,#149010,#149011,#149012,#149013,#149014,#149015,#149016,#149017,
#149018,#149019,#149020,#149021,#149022,#149023,#149024,#149025,#149026,
#149027,#149028,#149029,#149030,#149031,#149032,#149033,#149034,#149035,
#149036,#149037,#149038,#149039,#149040,#149041,#149042,#149043,#149044,
#149045,#149046,#149047,#149048,#149049,#149050,#149051,#149052,#149053,
#149054,#149055,#149056,#149057,#149058,#149059,#149060,#149061,#149062,
#149063,#149064,#149065,#149066,#149067,#149068,#149069,#149070,#149071,
#149072,#149073,#149074,#149075,#149076,#149077,#149078,#149079,#149080,
#149081,#149082,#149083,#149084,#149085,#149086,#149087,#149088,#149089,
#149090,#149091,#149092,#149093,#149094,#149095,#149096,#149097,#149098,
#149099,#149100,#149101,#149102,#149103,#149104,#149105,#149106,#149107,
#149108,#149109,#149110,#149111,#149112,#149113,#149114,#149115,#149116,
#149117,#149118,#149119,#149120,#149121,#149122,#149123,#149124,#149125,
#149126,#149127,#149128,#149129,#149130,#149131,#149132,#149133,#149134,
#149135,#149136,#149137,#149138,#149139,#149140,#149141,#149142,#149143,
#149144,#149145,#149146,#149147,#149148,#149149,#149150,#149151,#149152,
#149153,#149154,#149155,#149156,#149157,#149158,#149159,#149160,#149161,
#149162,#149163,#149164,#149165,#149166,#149167,#149168,#149169,#149170,
#149171,#149172,#149173,#149174,#149175,#149176,#149177,#149178,#149179,
#149180,#149181,#149182,#149183,#149184,#149185,#149186,#149187,#149188,
#149189,#149190,#149191,#149192,#149193,#149194,#149195,#149196,#149197,
#149198,#149199,#149200,#149201,#149202,#149203,#149204,#149205,#149206,
#149207,#149208,#149209,#149210,#149211,#149212,#149213,#149214,#149215,
#149216,#149217,#149218,#149219,#149220,#149221,#149222,#149223,#149224,
#149225,#149226,#149227,#149228,#149229,#149230,#149231,#149232,#149233,
#149234,#149235,#149236,#149237,#149238,#149239,#149240,#149241,#149242,
#149243,#149244,#149245,#149246,#149247,#149248,#149249,#149250,#149251,
#149252,#149253,#149254,#149255,#149256,#149257,#149258,#149259,#149260,
#149261,#149262,#149263,#149264,#149265,#149266,#149267,#149268,#149269,
#149270,#149271,#149272,#149273,#149274,#149275,#149276,#149277,#149278,
#149279,#149280,#149281,#149282,#149283,#149284,#149285,#149286,#149287,
#149288,#149289,#149290,#149291,#149292,#149293,#149294,#149295,#149296,
#149297,#149298,#149299,#149300,#149301,#149302,#149303,#149304,#149305,
#149306,#149307,#149308,#149309,#149310,#149311,#149312,#149313,#149314,
#149315,#149316,#149317,#149318,#149319,#149320,#149321,#149322,#149323,
#149324,#149325,#149326,#149327,#149328,#149329,#149330,#149331,#149332,
#149333,#149334,#149335,#149336,#149337,#149338,#149339,#149340,#149341,
#149342,#149343,#149344,#149345,#149346,#149347,#149348,#149349,#149350,
#149351,#149352,#149353,#149354,#149355,#149356,#149357,#149358,#149359,
#149360,#149361,#149362,#149363,#149364,#149365,#149366,#149367,#149368,
#149369,#149370,#149371,#149372,#149373,#149374,#149375,#149376,#149377,
#149378,#149379,#149380,#149381,#149382,#149383,#149384,#149385,#149386,
#149387,#149388,#149389,#149390,#149391,#149392,#149393,#149394,#149395,
#149396,#149397,#149398,#149399,#149400,#149401,#149402,#149403,#149404,
#149405,#149406,#149407,#149408,#149409,#149410,#149411,#149412,#149413,
#149414,#149415,#149416,#149417,#149418,#149419,#149420,#149421,#149422,
#149423,#149424,#149425,#149426,#149427,#149428,#149429,#149430,#149431,
#149432,#149433,#149434,#149435,#149436,#149437,#149438,#149439,#149440,
#149441,#149442,#149443,#149444,#149445,#149446,#149447,#149448,#149449,
#149450,#149451,#149452,#149453,#149454,#149455,#149456,#149457,#149458,
#149459,#149460,#149461,#149462,#149463,#149464,#149465,#149466,#149467,
#149468,#149469,#149470,#149471,#149472,#149473,#149474,#149475,#149476,
#149477,#149478,#149479,#149480,#149481,#149482,#149483,#149484,#149485,
#149486,#149487,#149488,#149489,#149490,#149491,#149492,#149493,#149494,
#149495,#149496,#149497,#149498,#149499,#149500,#149501,#149502,#149503,
#149504,#149505,#149506,#149507,#149508,#149509,#149510,#149511,#149512,
#149513,#149514,#149515,#149516,#149517,#149518,#149519,#149520,#149521,
#149522,#149523,#149524,#149525,#149526,#149527,#149528,#149529,#149530,
#149531,#149532,#149533,#149534,#149535,#149536,#149537,#149538,#149539,
#149540,#149541,#149542,#149543,#149544,#149545,#149546,#149547,#149548,
#149549,#149550,#149551,#149552,#149553,#149554,#149555,#149556,#149557,
#149558,#149559,#149560,#149561,#149562,#149563,#149564,#149565,#149566,
#149567,#149568,#149569,#149570,#149571,#149572,#149573,#149574,#149575,
#149576,#149577,#149578,#149579,#149580,#149581,#149582,#149583,#149584,
#149585,#149586,#149587,#149588,#149589,#149590,#149591,#149592,#149593,
#149594,#149595,#149596,#149597,#149598,#149599,#149600,#149601,#149602,
#149603,#149604,#149605,#149606,#149607,#149608,#149609,#149610,#149611,
#149612,#149613,#149614,#149615,#149616,#149617,#149618,#149619,#149620,
#149621,#149622,#149623,#149624,#149625,#149626,#149627,#149628,#149629,
#149630,#149631,#149632,#149633,#149634,#149635,#149636,#149637,#149638,
#149639,#149640,#149641,#149642,#149643,#149644,#149645,#149646,#149647,
#149648,#149649,#149650,#149651,#149652,#149653,#149654,#149655,#149656,
#149657,#149658,#149659,#149660,#149661,#149662,#149663,#149664,#149665,
#149666,#149667,#149668,#149669,#149670,#149671,#149672,#149673,#149674,
#149675,#149676,#149677,#149678,#149679,#149680,#149681,#149682,#149683,
#149684,#149685,#149686,#149687,#149688,#149689,#149690,#149691,#149692,
#149693,#149694,#149695,#149696,#149697,#149698,#149699,#149700,#149701,
#149702,#149703,#149704,#149705,#149706,#149707,#149708,#149709,#149710,
#149711,#149712,#149713,#149714,#149715,#149716,#149717,#149718,#149719,
#149720,#149721,#149722,#149723,#149724,#149725,#149726,#149727,#149728,
#149729,#149730,#149731,#149732,#149733,#149734,#149735,#149736,#149737,
#149738,#149739,#149740,#149741,#149742,#149743,#149744,#149745,#149746,
#149747,#149748,#149749,#149750,#149751,#149752,#149753,#149754,#149755,
#149756,#149757,#149758,#149759,#149760,#149761,#149762,#149763,#149764,
#149765,#149766,#149767,#149768,#149769,#149770,#149771,#149772,#149773,
#149774,#149775,#149776,#149777,#149778,#149779,#149780,#149781,#149782,
#149783,#149784,#149785,#149786,#149787,#149788,#149789,#149790,#149791,
#149792,#149793,#149794,#149795,#149796,#149797,#149798,#149799,#149800,
#149801,#149802,#149803,#149804,#149805,#149806,#149807,#149808,#149809,
#149810,#149811,#149812,#149813,#149814,#149815,#149816,#149817,#149818,
#149819,#149820,#149821,#149822,#149823,#149824,#149825,#149826,#149827,
#149828,#149829,#149830,#149831,#149832,#149833,#149834,#149835,#149836,
#149837,#149838,#149839,#149840,#149841,#149842,#149843,#149844,#149845,
#149846,#149847,#149848,#149849,#149850,#149851,#149852,#149853,#149854,
#149855,#149856,#149857,#149858,#149859,#149860,#149861,#149862,#149863,
#149864,#149865,#149866,#149867,#149868,#149869,#149870,#149871,#149872,
#149873,#149874,#149875,#149876,#149877,#149878,#149879,#149880,#149881,
#149882,#149883,#149884,#149885,#149886,#149887,#149888,#149889,#149890,
#149891,#149892,#149893,#149894,#149895,#149896,#149897,#149898,#149899,
#149900,#149901,#149902,#149903,#149904,#149905,#149906,#149907,#149908,
#149909,#149910,#149911,#149912,#149913,#149914,#149915,#149916,#149917,
#149918,#149919,#149920,#149921,#149922,#149923,#149924,#149925,#149926,
#149927,#149928,#149929,#149930,#149931,#149932,#149933,#149934,#149935,
#149936,#149937,#149938,#149939,#149940,#149941,#149942,#149943,#149944,
#149945,#149946,#149947,#149948,#149949,#149950,#149951,#149952,#149953,
#149954,#149955,#149956,#149957,#149958,#149959,#149960,#149961,#149962,
#149963,#149964,#149965,#149966,#149967,#149968,#149969,#149970,#149971,
#149972,#149973,#149974,#149975,#149976,#149977,#149978,#149979,#149980,
#149981,#149982,#149983,#149984,#149985,#149986,#149987,#149988,#149989,
#149990,#149991,#149992,#149993,#149994,#149995,#149996,#149997,#149998,
#149999,#150000,#150001,#150002,#150003,#150004,#150005,#150006,#150007,
#150008,#150009,#150010,#150011,#150012,#150013,#150014,#150015,#150016,
#150017,#150018,#150019,#150020,#150021,#150022,#150023,#150024,#150025,
#150026,#150027,#150028,#150029,#150030,#150031,#150032,#150033,#150034,
#150035,#150036,#150037,#150038,#150039,#150040,#150041,#150042,#150043,
#150044,#150045,#150046,#150047,#150048,#150049,#150050,#150051,#150052,
#150053,#150054,#150055,#150056,#150057,#150058,#150059,#150060,#150061,
#150062,#150063,#150064,#150065,#150066,#150067,#150068,#150069,#150070,
#150071,#150072,#150073,#150074,#150075,#150076,#150077,#150078,#150079,
#150080,#150081,#150082,#150083,#150084,#150085,#150086,#150087,#150088,
#150089,#150090,#150091,#150092,#150093,#150094,#150095,#150096,#150097,
#150098,#150099,#150100,#150101,#150102,#150103,#150104,#150105,#150106,
#150107,#150108,#150109,#150110,#150111,#150112,#150113,#150114,#150115,
#150116,#150117,#150118,#150119,#150120,#150121,#150122,#150123,#150124,
#150125,#150126,#150127,#150128,#150129,#150130,#150131,#150132,#150133,
#150134,#150135,#150136,#150137,#150138,#150139,#150140,#150141,#150142,
#150143,#150144,#150145,#150146,#150147,#150148,#150149,#150150,#150151,
#150152,#150153,#150154,#150155,#150156,#150157,#150158,#150159,#150160,
#150161,#150162,#150163,#150164,#150165,#150166,#150167,#150168,#150169,
#150170,#150171,#150172,#150173,#150174,#150175,#150176,#150177,#150178,
#150179,#150180,#150181,#150182,#150183,#150184,#150185,#150186,#150187,
#150188,#150189,#150190,#150191,#150192,#150193,#150194,#150195,#150196,
#150197,#150198,#150199,#150200,#150201,#150202,#150203,#150204,#150205,
#150206,#150207,#150208,#150209,#150210,#150211,#150212,#150213,#150214,
#150215,#150216,#150217,#150218,#150219,#150220,#150221,#150222,#150223,
#150224,#150225,#150226,#150227,#150228,#150229,#150230,#150231,#150232,
#150233,#150234,#150235,#150236,#150237,#150238,#150239,#150240,#150241,
#150242,#150243,#150244,#150245,#150246,#150247,#150248,#150249,#150250,
#150251,#150252,#150253,#150254,#150255,#150256,#150257,#150258,#150259,
#150260,#150261,#150262,#150263,#150264,#150265,#150266,#150267,#150268,
#150269,#150270,#150271,#150272,#150273,#150274,#150275,#150276,#150277,
#150278,#150279,#150280,#150281,#150282,#150283,#150284,#150285,#150286,
#150287,#150288,#150289,#150290,#150291,#150292,#150293,#150294,#150295,
#150296,#150297,#150298,#150299,#150300,#150301,#150302,#150303,#150304,
#150305,#150306,#150307,#150308,#150309,#150310,#150311,#150312,#150313,
#150314,#150315,#150316,#150317,#150318,#150319,#150320,#150321,#150322,
#150323,#150324,#150325,#150326,#150327,#150328,#150329,#150330,#150331,
#150332,#150333,#150334,#150335,#150336,#150337,#150338,#150339,#150340,
#150341,#150342,#150343,#150344,#150345,#150346,#150347,#150348,#150349,
#150350,#150351,#150352,#150353,#150354,#150355,#150356,#150357,#150358,
#150359,#150360,#150361,#150362,#150363,#150364,#150365,#150366,#150367,
#150368,#150369,#150370,#150371,#150372,#150373,#150374,#150375,#150376,
#150377,#150378,#150379,#150380,#150381,#150382,#150383,#150384,#150385,
#150386,#150387,#150388,#150389,#150390,#150391,#150392,#150393,#150394,
#150395,#150396,#150397,#150398,#150399,#150400,#150401,#150402,#150403,
#150404,#150405,#150406,#150407,#150408,#150409,#150410,#150411,#150412,
#150413,#150414,#150415,#150416,#150417,#150418,#150419,#150420,#150421,
#150422,#150423,#150424,#150425,#150426,#150427,#150428,#150429,#150430,
#150431,#150432,#150433,#150434,#150435,#150436,#150437,#150438,#150439,
#150440,#150441,#150442,#150443,#150444,#150445,#150446,#150447,#150448,
#150449,#150450,#150451,#150452,#150453,#150454,#150455,#150456,#150457,
#150458,#150459,#150460,#150461,#150462,#150463,#150464,#150465,#150466,
#150467,#150468,#150469,#150470,#150471,#150472,#150473,#150474,#150475,
#150476,#150477,#150478,#150479,#150480,#150481,#150482,#150483,#150484,
#150485,#150486,#150487,#150488,#150489,#150490,#150491,#150492,#150493,
#150494,#150495,#150496,#150497,#150498,#150499,#150500,#150501,#150502,
#150503,#150504,#150505,#150506,#150507,#150508,#150509,#150510,#150511,
#150512,#150513,#150514,#150515,#150516,#150517,#150518,#150519,#150520,
#150521,#150522,#150523,#150524,#150525,#150526,#150527,#150528,#150529,
#150530,#150531,#150532,#150533,#150534,#150535,#150536,#150537,#150538,
#150539,#150540,#150541,#150542,#150543,#150544,#150545,#150546,#150547,
#150548,#150549,#150550,#150551,#150552,#150553,#150554,#150555,#150556,
#150557,#150558,#150559,#150560,#150561,#150562,#150563,#150564,#150565,
#150566,#150567,#150568,#150569,#150570,#150571,#150572,#150573,#150574,
#150575,#150576,#150577,#150578,#150579,#150580,#150581,#150582,#150583,
#150584,#150585,#150586,#150587,#150588,#150589,#150590,#150591,#150592,
#150593,#150594,#150595,#150596,#150597,#150598,#150599,#150600,#150601,
#150602,#150603,#150604,#150605,#150606,#150607,#150608,#150609,#150610,
#150611,#150612,#150613,#150614,#150615,#150616,#150617,#150618,#150619,
#150620,#150621,#150622,#150623,#150624,#150625,#150626,#150627,#150628,
#150629,#150630,#150631,#150632,#150633,#150634,#150635,#150636,#150637,
#150638,#150639,#150640,#150641,#150642,#150643,#150644,#150645,#150646,
#150647,#150648,#150649,#150650,#150651,#150652,#150653,#150654,#150655,
#150656,#150657,#150658,#150659,#150660,#150661,#150662,#150663,#150664,
#150665,#150666,#150667,#150668,#150669,#150670,#150671,#150672,#150673,
#150674,#150675,#150676,#150677,#150678,#150679,#150680,#150681,#150682,
#150683,#150684,#150685,#150686,#150687,#150688,#150689,#150690,#150691,
#150692,#150693,#150694,#150695,#150696,#150697,#150698,#150699,#150700,
#150701,#150702,#150703,#150704,#150705,#150706,#150707,#150708,#150709,
#150710,#150711,#150712,#150713,#150714,#150715,#150716,#150717,#150718,
#150719,#150720,#150721,#150722,#150723,#150724,#150725,#150726,#150727,
#150728,#150729,#150730,#150731,#150732,#150733,#150734,#150735,#150736,
#150737,#150738,#150739,#150740,#150741,#150742,#150743,#150744,#150745,
#150746,#150747,#150748,#150749,#150750,#150751,#150752,#150753,#150754,
#150755,#150756,#150757,#150758,#150759,#150760,#150761,#150762,#150763,
#150764,#150765,#150766,#150767,#150768,#150769,#150770,#150771,#150772,
#150773,#150774,#150775,#150776),(#150777,#150778,#150779,#150780,#150781,
#150782,#150783,#150784,#150785,#150786,#150787,#150788,#150789,#150790,
#150791,#150792,#150793,#150794,#150795,#150796,#150797,#150798,#150799,
#150800,#150801,#150802,#150803,#150804,#150805,#150806,#150807,#150808,
#150809,#150810,#150811,#150812,#150813,#150814,#150815,#150816,#150817,
#150818,#150819,#150820,#150821,#150822,#150823,#150824,#150825,#150826,
#150827,#150828,#150829,#150830,#150831,#150832,#150833,#150834,#150835,
#150836,#150837,#150838,#150839,#150840,#150841,#150842,#150843,#150844,
#150845,#150846,#150847,#150848,#150849,#150850,#150851,#150852,#150853,
#150854,#150855,#150856,#150857,#150858,#150859,#150860,#150861,#150862,
#150863,#150864,#150865,#150866,#150867,#150868,#150869,#150870,#150871,
#150872,#150873,#150874,#150875,#150876,#150877,#150878,#150879,#150880,
#150881,#150882,#150883,#150884,#150885,#150886,#150887,#150888,#150889,
#150890,#150891,#150892,#150893,#150894,#150895,#150896,#150897,#150898,
#150899,#150900,#150901,#150902,#150903,#150904,#150905,#150906,#150907,
#150908,#150909,#150910,#150911,#150912,#150913,#150914,#150915,#150916,
#150917,#150918,#150919,#150920,#150921,#150922,#150923,#150924,#150925,
#150926,#150927,#150928,#150929,#150930,#150931,#150932,#150933,#150934,
#150935,#150936,#150937,#150938,#150939,#150940,#150941,#150942,#150943,
#150944,#150945,#150946,#150947,#150948,#150949,#150950,#150951,#150952,
#150953,#150954,#150955,#150956,#150957,#150958,#150959,#150960,#150961,
#150962,#150963,#150964,#150965,#150966,#150967,#150968,#150969,#150970,
#150971,#150972,#150973,#150974,#150975,#150976,#150977,#150978,#150979,
#150980,#150981,#150982,#150983,#150984,#150985,#150986,#150987,#150988,
#150989,#150990,#150991,#150992,#150993,#150994,#150995,#150996,#150997,
#150998,#150999,#151000,#151001,#151002,#151003,#151004,#151005,#151006,
#151007,#151008,#151009,#151010,#151011,#151012,#151013,#151014,#151015,
#151016,#151017,#151018,#151019,#151020,#151021,#151022,#151023,#151024,
#151025,#151026,#151027,#151028,#151029,#151030,#151031,#151032,#151033,
#151034,#151035,#151036,#151037,#151038,#151039,#151040,#151041,#151042,
#151043,#151044,#151045,#151046,#151047,#151048,#151049,#151050,#151051,
#151052,#151053,#151054,#151055,#151056,#151057,#151058,#151059,#151060,
#151061,#151062,#151063,#151064,#151065,#151066,#151067,#151068,#151069,
#151070,#151071,#151072,#151073,#151074,#151075,#151076,#151077,#151078,
#151079,#151080,#151081,#151082,#151083,#151084,#151085,#151086,#151087,
#151088,#151089,#151090,#151091,#151092,#151093,#151094,#151095,#151096,
#151097,#151098,#151099,#151100,#151101,#151102,#151103,#151104,#151105,
#151106,#151107,#151108,#151109,#151110,#151111,#151112,#151113,#151114,
#151115,#151116,#151117,#151118,#151119,#151120,#151121,#151122,#151123,
#151124,#151125,#151126,#151127,#151128,#151129,#151130,#151131,#151132,
#151133,#151134,#151135,#151136,#151137,#151138,#151139,#151140,#151141,
#151142,#151143,#151144,#151145,#151146,#151147,#151148,#151149,#151150,
#151151,#151152,#151153,#151154,#151155,#151156,#151157,#151158,#151159,
#151160,#151161,#151162,#151163,#151164,#151165,#151166,#151167,#151168,
#151169,#151170,#151171,#151172,#151173,#151174,#151175,#151176,#151177,
#151178,#151179,#151180,#151181,#151182,#151183,#151184,#151185,#151186,
#151187,#151188,#151189,#151190,#151191,#151192,#151193,#151194,#151195,
#151196,#151197,#151198,#151199,#151200,#151201,#151202,#151203,#151204,
#151205,#151206,#151207,#151208,#151209,#151210,#151211,#151212,#151213,
#151214,#151215,#151216,#151217,#151218,#151219,#151220,#151221,#151222,
#151223,#151224,#151225,#151226,#151227,#151228,#151229,#151230,#151231,
#151232,#151233,#151234,#151235,#151236,#151237,#151238,#151239,#151240,
#151241,#151242,#151243,#151244,#151245,#151246,#151247,#151248,#151249,
#151250,#151251,#151252,#151253,#151254,#151255,#151256,#151257,#151258,
#151259,#151260,#151261,#151262,#151263,#151264,#151265,#151266,#151267,
#151268,#151269,#151270,#151271,#151272,#151273,#151274,#151275,#151276,
#151277,#151278,#151279,#151280,#151281,#151282,#151283,#151284,#151285,
#151286,#151287,#151288,#151289,#151290,#151291,#151292,#151293,#151294,
#151295,#151296,#151297,#151298,#151299,#151300,#151301,#151302,#151303,
#151304,#151305,#151306,#151307,#151308,#151309,#151310,#151311,#151312,
#151313,#151314,#151315,#151316,#151317,#151318,#151319,#151320,#151321,
#151322,#151323,#151324,#151325,#151326,#151327,#151328,#151329,#151330,
#151331,#151332,#151333,#151334,#151335,#151336,#151337,#151338,#151339,
#151340,#151341,#151342,#151343,#151344,#151345,#151346,#151347,#151348,
#151349,#151350,#151351,#151352,#151353,#151354,#151355,#151356,#151357,
#151358,#151359,#151360,#151361,#151362,#151363,#151364,#151365,#151366,
#151367,#151368,#151369,#151370,#151371,#151372,#151373,#151374,#151375,
#151376,#151377,#151378,#151379,#151380,#151381,#151382,#151383,#151384,
#151385,#151386,#151387,#151388,#151389,#151390,#151391,#151392,#151393,
#151394,#151395,#151396,#151397,#151398,#151399,#151400,#151401,#151402,
#151403,#151404,#151405,#151406,#151407,#151408,#151409,#151410,#151411,
#151412,#151413,#151414,#151415,#151416,#151417,#151418,#151419,#151420,
#151421,#151422,#151423,#151424,#151425,#151426,#151427,#151428,#151429,
#151430,#151431,#151432,#151433,#151434,#151435,#151436,#151437,#151438,
#151439,#151440,#151441,#151442,#151443,#151444,#151445,#151446,#151447,
#151448,#151449,#151450,#151451,#151452,#151453,#151454,#151455,#151456,
#151457,#151458,#151459,#151460,#151461,#151462,#151463,#151464,#151465,
#151466,#151467,#151468,#151469,#151470,#151471,#151472,#151473,#151474,
#151475,#151476,#151477,#151478,#151479,#151480,#151481,#151482,#151483,
#151484,#151485,#151486,#151487,#151488,#151489,#151490,#151491,#151492,
#151493,#151494,#151495,#151496,#151497,#151498,#151499,#151500,#151501,
#151502,#151503,#151504,#151505,#151506,#151507,#151508,#151509,#151510,
#151511,#151512,#151513,#151514,#151515,#151516,#151517,#151518,#151519,
#151520,#151521,#151522,#151523,#151524,#151525,#151526,#151527,#151528,
#151529,#151530,#151531,#151532,#151533,#151534,#151535,#151536,#151537,
#151538,#151539,#151540,#151541,#151542,#151543,#151544,#151545,#151546,
#151547,#151548,#151549,#151550,#151551,#151552,#151553,#151554,#151555,
#151556,#151557,#151558,#151559,#151560,#151561,#151562,#151563,#151564,
#151565,#151566,#151567,#151568,#151569,#151570,#151571,#151572,#151573,
#151574,#151575,#151576,#151577,#151578,#151579,#151580,#151581,#151582,
#151583,#151584,#151585,#151586,#151587,#151588,#151589,#151590,#151591,
#151592,#151593,#151594,#151595,#151596,#151597,#151598,#151599,#151600,
#151601,#151602,#151603,#151604,#151605,#151606,#151607,#151608,#151609,
#151610,#151611,#151612,#151613,#151614,#151615,#151616,#151617,#151618,
#151619,#151620,#151621,#151622,#151623,#151624,#151625,#151626,#151627,
#151628,#151629,#151630,#151631,#151632,#151633,#151634,#151635,#151636,
#151637,#151638,#151639,#151640,#151641,#151642,#151643,#151644,#151645,
#151646,#151647,#151648,#151649,#151650,#151651,#151652,#151653,#151654,
#151655,#151656,#151657,#151658,#151659,#151660,#151661,#151662,#151663,
#151664,#151665,#151666,#151667,#151668,#151669,#151670,#151671,#151672,
#151673,#151674,#151675,#151676,#151677,#151678,#151679,#151680,#151681,
#151682,#151683,#151684,#151685,#151686,#151687,#151688,#151689,#151690,
#151691,#151692,#151693,#151694,#151695,#151696,#151697,#151698,#151699,
#151700,#151701,#151702,#151703,#151704,#151705,#151706,#151707,#151708,
#151709,#151710,#151711,#151712,#151713,#151714,#151715,#151716,#151717,
#151718,#151719,#151720,#151721,#151722,#151723,#151724,#151725,#151726,
#151727,#151728,#151729,#151730,#151731,#151732,#151733,#151734,#151735,
#151736,#151737,#151738,#151739,#151740,#151741,#151742,#151743,#151744,
#151745,#151746,#151747,#151748,#151749,#151750,#151751,#151752,#151753,
#151754,#151755,#151756,#151757,#151758,#151759,#151760,#151761,#151762,
#151763,#151764,#151765,#151766,#151767,#151768,#151769,#151770,#151771,
#151772,#151773,#151774,#151775,#151776,#151777,#151778,#151779,#151780,
#151781,#151782,#151783,#151784,#151785,#151786,#151787,#151788,#151789,
#151790,#151791,#151792,#151793,#151794,#151795,#151796,#151797,#151798,
#151799,#151800,#151801,#151802,#151803,#151804,#151805,#151806,#151807,
#151808,#151809,#151810,#151811,#151812,#151813,#151814,#151815,#151816,
#151817,#151818,#151819,#151820,#151821,#151822,#151823,#151824,#151825,
#151826,#151827,#151828,#151829,#151830,#151831,#151832,#151833,#151834,
#151835,#151836,#151837,#151838,#151839,#151840,#151841,#151842,#151843,
#151844,#151845,#151846,#151847,#151848,#151849,#151850,#151851,#151852,
#151853,#151854,#151855,#151856,#151857,#151858,#151859,#151860,#151861,
#151862,#151863,#151864,#151865,#151866,#151867,#151868,#151869,#151870,
#151871,#151872,#151873,#151874,#151875,#151876,#151877,#151878,#151879,
#151880,#151881,#151882,#151883,#151884,#151885,#151886,#151887,#151888,
#151889,#151890,#151891,#151892,#151893,#151894,#151895,#151896,#151897,
#151898,#151899,#151900,#151901,#151902,#151903,#151904,#151905,#151906,
#151907,#151908,#151909,#151910,#151911,#151912,#151913,#151914,#151915,
#151916,#151917,#151918,#151919,#151920,#151921,#151922,#151923,#151924,
#151925,#151926,#151927,#151928,#151929,#151930,#151931,#151932,#151933,
#151934,#151935,#151936,#151937,#151938,#151939,#151940,#151941,#151942,
#151943,#151944,#151945,#151946,#151947,#151948,#151949,#151950,#151951,
#151952,#151953,#151954,#151955,#151956,#151957,#151958,#151959,#151960,
#151961,#151962,#151963,#151964,#151965,#151966,#151967,#151968,#151969,
#151970,#151971,#151972,#151973,#151974,#151975,#151976,#151977,#151978,
#151979,#151980,#151981,#151982,#151983,#151984,#151985,#151986,#151987,
#151988,#151989,#151990,#151991,#151992,#151993,#151994,#151995,#151996,
#151997,#151998,#151999,#152000,#152001,#152002,#152003,#152004,#152005,
#152006,#152007,#152008,#152009,#152010,#152011,#152012,#152013,#152014,
#152015,#152016,#152017,#152018,#152019,#152020,#152021,#152022,#152023,
#152024,#152025,#152026,#152027,#152028,#152029,#152030,#152031,#152032,
#152033,#152034,#152035,#152036,#152037,#152038,#152039,#152040,#152041,
#152042,#152043,#152044,#152045,#152046,#152047,#152048,#152049,#152050,
#152051,#152052,#152053,#152054,#152055,#152056,#152057,#152058,#152059,
#152060,#152061,#152062,#152063,#152064,#152065,#152066,#152067,#152068,
#152069,#152070,#152071,#152072,#152073,#152074,#152075,#152076,#152077,
#152078,#152079,#152080,#152081,#152082,#152083,#152084,#152085,#152086,
#152087,#152088,#152089,#152090,#152091,#152092,#152093,#152094,#152095,
#152096,#152097,#152098,#152099,#152100,#152101,#152102,#152103,#152104,
#152105,#152106,#152107,#152108,#152109,#152110,#152111,#152112,#152113,
#152114,#152115,#152116,#152117,#152118,#152119,#152120,#152121,#152122,
#152123,#152124,#152125,#152126,#152127,#152128,#152129,#152130,#152131,
#152132,#152133,#152134,#152135,#152136,#152137,#152138,#152139,#152140,
#152141,#152142,#152143,#152144,#152145,#152146,#152147,#152148,#152149,
#152150,#152151,#152152,#152153,#152154,#152155,#152156,#152157,#152158,
#152159,#152160,#152161,#152162,#152163,#152164,#152165,#152166,#152167,
#152168,#152169,#152170,#152171,#152172,#152173,#152174,#152175,#152176,
#152177,#152178,#152179,#152180,#152181,#152182,#152183,#152184,#152185,
#152186,#152187,#152188,#152189,#152190,#152191,#152192,#152193,#152194,
#152195,#152196,#152197,#152198,#152199,#152200,#152201,#152202,#152203,
#152204,#152205,#152206,#152207,#152208,#152209,#152210,#152211,#152212,
#152213,#152214,#152215,#152216,#152217,#152218,#152219,#152220,#152221,
#152222,#152223,#152224,#152225,#152226,#152227,#152228,#152229,#152230,
#152231,#152232,#152233,#152234,#152235,#152236,#152237,#152238,#152239,
#152240,#152241,#152242,#152243,#152244,#152245,#152246,#152247,#152248,
#152249,#152250,#152251,#152252,#152253,#152254,#152255,#152256,#152257,
#152258,#152259,#152260,#152261,#152262,#152263,#152264,#152265,#152266,
#152267,#152268,#152269,#152270,#152271,#152272,#152273,#152274,#152275,
#152276,#152277,#152278,#152279,#152280,#152281,#152282,#152283,#152284,
#152285,#152286,#152287,#152288,#152289,#152290,#152291,#152292,#152293,
#152294,#152295,#152296,#152297,#152298,#152299,#152300,#152301,#152302,
#152303,#152304,#152305,#152306,#152307,#152308,#152309,#152310,#152311,
#152312,#152313,#152314,#152315,#152316,#152317,#152318,#152319,#152320,
#152321,#152322,#152323,#152324,#152325,#152326,#152327,#152328,#152329,
#152330,#152331,#152332,#152333,#152334,#152335,#152336,#152337,#152338,
#152339,#152340,#152341,#152342,#152343,#152344,#152345,#152346,#152347,
#152348,#152349,#152350,#152351,#152352,#152353,#152354,#152355,#152356,
#152357,#152358,#152359,#152360,#152361,#152362,#152363,#152364,#152365,
#152366,#152367,#152368,#152369,#152370,#152371,#152372,#152373,#152374,
#152375,#152376,#152377,#152378,#152379,#152380,#152381,#152382,#152383,
#152384,#152385,#152386,#152387,#152388,#152389,#152390,#152391,#152392,
#152393,#152394,#152395,#152396,#152397,#152398,#152399,#152400,#152401,
#152402,#152403,#152404,#152405,#152406,#152407,#152408,#152409,#152410,
#152411,#152412,#152413,#152414,#152415,#152416,#152417,#152418,#152419,
#152420,#152421,#152422,#152423,#152424,#152425,#152426,#152427,#152428,
#152429,#152430,#152431,#152432,#152433,#152434,#152435,#152436,#152437,
#152438,#152439,#152440,#152441,#152442,#152443,#152444,#152445,#152446,
#152447,#152448,#152449,#152450,#152451,#152452,#152453,#152454,#152455,
#152456,#152457,#152458,#152459,#152460,#152461,#152462,#152463,#152464,
#152465,#152466,#152467,#152468,#152469,#152470,#152471,#152472,#152473,
#152474,#152475,#152476,#152477,#152478,#152479,#152480,#152481,#152482,
#152483,#152484,#152485,#152486,#152487,#152488,#152489,#152490,#152491,
#152492,#152493,#152494,#152495,#152496,#152497,#152498,#152499,#152500,
#152501,#152502,#152503,#152504,#152505,#152506,#152507,#152508,#152509,
#152510,#152511,#152512,#152513,#152514,#152515,#152516,#152517,#152518,
#152519,#152520,#152521,#152522,#152523,#152524,#152525,#152526,#152527,
#152528,#152529,#152530,#152531,#152532,#152533,#152534,#152535,#152536,
#152537,#152538,#152539,#152540,#152541,#152542,#152543,#152544,#152545,
#152546,#152547,#152548,#152549,#152550,#152551,#152552,#152553,#152554,
#152555,#152556,#152557,#152558,#152559,#152560,#152561,#152562,#152563,
#152564,#152565,#152566,#152567,#152568,#152569,#152570,#152571,#152572,
#152573,#152574,#152575,#152576,#152577,#152578,#152579,#152580,#152581,
#152582,#152583,#152584,#152585,#152586,#152587,#152588,#152589,#152590,
#152591,#152592,#152593,#152594,#152595,#152596,#152597,#152598,#152599,
#152600,#152601,#152602,#152603,#152604,#152605,#152606,#152607,#152608,
#152609,#152610,#152611,#152612,#152613,#152614,#152615,#152616,#152617,
#152618,#152619,#152620,#152621,#152622,#152623,#152624,#152625,#152626,
#152627,#152628,#152629,#152630,#152631,#152632,#152633,#152634,#152635,
#152636,#152637,#152638,#152639,#152640,#152641,#152642,#152643,#152644,
#152645,#152646,#152647,#152648,#152649,#152650,#152651,#152652,#152653,
#152654,#152655,#152656,#152657,#152658,#152659,#152660,#152661,#152662,
#152663,#152664,#152665,#152666,#152667,#152668,#152669,#152670,#152671,
#152672,#152673,#152674,#152675,#152676,#152677,#152678,#152679,#152680,
#152681,#152682,#152683,#152684,#152685,#152686,#152687,#152688,#152689,
#152690,#152691,#152692,#152693,#152694,#152695,#152696,#152697,#152698,
#152699,#152700,#152701,#152702,#152703,#152704,#152705,#152706,#152707,
#152708,#152709,#152710,#152711,#152712,#152713,#152714,#152715,#152716,
#152717,#152718,#152719,#152720,#152721,#152722,#152723,#152724,#152725,
#152726,#152727,#152728,#152729,#152730,#152731,#152732,#152733,#152734,
#152735,#152736,#152737,#152738,#152739,#152740,#152741,#152742,#152743,
#152744,#152745,#152746,#152747,#152748,#152749,#152750,#152751,#152752,
#152753,#152754,#152755,#152756,#152757,#152758,#152759,#152760,#152761,
#152762,#152763,#152764,#152765,#152766,#152767,#152768,#152769,#152770,
#152771,#152772,#152773,#152774,#152775,#152776,#152777,#152778,#152779,
#152780,#152781,#152782,#152783,#152784,#152785,#152786,#152787,#152788,
#152789,#152790,#152791,#152792,#152793,#152794,#152795,#152796,#152797,
#152798,#152799,#152800,#152801,#152802,#152803,#152804,#152805,#152806,
#152807,#152808,#152809,#152810,#152811,#152812,#152813,#152814,#152815,
#152816,#152817,#152818,#152819,#152820,#152821,#152822,#152823,#152824,
#152825,#152826,#152827)),.UNSPECIFIED.,.T.,.F.,.F.)
B_SPLINE_SURFACE_WITH_KNOTS((3,2,2,2,3),(4,1,1,1,1,1,1,1,1,1,1,1,1,1,1,
1,1,1,1,1,1,1,1,1,1,1,1,1,1,1,1,1,1,1,1,1,1,1,1,1,1,1,1,1,1,1,1,1,1,1,1,
1,1,1,1,1,1,1,1,1,1,1,1,1,1,1,1,1,1,1,1,1,1,1,1,1,1,1,1,1,1,1,1,1,1,1,1,
1,1,1,1,1,1,1,1,1,1,1,1,1,1,1,1,1,1,1,1,1,1,1,1,1,1,1,1,1,1,1,1,1,1,1,1,
1,1,1,1,1,1,1,1,1,1,1,1,1,1,1,1,1,1,1,1,1,1,1,1,1,1,1,1,1,1,1,1,1,1,1,1,
1,1,1,1,1,1,1,1,1,1,1,1,1,1,1,1,1,1,1,1,1,1,1,1,1,1,1,1,1,1,1,1,1,1,1,1,
1,1,1,1,1,1,1,1,1,1,1,1,1,1,1,1,1,1,1,1,1,1,1,1,1,1,1,1,1,1,1,1,1,1,1,1,
1,1,1,1,1,1,1,1,1,1,1,1,1,1,1,1,1,1,1,1,1,1,1,1,1,1,1,1,1,1,1,1,1,1,1,1,
1,1,1,1,1,1,1,1,1,1,1,1,1,1,1,1,1,1,1,1,1,1,1,1,1,1,1,1,1,1,1,1,1,1,1,1,
1,1,1,1,1,1,1,1,1,1,1,1,1,1,1,1,1,1,1,1,1,1,1,1,1,1,1,1,1,1,1,1,1,1,1,1,
1,1,1,1,1,1,1,1,1,1,1,1,1,1,1,1,1,1,1,1,1,1,1,1,1,1,1,1,1,1,1,1,1,1,1,1,
1,1,1,1,1,1,1,1,1,1,1,1,1,1,1,1,1,1,1,1,1,1,1,1,1,1,1,1,1,1,1,1,1,1,1,1,
1,1,1,1,1,1,1,1,1,1,1,1,1,1,1,1,1,1,1,1,1,1,1,1,1,1,1,1,1,1,1,1,1,1,1,1,
1,1,1,1,1,1,1,1,1,1,1,1,1,1,1,1,1,1,1,1,1,1,1,1,1,1,1,1,1,1,1,1,1,1,1,1,
1,1,1,1,1,1,1,1,1,1,1,1,1,1,1,1,1,1,1,1,1,1,1,1,1,1,1,1,1,1,1,1,1,1,1,1,
1,1,1,1,1,1,1,1,1,1,1,1,1,1,1,1,1,1,1,1,1,1,1,1,1,1,1,1,1,1,1,1,1,1,1,1,
1,1,1,1,1,1,1,1,1,1,1,1,1,1,1,1,1,1,1,1,1,1,1,1,1,1,1,1,1,1,1,1,1,1,1,1,
1,1,1,1,1,1,1,1,1,1,1,1,1,1,1,1,1,1,1,1,1,1,1,1,1,1,1,1,1,1,1,1,1,1,1,1,
1,1,1,1,1,1,1,1,1,1,1,1,1,1,1,1,1,1,1,1,1,1,1,1,1,1,1,1,1,1,1,1,1,1,1,1,
1,1,1,1,1,1,1,1,1,1,1,1,1,1,1,1,1,1,1,1,1,1,1,1,1,1,1,1,1,1,1,1,1,1,1,1,
1,1,1,1,1,1,1,1,1,1,1,1,1,1,1,1,1,1,1,1,1,1,1,1,1,1,1,1,1,1,1,1,1,1,1,1,
1,1,1,1,1,1,1,1,1,1,1,1,1,1,1,1,1,1,1,1,1,1,1,1,1,1,1,1,1,1,1,1,1,1,1,1,
1,1,1,1,1,1,1,1,1,1,1,1,1,1,1,1,1,1,1,1,1,1,1,1,1,1,1,1,1,1,1,1,1,1,1,1,
1,1,1,1,1,1,1,1,1,1,1,1,1,1,1,1,1,1,1,1,1,1,1,1,1,1,1,1,1,1,1,1,1,1,1,1,
1,1,1,1,1,1,1,1,1,1,1,1,1,1,1,1,1,1,1,1,1,1,1,1,1,1,1,1,1,1,1,1,1,1,1,1,
1,1,1,1,1,1,1,1,1,1,1,1,1,1,1,1,1,1,1,1,1,1,1,1,1,1,1,1,1,1,1,1,1,1,1,1,
1,1,1,1,1,1,1,1,1,1,1,1,1,1,1,1,1,1,1,1,1,1,1,1,1,1,1,1,1,1,1,1,1,1,1,1,
1,1,1,1,1,1,1,1,1,1,1,1,1,1,1,1,1,1,1,1,1,1,1,1,1,1,1,1,1,1,1,1,1,1,1,1,
1,1,1,1,1,1,1,1,1,1,1,1,1,1,1,1,1,1,1,1,1,1,1,1,1,1,1,1,1,1,1,1,1,1,1,1,
1,1,1,1,1,1,1,1,1,1,1,1,1,1,1,1,1,1,1,1,1,1,1,1,1,1,1,1,1,1,1,1,1,1,1,1,
1,1,1,1,1,1,1,1,1,1,1,1,1,1,1,1,1,1,1,1,1,1,1,1,1,1,1,1,1,1,1,1,1,1,1,1,
1,1,1,1,1,1,1,1,1,1,1,1,1,1,1,1,1,1,1,1,1,1,1,1,1,1,1,1,1,1,1,1,1,1,1,1,
1,1,1,1,1,1,1,1,1,1,1,1,1,1,1,1,1,1,1,1,1,1,1,1,1,1,1,1,1,1,1,1,1,1,1,1,
1,1,1,1,1,1,1,1,1,1,1,1,1,1,1,1,1,1,1,1,1,1,1,1,1,1,1,1,1,1,1,1,1,1,1,1,
1,1,1,1,1,1,1,1,1,1,1,1,1,1,1,1,1,1,1,1,1,1,1,1,1,1,1,1,1,1,1,1,1,1,1,1,
1,1,1,1,1,1,1,1,1,1,1,1,1,1,1,1,1,1,1,1,1,1,1,1,1,1,1,1,1,1,1,1,1,1,1,1,
1,1,1,1,1,1,1,1,1,1,1,1,1,1,1,1,1,1,1,1,1,1,1,1,1,1,1,1,1,1,1,1,1,1,1,1,
1,1,1,1,1,1,1,1,1,1,1,1,1,1,1,1,1,1,1,1,1,1,1,1,1,1,1,1,1,1,1,1,1,1,1,1,
1,1,1,1,1,1,1,1,1,1,1,1,1,1,1,1,1,1,1,1,1,1,1,1,1,1,1,1,1,1,1,1,1,1,1,1,
1,1,1,1,1,1,1,1,1,1,1,1,1,1,1,1,1,1,1,1,1,1,1,1,1,1,1,1,1,1,1,1,1,1,1,1,
1,1,1,1,1,1,1,1,1,1,1,1,1,1,1,1,1,1,1,1,1,1,1,1,1,1,1,1,1,1,1,1,1,1,1,1,
1,1,1,1,1,1,1,1,1,1,1,1,1,1,1,1,1,1,1,1,1,1,1,1,1,1,1,1,1,1,1,1,1,1,1,1,
1,1,1,1,1,1,1,1,1,1,1,1,1,1,1,1,1,1,1,1,1,1,1,1,1,1,1,1,1,1,1,1,1,1,1,1,
1,1,1,1,1,1,1,1,1,1,1,1,1,1,1,1,1,1,1,1,1,1,1,1,1,1,1,1,1,1,1,1,1,1,1,1,
1,1,1,1,1,1,1,1,1,1,1,1,1,1,1,1,1,1,1,1,1,1,1,1,1,1,1,1,1,1,1,1,1,1,1,1,
1,1,1,1,1,1,1,1,1,1,1,1,1,1,1,1,1,1,1,1,1,1,1,1,1,1,1,1,1,1,1,1,1,1,1,1,
1,1,1,1,1,1,1,1,1,1,1,1,1,1,1,1,1,1,1,1,1,1,1,1,1,1,1,1,1,1,1,1,1,1,1,1,
1,1,1,1,1,1,1,1,1,1,1,1,1,1,1,1,1,1,1,1,1,1,1,1,1,1,1,1,1,1,1,1,1,1,1,1,
1,1,1,1,1,1,1,1,1,1,1,1,1,1,1,1,1,1,1,1,1,1,1,1,1,1,1,1,1,1,1,1,1,1,1,1,
1,1,1,1,1,1,1,1,1,1,1,1,1,1,1,1,1,1,1,1,1,1,1,1,1,1,1,1,1,1,1,1,1,1,1,1,
1,1,1,1,1,1,1,1,1,1,1,1,1,1,1,1,1,1,1,1,1,1,1,1,1,1,1,1,1,1,1,1,1,1,1,1,
1,1,1,1,1,1,1,1,1,1,1,1,1,1,1,1,1,1,1,1,1,1,1,1,1,1,1,1,1,1,1,1,1,1,1,1,
1,1,1,1,1,1,1,1,1,1,1,1,1,1,1,1,1,1,1,1,1,1,1,1,1,1,1,1,1,1,1,1,1,1,1,1,
1,1,1,1,1,1,1,1,1,1,1,1,1,1,1,1,1,1,1,1,1,1,1,1,1,1,1,1,1,1,1,1,1,1,1,1,
1,1,1,1,1,1,1,1,1,1,1,1,1,1,1,1,1,1,1,1,1,1,1,1,1,1,1,1,1,1,1,1,1,1,1,1,
1,1,1,1,1,1,1,1,1,1,1,1,1,1,1,1,1,1,1,1,1,1,1,1,1,1,1,1,1,1,1,1,1,1,1,1,
1,1,1,1,1,1,1,1,1,1,1,1,1,1,1,1,1,1,1,1,1,1,1,1,1,1,1,1,1,1,1,1,1,1,1,1,
1,1,1,1,1,1,1,1,1,1,1,1,1,1,1,1,1,4),(0.,0.117809724509617,0.235619449019234,
0.353429173528852,0.471238898038469),(0.,0.01797683372391,0.286633051710584,
0.555289278308216,0.823945516665782,1.09260176953922,1.36125803873948,1.62991432588463,
1.89857063164012,2.16722695661301,2.43588330050525,2.70453966304674,2.9731960431531,
3.24185243981471,3.51050885133453,3.77916527610465,4.04782171198515,4.31647815691489,
4.58513460847725,4.85379106430677,5.12244752187208,5.39110397865606,5.65976043217153,
5.92841687990537,6.19707331956994,6.46572974881596,6.73438616570634,7.00304256821933,
7.2716989549161,7.5403553242696,7.809011675483,8.07766800769526,8.34632432089157,
8.61498061505147,8.8836368910788,9.15229314997201,9.4209493936865,9.68960562442157,
9.95826184531348,10.226918059948,10.4955742727586,10.7642304884925,11.0328867113173,
11.3015429448574,11.5701991918227,11.8388554546081,12.1075117346518,12.3761680332469,
12.6448243507434,12.9134806874637,13.1821370428496,13.450793416388,13.7194498067883,
13.9881062128412,14.2567626326955,14.5254190645885,14.7940755062772,15.0627319555912,
15.3313884100611,15.6000448672586,15.8687013246492,16.1373577797,16.4060142299691,
16.6746706729765,16.9433271065265,17.2119835283531,17.4806399366567,17.7492963295502,
18.0179527057767,18.286609063996,18.555265403637,18.8239217240786,19.0925780255742,
19.3612343083975,19.6298905737625,19.898546823017,20.1672030584666,20.4358592827168,
20.7045154992928,20.973171712245,21.2418279262962,21.5104841459723,21.7791403749736,
22.0477966165324,22.316452872948,22.585109146262,22.8537654375589,23.1224217478187,
23.3910780770929,23.6597344254327,23.9283907920352,24.197047176159,24.4657035763222,
24.7343599911301,25.0030164185931,25.2716728568073,25.5403293034427,25.8089857562333,
26.0776422126729,26.3462986702843,26.6149551265448,26.8836115789212,27.1522680250308,
27.4209244624423,27.6895808890659,27.9582373027346,28.2268937018004,28.4955500845261,
28.7642064498512,29.0328627966379,29.3015191245544,29.5701754332357,29.838831723217,
30.1074879950829,30.3761442503694,30.6448004907916,30.9134567190168,31.1821129380756,
31.450769151893,31.7194253649682,31.9880815819663,32.2567378070174,32.5253940433706,
32.7940502938785,33.0627065604467,33.3313628447765,33.6000191476151,33.8686754696427,
34.1373318106287,34.405988170366,34.6746445478242,34.9433009420458,35.2119573513747,
35.480613774244,35.7492702085419,36.0179266522368,36.2865831029275,36.5552395582669,
36.8238960157264,37.0925524727952,37.3612089269773,37.6298653757534,37.8985218168153,
38.1671782477952,38.4358346667239,38.7044910715485,38.9731474607866,39.2418038328672,
39.5104601869391,39.7791165220837,40.0477728382212,40.3164291352602,40.5850854140292,
40.8537416754418,41.1223979213679,41.3910541539077,41.6597103761025,41.9283665914244,
42.1970228042084,42.4656790192,42.7343352406829,43.0029914723808,43.2716477171096,
43.540303977354,43.8089602546436,44.0776165503516,44.3462728649052,44.614929198697,
44.883585551232,45.1522419220568,45.4208983099307,45.6895547136931,45.9582111315299,
46.2268675617156,46.4955240020317,46.7641804503338,47.0328369041642,47.3014933611089,
47.5701498186329,47.8388062742058,48.107462725373,48.3761191696448,48.6447756048012,
48.9134320285537,49.1820884390673,49.4507448344197,49.7194012133072,49.9880575743413,
50.2567139168934,50.5253702402807,50.7940265446884,51.0626828303152,51.3313390982961,
51.5999953498901,51.8686515873141,52.1373078130706,52.4059640305862,52.6746202437936,
52.9432764573682,53.211932675918,53.480588903259,53.7492451427202,54.0179013967021,
54.2865576673334,54.5552139557853,54.823870263115,55.0925265894471,55.3611829348992,
55.6298392987282,55.8984956802486,56.1671520780245,56.4358084907065,56.7044649163381,
56.9731213530494,57.2417777985307,57.5104342505384,57.7790907065743,58.0477471641719,
58.3164036208043,58.5850600739368,58.8537165211707,59.1223729600609,59.39102938849,
59.6596858042645,59.9283422056975,60.1969985910129,60.4656549590995,60.7343113087676,
61.0029676396243,61.2716239512389,61.540280244075,61.808936518638,62.0775927763821,
62.3462490189291,62.6149052488546,62.8835614690812,63.1522176834332,63.4208738963055,
63.6895301124163,63.9581863359981,64.2268425704115,64.4954988186027,64.7641550825741,
65.0328113641112,65.3014676640435,65.5701239831253,65.8387803211949,66.1074366781083,
66.3760930528907,66.6447494446373,66.9134058517341,67.1820622726558,67.4507187053199,
67.7193751477252,67.988031597487,68.256688052277,68.5253445095709,68.7940009668648,
69.0626574216546,69.3313138714164,69.5999703138218,69.8686267464858,70.1372831674076,
70.4059395745042,70.6745959662509,70.9432523410334,71.2119086979469,71.4805650360164,
71.7492213550982,72.0178776550306,72.2865339365675,72.5551902005389,72.8238464487301,
73.0925026831433,73.3611589067251,73.6298151228357,73.8984713357081,74.1671275500599,
74.4357837702864,74.7044400002118,74.9730962427587,75.2417525005027,75.5104087750655,
75.7790650679015,76.047721379516,76.3163777103726,76.5850340600405,76.853690428127,
77.1223468134422,77.391003214875,77.6596596306495,77.9283160590784,78.1969724979684,
78.4656289452021,78.7342853983344,79.0029418549666,79.2715983125641,79.5402547685998,
79.8089112206075,80.0775676660886,80.3462241027997,80.6148805284312,80.8835369411131,
81.1521933388889,81.4208497204091,81.689506084238,81.9581624296899,82.2268187560219,
82.4954750633515,82.7641313518033,83.0327876224345,83.3014438764161,83.5701001158772,
83.838756343218,84.1074125617677,84.3760687753422,84.6447249885494,84.913381206065,
85.1820374318212,85.4506936692451,85.719349920839,85.9880061888197,86.2566624744465,
86.5253187788541,86.7939751022413,87.0626314447932,87.3312878058273,87.5999441847146,
87.8686005800667,88.1372569905802,88.4059134143327,88.6745698494889,88.9432262937606,
89.2118827449277,89.4805392005005,89.7491956580243,90.0178521149689,90.2865085687992,
90.5551650171012,90.8238214574172,91.0924778876028,91.3611343054394,91.6297907092016,
91.8984470970753,92.1671034679,92.4357598204347,92.7044161542264,92.9730724687798,
93.2417287644878,93.5103850417773,93.7790413020216,94.0476975467502,94.3163537784479,
94.5850099999307,94.8536662149221,95.1223224277061,95.390978643028,95.6596348652226,
95.9282910977624,96.1969473436883,96.4656036051009,96.7342598838697,97.0029161809086,
97.2715724970461,97.5402288321905,97.8088851862623,98.0775415583427,98.3461979475807,
98.6148543524051,98.8835107713336,99.1521672023136,99.4208236433754,99.6894800921513,
99.9581365463333,100.226793003402,100.495449460861,100.7641059162,101.032762366891,
101.301418810586,101.570075244884,101.838731667753,102.107388077082,102.376044471303,
102.644700848761,102.913357208498,103.182013549484,103.450669871511,103.71932617435,
103.98798245868,104.256638725248,104.525294975755,104.793951212108,105.062607437159,
105.331263654157,105.599919867233,105.86857608105,106.137232300108,106.405888528334,
106.674544768756,106.943201024042,107.211857295908,107.480513585889,107.74916989457,
108.017826222487,108.286482569273,108.555138934598,108.823795317324,109.09245171639,
109.361108130058,109.629764556682,109.898420994093,110.167077440202,110.435733892579,
110.704390348839,110.97304680645,111.24170326289,111.51035971568,111.779016162316,
112.04767260053,112.316329027993,112.5849854428,112.853641842963,113.122298227087,
113.39095459369,113.659610942029,113.928267271303,114.196923581563,114.46557987286,
114.734236146174,115.002892402589,115.271548644148,115.540204873149,115.808861092825,
116.077517306876,116.346173519828,116.614829736404,116.883485960654,117.152142196103,
117.420798445358,117.689454710722,117.958110993546,118.226767295041,118.495423615483,
118.764079955123,119.032736313343,119.301392689569,119.570049082462,119.838705490766,
120.107361912592,120.376018346142,120.644674789149,120.913331239418,121.181987694469,
121.45064415186,121.719300609057,121.987957063527,122.256613512841,122.525269954529,
122.793926386422,123.062582806276,123.331239212329,123.599895602729,123.868551976268,
124.137208331653,124.405864668374,124.67452098587,124.943177284465,125.211833564508,
125.480489827294,125.749146074259,126.017802307799,126.286458530624,126.555114746357,
126.823770959168,127.092427173802,127.361083394694,127.629739625429,127.898395869143,
128.167052128037,128.435708404064,128.704364698224,128.97302101142,129.241677343633,
129.510333694846,129.7789900642,130.047646450897,130.31630285341,130.5849592703,
130.853615699547,131.122272139211,131.390928586945,131.659585040461,131.928241497245,
132.19689795481,132.46555441064,132.734210862202,133.002867307132,133.271523743013,
133.540180167783,133.808836579303,134.077492975965,134.346149356071,134.614805718613,
134.883462062505,135.152118387478,135.420774693234,135.689430980379,135.958087249579,
136.226743502453,136.49539974081,136.76405596741,137.032712185392,137.301368398783,
137.570024612174,137.838680830155,138.107337056755,138.375993295112,138.644649547986,
138.913305817186,139.181962104332,139.450618410087,139.71927473506,139.987931078952,
140.256587441494,140.525243821601,140.793900218262,141.062556629782,141.331213054552,
141.599869490433,141.868525935363,142.137182386925,142.405838842755,142.67449530032,
142.943151757104,143.21180821062,143.480464658354,143.749121098019,144.017777527265,
144.286433944155,144.555090346668,144.823746733365,145.092403102719,145.361059453932,
145.629715786145,145.898372099341,146.167028393501,146.435684669529,146.704340928422,
146.972997172137,147.241653402872,147.510309623764,147.778965838398,148.047622051209,
148.316278266943,148.584934489768,148.853590723308,149.122246970274,149.390903233059,
149.659559513103,149.928215811698,150.196872129195,150.465528465915,150.734184821301,
151.00284119484,151.27149758524,151.540153991293,151.808810411148,152.077466843041,
152.34612328473,152.614779734044,152.883436188514,153.152092645711,153.420749103102,
153.689405558153,153.958062008422,154.22671845143,154.49537488498,154.764031306806,
155.03268771511,155.301344108004,155.57000048423,155.838656842449,156.107313182091,
156.375969502532,156.644625804028,156.913282086851,157.181938352216,157.450594601471,
157.719250836921,157.987907061171,158.256563277747,158.525219490699,158.793875704751,
159.062531924427,159.331188153428,159.599844394987,159.868500651403,160.137156924717,
160.405813216014,160.674469526274,160.943125855548,161.211782203888,161.480438570491,
161.749094954615,162.017751354778,162.286407769586,162.555064197049,162.823720635263,
163.092377081899,163.361033534689,163.629689991129,163.898346448741,164.167002905001,
164.435659357378,164.704315803488,164.972972240899,165.241628667523,165.510285081192,
165.778941480257,166.047597862983,166.316254228308,166.584910575095,166.853566903012,
167.122223211693,167.390879501675,167.659535773541,167.928192028827,168.19684826925,
168.465504497475,168.734160716534,169.002816930351,169.271473143427,169.540129360425,
169.808785585476,170.077441821829,170.346098072337,170.614754338905,170.883410623235,
171.152066926074,171.420723248102,171.689379589088,171.958035948825,172.226692326284,
172.495348720505,172.764005129834,173.032661552704,173.301317987002,173.569974430697,
173.838630881388,174.107287336727,174.375943794187,174.644600251255,174.913256705437,
175.181913154214,175.450569595276,175.719226026256,175.987882445184,176.256538850009,
176.525195239247,176.793851611328,177.0625079654,177.331164300545,177.599820616682,
177.868476913721,178.137133192491,178.405789453903,178.674445699829,178.943101932369,
179.211758154564,179.480414369886,179.74907058267,180.017726797662,180.286383019145,
180.555039250843,180.823695495572,181.092351755816,181.361008033106,181.629664328814,
181.898320643368,182.16697697716,182.435633329695,182.70428970052,182.972946088394,
183.241602492156,183.510258909993,183.778915340179,184.047571780495,184.316228228797,
184.584884682628,184.853541139572,185.122197597096,185.39085405267,185.659510503837,
185.928166948109,186.196823383265,186.465479807018,186.734136217531,187.002792612884,
187.271448991771,187.540105352806,187.808761695358,188.077418018745,188.346074323153,
188.61473060878,188.883386876761,189.152043128355,189.420699365779,189.689355591536,
189.958011809051,190.226668022259,190.495324235834,190.763980454383,191.032636681725,
191.301292921186,191.569949175168,191.838605445799,192.107261734251,192.375918041581,
192.644574367913,192.913230713365,193.181887077194,193.450543458715,193.719199856491,
193.987856269173,194.256512694805,194.525169131516,194.793825576997,195.062482029005,
195.331138485041,195.599794942639,195.868451399271,196.137107852404,196.405764299638,
196.674420738528,196.943077166957,197.211733582732,197.480389984165,197.749046369481,
198.017702737567,198.286359087236,198.555015418092,198.823671729707,199.092328022543,
199.360984297106,199.62964055485,199.898296797397,200.166953027323,200.43560924755,
200.704265461902,200.972921674774,201.241577890885,201.510234114467,201.77889034888,
202.047546597072,202.316202861043,202.584859142581,202.853515442513,203.122171761595,
203.390828099665,203.659484456579,203.928140831361,204.196797223108,204.465453630205,
204.734110051127,205.002766483791,205.271422926197,205.540079375959,205.808735830749,
206.077392288043,206.346048745337,206.614705200127,206.883361649889,207.152018092295,
207.420674524959,207.689330945881,207.957987352978,208.226643744725,208.495300119508,
208.763956476421,209.032612814491,209.301269133573,209.569925433505,209.838581715043,
210.107237979014,210.375894227206,210.644550461619,210.913206685201,211.181862901312,
211.450519114184,211.719175328536,211.987831548763,212.256487778689,212.525144021236,
212.79380027898,213.062456553543,213.331112846379,213.599769157994,213.868425488851,
214.137081838519,214.405738206606,214.674394591921,214.943050993354,215.211707409129,
215.480363837558,215.749020276448,216.017676723682,216.286333176815,216.554989633447,
216.823646091045,217.092302547081,217.360958999089,217.62961544457,217.898271881281,
218.166928306913,218.435584719595,218.704241117371,218.972897498892,219.241553862721,
219.510210208173,219.778866534505,220.047522841835,220.316179130287,220.584835400918,
220.8534916549,221.122147894361,221.390804121702,221.659460340252,221.928116553827,
222.196772767034,222.46542898455,222.734085210306,223.00274144773,223.271397699324,
223.540053967305,223.808710252932,224.07736655734,224.346022880728,224.61467922328,
224.883335584314,225.151991963201,225.420648358554,225.689304769068,225.95796119282,
226.226617627977,226.495274072249,226.763930523416,227.032586978989,227.301243436513,
227.569899893458,227.838556347288,228.10721279559,228.375869235907,228.644525666093,
228.913182083929,229.181838487692,229.450494875566,229.719151246391,229.987807598926,
230.256463932718,230.525120247271,230.79377654298,231.062432820269,231.331089080514,
231.599745325243,231.868401556941,232.137057778424,232.405713993415,232.674370206199,
232.943026421521,233.211682643716,233.480338876256,233.748995122182,234.017651383595,
234.286307662364,234.554963959403,234.823620275541,235.092276610685,235.360932964757,
235.629589336838,235.898245726076,236.166902130901,236.43555854983,236.70421498081,
236.972871421872,237.241527870648,237.51018432483,237.778840781899,238.047497239359,
238.316153694698,238.584810145389,238.853466589084,239.122123023382,239.390779446251,
239.65943585558,239.928092249802,240.19674862726,240.465404986998,240.734061327984,
241.002717650011,241.27137395285,241.54003023718,241.808686503748,242.077342754256,
242.345998990609,242.614655215661,242.883311432659,243.151967645734,243.420623859552,
243.68928007861,243.957936306836,244.226592547258,244.495248802545,244.763905074411,
245.032561364392,245.301217673074,245.56987400099,245.838530347777,246.107186713102,
246.375843095828,246.644499494894,246.913155908563,247.181812335186,247.450468772598,
247.719125218708,247.987781671084,248.256438127345,248.525094584956,248.793751041396,
249.062407494187,249.331063940822,249.599720379036,249.8683768065,250.137033221308,
250.405689621471,250.674346005595,250.943002372197,251.211658720537,251.480315049812,
251.748971360071,252.017627651368,252.286283924683,252.554940181098,252.823596422657,
253.092252651658,253.360908871335,253.629565085386,253.898221298338,254.166877514914,
254.435533739165,254.704189974614,254.972846223869,255.241502489234,255.510158772057,
255.778815073553,256.047471393995,256.316127733635,256.584784091854,256.85344046808,
257.122096860973,257.390753269276,257.659409691102,257.928066124652,258.196722567659,
258.465379017928,258.734035472978,259.002691930368,259.271348387566,259.540004842035,
259.808661291349,260.077317733037,260.345974164929,260.614630584783,260.883286990836,
261.151943381235,261.420599754774,261.689256110159,261.957912446879,262.226568764375,
262.49522506297,262.763881343014,263.032537605798,263.301193852763,263.569850086303,
263.838506309127,264.107162524861,264.375818737671,264.644474952305,264.913131173196,
265.181787403931,265.450443647645,265.719099906538,265.987756182565,266.256412476724,
266.52506878992,266.793725122132,267.062381473345,267.331037842698,267.599694229394,
267.868350631907,268.137007048797,268.405663478042,268.674319917706,268.94297636544,
269.211632818955,269.480289275739,269.748945733304,270.017602189133,270.286258640695,
270.554915085624,270.823571521504,271.092227946274,271.360884357793,271.629540754454,
271.89819713456,272.166853497101,272.435509840993,272.704166165965,272.97282247172,
273.241478758865,273.510135028065,273.778791280938,274.047447519295,274.316103745894,
274.584759963875,274.853416177266,275.122072390656,275.390728608637,275.659384835237,
275.928041073593,276.196697326466,276.465353595666,276.734009882811,277.002666188566,
277.271322513539,277.53997885743,277.808635219972,278.077291600077,278.345947996739,
278.614604408258,278.883260833028,279.151917268908,279.420573713837,279.689230165399,
279.957886621228,280.226543078793,280.495199535576,280.763855989092,281.032512436825,
281.301168876489,281.569825305735,281.838481722625,282.107138125138,282.375794511834,
282.644450881187,282.9131072324,283.181763564612,283.450419877808,283.719076171967,
283.987732447994,284.256388706887,284.525044950601,284.793701181336,285.062357402228,
285.331013616862,285.599669829672,285.868326045405,286.136982268229,286.405638501769,
286.674294748734,286.942951011519,287.211607291562,287.480263590157,287.748919907653,
288.017576244373,288.286232599758,288.554888973296,288.823545363696,289.092201769749,
289.360858189603,289.629514621495,289.898171063183,290.166827512497,290.435483966966,
290.704140424163,290.972796881554,291.241453336604,291.510109786873,291.77876622988,
292.047422663429,292.316079085255,292.584735493559,292.853391886452,293.122048262678,
293.390704620897,293.659360960537,293.928017280978,294.196673582474,294.465329865297,
294.733986130661,295.002642379915,295.271298615364,295.539954839614,295.808611056189,
296.077267269141,296.345923483192,296.614579702867,296.883235931868,297.151892173427,
297.420548429842,297.689204703155,297.957860994452,298.226517304711,298.495173633985,
298.763829982324,299.032486348927,299.30114273305,299.569799133212,299.83845554802,
300.107111975482,300.375768413696,300.644424860331,300.913081313121,301.181737769561,
301.450394227172,301.719050683432,301.987707135808,302.256363581917,302.525020019328,
302.793676445951,303.062332859619,303.330989258684,303.59964564141,303.868302006734,
304.136958353521,304.405614681437,304.674270990118,304.942927280098,305.211583551964,
305.48023980725,305.748896047671,306.017552275896,306.286208494954,306.554864708772,
306.823520921846,307.092177138844,307.360833363895,307.629489600247,307.898145850755,
308.166802117323,308.435458401652,308.70411470449,308.972771026517,309.241427367503,
309.51008372724,309.778740104698,310.047396498919,310.316052908247,310.584709331116,
310.853365765414,311.122022209108,311.390678659798,311.659335115137,311.927991572596,
312.196648029665,312.465304483846,312.733960932622,313.002617373684,313.271273804663,
313.539930223591,313.808586628416,314.077243017653,314.345899389733,314.614555743805,
314.883212078949,315.151868395086,315.420524692125,315.689180970894,315.957837232306,
316.226493478231,316.495149710771,316.763805932965,317.032462148286,317.30111836107,
317.569774576061,317.838430797543,318.107087029241,318.375743273969,318.644399534213,
318.913055811502,319.18171210721,319.450368421763,319.719024755555,319.987681108089,
320.256337478914,320.524993866787,320.793650270549,321.062306688385,321.33096311857,
321.599619558886,321.868276007188,322.136932461018,322.405588917962,322.674245375486,
322.942901831059,323.211558282225,323.480214726497,323.748871161653,324.017527585405,
324.286183995918,324.55484039127,324.823496770157,325.09215313119,325.360809473742,
325.629465797129,325.898122101536,326.166778387163,326.435434655143,326.704090906737,
326.97274714416,327.241403369916,327.510059587432,327.778715800638,328.047372014213,
328.316028232762,328.584684460102,328.853340699563,329.121996953545,329.390653224175,
329.659309512627,329.927965819956,330.196622146288,330.46527849174,330.733934855568,
331.002591237088,331.271247634863,331.539904047545,331.808560473176,332.077216909887,
332.345873355368,332.614529807375,332.883186263411,333.151842721008,333.42049917764,
333.689155630772,333.957812078005,334.226468516895,334.495124945324,334.763781361098,
335.03243776253,335.301094147845,335.569750515931,335.838406865599,336.107063196455,
336.375719508069,336.644375800905,336.913032075468,337.181688333211,337.450344575758,
337.719000805683,337.987657025909,338.256313240261,338.524969453133,338.793625669243,
339.062281892824,339.330938127237,339.599594375428,339.868250639399,340.136906920936,
340.405563220868,340.674219539949,340.942875878019,341.211532234932,341.480188609714,
341.74884500146,342.017501408557,342.286157829478,342.554814262142,342.823470704547,
343.092127154308,343.360783609098,343.629440066391,343.898096523685,344.166752978475,
344.435409428236,344.704065870641,344.972722303305,345.241378724226,345.510035131323,
345.778691523069,346.047347897851,346.316004254764,346.584660592834,346.853316911915,
347.121973211847,347.390629493384,347.659285757355,347.927942005546,348.196598239959,
348.46525446354,348.733910679651,349.002566892523,349.271223106874,349.5398793271,
349.808535557025,350.077191799572,350.345848057315,350.614504331878,350.883160624714,
351.151816936328,351.420473267184,351.689129616852,351.957785984938,352.226442370253,
352.495098771685,352.76375518746,353.032411615888,353.301068054778,353.569724502012,
353.838380955144,354.107037411776,354.375693869373,354.644350325408,354.913006777416,
355.181663222896,355.450319659607,355.718976085238,355.98763249792,356.256288895695,
356.524945277215,356.793601641044,357.062257986496,357.330914312827,357.599570620156,
357.868226908608,358.136883179239,358.40553943322,358.674195672681,358.942851900021,
359.211508118571,359.480164332145,359.748820545352,360.017476762867,360.286132988623,
360.554789226047,360.82344547764,361.09210174562,361.360758031247,361.629414335654,
361.898070659041,362.166727001593,362.435383362626,362.704039741513,362.972696136865,
363.241352547378,363.510008971131,363.778665406287,364.047321850558,364.315978301725,
364.584634757297,364.853291214821,365.121947671765,365.390604125595,365.659260573897,
365.927917014213,366.196573444398,366.465229862234,366.733886265996,367.002542653869,
367.271199024694,367.539855377228,367.808511711019,368.077168025573,368.34582432128,
368.614480598569,368.883136858813,369.151793103542,369.420449335239,369.689105556722,
369.957761771713,370.226417984496,370.495074199818,370.763730422012,371.032386654551,
371.301042900477,371.569699161889,371.838355440658,372.107011737697,372.375668053834,
372.644324388978,372.912980743049,373.18163711513,373.450293504367,373.718949909191,
373.98760632812,374.256262759099,374.524919200161,374.793575648936,375.062232103118,
375.330888560186,375.599545017646,375.868201472985,376.136857923675,376.40551436737,
376.674170801667,376.942827224536,377.211483633864,377.480140028085,377.748796405543,
378.01745276528,378.286109106266,378.554765428293,378.823421731131,379.092078015461,
379.360734282028,379.629390532536,379.898046768888,380.166702993939,380.435359210937,
380.704015424011,380.972671637828,381.241327856887,381.509984085112,381.778640325533,
382.047296580819,382.315952852685,382.584609142666,382.853265451347,383.121921779263,
383.390578126049,383.659234491374,383.927890874099,384.196547273165,384.465203686833,
384.733860113456,385.002516550867,385.271172996977,385.539829449352,385.808485905613,
386.077142363224,386.345798819663,386.614455272453,386.883111719088,387.151768157302,
387.420424584764,387.689080999572,387.957737399735,388.226393783858,388.49505015046,
388.7637064988,389.032362828074,389.301019138333,389.56967542963,389.838331702943,
390.106987959358,390.375644200917,390.644300429918,390.912956649593,391.181612863644,
391.450269076596,391.718925293171,391.987581517421,392.25623775287,392.524894002124,
392.793550267489,393.062206550312,393.330862851807,393.599519172248,393.868175511888,
394.136831870107,394.405488246334,394.674144639227,394.94280104753,395.211457469356,
395.480113902905,395.748770345913,396.017426796181,396.286083251232,396.554739708622,
396.823396165819,397.092052620289,397.360709069602,397.629365511291,397.898021943183,
398.166678363037,398.43533476909,398.703991159489,398.972647533028,399.241303888413,
399.509960225133,399.778616542629,400.047272841224,400.315929121267,400.584585384052,
400.853241631017,401.121897864557,401.390554087381,401.659210303115,401.927866515925,
402.196522730559,402.465178951451,402.733835182185,403.002491425899,403.271147684792,
403.539803960819,403.808460254978,404.077116568174,404.345772900386,404.614429251599,
404.883085620952,405.151742007649,405.420398410161,405.689054827051,405.957711256297,
406.226367695961,406.495024143695,406.76368059721,407.032337053993,407.300993511558,
407.569649967387,407.838306418949,408.106962863879,408.375619299759,408.644275724528,
408.912932136048,409.181588532709,409.450244912815,409.718901275356,409.987557619248,
410.25621394422,410.524870249975,410.79352653712,411.06218280632,411.330839059193,
411.599495297549,411.868151524149,412.13680774213,412.40546395552,412.674120168911,
412.942776386892,413.211432613491,413.480088851848,413.748745104721,414.017401373921,
414.286057661065,414.55471396682,414.823370291793,415.092026635685,415.360682998226,
415.629339378332,415.897995774993,416.166652186512,416.435308611282,416.703965047162,
416.972621492092,417.241277943654,417.509934399483,417.778590857048,418.047247313831,
418.315903767346,418.58456021508,418.853216654744,419.121873083989,419.390529500879,
419.659185903392,419.927842290088,420.196498659441,420.465155010654,420.733811342866,
421.002467656062,421.271123950222,421.539780226249,421.808436485141,422.077092728855,
422.34574895959,422.614405180482,422.883061395116,423.151717607926,423.42037382366,
423.689030046484,423.957686280024,424.226342526988,424.494998789773,424.763655069817,
425.032311368411,425.300967685907,425.569624022627,425.838280378013,426.106936751551,
426.375593141951,426.644249548003,426.912905967857,427.18156239975,427.450218841438,
427.718875290752,427.987531745221,428.256188202418,428.524844659809,428.793501114859,
429.062157565128,429.330814008135,429.599470441684,429.868126863511,430.136783271814,
430.405439664707,430.674096040933,430.942752399152,431.211408738792,431.480065059233,
431.748721360729,432.017377643552,432.286033908916,432.554690158171,432.823346393619,
433.092002617869,433.360658834445,433.629315047397,433.897971261447,434.166627481123,
434.435283710124,434.703939951682,434.972596208097,435.241252481411,435.509908772707,
435.778565082967,436.047221412241,436.31587776058,436.584534127182,436.853190511305,
437.121846911468,437.390503326275,437.659159753738,437.927816191952,438.196472638587,
438.465129091377,438.733785547816,439.002442005427,439.271098461688,439.539754914064,
439.808411360173,440.077067797584,440.345724224207,440.614380637875,440.883037036941,
441.151693419666,441.420349784991,441.689006131777,441.957662459693,442.226318768374,
442.494975058355,442.763631330221,443.032287585506,443.300943825928,443.569600054153,
443.838256273211,444.106912487028,444.375568700103,444.644224917101,444.912881142151,
445.181537378504,445.450193629011,445.718849895579,445.987506179909,446.256162482747,
446.524818804774,446.79347514576,447.062131505496,447.330787882954,447.599444277176,
447.868100686504,448.136757109373,448.40541354367,448.674069987365,448.942726438055,
449.211382893394,449.480039350853,449.748695807921,450.017352262103,450.286008710879,
450.55466515194,450.82332158292,451.091978001848,451.360634406672,451.62929079591,
451.89794716799,452.166603522061,452.435259857205,452.703916173343,452.972572470381,
453.24122874915,453.509885010562,453.778541256488,454.047197489028,454.315853711222,
454.584509926543,454.853166139327,455.121822354318,455.3904785758,455.659134807498,
455.927791052226,456.19644731247,456.465103589759,456.733759885467,457.00241620002,
457.271072533811,457.539728886346,457.80838525717,458.077041645044,458.345698048806,
458.614354466642,458.883010896827,459.151667337143,459.420323785445,459.688980239275,
459.957636696219,460.226293153743,460.494949609316,460.763606060482,461.032262504754,
461.300918939909,461.569575363662,461.838231774175,462.106888169527,462.375544548414,
462.644200909447,462.912857251999,463.181513575386,463.450169879794,463.71882616542,
463.987482433401,464.256138684994,464.524794922418,464.793451148174,465.062107365689,
465.330763578896,465.59941979247,465.86807601102,466.13673223836,466.405388477821,
466.674044731802,466.942701002433,467.211357290885,467.480013598214,467.748669924546,
468.017326269997,468.285982633826,468.554639015346,468.823295413121,469.091951825803,
469.360608251434,469.629264688145,469.897921133626,470.166577585633,470.435234041669,
470.703890499266,470.972546955898,471.24120340903,471.509859856263,471.778516295153,
472.047172723582,472.315829139356,472.584485540789,472.853141926103,473.12179829419,
473.390454643857,473.659110974714,473.927767286328,474.196423579164,474.465079853726,
474.73373611147,475.002392354016,475.271048583941,475.539704804167,475.808361018519,
476.077017231391,476.345673447501,476.614329671083,476.882985905496,477.151642153686,
477.420298417658,477.688954699194,477.957610999126,478.226267318208,478.494923656277,
478.76358001319,479.032236387973,479.300892779719,479.569549186815,479.838205607737,
480.106862040401,480.375518482806,480.644174932567,480.912831387357,481.18148784465,
481.450144301944,481.718800756733,481.987457206495,482.2561136489,482.524770081563,
482.793426502485,483.062082909582,483.330739301328,483.59939567611,483.868052033023,
484.136708371092,484.405364690174,484.674020990106,484.942677271643,485.211333535614,
485.479989783805,485.748646018218,486.017302241799,486.28595845791,486.554614670781,
486.823270885133,487.091927105359,487.360583335284,487.629239577831,487.897895835574,
488.166552110137,488.435208402973,488.703864714587,488.972521045443,489.241177395111,
489.509833763197,489.778490148512,490.047146549945,490.315802965719,490.584459394147,
490.853115833037,491.12177228027,491.390428733402,491.659085190034,491.927741647632,
492.196398103667,492.465054555674,492.733711001155,493.002367437866,493.271023863497,
493.539680276179,493.808336673954,494.076993055474,494.345649419303,494.614305764754,
494.882962091086,495.151618398416,495.420274686867,495.688930957498,495.95758721148,
496.22624345094,496.494899678281,496.76355589683,497.032212110404,497.300868323611,
497.569524541126,497.838180766882,498.106837004306,498.3754932559,498.64414952388,
498.912805809507,499.181462113914,499.450118437301,499.718774779852,499.987431140886,
500.256087519773,500.524743915125,500.793400325638,501.06205674939,501.330713184546,
501.599369628818,501.868026079984,502.136682535557,502.40533899308,502.673995450025,
502.942651903855,503.211308352156,503.479964792472,503.748621222657,504.017277640494,
504.285934044256,504.554590432129,504.823246802954,505.091903155488,505.360559489279,
505.629215803832,505.89787209954,506.166528376829,506.435184637073,506.703840881801,
506.972497113499,507.241153334981,507.509809549972,507.778465762756,508.047121978078,
508.315778200272,508.584434432811,508.853090678737,509.121746940149,509.390403218918,
509.659059515956,509.927715832093,510.196372167238,510.465028521309,510.733684893389,
511.002341282627,511.270997687451,511.53965410638,511.808310537359,512.076966978421,
512.345623427198,512.614279881382,512.882936338452,513.151592795914,513.420249251254,
513.688905701946,513.957562145643,514.226218579942,514.494875002812,514.763531412143,
515.032187806366,515.300844183826,515.569500543564,515.838156884552,516.106813206581,
516.375469509421,516.644125793752,516.912782060321,517.181438310831,517.450094547186,
517.718750772238,517.987406989238,518.256063202315,518.524719416134,518.793375635194,
519.062031863421,519.330688103845,519.599344359133,519.868000631,520.136656920983,
520.405313229665,520.673969557583,520.942625904371,521.211282269698,521.479938652425,
521.748595051492,522.017251465163,522.285907891788,522.554564329201,522.823220775312,
523.091877227689,523.360533683951,523.629190141564,523.897846598005,524.166503050797,
524.435159497434,524.70381593565,524.972472363114,525.241128777924,525.509785178088,
525.778441562214,526.047097928818,526.315754277159,526.584410606435,526.853066916696,
527.121723207994,527.390379481309,527.659035737726,527.927691979287,528.19634820829,
528.465004427967,528.73366064202,529.002316854973,529.270973071551,529.539629295803,
529.808285531254,530.07694178051,530.345598045876,530.614254328701,530.882910630198,
531.151566950641,531.420223290284,531.688879648504,531.957536024733,532.226192417628,
532.494848825933,532.76350524776,533.032161681312,533.30081812432,533.569474574591,
533.838131029643,534.106787487035,534.375443944235,534.644100398706,534.912756848021,
535.181413289711,535.450069721605,535.718726141461,535.987382547516,536.256038937917,
536.524695311458,536.793351666845,537.062008003567,537.330664321065,537.599320619661,
537.867976899706,538.136633162493,538.40528940946,538.673945643001,538.942601865828,
539.211258081563,539.479914294375,539.748570509011,540.017226729904,540.285882960641,
540.554539204357,540.823195463252,541.09185173928,541.360508033441,541.629164346639,
541.897820678853,542.166477030068,542.435133399423,542.703789786121,542.972446188636,
543.241102605527,543.509759034775,543.778415474441,544.047071922176,544.315728375693,
544.584384832479,544.853041290046,545.121697745877,545.390354197441,545.659010642372,
545.927667078254,546.196323503025,546.464979914547,546.733636311202,547.002292691334,
547.270949053789,547.539605397955,547.808261722147,548.076918029812,548.345574313508,
548.614230583738,548.882886864851,549.151542935882,549.420199787641,549.68885445376,
549.957511414581),.UNSPECIFIED.)
GEOMETRIC_REPRESENTATION_ITEM()
RATIONAL_B_SPLINE_SURFACE(((1.,1.,1.,1.,1.,1.,1.,1.,1.,1.,1.,1.,1.,1.,1.,
1.,1.,1.,1.,1.,1.,1.,1.,1.,1.,1.,1.,1.,1.,1.,1.,1.,1.,1.,1.,1.,1.,1.,1.,
1.,1.,1.,1.,1.,1.,1.,1.,1.,1.,1.,1.,1.,1.,1.,1.,1.,1.,1.,1.,1.,1.,1.,1.,
1.,1.,1.,1.,1.,1.,1.,1.,1.,1.,1.,1.,1.,1.,1.,1.,1.,1.,1.,1.,1.,1.,1.,1.,
1.,1.,1.,1.,1.,1.,1.,1.,1.,1.,1.,1.,1.,1.,1.,1.,1.,1.,1.,1.,1.,1.,1.,1.,
1.,1.,1.,1.,1.,1.,1.,1.,1.,1.,1.,1.,1.,1.,1.,1.,1.,1.,1.,1.,1.,1.,1.,1.,
1.,1.,1.,1.,1.,1.,1.,1.,1.,1.,1.,1.,1.,1.,1.,1.,1.,1.,1.,1.,1.,1.,1.,1.,
1.,1.,1.,1.,1.,1.,1.,1.,1.,1.,1.,1.,1.,1.,1.,1.,1.,1.,1.,1.,1.,1.,1.,1.,
1.,1.,1.,1.,1.,1.,1.,1.,1.,1.,1.,1.,1.,1.,1.,1.,1.,1.,1.,1.,1.,1.,1.,1.,
1.,1.,1.,1.,1.,1.,1.,1.,1.,1.,1.,1.,1.,1.,1.,1.,1.,1.,1.,1.,1.,1.,1.,1.,
1.,1.,1.,1.,1.,1.,1.,1.,1.,1.,1.,1.,1.,1.,1.,1.,1.,1.,1.,1.,1.,1.,1.,1.,
1.,1.,1.,1.,1.,1.,1.,1.,1.,1.,1.,1.,1.,1.,1.,1.,1.,1.,1.,1.,1.,1.,1.,1.,
1.,1.,1.,1.,1.,1.,1.,1.,1.,1.,1.,1.,1.,1.,1.,1.,1.,1.,1.,1.,1.,1.,1.,1.,
1.,1.,1.,1.,1.,1.,1.,1.,1.,1.,1.,1.,1.,1.,1.,1.,1.,1.,1.,1.,1.,1.,1.,1.,
1.,1.,1.,1.,1.,1.,1.,1.,1.,1.,1.,1.,1.,1.,1.,1.,1.,1.,1.,1.,1.,1.,1.,1.,
1.,1.,1.,1.,1.,1.,1.,1.,1.,1.,1.,1.,1.,1.,1.,1.,1.,1.,1.,1.,1.,1.,1.,1.,
1.,1.,1.,1.,1.,1.,1.,1.,1.,1.,1.,1.,1.,1.,1.,1.,1.,1.,1.,1.,1.,1.,1.,1.,
1.,1.,1.,1.,1.,1.,1.,1.,1.,1.,1.,1.,1.,1.,1.,1.,1.,1.,1.,1.,1.,1.,1.,1.,
1.,1.,1.,1.,1.,1.,1.,1.,1.,1.,1.,1.,1.,1.,1.,1.,1.,1.,1.,1.,1.,1.,1.,1.,
1.,1.,1.,1.,1.,1.,1.,1.,1.,1.,1.,1.,1.,1.,1.,1.,1.,1.,1.,1.,1.,1.,1.,1.,
1.,1.,1.,1.,1.,1.,1.,1.,1.,1.,1.,1.,1.,1.,1.,1.,1.,1.,1.,1.,1.,1.,1.,1.,
1.,1.,1.,1.,1.,1.,1.,1.,1.,1.,1.,1.,1.,1.,1.,1.,1.,1.,1.,1.,1.,1.,1.,1.,
1.,1.,1.,1.,1.,1.,1.,1.,1.,1.,1.,1.,1.,1.,1.,1.,1.,1.,1.,1.,1.,1.,1.,1.,
1.,1.,1.,1.,1.,1.,1.,1.,1.,1.,1.,1.,1.,1.,1.,1.,1.,1.,1.,1.,1.,1.,1.,1.,
1.,1.,1.,1.,1.,1.,1.,1.,1.,1.,1.,1.,1.,1.,1.,1.,1.,1.,1.,1.,1.,1.,1.,1.,
1.,1.,1.,1.,1.,1.,1.,1.,1.,1.,1.,1.,1.,1.,1.,1.,1.,1.,1.,1.,1.,1.,1.,1.,
1.,1.,1.,1.,1.,1.,1.,1.,1.,1.,1.,1.,1.,1.,1.,1.,1.,1.,1.,1.,1.,1.,1.,1.,
1.,1.,1.,1.,1.,1.,1.,1.,1.,1.,1.,1.,1.,1.,1.,1.,1.,1.,1.,1.,1.,1.,1.,1.,
1.,1.,1.,1.,1.,1.,1.,1.,1.,1.,1.,1.,1.,1.,1.,1.,1.,1.,1.,1.,1.,1.,1.,1.,
1.,1.,1.,1.,1.,1.,1.,1.,1.,1.,1.,1.,1.,1.,1.,1.,1.,1.,1.,1.,1.,1.,1.,1.,
1.,1.,1.,1.,1.,1.,1.,1.,1.,1.,1.,1.,1.,1.,1.,1.,1.,1.,1.,1.,1.,1.,1.,1.,
1.,1.,1.,1.,1.,1.,1.,1.,1.,1.,1.,1.,1.,1.,1.,1.,1.,1.,1.,1.,1.,1.,1.,1.,
1.,1.,1.,1.,1.,1.,1.,1.,1.,1.,1.,1.,1.,1.,1.,1.,1.,1.,1.,1.,1.,1.,1.,1.,
1.,1.,1.,1.,1.,1.,1.,1.,1.,1.,1.,1.,1.,1.,1.,1.,1.,1.,1.,1.,1.,1.,1.,1.,
1.,1.,1.,1.,1.,1.,1.,1.,1.,1.,1.,1.,1.,1.,1.,1.,1.,1.,1.,1.,1.,1.,1.,1.,
1.,1.,1.,1.,1.,1.,1.,1.,1.,1.,1.,1.,1.,1.,1.,1.,1.,1.,1.,1.,1.,1.,1.,1.,
1.,1.,1.,1.,1.,1.,1.,1.,1.,1.,1.,1.,1.,1.,1.,1.,1.,1.,1.,1.,1.,1.,1.,1.,
1.,1.,1.,1.,1.,1.,1.,1.,1.,1.,1.,1.,1.,1.,1.,1.,1.,1.,1.,1.,1.,1.,1.,1.,
1.,1.,1.,1.,1.,1.,1.,1.,1.,1.,1.,1.,1.,1.,1.,1.,1.,1.,1.,1.,1.,1.,1.,1.,
1.,1.,1.,1.,1.,1.,1.,1.,1.,1.,1.,1.,1.,1.,1.,1.,1.,1.,1.,1.,1.,1.,1.,1.,
1.,1.,1.,1.,1.,1.,1.,1.,1.,1.,1.,1.,1.,1.,1.,1.,1.,1.,1.,1.,1.,1.,1.,1.,
1.,1.,1.,1.,1.,1.,1.,1.,1.,1.,1.,1.,1.,1.,1.,1.,1.,1.,1.,1.,1.,1.,1.,1.,
1.,1.,1.,1.,1.,1.,1.,1.,1.,1.,1.,1.,1.,1.,1.,1.,1.,1.,1.,1.,1.,1.,1.,1.,
1.,1.,1.,1.,1.,1.,1.,1.,1.,1.,1.,1.,1.,1.,1.,1.,1.,1.,1.,1.,1.,1.,1.,1.,
1.,1.,1.,1.,1.,1.,1.,1.,1.,1.,1.,1.,1.,1.,1.,1.,1.,1.,1.,1.,1.,1.,1.,1.,
1.,1.,1.,1.,1.,1.,1.,1.,1.,1.,1.,1.,1.,1.,1.,1.,1.,1.,1.,1.,1.,1.,1.,1.,
1.,1.,1.,1.,1.,1.,1.,1.,1.,1.,1.,1.,1.,1.,1.,1.,1.,1.,1.,1.,1.,1.,1.,1.,
1.,1.,1.,1.,1.,1.,1.,1.,1.,1.,1.,1.,1.,1.,1.,1.,1.,1.,1.,1.,1.,1.,1.,1.,
1.,1.,1.,1.,1.,1.,1.,1.,1.,1.,1.,1.,1.,1.,1.,1.,1.,1.,1.,1.,1.,1.,1.,1.,
1.,1.,1.,1.,1.,1.,1.,1.,1.,1.,1.,1.,1.,1.,1.,1.,1.,1.,1.,1.,1.,1.,1.,1.,
1.,1.,1.,1.,1.,1.,1.,1.,1.,1.,1.,1.,1.,1.,1.,1.,1.,1.,1.,1.,1.,1.,1.,1.,
1.,1.,1.,1.,1.,1.,1.,1.,1.,1.,1.,1.,1.,1.,1.,1.,1.,1.,1.,1.,1.,1.,1.,1.,
1.,1.,1.,1.,1.,1.,1.,1.,1.,1.,1.,1.,1.,1.,1.,1.,1.,1.,1.,1.,1.,1.,1.,1.,
1.,1.,1.,1.,1.,1.,1.,1.,1.,1.,1.,1.,1.,1.,1.,1.,1.,1.,1.,1.,1.,1.,1.,1.,
1.,1.,1.,1.,1.,1.,1.,1.,1.,1.,1.,1.,1.,1.,1.,1.,1.,1.,1.,1.,1.,1.,1.,1.,
1.,1.,1.,1.,1.,1.,1.,1.,1.,1.,1.,1.,1.,1.,1.,1.,1.,1.,1.,1.,1.,1.,1.,1.,
1.,1.,1.,1.,1.,1.,1.,1.,1.,1.,1.,1.,1.,1.,1.,1.,1.,1.,1.,1.,1.,1.,1.,1.,
1.,1.,1.,1.,1.,1.,1.,1.,1.,1.,1.,1.,1.,1.,1.,1.,1.,1.,1.,1.,1.,1.,1.,1.,
1.,1.,1.,1.,1.,1.,1.,1.,1.,1.,1.,1.,1.,1.,1.,1.,1.,1.,1.,1.,1.,1.,1.,1.,
1.,1.,1.,1.,1.,1.,1.,1.,1.,1.,1.,1.,1.,1.,1.,1.,1.,1.,1.,1.,1.,1.,1.,1.,
1.,1.,1.,1.,1.,1.,1.,1.,1.,1.,1.,1.,1.,1.,1.,1.,1.,1.,1.,1.,1.,1.,1.,1.,
1.,1.,1.,1.,1.,1.,1.,1.,1.,1.,1.,1.,1.,1.,1.,1.,1.,1.,1.,1.,1.,1.,1.,1.,
1.,1.,1.,1.,1.,1.,1.,1.,1.,1.,1.,1.,1.,1.,1.,1.,1.,1.,1.,1.,1.,1.,1.,1.,
1.,1.,1.,1.,1.,1.,1.,1.,1.,1.,1.,1.,1.,1.,1.,1.,1.,1.,1.,1.,1.,1.,1.,1.,
1.,1.,1.,1.,1.,1.,1.,1.,1.,1.,1.,1.,1.,1.,1.,1.,1.,1.,1.,1.,1.,1.,1.,1.,
1.,1.,1.,1.,1.,1.,1.,1.,1.,1.,1.,1.,1.,1.,1.,1.,1.,1.,1.,1.,1.,1.,1.,1.,
1.,1.,1.,1.,1.,1.,1.,1.,1.,1.,1.,1.,1.,1.,1.,1.,1.,1.,1.,1.,1.,1.,1.,1.,
1.,1.,1.,1.,1.,1.,1.,1.,1.,1.,1.,1.,1.,1.,1.,1.,1.,1.,1.,1.,1.,1.,1.,1.,
1.,1.,1.,1.,1.,1.,1.,1.,1.,1.,1.,1.,1.,1.,1.,1.,1.,1.,1.,1.,1.,1.,1.,1.,
1.,1.,1.,1.,1.,1.,1.,1.,1.,1.,1.,1.,1.,1.,1.,1.,1.,1.,1.,1.,1.,1.,1.,1.,
1.,1.,1.,1.,1.,1.,1.,1.,1.,1.,1.,1.,1.,1.,1.,1.,1.,1.,1.,1.,1.,1.,1.,1.,
1.,1.,1.,1.,1.,1.,1.,1.,1.,1.,1.,1.,1.,1.,1.,1.,1.,1.,1.,1.,1.,1.,1.,1.,
1.,1.,1.,1.,1.,1.,1.,1.,1.,1.,1.,1.,1.,1.,1.,1.,1.,1.,1.,1.,1.,1.,1.,1.,
1.,1.,1.,1.,1.,1.,1.,1.,1.,1.,1.,1.,1.,1.,1.,1.,1.,1.,1.,1.,1.,1.,1.,1.,
1.,1.,1.,1.,1.,1.,1.,1.,1.,1.,1.,1.,1.,1.,1.,1.,1.,1.,1.,1.,1.,1.,1.,1.,
1.,1.,1.,1.,1.,1.,1.,1.,1.,1.,1.,1.,1.,1.,1.,1.,1.,1.,1.,1.,1.,1.,1.,1.,
1.,1.,1.,1.,1.,1.,1.,1.,1.,1.,1.,1.,1.,1.,1.,1.,1.,1.,1.,1.,1.,1.,1.,1.,
1.,1.,1.,1.,1.,1.,1.,1.,1.,1.,1.,1.,1.,1.,1.,1.,1.,1.,1.,1.,1.,1.,1.,1.,
1.,1.,1.,1.,1.,1.,1.,1.,1.,1.,1.,1.,1.,1.,1.,1.,1.,1.,1.,1.,1.,1.,1.,1.,
1.,1.,1.,1.,1.,1.,1.,1.,1.,1.,1.,1.,1.,1.,1.,1.,1.,1.,1.,1.,1.,1.,1.,1.,
1.,1.,1.,1.,1.,1.,1.,1.,1.,1.,1.,1.,1.,1.,1.,1.,1.,1.,1.,1.,1.,1.,1.,1.,
1.,1.,1.,1.,1.,1.,1.,1.,1.,1.,1.,1.,1.,1.,1.,1.,1.,1.,1.,1.,1.,1.,1.,1.,
1.,1.,1.,1.,1.,1.,1.,1.,1.,1.,1.,1.,1.,1.,1.,1.,1.,1.,1.,1.,1.,1.,1.,1.,
1.,1.,1.,1.,1.,1.,1.,1.,1.,1.,1.,1.,1.,1.,1.,1.,1.,1.,1.,1.,1.,1.,1.,1.,
1.,1.,1.,1.,1.,1.,1.,1.,1.,1.,1.,1.,1.,1.,1.,1.,1.,1.,1.,1.,1.,1.,1.,1.,
1.,1.,1.,1.,1.,1.,1.,1.,1.,1.,1.,1.,1.,1.,1.,1.,1.,1.,1.,1.),(0.707106781186548,
0.707106781186548,0.707106781186548,0.707106781186547,0.707106781186547,
0.707106781186548,0.707106781186547,0.707106781186547,0.707106781186547,
0.707106781186547,0.707106781186547,0.707106781186548,0.707106781186548,
0.707106781186548,0.707106781186547,0.707106781186548,0.707106781186547,
0.707106781186547,0.707106781186548,0.707106781186547,0.707106781186548,
0.707106781186547,0.707106781186548,0.707106781186547,0.707106781186548,
0.707106781186547,0.707106781186547,0.707106781186547,0.707106781186547,
0.707106781186547,0.707106781186548,0.707106781186547,0.707106781186547,
0.707106781186548,0.707106781186547,0.707106781186547,0.707106781186548,
0.707106781186547,0.707106781186547,0.707106781186548,0.707106781186548,
0.707106781186547,0.707106781186548,0.707106781186547,0.707106781186547,
0.707106781186547,0.707106781186548,0.707106781186548,0.707106781186547,
0.707106781186547,0.707106781186548,0.707106781186547,0.707106781186548,
0.707106781186547,0.707106781186547,0.707106781186547,0.707106781186547,
0.707106781186547,0.707106781186548,0.707106781186547,0.707106781186548,
0.707106781186547,0.707106781186548,0.707106781186547,0.707106781186548,
0.707106781186547,0.707106781186547,0.707106781186548,0.707106781186547,
0.707106781186547,0.707106781186548,0.707106781186547,0.707106781186548,
0.707106781186547,0.707106781186548,0.707106781186548,0.707106781186547,
0.707106781186548,0.707106781186547,0.707106781186547,0.707106781186548,
0.707106781186547,0.707106781186547,0.707106781186547,0.707106781186548,
0.707106781186547,0.707106781186547,0.707106781186547,0.707106781186547,
0.707106781186547,0.707106781186547,0.707106781186548,0.707106781186548,
0.707106781186547,0.707106781186548,0.707106781186547,0.707106781186548,
0.707106781186548,0.707106781186547,0.707106781186548,0.707106781186548,
0.707106781186548,0.707106781186547,0.707106781186548,0.707106781186547,
0.707106781186548,0.707106781186548,0.707106781186548,0.707106781186547,
0.707106781186547,0.707106781186547,0.707106781186548,0.707106781186548,
0.707106781186548,0.707106781186547,0.707106781186547,0.707106781186547,
0.707106781186548,0.707106781186548,0.707106781186547,0.707106781186547,
0.707106781186548,0.707106781186547,0.707106781186547,0.707106781186547,
0.707106781186547,0.707106781186548,0.707106781186547,0.707106781186548,
0.707106781186547,0.707106781186547,0.707106781186547,0.707106781186548,
0.707106781186548,0.707106781186547,0.707106781186548,0.707106781186548,
0.707106781186547,0.707106781186548,0.707106781186547,0.707106781186548,
0.707106781186547,0.707106781186548,0.707106781186547,0.707106781186547,
0.707106781186548,0.707106781186547,0.707106781186547,0.707106781186548,
0.707106781186547,0.707106781186547,0.707106781186548,0.707106781186547,
0.707106781186548,0.707106781186547,0.707106781186547,0.707106781186548,
0.707106781186548,0.707106781186547,0.707106781186548,0.707106781186547,
0.707106781186548,0.707106781186547,0.707106781186548,0.707106781186547,
0.707106781186548,0.707106781186547,0.707106781186548,0.707106781186547,
0.707106781186548,0.707106781186547,0.707106781186548,0.707106781186547,
0.707106781186547,0.707106781186548,0.707106781186547,0.707106781186548,
0.707106781186547,0.707106781186548,0.707106781186547,0.707106781186548,
0.707106781186547,0.707106781186547,0.707106781186548,0.707106781186547,
0.707106781186548,0.707106781186548,0.707106781186548,0.707106781186547,
0.707106781186547,0.707106781186547,0.707106781186547,0.707106781186548,
0.707106781186547,0.707106781186548,0.707106781186548,0.707106781186547,
0.707106781186547,0.707106781186548,0.707106781186548,0.707106781186547,
0.707106781186547,0.707106781186548,0.707106781186547,0.707106781186548,
0.707106781186547,0.707106781186547,0.707106781186547,0.707106781186547,
0.707106781186547,0.707106781186547,0.707106781186547,0.707106781186548,
0.707106781186547,0.707106781186548,0.707106781186547,0.707106781186548,
0.707106781186548,0.707106781186547,0.707106781186548,0.707106781186548,
0.707106781186548,0.707106781186548,0.707106781186547,0.707106781186548,
0.707106781186547,0.707106781186548,0.707106781186547,0.707106781186547,
0.707106781186548,0.707106781186548,0.707106781186547,0.707106781186547,
0.707106781186547,0.707106781186547,0.707106781186547,0.707106781186548,
0.707106781186548,0.707106781186547,0.707106781186547,0.707106781186548,
0.707106781186548,0.707106781186547,0.707106781186548,0.707106781186547,
0.707106781186548,0.707106781186548,0.707106781186547,0.707106781186547,
0.707106781186548,0.707106781186547,0.707106781186547,0.707106781186548,
0.707106781186547,0.707106781186548,0.707106781186547,0.707106781186548,
0.707106781186547,0.707106781186547,0.707106781186548,0.707106781186548,
0.707106781186547,0.707106781186547,0.707106781186548,0.707106781186547,
0.707106781186547,0.707106781186548,0.707106781186547,0.707106781186548,
0.707106781186547,0.707106781186548,0.707106781186547,0.707106781186548,
0.707106781186547,0.707106781186547,0.707106781186547,0.707106781186547,
0.707106781186547,0.707106781186547,0.707106781186548,0.707106781186547,
0.707106781186548,0.707106781186547,0.707106781186548,0.707106781186548,
0.707106781186547,0.707106781186548,0.707106781186548,0.707106781186547,
0.707106781186548,0.707106781186547,0.707106781186547,0.707106781186547,
0.707106781186548,0.707106781186547,0.707106781186547,0.707106781186548,
0.707106781186547,0.707106781186548,0.707106781186547,0.707106781186547,
0.707106781186547,0.707106781186548,0.707106781186548,0.707106781186547,
0.707106781186548,0.707106781186548,0.707106781186547,0.707106781186548,
0.707106781186547,0.707106781186548,0.707106781186548,0.707106781186547,
0.707106781186548,0.707106781186548,0.707106781186548,0.707106781186547,
0.707106781186547,0.707106781186548,0.707106781186547,0.707106781186548,
0.707106781186547,0.707106781186547,0.707106781186548,0.707106781186548,
0.707106781186548,0.707106781186547,0.707106781186547,0.707106781186548,
0.707106781186548,0.707106781186547,0.707106781186547,0.707106781186548,
0.707106781186547,0.707106781186547,0.707106781186548,0.707106781186548,
0.707106781186547,0.707106781186547,0.707106781186547,0.707106781186548,
0.707106781186547,0.707106781186547,0.707106781186547,0.707106781186548,
0.707106781186548,0.707106781186547,0.707106781186548,0.707106781186547,
0.707106781186548,0.707106781186547,0.707106781186548,0.707106781186548,
0.707106781186547,0.707106781186547,0.707106781186548,0.707106781186547,
0.707106781186547,0.707106781186548,0.707106781186547,0.707106781186548,
0.707106781186548,0.707106781186547,0.707106781186548,0.707106781186547,
0.707106781186547,0.707106781186547,0.707106781186548,0.707106781186548,
0.707106781186548,0.707106781186547,0.707106781186548,0.707106781186547,
0.707106781186548,0.707106781186547,0.707106781186547,0.707106781186547,
0.707106781186547,0.707106781186548,0.707106781186548,0.707106781186547,
0.707106781186547,0.707106781186548,0.707106781186547,0.707106781186548,
0.707106781186547,0.707106781186548,0.707106781186547,0.707106781186547,
0.707106781186548,0.707106781186547,0.707106781186548,0.707106781186547,
0.707106781186548,0.707106781186548,0.707106781186547,0.707106781186548,
0.707106781186547,0.707106781186548,0.707106781186548,0.707106781186547,
0.707106781186548,0.707106781186547,0.707106781186547,0.707106781186548,
0.707106781186547,0.707106781186548,0.707106781186547,0.707106781186548,
0.707106781186547,0.707106781186547,0.707106781186548,0.707106781186548,
0.707106781186548,0.707106781186548,0.707106781186547,0.707106781186548,
0.707106781186548,0.707106781186548,0.707106781186547,0.707106781186548,
0.707106781186548,0.707106781186548,0.707106781186547,0.707106781186547,
0.707106781186548,0.707106781186547,0.707106781186548,0.707106781186547,
0.707106781186548,0.707106781186548,0.707106781186547,0.707106781186547,
0.707106781186548,0.707106781186547,0.707106781186548,0.707106781186547,
0.707106781186548,0.707106781186548,0.707106781186547,0.707106781186547,
0.707106781186547,0.707106781186548,0.707106781186548,0.707106781186547,
0.707106781186547,0.707106781186548,0.707106781186548,0.707106781186548,
0.707106781186548,0.707106781186547,0.707106781186547,0.707106781186548,
0.707106781186548,0.707106781186547,0.707106781186548,0.707106781186547,
0.707106781186548,0.707106781186547,0.707106781186548,0.707106781186547,
0.707106781186547,0.707106781186548,0.707106781186547,0.707106781186547,
0.707106781186548,0.707106781186547,0.707106781186548,0.707106781186547,
0.707106781186548,0.707106781186547,0.707106781186548,0.707106781186547,
0.707106781186548,0.707106781186547,0.707106781186548,0.707106781186547,
0.707106781186547,0.707106781186548,0.707106781186548,0.707106781186547,
0.707106781186547,0.707106781186547,0.707106781186548,0.707106781186547,
0.707106781186548,0.707106781186547,0.707106781186548,0.707106781186547,
0.707106781186548,0.707106781186547,0.707106781186547,0.707106781186547,
0.707106781186548,0.707106781186547,0.707106781186548,0.707106781186548,
0.707106781186547,0.707106781186548,0.707106781186547,0.707106781186547,
0.707106781186548,0.707106781186547,0.707106781186547,0.707106781186548,
0.707106781186547,0.707106781186547,0.707106781186547,0.707106781186547,
0.707106781186548,0.707106781186547,0.707106781186547,0.707106781186547,
0.707106781186548,0.707106781186547,0.707106781186547,0.707106781186548,
0.707106781186548,0.707106781186547,0.707106781186548,0.707106781186548,
0.707106781186547,0.707106781186547,0.707106781186548,0.707106781186547,
0.707106781186547,0.707106781186548,0.707106781186547,0.707106781186547,
0.707106781186547,0.707106781186548,0.707106781186547,0.707106781186548,
0.707106781186547,0.707106781186548,0.707106781186547,0.707106781186548,
0.707106781186547,0.707106781186548,0.707106781186547,0.707106781186548,
0.707106781186548,0.707106781186547,0.707106781186547,0.707106781186548,
0.707106781186547,0.707106781186548,0.707106781186547,0.707106781186548,
0.707106781186548,0.707106781186547,0.707106781186548,0.707106781186547,
0.707106781186548,0.707106781186548,0.707106781186547,0.707106781186547,
0.707106781186548,0.707106781186547,0.707106781186548,0.707106781186547,
0.707106781186548,0.707106781186547,0.707106781186548,0.707106781186547,
0.707106781186547,0.707106781186547,0.707106781186547,0.707106781186547,
0.707106781186547,0.707106781186547,0.707106781186547,0.707106781186548,
0.707106781186547,0.707106781186548,0.707106781186547,0.707106781186547,
0.707106781186548,0.707106781186547,0.707106781186548,0.707106781186547,
0.707106781186547,0.707106781186548,0.707106781186547,0.707106781186548,
0.707106781186547,0.707106781186548,0.707106781186547,0.707106781186548,
0.707106781186547,0.707106781186548,0.707106781186547,0.707106781186548,
0.707106781186547,0.707106781186548,0.707106781186548,0.707106781186547,
0.707106781186548,0.707106781186547,0.707106781186547,0.707106781186547,
0.707106781186548,0.707106781186547,0.707106781186547,0.707106781186547,
0.707106781186548,0.707106781186547,0.707106781186547,0.707106781186548,
0.707106781186547,0.707106781186547,0.707106781186547,0.707106781186547,
0.707106781186548,0.707106781186547,0.707106781186547,0.707106781186547,
0.707106781186548,0.707106781186548,0.707106781186548,0.707106781186548,
0.707106781186547,0.707106781186548,0.707106781186547,0.707106781186547,
0.707106781186548,0.707106781186547,0.707106781186548,0.707106781186547,
0.707106781186547,0.707106781186548,0.707106781186547,0.707106781186547,
0.707106781186547,0.707106781186547,0.707106781186548,0.707106781186548,
0.707106781186547,0.707106781186547,0.707106781186548,0.707106781186547,
0.707106781186548,0.707106781186547,0.707106781186548,0.707106781186548,
0.707106781186547,0.707106781186547,0.707106781186548,0.707106781186548,
0.707106781186547,0.707106781186548,0.707106781186548,0.707106781186547,
0.707106781186548,0.707106781186548,0.707106781186548,0.707106781186547,
0.707106781186548,0.707106781186547,0.707106781186548,0.707106781186547,
0.707106781186548,0.707106781186547,0.707106781186548,0.707106781186547,
0.707106781186548,0.707106781186548,0.707106781186547,0.707106781186547,
0.707106781186548,0.707106781186547,0.707106781186548,0.707106781186547,
0.707106781186548,0.707106781186548,0.707106781186548,0.707106781186548,
0.707106781186548,0.707106781186547,0.707106781186547,0.707106781186547,
0.707106781186547,0.707106781186548,0.707106781186547,0.707106781186548,
0.707106781186547,0.707106781186547,0.707106781186548,0.707106781186548,
0.707106781186547,0.707106781186548,0.707106781186547,0.707106781186548,
0.707106781186548,0.707106781186547,0.707106781186547,0.707106781186548,
0.707106781186547,0.707106781186548,0.707106781186547,0.707106781186548,
0.707106781186547,0.707106781186548,0.707106781186547,0.707106781186548,
0.707106781186547,0.707106781186548,0.707106781186547,0.707106781186548,
0.707106781186548,0.707106781186547,0.707106781186548,0.707106781186547,
0.707106781186548,0.707106781186547,0.707106781186548,0.707106781186548,
0.707106781186548,0.707106781186547,0.707106781186547,0.707106781186548,
0.707106781186548,0.707106781186547,0.707106781186547,0.707106781186547,
0.707106781186548,0.707106781186547,0.707106781186548,0.707106781186547,
0.707106781186548,0.707106781186547,0.707106781186547,0.707106781186547,
0.707106781186548,0.707106781186547,0.707106781186548,0.707106781186547,
0.707106781186548,0.707106781186547,0.707106781186548,0.707106781186547,
0.707106781186547,0.707106781186548,0.707106781186547,0.707106781186547,
0.707106781186548,0.707106781186547,0.707106781186547,0.707106781186548,
0.707106781186547,0.707106781186547,0.707106781186547,0.707106781186548,
0.707106781186547,0.707106781186548,0.707106781186547,0.707106781186547,
0.707106781186547,0.707106781186548,0.707106781186548,0.707106781186547,
0.707106781186547,0.707106781186548,0.707106781186548,0.707106781186548,
0.707106781186547,0.707106781186548,0.707106781186547,0.707106781186548,
0.707106781186547,0.707106781186548,0.707106781186547,0.707106781186547,
0.707106781186547,0.707106781186547,0.707106781186548,0.707106781186547,
0.707106781186548,0.707106781186548,0.707106781186547,0.707106781186548,
0.707106781186547,0.707106781186547,0.707106781186547,0.707106781186547,
0.707106781186548,0.707106781186547,0.707106781186548,0.707106781186547,
0.707106781186548,0.707106781186548,0.707106781186547,0.707106781186548,
0.707106781186547,0.707106781186547,0.707106781186547,0.707106781186547,
0.707106781186548,0.707106781186547,0.707106781186548,0.707106781186548,
0.707106781186547,0.707106781186548,0.707106781186547,0.707106781186548,
0.707106781186547,0.707106781186547,0.707106781186548,0.707106781186547,
0.707106781186548,0.707106781186548,0.707106781186547,0.707106781186547,
0.707106781186548,0.707106781186548,0.707106781186547,0.707106781186547,
0.707106781186548,0.707106781186547,0.707106781186547,0.707106781186548,
0.707106781186547,0.707106781186547,0.707106781186548,0.707106781186547,
0.707106781186548,0.707106781186547,0.707106781186547,0.707106781186548,
0.707106781186547,0.707106781186548,0.707106781186547,0.707106781186548,
0.707106781186547,0.707106781186547,0.707106781186547,0.707106781186548,
0.707106781186547,0.707106781186548,0.707106781186547,0.707106781186548,
0.707106781186548,0.707106781186548,0.707106781186548,0.707106781186547,
0.707106781186547,0.707106781186547,0.707106781186548,0.707106781186547,
0.707106781186548,0.707106781186547,0.707106781186547,0.707106781186548,
0.707106781186547,0.707106781186547,0.707106781186548,0.707106781186547,
0.707106781186547,0.707106781186548,0.707106781186548,0.707106781186547,
0.707106781186548,0.707106781186547,0.707106781186547,0.707106781186548,
0.707106781186547,0.707106781186548,0.707106781186547,0.707106781186548,
0.707106781186547,0.707106781186547,0.707106781186547,0.707106781186548,
0.707106781186547,0.707106781186548,0.707106781186547,0.707106781186548,
0.707106781186547,0.707106781186547,0.707106781186548,0.707106781186548,
0.707106781186548,0.707106781186547,0.707106781186548,0.707106781186547,
0.707106781186548,0.707106781186547,0.707106781186548,0.707106781186547,
0.707106781186548,0.707106781186548,0.707106781186547,0.707106781186547,
0.707106781186547,0.707106781186548,0.707106781186547,0.707106781186547,
0.707106781186548,0.707106781186547,0.707106781186547,0.707106781186548,
0.707106781186547,0.707106781186548,0.707106781186548,0.707106781186548,
0.707106781186547,0.707106781186548,0.707106781186547,0.707106781186548,
0.707106781186547,0.707106781186548,0.707106781186547,0.707106781186548,
0.707106781186547,0.707106781186548,0.707106781186547,0.707106781186548,
0.707106781186548,0.707106781186547,0.707106781186548,0.707106781186547,
0.707106781186548,0.707106781186548,0.707106781186547,0.707106781186547,
0.707106781186548,0.707106781186547,0.707106781186547,0.707106781186548,
0.707106781186547,0.707106781186548,0.707106781186548,0.707106781186547,
0.707106781186548,0.707106781186548,0.707106781186548,0.707106781186548,
0.707106781186548,0.707106781186547,0.707106781186548,0.707106781186548,
0.707106781186548,0.707106781186547,0.707106781186548,0.707106781186547,
0.707106781186548,0.707106781186547,0.707106781186548,0.707106781186547,
0.707106781186548,0.707106781186547,0.707106781186548,0.707106781186547,
0.707106781186547,0.707106781186548,0.707106781186547,0.707106781186547,
0.707106781186548,0.707106781186547,0.707106781186548,0.707106781186547,
0.707106781186548,0.707106781186547,0.707106781186548,0.707106781186547,
0.707106781186547,0.707106781186548,0.707106781186547,0.707106781186547,
0.707106781186548,0.707106781186547,0.707106781186548,0.707106781186547,
0.707106781186547,0.707106781186548,0.707106781186548,0.707106781186547,
0.707106781186548,0.707106781186547,0.707106781186547,0.707106781186547,
0.707106781186548,0.707106781186547,0.707106781186547,0.707106781186548,
0.707106781186547,0.707106781186547,0.707106781186547,0.707106781186548,
0.707106781186548,0.707106781186547,0.707106781186548,0.707106781186547,
0.707106781186548,0.707106781186547,0.707106781186547,0.707106781186548,
0.707106781186547,0.707106781186548,0.707106781186547,0.707106781186547,
0.707106781186547,0.707106781186547,0.707106781186548,0.707106781186547,
0.707106781186547,0.707106781186547,0.707106781186547,0.707106781186547,
0.707106781186548,0.707106781186547,0.707106781186547,0.707106781186547,
0.707106781186547,0.707106781186548,0.707106781186547,0.707106781186548,
0.707106781186547,0.707106781186547,0.707106781186548,0.707106781186547,
0.707106781186548,0.707106781186547,0.707106781186547,0.707106781186548,
0.707106781186547,0.707106781186547,0.707106781186548,0.707106781186547,
0.707106781186547,0.707106781186547,0.707106781186547,0.707106781186548,
0.707106781186547,0.707106781186548,0.707106781186548,0.707106781186547,
0.707106781186548,0.707106781186548,0.707106781186547,0.707106781186547,
0.707106781186548,0.707106781186547,0.707106781186547,0.707106781186547,
0.707106781186548,0.707106781186547,0.707106781186547,0.707106781186548,
0.707106781186547,0.707106781186548,0.707106781186547,0.707106781186548,
0.707106781186547,0.707106781186547,0.707106781186548,0.707106781186547,
0.707106781186548,0.707106781186547,0.707106781186548,0.707106781186547,
0.707106781186548,0.707106781186547,0.707106781186548,0.707106781186547,
0.707106781186547,0.707106781186547,0.707106781186547,0.707106781186548,
0.707106781186548,0.707106781186547,0.707106781186548,0.707106781186548,
0.707106781186547,0.707106781186548,0.707106781186547,0.707106781186547,
0.707106781186548,0.707106781186547,0.707106781186547,0.707106781186547,
0.707106781186547,0.707106781186548,0.707106781186547,0.707106781186547,
0.707106781186547,0.707106781186548,0.707106781186547,0.707106781186547,
0.707106781186548,0.707106781186547,0.707106781186548,0.707106781186548,
0.707106781186547,0.707106781186548,0.707106781186547,0.707106781186548,
0.707106781186547,0.707106781186548,0.707106781186547,0.707106781186547,
0.707106781186548,0.707106781186547,0.707106781186548,0.707106781186548,
0.707106781186547,0.707106781186547,0.707106781186548,0.707106781186547,
0.707106781186548,0.707106781186547,0.707106781186548,0.707106781186547,
0.707106781186547,0.707106781186548,0.707106781186548,0.707106781186547,
0.707106781186548,0.707106781186548,0.707106781186547,0.707106781186548,
0.707106781186548,0.707106781186547,0.707106781186548,0.707106781186547,
0.707106781186548,0.707106781186547,0.707106781186548,0.707106781186547,
0.707106781186548,0.707106781186547,0.707106781186547,0.707106781186548,
0.707106781186547,0.707106781186547,0.707106781186548,0.707106781186547,
0.707106781186548,0.707106781186548,0.707106781186547,0.707106781186547,
0.707106781186547,0.707106781186548,0.707106781186547,0.707106781186548,
0.707106781186548,0.707106781186547,0.707106781186548,0.707106781186547,
0.707106781186548,0.707106781186547,0.707106781186548,0.707106781186547,
0.707106781186547,0.707106781186548,0.707106781186548,0.707106781186548,
0.707106781186547,0.707106781186548,0.707106781186548,0.707106781186547,
0.707106781186548,0.707106781186547,0.707106781186548,0.707106781186548,
0.707106781186548,0.707106781186548,0.707106781186548,0.707106781186548,
0.707106781186547,0.707106781186547,0.707106781186548,0.707106781186547,
0.707106781186547,0.707106781186548,0.707106781186547,0.707106781186547,
0.707106781186548,0.707106781186547,0.707106781186548,0.707106781186547,
0.707106781186548,0.707106781186547,0.707106781186547,0.707106781186547,
0.707106781186548,0.707106781186547,0.707106781186547,0.707106781186548,
0.707106781186547,0.707106781186548,0.707106781186547,0.707106781186548,
0.707106781186547,0.707106781186547,0.707106781186547,0.707106781186547,
0.707106781186548,0.707106781186547,0.707106781186547,0.707106781186548,
0.707106781186548,0.707106781186547,0.707106781186548,0.707106781186547,
0.707106781186548,0.707106781186547,0.707106781186547,0.707106781186548,
0.707106781186547,0.707106781186548,0.707106781186547,0.707106781186548,
0.707106781186547,0.707106781186548,0.707106781186548,0.707106781186547,
0.707106781186548,0.707106781186547,0.707106781186547,0.707106781186548,
0.707106781186547,0.707106781186547,0.707106781186548,0.707106781186548,
0.707106781186548,0.707106781186547,0.707106781186548,0.707106781186547,
0.707106781186547,0.707106781186547,0.707106781186548,0.707106781186547,
0.707106781186548,0.707106781186548,0.707106781186548,0.707106781186547,
0.707106781186547,0.707106781186547,0.707106781186547,0.707106781186548,
0.707106781186547,0.707106781186547,0.707106781186548,0.707106781186547,
0.707106781186548,0.707106781186547,0.707106781186547,0.707106781186548,
0.707106781186547,0.707106781186548,0.707106781186547,0.707106781186548,
0.707106781186547,0.707106781186547,0.707106781186547,0.707106781186547,
0.707106781186547,0.707106781186547,0.707106781186548,0.707106781186547,
0.707106781186547,0.707106781186548,0.707106781186548,0.707106781186547,
0.707106781186548,0.707106781186548,0.707106781186547,0.707106781186547,
0.707106781186548,0.707106781186547,0.707106781186547,0.707106781186548,
0.707106781186547,0.707106781186548,0.707106781186548,0.707106781186548,
0.707106781186547,0.707106781186547,0.707106781186547,0.707106781186547,
0.707106781186548,0.707106781186548,0.707106781186548,0.707106781186547,
0.707106781186548,0.707106781186547,0.707106781186548,0.707106781186548,
0.707106781186547,0.707106781186548,0.707106781186547,0.707106781186548,
0.707106781186548,0.707106781186547,0.707106781186547,0.707106781186548,
0.707106781186547,0.707106781186548,0.707106781186547,0.707106781186548,
0.707106781186548,0.707106781186548,0.707106781186547,0.707106781186548,
0.707106781186547,0.707106781186547,0.707106781186547,0.707106781186547,
0.707106781186548,0.707106781186548,0.707106781186547,0.707106781186547,
0.707106781186547,0.707106781186548,0.707106781186547,0.707106781186547,
0.707106781186548,0.707106781186547,0.707106781186548,0.707106781186548,
0.707106781186548,0.707106781186547,0.707106781186547,0.707106781186547,
0.707106781186547,0.707106781186548,0.707106781186548,0.707106781186547,
0.707106781186548,0.707106781186547,0.707106781186548,0.707106781186548,
0.707106781186547,0.707106781186548,0.707106781186547,0.707106781186548,
0.707106781186547,0.707106781186547,0.707106781186547,0.707106781186548,
0.707106781186547,0.707106781186548,0.707106781186547,0.707106781186548,
0.707106781186547,0.707106781186548,0.707106781186547,0.707106781186548,
0.707106781186547,0.707106781186547,0.707106781186548,0.707106781186547,
0.707106781186548,0.707106781186547,0.707106781186547,0.707106781186548,
0.707106781186548,0.707106781186547,0.707106781186548,0.707106781186548,
0.707106781186547,0.707106781186548,0.707106781186547,0.707106781186548,
0.707106781186547,0.707106781186547,0.707106781186547,0.707106781186548,
0.707106781186547,0.707106781186547,0.707106781186548,0.707106781186547,
0.707106781186548,0.707106781186547,0.707106781186548,0.707106781186548,
0.707106781186547,0.707106781186548,0.707106781186547,0.707106781186548,
0.707106781186548,0.707106781186548,0.707106781186548,0.707106781186547,
0.707106781186547,0.707106781186548,0.707106781186547,0.707106781186547,
0.707106781186548,0.707106781186548,0.707106781186547,0.707106781186547,
0.707106781186548,0.707106781186547,0.707106781186547,0.707106781186548,
0.707106781186547,0.707106781186548,0.707106781186547,0.707106781186548,
0.707106781186547,0.707106781186547,0.707106781186547,0.707106781186548,
0.707106781186547,0.707106781186547,0.707106781186548,0.707106781186547,
0.707106781186548,0.707106781186548,0.707106781186548,0.707106781186547,
0.707106781186547,0.707106781186547,0.707106781186548,0.707106781186548,
0.707106781186547,0.707106781186547,0.707106781186547,0.707106781186547,
0.707106781186548,0.707106781186548,0.707106781186547,0.707106781186547,
0.707106781186547,0.707106781186548,0.707106781186548,0.707106781186547,
0.707106781186548,0.707106781186547,0.707106781186548,0.707106781186547,
0.707106781186548,0.707106781186548,0.707106781186547,0.707106781186548,
0.707106781186548,0.707106781186548,0.707106781186547,0.707106781186547,
0.707106781186547,0.707106781186548,0.707106781186548,0.707106781186548,
0.707106781186547,0.707106781186547,0.707106781186548,0.707106781186548,
0.707106781186547,0.707106781186548,0.707106781186547,0.707106781186547,
0.707106781186548,0.707106781186547,0.707106781186548,0.707106781186547,
0.707106781186547,0.707106781186548,0.707106781186547,0.707106781186548,
0.707106781186548,0.707106781186547,0.707106781186547,0.707106781186548,
0.707106781186547,0.707106781186548,0.707106781186547,0.707106781186547,
0.707106781186548,0.707106781186547,0.707106781186548,0.707106781186547,
0.707106781186548,0.707106781186547,0.707106781186547,0.707106781186548,
0.707106781186547,0.707106781186547,0.707106781186547,0.707106781186547,
0.707106781186547,0.707106781186547,0.707106781186548,0.707106781186547,
0.707106781186548,0.707106781186548,0.707106781186548,0.707106781186547,
0.707106781186547,0.707106781186547,0.707106781186548,0.707106781186547,
0.707106781186548,0.707106781186547,0.707106781186547,0.707106781186548,
0.707106781186547,0.707106781186547,0.707106781186547,0.707106781186547,
0.707106781186547,0.707106781186548,0.707106781186547,0.707106781186548,
0.707106781186547,0.707106781186547,0.707106781186548,0.707106781186548,
0.707106781186547,0.707106781186547,0.707106781186547,0.707106781186548,
0.707106781186547,0.707106781186547,0.707106781186548,0.707106781186548,
0.707106781186547,0.707106781186548,0.707106781186547,0.707106781186548,
0.707106781186548,0.707106781186547,0.707106781186547,0.707106781186547,
0.707106781186548,0.707106781186548,0.707106781186547,0.707106781186548,
0.707106781186547,0.707106781186548,0.707106781186548,0.707106781186547,
0.707106781186548,0.707106781186547,0.707106781186547,0.707106781186547,
0.707106781186548,0.707106781186547,0.707106781186548,0.707106781186547,
0.707106781186548,0.707106781186547,0.707106781186547,0.707106781186547,
0.707106781186547,0.707106781186547,0.707106781186548,0.707106781186547,
0.707106781186548,0.707106781186547,0.707106781186548,0.707106781186547,
0.707106781186548,0.707106781186547,0.707106781186547,0.707106781186547,
0.707106781186547,0.707106781186547,0.707106781186548,0.707106781186548,
0.707106781186548,0.707106781186547,0.707106781186548,0.707106781186547,
0.707106781186548,0.707106781186547,0.707106781186547,0.707106781186548,
0.707106781186547,0.707106781186548,0.707106781186547,0.707106781186547,
0.707106781186547,0.707106781186548,0.707106781186548,0.707106781186547,
0.707106781186548,0.707106781186547,0.707106781186548,0.707106781186548,
0.707106781186547,0.707106781186548,0.707106781186547,0.707106781186548,
0.707106781186548,0.707106781186547,0.707106781186547,0.707106781186547,
0.707106781186547,0.707106781186547,0.707106781186547,0.707106781186548,
0.707106781186548,0.707106781186547,0.707106781186548,0.707106781186547,
0.707106781186547,0.707106781186548,0.707106781186547,0.707106781186547,
0.707106781186548,0.707106781186547,0.707106781186547,0.707106781186547,
0.707106781186548,0.707106781186547,0.707106781186547,0.707106781186548,
0.707106781186547,0.707106781186548,0.707106781186548,0.707106781186547,
0.707106781186547,0.707106781186547,0.707106781186548,0.707106781186547,
0.707106781186547,0.707106781186548,0.707106781186548,0.707106781186548,
0.707106781186548,0.707106781186547,0.707106781186548,0.707106781186548,
0.707106781186547,0.707106781186547,0.707106781186548,0.707106781186547,
0.707106781186548,0.707106781186547,0.707106781186547,0.707106781186548,
0.707106781186547,0.707106781186547,0.707106781186548,0.707106781186547,
0.707106781186548,0.707106781186547,0.707106781186548,0.707106781186547,
0.707106781186548,0.707106781186547,0.707106781186548,0.707106781186547,
0.707106781186548,0.707106781186548,0.707106781186547,0.707106781186547,
0.707106781186548,0.707106781186548,0.707106781186547,0.707106781186547,
0.707106781186547,0.707106781186547,0.707106781186547,0.707106781186548,
0.707106781186547,0.707106781186547,0.707106781186548,0.707106781186547,
0.707106781186548,0.707106781186548,0.707106781186547,0.707106781186548,
0.707106781186547,0.707106781186548,0.707106781186547,0.707106781186548,
0.707106781186547,0.707106781186547,0.707106781186547,0.707106781186547,
0.707106781186547,0.707106781186547,0.707106781186548,0.707106781186547,
0.707106781186548,0.707106781186547,0.707106781186547,0.707106781186547,
0.707106781186548,0.707106781186547,0.707106781186548,0.707106781186548,
0.707106781186547,0.707106781186547,0.707106781186548,0.707106781186547,
0.707106781186548,0.707106781186547,0.707106781186548,0.707106781186547,
0.707106781186548,0.707106781186547,0.707106781186547,0.707106781186548,
0.707106781186547,0.707106781186548,0.707106781186547,0.707106781186548,
0.707106781186548,0.707106781186548,0.707106781186548,0.707106781186547,
0.707106781186548,0.707106781186548,0.707106781186548,0.707106781186547,
0.707106781186548,0.707106781186548,0.707106781186547,0.707106781186548,
0.707106781186547,0.707106781186548,0.707106781186547,0.707106781186547,
0.707106781186547,0.707106781186548,0.707106781186548,0.707106781186547,
0.707106781186548,0.707106781186547,0.707106781186548,0.707106781186547,
0.707106781186548,0.707106781186548,0.707106781186547,0.707106781186548,
0.707106781186547,0.707106781186547,0.707106781186548,0.707106781186547,
0.707106781186547,0.707106781186547,0.707106781186548,0.707106781186547,
0.707106781186548,0.707106781186548,0.707106781186547,0.707106781186548,
0.707106781186547,0.707106781186548,0.707106781186548,0.707106781186548,
0.707106781186548,0.707106781186547,0.707106781186548,0.707106781186547,
0.707106781186548,0.707106781186547,0.707106781186548,0.707106781186547,
0.707106781186547,0.707106781186547,0.707106781186547,0.707106781186548,
0.707106781186547,0.707106781186548,0.707106781186547,0.707106781186547,
0.707106781186548,0.707106781186547,0.707106781186548,0.707106781186547,
0.707106781186548,0.707106781186547,0.707106781186548,0.707106781186548,
0.707106781186548,0.707106781186548,0.707106781186547,0.707106781186548,
0.707106781186548,0.707106781186547,0.707106781186548,0.707106781186547,
0.707106781186548,0.707106781186547,0.707106781186548,0.707106781186547,
0.707106781186547,0.707106781186548,0.707106781186547,0.707106781186548,
0.707106781186547,0.707106781186547,0.707106781186548,0.707106781186547,
0.707106781186548,0.707106781186547,0.707106781186547,0.707106781186548,
0.707106781186548,0.707106781186548,0.707106781186548,0.707106781186548,
0.707106781186548,0.707106781186548,0.707106781186548,0.707106781186548,
0.707106781186547,0.707106781186548,0.707106781186547,0.707106781186547,
0.707106781186548,0.707106781186547,0.707106781186548,0.707106781186548,
0.707106781186547,0.707106781186547,0.707106781186548,0.707106781186548,
0.707106781186547,0.707106781186547,0.707106781186547,0.707106781186547,
0.707106781186547,0.707106781186548,0.707106781186547,0.707106781186548,
0.707106781186548,0.707106781186548,0.707106781186547,0.707106781186548,
0.707106781186547,0.707106781186548,0.707106781186547,0.707106781186548,
0.707106781186547,0.707106781186548,0.707106781186548,0.707106781186547,
0.707106781186547,0.707106781186548,0.707106781186548,0.707106781186548,
0.707106781186547,0.707106781186547,0.707106781186548,0.707106781186547,
0.707106781186547,0.707106781186548,0.707106781186547,0.707106781186548,
0.707106781186547,0.707106781186547,0.707106781186548,0.707106781186548,
0.707106781186548,0.707106781186547,0.707106781186547,0.707106781186548,
0.707106781186547,0.707106781186548,0.707106781186547,0.707106781186548,
0.707106781186547,0.707106781186548,0.707106781186548,0.707106781186547,
0.707106781186548,0.707106781186547,0.707106781186548,0.707106781186547,
0.707106781186547,0.707106781186547,0.707106781186548,0.707106781186547,
0.707106781186548,0.707106781186547,0.707106781186547,0.707106781186547,
0.707106781186548,0.707106781186547,0.707106781186547,0.707106781186548,
0.707106781186548,0.707106781186547,0.707106781186548,0.707106781186547,
0.707106781186548,0.707106781186548,0.707106781186547,0.707106781186548,
0.707106781186547,0.707106781186547,0.707106781186548,0.707106781186547,
0.707106781186547,0.707106781186547,0.707106781186548,0.707106781186547,
0.707106781186548,0.707106781186547,0.707106781186548,0.707106781186548,
0.707106781186548,0.707106781186547,0.707106781186548,0.707106781186548,
0.707106781186548,0.707106781186547,0.707106781186548,0.707106781186547,
0.707106781186547,0.707106781186548,0.707106781186547,0.707106781186547,
0.707106781186548,0.707106781186548,0.707106781186547,0.707106781186548,
0.707106781186547,0.707106781186548,0.707106781186548,0.707106781186547,
0.707106781186548,0.707106781186547,0.707106781186548,0.707106781186547,
0.707106781186548,0.707106781186547,0.707106781186548,0.707106781186548,
0.707106781186548,0.707106781186547,0.707106781186548,0.707106781186548,
0.707106781186547,0.707106781186547,0.707106781186548,0.707106781186547,
0.707106781186548,0.707106781186548,0.707106781186547,0.707106781186548,
0.707106781186548,0.707106781186547,0.707106781186548,0.707106781186548,
0.707106781186547,0.707106781186547,0.707106781186548,0.707106781186547,
0.707106781186548,0.707106781186547,0.707106781186548,0.707106781186547,
0.707106781186548,0.707106781186548,0.707106781186548,0.707106781186547,
0.707106781186548,0.707106781186547,0.707106781186548,0.707106781186547,
0.707106781186548,0.707106781186547,0.707106781186548,0.707106781186547,
0.707106781186548,0.707106781186547,0.707106781186548,0.707106781186547,
0.707106781186547,0.707106781186547,0.707106781186548,0.707106781186547,
0.707106781186548,0.707106781186547,0.707106781186548,0.707106781186547,
0.707106781186548,0.707106781186547,0.707106781186548,0.707106781186548,
0.707106781186548,0.707106781186547,0.707106781186548,0.707106781186547,
0.707106781186548,0.707106781186548,0.707106781186547,0.707106781186548,
0.707106781186547,0.707106781186548,0.707106781186547,0.707106781186548,
0.707106781186547,0.707106781186548,0.707106781186547,0.707106781186547,
0.707106781186547,0.707106781186548,0.707106781186547,0.707106781186547,
0.707106781186548,0.707106781186547,0.707106781186548,0.707106781186547,
0.707106781186547,0.707106781186548,0.707106781186547,0.707106781186548,
0.707106781186547,0.707106781186548,0.707106781186548,0.707106781186548,
0.707106781186547,0.707106781186547,0.707106781186548,0.707106781186548,
0.707106781186547,0.707106781186548,0.707106781186547,0.707106781186547,
0.707106781186547,0.707106781186548,0.707106781186547,0.707106781186548,
0.707106781186547,0.707106781186548,0.707106781186548,0.707106781186548,
0.707106781186547,0.707106781186547,0.707106781186547,0.707106781186547,
0.707106781186547,0.707106781186547,0.707106781186548,0.707106781186547,
0.707106781186548,0.707106781186547,0.707106781186548,0.707106781186547,
0.707106781186547,0.707106781186548,0.707106781186547,0.707106781186547,
0.707106781186548,0.707106781186548,0.707106781186547,0.707106781186547,
0.707106781186547,0.707106781186548,0.707106781186547,0.707106781186547,
0.707106781186548,0.707106781186548),(1.,1.,1.,1.,1.,1.,1.,1.,1.,1.,1.,
1.,1.,1.,1.,1.,1.,1.,1.,1.,1.,1.,1.,1.,1.,1.,1.,1.,1.,1.,1.,1.,1.,1.,1.,
1.,1.,1.,1.,1.,1.,1.,1.,1.,1.,1.,1.,1.,1.,1.,1.,1.,1.,1.,1.,1.,1.,1.,1.,
1.,1.,1.,1.,1.,1.,1.,1.,1.,1.,1.,1.,1.,1.,1.,1.,1.,1.,1.,1.,1.,1.,1.,1.,
1.,1.,1.,1.,1.,1.,1.,1.,1.,1.,1.,1.,1.,1.,1.,1.,1.,1.,1.,1.,1.,1.,1.,1.,
1.,1.,1.,1.,1.,1.,1.,1.,1.,1.,1.,1.,1.,1.,1.,1.,1.,1.,1.,1.,1.,1.,1.,1.,
1.,1.,1.,1.,1.,1.,1.,1.,1.,1.,1.,1.,1.,1.,1.,1.,1.,1.,1.,1.,1.,1.,1.,1.,
1.,1.,1.,1.,1.,1.,1.,1.,1.,1.,1.,1.,1.,1.,1.,1.,1.,1.,1.,1.,1.,1.,1.,1.,
1.,1.,1.,1.,1.,1.,1.,1.,1.,1.,1.,1.,1.,1.,1.,1.,1.,1.,1.,1.,1.,1.,1.,1.,
1.,1.,1.,1.,1.,1.,1.,1.,1.,1.,1.,1.,1.,1.,1.,1.,1.,1.,1.,1.,1.,1.,1.,1.,
1.,1.,1.,1.,1.,1.,1.,1.,1.,1.,1.,1.,1.,1.,1.,1.,1.,1.,1.,1.,1.,1.,1.,1.,
1.,1.,1.,1.,1.,1.,1.,1.,1.,1.,1.,1.,1.,1.,1.,1.,1.,1.,1.,1.,1.,1.,1.,1.,
1.,1.,1.,1.,1.,1.,1.,1.,1.,1.,1.,1.,1.,1.,1.,1.,1.,1.,1.,1.,1.,1.,1.,1.,
1.,1.,1.,1.,1.,1.,1.,1.,1.,1.,1.,1.,1.,1.,1.,1.,1.,1.,1.,1.,1.,1.,1.,1.,
1.,1.,1.,1.,1.,1.,1.,1.,1.,1.,1.,1.,1.,1.,1.,1.,1.,1.,1.,1.,1.,1.,1.,1.,
1.,1.,1.,1.,1.,1.,1.,1.,1.,1.,1.,1.,1.,1.,1.,1.,1.,1.,1.,1.,1.,1.,1.,1.,
1.,1.,1.,1.,1.,1.,1.,1.,1.,1.,1.,1.,1.,1.,1.,1.,1.,1.,1.,1.,1.,1.,1.,1.,
1.,1.,1.,1.,1.,1.,1.,1.,1.,1.,1.,1.,1.,1.,1.,1.,1.,1.,1.,1.,1.,1.,1.,1.,
1.,1.,1.,1.,1.,1.,1.,1.,1.,1.,1.,1.,1.,1.,1.,1.,1.,1.,1.,1.,1.,1.,1.,1.,
1.,1.,1.,1.,1.,1.,1.,1.,1.,1.,1.,1.,1.,1.,1.,1.,1.,1.,1.,1.,1.,1.,1.,1.,
1.,1.,1.,1.,1.,1.,1.,1.,1.,1.,1.,1.,1.,1.,1.,1.,1.,1.,1.,1.,1.,1.,1.,1.,
1.,1.,1.,1.,1.,1.,1.,1.,1.,1.,1.,1.,1.,1.,1.,1.,1.,1.,1.,1.,1.,1.,1.,1.,
1.,1.,1.,1.,1.,1.,1.,1.,1.,1.,1.,1.,1.,1.,1.,1.,1.,1.,1.,1.,1.,1.,1.,1.,
1.,1.,1.,1.,1.,1.,1.,1.,1.,1.,1.,1.,1.,1.,1.,1.,1.,1.,1.,1.,1.,1.,1.,1.,
1.,1.,1.,1.,1.,1.,1.,1.,1.,1.,1.,1.,1.,1.,1.,1.,1.,1.,1.,1.,1.,1.,1.,1.,
1.,1.,1.,1.,1.,1.,1.,1.,1.,1.,1.,1.,1.,1.,1.,1.,1.,1.,1.,1.,1.,1.,1.,1.,
1.,1.,1.,1.,1.,1.,1.,1.,1.,1.,1.,1.,1.,1.,1.,1.,1.,1.,1.,1.,1.,1.,1.,1.,
1.,1.,1.,1.,1.,1.,1.,1.,1.,1.,1.,1.,1.,1.,1.,1.,1.,1.,1.,1.,1.,1.,1.,1.,
1.,1.,1.,1.,1.,1.,1.,1.,1.,1.,1.,1.,1.,1.,1.,1.,1.,1.,1.,1.,1.,1.,1.,1.,
1.,1.,1.,1.,1.,1.,1.,1.,1.,1.,1.,1.,1.,1.,1.,1.,1.,1.,1.,1.,1.,1.,1.,1.,
1.,1.,1.,1.,1.,1.,1.,1.,1.,1.,1.,1.,1.,1.,1.,1.,1.,1.,1.,1.,1.,1.,1.,1.,
1.,1.,1.,1.,1.,1.,1.,1.,1.,1.,1.,1.,1.,1.,1.,1.,1.,1.,1.,1.,1.,1.,1.,1.,
1.,1.,1.,1.,1.,1.,1.,1.,1.,1.,1.,1.,1.,1.,1.,1.,1.,1.,1.,1.,1.,1.,1.,1.,
1.,1.,1.,1.,1.,1.,1.,1.,1.,1.,1.,1.,1.,1.,1.,1.,1.,1.,1.,1.,1.,1.,1.,1.,
1.,1.,1.,1.,1.,1.,1.,1.,1.,1.,1.,1.,1.,1.,1.,1.,1.,1.,1.,1.,1.,1.,1.,1.,
1.,1.,1.,1.,1.,1.,1.,1.,1.,1.,1.,1.,1.,1.,1.,1.,1.,1.,1.,1.,1.,1.,1.,1.,
1.,1.,1.,1.,1.,1.,1.,1.,1.,1.,1.,1.,1.,1.,1.,1.,1.,1.,1.,1.,1.,1.,1.,1.,
1.,1.,1.,1.,1.,1.,1.,1.,1.,1.,1.,1.,1.,1.,1.,1.,1.,1.,1.,1.,1.,1.,1.,1.,
1.,1.,1.,1.,1.,1.,1.,1.,1.,1.,1.,1.,1.,1.,1.,1.,1.,1.,1.,1.,1.,1.,1.,1.,
1.,1.,1.,1.,1.,1.,1.,1.,1.,1.,1.,1.,1.,1.,1.,1.,1.,1.,1.,1.,1.,1.,1.,1.,
1.,1.,1.,1.,1.,1.,1.,1.,1.,1.,1.,1.,1.,1.,1.,1.,1.,1.,1.,1.,1.,1.,1.,1.,
1.,1.,1.,1.,1.,1.,1.,1.,1.,1.,1.,1.,1.,1.,1.,1.,1.,1.,1.,1.,1.,1.,1.,1.,
1.,1.,1.,1.,1.,1.,1.,1.,1.,1.,1.,1.,1.,1.,1.,1.,1.,1.,1.,1.,1.,1.,1.,1.,
1.,1.,1.,1.,1.,1.,1.,1.,1.,1.,1.,1.,1.,1.,1.,1.,1.,1.,1.,1.,1.,1.,1.,1.,
1.,1.,1.,1.,1.,1.,1.,1.,1.,1.,1.,1.,1.,1.,1.,1.,1.,1.,1.,1.,1.,1.,1.,1.,
1.,1.,1.,1.,1.,1.,1.,1.,1.,1.,1.,1.,1.,1.,1.,1.,1.,1.,1.,1.,1.,1.,1.,1.,
1.,1.,1.,1.,1.,1.,1.,1.,1.,1.,1.,1.,1.,1.,1.,1.,1.,1.,1.,1.,1.,1.,1.,1.,
1.,1.,1.,1.,1.,1.,1.,1.,1.,1.,1.,1.,1.,1.,1.,1.,1.,1.,1.,1.,1.,1.,1.,1.,
1.,1.,1.,1.,1.,1.,1.,1.,1.,1.,1.,1.,1.,1.,1.,1.,1.,1.,1.,1.,1.,1.,1.,1.,
1.,1.,1.,1.,1.,1.,1.,1.,1.,1.,1.,1.,1.,1.,1.,1.,1.,1.,1.,1.,1.,1.,1.,1.,
1.,1.,1.,1.,1.,1.,1.,1.,1.,1.,1.,1.,1.,1.,1.,1.,1.,1.,1.,1.,1.,1.,1.,1.,
1.,1.,1.,1.,1.,1.,1.,1.,1.,1.,1.,1.,1.,1.,1.,1.,1.,1.,1.,1.,1.,1.,1.,1.,
1.,1.,1.,1.,1.,1.,1.,1.,1.,1.,1.,1.,1.,1.,1.,1.,1.,1.,1.,1.,1.,1.,1.,1.,
1.,1.,1.,1.,1.,1.,1.,1.,1.,1.,1.,1.,1.,1.,1.,1.,1.,1.,1.,1.,1.,1.,1.,1.,
1.,1.,1.,1.,1.,1.,1.,1.,1.,1.,1.,1.,1.,1.,1.,1.,1.,1.,1.,1.,1.,1.,1.,1.,
1.,1.,1.,1.,1.,1.,1.,1.,1.,1.,1.,1.,1.,1.,1.,1.,1.,1.,1.,1.,1.,1.,1.,1.,
1.,1.,1.,1.,1.,1.,1.,1.,1.,1.,1.,1.,1.,1.,1.,1.,1.,1.,1.,1.,1.,1.,1.,1.,
1.,1.,1.,1.,1.,1.,1.,1.,1.,1.,1.,1.,1.,1.,1.,1.,1.,1.,1.,1.,1.,1.,1.,1.,
1.,1.,1.,1.,1.,1.,1.,1.,1.,1.,1.,1.,1.,1.,1.,1.,1.,1.,1.,1.,1.,1.,1.,1.,
1.,1.,1.,1.,1.,1.,1.,1.,1.,1.,1.,1.,1.,1.,1.,1.,1.,1.,1.,1.,1.,1.,1.,1.,
1.,1.,1.,1.,1.,1.,1.,1.,1.,1.,1.,1.,1.,1.,1.,1.,1.,1.,1.,1.,1.,1.,1.,1.,
1.,1.,1.,1.,1.,1.,1.,1.,1.,1.,1.,1.,1.,1.,1.,1.,1.,1.,1.,1.,1.,1.,1.,1.,
1.,1.,1.,1.,1.,1.,1.,1.,1.,1.,1.,1.,1.,1.,1.,1.,1.,1.,1.,1.,1.,1.,1.,1.,
1.,1.,1.,1.,1.,1.,1.,1.,1.,1.,1.,1.,1.,1.,1.,1.,1.,1.,1.,1.,1.,1.,1.,1.,
1.,1.,1.,1.,1.,1.,1.,1.,1.,1.,1.,1.,1.,1.,1.,1.,1.,1.,1.,1.,1.,1.,1.,1.,
1.,1.,1.,1.,1.,1.,1.,1.,1.,1.,1.,1.,1.,1.,1.,1.,1.,1.,1.,1.,1.,1.,1.,1.,
1.,1.,1.,1.,1.,1.,1.,1.,1.,1.,1.,1.,1.,1.,1.,1.,1.,1.,1.,1.,1.,1.,1.,1.,
1.,1.,1.,1.,1.,1.,1.,1.,1.,1.,1.,1.,1.,1.,1.,1.,1.,1.,1.,1.,1.,1.,1.,1.,
1.,1.,1.,1.,1.,1.,1.,1.,1.,1.,1.,1.,1.,1.,1.,1.,1.,1.,1.,1.,1.,1.,1.,1.,
1.,1.,1.,1.,1.,1.,1.,1.,1.,1.,1.,1.,1.,1.,1.,1.,1.,1.,1.,1.,1.,1.,1.,1.,
1.,1.,1.,1.,1.,1.,1.,1.,1.,1.,1.,1.,1.,1.,1.,1.,1.,1.,1.,1.,1.,1.,1.,1.,
1.,1.,1.,1.,1.,1.,1.,1.,1.,1.,1.,1.,1.,1.,1.,1.,1.,1.,1.,1.,1.,1.,1.,1.,
1.,1.,1.,1.,1.,1.,1.,1.,1.,1.,1.,1.,1.,1.,1.,1.,1.,1.,1.,1.,1.,1.,1.,1.,
1.,1.,1.,1.,1.,1.,1.,1.,1.,1.,1.,1.,1.,1.,1.,1.,1.,1.,1.,1.,1.,1.,1.,1.,
1.,1.,1.,1.,1.,1.,1.,1.,1.,1.,1.,1.,1.,1.,1.,1.,1.,1.,1.,1.,1.,1.,1.,1.,
1.,1.,1.,1.,1.,1.,1.,1.,1.,1.,1.,1.,1.,1.,1.,1.,1.,1.,1.,1.,1.,1.,1.,1.,
1.,1.,1.,1.,1.,1.,1.,1.,1.,1.,1.,1.,1.,1.,1.,1.,1.,1.,1.,1.,1.,1.,1.,1.,
1.,1.,1.,1.,1.,1.,1.,1.,1.,1.,1.,1.,1.,1.,1.,1.,1.,1.,1.,1.,1.,1.,1.,1.,
1.,1.,1.,1.,1.,1.,1.,1.,1.,1.,1.,1.,1.,1.,1.,1.,1.,1.,1.,1.,1.,1.,1.,1.,
1.,1.,1.,1.,1.,1.,1.,1.,1.,1.,1.,1.,1.,1.,1.,1.,1.,1.,1.,1.,1.,1.,1.,1.,
1.,1.,1.,1.,1.,1.,1.,1.,1.,1.,1.,1.,1.,1.,1.,1.,1.,1.,1.,1.,1.,1.,1.,1.,
1.,1.,1.,1.,1.,1.,1.,1.,1.,1.,1.,1.,1.,1.,1.,1.,1.,1.,1.,1.,1.,1.,1.,1.,
1.,1.,1.,1.,1.,1.,1.,1.,1.,1.,1.,1.,1.,1.,1.,1.,1.,1.,1.,1.,1.,1.,1.,1.,
1.,1.,1.,1.,1.,1.,1.,1.,1.,1.,1.,1.,1.,1.,1.,1.,1.,1.,1.,1.,1.,1.,1.,1.,
1.,1.,1.,1.,1.,1.,1.,1.,1.,1.,1.,1.,1.,1.,1.,1.,1.,1.,1.,1.,1.,1.,1.,1.,
1.,1.,1.,1.,1.,1.,1.,1.,1.,1.,1.,1.,1.,1.,1.,1.,1.,1.,1.,1.,1.,1.,1.,1.),
(0.707106781186548,0.707106781186548,0.707106781186548,0.707106781186547,
0.707106781186547,0.707106781186548,0.707106781186547,0.707106781186547,
0.707106781186547,0.707106781186547,0.707106781186547,0.707106781186548,
0.707106781186548,0.707106781186548,0.707106781186547,0.707106781186548,
0.707106781186547,0.707106781186547,0.707106781186548,0.707106781186547,
0.707106781186548,0.707106781186547,0.707106781186548,0.707106781186547,
0.707106781186548,0.707106781186547,0.707106781186547,0.707106781186547,
0.707106781186547,0.707106781186547,0.707106781186548,0.707106781186547,
0.707106781186547,0.707106781186548,0.707106781186547,0.707106781186547,
0.707106781186548,0.707106781186547,0.707106781186547,0.707106781186548,
0.707106781186548,0.707106781186547,0.707106781186548,0.707106781186547,
0.707106781186547,0.707106781186547,0.707106781186548,0.707106781186548,
0.707106781186547,0.707106781186547,0.707106781186548,0.707106781186547,
0.707106781186548,0.707106781186547,0.707106781186547,0.707106781186547,
0.707106781186547,0.707106781186547,0.707106781186548,0.707106781186547,
0.707106781186548,0.707106781186547,0.707106781186548,0.707106781186547,
0.707106781186548,0.707106781186547,0.707106781186547,0.707106781186548,
0.707106781186547,0.707106781186547,0.707106781186548,0.707106781186547,
0.707106781186548,0.707106781186547,0.707106781186548,0.707106781186548,
0.707106781186547,0.707106781186548,0.707106781186547,0.707106781186547,
0.707106781186548,0.707106781186547,0.707106781186547,0.707106781186547,
0.707106781186548,0.707106781186547,0.707106781186547,0.707106781186547,
0.707106781186547,0.707106781186547,0.707106781186547,0.707106781186548,
0.707106781186548,0.707106781186547,0.707106781186548,0.707106781186547,
0.707106781186548,0.707106781186548,0.707106781186547,0.707106781186548,
0.707106781186548,0.707106781186548,0.707106781186547,0.707106781186548,
0.707106781186547,0.707106781186548,0.707106781186548,0.707106781186548,
0.707106781186547,0.707106781186547,0.707106781186547,0.707106781186548,
0.707106781186548,0.707106781186548,0.707106781186547,0.707106781186547,
0.707106781186547,0.707106781186548,0.707106781186548,0.707106781186547,
0.707106781186547,0.707106781186548,0.707106781186547,0.707106781186547,
0.707106781186547,0.707106781186547,0.707106781186548,0.707106781186547,
0.707106781186548,0.707106781186547,0.707106781186547,0.707106781186547,
0.707106781186548,0.707106781186548,0.707106781186547,0.707106781186548,
0.707106781186548,0.707106781186547,0.707106781186548,0.707106781186547,
0.707106781186548,0.707106781186547,0.707106781186548,0.707106781186547,
0.707106781186547,0.707106781186548,0.707106781186547,0.707106781186547,
0.707106781186548,0.707106781186547,0.707106781186547,0.707106781186548,
0.707106781186547,0.707106781186548,0.707106781186547,0.707106781186547,
0.707106781186548,0.707106781186548,0.707106781186547,0.707106781186548,
0.707106781186547,0.707106781186548,0.707106781186547,0.707106781186548,
0.707106781186547,0.707106781186548,0.707106781186547,0.707106781186548,
0.707106781186547,0.707106781186548,0.707106781186547,0.707106781186548,
0.707106781186547,0.707106781186547,0.707106781186548,0.707106781186547,
0.707106781186548,0.707106781186547,0.707106781186548,0.707106781186547,
0.707106781186548,0.707106781186547,0.707106781186547,0.707106781186548,
0.707106781186547,0.707106781186548,0.707106781186548,0.707106781186548,
0.707106781186547,0.707106781186547,0.707106781186547,0.707106781186547,
0.707106781186548,0.707106781186547,0.707106781186548,0.707106781186548,
0.707106781186547,0.707106781186547,0.707106781186548,0.707106781186548,
0.707106781186547,0.707106781186547,0.707106781186548,0.707106781186547,
0.707106781186548,0.707106781186547,0.707106781186547,0.707106781186547,
0.707106781186547,0.707106781186547,0.707106781186547,0.707106781186547,
0.707106781186548,0.707106781186547,0.707106781186548,0.707106781186547,
0.707106781186548,0.707106781186548,0.707106781186547,0.707106781186548,
0.707106781186548,0.707106781186548,0.707106781186548,0.707106781186547,
0.707106781186548,0.707106781186547,0.707106781186548,0.707106781186547,
0.707106781186547,0.707106781186548,0.707106781186548,0.707106781186547,
0.707106781186547,0.707106781186547,0.707106781186547,0.707106781186547,
0.707106781186548,0.707106781186548,0.707106781186547,0.707106781186547,
0.707106781186548,0.707106781186548,0.707106781186547,0.707106781186548,
0.707106781186547,0.707106781186548,0.707106781186548,0.707106781186547,
0.707106781186547,0.707106781186548,0.707106781186547,0.707106781186547,
0.707106781186548,0.707106781186547,0.707106781186548,0.707106781186547,
0.707106781186548,0.707106781186547,0.707106781186547,0.707106781186548,
0.707106781186548,0.707106781186547,0.707106781186547,0.707106781186548,
0.707106781186547,0.707106781186547,0.707106781186548,0.707106781186547,
0.707106781186548,0.707106781186547,0.707106781186548,0.707106781186547,
0.707106781186548,0.707106781186547,0.707106781186547,0.707106781186547,
0.707106781186547,0.707106781186547,0.707106781186547,0.707106781186548,
0.707106781186547,0.707106781186548,0.707106781186547,0.707106781186548,
0.707106781186548,0.707106781186547,0.707106781186548,0.707106781186548,
0.707106781186547,0.707106781186548,0.707106781186547,0.707106781186547,
0.707106781186547,0.707106781186548,0.707106781186547,0.707106781186547,
0.707106781186548,0.707106781186547,0.707106781186548,0.707106781186547,
0.707106781186547,0.707106781186547,0.707106781186548,0.707106781186548,
0.707106781186547,0.707106781186548,0.707106781186548,0.707106781186547,
0.707106781186548,0.707106781186547,0.707106781186548,0.707106781186548,
0.707106781186547,0.707106781186548,0.707106781186548,0.707106781186548,
0.707106781186547,0.707106781186547,0.707106781186548,0.707106781186547,
0.707106781186548,0.707106781186547,0.707106781186547,0.707106781186548,
0.707106781186548,0.707106781186548,0.707106781186547,0.707106781186547,
0.707106781186548,0.707106781186548,0.707106781186547,0.707106781186547,
0.707106781186548,0.707106781186547,0.707106781186547,0.707106781186548,
0.707106781186548,0.707106781186547,0.707106781186547,0.707106781186547,
0.707106781186548,0.707106781186547,0.707106781186547,0.707106781186547,
0.707106781186548,0.707106781186548,0.707106781186547,0.707106781186548,
0.707106781186547,0.707106781186548,0.707106781186547,0.707106781186548,
0.707106781186548,0.707106781186547,0.707106781186547,0.707106781186548,
0.707106781186547,0.707106781186547,0.707106781186548,0.707106781186547,
0.707106781186548,0.707106781186548,0.707106781186547,0.707106781186548,
0.707106781186547,0.707106781186547,0.707106781186547,0.707106781186548,
0.707106781186548,0.707106781186548,0.707106781186547,0.707106781186548,
0.707106781186547,0.707106781186548,0.707106781186547,0.707106781186547,
0.707106781186547,0.707106781186547,0.707106781186548,0.707106781186548,
0.707106781186547,0.707106781186547,0.707106781186548,0.707106781186547,
0.707106781186548,0.707106781186547,0.707106781186548,0.707106781186547,
0.707106781186547,0.707106781186548,0.707106781186547,0.707106781186548,
0.707106781186547,0.707106781186548,0.707106781186548,0.707106781186547,
0.707106781186548,0.707106781186547,0.707106781186548,0.707106781186548,
0.707106781186547,0.707106781186548,0.707106781186547,0.707106781186547,
0.707106781186548,0.707106781186547,0.707106781186548,0.707106781186547,
0.707106781186548,0.707106781186547,0.707106781186547,0.707106781186548,
0.707106781186548,0.707106781186548,0.707106781186548,0.707106781186547,
0.707106781186548,0.707106781186548,0.707106781186548,0.707106781186547,
0.707106781186548,0.707106781186548,0.707106781186548,0.707106781186547,
0.707106781186547,0.707106781186548,0.707106781186547,0.707106781186548,
0.707106781186547,0.707106781186548,0.707106781186548,0.707106781186547,
0.707106781186547,0.707106781186548,0.707106781186547,0.707106781186548,
0.707106781186547,0.707106781186548,0.707106781186548,0.707106781186547,
0.707106781186547,0.707106781186547,0.707106781186548,0.707106781186548,
0.707106781186547,0.707106781186547,0.707106781186548,0.707106781186548,
0.707106781186548,0.707106781186548,0.707106781186547,0.707106781186547,
0.707106781186548,0.707106781186548,0.707106781186547,0.707106781186548,
0.707106781186547,0.707106781186548,0.707106781186547,0.707106781186548,
0.707106781186547,0.707106781186547,0.707106781186548,0.707106781186547,
0.707106781186547,0.707106781186548,0.707106781186547,0.707106781186548,
0.707106781186547,0.707106781186548,0.707106781186547,0.707106781186548,
0.707106781186547,0.707106781186548,0.707106781186547,0.707106781186548,
0.707106781186547,0.707106781186547,0.707106781186548,0.707106781186548,
0.707106781186547,0.707106781186547,0.707106781186547,0.707106781186548,
0.707106781186547,0.707106781186548,0.707106781186547,0.707106781186548,
0.707106781186547,0.707106781186548,0.707106781186547,0.707106781186547,
0.707106781186547,0.707106781186548,0.707106781186547,0.707106781186548,
0.707106781186548,0.707106781186547,0.707106781186548,0.707106781186547,
0.707106781186547,0.707106781186548,0.707106781186547,0.707106781186547,
0.707106781186548,0.707106781186547,0.707106781186547,0.707106781186547,
0.707106781186547,0.707106781186548,0.707106781186547,0.707106781186547,
0.707106781186547,0.707106781186548,0.707106781186547,0.707106781186547,
0.707106781186548,0.707106781186548,0.707106781186547,0.707106781186548,
0.707106781186548,0.707106781186547,0.707106781186547,0.707106781186548,
0.707106781186547,0.707106781186547,0.707106781186548,0.707106781186547,
0.707106781186547,0.707106781186547,0.707106781186548,0.707106781186547,
0.707106781186548,0.707106781186547,0.707106781186548,0.707106781186547,
0.707106781186548,0.707106781186547,0.707106781186548,0.707106781186547,
0.707106781186548,0.707106781186548,0.707106781186547,0.707106781186547,
0.707106781186548,0.707106781186547,0.707106781186548,0.707106781186547,
0.707106781186548,0.707106781186548,0.707106781186547,0.707106781186548,
0.707106781186547,0.707106781186548,0.707106781186548,0.707106781186547,
0.707106781186547,0.707106781186548,0.707106781186547,0.707106781186548,
0.707106781186547,0.707106781186548,0.707106781186547,0.707106781186548,
0.707106781186547,0.707106781186547,0.707106781186547,0.707106781186547,
0.707106781186547,0.707106781186547,0.707106781186547,0.707106781186547,
0.707106781186548,0.707106781186547,0.707106781186548,0.707106781186547,
0.707106781186547,0.707106781186548,0.707106781186547,0.707106781186548,
0.707106781186547,0.707106781186547,0.707106781186548,0.707106781186547,
0.707106781186548,0.707106781186547,0.707106781186548,0.707106781186547,
0.707106781186548,0.707106781186547,0.707106781186548,0.707106781186547,
0.707106781186548,0.707106781186547,0.707106781186548,0.707106781186548,
0.707106781186547,0.707106781186548,0.707106781186547,0.707106781186547,
0.707106781186547,0.707106781186548,0.707106781186547,0.707106781186547,
0.707106781186547,0.707106781186548,0.707106781186547,0.707106781186547,
0.707106781186548,0.707106781186547,0.707106781186547,0.707106781186547,
0.707106781186547,0.707106781186548,0.707106781186547,0.707106781186547,
0.707106781186547,0.707106781186548,0.707106781186548,0.707106781186548,
0.707106781186548,0.707106781186547,0.707106781186548,0.707106781186547,
0.707106781186547,0.707106781186548,0.707106781186547,0.707106781186548,
0.707106781186547,0.707106781186547,0.707106781186548,0.707106781186547,
0.707106781186547,0.707106781186547,0.707106781186547,0.707106781186548,
0.707106781186548,0.707106781186547,0.707106781186547,0.707106781186548,
0.707106781186547,0.707106781186548,0.707106781186547,0.707106781186548,
0.707106781186548,0.707106781186547,0.707106781186547,0.707106781186548,
0.707106781186548,0.707106781186547,0.707106781186548,0.707106781186548,
0.707106781186547,0.707106781186548,0.707106781186548,0.707106781186548,
0.707106781186547,0.707106781186548,0.707106781186547,0.707106781186548,
0.707106781186547,0.707106781186548,0.707106781186547,0.707106781186548,
0.707106781186547,0.707106781186548,0.707106781186548,0.707106781186547,
0.707106781186547,0.707106781186548,0.707106781186547,0.707106781186548,
0.707106781186547,0.707106781186548,0.707106781186548,0.707106781186548,
0.707106781186548,0.707106781186548,0.707106781186547,0.707106781186547,
0.707106781186547,0.707106781186547,0.707106781186548,0.707106781186547,
0.707106781186548,0.707106781186547,0.707106781186547,0.707106781186548,
0.707106781186548,0.707106781186547,0.707106781186548,0.707106781186547,
0.707106781186548,0.707106781186548,0.707106781186547,0.707106781186547,
0.707106781186548,0.707106781186547,0.707106781186548,0.707106781186547,
0.707106781186548,0.707106781186547,0.707106781186548,0.707106781186547,
0.707106781186548,0.707106781186547,0.707106781186548,0.707106781186547,
0.707106781186548,0.707106781186548,0.707106781186547,0.707106781186548,
0.707106781186547,0.707106781186548,0.707106781186547,0.707106781186548,
0.707106781186548,0.707106781186548,0.707106781186547,0.707106781186547,
0.707106781186548,0.707106781186548,0.707106781186547,0.707106781186547,
0.707106781186547,0.707106781186548,0.707106781186547,0.707106781186548,
0.707106781186547,0.707106781186548,0.707106781186547,0.707106781186547,
0.707106781186547,0.707106781186548,0.707106781186547,0.707106781186548,
0.707106781186547,0.707106781186548,0.707106781186547,0.707106781186548,
0.707106781186547,0.707106781186547,0.707106781186548,0.707106781186547,
0.707106781186547,0.707106781186548,0.707106781186547,0.707106781186547,
0.707106781186548,0.707106781186547,0.707106781186547,0.707106781186547,
0.707106781186548,0.707106781186547,0.707106781186548,0.707106781186547,
0.707106781186547,0.707106781186547,0.707106781186548,0.707106781186548,
0.707106781186547,0.707106781186547,0.707106781186548,0.707106781186548,
0.707106781186548,0.707106781186547,0.707106781186548,0.707106781186547,
0.707106781186548,0.707106781186547,0.707106781186548,0.707106781186547,
0.707106781186547,0.707106781186547,0.707106781186547,0.707106781186548,
0.707106781186547,0.707106781186548,0.707106781186548,0.707106781186547,
0.707106781186548,0.707106781186547,0.707106781186547,0.707106781186547,
0.707106781186547,0.707106781186548,0.707106781186547,0.707106781186548,
0.707106781186547,0.707106781186548,0.707106781186548,0.707106781186547,
0.707106781186548,0.707106781186547,0.707106781186547,0.707106781186547,
0.707106781186547,0.707106781186548,0.707106781186547,0.707106781186548,
0.707106781186548,0.707106781186547,0.707106781186548,0.707106781186547,
0.707106781186548,0.707106781186547,0.707106781186547,0.707106781186548,
0.707106781186547,0.707106781186548,0.707106781186548,0.707106781186547,
0.707106781186547,0.707106781186548,0.707106781186548,0.707106781186547,
0.707106781186547,0.707106781186548,0.707106781186547,0.707106781186547,
0.707106781186548,0.707106781186547,0.707106781186547,0.707106781186548,
0.707106781186547,0.707106781186548,0.707106781186547,0.707106781186547,
0.707106781186548,0.707106781186547,0.707106781186548,0.707106781186547,
0.707106781186548,0.707106781186547,0.707106781186547,0.707106781186547,
0.707106781186548,0.707106781186547,0.707106781186548,0.707106781186547,
0.707106781186548,0.707106781186548,0.707106781186548,0.707106781186548,
0.707106781186547,0.707106781186547,0.707106781186547,0.707106781186548,
0.707106781186547,0.707106781186548,0.707106781186547,0.707106781186547,
0.707106781186548,0.707106781186547,0.707106781186547,0.707106781186548,
0.707106781186547,0.707106781186547,0.707106781186548,0.707106781186548,
0.707106781186547,0.707106781186548,0.707106781186547,0.707106781186547,
0.707106781186548,0.707106781186547,0.707106781186548,0.707106781186547,
0.707106781186548,0.707106781186547,0.707106781186547,0.707106781186547,
0.707106781186548,0.707106781186547,0.707106781186548,0.707106781186547,
0.707106781186548,0.707106781186547,0.707106781186547,0.707106781186548,
0.707106781186548,0.707106781186548,0.707106781186547,0.707106781186548,
0.707106781186547,0.707106781186548,0.707106781186547,0.707106781186548,
0.707106781186547,0.707106781186548,0.707106781186548,0.707106781186547,
0.707106781186547,0.707106781186547,0.707106781186548,0.707106781186547,
0.707106781186547,0.707106781186548,0.707106781186547,0.707106781186547,
0.707106781186548,0.707106781186547,0.707106781186548,0.707106781186548,
0.707106781186548,0.707106781186547,0.707106781186548,0.707106781186547,
0.707106781186548,0.707106781186547,0.707106781186548,0.707106781186547,
0.707106781186548,0.707106781186547,0.707106781186548,0.707106781186547,
0.707106781186548,0.707106781186548,0.707106781186547,0.707106781186548,
0.707106781186547,0.707106781186548,0.707106781186548,0.707106781186547,
0.707106781186547,0.707106781186548,0.707106781186547,0.707106781186547,
0.707106781186548,0.707106781186547,0.707106781186548,0.707106781186548,
0.707106781186547,0.707106781186548,0.707106781186548,0.707106781186548,
0.707106781186548,0.707106781186548,0.707106781186547,0.707106781186548,
0.707106781186548,0.707106781186548,0.707106781186547,0.707106781186548,
0.707106781186547,0.707106781186548,0.707106781186547,0.707106781186548,
0.707106781186547,0.707106781186548,0.707106781186547,0.707106781186548,
0.707106781186547,0.707106781186547,0.707106781186548,0.707106781186547,
0.707106781186547,0.707106781186548,0.707106781186547,0.707106781186548,
0.707106781186547,0.707106781186548,0.707106781186547,0.707106781186548,
0.707106781186547,0.707106781186547,0.707106781186548,0.707106781186547,
0.707106781186547,0.707106781186548,0.707106781186547,0.707106781186548,
0.707106781186547,0.707106781186547,0.707106781186548,0.707106781186548,
0.707106781186547,0.707106781186548,0.707106781186547,0.707106781186547,
0.707106781186547,0.707106781186548,0.707106781186547,0.707106781186547,
0.707106781186548,0.707106781186547,0.707106781186547,0.707106781186547,
0.707106781186548,0.707106781186548,0.707106781186547,0.707106781186548,
0.707106781186547,0.707106781186548,0.707106781186547,0.707106781186547,
0.707106781186548,0.707106781186547,0.707106781186548,0.707106781186547,
0.707106781186547,0.707106781186547,0.707106781186547,0.707106781186548,
0.707106781186547,0.707106781186547,0.707106781186547,0.707106781186547,
0.707106781186547,0.707106781186548,0.707106781186547,0.707106781186547,
0.707106781186547,0.707106781186547,0.707106781186548,0.707106781186547,
0.707106781186548,0.707106781186547,0.707106781186547,0.707106781186548,
0.707106781186547,0.707106781186548,0.707106781186547,0.707106781186547,
0.707106781186548,0.707106781186547,0.707106781186547,0.707106781186548,
0.707106781186547,0.707106781186547,0.707106781186547,0.707106781186547,
0.707106781186548,0.707106781186547,0.707106781186548,0.707106781186548,
0.707106781186547,0.707106781186548,0.707106781186548,0.707106781186547,
0.707106781186547,0.707106781186548,0.707106781186547,0.707106781186547,
0.707106781186547,0.707106781186548,0.707106781186547,0.707106781186547,
0.707106781186548,0.707106781186547,0.707106781186548,0.707106781186547,
0.707106781186548,0.707106781186547,0.707106781186547,0.707106781186548,
0.707106781186547,0.707106781186548,0.707106781186547,0.707106781186548,
0.707106781186547,0.707106781186548,0.707106781186547,0.707106781186548,
0.707106781186547,0.707106781186547,0.707106781186547,0.707106781186547,
0.707106781186548,0.707106781186548,0.707106781186547,0.707106781186548,
0.707106781186548,0.707106781186547,0.707106781186548,0.707106781186547,
0.707106781186547,0.707106781186548,0.707106781186547,0.707106781186547,
0.707106781186547,0.707106781186547,0.707106781186548,0.707106781186547,
0.707106781186547,0.707106781186547,0.707106781186548,0.707106781186547,
0.707106781186547,0.707106781186548,0.707106781186547,0.707106781186548,
0.707106781186548,0.707106781186547,0.707106781186548,0.707106781186547,
0.707106781186548,0.707106781186547,0.707106781186548,0.707106781186547,
0.707106781186547,0.707106781186548,0.707106781186547,0.707106781186548,
0.707106781186548,0.707106781186547,0.707106781186547,0.707106781186548,
0.707106781186547,0.707106781186548,0.707106781186547,0.707106781186548,
0.707106781186547,0.707106781186547,0.707106781186548,0.707106781186548,
0.707106781186547,0.707106781186548,0.707106781186548,0.707106781186547,
0.707106781186548,0.707106781186548,0.707106781186547,0.707106781186548,
0.707106781186547,0.707106781186548,0.707106781186547,0.707106781186548,
0.707106781186547,0.707106781186548,0.707106781186547,0.707106781186547,
0.707106781186548,0.707106781186547,0.707106781186547,0.707106781186548,
0.707106781186547,0.707106781186548,0.707106781186548,0.707106781186547,
0.707106781186547,0.707106781186547,0.707106781186548,0.707106781186547,
0.707106781186548,0.707106781186548,0.707106781186547,0.707106781186548,
0.707106781186547,0.707106781186548,0.707106781186547,0.707106781186548,
0.707106781186547,0.707106781186547,0.707106781186548,0.707106781186548,
0.707106781186548,0.707106781186547,0.707106781186548,0.707106781186548,
0.707106781186547,0.707106781186548,0.707106781186547,0.707106781186548,
0.707106781186548,0.707106781186548,0.707106781186548,0.707106781186548,
0.707106781186548,0.707106781186547,0.707106781186547,0.707106781186548,
0.707106781186547,0.707106781186547,0.707106781186548,0.707106781186547,
0.707106781186547,0.707106781186548,0.707106781186547,0.707106781186548,
0.707106781186547,0.707106781186548,0.707106781186547,0.707106781186547,
0.707106781186547,0.707106781186548,0.707106781186547,0.707106781186547,
0.707106781186548,0.707106781186547,0.707106781186548,0.707106781186547,
0.707106781186548,0.707106781186547,0.707106781186547,0.707106781186547,
0.707106781186547,0.707106781186548,0.707106781186547,0.707106781186547,
0.707106781186548,0.707106781186548,0.707106781186547,0.707106781186548,
0.707106781186547,0.707106781186548,0.707106781186547,0.707106781186547,
0.707106781186548,0.707106781186547,0.707106781186548,0.707106781186547,
0.707106781186548,0.707106781186547,0.707106781186548,0.707106781186548,
0.707106781186547,0.707106781186548,0.707106781186547,0.707106781186547,
0.707106781186548,0.707106781186547,0.707106781186547,0.707106781186548,
0.707106781186548,0.707106781186548,0.707106781186547,0.707106781186548,
0.707106781186547,0.707106781186547,0.707106781186547,0.707106781186548,
0.707106781186547,0.707106781186548,0.707106781186548,0.707106781186548,
0.707106781186547,0.707106781186547,0.707106781186547,0.707106781186547,
0.707106781186548,0.707106781186547,0.707106781186547,0.707106781186548,
0.707106781186547,0.707106781186548,0.707106781186547,0.707106781186547,
0.707106781186548,0.707106781186547,0.707106781186548,0.707106781186547,
0.707106781186548,0.707106781186547,0.707106781186547,0.707106781186547,
0.707106781186547,0.707106781186547,0.707106781186547,0.707106781186548,
0.707106781186547,0.707106781186547,0.707106781186548,0.707106781186548,
0.707106781186547,0.707106781186548,0.707106781186548,0.707106781186547,
0.707106781186547,0.707106781186548,0.707106781186547,0.707106781186547,
0.707106781186548,0.707106781186547,0.707106781186548,0.707106781186548,
0.707106781186548,0.707106781186547,0.707106781186547,0.707106781186547,
0.707106781186547,0.707106781186548,0.707106781186548,0.707106781186548,
0.707106781186547,0.707106781186548,0.707106781186547,0.707106781186548,
0.707106781186548,0.707106781186547,0.707106781186548,0.707106781186547,
0.707106781186548,0.707106781186548,0.707106781186547,0.707106781186547,
0.707106781186548,0.707106781186547,0.707106781186548,0.707106781186547,
0.707106781186548,0.707106781186548,0.707106781186548,0.707106781186547,
0.707106781186548,0.707106781186547,0.707106781186547,0.707106781186547,
0.707106781186547,0.707106781186548,0.707106781186548,0.707106781186547,
0.707106781186547,0.707106781186547,0.707106781186548,0.707106781186547,
0.707106781186547,0.707106781186548,0.707106781186547,0.707106781186548,
0.707106781186548,0.707106781186548,0.707106781186547,0.707106781186547,
0.707106781186547,0.707106781186547,0.707106781186548,0.707106781186548,
0.707106781186547,0.707106781186548,0.707106781186547,0.707106781186548,
0.707106781186548,0.707106781186547,0.707106781186548,0.707106781186547,
0.707106781186548,0.707106781186547,0.707106781186547,0.707106781186547,
0.707106781186548,0.707106781186547,0.707106781186548,0.707106781186547,
0.707106781186548,0.707106781186547,0.707106781186548,0.707106781186547,
0.707106781186548,0.707106781186547,0.707106781186547,0.707106781186548,
0.707106781186547,0.707106781186548,0.707106781186547,0.707106781186547,
0.707106781186548,0.707106781186548,0.707106781186547,0.707106781186548,
0.707106781186548,0.707106781186547,0.707106781186548,0.707106781186547,
0.707106781186548,0.707106781186547,0.707106781186547,0.707106781186547,
0.707106781186548,0.707106781186547,0.707106781186547,0.707106781186548,
0.707106781186547,0.707106781186548,0.707106781186547,0.707106781186548,
0.707106781186548,0.707106781186547,0.707106781186548,0.707106781186547,
0.707106781186548,0.707106781186548,0.707106781186548,0.707106781186548,
0.707106781186547,0.707106781186547,0.707106781186548,0.707106781186547,
0.707106781186547,0.707106781186548,0.707106781186548,0.707106781186547,
0.707106781186547,0.707106781186548,0.707106781186547,0.707106781186547,
0.707106781186548,0.707106781186547,0.707106781186548,0.707106781186547,
0.707106781186548,0.707106781186547,0.707106781186547,0.707106781186547,
0.707106781186548,0.707106781186547,0.707106781186547,0.707106781186548,
0.707106781186547,0.707106781186548,0.707106781186548,0.707106781186548,
0.707106781186547,0.707106781186547,0.707106781186547,0.707106781186548,
0.707106781186548,0.707106781186547,0.707106781186547,0.707106781186547,
0.707106781186547,0.707106781186548,0.707106781186548,0.707106781186547,
0.707106781186547,0.707106781186547,0.707106781186548,0.707106781186548,
0.707106781186547,0.707106781186548,0.707106781186547,0.707106781186548,
0.707106781186547,0.707106781186548,0.707106781186548,0.707106781186547,
0.707106781186548,0.707106781186548,0.707106781186548,0.707106781186547,
0.707106781186547,0.707106781186547,0.707106781186548,0.707106781186548,
0.707106781186548,0.707106781186547,0.707106781186547,0.707106781186548,
0.707106781186548,0.707106781186547,0.707106781186548,0.707106781186547,
0.707106781186547,0.707106781186548,0.707106781186547,0.707106781186548,
0.707106781186547,0.707106781186547,0.707106781186548,0.707106781186547,
0.707106781186548,0.707106781186548,0.707106781186547,0.707106781186547,
0.707106781186548,0.707106781186547,0.707106781186548,0.707106781186547,
0.707106781186547,0.707106781186548,0.707106781186547,0.707106781186548,
0.707106781186547,0.707106781186548,0.707106781186547,0.707106781186547,
0.707106781186548,0.707106781186547,0.707106781186547,0.707106781186547,
0.707106781186547,0.707106781186547,0.707106781186547,0.707106781186548,
0.707106781186547,0.707106781186548,0.707106781186548,0.707106781186548,
0.707106781186547,0.707106781186547,0.707106781186547,0.707106781186548,
0.707106781186547,0.707106781186548,0.707106781186547,0.707106781186547,
0.707106781186548,0.707106781186547,0.707106781186547,0.707106781186547,
0.707106781186547,0.707106781186547,0.707106781186548,0.707106781186547,
0.707106781186548,0.707106781186547,0.707106781186547,0.707106781186548,
0.707106781186548,0.707106781186547,0.707106781186547,0.707106781186547,
0.707106781186548,0.707106781186547,0.707106781186547,0.707106781186548,
0.707106781186548,0.707106781186547,0.707106781186548,0.707106781186547,
0.707106781186548,0.707106781186548,0.707106781186547,0.707106781186547,
0.707106781186547,0.707106781186548,0.707106781186548,0.707106781186547,
0.707106781186548,0.707106781186547,0.707106781186548,0.707106781186548,
0.707106781186547,0.707106781186548,0.707106781186547,0.707106781186547,
0.707106781186547,0.707106781186548,0.707106781186547,0.707106781186548,
0.707106781186547,0.707106781186548,0.707106781186547,0.707106781186547,
0.707106781186547,0.707106781186547,0.707106781186547,0.707106781186548,
0.707106781186547,0.707106781186548,0.707106781186547,0.707106781186548,
0.707106781186547,0.707106781186548,0.707106781186547,0.707106781186547,
0.707106781186547,0.707106781186547,0.707106781186547,0.707106781186548,
0.707106781186548,0.707106781186548,0.707106781186547,0.707106781186548,
0.707106781186547,0.707106781186548,0.707106781186547,0.707106781186547,
0.707106781186548,0.707106781186547,0.707106781186548,0.707106781186547,
0.707106781186547,0.707106781186547,0.707106781186548,0.707106781186548,
0.707106781186547,0.707106781186548,0.707106781186547,0.707106781186548,
0.707106781186548,0.707106781186547,0.707106781186548,0.707106781186547,
0.707106781186548,0.707106781186548,0.707106781186547,0.707106781186547,
0.707106781186547,0.707106781186547,0.707106781186547,0.707106781186547,
0.707106781186548,0.707106781186548,0.707106781186547,0.707106781186548,
0.707106781186547,0.707106781186547,0.707106781186548,0.707106781186547,
0.707106781186547,0.707106781186548,0.707106781186547,0.707106781186547,
0.707106781186547,0.707106781186548,0.707106781186547,0.707106781186547,
0.707106781186548,0.707106781186547,0.707106781186548,0.707106781186548,
0.707106781186547,0.707106781186547,0.707106781186547,0.707106781186548,
0.707106781186547,0.707106781186547,0.707106781186548,0.707106781186548,
0.707106781186548,0.707106781186548,0.707106781186547,0.707106781186548,
0.707106781186548,0.707106781186547,0.707106781186547,0.707106781186548,
0.707106781186547,0.707106781186548,0.707106781186547,0.707106781186547,
0.707106781186548,0.707106781186547,0.707106781186547,0.707106781186548,
0.707106781186547,0.707106781186548,0.707106781186547,0.707106781186548,
0.707106781186547,0.707106781186548,0.707106781186547,0.707106781186548,
0.707106781186547,0.707106781186548,0.707106781186548,0.707106781186547,
0.707106781186547,0.707106781186548,0.707106781186548,0.707106781186547,
0.707106781186547,0.707106781186547,0.707106781186547,0.707106781186547,
0.707106781186548,0.707106781186547,0.707106781186547,0.707106781186548,
0.707106781186547,0.707106781186548,0.707106781186548,0.707106781186547,
0.707106781186548,0.707106781186547,0.707106781186548,0.707106781186547,
0.707106781186548,0.707106781186547,0.707106781186547,0.707106781186547,
0.707106781186547,0.707106781186547,0.707106781186547,0.707106781186548,
0.707106781186547,0.707106781186548,0.707106781186547,0.707106781186547,
0.707106781186547,0.707106781186548,0.707106781186547,0.707106781186548,
0.707106781186548,0.707106781186547,0.707106781186547,0.707106781186548,
0.707106781186547,0.707106781186548,0.707106781186547,0.707106781186548,
0.707106781186547,0.707106781186548,0.707106781186547,0.707106781186547,
0.707106781186548,0.707106781186547,0.707106781186548,0.707106781186547,
0.707106781186548,0.707106781186548,0.707106781186548,0.707106781186548,
0.707106781186547,0.707106781186548,0.707106781186548,0.707106781186548,
0.707106781186547,0.707106781186548,0.707106781186548,0.707106781186547,
0.707106781186548,0.707106781186547,0.707106781186548,0.707106781186547,
0.707106781186547,0.707106781186547,0.707106781186548,0.707106781186548,
0.707106781186547,0.707106781186548,0.707106781186547,0.707106781186548,
0.707106781186547,0.707106781186548,0.707106781186548,0.707106781186547,
0.707106781186548,0.707106781186547,0.707106781186547,0.707106781186548,
0.707106781186547,0.707106781186547,0.707106781186547,0.707106781186548,
0.707106781186547,0.707106781186548,0.707106781186548,0.707106781186547,
0.707106781186548,0.707106781186547,0.707106781186548,0.707106781186548,
0.707106781186548,0.707106781186548,0.707106781186547,0.707106781186548,
0.707106781186547,0.707106781186548,0.707106781186547,0.707106781186548,
0.707106781186547,0.707106781186547,0.707106781186547,0.707106781186547,
0.707106781186548,0.707106781186547,0.707106781186548,0.707106781186547,
0.707106781186547,0.707106781186548,0.707106781186547,0.707106781186548,
0.707106781186547,0.707106781186548,0.707106781186547,0.707106781186548,
0.707106781186548,0.707106781186548,0.707106781186548,0.707106781186547,
0.707106781186548,0.707106781186548,0.707106781186547,0.707106781186548,
0.707106781186547,0.707106781186548,0.707106781186547,0.707106781186548,
0.707106781186547,0.707106781186547,0.707106781186548,0.707106781186547,
0.707106781186548,0.707106781186547,0.707106781186547,0.707106781186548,
0.707106781186547,0.707106781186548,0.707106781186547,0.707106781186547,
0.707106781186548,0.707106781186548,0.707106781186548,0.707106781186548,
0.707106781186548,0.707106781186548,0.707106781186548,0.707106781186548,
0.707106781186548,0.707106781186547,0.707106781186548,0.707106781186547,
0.707106781186547,0.707106781186548,0.707106781186547,0.707106781186548,
0.707106781186548,0.707106781186547,0.707106781186547,0.707106781186548,
0.707106781186548,0.707106781186547,0.707106781186547,0.707106781186547,
0.707106781186547,0.707106781186547,0.707106781186548,0.707106781186547,
0.707106781186548,0.707106781186548,0.707106781186548,0.707106781186547,
0.707106781186548,0.707106781186547,0.707106781186548,0.707106781186547,
0.707106781186548,0.707106781186547,0.707106781186548,0.707106781186548,
0.707106781186547,0.707106781186547,0.707106781186548,0.707106781186548,
0.707106781186548,0.707106781186547,0.707106781186547,0.707106781186548,
0.707106781186547,0.707106781186547,0.707106781186548,0.707106781186547,
0.707106781186548,0.707106781186547,0.707106781186547,0.707106781186548,
0.707106781186548,0.707106781186548,0.707106781186547,0.707106781186547,
0.707106781186548,0.707106781186547,0.707106781186548,0.707106781186547,
0.707106781186548,0.707106781186547,0.707106781186548,0.707106781186548,
0.707106781186547,0.707106781186548,0.707106781186547,0.707106781186548,
0.707106781186547,0.707106781186547,0.707106781186547,0.707106781186548,
0.707106781186547,0.707106781186548,0.707106781186547,0.707106781186547,
0.707106781186547,0.707106781186548,0.707106781186547,0.707106781186547,
0.707106781186548,0.707106781186548,0.707106781186547,0.707106781186548,
0.707106781186547,0.707106781186548,0.707106781186548,0.707106781186547,
0.707106781186548,0.707106781186547,0.707106781186547,0.707106781186548,
0.707106781186547,0.707106781186547,0.707106781186547,0.707106781186548,
0.707106781186547,0.707106781186548,0.707106781186547,0.707106781186548,
0.707106781186548,0.707106781186548,0.707106781186547,0.707106781186548,
0.707106781186548,0.707106781186548,0.707106781186547,0.707106781186548,
0.707106781186547,0.707106781186547,0.707106781186548,0.707106781186547,
0.707106781186547,0.707106781186548,0.707106781186548,0.707106781186547,
0.707106781186548,0.707106781186547,0.707106781186548,0.707106781186548,
0.707106781186547,0.707106781186548,0.707106781186547,0.707106781186548,
0.707106781186547,0.707106781186548,0.707106781186547,0.707106781186548,
0.707106781186548,0.707106781186548,0.707106781186547,0.707106781186548,
0.707106781186548,0.707106781186547,0.707106781186547,0.707106781186548,
0.707106781186547,0.707106781186548,0.707106781186548,0.707106781186547,
0.707106781186548,0.707106781186548,0.707106781186547,0.707106781186548,
0.707106781186548,0.707106781186547,0.707106781186547,0.707106781186548,
0.707106781186547,0.707106781186548,0.707106781186547,0.707106781186548,
0.707106781186547,0.707106781186548,0.707106781186548,0.707106781186548,
0.707106781186547,0.707106781186548,0.707106781186547,0.707106781186548,
0.707106781186547,0.707106781186548,0.707106781186547,0.707106781186548,
0.707106781186547,0.707106781186548,0.707106781186547,0.707106781186548,
0.707106781186547,0.707106781186547,0.707106781186547,0.707106781186548,
0.707106781186547,0.707106781186548,0.707106781186547,0.707106781186548,
0.707106781186547,0.707106781186548,0.707106781186547,0.707106781186548,
0.707106781186548,0.707106781186548,0.707106781186547,0.707106781186548,
0.707106781186547,0.707106781186548,0.707106781186548,0.707106781186547,
0.707106781186548,0.707106781186547,0.707106781186548,0.707106781186547,
0.707106781186548,0.707106781186547,0.707106781186548,0.707106781186547,
0.707106781186547,0.707106781186547,0.707106781186548,0.707106781186547,
0.707106781186547,0.707106781186548,0.707106781186547,0.707106781186548,
0.707106781186547,0.707106781186547,0.707106781186548,0.707106781186547,
0.707106781186548,0.707106781186547,0.707106781186548,0.707106781186548,
0.707106781186548,0.707106781186547,0.707106781186547,0.707106781186548,
0.707106781186548,0.707106781186547,0.707106781186548,0.707106781186547,
0.707106781186547,0.707106781186547,0.707106781186548,0.707106781186547,
0.707106781186548,0.707106781186547,0.707106781186548,0.707106781186548,
0.707106781186548,0.707106781186547,0.707106781186547,0.707106781186547,
0.707106781186547,0.707106781186547,0.707106781186547,0.707106781186548,
0.707106781186547,0.707106781186548,0.707106781186547,0.707106781186548,
0.707106781186547,0.707106781186547,0.707106781186548,0.707106781186547,
0.707106781186547,0.707106781186548,0.707106781186548,0.707106781186547,
0.707106781186547,0.707106781186547,0.707106781186548,0.707106781186547,
0.707106781186547,0.707106781186548,0.707106781186548),(1.,1.,1.,1.,1.,
1.,1.,1.,1.,1.,1.,1.,1.,1.,1.,1.,1.,1.,1.,1.,1.,1.,1.,1.,1.,1.,1.,1.,1.,
1.,1.,1.,1.,1.,1.,1.,1.,1.,1.,1.,1.,1.,1.,1.,1.,1.,1.,1.,1.,1.,1.,1.,1.,
1.,1.,1.,1.,1.,1.,1.,1.,1.,1.,1.,1.,1.,1.,1.,1.,1.,1.,1.,1.,1.,1.,1.,1.,
1.,1.,1.,1.,1.,1.,1.,1.,1.,1.,1.,1.,1.,1.,1.,1.,1.,1.,1.,1.,1.,1.,1.,1.,
1.,1.,1.,1.,1.,1.,1.,1.,1.,1.,1.,1.,1.,1.,1.,1.,1.,1.,1.,1.,1.,1.,1.,1.,
1.,1.,1.,1.,1.,1.,1.,1.,1.,1.,1.,1.,1.,1.,1.,1.,1.,1.,1.,1.,1.,1.,1.,1.,
1.,1.,1.,1.,1.,1.,1.,1.,1.,1.,1.,1.,1.,1.,1.,1.,1.,1.,1.,1.,1.,1.,1.,1.,
1.,1.,1.,1.,1.,1.,1.,1.,1.,1.,1.,1.,1.,1.,1.,1.,1.,1.,1.,1.,1.,1.,1.,1.,
1.,1.,1.,1.,1.,1.,1.,1.,1.,1.,1.,1.,1.,1.,1.,1.,1.,1.,1.,1.,1.,1.,1.,1.,
1.,1.,1.,1.,1.,1.,1.,1.,1.,1.,1.,1.,1.,1.,1.,1.,1.,1.,1.,1.,1.,1.,1.,1.,
1.,1.,1.,1.,1.,1.,1.,1.,1.,1.,1.,1.,1.,1.,1.,1.,1.,1.,1.,1.,1.,1.,1.,1.,
1.,1.,1.,1.,1.,1.,1.,1.,1.,1.,1.,1.,1.,1.,1.,1.,1.,1.,1.,1.,1.,1.,1.,1.,
1.,1.,1.,1.,1.,1.,1.,1.,1.,1.,1.,1.,1.,1.,1.,1.,1.,1.,1.,1.,1.,1.,1.,1.,
1.,1.,1.,1.,1.,1.,1.,1.,1.,1.,1.,1.,1.,1.,1.,1.,1.,1.,1.,1.,1.,1.,1.,1.,
1.,1.,1.,1.,1.,1.,1.,1.,1.,1.,1.,1.,1.,1.,1.,1.,1.,1.,1.,1.,1.,1.,1.,1.,
1.,1.,1.,1.,1.,1.,1.,1.,1.,1.,1.,1.,1.,1.,1.,1.,1.,1.,1.,1.,1.,1.,1.,1.,
1.,1.,1.,1.,1.,1.,1.,1.,1.,1.,1.,1.,1.,1.,1.,1.,1.,1.,1.,1.,1.,1.,1.,1.,
1.,1.,1.,1.,1.,1.,1.,1.,1.,1.,1.,1.,1.,1.,1.,1.,1.,1.,1.,1.,1.,1.,1.,1.,
1.,1.,1.,1.,1.,1.,1.,1.,1.,1.,1.,1.,1.,1.,1.,1.,1.,1.,1.,1.,1.,1.,1.,1.,
1.,1.,1.,1.,1.,1.,1.,1.,1.,1.,1.,1.,1.,1.,1.,1.,1.,1.,1.,1.,1.,1.,1.,1.,
1.,1.,1.,1.,1.,1.,1.,1.,1.,1.,1.,1.,1.,1.,1.,1.,1.,1.,1.,1.,1.,1.,1.,1.,
1.,1.,1.,1.,1.,1.,1.,1.,1.,1.,1.,1.,1.,1.,1.,1.,1.,1.,1.,1.,1.,1.,1.,1.,
1.,1.,1.,1.,1.,1.,1.,1.,1.,1.,1.,1.,1.,1.,1.,1.,1.,1.,1.,1.,1.,1.,1.,1.,
1.,1.,1.,1.,1.,1.,1.,1.,1.,1.,1.,1.,1.,1.,1.,1.,1.,1.,1.,1.,1.,1.,1.,1.,
1.,1.,1.,1.,1.,1.,1.,1.,1.,1.,1.,1.,1.,1.,1.,1.,1.,1.,1.,1.,1.,1.,1.,1.,
1.,1.,1.,1.,1.,1.,1.,1.,1.,1.,1.,1.,1.,1.,1.,1.,1.,1.,1.,1.,1.,1.,1.,1.,
1.,1.,1.,1.,1.,1.,1.,1.,1.,1.,1.,1.,1.,1.,1.,1.,1.,1.,1.,1.,1.,1.,1.,1.,
1.,1.,1.,1.,1.,1.,1.,1.,1.,1.,1.,1.,1.,1.,1.,1.,1.,1.,1.,1.,1.,1.,1.,1.,
1.,1.,1.,1.,1.,1.,1.,1.,1.,1.,1.,1.,1.,1.,1.,1.,1.,1.,1.,1.,1.,1.,1.,1.,
1.,1.,1.,1.,1.,1.,1.,1.,1.,1.,1.,1.,1.,1.,1.,1.,1.,1.,1.,1.,1.,1.,1.,1.,
1.,1.,1.,1.,1.,1.,1.,1.,1.,1.,1.,1.,1.,1.,1.,1.,1.,1.,1.,1.,1.,1.,1.,1.,
1.,1.,1.,1.,1.,1.,1.,1.,1.,1.,1.,1.,1.,1.,1.,1.,1.,1.,1.,1.,1.,1.,1.,1.,
1.,1.,1.,1.,1.,1.,1.,1.,1.,1.,1.,1.,1.,1.,1.,1.,1.,1.,1.,1.,1.,1.,1.,1.,
1.,1.,1.,1.,1.,1.,1.,1.,1.,1.,1.,1.,1.,1.,1.,1.,1.,1.,1.,1.,1.,1.,1.,1.,
1.,1.,1.,1.,1.,1.,1.,1.,1.,1.,1.,1.,1.,1.,1.,1.,1.,1.,1.,1.,1.,1.,1.,1.,
1.,1.,1.,1.,1.,1.,1.,1.,1.,1.,1.,1.,1.,1.,1.,1.,1.,1.,1.,1.,1.,1.,1.,1.,
1.,1.,1.,1.,1.,1.,1.,1.,1.,1.,1.,1.,1.,1.,1.,1.,1.,1.,1.,1.,1.,1.,1.,1.,
1.,1.,1.,1.,1.,1.,1.,1.,1.,1.,1.,1.,1.,1.,1.,1.,1.,1.,1.,1.,1.,1.,1.,1.,
1.,1.,1.,1.,1.,1.,1.,1.,1.,1.,1.,1.,1.,1.,1.,1.,1.,1.,1.,1.,1.,1.,1.,1.,
1.,1.,1.,1.,1.,1.,1.,1.,1.,1.,1.,1.,1.,1.,1.,1.,1.,1.,1.,1.,1.,1.,1.,1.,
1.,1.,1.,1.,1.,1.,1.,1.,1.,1.,1.,1.,1.,1.,1.,1.,1.,1.,1.,1.,1.,1.,1.,1.,
1.,1.,1.,1.,1.,1.,1.,1.,1.,1.,1.,1.,1.,1.,1.,1.,1.,1.,1.,1.,1.,1.,1.,1.,
1.,1.,1.,1.,1.,1.,1.,1.,1.,1.,1.,1.,1.,1.,1.,1.,1.,1.,1.,1.,1.,1.,1.,1.,
1.,1.,1.,1.,1.,1.,1.,1.,1.,1.,1.,1.,1.,1.,1.,1.,1.,1.,1.,1.,1.,1.,1.,1.,
1.,1.,1.,1.,1.,1.,1.,1.,1.,1.,1.,1.,1.,1.,1.,1.,1.,1.,1.,1.,1.,1.,1.,1.,
1.,1.,1.,1.,1.,1.,1.,1.,1.,1.,1.,1.,1.,1.,1.,1.,1.,1.,1.,1.,1.,1.,1.,1.,
1.,1.,1.,1.,1.,1.,1.,1.,1.,1.,1.,1.,1.,1.,1.,1.,1.,1.,1.,1.,1.,1.,1.,1.,
1.,1.,1.,1.,1.,1.,1.,1.,1.,1.,1.,1.,1.,1.,1.,1.,1.,1.,1.,1.,1.,1.,1.,1.,
1.,1.,1.,1.,1.,1.,1.,1.,1.,1.,1.,1.,1.,1.,1.,1.,1.,1.,1.,1.,1.,1.,1.,1.,
1.,1.,1.,1.,1.,1.,1.,1.,1.,1.,1.,1.,1.,1.,1.,1.,1.,1.,1.,1.,1.,1.,1.,1.,
1.,1.,1.,1.,1.,1.,1.,1.,1.,1.,1.,1.,1.,1.,1.,1.,1.,1.,1.,1.,1.,1.,1.,1.,
1.,1.,1.,1.,1.,1.,1.,1.,1.,1.,1.,1.,1.,1.,1.,1.,1.,1.,1.,1.,1.,1.,1.,1.,
1.,1.,1.,1.,1.,1.,1.,1.,1.,1.,1.,1.,1.,1.,1.,1.,1.,1.,1.,1.,1.,1.,1.,1.,
1.,1.,1.,1.,1.,1.,1.,1.,1.,1.,1.,1.,1.,1.,1.,1.,1.,1.,1.,1.,1.,1.,1.,1.,
1.,1.,1.,1.,1.,1.,1.,1.,1.,1.,1.,1.,1.,1.,1.,1.,1.,1.,1.,1.,1.,1.,1.,1.,
1.,1.,1.,1.,1.,1.,1.,1.,1.,1.,1.,1.,1.,1.,1.,1.,1.,1.,1.,1.,1.,1.,1.,1.,
1.,1.,1.,1.,1.,1.,1.,1.,1.,1.,1.,1.,1.,1.,1.,1.,1.,1.,1.,1.,1.,1.,1.,1.,
1.,1.,1.,1.,1.,1.,1.,1.,1.,1.,1.,1.,1.,1.,1.,1.,1.,1.,1.,1.,1.,1.,1.,1.,
1.,1.,1.,1.,1.,1.,1.,1.,1.,1.,1.,1.,1.,1.,1.,1.,1.,1.,1.,1.,1.,1.,1.,1.,
1.,1.,1.,1.,1.,1.,1.,1.,1.,1.,1.,1.,1.,1.,1.,1.,1.,1.,1.,1.,1.,1.,1.,1.,
1.,1.,1.,1.,1.,1.,1.,1.,1.,1.,1.,1.,1.,1.,1.,1.,1.,1.,1.,1.,1.,1.,1.,1.,
1.,1.,1.,1.,1.,1.,1.,1.,1.,1.,1.,1.,1.,1.,1.,1.,1.,1.,1.,1.,1.,1.,1.,1.,
1.,1.,1.,1.,1.,1.,1.,1.,1.,1.,1.,1.,1.,1.,1.,1.,1.,1.,1.,1.,1.,1.,1.,1.,
1.,1.,1.,1.,1.,1.,1.,1.,1.,1.,1.,1.,1.,1.,1.,1.,1.,1.,1.,1.,1.,1.,1.,1.,
1.,1.,1.,1.,1.,1.,1.,1.,1.,1.,1.,1.,1.,1.,1.,1.,1.,1.,1.,1.,1.,1.,1.,1.,
1.,1.,1.,1.,1.,1.,1.,1.,1.,1.,1.,1.,1.,1.,1.,1.,1.,1.,1.,1.,1.,1.,1.,1.,
1.,1.,1.,1.,1.,1.,1.,1.,1.,1.,1.,1.,1.,1.,1.,1.,1.,1.,1.,1.,1.,1.,1.,1.,
1.,1.,1.,1.,1.,1.,1.,1.,1.,1.,1.,1.,1.,1.,1.,1.,1.,1.,1.,1.,1.,1.,1.,1.,
1.,1.,1.,1.,1.,1.,1.,1.,1.,1.,1.,1.,1.,1.,1.,1.,1.,1.,1.,1.,1.,1.,1.,1.,
1.,1.,1.,1.,1.,1.,1.,1.,1.,1.,1.,1.,1.,1.,1.,1.,1.,1.,1.,1.,1.,1.,1.,1.,
1.,1.,1.,1.,1.,1.,1.,1.,1.,1.,1.,1.,1.,1.,1.,1.,1.,1.,1.,1.,1.,1.,1.,1.,
1.,1.,1.,1.,1.,1.,1.,1.,1.,1.,1.,1.,1.,1.,1.,1.,1.,1.,1.,1.,1.,1.,1.,1.,
1.,1.,1.,1.,1.,1.,1.,1.,1.,1.,1.,1.,1.,1.,1.,1.,1.,1.,1.,1.,1.,1.,1.,1.,
1.,1.,1.,1.,1.,1.,1.,1.,1.,1.,1.,1.,1.,1.,1.,1.,1.,1.,1.,1.,1.,1.,1.,1.,
1.,1.,1.,1.,1.,1.,1.,1.,1.,1.,1.,1.,1.,1.,1.,1.,1.,1.,1.,1.,1.,1.,1.,1.,
1.,1.,1.,1.,1.,1.,1.,1.,1.,1.,1.,1.,1.,1.,1.,1.,1.,1.,1.,1.,1.,1.,1.,1.,
1.,1.,1.,1.,1.,1.,1.,1.,1.,1.,1.,1.,1.,1.,1.,1.,1.,1.,1.,1.,1.,1.,1.,1.,
1.,1.,1.,1.,1.,1.,1.,1.,1.,1.,1.,1.,1.,1.,1.,1.,1.,1.,1.,1.,1.,1.,1.,1.,
1.,1.,1.,1.,1.,1.,1.,1.,1.,1.,1.,1.,1.,1.,1.,1.,1.,1.,1.,1.,1.,1.,1.,1.,
1.,1.,1.,1.,1.,1.,1.,1.,1.,1.,1.,1.,1.,1.,1.,1.,1.,1.,1.,1.,1.,1.,1.,1.,
1.,1.,1.,1.,1.,1.,1.,1.,1.,1.,1.,1.,1.,1.,1.,1.,1.,1.,1.,1.,1.,1.,1.,1.,
1.,1.,1.,1.,1.,1.,1.,1.,1.,1.,1.,1.,1.,1.,1.,1.,1.,1.,1.,1.,1.,1.,1.,1.,
1.,1.,1.,1.,1.,1.,1.,1.,1.,1.,1.,1.,1.,1.,1.,1.,1.,1.,1.,1.,1.,1.,1.,1.,
1.,1.,1.,1.,1.,1.,1.,1.,1.,1.,1.,1.,1.,1.,1.,1.,1.,1.,1.,1.,1.,1.,1.,1.,
1.,1.,1.,1.,1.,1.,1.,1.,1.,1.,1.,1.,1.,1.,1.,1.,1.,1.,1.,1.,1.,1.,1.,1.,
1.,1.,1.,1.,1.,1.),(0.707106781186548,0.707106781186548,0.707106781186548,
0.707106781186547,0.707106781186547,0.707106781186548,0.707106781186547,
0.707106781186547,0.707106781186547,0.707106781186547,0.707106781186547,
0.707106781186548,0.707106781186548,0.707106781186548,0.707106781186547,
0.707106781186548,0.707106781186547,0.707106781186547,0.707106781186548,
0.707106781186547,0.707106781186548,0.707106781186547,0.707106781186548,
0.707106781186547,0.707106781186548,0.707106781186547,0.707106781186547,
0.707106781186547,0.707106781186547,0.707106781186547,0.707106781186548,
0.707106781186547,0.707106781186547,0.707106781186548,0.707106781186547,
0.707106781186547,0.707106781186548,0.707106781186547,0.707106781186547,
0.707106781186548,0.707106781186548,0.707106781186547,0.707106781186548,
0.707106781186547,0.707106781186547,0.707106781186547,0.707106781186548,
0.707106781186548,0.707106781186547,0.707106781186547,0.707106781186548,
0.707106781186547,0.707106781186548,0.707106781186547,0.707106781186547,
0.707106781186547,0.707106781186547,0.707106781186547,0.707106781186548,
0.707106781186547,0.707106781186548,0.707106781186547,0.707106781186548,
0.707106781186547,0.707106781186548,0.707106781186547,0.707106781186547,
0.707106781186548,0.707106781186547,0.707106781186547,0.707106781186548,
0.707106781186547,0.707106781186548,0.707106781186547,0.707106781186548,
0.707106781186548,0.707106781186547,0.707106781186548,0.707106781186547,
0.707106781186547,0.707106781186548,0.707106781186547,0.707106781186547,
0.707106781186547,0.707106781186548,0.707106781186547,0.707106781186547,
0.707106781186547,0.707106781186547,0.707106781186547,0.707106781186547,
0.707106781186548,0.707106781186548,0.707106781186547,0.707106781186548,
0.707106781186547,0.707106781186548,0.707106781186548,0.707106781186547,
0.707106781186548,0.707106781186548,0.707106781186548,0.707106781186547,
0.707106781186548,0.707106781186547,0.707106781186548,0.707106781186548,
0.707106781186548,0.707106781186547,0.707106781186547,0.707106781186547,
0.707106781186548,0.707106781186548,0.707106781186548,0.707106781186547,
0.707106781186547,0.707106781186547,0.707106781186548,0.707106781186548,
0.707106781186547,0.707106781186547,0.707106781186548,0.707106781186547,
0.707106781186547,0.707106781186547,0.707106781186547,0.707106781186548,
0.707106781186547,0.707106781186548,0.707106781186547,0.707106781186547,
0.707106781186547,0.707106781186548,0.707106781186548,0.707106781186547,
0.707106781186548,0.707106781186548,0.707106781186547,0.707106781186548,
0.707106781186547,0.707106781186548,0.707106781186547,0.707106781186548,
0.707106781186547,0.707106781186547,0.707106781186548,0.707106781186547,
0.707106781186547,0.707106781186548,0.707106781186547,0.707106781186547,
0.707106781186548,0.707106781186547,0.707106781186548,0.707106781186547,
0.707106781186547,0.707106781186548,0.707106781186548,0.707106781186547,
0.707106781186548,0.707106781186547,0.707106781186548,0.707106781186547,
0.707106781186548,0.707106781186547,0.707106781186548,0.707106781186547,
0.707106781186548,0.707106781186547,0.707106781186548,0.707106781186547,
0.707106781186548,0.707106781186547,0.707106781186547,0.707106781186548,
0.707106781186547,0.707106781186548,0.707106781186547,0.707106781186548,
0.707106781186547,0.707106781186548,0.707106781186547,0.707106781186547,
0.707106781186548,0.707106781186547,0.707106781186548,0.707106781186548,
0.707106781186548,0.707106781186547,0.707106781186547,0.707106781186547,
0.707106781186547,0.707106781186548,0.707106781186547,0.707106781186548,
0.707106781186548,0.707106781186547,0.707106781186547,0.707106781186548,
0.707106781186548,0.707106781186547,0.707106781186547,0.707106781186548,
0.707106781186547,0.707106781186548,0.707106781186547,0.707106781186547,
0.707106781186547,0.707106781186547,0.707106781186547,0.707106781186547,
0.707106781186547,0.707106781186548,0.707106781186547,0.707106781186548,
0.707106781186547,0.707106781186548,0.707106781186548,0.707106781186547,
0.707106781186548,0.707106781186548,0.707106781186548,0.707106781186548,
0.707106781186547,0.707106781186548,0.707106781186547,0.707106781186548,
0.707106781186547,0.707106781186547,0.707106781186548,0.707106781186548,
0.707106781186547,0.707106781186547,0.707106781186547,0.707106781186547,
0.707106781186547,0.707106781186548,0.707106781186548,0.707106781186547,
0.707106781186547,0.707106781186548,0.707106781186548,0.707106781186547,
0.707106781186548,0.707106781186547,0.707106781186548,0.707106781186548,
0.707106781186547,0.707106781186547,0.707106781186548,0.707106781186547,
0.707106781186547,0.707106781186548,0.707106781186547,0.707106781186548,
0.707106781186547,0.707106781186548,0.707106781186547,0.707106781186547,
0.707106781186548,0.707106781186548,0.707106781186547,0.707106781186547,
0.707106781186548,0.707106781186547,0.707106781186547,0.707106781186548,
0.707106781186547,0.707106781186548,0.707106781186547,0.707106781186548,
0.707106781186547,0.707106781186548,0.707106781186547,0.707106781186547,
0.707106781186547,0.707106781186547,0.707106781186547,0.707106781186547,
0.707106781186548,0.707106781186547,0.707106781186548,0.707106781186547,
0.707106781186548,0.707106781186548,0.707106781186547,0.707106781186548,
0.707106781186548,0.707106781186547,0.707106781186548,0.707106781186547,
0.707106781186547,0.707106781186547,0.707106781186548,0.707106781186547,
0.707106781186547,0.707106781186548,0.707106781186547,0.707106781186548,
0.707106781186547,0.707106781186547,0.707106781186547,0.707106781186548,
0.707106781186548,0.707106781186547,0.707106781186548,0.707106781186548,
0.707106781186547,0.707106781186548,0.707106781186547,0.707106781186548,
0.707106781186548,0.707106781186547,0.707106781186548,0.707106781186548,
0.707106781186548,0.707106781186547,0.707106781186547,0.707106781186548,
0.707106781186547,0.707106781186548,0.707106781186547,0.707106781186547,
0.707106781186548,0.707106781186548,0.707106781186548,0.707106781186547,
0.707106781186547,0.707106781186548,0.707106781186548,0.707106781186547,
0.707106781186547,0.707106781186548,0.707106781186547,0.707106781186547,
0.707106781186548,0.707106781186548,0.707106781186547,0.707106781186547,
0.707106781186547,0.707106781186548,0.707106781186547,0.707106781186547,
0.707106781186547,0.707106781186548,0.707106781186548,0.707106781186547,
0.707106781186548,0.707106781186547,0.707106781186548,0.707106781186547,
0.707106781186548,0.707106781186548,0.707106781186547,0.707106781186547,
0.707106781186548,0.707106781186547,0.707106781186547,0.707106781186548,
0.707106781186547,0.707106781186548,0.707106781186548,0.707106781186547,
0.707106781186548,0.707106781186547,0.707106781186547,0.707106781186547,
0.707106781186548,0.707106781186548,0.707106781186548,0.707106781186547,
0.707106781186548,0.707106781186547,0.707106781186548,0.707106781186547,
0.707106781186547,0.707106781186547,0.707106781186547,0.707106781186548,
0.707106781186548,0.707106781186547,0.707106781186547,0.707106781186548,
0.707106781186547,0.707106781186548,0.707106781186547,0.707106781186548,
0.707106781186547,0.707106781186547,0.707106781186548,0.707106781186547,
0.707106781186548,0.707106781186547,0.707106781186548,0.707106781186548,
0.707106781186547,0.707106781186548,0.707106781186547,0.707106781186548,
0.707106781186548,0.707106781186547,0.707106781186548,0.707106781186547,
0.707106781186547,0.707106781186548,0.707106781186547,0.707106781186548,
0.707106781186547,0.707106781186548,0.707106781186547,0.707106781186547,
0.707106781186548,0.707106781186548,0.707106781186548,0.707106781186548,
0.707106781186547,0.707106781186548,0.707106781186548,0.707106781186548,
0.707106781186547,0.707106781186548,0.707106781186548,0.707106781186548,
0.707106781186547,0.707106781186547,0.707106781186548,0.707106781186547,
0.707106781186548,0.707106781186547,0.707106781186548,0.707106781186548,
0.707106781186547,0.707106781186547,0.707106781186548,0.707106781186547,
0.707106781186548,0.707106781186547,0.707106781186548,0.707106781186548,
0.707106781186547,0.707106781186547,0.707106781186547,0.707106781186548,
0.707106781186548,0.707106781186547,0.707106781186547,0.707106781186548,
0.707106781186548,0.707106781186548,0.707106781186548,0.707106781186547,
0.707106781186547,0.707106781186548,0.707106781186548,0.707106781186547,
0.707106781186548,0.707106781186547,0.707106781186548,0.707106781186547,
0.707106781186548,0.707106781186547,0.707106781186547,0.707106781186548,
0.707106781186547,0.707106781186547,0.707106781186548,0.707106781186547,
0.707106781186548,0.707106781186547,0.707106781186548,0.707106781186547,
0.707106781186548,0.707106781186547,0.707106781186548,0.707106781186547,
0.707106781186548,0.707106781186547,0.707106781186547,0.707106781186548,
0.707106781186548,0.707106781186547,0.707106781186547,0.707106781186547,
0.707106781186548,0.707106781186547,0.707106781186548,0.707106781186547,
0.707106781186548,0.707106781186547,0.707106781186548,0.707106781186547,
0.707106781186547,0.707106781186547,0.707106781186548,0.707106781186547,
0.707106781186548,0.707106781186548,0.707106781186547,0.707106781186548,
0.707106781186547,0.707106781186547,0.707106781186548,0.707106781186547,
0.707106781186547,0.707106781186548,0.707106781186547,0.707106781186547,
0.707106781186547,0.707106781186547,0.707106781186548,0.707106781186547,
0.707106781186547,0.707106781186547,0.707106781186548,0.707106781186547,
0.707106781186547,0.707106781186548,0.707106781186548,0.707106781186547,
0.707106781186548,0.707106781186548,0.707106781186547,0.707106781186547,
0.707106781186548,0.707106781186547,0.707106781186547,0.707106781186548,
0.707106781186547,0.707106781186547,0.707106781186547,0.707106781186548,
0.707106781186547,0.707106781186548,0.707106781186547,0.707106781186548,
0.707106781186547,0.707106781186548,0.707106781186547,0.707106781186548,
0.707106781186547,0.707106781186548,0.707106781186548,0.707106781186547,
0.707106781186547,0.707106781186548,0.707106781186547,0.707106781186548,
0.707106781186547,0.707106781186548,0.707106781186548,0.707106781186547,
0.707106781186548,0.707106781186547,0.707106781186548,0.707106781186548,
0.707106781186547,0.707106781186547,0.707106781186548,0.707106781186547,
0.707106781186548,0.707106781186547,0.707106781186548,0.707106781186547,
0.707106781186548,0.707106781186547,0.707106781186547,0.707106781186547,
0.707106781186547,0.707106781186547,0.707106781186547,0.707106781186547,
0.707106781186547,0.707106781186548,0.707106781186547,0.707106781186548,
0.707106781186547,0.707106781186547,0.707106781186548,0.707106781186547,
0.707106781186548,0.707106781186547,0.707106781186547,0.707106781186548,
0.707106781186547,0.707106781186548,0.707106781186547,0.707106781186548,
0.707106781186547,0.707106781186548,0.707106781186547,0.707106781186548,
0.707106781186547,0.707106781186548,0.707106781186547,0.707106781186548,
0.707106781186548,0.707106781186547,0.707106781186548,0.707106781186547,
0.707106781186547,0.707106781186547,0.707106781186548,0.707106781186547,
0.707106781186547,0.707106781186547,0.707106781186548,0.707106781186547,
0.707106781186547,0.707106781186548,0.707106781186547,0.707106781186547,
0.707106781186547,0.707106781186547,0.707106781186548,0.707106781186547,
0.707106781186547,0.707106781186547,0.707106781186548,0.707106781186548,
0.707106781186548,0.707106781186548,0.707106781186547,0.707106781186548,
0.707106781186547,0.707106781186547,0.707106781186548,0.707106781186547,
0.707106781186548,0.707106781186547,0.707106781186547,0.707106781186548,
0.707106781186547,0.707106781186547,0.707106781186547,0.707106781186547,
0.707106781186548,0.707106781186548,0.707106781186547,0.707106781186547,
0.707106781186548,0.707106781186547,0.707106781186548,0.707106781186547,
0.707106781186548,0.707106781186548,0.707106781186547,0.707106781186547,
0.707106781186548,0.707106781186548,0.707106781186547,0.707106781186548,
0.707106781186548,0.707106781186547,0.707106781186548,0.707106781186548,
0.707106781186548,0.707106781186547,0.707106781186548,0.707106781186547,
0.707106781186548,0.707106781186547,0.707106781186548,0.707106781186547,
0.707106781186548,0.707106781186547,0.707106781186548,0.707106781186548,
0.707106781186547,0.707106781186547,0.707106781186548,0.707106781186547,
0.707106781186548,0.707106781186547,0.707106781186548,0.707106781186548,
0.707106781186548,0.707106781186548,0.707106781186548,0.707106781186547,
0.707106781186547,0.707106781186547,0.707106781186547,0.707106781186548,
0.707106781186547,0.707106781186548,0.707106781186547,0.707106781186547,
0.707106781186548,0.707106781186548,0.707106781186547,0.707106781186548,
0.707106781186547,0.707106781186548,0.707106781186548,0.707106781186547,
0.707106781186547,0.707106781186548,0.707106781186547,0.707106781186548,
0.707106781186547,0.707106781186548,0.707106781186547,0.707106781186548,
0.707106781186547,0.707106781186548,0.707106781186547,0.707106781186548,
0.707106781186547,0.707106781186548,0.707106781186548,0.707106781186547,
0.707106781186548,0.707106781186547,0.707106781186548,0.707106781186547,
0.707106781186548,0.707106781186548,0.707106781186548,0.707106781186547,
0.707106781186547,0.707106781186548,0.707106781186548,0.707106781186547,
0.707106781186547,0.707106781186547,0.707106781186548,0.707106781186547,
0.707106781186548,0.707106781186547,0.707106781186548,0.707106781186547,
0.707106781186547,0.707106781186547,0.707106781186548,0.707106781186547,
0.707106781186548,0.707106781186547,0.707106781186548,0.707106781186547,
0.707106781186548,0.707106781186547,0.707106781186547,0.707106781186548,
0.707106781186547,0.707106781186547,0.707106781186548,0.707106781186547,
0.707106781186547,0.707106781186548,0.707106781186547,0.707106781186547,
0.707106781186547,0.707106781186548,0.707106781186547,0.707106781186548,
0.707106781186547,0.707106781186547,0.707106781186547,0.707106781186548,
0.707106781186548,0.707106781186547,0.707106781186547,0.707106781186548,
0.707106781186548,0.707106781186548,0.707106781186547,0.707106781186548,
0.707106781186547,0.707106781186548,0.707106781186547,0.707106781186548,
0.707106781186547,0.707106781186547,0.707106781186547,0.707106781186547,
0.707106781186548,0.707106781186547,0.707106781186548,0.707106781186548,
0.707106781186547,0.707106781186548,0.707106781186547,0.707106781186547,
0.707106781186547,0.707106781186547,0.707106781186548,0.707106781186547,
0.707106781186548,0.707106781186547,0.707106781186548,0.707106781186548,
0.707106781186547,0.707106781186548,0.707106781186547,0.707106781186547,
0.707106781186547,0.707106781186547,0.707106781186548,0.707106781186547,
0.707106781186548,0.707106781186548,0.707106781186547,0.707106781186548,
0.707106781186547,0.707106781186548,0.707106781186547,0.707106781186547,
0.707106781186548,0.707106781186547,0.707106781186548,0.707106781186548,
0.707106781186547,0.707106781186547,0.707106781186548,0.707106781186548,
0.707106781186547,0.707106781186547,0.707106781186548,0.707106781186547,
0.707106781186547,0.707106781186548,0.707106781186547,0.707106781186547,
0.707106781186548,0.707106781186547,0.707106781186548,0.707106781186547,
0.707106781186547,0.707106781186548,0.707106781186547,0.707106781186548,
0.707106781186547,0.707106781186548,0.707106781186547,0.707106781186547,
0.707106781186547,0.707106781186548,0.707106781186547,0.707106781186548,
0.707106781186547,0.707106781186548,0.707106781186548,0.707106781186548,
0.707106781186548,0.707106781186547,0.707106781186547,0.707106781186547,
0.707106781186548,0.707106781186547,0.707106781186548,0.707106781186547,
0.707106781186547,0.707106781186548,0.707106781186547,0.707106781186547,
0.707106781186548,0.707106781186547,0.707106781186547,0.707106781186548,
0.707106781186548,0.707106781186547,0.707106781186548,0.707106781186547,
0.707106781186547,0.707106781186548,0.707106781186547,0.707106781186548,
0.707106781186547,0.707106781186548,0.707106781186547,0.707106781186547,
0.707106781186547,0.707106781186548,0.707106781186547,0.707106781186548,
0.707106781186547,0.707106781186548,0.707106781186547,0.707106781186547,
0.707106781186548,0.707106781186548,0.707106781186548,0.707106781186547,
0.707106781186548,0.707106781186547,0.707106781186548,0.707106781186547,
0.707106781186548,0.707106781186547,0.707106781186548,0.707106781186548,
0.707106781186547,0.707106781186547,0.707106781186547,0.707106781186548,
0.707106781186547,0.707106781186547,0.707106781186548,0.707106781186547,
0.707106781186547,0.707106781186548,0.707106781186547,0.707106781186548,
0.707106781186548,0.707106781186548,0.707106781186547,0.707106781186548,
0.707106781186547,0.707106781186548,0.707106781186547,0.707106781186548,
0.707106781186547,0.707106781186548,0.707106781186547,0.707106781186548,
0.707106781186547,0.707106781186548,0.707106781186548,0.707106781186547,
0.707106781186548,0.707106781186547,0.707106781186548,0.707106781186548,
0.707106781186547,0.707106781186547,0.707106781186548,0.707106781186547,
0.707106781186547,0.707106781186548,0.707106781186547,0.707106781186548,
0.707106781186548,0.707106781186547,0.707106781186548,0.707106781186548,
0.707106781186548,0.707106781186548,0.707106781186548,0.707106781186547,
0.707106781186548,0.707106781186548,0.707106781186548,0.707106781186547,
0.707106781186548,0.707106781186547,0.707106781186548,0.707106781186547,
0.707106781186548,0.707106781186547,0.707106781186548,0.707106781186547,
0.707106781186548,0.707106781186547,0.707106781186547,0.707106781186548,
0.707106781186547,0.707106781186547,0.707106781186548,0.707106781186547,
0.707106781186548,0.707106781186547,0.707106781186548,0.707106781186547,
0.707106781186548,0.707106781186547,0.707106781186547,0.707106781186548,
0.707106781186547,0.707106781186547,0.707106781186548,0.707106781186547,
0.707106781186548,0.707106781186547,0.707106781186547,0.707106781186548,
0.707106781186548,0.707106781186547,0.707106781186548,0.707106781186547,
0.707106781186547,0.707106781186547,0.707106781186548,0.707106781186547,
0.707106781186547,0.707106781186548,0.707106781186547,0.707106781186547,
0.707106781186547,0.707106781186548,0.707106781186548,0.707106781186547,
0.707106781186548,0.707106781186547,0.707106781186548,0.707106781186547,
0.707106781186547,0.707106781186548,0.707106781186547,0.707106781186548,
0.707106781186547,0.707106781186547,0.707106781186547,0.707106781186547,
0.707106781186548,0.707106781186547,0.707106781186547,0.707106781186547,
0.707106781186547,0.707106781186547,0.707106781186548,0.707106781186547,
0.707106781186547,0.707106781186547,0.707106781186547,0.707106781186548,
0.707106781186547,0.707106781186548,0.707106781186547,0.707106781186547,
0.707106781186548,0.707106781186547,0.707106781186548,0.707106781186547,
0.707106781186547,0.707106781186548,0.707106781186547,0.707106781186547,
0.707106781186548,0.707106781186547,0.707106781186547,0.707106781186547,
0.707106781186547,0.707106781186548,0.707106781186547,0.707106781186548,
0.707106781186548,0.707106781186547,0.707106781186548,0.707106781186548,
0.707106781186547,0.707106781186547,0.707106781186548,0.707106781186547,
0.707106781186547,0.707106781186547,0.707106781186548,0.707106781186547,
0.707106781186547,0.707106781186548,0.707106781186547,0.707106781186548,
0.707106781186547,0.707106781186548,0.707106781186547,0.707106781186547,
0.707106781186548,0.707106781186547,0.707106781186548,0.707106781186547,
0.707106781186548,0.707106781186547,0.707106781186548,0.707106781186547,
0.707106781186548,0.707106781186547,0.707106781186547,0.707106781186547,
0.707106781186547,0.707106781186548,0.707106781186548,0.707106781186547,
0.707106781186548,0.707106781186548,0.707106781186547,0.707106781186548,
0.707106781186547,0.707106781186547,0.707106781186548,0.707106781186547,
0.707106781186547,0.707106781186547,0.707106781186547,0.707106781186548,
0.707106781186547,0.707106781186547,0.707106781186547,0.707106781186548,
0.707106781186547,0.707106781186547,0.707106781186548,0.707106781186547,
0.707106781186548,0.707106781186548,0.707106781186547,0.707106781186548,
0.707106781186547,0.707106781186548,0.707106781186547,0.707106781186548,
0.707106781186547,0.707106781186547,0.707106781186548,0.707106781186547,
0.707106781186548,0.707106781186548,0.707106781186547,0.707106781186547,
0.707106781186548,0.707106781186547,0.707106781186548,0.707106781186547,
0.707106781186548,0.707106781186547,0.707106781186547,0.707106781186548,
0.707106781186548,0.707106781186547,0.707106781186548,0.707106781186548,
0.707106781186547,0.707106781186548,0.707106781186548,0.707106781186547,
0.707106781186548,0.707106781186547,0.707106781186548,0.707106781186547,
0.707106781186548,0.707106781186547,0.707106781186548,0.707106781186547,
0.707106781186547,0.707106781186548,0.707106781186547,0.707106781186547,
0.707106781186548,0.707106781186547,0.707106781186548,0.707106781186548,
0.707106781186547,0.707106781186547,0.707106781186547,0.707106781186548,
0.707106781186547,0.707106781186548,0.707106781186548,0.707106781186547,
0.707106781186548,0.707106781186547,0.707106781186548,0.707106781186547,
0.707106781186548,0.707106781186547,0.707106781186547,0.707106781186548,
0.707106781186548,0.707106781186548,0.707106781186547,0.707106781186548,
0.707106781186548,0.707106781186547,0.707106781186548,0.707106781186547,
0.707106781186548,0.707106781186548,0.707106781186548,0.707106781186548,
0.707106781186548,0.707106781186548,0.707106781186547,0.707106781186547,
0.707106781186548,0.707106781186547,0.707106781186547,0.707106781186548,
0.707106781186547,0.707106781186547,0.707106781186548,0.707106781186547,
0.707106781186548,0.707106781186547,0.707106781186548,0.707106781186547,
0.707106781186547,0.707106781186547,0.707106781186548,0.707106781186547,
0.707106781186547,0.707106781186548,0.707106781186547,0.707106781186548,
0.707106781186547,0.707106781186548,0.707106781186547,0.707106781186547,
0.707106781186547,0.707106781186547,0.707106781186548,0.707106781186547,
0.707106781186547,0.707106781186548,0.707106781186548,0.707106781186547,
0.707106781186548,0.707106781186547,0.707106781186548,0.707106781186547,
0.707106781186547,0.707106781186548,0.707106781186547,0.707106781186548,
0.707106781186547,0.707106781186548,0.707106781186547,0.707106781186548,
0.707106781186548,0.707106781186547,0.707106781186548,0.707106781186547,
0.707106781186547,0.707106781186548,0.707106781186547,0.707106781186547,
0.707106781186548,0.707106781186548,0.707106781186548,0.707106781186547,
0.707106781186548,0.707106781186547,0.707106781186547,0.707106781186547,
0.707106781186548,0.707106781186547,0.707106781186548,0.707106781186548,
0.707106781186548,0.707106781186547,0.707106781186547,0.707106781186547,
0.707106781186547,0.707106781186548,0.707106781186547,0.707106781186547,
0.707106781186548,0.707106781186547,0.707106781186548,0.707106781186547,
0.707106781186547,0.707106781186548,0.707106781186547,0.707106781186548,
0.707106781186547,0.707106781186548,0.707106781186547,0.707106781186547,
0.707106781186547,0.707106781186547,0.707106781186547,0.707106781186547,
0.707106781186548,0.707106781186547,0.707106781186547,0.707106781186548,
0.707106781186548,0.707106781186547,0.707106781186548,0.707106781186548,
0.707106781186547,0.707106781186547,0.707106781186548,0.707106781186547,
0.707106781186547,0.707106781186548,0.707106781186547,0.707106781186548,
0.707106781186548,0.707106781186548,0.707106781186547,0.707106781186547,
0.707106781186547,0.707106781186547,0.707106781186548,0.707106781186548,
0.707106781186548,0.707106781186547,0.707106781186548,0.707106781186547,
0.707106781186548,0.707106781186548,0.707106781186547,0.707106781186548,
0.707106781186547,0.707106781186548,0.707106781186548,0.707106781186547,
0.707106781186547,0.707106781186548,0.707106781186547,0.707106781186548,
0.707106781186547,0.707106781186548,0.707106781186548,0.707106781186548,
0.707106781186547,0.707106781186548,0.707106781186547,0.707106781186547,
0.707106781186547,0.707106781186547,0.707106781186548,0.707106781186548,
0.707106781186547,0.707106781186547,0.707106781186547,0.707106781186548,
0.707106781186547,0.707106781186547,0.707106781186548,0.707106781186547,
0.707106781186548,0.707106781186548,0.707106781186548,0.707106781186547,
0.707106781186547,0.707106781186547,0.707106781186547,0.707106781186548,
0.707106781186548,0.707106781186547,0.707106781186548,0.707106781186547,
0.707106781186548,0.707106781186548,0.707106781186547,0.707106781186548,
0.707106781186547,0.707106781186548,0.707106781186547,0.707106781186547,
0.707106781186547,0.707106781186548,0.707106781186547,0.707106781186548,
0.707106781186547,0.707106781186548,0.707106781186547,0.707106781186548,
0.707106781186547,0.707106781186548,0.707106781186547,0.707106781186547,
0.707106781186548,0.707106781186547,0.707106781186548,0.707106781186547,
0.707106781186547,0.707106781186548,0.707106781186548,0.707106781186547,
0.707106781186548,0.707106781186548,0.707106781186547,0.707106781186548,
0.707106781186547,0.707106781186548,0.707106781186547,0.707106781186547,
0.707106781186547,0.707106781186548,0.707106781186547,0.707106781186547,
0.707106781186548,0.707106781186547,0.707106781186548,0.707106781186547,
0.707106781186548,0.707106781186548,0.707106781186547,0.707106781186548,
0.707106781186547,0.707106781186548,0.707106781186548,0.707106781186548,
0.707106781186548,0.707106781186547,0.707106781186547,0.707106781186548,
0.707106781186547,0.707106781186547,0.707106781186548,0.707106781186548,
0.707106781186547,0.707106781186547,0.707106781186548,0.707106781186547,
0.707106781186547,0.707106781186548,0.707106781186547,0.707106781186548,
0.707106781186547,0.707106781186548,0.707106781186547,0.707106781186547,
0.707106781186547,0.707106781186548,0.707106781186547,0.707106781186547,
0.707106781186548,0.707106781186547,0.707106781186548,0.707106781186548,
0.707106781186548,0.707106781186547,0.707106781186547,0.707106781186547,
0.707106781186548,0.707106781186548,0.707106781186547,0.707106781186547,
0.707106781186547,0.707106781186547,0.707106781186548,0.707106781186548,
0.707106781186547,0.707106781186547,0.707106781186547,0.707106781186548,
0.707106781186548,0.707106781186547,0.707106781186548,0.707106781186547,
0.707106781186548,0.707106781186547,0.707106781186548,0.707106781186548,
0.707106781186547,0.707106781186548,0.707106781186548,0.707106781186548,
0.707106781186547,0.707106781186547,0.707106781186547,0.707106781186548,
0.707106781186548,0.707106781186548,0.707106781186547,0.707106781186547,
0.707106781186548,0.707106781186548,0.707106781186547,0.707106781186548,
0.707106781186547,0.707106781186547,0.707106781186548,0.707106781186547,
0.707106781186548,0.707106781186547,0.707106781186547,0.707106781186548,
0.707106781186547,0.707106781186548,0.707106781186548,0.707106781186547,
0.707106781186547,0.707106781186548,0.707106781186547,0.707106781186548,
0.707106781186547,0.707106781186547,0.707106781186548,0.707106781186547,
0.707106781186548,0.707106781186547,0.707106781186548,0.707106781186547,
0.707106781186547,0.707106781186548,0.707106781186547,0.707106781186547,
0.707106781186547,0.707106781186547,0.707106781186547,0.707106781186547,
0.707106781186548,0.707106781186547,0.707106781186548,0.707106781186548,
0.707106781186548,0.707106781186547,0.707106781186547,0.707106781186547,
0.707106781186548,0.707106781186547,0.707106781186548,0.707106781186547,
0.707106781186547,0.707106781186548,0.707106781186547,0.707106781186547,
0.707106781186547,0.707106781186547,0.707106781186547,0.707106781186548,
0.707106781186547,0.707106781186548,0.707106781186547,0.707106781186547,
0.707106781186548,0.707106781186548,0.707106781186547,0.707106781186547,
0.707106781186547,0.707106781186548,0.707106781186547,0.707106781186547,
0.707106781186548,0.707106781186548,0.707106781186547,0.707106781186548,
0.707106781186547,0.707106781186548,0.707106781186548,0.707106781186547,
0.707106781186547,0.707106781186547,0.707106781186548,0.707106781186548,
0.707106781186547,0.707106781186548,0.707106781186547,0.707106781186548,
0.707106781186548,0.707106781186547,0.707106781186548,0.707106781186547,
0.707106781186547,0.707106781186547,0.707106781186548,0.707106781186547,
0.707106781186548,0.707106781186547,0.707106781186548,0.707106781186547,
0.707106781186547,0.707106781186547,0.707106781186547,0.707106781186547,
0.707106781186548,0.707106781186547,0.707106781186548,0.707106781186547,
0.707106781186548,0.707106781186547,0.707106781186548,0.707106781186547,
0.707106781186547,0.707106781186547,0.707106781186547,0.707106781186547,
0.707106781186548,0.707106781186548,0.707106781186548,0.707106781186547,
0.707106781186548,0.707106781186547,0.707106781186548,0.707106781186547,
0.707106781186547,0.707106781186548,0.707106781186547,0.707106781186548,
0.707106781186547,0.707106781186547,0.707106781186547,0.707106781186548,
0.707106781186548,0.707106781186547,0.707106781186548,0.707106781186547,
0.707106781186548,0.707106781186548,0.707106781186547,0.707106781186548,
0.707106781186547,0.707106781186548,0.707106781186548,0.707106781186547,
0.707106781186547,0.707106781186547,0.707106781186547,0.707106781186547,
0.707106781186547,0.707106781186548,0.707106781186548,0.707106781186547,
0.707106781186548,0.707106781186547,0.707106781186547,0.707106781186548,
0.707106781186547,0.707106781186547,0.707106781186548,0.707106781186547,
0.707106781186547,0.707106781186547,0.707106781186548,0.707106781186547,
0.707106781186547,0.707106781186548,0.707106781186547,0.707106781186548,
0.707106781186548,0.707106781186547,0.707106781186547,0.707106781186547,
0.707106781186548,0.707106781186547,0.707106781186547,0.707106781186548,
0.707106781186548,0.707106781186548,0.707106781186548,0.707106781186547,
0.707106781186548,0.707106781186548,0.707106781186547,0.707106781186547,
0.707106781186548,0.707106781186547,0.707106781186548,0.707106781186547,
0.707106781186547,0.707106781186548,0.707106781186547,0.707106781186547,
0.707106781186548,0.707106781186547,0.707106781186548,0.707106781186547,
0.707106781186548,0.707106781186547,0.707106781186548,0.707106781186547,
0.707106781186548,0.707106781186547,0.707106781186548,0.707106781186548,
0.707106781186547,0.707106781186547,0.707106781186548,0.707106781186548,
0.707106781186547,0.707106781186547,0.707106781186547,0.707106781186547,
0.707106781186547,0.707106781186548,0.707106781186547,0.707106781186547,
0.707106781186548,0.707106781186547,0.707106781186548,0.707106781186548,
0.707106781186547,0.707106781186548,0.707106781186547,0.707106781186548,
0.707106781186547,0.707106781186548,0.707106781186547,0.707106781186547,
0.707106781186547,0.707106781186547,0.707106781186547,0.707106781186547,
0.707106781186548,0.707106781186547,0.707106781186548,0.707106781186547,
0.707106781186547,0.707106781186547,0.707106781186548,0.707106781186547,
0.707106781186548,0.707106781186548,0.707106781186547,0.707106781186547,
0.707106781186548,0.707106781186547,0.707106781186548,0.707106781186547,
0.707106781186548,0.707106781186547,0.707106781186548,0.707106781186547,
0.707106781186547,0.707106781186548,0.707106781186547,0.707106781186548,
0.707106781186547,0.707106781186548,0.707106781186548,0.707106781186548,
0.707106781186548,0.707106781186547,0.707106781186548,0.707106781186548,
0.707106781186548,0.707106781186547,0.707106781186548,0.707106781186548,
0.707106781186547,0.707106781186548,0.707106781186547,0.707106781186548,
0.707106781186547,0.707106781186547,0.707106781186547,0.707106781186548,
0.707106781186548,0.707106781186547,0.707106781186548,0.707106781186547,
0.707106781186548,0.707106781186547,0.707106781186548,0.707106781186548,
0.707106781186547,0.707106781186548,0.707106781186547,0.707106781186547,
0.707106781186548,0.707106781186547,0.707106781186547,0.707106781186547,
0.707106781186548,0.707106781186547,0.707106781186548,0.707106781186548,
0.707106781186547,0.707106781186548,0.707106781186547,0.707106781186548,
0.707106781186548,0.707106781186548,0.707106781186548,0.707106781186547,
0.707106781186548,0.707106781186547,0.707106781186548,0.707106781186547,
0.707106781186548,0.707106781186547,0.707106781186547,0.707106781186547,
0.707106781186547,0.707106781186548,0.707106781186547,0.707106781186548,
0.707106781186547,0.707106781186547,0.707106781186548,0.707106781186547,
0.707106781186548,0.707106781186547,0.707106781186548,0.707106781186547,
0.707106781186548,0.707106781186548,0.707106781186548,0.707106781186548,
0.707106781186547,0.707106781186548,0.707106781186548,0.707106781186547,
0.707106781186548,0.707106781186547,0.707106781186548,0.707106781186547,
0.707106781186548,0.707106781186547,0.707106781186547,0.707106781186548,
0.707106781186547,0.707106781186548,0.707106781186547,0.707106781186547,
0.707106781186548,0.707106781186547,0.707106781186548,0.707106781186547,
0.707106781186547,0.707106781186548,0.707106781186548,0.707106781186548,
0.707106781186548,0.707106781186548,0.707106781186548,0.707106781186548,
0.707106781186548,0.707106781186548,0.707106781186547,0.707106781186548,
0.707106781186547,0.707106781186547,0.707106781186548,0.707106781186547,
0.707106781186548,0.707106781186548,0.707106781186547,0.707106781186547,
0.707106781186548,0.707106781186548,0.707106781186547,0.707106781186547,
0.707106781186547,0.707106781186547,0.707106781186547,0.707106781186548,
0.707106781186547,0.707106781186548,0.707106781186548,0.707106781186548,
0.707106781186547,0.707106781186548,0.707106781186547,0.707106781186548,
0.707106781186547,0.707106781186548,0.707106781186547,0.707106781186548,
0.707106781186548,0.707106781186547,0.707106781186547,0.707106781186548,
0.707106781186548,0.707106781186548,0.707106781186547,0.707106781186547,
0.707106781186548,0.707106781186547,0.707106781186547,0.707106781186548,
0.707106781186547,0.707106781186548,0.707106781186547,0.707106781186547,
0.707106781186548,0.707106781186548,0.707106781186548,0.707106781186547,
0.707106781186547,0.707106781186548,0.707106781186547,0.707106781186548,
0.707106781186547,0.707106781186548,0.707106781186547,0.707106781186548,
0.707106781186548,0.707106781186547,0.707106781186548,0.707106781186547,
0.707106781186548,0.707106781186547,0.707106781186547,0.707106781186547,
0.707106781186548,0.707106781186547,0.707106781186548,0.707106781186547,
0.707106781186547,0.707106781186547,0.707106781186548,0.707106781186547,
0.707106781186547,0.707106781186548,0.707106781186548,0.707106781186547,
0.707106781186548,0.707106781186547,0.707106781186548,0.707106781186548,
0.707106781186547,0.707106781186548,0.707106781186547,0.707106781186547,
0.707106781186548,0.707106781186547,0.707106781186547,0.707106781186547,
0.707106781186548,0.707106781186547,0.707106781186548,0.707106781186547,
0.707106781186548,0.707106781186548,0.707106781186548,0.707106781186547,
0.707106781186548,0.707106781186548,0.707106781186548,0.707106781186547,
0.707106781186548,0.707106781186547,0.707106781186547,0.707106781186548,
0.707106781186547,0.707106781186547,0.707106781186548,0.707106781186548,
0.707106781186547,0.707106781186548,0.707106781186547,0.707106781186548,
0.707106781186548,0.707106781186547,0.707106781186548,0.707106781186547,
0.707106781186548,0.707106781186547,0.707106781186548,0.707106781186547,
0.707106781186548,0.707106781186548,0.707106781186548,0.707106781186547,
0.707106781186548,0.707106781186548,0.707106781186547,0.707106781186547,
0.707106781186548,0.707106781186547,0.707106781186548,0.707106781186548,
0.707106781186547,0.707106781186548,0.707106781186548,0.707106781186547,
0.707106781186548,0.707106781186548,0.707106781186547,0.707106781186547,
0.707106781186548,0.707106781186547,0.707106781186548,0.707106781186547,
0.707106781186548,0.707106781186547,0.707106781186548,0.707106781186548,
0.707106781186548,0.707106781186547,0.707106781186548,0.707106781186547,
0.707106781186548,0.707106781186547,0.707106781186548,0.707106781186547,
0.707106781186548,0.707106781186547,0.707106781186548,0.707106781186547,
0.707106781186548,0.707106781186547,0.707106781186547,0.707106781186547,
0.707106781186548,0.707106781186547,0.707106781186548,0.707106781186547,
0.707106781186548,0.707106781186547,0.707106781186548,0.707106781186547,
0.707106781186548,0.707106781186548,0.707106781186548,0.707106781186547,
0.707106781186548,0.707106781186547,0.707106781186548,0.707106781186548,
0.707106781186547,0.707106781186548,0.707106781186547,0.707106781186548,
0.707106781186547,0.707106781186548,0.707106781186547,0.707106781186548,
0.707106781186547,0.707106781186547,0.707106781186547,0.707106781186548,
0.707106781186547,0.707106781186547,0.707106781186548,0.707106781186547,
0.707106781186548,0.707106781186547,0.707106781186547,0.707106781186548,
0.707106781186547,0.707106781186548,0.707106781186547,0.707106781186548,
0.707106781186548,0.707106781186548,0.707106781186547,0.707106781186547,
0.707106781186548,0.707106781186548,0.707106781186547,0.707106781186548,
0.707106781186547,0.707106781186547,0.707106781186547,0.707106781186548,
0.707106781186547,0.707106781186548,0.707106781186547,0.707106781186548,
0.707106781186548,0.707106781186548,0.707106781186547,0.707106781186547,
0.707106781186547,0.707106781186547,0.707106781186547,0.707106781186547,
0.707106781186548,0.707106781186547,0.707106781186548,0.707106781186547,
0.707106781186548,0.707106781186547,0.707106781186547,0.707106781186548,
0.707106781186547,0.707106781186547,0.707106781186548,0.707106781186548,
0.707106781186547,0.707106781186547,0.707106781186547,0.707106781186548,
0.707106781186547,0.707106781186547,0.707106781186548,0.707106781186548),
(1.,1.,1.,1.,1.,1.,1.,1.,1.,1.,1.,1.,1.,1.,1.,1.,1.,1.,1.,1.,1.,1.,1.,1.,
1.,1.,1.,1.,1.,1.,1.,1.,1.,1.,1.,1.,1.,1.,1.,1.,1.,1.,1.,1.,1.,1.,1.,1.,
1.,1.,1.,1.,1.,1.,1.,1.,1.,1.,1.,1.,1.,1.,1.,1.,1.,1.,1.,1.,1.,1.,1.,1.,
1.,1.,1.,1.,1.,1.,1.,1.,1.,1.,1.,1.,1.,1.,1.,1.,1.,1.,1.,1.,1.,1.,1.,1.,
1.,1.,1.,1.,1.,1.,1.,1.,1.,1.,1.,1.,1.,1.,1.,1.,1.,1.,1.,1.,1.,1.,1.,1.,
1.,1.,1.,1.,1.,1.,1.,1.,1.,1.,1.,1.,1.,1.,1.,1.,1.,1.,1.,1.,1.,1.,1.,1.,
1.,1.,1.,1.,1.,1.,1.,1.,1.,1.,1.,1.,1.,1.,1.,1.,1.,1.,1.,1.,1.,1.,1.,1.,
1.,1.,1.,1.,1.,1.,1.,1.,1.,1.,1.,1.,1.,1.,1.,1.,1.,1.,1.,1.,1.,1.,1.,1.,
1.,1.,1.,1.,1.,1.,1.,1.,1.,1.,1.,1.,1.,1.,1.,1.,1.,1.,1.,1.,1.,1.,1.,1.,
1.,1.,1.,1.,1.,1.,1.,1.,1.,1.,1.,1.,1.,1.,1.,1.,1.,1.,1.,1.,1.,1.,1.,1.,
1.,1.,1.,1.,1.,1.,1.,1.,1.,1.,1.,1.,1.,1.,1.,1.,1.,1.,1.,1.,1.,1.,1.,1.,
1.,1.,1.,1.,1.,1.,1.,1.,1.,1.,1.,1.,1.,1.,1.,1.,1.,1.,1.,1.,1.,1.,1.,1.,
1.,1.,1.,1.,1.,1.,1.,1.,1.,1.,1.,1.,1.,1.,1.,1.,1.,1.,1.,1.,1.,1.,1.,1.,
1.,1.,1.,1.,1.,1.,1.,1.,1.,1.,1.,1.,1.,1.,1.,1.,1.,1.,1.,1.,1.,1.,1.,1.,
1.,1.,1.,1.,1.,1.,1.,1.,1.,1.,1.,1.,1.,1.,1.,1.,1.,1.,1.,1.,1.,1.,1.,1.,
1.,1.,1.,1.,1.,1.,1.,1.,1.,1.,1.,1.,1.,1.,1.,1.,1.,1.,1.,1.,1.,1.,1.,1.,
1.,1.,1.,1.,1.,1.,1.,1.,1.,1.,1.,1.,1.,1.,1.,1.,1.,1.,1.,1.,1.,1.,1.,1.,
1.,1.,1.,1.,1.,1.,1.,1.,1.,1.,1.,1.,1.,1.,1.,1.,1.,1.,1.,1.,1.,1.,1.,1.,
1.,1.,1.,1.,1.,1.,1.,1.,1.,1.,1.,1.,1.,1.,1.,1.,1.,1.,1.,1.,1.,1.,1.,1.,
1.,1.,1.,1.,1.,1.,1.,1.,1.,1.,1.,1.,1.,1.,1.,1.,1.,1.,1.,1.,1.,1.,1.,1.,
1.,1.,1.,1.,1.,1.,1.,1.,1.,1.,1.,1.,1.,1.,1.,1.,1.,1.,1.,1.,1.,1.,1.,1.,
1.,1.,1.,1.,1.,1.,1.,1.,1.,1.,1.,1.,1.,1.,1.,1.,1.,1.,1.,1.,1.,1.,1.,1.,
1.,1.,1.,1.,1.,1.,1.,1.,1.,1.,1.,1.,1.,1.,1.,1.,1.,1.,1.,1.,1.,1.,1.,1.,
1.,1.,1.,1.,1.,1.,1.,1.,1.,1.,1.,1.,1.,1.,1.,1.,1.,1.,1.,1.,1.,1.,1.,1.,
1.,1.,1.,1.,1.,1.,1.,1.,1.,1.,1.,1.,1.,1.,1.,1.,1.,1.,1.,1.,1.,1.,1.,1.,
1.,1.,1.,1.,1.,1.,1.,1.,1.,1.,1.,1.,1.,1.,1.,1.,1.,1.,1.,1.,1.,1.,1.,1.,
1.,1.,1.,1.,1.,1.,1.,1.,1.,1.,1.,1.,1.,1.,1.,1.,1.,1.,1.,1.,1.,1.,1.,1.,
1.,1.,1.,1.,1.,1.,1.,1.,1.,1.,1.,1.,1.,1.,1.,1.,1.,1.,1.,1.,1.,1.,1.,1.,
1.,1.,1.,1.,1.,1.,1.,1.,1.,1.,1.,1.,1.,1.,1.,1.,1.,1.,1.,1.,1.,1.,1.,1.,
1.,1.,1.,1.,1.,1.,1.,1.,1.,1.,1.,1.,1.,1.,1.,1.,1.,1.,1.,1.,1.,1.,1.,1.,
1.,1.,1.,1.,1.,1.,1.,1.,1.,1.,1.,1.,1.,1.,1.,1.,1.,1.,1.,1.,1.,1.,1.,1.,
1.,1.,1.,1.,1.,1.,1.,1.,1.,1.,1.,1.,1.,1.,1.,1.,1.,1.,1.,1.,1.,1.,1.,1.,
1.,1.,1.,1.,1.,1.,1.,1.,1.,1.,1.,1.,1.,1.,1.,1.,1.,1.,1.,1.,1.,1.,1.,1.,
1.,1.,1.,1.,1.,1.,1.,1.,1.,1.,1.,1.,1.,1.,1.,1.,1.,1.,1.,1.,1.,1.,1.,1.,
1.,1.,1.,1.,1.,1.,1.,1.,1.,1.,1.,1.,1.,1.,1.,1.,1.,1.,1.,1.,1.,1.,1.,1.,
1.,1.,1.,1.,1.,1.,1.,1.,1.,1.,1.,1.,1.,1.,1.,1.,1.,1.,1.,1.,1.,1.,1.,1.,
1.,1.,1.,1.,1.,1.,1.,1.,1.,1.,1.,1.,1.,1.,1.,1.,1.,1.,1.,1.,1.,1.,1.,1.,
1.,1.,1.,1.,1.,1.,1.,1.,1.,1.,1.,1.,1.,1.,1.,1.,1.,1.,1.,1.,1.,1.,1.,1.,
1.,1.,1.,1.,1.,1.,1.,1.,1.,1.,1.,1.,1.,1.,1.,1.,1.,1.,1.,1.,1.,1.,1.,1.,
1.,1.,1.,1.,1.,1.,1.,1.,1.,1.,1.,1.,1.,1.,1.,1.,1.,1.,1.,1.,1.,1.,1.,1.,
1.,1.,1.,1.,1.,1.,1.,1.,1.,1.,1.,1.,1.,1.,1.,1.,1.,1.,1.,1.,1.,1.,1.,1.,
1.,1.,1.,1.,1.,1.,1.,1.,1.,1.,1.,1.,1.,1.,1.,1.,1.,1.,1.,1.,1.,1.,1.,1.,
1.,1.,1.,1.,1.,1.,1.,1.,1.,1.,1.,1.,1.,1.,1.,1.,1.,1.,1.,1.,1.,1.,1.,1.,
1.,1.,1.,1.,1.,1.,1.,1.,1.,1.,1.,1.,1.,1.,1.,1.,1.,1.,1.,1.,1.,1.,1.,1.,
1.,1.,1.,1.,1.,1.,1.,1.,1.,1.,1.,1.,1.,1.,1.,1.,1.,1.,1.,1.,1.,1.,1.,1.,
1.,1.,1.,1.,1.,1.,1.,1.,1.,1.,1.,1.,1.,1.,1.,1.,1.,1.,1.,1.,1.,1.,1.,1.,
1.,1.,1.,1.,1.,1.,1.,1.,1.,1.,1.,1.,1.,1.,1.,1.,1.,1.,1.,1.,1.,1.,1.,1.,
1.,1.,1.,1.,1.,1.,1.,1.,1.,1.,1.,1.,1.,1.,1.,1.,1.,1.,1.,1.,1.,1.,1.,1.,
1.,1.,1.,1.,1.,1.,1.,1.,1.,1.,1.,1.,1.,1.,1.,1.,1.,1.,1.,1.,1.,1.,1.,1.,
1.,1.,1.,1.,1.,1.,1.,1.,1.,1.,1.,1.,1.,1.,1.,1.,1.,1.,1.,1.,1.,1.,1.,1.,
1.,1.,1.,1.,1.,1.,1.,1.,1.,1.,1.,1.,1.,1.,1.,1.,1.,1.,1.,1.,1.,1.,1.,1.,
1.,1.,1.,1.,1.,1.,1.,1.,1.,1.,1.,1.,1.,1.,1.,1.,1.,1.,1.,1.,1.,1.,1.,1.,
1.,1.,1.,1.,1.,1.,1.,1.,1.,1.,1.,1.,1.,1.,1.,1.,1.,1.,1.,1.,1.,1.,1.,1.,
1.,1.,1.,1.,1.,1.,1.,1.,1.,1.,1.,1.,1.,1.,1.,1.,1.,1.,1.,1.,1.,1.,1.,1.,
1.,1.,1.,1.,1.,1.,1.,1.,1.,1.,1.,1.,1.,1.,1.,1.,1.,1.,1.,1.,1.,1.,1.,1.,
1.,1.,1.,1.,1.,1.,1.,1.,1.,1.,1.,1.,1.,1.,1.,1.,1.,1.,1.,1.,1.,1.,1.,1.,
1.,1.,1.,1.,1.,1.,1.,1.,1.,1.,1.,1.,1.,1.,1.,1.,1.,1.,1.,1.,1.,1.,1.,1.,
1.,1.,1.,1.,1.,1.,1.,1.,1.,1.,1.,1.,1.,1.,1.,1.,1.,1.,1.,1.,1.,1.,1.,1.,
1.,1.,1.,1.,1.,1.,1.,1.,1.,1.,1.,1.,1.,1.,1.,1.,1.,1.,1.,1.,1.,1.,1.,1.,
1.,1.,1.,1.,1.,1.,1.,1.,1.,1.,1.,1.,1.,1.,1.,1.,1.,1.,1.,1.,1.,1.,1.,1.,
1.,1.,1.,1.,1.,1.,1.,1.,1.,1.,1.,1.,1.,1.,1.,1.,1.,1.,1.,1.,1.,1.,1.,1.,
1.,1.,1.,1.,1.,1.,1.,1.,1.,1.,1.,1.,1.,1.,1.,1.,1.,1.,1.,1.,1.,1.,1.,1.,
1.,1.,1.,1.,1.,1.,1.,1.,1.,1.,1.,1.,1.,1.,1.,1.,1.,1.,1.,1.,1.,1.,1.,1.,
1.,1.,1.,1.,1.,1.,1.,1.,1.,1.,1.,1.,1.,1.,1.,1.,1.,1.,1.,1.,1.,1.,1.,1.,
1.,1.,1.,1.,1.,1.,1.,1.,1.,1.,1.,1.,1.,1.,1.,1.,1.,1.,1.,1.,1.,1.,1.,1.,
1.,1.,1.,1.,1.,1.,1.,1.,1.,1.,1.,1.,1.,1.,1.,1.,1.,1.,1.,1.,1.,1.,1.,1.,
1.,1.,1.,1.,1.,1.,1.,1.,1.,1.,1.,1.,1.,1.,1.,1.,1.,1.,1.,1.,1.,1.,1.,1.,
1.,1.,1.,1.,1.,1.,1.,1.,1.,1.,1.,1.,1.,1.,1.,1.,1.,1.,1.,1.,1.,1.,1.,1.,
1.,1.,1.,1.,1.,1.,1.,1.,1.,1.,1.,1.,1.,1.,1.,1.,1.,1.,1.,1.,1.,1.,1.,1.,
1.,1.,1.,1.,1.,1.,1.,1.,1.,1.,1.,1.,1.,1.,1.,1.,1.,1.,1.,1.,1.,1.,1.,1.,
1.,1.,1.,1.,1.,1.,1.,1.,1.,1.,1.,1.,1.,1.,1.,1.,1.,1.,1.,1.,1.,1.,1.,1.,
1.,1.,1.,1.,1.,1.,1.,1.,1.,1.,1.,1.,1.,1.,1.,1.,1.,1.,1.,1.,1.,1.,1.,1.,
1.,1.,1.,1.,1.,1.,1.,1.,1.,1.,1.,1.,1.,1.,1.,1.,1.,1.,1.,1.,1.,1.,1.,1.,
1.,1.,1.,1.,1.,1.,1.,1.,1.,1.,1.,1.,1.,1.,1.,1.,1.,1.,1.,1.,1.,1.,1.,1.,
1.,1.,1.,1.,1.,1.,1.,1.,1.,1.,1.,1.,1.,1.,1.,1.,1.,1.,1.,1.,1.,1.,1.,1.,
1.,1.,1.,1.,1.,1.,1.,1.,1.,1.,1.,1.,1.,1.,1.,1.,1.,1.,1.,1.,1.,1.,1.,1.,
1.,1.,1.,1.,1.,1.,1.,1.,1.,1.,1.,1.,1.,1.,1.,1.,1.,1.,1.,1.,1.,1.,1.,1.,
1.,1.,1.,1.,1.,1.,1.,1.,1.,1.,1.,1.,1.,1.,1.,1.,1.,1.,1.,1.,1.,1.,1.,1.,
1.,1.,1.,1.,1.,1.,1.,1.,1.,1.,1.,1.,1.,1.,1.,1.,1.,1.,1.,1.,1.,1.,1.,1.,
1.,1.,1.,1.,1.,1.,1.,1.,1.,1.,1.,1.,1.,1.,1.,1.,1.,1.,1.,1.,1.,1.,1.,1.,
1.,1.,1.,1.,1.,1.,1.,1.,1.,1.,1.,1.,1.,1.,1.,1.,1.,1.,1.,1.,1.,1.,1.,1.,
1.,1.,1.,1.,1.,1.,1.,1.,1.,1.,1.,1.,1.,1.,1.,1.,1.,1.,1.,1.,1.,1.,1.,1.,
1.,1.,1.,1.,1.,1.,1.,1.,1.,1.,1.,1.,1.,1.,1.,1.,1.,1.,1.,1.,1.,1.,1.,1.,
1.,1.,1.,1.,1.,1.,1.,1.,1.,1.,1.,1.,1.,1.,1.,1.,1.,1.,1.,1.,1.,1.,1.,1.,
1.,1.,1.,1.,1.,1.,1.,1.,1.,1.,1.,1.,1.,1.,1.,1.,1.,1.,1.,1.,1.,1.,1.,1.,
1.,1.,1.,1.,1.,1.,1.,1.,1.,1.,1.),(0.707106781186548,0.707106781186548,
0.707106781186548,0.707106781186547,0.707106781186547,0.707106781186548,
0.707106781186547,0.707106781186547,0.707106781186547,0.707106781186547,
0.707106781186547,0.707106781186548,0.707106781186548,0.707106781186548,
0.707106781186547,0.707106781186548,0.707106781186547,0.707106781186547,
0.707106781186548,0.707106781186547,0.707106781186548,0.707106781186547,
0.707106781186548,0.707106781186547,0.707106781186548,0.707106781186547,
0.707106781186547,0.707106781186547,0.707106781186547,0.707106781186547,
0.707106781186548,0.707106781186547,0.707106781186547,0.707106781186548,
0.707106781186547,0.707106781186547,0.707106781186548,0.707106781186547,
0.707106781186547,0.707106781186548,0.707106781186548,0.707106781186547,
0.707106781186548,0.707106781186547,0.707106781186547,0.707106781186547,
0.707106781186548,0.707106781186548,0.707106781186547,0.707106781186547,
0.707106781186548,0.707106781186547,0.707106781186548,0.707106781186547,
0.707106781186547,0.707106781186547,0.707106781186547,0.707106781186547,
0.707106781186548,0.707106781186547,0.707106781186548,0.707106781186547,
0.707106781186548,0.707106781186547,0.707106781186548,0.707106781186547,
0.707106781186547,0.707106781186548,0.707106781186547,0.707106781186547,
0.707106781186548,0.707106781186547,0.707106781186548,0.707106781186547,
0.707106781186548,0.707106781186548,0.707106781186547,0.707106781186548,
0.707106781186547,0.707106781186547,0.707106781186548,0.707106781186547,
0.707106781186547,0.707106781186547,0.707106781186548,0.707106781186547,
0.707106781186547,0.707106781186547,0.707106781186547,0.707106781186547,
0.707106781186547,0.707106781186548,0.707106781186548,0.707106781186547,
0.707106781186548,0.707106781186547,0.707106781186548,0.707106781186548,
0.707106781186547,0.707106781186548,0.707106781186548,0.707106781186548,
0.707106781186547,0.707106781186548,0.707106781186547,0.707106781186548,
0.707106781186548,0.707106781186548,0.707106781186547,0.707106781186547,
0.707106781186547,0.707106781186548,0.707106781186548,0.707106781186548,
0.707106781186547,0.707106781186547,0.707106781186547,0.707106781186548,
0.707106781186548,0.707106781186547,0.707106781186547,0.707106781186548,
0.707106781186547,0.707106781186547,0.707106781186547,0.707106781186547,
0.707106781186548,0.707106781186547,0.707106781186548,0.707106781186547,
0.707106781186547,0.707106781186547,0.707106781186548,0.707106781186548,
0.707106781186547,0.707106781186548,0.707106781186548,0.707106781186547,
0.707106781186548,0.707106781186547,0.707106781186548,0.707106781186547,
0.707106781186548,0.707106781186547,0.707106781186547,0.707106781186548,
0.707106781186547,0.707106781186547,0.707106781186548,0.707106781186547,
0.707106781186547,0.707106781186548,0.707106781186547,0.707106781186548,
0.707106781186547,0.707106781186547,0.707106781186548,0.707106781186548,
0.707106781186547,0.707106781186548,0.707106781186547,0.707106781186548,
0.707106781186547,0.707106781186548,0.707106781186547,0.707106781186548,
0.707106781186547,0.707106781186548,0.707106781186547,0.707106781186548,
0.707106781186547,0.707106781186548,0.707106781186547,0.707106781186547,
0.707106781186548,0.707106781186547,0.707106781186548,0.707106781186547,
0.707106781186548,0.707106781186547,0.707106781186548,0.707106781186547,
0.707106781186547,0.707106781186548,0.707106781186547,0.707106781186548,
0.707106781186548,0.707106781186548,0.707106781186547,0.707106781186547,
0.707106781186547,0.707106781186547,0.707106781186548,0.707106781186547,
0.707106781186548,0.707106781186548,0.707106781186547,0.707106781186547,
0.707106781186548,0.707106781186548,0.707106781186547,0.707106781186547,
0.707106781186548,0.707106781186547,0.707106781186548,0.707106781186547,
0.707106781186547,0.707106781186547,0.707106781186547,0.707106781186547,
0.707106781186547,0.707106781186547,0.707106781186548,0.707106781186547,
0.707106781186548,0.707106781186547,0.707106781186548,0.707106781186548,
0.707106781186547,0.707106781186548,0.707106781186548,0.707106781186548,
0.707106781186548,0.707106781186547,0.707106781186548,0.707106781186547,
0.707106781186548,0.707106781186547,0.707106781186547,0.707106781186548,
0.707106781186548,0.707106781186547,0.707106781186547,0.707106781186547,
0.707106781186547,0.707106781186547,0.707106781186548,0.707106781186548,
0.707106781186547,0.707106781186547,0.707106781186548,0.707106781186548,
0.707106781186547,0.707106781186548,0.707106781186547,0.707106781186548,
0.707106781186548,0.707106781186547,0.707106781186547,0.707106781186548,
0.707106781186547,0.707106781186547,0.707106781186548,0.707106781186547,
0.707106781186548,0.707106781186547,0.707106781186548,0.707106781186547,
0.707106781186547,0.707106781186548,0.707106781186548,0.707106781186547,
0.707106781186547,0.707106781186548,0.707106781186547,0.707106781186547,
0.707106781186548,0.707106781186547,0.707106781186548,0.707106781186547,
0.707106781186548,0.707106781186547,0.707106781186548,0.707106781186547,
0.707106781186547,0.707106781186547,0.707106781186547,0.707106781186547,
0.707106781186547,0.707106781186548,0.707106781186547,0.707106781186548,
0.707106781186547,0.707106781186548,0.707106781186548,0.707106781186547,
0.707106781186548,0.707106781186548,0.707106781186547,0.707106781186548,
0.707106781186547,0.707106781186547,0.707106781186547,0.707106781186548,
0.707106781186547,0.707106781186547,0.707106781186548,0.707106781186547,
0.707106781186548,0.707106781186547,0.707106781186547,0.707106781186547,
0.707106781186548,0.707106781186548,0.707106781186547,0.707106781186548,
0.707106781186548,0.707106781186547,0.707106781186548,0.707106781186547,
0.707106781186548,0.707106781186548,0.707106781186547,0.707106781186548,
0.707106781186548,0.707106781186548,0.707106781186547,0.707106781186547,
0.707106781186548,0.707106781186547,0.707106781186548,0.707106781186547,
0.707106781186547,0.707106781186548,0.707106781186548,0.707106781186548,
0.707106781186547,0.707106781186547,0.707106781186548,0.707106781186548,
0.707106781186547,0.707106781186547,0.707106781186548,0.707106781186547,
0.707106781186547,0.707106781186548,0.707106781186548,0.707106781186547,
0.707106781186547,0.707106781186547,0.707106781186548,0.707106781186547,
0.707106781186547,0.707106781186547,0.707106781186548,0.707106781186548,
0.707106781186547,0.707106781186548,0.707106781186547,0.707106781186548,
0.707106781186547,0.707106781186548,0.707106781186548,0.707106781186547,
0.707106781186547,0.707106781186548,0.707106781186547,0.707106781186547,
0.707106781186548,0.707106781186547,0.707106781186548,0.707106781186548,
0.707106781186547,0.707106781186548,0.707106781186547,0.707106781186547,
0.707106781186547,0.707106781186548,0.707106781186548,0.707106781186548,
0.707106781186547,0.707106781186548,0.707106781186547,0.707106781186548,
0.707106781186547,0.707106781186547,0.707106781186547,0.707106781186547,
0.707106781186548,0.707106781186548,0.707106781186547,0.707106781186547,
0.707106781186548,0.707106781186547,0.707106781186548,0.707106781186547,
0.707106781186548,0.707106781186547,0.707106781186547,0.707106781186548,
0.707106781186547,0.707106781186548,0.707106781186547,0.707106781186548,
0.707106781186548,0.707106781186547,0.707106781186548,0.707106781186547,
0.707106781186548,0.707106781186548,0.707106781186547,0.707106781186548,
0.707106781186547,0.707106781186547,0.707106781186548,0.707106781186547,
0.707106781186548,0.707106781186547,0.707106781186548,0.707106781186547,
0.707106781186547,0.707106781186548,0.707106781186548,0.707106781186548,
0.707106781186548,0.707106781186547,0.707106781186548,0.707106781186548,
0.707106781186548,0.707106781186547,0.707106781186548,0.707106781186548,
0.707106781186548,0.707106781186547,0.707106781186547,0.707106781186548,
0.707106781186547,0.707106781186548,0.707106781186547,0.707106781186548,
0.707106781186548,0.707106781186547,0.707106781186547,0.707106781186548,
0.707106781186547,0.707106781186548,0.707106781186547,0.707106781186548,
0.707106781186548,0.707106781186547,0.707106781186547,0.707106781186547,
0.707106781186548,0.707106781186548,0.707106781186547,0.707106781186547,
0.707106781186548,0.707106781186548,0.707106781186548,0.707106781186548,
0.707106781186547,0.707106781186547,0.707106781186548,0.707106781186548,
0.707106781186547,0.707106781186548,0.707106781186547,0.707106781186548,
0.707106781186547,0.707106781186548,0.707106781186547,0.707106781186547,
0.707106781186548,0.707106781186547,0.707106781186547,0.707106781186548,
0.707106781186547,0.707106781186548,0.707106781186547,0.707106781186548,
0.707106781186547,0.707106781186548,0.707106781186547,0.707106781186548,
0.707106781186547,0.707106781186548,0.707106781186547,0.707106781186547,
0.707106781186548,0.707106781186548,0.707106781186547,0.707106781186547,
0.707106781186547,0.707106781186548,0.707106781186547,0.707106781186548,
0.707106781186547,0.707106781186548,0.707106781186547,0.707106781186548,
0.707106781186547,0.707106781186547,0.707106781186547,0.707106781186548,
0.707106781186547,0.707106781186548,0.707106781186548,0.707106781186547,
0.707106781186548,0.707106781186547,0.707106781186547,0.707106781186548,
0.707106781186547,0.707106781186547,0.707106781186548,0.707106781186547,
0.707106781186547,0.707106781186547,0.707106781186547,0.707106781186548,
0.707106781186547,0.707106781186547,0.707106781186547,0.707106781186548,
0.707106781186547,0.707106781186547,0.707106781186548,0.707106781186548,
0.707106781186547,0.707106781186548,0.707106781186548,0.707106781186547,
0.707106781186547,0.707106781186548,0.707106781186547,0.707106781186547,
0.707106781186548,0.707106781186547,0.707106781186547,0.707106781186547,
0.707106781186548,0.707106781186547,0.707106781186548,0.707106781186547,
0.707106781186548,0.707106781186547,0.707106781186548,0.707106781186547,
0.707106781186548,0.707106781186547,0.707106781186548,0.707106781186548,
0.707106781186547,0.707106781186547,0.707106781186548,0.707106781186547,
0.707106781186548,0.707106781186547,0.707106781186548,0.707106781186548,
0.707106781186547,0.707106781186548,0.707106781186547,0.707106781186548,
0.707106781186548,0.707106781186547,0.707106781186547,0.707106781186548,
0.707106781186547,0.707106781186548,0.707106781186547,0.707106781186548,
0.707106781186547,0.707106781186548,0.707106781186547,0.707106781186547,
0.707106781186547,0.707106781186547,0.707106781186547,0.707106781186547,
0.707106781186547,0.707106781186547,0.707106781186548,0.707106781186547,
0.707106781186548,0.707106781186547,0.707106781186547,0.707106781186548,
0.707106781186547,0.707106781186548,0.707106781186547,0.707106781186547,
0.707106781186548,0.707106781186547,0.707106781186548,0.707106781186547,
0.707106781186548,0.707106781186547,0.707106781186548,0.707106781186547,
0.707106781186548,0.707106781186547,0.707106781186548,0.707106781186547,
0.707106781186548,0.707106781186548,0.707106781186547,0.707106781186548,
0.707106781186547,0.707106781186547,0.707106781186547,0.707106781186548,
0.707106781186547,0.707106781186547,0.707106781186547,0.707106781186548,
0.707106781186547,0.707106781186547,0.707106781186548,0.707106781186547,
0.707106781186547,0.707106781186547,0.707106781186547,0.707106781186548,
0.707106781186547,0.707106781186547,0.707106781186547,0.707106781186548,
0.707106781186548,0.707106781186548,0.707106781186548,0.707106781186547,
0.707106781186548,0.707106781186547,0.707106781186547,0.707106781186548,
0.707106781186547,0.707106781186548,0.707106781186547,0.707106781186547,
0.707106781186548,0.707106781186547,0.707106781186547,0.707106781186547,
0.707106781186547,0.707106781186548,0.707106781186548,0.707106781186547,
0.707106781186547,0.707106781186548,0.707106781186547,0.707106781186548,
0.707106781186547,0.707106781186548,0.707106781186548,0.707106781186547,
0.707106781186547,0.707106781186548,0.707106781186548,0.707106781186547,
0.707106781186548,0.707106781186548,0.707106781186547,0.707106781186548,
0.707106781186548,0.707106781186548,0.707106781186547,0.707106781186548,
0.707106781186547,0.707106781186548,0.707106781186547,0.707106781186548,
0.707106781186547,0.707106781186548,0.707106781186547,0.707106781186548,
0.707106781186548,0.707106781186547,0.707106781186547,0.707106781186548,
0.707106781186547,0.707106781186548,0.707106781186547,0.707106781186548,
0.707106781186548,0.707106781186548,0.707106781186548,0.707106781186548,
0.707106781186547,0.707106781186547,0.707106781186547,0.707106781186547,
0.707106781186548,0.707106781186547,0.707106781186548,0.707106781186547,
0.707106781186547,0.707106781186548,0.707106781186548,0.707106781186547,
0.707106781186548,0.707106781186547,0.707106781186548,0.707106781186548,
0.707106781186547,0.707106781186547,0.707106781186548,0.707106781186547,
0.707106781186548,0.707106781186547,0.707106781186548,0.707106781186547,
0.707106781186548,0.707106781186547,0.707106781186548,0.707106781186547,
0.707106781186548,0.707106781186547,0.707106781186548,0.707106781186548,
0.707106781186547,0.707106781186548,0.707106781186547,0.707106781186548,
0.707106781186547,0.707106781186548,0.707106781186548,0.707106781186548,
0.707106781186547,0.707106781186547,0.707106781186548,0.707106781186548,
0.707106781186547,0.707106781186547,0.707106781186547,0.707106781186548,
0.707106781186547,0.707106781186548,0.707106781186547,0.707106781186548,
0.707106781186547,0.707106781186547,0.707106781186547,0.707106781186548,
0.707106781186547,0.707106781186548,0.707106781186547,0.707106781186548,
0.707106781186547,0.707106781186548,0.707106781186547,0.707106781186547,
0.707106781186548,0.707106781186547,0.707106781186547,0.707106781186548,
0.707106781186547,0.707106781186547,0.707106781186548,0.707106781186547,
0.707106781186547,0.707106781186547,0.707106781186548,0.707106781186547,
0.707106781186548,0.707106781186547,0.707106781186547,0.707106781186547,
0.707106781186548,0.707106781186548,0.707106781186547,0.707106781186547,
0.707106781186548,0.707106781186548,0.707106781186548,0.707106781186547,
0.707106781186548,0.707106781186547,0.707106781186548,0.707106781186547,
0.707106781186548,0.707106781186547,0.707106781186547,0.707106781186547,
0.707106781186547,0.707106781186548,0.707106781186547,0.707106781186548,
0.707106781186548,0.707106781186547,0.707106781186548,0.707106781186547,
0.707106781186547,0.707106781186547,0.707106781186547,0.707106781186548,
0.707106781186547,0.707106781186548,0.707106781186547,0.707106781186548,
0.707106781186548,0.707106781186547,0.707106781186548,0.707106781186547,
0.707106781186547,0.707106781186547,0.707106781186547,0.707106781186548,
0.707106781186547,0.707106781186548,0.707106781186548,0.707106781186547,
0.707106781186548,0.707106781186547,0.707106781186548,0.707106781186547,
0.707106781186547,0.707106781186548,0.707106781186547,0.707106781186548,
0.707106781186548,0.707106781186547,0.707106781186547,0.707106781186548,
0.707106781186548,0.707106781186547,0.707106781186547,0.707106781186548,
0.707106781186547,0.707106781186547,0.707106781186548,0.707106781186547,
0.707106781186547,0.707106781186548,0.707106781186547,0.707106781186548,
0.707106781186547,0.707106781186547,0.707106781186548,0.707106781186547,
0.707106781186548,0.707106781186547,0.707106781186548,0.707106781186547,
0.707106781186547,0.707106781186547,0.707106781186548,0.707106781186547,
0.707106781186548,0.707106781186547,0.707106781186548,0.707106781186548,
0.707106781186548,0.707106781186548,0.707106781186547,0.707106781186547,
0.707106781186547,0.707106781186548,0.707106781186547,0.707106781186548,
0.707106781186547,0.707106781186547,0.707106781186548,0.707106781186547,
0.707106781186547,0.707106781186548,0.707106781186547,0.707106781186547,
0.707106781186548,0.707106781186548,0.707106781186547,0.707106781186548,
0.707106781186547,0.707106781186547,0.707106781186548,0.707106781186547,
0.707106781186548,0.707106781186547,0.707106781186548,0.707106781186547,
0.707106781186547,0.707106781186547,0.707106781186548,0.707106781186547,
0.707106781186548,0.707106781186547,0.707106781186548,0.707106781186547,
0.707106781186547,0.707106781186548,0.707106781186548,0.707106781186548,
0.707106781186547,0.707106781186548,0.707106781186547,0.707106781186548,
0.707106781186547,0.707106781186548,0.707106781186547,0.707106781186548,
0.707106781186548,0.707106781186547,0.707106781186547,0.707106781186547,
0.707106781186548,0.707106781186547,0.707106781186547,0.707106781186548,
0.707106781186547,0.707106781186547,0.707106781186548,0.707106781186547,
0.707106781186548,0.707106781186548,0.707106781186548,0.707106781186547,
0.707106781186548,0.707106781186547,0.707106781186548,0.707106781186547,
0.707106781186548,0.707106781186547,0.707106781186548,0.707106781186547,
0.707106781186548,0.707106781186547,0.707106781186548,0.707106781186548,
0.707106781186547,0.707106781186548,0.707106781186547,0.707106781186548,
0.707106781186548,0.707106781186547,0.707106781186547,0.707106781186548,
0.707106781186547,0.707106781186547,0.707106781186548,0.707106781186547,
0.707106781186548,0.707106781186548,0.707106781186547,0.707106781186548,
0.707106781186548,0.707106781186548,0.707106781186548,0.707106781186548,
0.707106781186547,0.707106781186548,0.707106781186548,0.707106781186548,
0.707106781186547,0.707106781186548,0.707106781186547,0.707106781186548,
0.707106781186547,0.707106781186548,0.707106781186547,0.707106781186548,
0.707106781186547,0.707106781186548,0.707106781186547,0.707106781186547,
0.707106781186548,0.707106781186547,0.707106781186547,0.707106781186548,
0.707106781186547,0.707106781186548,0.707106781186547,0.707106781186548,
0.707106781186547,0.707106781186548,0.707106781186547,0.707106781186547,
0.707106781186548,0.707106781186547,0.707106781186547,0.707106781186548,
0.707106781186547,0.707106781186548,0.707106781186547,0.707106781186547,
0.707106781186548,0.707106781186548,0.707106781186547,0.707106781186548,
0.707106781186547,0.707106781186547,0.707106781186547,0.707106781186548,
0.707106781186547,0.707106781186547,0.707106781186548,0.707106781186547,
0.707106781186547,0.707106781186547,0.707106781186548,0.707106781186548,
0.707106781186547,0.707106781186548,0.707106781186547,0.707106781186548,
0.707106781186547,0.707106781186547,0.707106781186548,0.707106781186547,
0.707106781186548,0.707106781186547,0.707106781186547,0.707106781186547,
0.707106781186547,0.707106781186548,0.707106781186547,0.707106781186547,
0.707106781186547,0.707106781186547,0.707106781186547,0.707106781186548,
0.707106781186547,0.707106781186547,0.707106781186547,0.707106781186547,
0.707106781186548,0.707106781186547,0.707106781186548,0.707106781186547,
0.707106781186547,0.707106781186548,0.707106781186547,0.707106781186548,
0.707106781186547,0.707106781186547,0.707106781186548,0.707106781186547,
0.707106781186547,0.707106781186548,0.707106781186547,0.707106781186547,
0.707106781186547,0.707106781186547,0.707106781186548,0.707106781186547,
0.707106781186548,0.707106781186548,0.707106781186547,0.707106781186548,
0.707106781186548,0.707106781186547,0.707106781186547,0.707106781186548,
0.707106781186547,0.707106781186547,0.707106781186547,0.707106781186548,
0.707106781186547,0.707106781186547,0.707106781186548,0.707106781186547,
0.707106781186548,0.707106781186547,0.707106781186548,0.707106781186547,
0.707106781186547,0.707106781186548,0.707106781186547,0.707106781186548,
0.707106781186547,0.707106781186548,0.707106781186547,0.707106781186548,
0.707106781186547,0.707106781186548,0.707106781186547,0.707106781186547,
0.707106781186547,0.707106781186547,0.707106781186548,0.707106781186548,
0.707106781186547,0.707106781186548,0.707106781186548,0.707106781186547,
0.707106781186548,0.707106781186547,0.707106781186547,0.707106781186548,
0.707106781186547,0.707106781186547,0.707106781186547,0.707106781186547,
0.707106781186548,0.707106781186547,0.707106781186547,0.707106781186547,
0.707106781186548,0.707106781186547,0.707106781186547,0.707106781186548,
0.707106781186547,0.707106781186548,0.707106781186548,0.707106781186547,
0.707106781186548,0.707106781186547,0.707106781186548,0.707106781186547,
0.707106781186548,0.707106781186547,0.707106781186547,0.707106781186548,
0.707106781186547,0.707106781186548,0.707106781186548,0.707106781186547,
0.707106781186547,0.707106781186548,0.707106781186547,0.707106781186548,
0.707106781186547,0.707106781186548,0.707106781186547,0.707106781186547,
0.707106781186548,0.707106781186548,0.707106781186547,0.707106781186548,
0.707106781186548,0.707106781186547,0.707106781186548,0.707106781186548,
0.707106781186547,0.707106781186548,0.707106781186547,0.707106781186548,
0.707106781186547,0.707106781186548,0.707106781186547,0.707106781186548,
0.707106781186547,0.707106781186547,0.707106781186548,0.707106781186547,
0.707106781186547,0.707106781186548,0.707106781186547,0.707106781186548,
0.707106781186548,0.707106781186547,0.707106781186547,0.707106781186547,
0.707106781186548,0.707106781186547,0.707106781186548,0.707106781186548,
0.707106781186547,0.707106781186548,0.707106781186547,0.707106781186548,
0.707106781186547,0.707106781186548,0.707106781186547,0.707106781186547,
0.707106781186548,0.707106781186548,0.707106781186548,0.707106781186547,
0.707106781186548,0.707106781186548,0.707106781186547,0.707106781186548,
0.707106781186547,0.707106781186548,0.707106781186548,0.707106781186548,
0.707106781186548,0.707106781186548,0.707106781186548,0.707106781186547,
0.707106781186547,0.707106781186548,0.707106781186547,0.707106781186547,
0.707106781186548,0.707106781186547,0.707106781186547,0.707106781186548,
0.707106781186547,0.707106781186548,0.707106781186547,0.707106781186548,
0.707106781186547,0.707106781186547,0.707106781186547,0.707106781186548,
0.707106781186547,0.707106781186547,0.707106781186548,0.707106781186547,
0.707106781186548,0.707106781186547,0.707106781186548,0.707106781186547,
0.707106781186547,0.707106781186547,0.707106781186547,0.707106781186548,
0.707106781186547,0.707106781186547,0.707106781186548,0.707106781186548,
0.707106781186547,0.707106781186548,0.707106781186547,0.707106781186548,
0.707106781186547,0.707106781186547,0.707106781186548,0.707106781186547,
0.707106781186548,0.707106781186547,0.707106781186548,0.707106781186547,
0.707106781186548,0.707106781186548,0.707106781186547,0.707106781186548,
0.707106781186547,0.707106781186547,0.707106781186548,0.707106781186547,
0.707106781186547,0.707106781186548,0.707106781186548,0.707106781186548,
0.707106781186547,0.707106781186548,0.707106781186547,0.707106781186547,
0.707106781186547,0.707106781186548,0.707106781186547,0.707106781186548,
0.707106781186548,0.707106781186548,0.707106781186547,0.707106781186547,
0.707106781186547,0.707106781186547,0.707106781186548,0.707106781186547,
0.707106781186547,0.707106781186548,0.707106781186547,0.707106781186548,
0.707106781186547,0.707106781186547,0.707106781186548,0.707106781186547,
0.707106781186548,0.707106781186547,0.707106781186548,0.707106781186547,
0.707106781186547,0.707106781186547,0.707106781186547,0.707106781186547,
0.707106781186547,0.707106781186548,0.707106781186547,0.707106781186547,
0.707106781186548,0.707106781186548,0.707106781186547,0.707106781186548,
0.707106781186548,0.707106781186547,0.707106781186547,0.707106781186548,
0.707106781186547,0.707106781186547,0.707106781186548,0.707106781186547,
0.707106781186548,0.707106781186548,0.707106781186548,0.707106781186547,
0.707106781186547,0.707106781186547,0.707106781186547,0.707106781186548,
0.707106781186548,0.707106781186548,0.707106781186547,0.707106781186548,
0.707106781186547,0.707106781186548,0.707106781186548,0.707106781186547,
0.707106781186548,0.707106781186547,0.707106781186548,0.707106781186548,
0.707106781186547,0.707106781186547,0.707106781186548,0.707106781186547,
0.707106781186548,0.707106781186547,0.707106781186548,0.707106781186548,
0.707106781186548,0.707106781186547,0.707106781186548,0.707106781186547,
0.707106781186547,0.707106781186547,0.707106781186547,0.707106781186548,
0.707106781186548,0.707106781186547,0.707106781186547,0.707106781186547,
0.707106781186548,0.707106781186547,0.707106781186547,0.707106781186548,
0.707106781186547,0.707106781186548,0.707106781186548,0.707106781186548,
0.707106781186547,0.707106781186547,0.707106781186547,0.707106781186547,
0.707106781186548,0.707106781186548,0.707106781186547,0.707106781186548,
0.707106781186547,0.707106781186548,0.707106781186548,0.707106781186547,
0.707106781186548,0.707106781186547,0.707106781186548,0.707106781186547,
0.707106781186547,0.707106781186547,0.707106781186548,0.707106781186547,
0.707106781186548,0.707106781186547,0.707106781186548,0.707106781186547,
0.707106781186548,0.707106781186547,0.707106781186548,0.707106781186547,
0.707106781186547,0.707106781186548,0.707106781186547,0.707106781186548,
0.707106781186547,0.707106781186547,0.707106781186548,0.707106781186548,
0.707106781186547,0.707106781186548,0.707106781186548,0.707106781186547,
0.707106781186548,0.707106781186547,0.707106781186548,0.707106781186547,
0.707106781186547,0.707106781186547,0.707106781186548,0.707106781186547,
0.707106781186547,0.707106781186548,0.707106781186547,0.707106781186548,
0.707106781186547,0.707106781186548,0.707106781186548,0.707106781186547,
0.707106781186548,0.707106781186547,0.707106781186548,0.707106781186548,
0.707106781186548,0.707106781186548,0.707106781186547,0.707106781186547,
0.707106781186548,0.707106781186547,0.707106781186547,0.707106781186548,
0.707106781186548,0.707106781186547,0.707106781186547,0.707106781186548,
0.707106781186547,0.707106781186547,0.707106781186548,0.707106781186547,
0.707106781186548,0.707106781186547,0.707106781186548,0.707106781186547,
0.707106781186547,0.707106781186547,0.707106781186548,0.707106781186547,
0.707106781186547,0.707106781186548,0.707106781186547,0.707106781186548,
0.707106781186548,0.707106781186548,0.707106781186547,0.707106781186547,
0.707106781186547,0.707106781186548,0.707106781186548,0.707106781186547,
0.707106781186547,0.707106781186547,0.707106781186547,0.707106781186548,
0.707106781186548,0.707106781186547,0.707106781186547,0.707106781186547,
0.707106781186548,0.707106781186548,0.707106781186547,0.707106781186548,
0.707106781186547,0.707106781186548,0.707106781186547,0.707106781186548,
0.707106781186548,0.707106781186547,0.707106781186548,0.707106781186548,
0.707106781186548,0.707106781186547,0.707106781186547,0.707106781186547,
0.707106781186548,0.707106781186548,0.707106781186548,0.707106781186547,
0.707106781186547,0.707106781186548,0.707106781186548,0.707106781186547,
0.707106781186548,0.707106781186547,0.707106781186547,0.707106781186548,
0.707106781186547,0.707106781186548,0.707106781186547,0.707106781186547,
0.707106781186548,0.707106781186547,0.707106781186548,0.707106781186548,
0.707106781186547,0.707106781186547,0.707106781186548,0.707106781186547,
0.707106781186548,0.707106781186547,0.707106781186547,0.707106781186548,
0.707106781186547,0.707106781186548,0.707106781186547,0.707106781186548,
0.707106781186547,0.707106781186547,0.707106781186548,0.707106781186547,
0.707106781186547,0.707106781186547,0.707106781186547,0.707106781186547,
0.707106781186547,0.707106781186548,0.707106781186547,0.707106781186548,
0.707106781186548,0.707106781186548,0.707106781186547,0.707106781186547,
0.707106781186547,0.707106781186548,0.707106781186547,0.707106781186548,
0.707106781186547,0.707106781186547,0.707106781186548,0.707106781186547,
0.707106781186547,0.707106781186547,0.707106781186547,0.707106781186547,
0.707106781186548,0.707106781186547,0.707106781186548,0.707106781186547,
0.707106781186547,0.707106781186548,0.707106781186548,0.707106781186547,
0.707106781186547,0.707106781186547,0.707106781186548,0.707106781186547,
0.707106781186547,0.707106781186548,0.707106781186548,0.707106781186547,
0.707106781186548,0.707106781186547,0.707106781186548,0.707106781186548,
0.707106781186547,0.707106781186547,0.707106781186547,0.707106781186548,
0.707106781186548,0.707106781186547,0.707106781186548,0.707106781186547,
0.707106781186548,0.707106781186548,0.707106781186547,0.707106781186548,
0.707106781186547,0.707106781186547,0.707106781186547,0.707106781186548,
0.707106781186547,0.707106781186548,0.707106781186547,0.707106781186548,
0.707106781186547,0.707106781186547,0.707106781186547,0.707106781186547,
0.707106781186547,0.707106781186548,0.707106781186547,0.707106781186548,
0.707106781186547,0.707106781186548,0.707106781186547,0.707106781186548,
0.707106781186547,0.707106781186547,0.707106781186547,0.707106781186547,
0.707106781186547,0.707106781186548,0.707106781186548,0.707106781186548,
0.707106781186547,0.707106781186548,0.707106781186547,0.707106781186548,
0.707106781186547,0.707106781186547,0.707106781186548,0.707106781186547,
0.707106781186548,0.707106781186547,0.707106781186547,0.707106781186547,
0.707106781186548,0.707106781186548,0.707106781186547,0.707106781186548,
0.707106781186547,0.707106781186548,0.707106781186548,0.707106781186547,
0.707106781186548,0.707106781186547,0.707106781186548,0.707106781186548,
0.707106781186547,0.707106781186547,0.707106781186547,0.707106781186547,
0.707106781186547,0.707106781186547,0.707106781186548,0.707106781186548,
0.707106781186547,0.707106781186548,0.707106781186547,0.707106781186547,
0.707106781186548,0.707106781186547,0.707106781186547,0.707106781186548,
0.707106781186547,0.707106781186547,0.707106781186547,0.707106781186548,
0.707106781186547,0.707106781186547,0.707106781186548,0.707106781186547,
0.707106781186548,0.707106781186548,0.707106781186547,0.707106781186547,
0.707106781186547,0.707106781186548,0.707106781186547,0.707106781186547,
0.707106781186548,0.707106781186548,0.707106781186548,0.707106781186548,
0.707106781186547,0.707106781186548,0.707106781186548,0.707106781186547,
0.707106781186547,0.707106781186548,0.707106781186547,0.707106781186548,
0.707106781186547,0.707106781186547,0.707106781186548,0.707106781186547,
0.707106781186547,0.707106781186548,0.707106781186547,0.707106781186548,
0.707106781186547,0.707106781186548,0.707106781186547,0.707106781186548,
0.707106781186547,0.707106781186548,0.707106781186547,0.707106781186548,
0.707106781186548,0.707106781186547,0.707106781186547,0.707106781186548,
0.707106781186548,0.707106781186547,0.707106781186547,0.707106781186547,
0.707106781186547,0.707106781186547,0.707106781186548,0.707106781186547,
0.707106781186547,0.707106781186548,0.707106781186547,0.707106781186548,
0.707106781186548,0.707106781186547,0.707106781186548,0.707106781186547,
0.707106781186548,0.707106781186547,0.707106781186548,0.707106781186547,
0.707106781186547,0.707106781186547,0.707106781186547,0.707106781186547,
0.707106781186547,0.707106781186548,0.707106781186547,0.707106781186548,
0.707106781186547,0.707106781186547,0.707106781186547,0.707106781186548,
0.707106781186547,0.707106781186548,0.707106781186548,0.707106781186547,
0.707106781186547,0.707106781186548,0.707106781186547,0.707106781186548,
0.707106781186547,0.707106781186548,0.707106781186547,0.707106781186548,
0.707106781186547,0.707106781186547,0.707106781186548,0.707106781186547,
0.707106781186548,0.707106781186547,0.707106781186548,0.707106781186548,
0.707106781186548,0.707106781186548,0.707106781186547,0.707106781186548,
0.707106781186548,0.707106781186548,0.707106781186547,0.707106781186548,
0.707106781186548,0.707106781186547,0.707106781186548,0.707106781186547,
0.707106781186548,0.707106781186547,0.707106781186547,0.707106781186547,
0.707106781186548,0.707106781186548,0.707106781186547,0.707106781186548,
0.707106781186547,0.707106781186548,0.707106781186547,0.707106781186548,
0.707106781186548,0.707106781186547,0.707106781186548,0.707106781186547,
0.707106781186547,0.707106781186548,0.707106781186547,0.707106781186547,
0.707106781186547,0.707106781186548,0.707106781186547,0.707106781186548,
0.707106781186548,0.707106781186547,0.707106781186548,0.707106781186547,
0.707106781186548,0.707106781186548,0.707106781186548,0.707106781186548,
0.707106781186547,0.707106781186548,0.707106781186547,0.707106781186548,
0.707106781186547,0.707106781186548,0.707106781186547,0.707106781186547,
0.707106781186547,0.707106781186547,0.707106781186548,0.707106781186547,
0.707106781186548,0.707106781186547,0.707106781186547,0.707106781186548,
0.707106781186547,0.707106781186548,0.707106781186547,0.707106781186548,
0.707106781186547,0.707106781186548,0.707106781186548,0.707106781186548,
0.707106781186548,0.707106781186547,0.707106781186548,0.707106781186548,
0.707106781186547,0.707106781186548,0.707106781186547,0.707106781186548,
0.707106781186547,0.707106781186548,0.707106781186547,0.707106781186547,
0.707106781186548,0.707106781186547,0.707106781186548,0.707106781186547,
0.707106781186547,0.707106781186548,0.707106781186547,0.707106781186548,
0.707106781186547,0.707106781186547,0.707106781186548,0.707106781186548,
0.707106781186548,0.707106781186548,0.707106781186548,0.707106781186548,
0.707106781186548,0.707106781186548,0.707106781186548,0.707106781186547,
0.707106781186548,0.707106781186547,0.707106781186547,0.707106781186548,
0.707106781186547,0.707106781186548,0.707106781186548,0.707106781186547,
0.707106781186547,0.707106781186548,0.707106781186548,0.707106781186547,
0.707106781186547,0.707106781186547,0.707106781186547,0.707106781186547,
0.707106781186548,0.707106781186547,0.707106781186548,0.707106781186548,
0.707106781186548,0.707106781186547,0.707106781186548,0.707106781186547,
0.707106781186548,0.707106781186547,0.707106781186548,0.707106781186547,
0.707106781186548,0.707106781186548,0.707106781186547,0.707106781186547,
0.707106781186548,0.707106781186548,0.707106781186548,0.707106781186547,
0.707106781186547,0.707106781186548,0.707106781186547,0.707106781186547,
0.707106781186548,0.707106781186547,0.707106781186548,0.707106781186547,
0.707106781186547,0.707106781186548,0.707106781186548,0.707106781186548,
0.707106781186547,0.707106781186547,0.707106781186548,0.707106781186547,
0.707106781186548,0.707106781186547,0.707106781186548,0.707106781186547,
0.707106781186548,0.707106781186548,0.707106781186547,0.707106781186548,
0.707106781186547,0.707106781186548,0.707106781186547,0.707106781186547,
0.707106781186547,0.707106781186548,0.707106781186547,0.707106781186548,
0.707106781186547,0.707106781186547,0.707106781186547,0.707106781186548,
0.707106781186547,0.707106781186547,0.707106781186548,0.707106781186548,
0.707106781186547,0.707106781186548,0.707106781186547,0.707106781186548,
0.707106781186548,0.707106781186547,0.707106781186548,0.707106781186547,
0.707106781186547,0.707106781186548,0.707106781186547,0.707106781186547,
0.707106781186547,0.707106781186548,0.707106781186547,0.707106781186548,
0.707106781186547,0.707106781186548,0.707106781186548,0.707106781186548,
0.707106781186547,0.707106781186548,0.707106781186548,0.707106781186548,
0.707106781186547,0.707106781186548,0.707106781186547,0.707106781186547,
0.707106781186548,0.707106781186547,0.707106781186547,0.707106781186548,
0.707106781186548,0.707106781186547,0.707106781186548,0.707106781186547,
0.707106781186548,0.707106781186548,0.707106781186547,0.707106781186548,
0.707106781186547,0.707106781186548,0.707106781186547,0.707106781186548,
0.707106781186547,0.707106781186548,0.707106781186548,0.707106781186548,
0.707106781186547,0.707106781186548,0.707106781186548,0.707106781186547,
0.707106781186547,0.707106781186548,0.707106781186547,0.707106781186548,
0.707106781186548,0.707106781186547,0.707106781186548,0.707106781186548,
0.707106781186547,0.707106781186548,0.707106781186548,0.707106781186547,
0.707106781186547,0.707106781186548,0.707106781186547,0.707106781186548,
0.707106781186547,0.707106781186548,0.707106781186547,0.707106781186548,
0.707106781186548,0.707106781186548,0.707106781186547,0.707106781186548,
0.707106781186547,0.707106781186548,0.707106781186547,0.707106781186548,
0.707106781186547,0.707106781186548,0.707106781186547,0.707106781186548,
0.707106781186547,0.707106781186548,0.707106781186547,0.707106781186547,
0.707106781186547,0.707106781186548,0.707106781186547,0.707106781186548,
0.707106781186547,0.707106781186548,0.707106781186547,0.707106781186548,
0.707106781186547,0.707106781186548,0.707106781186548,0.707106781186548,
0.707106781186547,0.707106781186548,0.707106781186547,0.707106781186548,
0.707106781186548,0.707106781186547,0.707106781186548,0.707106781186547,
0.707106781186548,0.707106781186547,0.707106781186548,0.707106781186547,
0.707106781186548,0.707106781186547,0.707106781186547,0.707106781186547,
0.707106781186548,0.707106781186547,0.707106781186547,0.707106781186548,
0.707106781186547,0.707106781186548,0.707106781186547,0.707106781186547,
0.707106781186548,0.707106781186547,0.707106781186548,0.707106781186547,
0.707106781186548,0.707106781186548,0.707106781186548,0.707106781186547,
0.707106781186547,0.707106781186548,0.707106781186548,0.707106781186547,
0.707106781186548,0.707106781186547,0.707106781186547,0.707106781186547,
0.707106781186548,0.707106781186547,0.707106781186548,0.707106781186547,
0.707106781186548,0.707106781186548,0.707106781186548,0.707106781186547,
0.707106781186547,0.707106781186547,0.707106781186547,0.707106781186547,
0.707106781186547,0.707106781186548,0.707106781186547,0.707106781186548,
0.707106781186547,0.707106781186548,0.707106781186547,0.707106781186547,
0.707106781186548,0.707106781186547,0.707106781186547,0.707106781186548,
0.707106781186548,0.707106781186547,0.707106781186547,0.707106781186547,
0.707106781186548,0.707106781186547,0.707106781186547,0.707106781186548,
0.707106781186548),(1.,1.,1.,1.,1.,1.,1.,1.,1.,1.,1.,1.,1.,1.,1.,1.,1.,
1.,1.,1.,1.,1.,1.,1.,1.,1.,1.,1.,1.,1.,1.,1.,1.,1.,1.,1.,1.,1.,1.,1.,1.,
1.,1.,1.,1.,1.,1.,1.,1.,1.,1.,1.,1.,1.,1.,1.,1.,1.,1.,1.,1.,1.,1.,1.,1.,
1.,1.,1.,1.,1.,1.,1.,1.,1.,1.,1.,1.,1.,1.,1.,1.,1.,1.,1.,1.,1.,1.,1.,1.,
1.,1.,1.,1.,1.,1.,1.,1.,1.,1.,1.,1.,1.,1.,1.,1.,1.,1.,1.,1.,1.,1.,1.,1.,
1.,1.,1.,1.,1.,1.,1.,1.,1.,1.,1.,1.,1.,1.,1.,1.,1.,1.,1.,1.,1.,1.,1.,1.,
1.,1.,1.,1.,1.,1.,1.,1.,1.,1.,1.,1.,1.,1.,1.,1.,1.,1.,1.,1.,1.,1.,1.,1.,
1.,1.,1.,1.,1.,1.,1.,1.,1.,1.,1.,1.,1.,1.,1.,1.,1.,1.,1.,1.,1.,1.,1.,1.,
1.,1.,1.,1.,1.,1.,1.,1.,1.,1.,1.,1.,1.,1.,1.,1.,1.,1.,1.,1.,1.,1.,1.,1.,
1.,1.,1.,1.,1.,1.,1.,1.,1.,1.,1.,1.,1.,1.,1.,1.,1.,1.,1.,1.,1.,1.,1.,1.,
1.,1.,1.,1.,1.,1.,1.,1.,1.,1.,1.,1.,1.,1.,1.,1.,1.,1.,1.,1.,1.,1.,1.,1.,
1.,1.,1.,1.,1.,1.,1.,1.,1.,1.,1.,1.,1.,1.,1.,1.,1.,1.,1.,1.,1.,1.,1.,1.,
1.,1.,1.,1.,1.,1.,1.,1.,1.,1.,1.,1.,1.,1.,1.,1.,1.,1.,1.,1.,1.,1.,1.,1.,
1.,1.,1.,1.,1.,1.,1.,1.,1.,1.,1.,1.,1.,1.,1.,1.,1.,1.,1.,1.,1.,1.,1.,1.,
1.,1.,1.,1.,1.,1.,1.,1.,1.,1.,1.,1.,1.,1.,1.,1.,1.,1.,1.,1.,1.,1.,1.,1.,
1.,1.,1.,1.,1.,1.,1.,1.,1.,1.,1.,1.,1.,1.,1.,1.,1.,1.,1.,1.,1.,1.,1.,1.,
1.,1.,1.,1.,1.,1.,1.,1.,1.,1.,1.,1.,1.,1.,1.,1.,1.,1.,1.,1.,1.,1.,1.,1.,
1.,1.,1.,1.,1.,1.,1.,1.,1.,1.,1.,1.,1.,1.,1.,1.,1.,1.,1.,1.,1.,1.,1.,1.,
1.,1.,1.,1.,1.,1.,1.,1.,1.,1.,1.,1.,1.,1.,1.,1.,1.,1.,1.,1.,1.,1.,1.,1.,
1.,1.,1.,1.,1.,1.,1.,1.,1.,1.,1.,1.,1.,1.,1.,1.,1.,1.,1.,1.,1.,1.,1.,1.,
1.,1.,1.,1.,1.,1.,1.,1.,1.,1.,1.,1.,1.,1.,1.,1.,1.,1.,1.,1.,1.,1.,1.,1.,
1.,1.,1.,1.,1.,1.,1.,1.,1.,1.,1.,1.,1.,1.,1.,1.,1.,1.,1.,1.,1.,1.,1.,1.,
1.,1.,1.,1.,1.,1.,1.,1.,1.,1.,1.,1.,1.,1.,1.,1.,1.,1.,1.,1.,1.,1.,1.,1.,
1.,1.,1.,1.,1.,1.,1.,1.,1.,1.,1.,1.,1.,1.,1.,1.,1.,1.,1.,1.,1.,1.,1.,1.,
1.,1.,1.,1.,1.,1.,1.,1.,1.,1.,1.,1.,1.,1.,1.,1.,1.,1.,1.,1.,1.,1.,1.,1.,
1.,1.,1.,1.,1.,1.,1.,1.,1.,1.,1.,1.,1.,1.,1.,1.,1.,1.,1.,1.,1.,1.,1.,1.,
1.,1.,1.,1.,1.,1.,1.,1.,1.,1.,1.,1.,1.,1.,1.,1.,1.,1.,1.,1.,1.,1.,1.,1.,
1.,1.,1.,1.,1.,1.,1.,1.,1.,1.,1.,1.,1.,1.,1.,1.,1.,1.,1.,1.,1.,1.,1.,1.,
1.,1.,1.,1.,1.,1.,1.,1.,1.,1.,1.,1.,1.,1.,1.,1.,1.,1.,1.,1.,1.,1.,1.,1.,
1.,1.,1.,1.,1.,1.,1.,1.,1.,1.,1.,1.,1.,1.,1.,1.,1.,1.,1.,1.,1.,1.,1.,1.,
1.,1.,1.,1.,1.,1.,1.,1.,1.,1.,1.,1.,1.,1.,1.,1.,1.,1.,1.,1.,1.,1.,1.,1.,
1.,1.,1.,1.,1.,1.,1.,1.,1.,1.,1.,1.,1.,1.,1.,1.,1.,1.,1.,1.,1.,1.,1.,1.,
1.,1.,1.,1.,1.,1.,1.,1.,1.,1.,1.,1.,1.,1.,1.,1.,1.,1.,1.,1.,1.,1.,1.,1.,
1.,1.,1.,1.,1.,1.,1.,1.,1.,1.,1.,1.,1.,1.,1.,1.,1.,1.,1.,1.,1.,1.,1.,1.,
1.,1.,1.,1.,1.,1.,1.,1.,1.,1.,1.,1.,1.,1.,1.,1.,1.,1.,1.,1.,1.,1.,1.,1.,
1.,1.,1.,1.,1.,1.,1.,1.,1.,1.,1.,1.,1.,1.,1.,1.,1.,1.,1.,1.,1.,1.,1.,1.,
1.,1.,1.,1.,1.,1.,1.,1.,1.,1.,1.,1.,1.,1.,1.,1.,1.,1.,1.,1.,1.,1.,1.,1.,
1.,1.,1.,1.,1.,1.,1.,1.,1.,1.,1.,1.,1.,1.,1.,1.,1.,1.,1.,1.,1.,1.,1.,1.,
1.,1.,1.,1.,1.,1.,1.,1.,1.,1.,1.,1.,1.,1.,1.,1.,1.,1.,1.,1.,1.,1.,1.,1.,
1.,1.,1.,1.,1.,1.,1.,1.,1.,1.,1.,1.,1.,1.,1.,1.,1.,1.,1.,1.,1.,1.,1.,1.,
1.,1.,1.,1.,1.,1.,1.,1.,1.,1.,1.,1.,1.,1.,1.,1.,1.,1.,1.,1.,1.,1.,1.,1.,
1.,1.,1.,1.,1.,1.,1.,1.,1.,1.,1.,1.,1.,1.,1.,1.,1.,1.,1.,1.,1.,1.,1.,1.,
1.,1.,1.,1.,1.,1.,1.,1.,1.,1.,1.,1.,1.,1.,1.,1.,1.,1.,1.,1.,1.,1.,1.,1.,
1.,1.,1.,1.,1.,1.,1.,1.,1.,1.,1.,1.,1.,1.,1.,1.,1.,1.,1.,1.,1.,1.,1.,1.,
1.,1.,1.,1.,1.,1.,1.,1.,1.,1.,1.,1.,1.,1.,1.,1.,1.,1.,1.,1.,1.,1.,1.,1.,
1.,1.,1.,1.,1.,1.,1.,1.,1.,1.,1.,1.,1.,1.,1.,1.,1.,1.,1.,1.,1.,1.,1.,1.,
1.,1.,1.,1.,1.,1.,1.,1.,1.,1.,1.,1.,1.,1.,1.,1.,1.,1.,1.,1.,1.,1.,1.,1.,
1.,1.,1.,1.,1.,1.,1.,1.,1.,1.,1.,1.,1.,1.,1.,1.,1.,1.,1.,1.,1.,1.,1.,1.,
1.,1.,1.,1.,1.,1.,1.,1.,1.,1.,1.,1.,1.,1.,1.,1.,1.,1.,1.,1.,1.,1.,1.,1.,
1.,1.,1.,1.,1.,1.,1.,1.,1.,1.,1.,1.,1.,1.,1.,1.,1.,1.,1.,1.,1.,1.,1.,1.,
1.,1.,1.,1.,1.,1.,1.,1.,1.,1.,1.,1.,1.,1.,1.,1.,1.,1.,1.,1.,1.,1.,1.,1.,
1.,1.,1.,1.,1.,1.,1.,1.,1.,1.,1.,1.,1.,1.,1.,1.,1.,1.,1.,1.,1.,1.,1.,1.,
1.,1.,1.,1.,1.,1.,1.,1.,1.,1.,1.,1.,1.,1.,1.,1.,1.,1.,1.,1.,1.,1.,1.,1.,
1.,1.,1.,1.,1.,1.,1.,1.,1.,1.,1.,1.,1.,1.,1.,1.,1.,1.,1.,1.,1.,1.,1.,1.,
1.,1.,1.,1.,1.,1.,1.,1.,1.,1.,1.,1.,1.,1.,1.,1.,1.,1.,1.,1.,1.,1.,1.,1.,
1.,1.,1.,1.,1.,1.,1.,1.,1.,1.,1.,1.,1.,1.,1.,1.,1.,1.,1.,1.,1.,1.,1.,1.,
1.,1.,1.,1.,1.,1.,1.,1.,1.,1.,1.,1.,1.,1.,1.,1.,1.,1.,1.,1.,1.,1.,1.,1.,
1.,1.,1.,1.,1.,1.,1.,1.,1.,1.,1.,1.,1.,1.,1.,1.,1.,1.,1.,1.,1.,1.,1.,1.,
1.,1.,1.,1.,1.,1.,1.,1.,1.,1.,1.,1.,1.,1.,1.,1.,1.,1.,1.,1.,1.,1.,1.,1.,
1.,1.,1.,1.,1.,1.,1.,1.,1.,1.,1.,1.,1.,1.,1.,1.,1.,1.,1.,1.,1.,1.,1.,1.,
1.,1.,1.,1.,1.,1.,1.,1.,1.,1.,1.,1.,1.,1.,1.,1.,1.,1.,1.,1.,1.,1.,1.,1.,
1.,1.,1.,1.,1.,1.,1.,1.,1.,1.,1.,1.,1.,1.,1.,1.,1.,1.,1.,1.,1.,1.,1.,1.,
1.,1.,1.,1.,1.,1.,1.,1.,1.,1.,1.,1.,1.,1.,1.,1.,1.,1.,1.,1.,1.,1.,1.,1.,
1.,1.,1.,1.,1.,1.,1.,1.,1.,1.,1.,1.,1.,1.,1.,1.,1.,1.,1.,1.,1.,1.,1.,1.,
1.,1.,1.,1.,1.,1.,1.,1.,1.,1.,1.,1.,1.,1.,1.,1.,1.,1.,1.,1.,1.,1.,1.,1.,
1.,1.,1.,1.,1.,1.,1.,1.,1.,1.,1.,1.,1.,1.,1.,1.,1.,1.,1.,1.,1.,1.,1.,1.,
1.,1.,1.,1.,1.,1.,1.,1.,1.,1.,1.,1.,1.,1.,1.,1.,1.,1.,1.,1.,1.,1.,1.,1.,
1.,1.,1.,1.,1.,1.,1.,1.,1.,1.,1.,1.,1.,1.,1.,1.,1.,1.,1.,1.,1.,1.,1.,1.,
1.,1.,1.,1.,1.,1.,1.,1.,1.,1.,1.,1.,1.,1.,1.,1.,1.,1.,1.,1.,1.,1.,1.,1.,
1.,1.,1.,1.,1.,1.,1.,1.,1.,1.,1.,1.,1.,1.,1.,1.,1.,1.,1.,1.,1.,1.,1.,1.,
1.,1.,1.,1.,1.,1.,1.,1.,1.,1.,1.,1.,1.,1.,1.,1.,1.,1.,1.,1.,1.,1.,1.,1.,
1.,1.,1.,1.,1.,1.,1.,1.,1.,1.,1.,1.,1.,1.,1.,1.,1.,1.,1.,1.,1.,1.,1.,1.,
1.,1.,1.,1.,1.,1.,1.,1.,1.,1.,1.,1.,1.,1.,1.,1.,1.,1.,1.,1.,1.,1.,1.,1.,
1.,1.,1.,1.,1.,1.,1.,1.,1.,1.,1.,1.,1.,1.,1.,1.,1.,1.,1.,1.,1.,1.,1.,1.,
1.,1.,1.,1.,1.,1.,1.,1.,1.,1.,1.,1.,1.,1.,1.,1.,1.,1.,1.,1.,1.,1.,1.,1.,
1.,1.,1.,1.,1.,1.,1.,1.,1.,1.,1.,1.,1.,1.,1.,1.,1.,1.,1.,1.,1.,1.,1.,1.,
1.,1.,1.,1.,1.,1.,1.,1.,1.,1.,1.,1.,1.,1.,1.,1.,1.,1.,1.,1.,1.,1.,1.,1.,
1.,1.,1.,1.,1.,1.,1.,1.,1.,1.,1.,1.,1.,1.,1.,1.,1.,1.,1.,1.,1.,1.,1.,1.,
1.,1.,1.,1.,1.,1.,1.,1.,1.,1.,1.,1.,1.,1.,1.,1.,1.,1.,1.,1.,1.,1.,1.,1.,
1.,1.,1.,1.,1.,1.,1.,1.,1.,1.,1.,1.,1.,1.,1.,1.,1.,1.,1.,1.,1.,1.,1.,1.,
1.,1.,1.,1.,1.,1.,1.,1.,1.,1.,1.,1.,1.,1.,1.,1.,1.,1.,1.,1.,1.,1.,1.,1.,
1.,1.,1.,1.,1.,1.,1.,1.,1.,1.,1.,1.,1.,1.,1.,1.,1.,1.,1.,1.,1.,1.,1.,1.,
1.,1.,1.,1.,1.,1.,1.,1.,1.,1.,1.,1.,1.,1.,1.,1.,1.,1.,1.,1.,1.,1.,1.,1.,
1.,1.,1.,1.,1.,1.,1.,1.,1.,1.,1.,1.,1.,1.,1.,1.,1.,1.,1.,1.,1.,1.,1.,1.,
1.,1.,1.,1.,1.,1.,1.,1.,1.,1.,1.,1.,1.,1.,1.,1.,1.,1.,1.,1.,1.,1.,1.,1.,
1.,1.,1.,1.,1.,1.,1.,1.,1.,1.,1.,1.,1.,1.,1.,1.,1.,1.)))
REPRESENTATION_ITEM('')
SURFACE()
) ;
#48=(
BOUNDED_SURFACE()
B_SPLINE_SURFACE(3,2,((#154048,#154049,#154050,#154051,#154052,#154053,
#154054,#154055,#154056),(#154057,#154058,#154059,#154060,#154061,#154062,
#154063,#154064,#154065),(#154066,#154067,#154068,#154069,#154070,#154071,
#154072,#154073,#154074),(#154075,#154076,#154077,#154078,#154079,#154080,
#154081,#154082,#154083),(#154084,#154085,#154086,#154087,#154088,#154089,
#154090,#154091,#154092),(#154093,#154094,#154095,#154096,#154097,#154098,
#154099,#154100,#154101),(#154102,#154103,#154104,#154105,#154106,#154107,
#154108,#154109,#154110)),.UNSPECIFIED.,.F.,.T.,.F.)
B_SPLINE_SURFACE_WITH_KNOTS((4,1,1,1,4),(3,2,2,2,3),(0.,0.0911446219616379,
0.182289243923276,0.273433865884915,0.364578487846551),(0.,0.117809724509617,
0.235619449019234,0.353429173528852,0.471238898038469),.UNSPECIFIED.)
GEOMETRIC_REPRESENTATION_ITEM()
RATIONAL_B_SPLINE_SURFACE(((1.,0.707106781186548,1.,0.707106781186548,1.,
0.707106781186548,1.,0.707106781186548,1.),(1.,0.707106781186548,1.,0.707106781186548,
1.,0.707106781186548,1.,0.707106781186548,1.),(1.,0.707106781186547,1.,
0.707106781186547,1.,0.707106781186547,1.,0.707106781186547,1.),(1.,0.707106781186548,
1.,0.707106781186548,1.,0.707106781186548,1.,0.707106781186548,1.),(1.,
0.707106781186547,1.,0.707106781186547,1.,0.707106781186547,1.,0.707106781186547,
1.),(1.,0.707106781186548,1.,0.707106781186548,1.,0.707106781186548,1.,
0.707106781186548,1.),(1.,0.707106781186548,1.,0.707106781186548,1.,0.707106781186548,
1.,0.707106781186548,1.)))
REPRESENTATION_ITEM('')
SURFACE()
) ;
#49=(
BOUNDED_SURFACE()
B_SPLINE_SURFACE(3,2,((#154120,#154121,#154122,#154123,#154124,#154125,
#154126,#154127,#154128),(#154129,#154130,#154131,#154132,#154133,#154134,
#154135,#154136,#154137),(#154138,#154139,#154140,#154141,#154142,#154143,
#154144,#154145,#154146),(#154147,#154148,#154149,#154150,#154151,#154152,
#154153,#154154,#154155)),.UNSPECIFIED.,.F.,.T.,.F.)
B_SPLINE_SURFACE_WITH_KNOTS((4,4),(3,2,2,2,3),(0.,1.1454147408364),(0.,
0.117809724509617,0.235619449019234,0.353429173528852,0.471238898038469),
 .UNSPECIFIED.)
GEOMETRIC_REPRESENTATION_ITEM()
RATIONAL_B_SPLINE_SURFACE(((1.,0.707106781186548,1.,0.707106781186548,1.,
0.707106781186548,1.,0.707106781186548,1.),(1.,0.707106781186548,1.,0.707106781186548,
1.,0.707106781186548,1.,0.707106781186548,1.),(1.,0.707106781186547,1.,
0.707106781186547,1.,0.707106781186547,1.,0.707106781186547,1.),(1.,0.707106781186548,
1.,0.707106781186548,1.,0.707106781186548,1.,0.707106781186548,1.)))
REPRESENTATION_ITEM('')
SURFACE()
) ;
#50=(
BOUNDED_SURFACE()
B_SPLINE_SURFACE(3,2,((#154163,#154164,#154165,#154166,#154167,#154168,
#154169,#154170,#154171),(#154172,#154173,#154174,#154175,#154176,#154177,
#154178,#154179,#154180),(#154181,#154182,#154183,#154184,#154185,#154186,
#154187,#154188,#154189),(#154190,#154191,#154192,#154193,#154194,#154195,
#154196,#154197,#154198),(#154199,#154200,#154201,#154202,#154203,#154204,
#154205,#154206,#154207),(#154208,#154209,#154210,#154211,#154212,#154213,
#154214,#154215,#154216),(#154217,#154218,#154219,#154220,#154221,#154222,
#154223,#154224,#154225),(#154226,#154227,#154228,#154229,#154230,#154231,
#154232,#154233,#154234),(#154235,#154236,#154237,#154238,#154239,#154240,
#154241,#154242,#154243),(#154244,#154245,#154246,#154247,#154248,#154249,
#154250,#154251,#154252),(#154253,#154254,#154255,#154256,#154257,#154258,
#154259,#154260,#154261),(#154262,#154263,#154264,#154265,#154266,#154267,
#154268,#154269,#154270),(#154271,#154272,#154273,#154274,#154275,#154276,
#154277,#154278,#154279),(#154280,#154281,#154282,#154283,#154284,#154285,
#154286,#154287,#154288),(#154289,#154290,#154291,#154292,#154293,#154294,
#154295,#154296,#154297),(#154298,#154299,#154300,#154301,#154302,#154303,
#154304,#154305,#154306),(#154307,#154308,#154309,#154310,#154311,#154312,
#154313,#154314,#154315),(#154316,#154317,#154318,#154319,#154320,#154321,
#154322,#154323,#154324),(#154325,#154326,#154327,#154328,#154329,#154330,
#154331,#154332,#154333)),.UNSPECIFIED.,.F.,.T.,.F.)
B_SPLINE_SURFACE_WITH_KNOTS((4,1,1,1,1,1,1,1,1,1,1,1,1,1,1,1,4),(3,2,2,
2,3),(0.,0.226732296973331,0.464902013928651,0.70307173088397,0.9298040278573,
1.15653632483063,1.39470604178595,1.63287575874127,1.8596080557146,2.08634035268793,
2.32451006964325,2.56267978659857,2.7894120835719,3.01614438054523,3.25431409750055,
3.49248381445586,3.7192161114292),(0.,0.117809724509617,0.235619449019234,
0.353429173528852,0.471238898038469),.UNSPECIFIED.)
GEOMETRIC_REPRESENTATION_ITEM()
RATIONAL_B_SPLINE_SURFACE(((1.,0.707106781186548,1.,0.707106781186548,1.,
0.707106781186548,1.,0.707106781186548,1.),(1.,0.707106781186547,1.,0.707106781186547,
1.,0.707106781186547,1.,0.707106781186547,1.),(1.,0.707106781186548,1.,
0.707106781186548,1.,0.707106781186548,1.,0.707106781186548,1.),(1.,0.707106781186547,
1.,0.707106781186547,1.,0.707106781186547,1.,0.707106781186547,1.),(1.,
0.707106781186548,1.,0.707106781186548,1.,0.707106781186548,1.,0.707106781186548,
1.),(1.,0.707106781186547,1.,0.707106781186547,1.,0.707106781186547,1.,
0.707106781186547,1.),(1.,0.707106781186548,1.,0.707106781186548,1.,0.707106781186548,
1.,0.707106781186548,1.),(1.,0.707106781186547,1.,0.707106781186547,1.,
0.707106781186547,1.,0.707106781186547,1.),(1.,0.707106781186547,1.,0.707106781186547,
1.,0.707106781186547,1.,0.707106781186547,1.),(1.,0.707106781186547,1.,
0.707106781186547,1.,0.707106781186547,1.,0.707106781186547,1.),(1.,0.707106781186548,
1.,0.707106781186548,1.,0.707106781186548,1.,0.707106781186548,1.),(1.,
0.707106781186547,1.,0.707106781186547,1.,0.707106781186547,1.,0.707106781186547,
1.),(1.,0.707106781186547,1.,0.707106781186547,1.,0.707106781186547,1.,
0.707106781186547,1.),(1.,0.707106781186547,1.,0.707106781186547,1.,0.707106781186547,
1.,0.707106781186547,1.),(1.,0.707106781186547,1.,0.707106781186547,1.,
0.707106781186547,1.,0.707106781186547,1.),(1.,0.707106781186547,1.,0.707106781186547,
1.,0.707106781186547,1.,0.707106781186547,1.),(1.,0.707106781186548,1.,
0.707106781186548,1.,0.707106781186548,1.,0.707106781186548,1.),(1.,0.707106781186547,
1.,0.707106781186547,1.,0.707106781186547,1.,0.707106781186547,1.),(1.,
0.707106781186548,1.,0.707106781186548,1.,0.707106781186548,1.,0.707106781186548,
1.)))
REPRESENTATION_ITEM('')
SURFACE()
) ;
#149=ELLIPSE('',#8989,0.0751099188439569,0.0750000000000024) ;
#150=ELLIPSE('',#8990,0.0753270884818842,0.07500000000001) ;
#151=ELLIPSE('',#8991,0.0753270884818842,0.07500000000001) ;
#152=ELLIPSE('',#8992,0.0753270884818842,0.07500000000001) ;
#153=ELLIPSE('',#8993,0.0752842013001122,0.0750000000000016) ;
#154=ELLIPSE('',#8994,0.0752842013001065,0.0750000000000022) ;
#155=ELLIPSE('',#8995,0.0752842013001065,0.0750000000000022) ;
#156=ELLIPSE('',#8996,0.0752842013001065,0.0750000000000022) ;
#157=ELLIPSE('',#8998,0.0751099188439449,0.0750000000000012) ;
#158=ELLIPSE('',#8999,0.0753270884818742,0.07500000000003) ;
#159=ELLIPSE('',#9000,0.0753270884818742,0.07500000000003) ;
#160=ELLIPSE('',#9001,0.0753270884818742,0.07500000000003) ;
#161=ELLIPSE('',#9002,0.0752842013001133,0.0749999999999984) ;
#162=ELLIPSE('',#9003,0.0752842013001184,0.074999999999999) ;
#163=ELLIPSE('',#9004,0.0752842013001184,0.074999999999999) ;
#164=ELLIPSE('',#9005,0.0752842013001184,0.074999999999999) ;
#331=STYLED_ITEM('',(#196765),#350) ;
#350=MANIFOLD_SOLID_BREP('Entry Return Spring',#8727) ;
#400=PLANE('',#8988) ;
#401=PLANE('',#8997) ;
#402=PLANE('',#9006) ;
#403=PLANE('',#9007) ;
#1042=FACE_OUTER_BOUND('',#1551,.T.) ;
#1043=FACE_OUTER_BOUND('',#1552,.T.) ;
#1044=FACE_OUTER_BOUND('',#1553,.T.) ;
#1045=FACE_OUTER_BOUND('',#1554,.T.) ;
#1046=FACE_OUTER_BOUND('',#1555,.T.) ;
#1047=FACE_OUTER_BOUND('',#1556,.T.) ;
#1048=FACE_OUTER_BOUND('',#1557,.T.) ;
#1049=FACE_OUTER_BOUND('',#1558,.T.) ;
#1050=FACE_OUTER_BOUND('',#1559,.T.) ;
#1051=FACE_OUTER_BOUND('',#1560,.T.) ;
#1052=FACE_OUTER_BOUND('',#1561,.T.) ;
#1053=FACE_OUTER_BOUND('',#1562,.T.) ;
#1551=EDGE_LOOP('',(#6492)) ;
#1552=EDGE_LOOP('',(#6493,#6494,#6495,#6496,#6497,#6498,#6499,#6500)) ;
#1553=EDGE_LOOP('',(#6501,#6502,#6503,#6504,#6505,#6506)) ;
#1554=EDGE_LOOP('',(#6507,#6508,#6509,#6510,#6511,#6512)) ;
#1555=EDGE_LOOP('',(#6513,#6514,#6515,#6516,#6517,#6518)) ;
#1556=EDGE_LOOP('',(#6519)) ;
#1557=EDGE_LOOP('',(#6520,#6521,#6522,#6523,#6524,#6525,#6526,#6527)) ;
#1558=EDGE_LOOP('',(#6528,#6529,#6530,#6531,#6532,#6533)) ;
#1559=EDGE_LOOP('',(#6534,#6535,#6536,#6537,#6538,#6539)) ;
#1560=EDGE_LOOP('',(#6540,#6541,#6542,#6543,#6544,#6545)) ;
#1561=EDGE_LOOP('',(#6546,#6547,#6548)) ;
#1562=EDGE_LOOP('',(#6549,#6550,#6551)) ;
#2042=LINE('',#134170,#2745) ;
#2043=LINE('',#154157,#2746) ;
#2745=VECTOR('',#10130,10.) ;
#2746=VECTOR('',#10149,10.) ;
#3435=B_SPLINE_CURVE_WITH_KNOTS('',3,(#133905,#133906,#133907,#133908,#133909,
#133910,#133911,#133912,#133913,#133914,#133915,#133916,#133917,#133918,
#133919,#133920,#133921,#133922,#133923,#133924,#133925,#133926,#133927,
#133928,#133929,#133930,#133931,#133932,#133933,#133934,#133935,#133936,
#133937,#133938,#133939,#133940,#133941,#133942,#133943,#133944,#133945,
#133946,#133947,#133948,#133949,#133950,#133951,#133952,#133953,#133954,
#133955,#133956,#133957,#133958,#133959,#133960,#133961,#133962,#133963,
#133964,#133965,#133966,#133967,#133968,#133969,#133970,#133971,#133972,
#133973,#133974,#133975,#133976,#133977,#133978,#133979,#133980,#133981,
#133982,#133983,#133984,#133985,#133986,#133987,#133988,#133989,#133990,
#133991,#133992,#133993,#133994,#133995),.UNSPECIFIED.,.F.,.F.,(4,3,3,3,
3,3,3,3,3,3,3,3,3,3,3,3,3,3,3,3,3,3,3,3,3,3,3,3,3,3,4),(5.88213542013056,
6.01172757014424,6.06553319243455,6.3179007861267,6.37548924090185,6.63206088097925,
6.68416207138069,6.92315601894786,6.99256132469663,7.21356160680289,7.29931351804432,
7.37778610342962,7.45630346085746,7.5348566545112,7.60445173491709,7.66483126169226,
7.72511131097227,7.78447083804811,7.84521114843021,7.9059514588123,7.94504552692403,
7.9844284737438,8.02381142056356,8.05269951431726,8.08176218026163,8.08494149672526,
8.10686730860061,8.11737739318286,8.13530591783441,8.14584296460486,8.16217407354799),
 .UNSPECIFIED.) ;
#3436=B_SPLINE_CURVE_WITH_KNOTS('',3,(#133997,#133998,#133999,#134000,#134001,
#134002,#134003,#134004,#134005,#134006,#134007,#134008,#134009,#134010,
#134011,#134012,#134013,#134014,#134015,#134016,#134017,#134018,#134019,
#134020,#134021,#134022,#134023,#134024,#134025,#134026,#134027,#134028,
#134029,#134030,#134031,#134032,#134033,#134034,#134035,#134036),
 .UNSPECIFIED.,.F.,.F.,(4,2,2,2,2,2,2,2,2,2,2,2,2,2,2,2,2,2,2,4),(-0.39127659712415,
-0.362669068199835,-0.333777979412566,-0.298294797615378,-0.264279211558204,
-0.227335226972421,-0.209250043988191,-0.205161811504485,-0.20408201623579,
-0.203429602940516,-0.202882771686664,-0.202269768258323,-0.2012554462146,
-0.198930919322328,-0.191706051626658,-0.146438477798862,-0.104948460896364,
-0.0633681945290975,-0.0314897645765271,-1.00000011526991E-6),
 .UNSPECIFIED.) ;
#3437=B_SPLINE_CURVE_WITH_KNOTS('',3,(#134037,#134038,#134039,#134040,#134041,
#134042,#134043,#134044,#134045,#134046,#134047,#134048,#134049,#134050,
#134051,#134052,#134053,#134054,#134055,#134056,#134057,#134058,#134059,
#134060),.UNSPECIFIED.,.F.,.F.,(4,2,2,2,2,2,2,2,2,2,2,4),(-0.201634045224376,
-0.201150550092067,-0.200600545085954,-0.19922381894873,-0.19585601760169,
-0.188262366788053,-0.170242357527641,-0.140254894616156,-0.102132640276839,
-0.061140945039494,-0.0300852443665849,-9.99700435461159E-7),
 .UNSPECIFIED.) ;
#3438=B_SPLINE_CURVE_WITH_KNOTS('',3,(#153893,#153894,#153895,#153896,#153897,
#153898,#153899,#153900,#153901,#153902,#153903,#153904,#153905,#153906,
#153907,#153908,#153909,#153910,#153911,#153912,#153913,#153914,#153915,
#153916,#153917,#153918,#153919,#153920,#153921,#153922,#153923,#153924,
#153925,#153926,#153927,#153928,#153929,#153930,#153931,#153932,#153933,
#153934,#153935,#153936,#153937,#153938,#153939,#153940,#153941,#153942,
#153943,#153944,#153945,#153946,#153947,#153948,#153949,#153950,#153951,
#153952,#153953,#153954,#153955,#153956,#153957,#153958,#153959,#153960,
#153961,#153962,#153963,#153964,#153965,#153966,#153967,#153968,#153969,
#153970,#153971,#153972,#153973,#153974,#153975,#153976,#153977,#153978,
#153979,#153980,#153981,#153982,#153983),.UNSPECIFIED.,.F.,.F.,(4,3,3,3,
3,3,3,3,3,3,3,3,3,3,3,3,3,3,3,3,3,3,3,3,3,3,3,3,3,3,4),(5.88213542013066,
6.01172757014427,6.06553319243458,6.31790078613558,6.37548924090187,6.63206088096672,
6.68416207138071,6.92315601894749,6.99256132469664,7.21356160680676,7.29931351804433,
7.3777861034297,7.45630346085931,7.53485665450175,7.6044517349171,7.66483126169192,
7.72511131097202,7.78447083804736,7.84521114842983,7.90595145881231,7.94504552692402,
7.98442847374379,8.02381142056356,8.05269951431751,8.08176218026769,8.08494149672526,
8.10686730860063,8.11737739318286,8.13530591783441,8.14584296460486,8.16217407354799),
 .UNSPECIFIED.) ;
#3439=B_SPLINE_CURVE_WITH_KNOTS('',3,(#153984,#153985,#153986,#153987,#153988,
#153989,#153990,#153991,#153992,#153993,#153994,#153995,#153996,#153997,
#153998,#153999,#154000,#154001,#154002,#154003,#154004,#154005,#154006,
#154007,#154008,#154009,#154010,#154011,#154012,#154013,#154014,#154015,
#154016,#154017,#154018,#154019,#154020,#154021,#154022,#154023),
 .UNSPECIFIED.,.F.,.F.,(4,2,2,2,2,2,2,2,2,2,2,2,2,2,2,2,2,2,2,4),(1.0000001190084E-6,
0.0314897645751662,0.0633681945262461,0.104948460893497,0.1464384777964,
0.191706051628097,0.198930919322058,0.201255446202256,0.202269768237498,
0.202882771658999,0.203429602908372,0.204082016198889,0.205161811456729,
0.209250043899134,0.227335226679599,0.264279210845935,0.298294796516944,
0.333777977911312,0.362669066370513,0.391276594970033),.UNSPECIFIED.) ;
#3440=B_SPLINE_CURVE_WITH_KNOTS('',3,(#154024,#154025,#154026,#154027,#154028,
#154029,#154030,#154031,#154032,#154033,#154034,#154035,#154036,#154037,
#154038,#154039,#154040,#154041,#154042,#154043,#154044,#154045,#154046,
#154047),.UNSPECIFIED.,.F.,.F.,(4,2,2,2,2,2,2,2,2,2,2,4),(-0.2016340451575,
-0.201150550045475,-0.200600545062619,-0.1992238189524,-0.19585601759736,
-0.188262366785114,-0.170242357526105,-0.140254894616092,-0.10213264027677,
-0.061140945039477,-0.030085244366594,-9.99700430853734E-7),
 .UNSPECIFIED.) ;
#3750=VERTEX_POINT('',#114378) ;
#3751=VERTEX_POINT('',#132839) ;
#3752=VERTEX_POINT('',#132840) ;
#3753=VERTEX_POINT('',#133899) ;
#3754=VERTEX_POINT('',#133901) ;
#3755=VERTEX_POINT('',#133904) ;
#3756=VERTEX_POINT('',#133996) ;
#3757=VERTEX_POINT('',#134124) ;
#3758=VERTEX_POINT('',#134169) ;
#3759=VERTEX_POINT('',#134171) ;
#3760=VERTEX_POINT('',#134173) ;
#3761=VERTEX_POINT('',#134367) ;
#3762=VERTEX_POINT('',#152828) ;
#3763=VERTEX_POINT('',#152829) ;
#3764=VERTEX_POINT('',#153888) ;
#3765=VERTEX_POINT('',#153890) ;
#3766=VERTEX_POINT('',#154111) ;
#3767=VERTEX_POINT('',#154156) ;
#3768=VERTEX_POINT('',#154158) ;
#3769=VERTEX_POINT('',#154160) ;
#4754=EDGE_CURVE('',#3750,#3750,#149,.T.) ;
#4755=EDGE_CURVE('',#3751,#3752,#19,.T.) ;
#4756=EDGE_CURVE('',#3753,#3751,#150,.T.) ;
#4757=EDGE_CURVE('',#3754,#3753,#151,.T.) ;
#4758=EDGE_CURVE('',#3751,#3754,#152,.T.) ;
#4759=EDGE_CURVE('',#3755,#3752,#3435,.T.) ;
#4760=EDGE_CURVE('',#3755,#3756,#3436,.T.) ;
#4761=EDGE_CURVE('',#3752,#3756,#3437,.T.) ;
#4762=EDGE_CURVE('',#3751,#3757,#20,.T.) ;
#4763=EDGE_CURVE('',#3757,#3757,#153,.T.) ;
#4764=EDGE_CURVE('',#3757,#3758,#2042,.T.) ;
#4765=EDGE_CURVE('',#3758,#3759,#154,.T.) ;
#4766=EDGE_CURVE('',#3759,#3760,#155,.T.) ;
#4767=EDGE_CURVE('',#3760,#3758,#156,.T.) ;
#4768=EDGE_CURVE('',#3758,#3750,#21,.T.) ;
#4769=EDGE_CURVE('',#3761,#3761,#157,.T.) ;
#4770=EDGE_CURVE('',#3762,#3763,#22,.T.) ;
#4771=EDGE_CURVE('',#3764,#3762,#158,.T.) ;
#4772=EDGE_CURVE('',#3765,#3764,#159,.T.) ;
#4773=EDGE_CURVE('',#3762,#3765,#160,.T.) ;
#4774=EDGE_CURVE('',#3755,#3763,#3438,.T.) ;
#4775=EDGE_CURVE('',#3756,#3755,#3439,.T.) ;
#4776=EDGE_CURVE('',#3763,#3756,#3440,.T.) ;
#4777=EDGE_CURVE('',#3762,#3766,#23,.T.) ;
#4778=EDGE_CURVE('',#3766,#3766,#161,.T.) ;
#4779=EDGE_CURVE('',#3766,#3767,#2043,.T.) ;
#4780=EDGE_CURVE('',#3767,#3768,#162,.T.) ;
#4781=EDGE_CURVE('',#3768,#3769,#163,.T.) ;
#4782=EDGE_CURVE('',#3769,#3767,#164,.T.) ;
#4783=EDGE_CURVE('',#3767,#3761,#24,.T.) ;
#6492=ORIENTED_EDGE('',*,*,#4754,.F.) ;
#6493=ORIENTED_EDGE('',*,*,#4755,.F.) ;
#6494=ORIENTED_EDGE('',*,*,#4756,.F.) ;
#6495=ORIENTED_EDGE('',*,*,#4757,.F.) ;
#6496=ORIENTED_EDGE('',*,*,#4758,.F.) ;
#6497=ORIENTED_EDGE('',*,*,#4755,.T.) ;
#6498=ORIENTED_EDGE('',*,*,#4759,.F.) ;
#6499=ORIENTED_EDGE('',*,*,#4760,.T.) ;
#6500=ORIENTED_EDGE('',*,*,#4761,.F.) ;
#6501=ORIENTED_EDGE('',*,*,#4762,.T.) ;
#6502=ORIENTED_EDGE('',*,*,#4763,.T.) ;
#6503=ORIENTED_EDGE('',*,*,#4762,.F.) ;
#6504=ORIENTED_EDGE('',*,*,#4758,.T.) ;
#6505=ORIENTED_EDGE('',*,*,#4757,.T.) ;
#6506=ORIENTED_EDGE('',*,*,#4756,.T.) ;
#6507=ORIENTED_EDGE('',*,*,#4764,.T.) ;
#6508=ORIENTED_EDGE('',*,*,#4765,.T.) ;
#6509=ORIENTED_EDGE('',*,*,#4766,.T.) ;
#6510=ORIENTED_EDGE('',*,*,#4767,.T.) ;
#6511=ORIENTED_EDGE('',*,*,#4764,.F.) ;
#6512=ORIENTED_EDGE('',*,*,#4763,.F.) ;
#6513=ORIENTED_EDGE('',*,*,#4768,.T.) ;
#6514=ORIENTED_EDGE('',*,*,#4754,.T.) ;
#6515=ORIENTED_EDGE('',*,*,#4768,.F.) ;
#6516=ORIENTED_EDGE('',*,*,#4767,.F.) ;
#6517=ORIENTED_EDGE('',*,*,#4766,.F.) ;
#6518=ORIENTED_EDGE('',*,*,#4765,.F.) ;
#6519=ORIENTED_EDGE('',*,*,#4769,.F.) ;
#6520=ORIENTED_EDGE('',*,*,#4770,.F.) ;
#6521=ORIENTED_EDGE('',*,*,#4771,.F.) ;
#6522=ORIENTED_EDGE('',*,*,#4772,.F.) ;
#6523=ORIENTED_EDGE('',*,*,#4773,.F.) ;
#6524=ORIENTED_EDGE('',*,*,#4770,.T.) ;
#6525=ORIENTED_EDGE('',*,*,#4774,.F.) ;
#6526=ORIENTED_EDGE('',*,*,#4775,.F.) ;
#6527=ORIENTED_EDGE('',*,*,#4776,.F.) ;
#6528=ORIENTED_EDGE('',*,*,#4777,.T.) ;
#6529=ORIENTED_EDGE('',*,*,#4778,.T.) ;
#6530=ORIENTED_EDGE('',*,*,#4777,.F.) ;
#6531=ORIENTED_EDGE('',*,*,#4773,.T.) ;
#6532=ORIENTED_EDGE('',*,*,#4772,.T.) ;
#6533=ORIENTED_EDGE('',*,*,#4771,.T.) ;
#6534=ORIENTED_EDGE('',*,*,#4779,.T.) ;
#6535=ORIENTED_EDGE('',*,*,#4780,.T.) ;
#6536=ORIENTED_EDGE('',*,*,#4781,.T.) ;
#6537=ORIENTED_EDGE('',*,*,#4782,.T.) ;
#6538=ORIENTED_EDGE('',*,*,#4779,.F.) ;
#6539=ORIENTED_EDGE('',*,*,#4778,.F.) ;
#6540=ORIENTED_EDGE('',*,*,#4783,.T.) ;
#6541=ORIENTED_EDGE('',*,*,#4769,.T.) ;
#6542=ORIENTED_EDGE('',*,*,#4783,.F.) ;
#6543=ORIENTED_EDGE('',*,*,#4782,.F.) ;
#6544=ORIENTED_EDGE('',*,*,#4781,.F.) ;
#6545=ORIENTED_EDGE('',*,*,#4780,.F.) ;
#6546=ORIENTED_EDGE('',*,*,#4774,.T.) ;
#6547=ORIENTED_EDGE('',*,*,#4776,.T.) ;
#6548=ORIENTED_EDGE('',*,*,#4760,.F.) ;
#6549=ORIENTED_EDGE('',*,*,#4775,.T.) ;
#6550=ORIENTED_EDGE('',*,*,#4759,.T.) ;
#6551=ORIENTED_EDGE('',*,*,#4761,.T.) ;
#8425=ADVANCED_FACE('',(#1042),#400,.T.) ;
#8426=ADVANCED_FACE('',(#1043),#43,.T.) ;
#8427=ADVANCED_FACE('',(#1044),#44,.T.) ;
#8428=ADVANCED_FACE('',(#1045),#45,.T.) ;
#8429=ADVANCED_FACE('',(#1046),#46,.T.) ;
#8430=ADVANCED_FACE('',(#1047),#401,.T.) ;
#8431=ADVANCED_FACE('',(#1048),#47,.T.) ;
#8432=ADVANCED_FACE('',(#1049),#48,.T.) ;
#8433=ADVANCED_FACE('',(#1050),#49,.T.) ;
#8434=ADVANCED_FACE('',(#1051),#50,.T.) ;
#8435=ADVANCED_FACE('',(#1052),#402,.T.) ;
#8436=ADVANCED_FACE('',(#1053),#403,.T.) ;
#8727=CLOSED_SHELL('',(#8425,#8426,#8427,#8428,#8429,#8430,#8431,#8432,
#8433,#8434,#8435,#8436)) ;
#8988=AXIS2_PLACEMENT_3D('',#114377,#10118,#10119) ;
#8989=AXIS2_PLACEMENT_3D('',#114379,#10120,#10121) ;
#8990=AXIS2_PLACEMENT_3D('',#133900,#10122,#10123) ;
#8991=AXIS2_PLACEMENT_3D('',#133902,#10124,#10125) ;
#8992=AXIS2_PLACEMENT_3D('',#133903,#10126,#10127) ;
#8993=AXIS2_PLACEMENT_3D('',#134132,#10128,#10129) ;
#8994=AXIS2_PLACEMENT_3D('',#134172,#10131,#10132) ;
#8995=AXIS2_PLACEMENT_3D('',#134174,#10133,#10134) ;
#8996=AXIS2_PLACEMENT_3D('',#134175,#10135,#10136) ;
#8997=AXIS2_PLACEMENT_3D('',#134366,#10137,#10138) ;
#8998=AXIS2_PLACEMENT_3D('',#134368,#10139,#10140) ;
#8999=AXIS2_PLACEMENT_3D('',#153889,#10141,#10142) ;
#9000=AXIS2_PLACEMENT_3D('',#153891,#10143,#10144) ;
#9001=AXIS2_PLACEMENT_3D('',#153892,#10145,#10146) ;
#9002=AXIS2_PLACEMENT_3D('',#154119,#10147,#10148) ;
#9003=AXIS2_PLACEMENT_3D('',#154159,#10150,#10151) ;
#9004=AXIS2_PLACEMENT_3D('',#154161,#10152,#10153) ;
#9005=AXIS2_PLACEMENT_3D('',#154162,#10154,#10155) ;
#9006=AXIS2_PLACEMENT_3D('',#154353,#10156,#10157) ;
#9007=AXIS2_PLACEMENT_3D('',#154354,#10158,#10159) ;
#10118=DIRECTION('center_axis',(-0.958097822844588,-0.0208105263954551,
0.285684238017439)) ;
#10119=DIRECTION('ref_axis',(0.285746119898407,0.,0.958305355804195)) ;
#10120=DIRECTION('center_axis',(0.958097822844581,0.0208105263955041,-0.285684238017459)) ;
#10121=DIRECTION('ref_axis',(0.286206169394248,-0.0291560893922151,0.957724360686322)) ;
#10122=DIRECTION('center_axis',(0.0789989380213253,0.96979445877955,-0.230776678873718)) ;
#10123=DIRECTION('ref_axis',(0.946102418132454,7.31486930126385E-12,0.323867587763771)) ;
#10124=DIRECTION('center_axis',(0.0789989380213253,0.96979445877955,-0.230776678873718)) ;
#10125=DIRECTION('ref_axis',(0.946102418132454,7.31486930126385E-12,0.323867587763771)) ;
#10126=DIRECTION('center_axis',(0.0789989380213253,0.96979445877955,-0.230776678873718)) ;
#10127=DIRECTION('ref_axis',(0.946102418132454,7.31486930126385E-12,0.323867587763771)) ;
#10128=DIRECTION('center_axis',(-0.0396714859666553,0.0207623501566727,
-0.998997046050272)) ;
#10129=DIRECTION('ref_axis',(0.999186758728018,0.00803913676004757,-0.0395119407616252)) ;
#10130=DIRECTION('',(0.00302837173055173,2.34500326237813E-6,0.999995414469068)) ;
#10131=DIRECTION('center_axis',(-0.03967148596651,0.020762350156785,-0.998997046050275)) ;
#10132=DIRECTION('ref_axis',(0.999186758728035,0.0080391367584932,-0.0395119407615118)) ;
#10133=DIRECTION('center_axis',(-0.03967148596651,0.020762350156785,-0.998997046050275)) ;
#10134=DIRECTION('ref_axis',(0.999186758728035,0.0080391367584932,-0.0395119407615118)) ;
#10135=DIRECTION('center_axis',(-0.03967148596651,0.020762350156785,-0.998997046050275)) ;
#10136=DIRECTION('ref_axis',(0.999186758728035,0.0080391367584932,-0.0395119407615118)) ;
#10137=DIRECTION('center_axis',(0.958097822844586,-0.0208105263955017,-0.285684238017442)) ;
#10138=DIRECTION('ref_axis',(-0.285746119898411,0.,-0.958305355804194)) ;
#10139=DIRECTION('center_axis',(-0.958097822844564,0.0208105263953766,0.285684238017527)) ;
#10140=DIRECTION('ref_axis',(0.286206169391818,0.0291560891774949,0.957724360693585)) ;
#10141=DIRECTION('center_axis',(-0.0789989380212596,0.969794458779555,0.230776678873719)) ;
#10142=DIRECTION('ref_axis',(0.946102418124642,-1.34456916771157E-11,0.32386758778659)) ;
#10143=DIRECTION('center_axis',(-0.0789989380212596,0.969794458779555,0.230776678873719)) ;
#10144=DIRECTION('ref_axis',(0.946102418124642,-1.34456916771157E-11,0.32386758778659)) ;
#10145=DIRECTION('center_axis',(-0.0789989380212596,0.969794458779555,0.230776678873719)) ;
#10146=DIRECTION('ref_axis',(0.946102418124642,-1.34456916771157E-11,0.32386758778659)) ;
#10147=DIRECTION('center_axis',(0.0396714859665023,0.0207623501562736,0.998997046050286)) ;
#10148=DIRECTION('ref_axis',(0.999186758727716,-0.00803913680279955,-0.0395119407605742)) ;
#10149=DIRECTION('',(-0.00302837173057115,2.34500326237817E-6,-0.999995414469068)) ;
#10150=DIRECTION('center_axis',(0.0396714859664518,0.0207623501564799,0.998997046050284)) ;
#10151=DIRECTION('ref_axis',(0.999186758728069,-0.00803913675410597,-0.0395119407615483)) ;
#10152=DIRECTION('center_axis',(0.0396714859664518,0.0207623501564799,0.998997046050284)) ;
#10153=DIRECTION('ref_axis',(0.999186758728069,-0.00803913675410597,-0.0395119407615483)) ;
#10154=DIRECTION('center_axis',(0.0396714859664518,0.0207623501564799,0.998997046050284)) ;
#10155=DIRECTION('ref_axis',(0.999186758728069,-0.00803913675410597,-0.0395119407615483)) ;
#10156=DIRECTION('center_axis',(0.94610241814194,0.,0.323867587736059)) ;
#10157=DIRECTION('ref_axis',(0.323867587736059,0.,-0.94610241814194)) ;
#10158=DIRECTION('center_axis',(-0.94610241814194,0.,-0.32386758773606)) ;
#10159=DIRECTION('ref_axis',(-0.32386758773606,0.,0.94610241814194)) ;
#114377=CARTESIAN_POINT('Origin',(-10.8407396157986,13.385947639229,133.868521514384)) ;
#114378=CARTESIAN_POINT('',(-10.8223318974888,13.4658311995141,133.936074466937)) ;
#114379=CARTESIAN_POINT('Origin',(-10.8428777772314,13.4930077522664,133.86914951366)) ;
#114380=CARTESIAN_POINT('Ctrl Pts',(-11.2812798643659,13.1551399285885,
133.225361312885)) ;
#114381=CARTESIAN_POINT('Ctrl Pts',(-11.2820187647633,13.1489709609094,
133.226788867079)) ;
#114382=CARTESIAN_POINT('Ctrl Pts',(-11.2940725891313,13.0505878441039,
133.250318667877)) ;
#114383=CARTESIAN_POINT('Ctrl Pts',(-11.3268196692865,12.8648900473044,
133.323006215356)) ;
#114384=CARTESIAN_POINT('Ctrl Pts',(-11.3955581347561,12.6378996894465,
133.490786092827)) ;
#114385=CARTESIAN_POINT('Ctrl Pts',(-11.4818126038911,12.4661938442505,
133.709651137204)) ;
#114386=CARTESIAN_POINT('Ctrl Pts',(-11.5806418499012,12.3629468779938,
133.965082777503)) ;
#114387=CARTESIAN_POINT('Ctrl Pts',(-11.6840920756584,12.3360866578135,
134.234357728742)) ;
#114388=CARTESIAN_POINT('Ctrl Pts',(-11.7874232958009,12.3868467815327,
134.502988211751)) ;
#114389=CARTESIAN_POINT('Ctrl Pts',(-11.8826517586958,12.5118616193735,
134.748082512994)) ;
#114390=CARTESIAN_POINT('Ctrl Pts',(-11.9642364503466,12.7022376314793,
134.953268302114)) ;
#114391=CARTESIAN_POINT('Ctrl Pts',(-12.0268555159077,12.9442211340136,
135.103070944459)) ;
#114392=CARTESIAN_POINT('Ctrl Pts',(-12.0667868417897,13.2203922331636,
135.186606249474)) ;
#114393=CARTESIAN_POINT('Ctrl Pts',(-12.0819921567622,13.5109001041669,
135.197934267535)) ;
#114394=CARTESIAN_POINT('Ctrl Pts',(-12.0718871830781,13.7967277450532,
135.135125417403)) ;
#114395=CARTESIAN_POINT('Ctrl Pts',(-12.0382787552941,14.0531634695327,
135.003985075531)) ;
#114396=CARTESIAN_POINT('Ctrl Pts',(-11.984040511163,14.2659161102292,134.812412340654)) ;
#114397=CARTESIAN_POINT('Ctrl Pts',(-11.9138317313736,14.4182155312585,
134.574200139104)) ;
#114398=CARTESIAN_POINT('Ctrl Pts',(-11.8331828494072,14.4993926065239,
134.305392211434)) ;
#114399=CARTESIAN_POINT('Ctrl Pts',(-11.7490444838035,14.5030674016304,
134.026483130585)) ;
#114400=CARTESIAN_POINT('Ctrl Pts',(-11.6680809986179,14.4296658181567,
133.756898311423)) ;
#114401=CARTESIAN_POINT('Ctrl Pts',(-11.5965958202758,14.2842405620309,
133.514968656249)) ;
#114402=CARTESIAN_POINT('Ctrl Pts',(-11.5404239481228,14.0768885755418,
133.31772524141)) ;
#114403=CARTESIAN_POINT('Ctrl Pts',(-11.5044626643021,13.821937566696,133.179448820527)) ;
#114404=CARTESIAN_POINT('Ctrl Pts',(-11.492115437901,13.5404397832619,133.110400577556)) ;
#114405=CARTESIAN_POINT('Ctrl Pts',(-11.5046895368218,13.2491903771815,
133.113990718504)) ;
#114406=CARTESIAN_POINT('Ctrl Pts',(-11.5423996819585,12.9699188880577,
133.190943520196)) ;
#114407=CARTESIAN_POINT('Ctrl Pts',(-11.6027127193453,12.7245502986717,
133.33412175314)) ;
#114408=CARTESIAN_POINT('Ctrl Pts',(-11.6827307770101,12.5279694687298,
133.534676781188)) ;
#114409=CARTESIAN_POINT('Ctrl Pts',(-11.7767909409935,12.3961377043517,
133.7763823545)) ;
#114410=CARTESIAN_POINT('Ctrl Pts',(-11.8796482494039,12.3376103677892,
134.043626665423)) ;
#114411=CARTESIAN_POINT('Ctrl Pts',(-11.9835249356267,12.3569098529355,
134.314074542349)) ;
#114412=CARTESIAN_POINT('Ctrl Pts',(-12.0830151650733,12.452769019898,134.571498333322)) ;
#114413=CARTESIAN_POINT('Ctrl Pts',(-12.1707022339469,12.6179593573441,
134.794565234874)) ;
#114414=CARTESIAN_POINT('Ctrl Pts',(-12.2415306520725,12.8405880377693,
134.968374154773)) ;
#114415=CARTESIAN_POINT('Ctrl Pts',(-12.2912076318387,13.1065246421439,
135.080214865833)) ;
#114416=CARTESIAN_POINT('Ctrl Pts',(-12.3163775691246,13.3925179674891,
135.12078307657)) ;
#114417=CARTESIAN_POINT('Ctrl Pts',(-12.3166058496797,13.6819916651313,
135.088335546118)) ;
#114418=CARTESIAN_POINT('Ctrl Pts',(-12.2921472081091,13.9537242418059,
134.983669295533)) ;
#114419=CARTESIAN_POINT('Ctrl Pts',(-12.2457390773696,14.1863734291659,
134.815010882744)) ;
#114420=CARTESIAN_POINT('Ctrl Pts',(-12.1814800516644,14.3643807985693,
134.59423567404)) ;
#114421=CARTESIAN_POINT('Ctrl Pts',(-12.1044683457898,14.4754559850244,
134.336147922274)) ;
#114422=CARTESIAN_POINT('Ctrl Pts',(-12.0208090250937,14.5110246739577,
134.058551574174)) ;
#114423=CARTESIAN_POINT('Ctrl Pts',(-11.9378612224862,14.4687063588107,
133.783197368949)) ;
#114424=CARTESIAN_POINT('Ctrl Pts',(-11.8615647632541,14.3514018815055,
133.527145574601)) ;
#114425=CARTESIAN_POINT('Ctrl Pts',(-11.798502564401,14.1671964752596,133.309749293991)) ;
#114426=CARTESIAN_POINT('Ctrl Pts',(-11.754049052173,13.9308608041133,133.146872132253)) ;
#114427=CARTESIAN_POINT('Ctrl Pts',(-11.7316977644638,13.6570089999716,
133.048397750488)) ;
#114428=CARTESIAN_POINT('Ctrl Pts',(-11.7341180951435,13.3664659574419,
133.022308686926)) ;
#114429=CARTESIAN_POINT('Ctrl Pts',(-11.761720921654,13.0805681472547,133.069846022257)) ;
#114430=CARTESIAN_POINT('Ctrl Pts',(-11.8131936002259,12.8190539470386,
133.187112979174)) ;
#114431=CARTESIAN_POINT('Ctrl Pts',(-11.886092857491,12.5999338423892,133.366806137464)) ;
#114432=CARTESIAN_POINT('Ctrl Pts',(-11.9747587487869,12.4413957528131,
133.592859241921)) ;
#114433=CARTESIAN_POINT('Ctrl Pts',(-12.0748052338517,12.3520378265489,
133.85195165464)) ;
#114434=CARTESIAN_POINT('Ctrl Pts',(-12.1791704719716,12.339734386482,134.123710421306)) ;
#114435=CARTESIAN_POINT('Ctrl Pts',(-12.2811942198852,12.4049383167358,
134.388634754176)) ;
#114436=CARTESIAN_POINT('Ctrl Pts',(-12.3743104910804,12.5429634979505,
134.627548525017)) ;
#114437=CARTESIAN_POINT('Ctrl Pts',(-12.4527350962615,12.7443553986761,
134.823486021638)) ;
#114438=CARTESIAN_POINT('Ctrl Pts',(-12.5113245953194,12.9943521537239,
134.961502568807)) ;
#114439=CARTESIAN_POINT('Ctrl Pts',(-12.5466491191103,13.2741647768729,
135.031655728832)) ;
#114440=CARTESIAN_POINT('Ctrl Pts',(-12.557133530808,13.565720269456,135.029118946566)) ;
#114441=CARTESIAN_POINT('Ctrl Pts',(-12.5424084976818,13.8474315556546,
134.952884078473)) ;
#114442=CARTESIAN_POINT('Ctrl Pts',(-12.504658245782,14.0971649669908,134.809596596871)) ;
#114443=CARTESIAN_POINT('Ctrl Pts',(-12.4468015681524,14.3002122843455,
134.607345660129)) ;
#114444=CARTESIAN_POINT('Ctrl Pts',(-12.3740820116557,14.4394509674979,
134.361774496034)) ;
#114445=CARTESIAN_POINT('Ctrl Pts',(-12.2928286579386,14.5058688200503,
134.091445642351)) ;
#114446=CARTESIAN_POINT('Ctrl Pts',(-12.2085754911848,14.4952594831202,
133.812133112469)) ;
#114447=CARTESIAN_POINT('Ctrl Pts',(-12.1285286312613,14.4071576912799,
133.54505905862)) ;
#114448=CARTESIAN_POINT('Ctrl Pts',(-12.0595995840032,14.2488070341169,
133.310594609379)) ;
#114449=CARTESIAN_POINT('Ctrl Pts',(-12.007204001394,14.032332595662,133.124541926762)) ;
#114450=CARTESIAN_POINT('Ctrl Pts',(-11.9754518623539,13.7715185673777,
132.998664946929)) ;
#114451=CARTESIAN_POINT('Ctrl Pts',(-11.9676077024159,13.4849968555095,
132.942553623633)) ;
#114452=CARTESIAN_POINT('Ctrl Pts',(-11.9852141495617,13.1936954317484,
132.960744777079)) ;
#114453=CARTESIAN_POINT('Ctrl Pts',(-12.0270155274854,12.9217410981826,
133.049976934939)) ;
#114454=CARTESIAN_POINT('Ctrl Pts',(-12.0916442917843,12.6826993167214,
133.205531163459)) ;
#114455=CARTESIAN_POINT('Ctrl Pts',(-12.1748344849184,12.4976839220085,
133.415374259801)) ;
#114456=CARTESIAN_POINT('Ctrl Pts',(-12.2706003786281,12.3794711428103,
133.662174391645)) ;
#114457=CARTESIAN_POINT('Ctrl Pts',(-12.3744503899862,12.3351744196322,
133.932269165389)) ;
#114458=CARTESIAN_POINT('Ctrl Pts',(-12.4782650208009,12.3695012763354,
134.202412750315)) ;
#114459=CARTESIAN_POINT('Ctrl Pts',(-12.5754721648271,12.4786183736045,
134.453365352351)) ;
#114460=CARTESIAN_POINT('Ctrl Pts',(-12.6605578265862,12.6556201701116,
134.668788412585)) ;
#114461=CARTESIAN_POINT('Ctrl Pts',(-12.7278290779799,12.8885376957079,
134.832076052564)) ;
#114462=CARTESIAN_POINT('Ctrl Pts',(-12.7727942038789,13.1578672277872,
134.93044163856)) ;
#114463=CARTESIAN_POINT('Ctrl Pts',(-12.7935589960753,13.4488181058444,
134.957796140316)) ;
#114464=CARTESIAN_POINT('Ctrl Pts',(-12.7888443918457,13.7357351250712,
134.91097260511)) ;
#114465=CARTESIAN_POINT('Ctrl Pts',(-12.7602605916963,14.0000244154435,
134.794478626913)) ;
#114466=CARTESIAN_POINT('Ctrl Pts',(-12.7099141607957,14.2248063693443,
134.614145960045)) ;
#114467=CARTESIAN_POINT('Ctrl Pts',(-12.6428897963242,14.3907221531774,
134.385334239461)) ;
#114468=CARTESIAN_POINT('Ctrl Pts',(-12.5640447774941,14.4880878052934,
134.121834427977)) ;
#114469=CARTESIAN_POINT('Ctrl Pts',(-12.4802617689659,14.5090844515927,
133.844015139513)) ;
#114470=CARTESIAN_POINT('Ctrl Pts',(-12.3974642832698,14.4517331277302,
133.568827359843)) ;
#114471=CARTESIAN_POINT('Ctrl Pts',(-12.3236763447296,14.3213873494252,
133.320287858352)) ;
#114472=CARTESIAN_POINT('Ctrl Pts',(-12.2637347152158,14.1266126254878,
133.112060420808)) ;
#114473=CARTESIAN_POINT('Ctrl Pts',(-12.2229774667805,13.8801113803002,
132.959735466426)) ;
#114474=CARTESIAN_POINT('Ctrl Pts',(-12.2053838579744,13.6025840232108,
132.875302084043)) ;
#114475=CARTESIAN_POINT('Ctrl Pts',(-12.2124772397581,13.3122088978665,
132.862974191922)) ;
#114476=CARTESIAN_POINT('Ctrl Pts',(-12.2448145015933,13.0284665595888,
132.924236901387)) ;
#114477=CARTESIAN_POINT('Ctrl Pts',(-12.3005599019218,12.7739765033465,
133.053999198988)) ;
#114478=CARTESIAN_POINT('Ctrl Pts',(-12.3766445028271,12.5655228915478,
133.243117582921)) ;
#114479=CARTESIAN_POINT('Ctrl Pts',(-12.4681423855166,12.4188418488155,
133.47731500825)) ;
#114480=CARTESIAN_POINT('Ctrl Pts',(-12.5692422546882,12.3438198182334,
133.739584235759)) ;
#114481=CARTESIAN_POINT('Ctrl Pts',(-12.6740334889537,12.3461749880073,
134.012474638995)) ;
#114482=CARTESIAN_POINT('Ctrl Pts',(-12.7747162224539,12.4256199459212,
134.273532924423)) ;
#114483=CARTESIAN_POINT('Ctrl Pts',(-12.8655945356852,12.5766359900473,
134.505860328425)) ;
#114484=CARTESIAN_POINT('Ctrl Pts',(-12.9405208029623,12.7882864475543,
134.691614915467)) ;
#114485=CARTESIAN_POINT('Ctrl Pts',(-12.9949316879518,13.0452019382586,
134.817458837911)) ;
#114486=CARTESIAN_POINT('Ctrl Pts',(-13.025720643168,13.3293877258915,134.874271333741)) ;
#114487=CARTESIAN_POINT('Ctrl Pts',(-13.0313457796955,13.6204035856812,
134.857561997613)) ;
#114488=CARTESIAN_POINT('Ctrl Pts',(-13.0121238177563,13.8971496153171,
134.768280402699)) ;
#114489=CARTESIAN_POINT('Ctrl Pts',(-12.9702433337836,14.1397539052331,
134.612839445253)) ;
#114490=CARTESIAN_POINT('Ctrl Pts',(-12.9092683557999,14.3313464702874,
134.401559637406)) ;
#114491=CARTESIAN_POINT('Ctrl Pts',(-12.8346344667875,14.4574458616527,
134.150487900523)) ;
#114492=CARTESIAN_POINT('Ctrl Pts',(-12.7520232585293,14.5099723944026,
133.876034599555)) ;
#114493=CARTESIAN_POINT('Ctrl Pts',(-12.6680149991839,14.4843439695083,
133.597416296755)) ;
#114494=CARTESIAN_POINT('Ctrl Pts',(-12.5898605639027,14.3827749410654,
133.336012913517)) ;
#114495=CARTESIAN_POINT('Ctrl Pts',(-12.5235110131134,14.2124739950545,
133.109063094795)) ;
#114496=CARTESIAN_POINT('Ctrl Pts',(-12.47454385575,13.9855789386979,132.932891873958)) ;
#114497=CARTESIAN_POINT('Ctrl Pts',(-12.44718714331,13.7185805864342,132.819871229684)) ;
#114498=CARTESIAN_POINT('Ctrl Pts',(-12.4441083202369,13.4303185636673,
132.777757800251)) ;
#114499=CARTESIAN_POINT('Ctrl Pts',(-12.4662081675216,13.1417758325219,
132.809228396078)) ;
#114500=CARTESIAN_POINT('Ctrl Pts',(-12.5128438608682,12.8725286043858,
132.912265477798)) ;
#114501=CARTESIAN_POINT('Ctrl Pts',(-12.5811355936144,12.6435096258014,
133.078662360882)) ;
#114502=CARTESIAN_POINT('Ctrl Pts',(-12.6670557983815,12.4701546223289,
133.296533072804)) ;
#114503=CARTESIAN_POINT('Ctrl Pts',(-12.7650980875458,12.3650501876111,
133.549835459936)) ;
#114504=CARTESIAN_POINT('Ctrl Pts',(-12.8692895553206,12.3357586674927,
133.821013809302)) ;
#114505=CARTESIAN_POINT('Ctrl Pts',(-12.9722194636702,12.3843195509594,
134.088641190149)) ;
#114506=CARTESIAN_POINT('Ctrl Pts',(-13.0679235169665,12.5073666683789,
134.335069106556)) ;
#114507=CARTESIAN_POINT('Ctrl Pts',(-13.1498474421669,12.6958200369819,
134.541296314724)) ;
#114508=CARTESIAN_POINT('Ctrl Pts',(-13.2130846476701,12.9363649293222,
134.692916583502)) ;
#114509=CARTESIAN_POINT('Ctrl Pts',(-13.2537553284003,13.212046231595,134.778583028313)) ;
#114510=CARTESIAN_POINT('Ctrl Pts',(-13.2696867588976,13.5022481067603,
134.792052779991)) ;
#114511=CARTESIAN_POINT('Ctrl Pts',(-13.2603291226857,13.7884016128943,
134.731444216182)) ;
#114512=CARTESIAN_POINT('Ctrl Pts',(-13.2274358441086,14.045945075732,134.602400846472)) ;
#114513=CARTESIAN_POINT('Ctrl Pts',(-13.1734739345736,14.2610680704969,
134.41149155897)) ;
#114514=CARTESIAN_POINT('Ctrl Pts',(-13.1038966633744,14.4145624165552,
134.175255364668)) ;
#114515=CARTESIAN_POINT('Ctrl Pts',(-13.0234728088093,14.4980852125695,
133.907100960487)) ;
#114516=CARTESIAN_POINT('Ctrl Pts',(-12.939325995419,14.5041312739862,133.628163299805)) ;
#114517=CARTESIAN_POINT('Ctrl Pts',(-12.8580140805557,14.4326962339747,
133.357486536545)) ;
#114518=CARTESIAN_POINT('Ctrl Pts',(-12.7862358410937,14.289424830309,133.114743545619)) ;
#114519=CARTESIAN_POINT('Ctrl Pts',(-12.7294171395877,14.0826507854277,
132.915479459106)) ;
#114520=CARTESIAN_POINT('Ctrl Pts',(-12.6931113261045,13.8312291814697,
132.77650858526)) ;
#114521=CARTESIAN_POINT('Ctrl Pts',(-12.6798565616288,13.5479805821752,
132.704527307887)) ;
#114522=CARTESIAN_POINT('Ctrl Pts',(-12.6918329131031,13.2572981016289,
132.706442366543)) ;
#114523=CARTESIAN_POINT('Ctrl Pts',(-12.7286154648152,12.9781391944844,
132.780789668285)) ;
#114524=CARTESIAN_POINT('Ctrl Pts',(-12.788841308569,12.7298471383749,132.923457407859)) ;
#114525=CARTESIAN_POINT('Ctrl Pts',(-12.8678064119023,12.5331718510569,
133.121190067536)) ;
#114526=CARTESIAN_POINT('Ctrl Pts',(-12.9619860922532,12.3987050488903,
133.3630746114)) ;
#114527=CARTESIAN_POINT('Ctrl Pts',(-13.0641173669679,12.3381977133859,
133.628393862531)) ;
#114528=CARTESIAN_POINT('Ctrl Pts',(-13.1689636586994,12.3556285786372,
133.901368958815)) ;
#114529=CARTESIAN_POINT('Ctrl Pts',(-13.2676215267395,12.448498640132,134.156721062578)) ;
#114530=CARTESIAN_POINT('Ctrl Pts',(-13.3562794099848,12.6124651727369,
134.382428532808)) ;
#114531=CARTESIAN_POINT('Ctrl Pts',(-13.4274024159188,12.8330193864531,
134.55721035227)) ;
#114532=CARTESIAN_POINT('Ctrl Pts',(-13.4778657839761,13.0981216515098,
134.671314825157)) ;
#114533=CARTESIAN_POINT('Ctrl Pts',(-13.5037873702561,13.3840423616995,
134.714047923931)) ;
#114534=CARTESIAN_POINT('Ctrl Pts',(-13.5047230832927,13.6738043197191,
134.683656575562)) ;
#114535=CARTESIAN_POINT('Ctrl Pts',(-13.4810350619758,13.9458856450603,
134.581307831703)) ;
#114536=CARTESIAN_POINT('Ctrl Pts',(-13.4350850950003,14.1805609741337,
134.413888828413)) ;
#114537=CARTESIAN_POINT('Ctrl Pts',(-13.3713435625267,14.3602096703021,
134.19466352274)) ;
#114538=CARTESIAN_POINT('Ctrl Pts',(-13.2941228668166,14.4737146563849,
133.935766751957)) ;
#114539=CARTESIAN_POINT('Ctrl Pts',(-13.2111150371913,14.510981736058,133.660304806086)) ;
#114540=CARTESIAN_POINT('Ctrl Pts',(-13.1279555516473,14.4710234538019,
133.384286573336)) ;
#114541=CARTESIAN_POINT('Ctrl Pts',(-13.0514607207591,14.3558611755068,
133.127695259553)) ;
#114542=CARTESIAN_POINT('Ctrl Pts',(-12.987929872837,14.1736059642118,132.908940703681)) ;
#114543=CARTESIAN_POINT('Ctrl Pts',(-12.9427874558613,13.9381264816024,
132.743987191645)) ;
#114544=CARTESIAN_POINT('Ctrl Pts',(-12.9198159126567,13.665192099168,132.643720985883)) ;
#114545=CARTESIAN_POINT('Ctrl Pts',(-12.9214159568252,13.3755914984187,
132.615321479283)) ;
#114546=CARTESIAN_POINT('Ctrl Pts',(-12.9485033871058,13.0874857506397,
132.661141600498)) ;
#114547=CARTESIAN_POINT('Ctrl Pts',(-12.9991534842726,12.8264337657975,
132.776172659393)) ;
#114548=CARTESIAN_POINT('Ctrl Pts',(-13.0712502877118,12.6060974389448,
132.953593799865)) ;
#114549=CARTESIAN_POINT('Ctrl Pts',(-13.1597261697062,12.4450313389733,
133.179001034814)) ;
#114550=CARTESIAN_POINT('Ctrl Pts',(-13.2598221399245,12.3534666197661,
133.438152169847)) ;
#114551=CARTESIAN_POINT('Ctrl Pts',(-13.3638496997786,12.3390029903486,
133.709021457282)) ;
#114552=CARTESIAN_POINT('Ctrl Pts',(-13.466268319613,12.4020392430349,133.975026492123)) ;
#114553=CARTESIAN_POINT('Ctrl Pts',(-13.5598211640111,12.5385711173323,
134.215165246668)) ;
#114554=CARTESIAN_POINT('Ctrl Pts',(-13.6383382505058,12.737337324062,134.411540597844)) ;
#114555=CARTESIAN_POINT('Ctrl Pts',(-13.6976697861643,12.9861206892308,
134.551707741949)) ;
#114556=CARTESIAN_POINT('Ctrl Pts',(-13.7337928936498,13.2660910782566,
134.62410596592)) ;
#114557=CARTESIAN_POINT('Ctrl Pts',(-13.7449404119012,13.5573227840952,
134.623538746113)) ;
#114558=CARTESIAN_POINT('Ctrl Pts',(-13.731057609949,13.8386952169897,134.549882879065)) ;
#114559=CARTESIAN_POINT('Ctrl Pts',(-13.6938267710482,14.0906007554108,
134.407982826979)) ;
#114560=CARTESIAN_POINT('Ctrl Pts',(-13.6366983945426,14.2945039762926,
134.207985282423)) ;
#114561=CARTESIAN_POINT('Ctrl Pts',(-13.5643971905334,14.4361574187858,
133.963631330981)) ;
#114562=CARTESIAN_POINT('Ctrl Pts',(-13.4829079562931,14.5051117570611,
133.692450855681)) ;
#114563=CARTESIAN_POINT('Ctrl Pts',(-13.398865589322,14.496582620466,133.413844416583)) ;
#114564=CARTESIAN_POINT('Ctrl Pts',(-13.3188758691256,14.4113394819302,
133.147064384826)) ;
#114565=CARTESIAN_POINT('Ctrl Pts',(-13.2492482094451,14.2546479447355,
132.910444808226)) ;
#114566=CARTESIAN_POINT('Ctrl Pts',(-13.1961963849046,14.039143877786,132.722400695126)) ;
#114567=CARTESIAN_POINT('Ctrl Pts',(-13.1638347550569,13.7793416572316,
132.594749383636)) ;
#114568=CARTESIAN_POINT('Ctrl Pts',(-13.1552775077889,13.4941095874199,
132.536650789137)) ;
#114569=CARTESIAN_POINT('Ctrl Pts',(-13.1720447629105,13.2026874966814,
132.552397812081)) ;
#114570=CARTESIAN_POINT('Ctrl Pts',(-13.2133004298939,12.928833346161,132.639904988231)) ;
#114571=CARTESIAN_POINT('Ctrl Pts',(-13.2774801251183,12.6885083712283,
132.794116581438)) ;
#114572=CARTESIAN_POINT('Ctrl Pts',(-13.3597053837363,12.5026390795781,
133.001327621254)) ;
#114573=CARTESIAN_POINT('Ctrl Pts',(-13.455701350823,12.3816810236162,133.248611444686)) ;
#114574=CARTESIAN_POINT('Ctrl Pts',(-13.5588450701788,12.3354826595071,
133.516837122875)) ;
#114575=CARTESIAN_POINT('Ctrl Pts',(-13.662986257812,12.3671988660942,133.787859387829)) ;
#114576=CARTESIAN_POINT('Ctrl Pts',(-13.7608857501055,12.4748749581507,
134.040689706046)) ;
#114577=CARTESIAN_POINT('Ctrl Pts',(-13.8461189502053,12.6498955190515,
134.256626571108)) ;
#114578=CARTESIAN_POINT('Ctrl Pts',(-13.9137641762851,12.8801431332148,
134.421162047123)) ;
#114579=CARTESIAN_POINT('Ctrl Pts',(-13.959688118663,13.1504415297617,134.52210348875)) ;
#114580=CARTESIAN_POINT('Ctrl Pts',(-13.9810355826832,13.438739202615,134.551438413197)) ;
#114581=CARTESIAN_POINT('Ctrl Pts',(-13.9771509252308,13.7280473502378,
134.50680820225)) ;
#114582=CARTESIAN_POINT('Ctrl Pts',(-13.9490883356948,13.9932362064335,
134.391820118097)) ;
#114583=CARTESIAN_POINT('Ctrl Pts',(-13.899552383743,14.2186783745982,134.213988401194)) ;
#114584=CARTESIAN_POINT('Ctrl Pts',(-13.8326088799132,14.3872014330787,
133.985246691092)) ;
#114585=CARTESIAN_POINT('Ctrl Pts',(-13.754354251272,14.486216521528,133.723625961275)) ;
#114586=CARTESIAN_POINT('Ctrl Pts',(-13.6703274653614,14.5095010567365,
133.444968044136)) ;
#114587=CARTESIAN_POINT('Ctrl Pts',(-13.587915515568,14.4548476689191,133.171125957688)) ;
#114588=CARTESIAN_POINT('Ctrl Pts',(-13.5132496102258,14.3259646517619,
132.919798090487)) ;
#114589=CARTESIAN_POINT('Ctrl Pts',(-13.4528381497739,14.1320240566172,
132.710133322283)) ;
#114590=CARTESIAN_POINT('Ctrl Pts',(-13.4117984923924,13.8890687487633,
132.557286539592)) ;
#114591=CARTESIAN_POINT('Ctrl Pts',(-13.3933038950219,13.6109288487181,
132.470050146704)) ;
#114592=CARTESIAN_POINT('Ctrl Pts',(-13.3996927101153,13.3205780973656,
132.455665139994)) ;
#114593=CARTESIAN_POINT('Ctrl Pts',(-13.4314451231204,13.0356410236252,
132.515132416829)) ;
#114594=CARTESIAN_POINT('Ctrl Pts',(-13.4863521726588,12.7811568557338,
132.642583088239)) ;
#114595=CARTESIAN_POINT('Ctrl Pts',(-13.5618719439237,12.5709851276515,
132.830045482527)) ;
#114596=CARTESIAN_POINT('Ctrl Pts',(-13.6530001533805,12.4221766619671,
133.063156221214)) ;
#114597=CARTESIAN_POINT('Ctrl Pts',(-13.7543438242653,12.3447406812541,
133.325997758698)) ;
#114598=CARTESIAN_POINT('Ctrl Pts',(-13.858979447707,12.3451621602759,133.598484050117)) ;
#114599=CARTESIAN_POINT('Ctrl Pts',(-13.9595871058779,12.4221617733591,
133.859413033911)) ;
#114600=CARTESIAN_POINT('Ctrl Pts',(-14.0509368702114,12.5713293574021,
134.093085140404)) ;
#114601=CARTESIAN_POINT('Ctrl Pts',(-14.1263288360547,12.7811357471148,
134.280239363245)) ;
#114602=CARTESIAN_POINT('Ctrl Pts',(-14.181464730297,13.037385413305,134.408146154191)) ;
#114603=CARTESIAN_POINT('Ctrl Pts',(-14.2129289597319,13.3202247802994,
134.46702998844)) ;
#114604=CARTESIAN_POINT('Ctrl Pts',(-14.2193168783918,13.6126649497902,
134.452393596522)) ;
#114605=CARTESIAN_POINT('Ctrl Pts',(-14.2008364796894,13.889109539137,134.365400616144)) ;
#114606=CARTESIAN_POINT('Ctrl Pts',(-14.1595000662705,14.1334576219234,
134.211477497111)) ;
#114607=CARTESIAN_POINT('Ctrl Pts',(-14.0992466494206,14.3262010857029,
134.002423062281)) ;
#114608=CARTESIAN_POINT('Ctrl Pts',(-14.0244678789738,14.4552702241494,
133.750713932904)) ;
#114609=CARTESIAN_POINT('Ctrl Pts',(-13.9418997721999,14.5094659873619,
133.476364746001)) ;
#114610=CARTESIAN_POINT('Ctrl Pts',(-13.8583861168424,14.48627928254,133.199410244325)) ;
#114611=CARTESIAN_POINT('Ctrl Pts',(-13.7797353567973,14.3867194330965,
132.936459435104)) ;
#114612=CARTESIAN_POINT('Ctrl Pts',(-13.7130105219871,14.2183273389604,
132.708437979387)) ;
#114613=CARTESIAN_POINT('Ctrl Pts',(-13.6633479068396,13.9922441011096,
132.530147180322)) ;
#114614=CARTESIAN_POINT('Ctrl Pts',(-13.6354328184579,13.7260908863955,
132.415503205816)) ;
#114615=CARTESIAN_POINT('Ctrl Pts',(-13.6315996421401,13.4392990683917,
132.371317925094)) ;
#114616=CARTESIAN_POINT('Ctrl Pts',(-13.6531002743803,13.1491383926391,
132.400878674979)) ;
#114617=CARTESIAN_POINT('Ctrl Pts',(-13.6988895423874,12.880138144259,132.501583429181)) ;
#114618=CARTESIAN_POINT('Ctrl Pts',(-13.7669016038619,12.6488312040692,
132.66702117208)) ;
#114619=CARTESIAN_POINT('Ctrl Pts',(-13.8519661020191,12.4746173052797,
132.882564533349)) ;
#114620=CARTESIAN_POINT('Ctrl Pts',(-13.9499918537797,12.3669410581914,
133.13572242046)) ;
#114621=CARTESIAN_POINT('Ctrl Pts',(-14.0540803057466,12.3355244467329,
133.406613758036)) ;
#114622=CARTESIAN_POINT('Ctrl Pts',(-14.1570770496498,12.3818824637266,
133.674448586604)) ;
#114623=CARTESIAN_POINT('Ctrl Pts',(-14.2529156063067,12.502442440452,133.921340780179)) ;
#114624=CARTESIAN_POINT('Ctrl Pts',(-14.3357164299663,12.6900860359651,
134.129966525958)) ;
#114625=CARTESIAN_POINT('Ctrl Pts',(-14.3993556473891,12.9290693621117,
134.282824648329)) ;
#114626=CARTESIAN_POINT('Ctrl Pts',(-14.4406746427025,13.2033802627449,
134.370454904131)) ;
#114627=CARTESIAN_POINT('Ctrl Pts',(-14.4573570221151,13.493885424346,134.386064394722)) ;
#114628=CARTESIAN_POINT('Ctrl Pts',(-14.4487939272164,13.7798208359641,
134.327863613174)) ;
#114629=CARTESIAN_POINT('Ctrl Pts',(-14.4163591296665,14.0398147256928,
134.199973199807)) ;
#114630=CARTESIAN_POINT('Ctrl Pts',(-14.3630430477874,14.2555980954836,
134.011057985321)) ;
#114631=CARTESIAN_POINT('Ctrl Pts',(-14.2938516112464,14.4112165057251,
133.775932908363)) ;
#114632=CARTESIAN_POINT('Ctrl Pts',(-14.213327419341,14.4969135755094,133.50736843725)) ;
#114633=CARTESIAN_POINT('Ctrl Pts',(-14.1296189321524,14.5049696810031,
133.229876903082)) ;
#114634=CARTESIAN_POINT('Ctrl Pts',(-14.0481698596881,14.4360249735447,
132.958821806314)) ;
#114635=CARTESIAN_POINT('Ctrl Pts',(-13.9759487851369,14.2945754362065,
132.714746600477)) ;
#114636=CARTESIAN_POINT('Ctrl Pts',(-13.9186392005941,14.0897548858671,
132.514089317548)) ;
#114637=CARTESIAN_POINT('Ctrl Pts',(-13.8816283734556,13.8387001375239,
132.372961040856)) ;
#114638=CARTESIAN_POINT('Ctrl Pts',(-13.86765973633,13.5574044598577,132.299056743724)) ;
#114639=CARTESIAN_POINT('Ctrl Pts',(-13.8789956043886,13.2644130009093,
132.2988381339)) ;
#114640=CARTESIAN_POINT('Ctrl Pts',(-13.9149994984909,12.9862195730077,
132.371090109727)) ;
#114641=CARTESIAN_POINT('Ctrl Pts',(-13.9743502243685,12.7371111819008,
132.511275565875)) ;
#114642=CARTESIAN_POINT('Ctrl Pts',(-14.0530557762854,12.5380203242925,
132.708138925323)) ;
#114643=CARTESIAN_POINT('Ctrl Pts',(-14.1469276806553,12.4015272632005,
132.949117652525)) ;
#114644=CARTESIAN_POINT('Ctrl Pts',(-14.2489833656644,12.3389470103484,
133.214189844898)) ;
#114645=CARTESIAN_POINT('Ctrl Pts',(-14.3533226131928,12.3537864997403,
133.485861761893)) ;
#114646=CARTESIAN_POINT('Ctrl Pts',(-14.4528614890508,12.4449099176858,
133.743576395913)) ;
#114647=CARTESIAN_POINT('Ctrl Pts',(-14.5418561425685,12.6072327563546,
133.97027761533)) ;
#114648=CARTESIAN_POINT('Ctrl Pts',(-14.6133813155202,12.8259751420657,
134.146289595912)) ;
#114649=CARTESIAN_POINT('Ctrl Pts',(-14.6644626717837,13.0894865209779,
134.262268329824)) ;
#114650=CARTESIAN_POINT('Ctrl Pts',(-14.6912354788188,13.3763086244584,
134.307339213758)) ;
#114651=CARTESIAN_POINT('Ctrl Pts',(-14.6927780845657,13.666102426872,134.278737035569)) ;
#114652=CARTESIAN_POINT('Ctrl Pts',(-14.6699098049705,13.9378774393092,
134.178922193569)) ;
#114653=CARTESIAN_POINT('Ctrl Pts',(-14.6244200591529,14.174793298913,134.012730262355)) ;
#114654=CARTESIAN_POINT('Ctrl Pts',(-14.5612019536203,14.355667987911,133.795095051057)) ;
#114655=CARTESIAN_POINT('Ctrl Pts',(-14.4846906294762,14.4711053294092,
133.538428577137)) ;
#114656=CARTESIAN_POINT('Ctrl Pts',(-14.4011850462511,14.511170979715,133.261273870169)) ;
#114657=CARTESIAN_POINT('Ctrl Pts',(-14.3178410780268,14.4729025341711,
132.984673903261)) ;
#114658=CARTESIAN_POINT('Ctrl Pts',(-14.2414431710577,14.3605014183323,
132.728538157581)) ;
#114659=CARTESIAN_POINT('Ctrl Pts',(-14.1770966200207,14.1789799497678,
132.507210107387)) ;
#114660=CARTESIAN_POINT('Ctrl Pts',(-14.1315848885081,13.9453130755044,
132.341277366815)) ;
#114661=CARTESIAN_POINT('Ctrl Pts',(-14.1079390036142,13.673613297581,132.239086339493)) ;
#114662=CARTESIAN_POINT('Ctrl Pts',(-14.1087830481224,13.3843416477693,
132.208491884339)) ;
#114663=CARTESIAN_POINT('Ctrl Pts',(-14.1351400941846,13.0956424787648,
132.252157038047)) ;
#114664=CARTESIAN_POINT('Ctrl Pts',(-14.1851403795369,12.8335787485534,
132.365283706234)) ;
#114665=CARTESIAN_POINT('Ctrl Pts',(-14.2566883427613,12.6116522531053,
132.541092961402)) ;
#114666=CARTESIAN_POINT('Ctrl Pts',(-14.3449178102994,12.4486058050818,
132.765728820733)) ;
#114667=CARTESIAN_POINT('Ctrl Pts',(-14.4444094609299,12.3551665981467,
133.023238128206)) ;
#114668=CARTESIAN_POINT('Ctrl Pts',(-14.5487260750023,12.3383111368361,
133.294844327139)) ;
#114669=CARTESIAN_POINT('Ctrl Pts',(-14.651135777708,12.3991318667188,133.560878201396)) ;
#114670=CARTESIAN_POINT('Ctrl Pts',(-14.7450247980916,12.5336133546432,
133.801997324254)) ;
#114671=CARTESIAN_POINT('Ctrl Pts',(-14.8240658891889,12.7304747525644,
133.999922781035)) ;
#114672=CARTESIAN_POINT('Ctrl Pts',(-14.8843591623108,12.9801493565206,
134.142645016146)) ;
#114673=CARTESIAN_POINT('Ctrl Pts',(-14.9207776314118,13.2569930870622,
134.216214669517)) ;
#114674=CARTESIAN_POINT('Ctrl Pts',(-14.9327904526555,13.5493201067258,
134.218039568247)) ;
#114675=CARTESIAN_POINT('Ctrl Pts',(-14.9195608823309,13.8310609228274,
134.146315593606)) ;
#114676=CARTESIAN_POINT('Ctrl Pts',(-14.8829071658904,14.0843638099265,
134.006060198745)) ;
#114677=CARTESIAN_POINT('Ctrl Pts',(-14.8262774665716,14.2896244491401,
133.807537482938)) ;
#114678=CARTESIAN_POINT('Ctrl Pts',(-14.7544509561564,14.4330063116879,
133.564623744753)) ;
#114679=CARTESIAN_POINT('Ctrl Pts',(-14.6730981695364,14.5042107415309,
133.293824015626)) ;
#114680=CARTESIAN_POINT('Ctrl Pts',(-14.5890044461905,14.4979449999679,
133.015056574469)) ;
#114681=CARTESIAN_POINT('Ctrl Pts',(-14.5085811345525,14.4144601779744,
132.746912885546)) ;
#114682=CARTESIAN_POINT('Ctrl Pts',(-14.4386966820867,14.2595209902124,
132.509575163383)) ;
#114683=CARTESIAN_POINT('Ctrl Pts',(-14.3852681727933,14.046214919979,132.32053362023)) ;
#114684=CARTESIAN_POINT('Ctrl Pts',(-14.3521879692475,13.7868053449528,
132.190703349274)) ;
#114685=CARTESIAN_POINT('Ctrl Pts',(-14.3429850788203,13.5027357390144,
132.130803960272)) ;
#114686=CARTESIAN_POINT('Ctrl Pts',(-14.3589256787532,13.2114164567146,
132.144166678592)) ;
#114687=CARTESIAN_POINT('Ctrl Pts',(-14.3996479591576,12.9359342983456,
132.230005501464)) ;
#114688=CARTESIAN_POINT('Ctrl Pts',(-14.4630310316759,12.6951562018299,
132.381999972268)) ;
#114689=CARTESIAN_POINT('Ctrl Pts',(-14.5447779273386,12.5073061272103,
132.587797294127)) ;
#114690=CARTESIAN_POINT('Ctrl Pts',(-14.6405874915994,12.3841592686752,
132.834495044115)) ;
#114691=CARTESIAN_POINT('Ctrl Pts',(-14.7436396651289,12.3356200239572,
133.102447533053)) ;
#114692=CARTESIAN_POINT('Ctrl Pts',(-14.8482334000072,12.3655842279676,
133.374661826652)) ;
#114693=CARTESIAN_POINT('Ctrl Pts',(-14.9456378863924,12.4702048591763,
133.62631542447)) ;
#114694=CARTESIAN_POINT('Ctrl Pts',(-15.032031341998,12.6448837976238,133.845354670619)) ;
#114695=CARTESIAN_POINT('Ctrl Pts',(-15.0997909854076,12.872508423284,134.010430965611)) ;
#114696=CARTESIAN_POINT('Ctrl Pts',(-15.1466624677231,13.1434988331289,
134.11394299587)) ;
#114697=CARTESIAN_POINT('Ctrl Pts',(-15.1684830221252,13.4301737780494,
134.144821454034)) ;
#114698=CARTESIAN_POINT('Ctrl Pts',(-15.1655029363779,13.7187795914099,
134.102960274335)) ;
#114699=CARTESIAN_POINT('Ctrl Pts',(-15.137871807278,13.9870154433738,133.988964277523)) ;
#114700=CARTESIAN_POINT('Ctrl Pts',(-15.089103500937,14.2124398345738,133.813561355081)) ;
#114701=CARTESIAN_POINT('Ctrl Pts',(-15.0226861816082,14.3830654461858,
133.586365342099)) ;
#114702=CARTESIAN_POINT('Ctrl Pts',(-14.9442977084689,14.4846609541733,
133.324197217531)) ;
#114703=CARTESIAN_POINT('Ctrl Pts',(-14.8603045751173,14.5097913616969,
133.045629352813)) ;
#114704=CARTESIAN_POINT('Ctrl Pts',(-14.7781158124174,14.4576093080194,
132.772584210679)) ;
#114705=CARTESIAN_POINT('Ctrl Pts',(-14.7029379087114,14.3304831317374,
132.519675058584)) ;
#114706=CARTESIAN_POINT('Ctrl Pts',(-14.6421746060609,14.1386183822934,
132.309056084948)) ;
#114707=CARTESIAN_POINT('Ctrl Pts',(-14.6004669656827,13.8965846856625,
132.154209706835)) ;
#114708=CARTESIAN_POINT('Ctrl Pts',(-14.5812880337956,13.6198365630073,
132.065057969682)) ;
#114709=CARTESIAN_POINT('Ctrl Pts',(-14.5869544254102,13.3288844737818,
132.048478781958)) ;
#114710=CARTESIAN_POINT('Ctrl Pts',(-14.6178077703533,13.0447399832046,
132.105475686592)) ;
#114711=CARTESIAN_POINT('Ctrl Pts',(-14.6721136258845,12.7881836368688,
132.231068090543)) ;
#114712=CARTESIAN_POINT('Ctrl Pts',(-14.7475386699193,12.5755910115287,
132.418091523374)) ;
#114713=CARTESIAN_POINT('Ctrl Pts',(-14.8378940236856,12.4257574465567,
132.649102005788)) ;
#114714=CARTESIAN_POINT('Ctrl Pts',(-14.9388209084364,12.3460112405744,
132.910787274949)) ;
#114715=CARTESIAN_POINT('Ctrl Pts',(-15.0435737078647,12.3439532504127,
133.183578235088)) ;
#114716=CARTESIAN_POINT('Ctrl Pts',(-15.1446091167616,12.4188218900739,
133.445686307793)) ;
#114717=CARTESIAN_POINT('Ctrl Pts',(-15.2365998734713,12.5668341062151,
133.681113263233)) ;
#114718=CARTESIAN_POINT('Ctrl Pts',(-15.3120455807105,12.7739565310488,
133.868616342754)) ;
#114719=CARTESIAN_POINT('Ctrl Pts',(-15.3679671650309,13.0292275295923,
133.998784482597)) ;
#114720=CARTESIAN_POINT('Ctrl Pts',(-15.4001513908772,13.3121167714202,
134.059708256056)) ;
#114721=CARTESIAN_POINT('Ctrl Pts',(-15.407302294284,13.6036711588795,134.047415072482)) ;
#114722=CARTESIAN_POINT('Ctrl Pts',(-15.3894117903854,13.8822010088686,
133.961971555951)) ;
#114723=CARTESIAN_POINT('Ctrl Pts',(-15.3488581880954,14.126534024312,133.810499271449)) ;
#114724=CARTESIAN_POINT('Ctrl Pts',(-15.2890058404676,14.3215277156221,
133.602541497692)) ;
#114725=CARTESIAN_POINT('Ctrl Pts',(-15.2146261037101,14.4523872469144,
133.352036701433)) ;
#114726=CARTESIAN_POINT('Ctrl Pts',(-15.132276398967,14.509081269933,133.078352393805)) ;
#114727=CARTESIAN_POINT('Ctrl Pts',(-15.048156334803,14.4877530584647,132.799404216537)) ;
#114728=CARTESIAN_POINT('Ctrl Pts',(-14.9697741972722,14.3906972492053,
132.537447195776)) ;
#114729=CARTESIAN_POINT('Ctrl Pts',(-14.9025432118204,14.2242127265294,
132.307919886886)) ;
#114730=CARTESIAN_POINT('Ctrl Pts',(-14.8524134830202,14.0000453961231,
132.128331876439)) ;
#114731=CARTESIAN_POINT('Ctrl Pts',(-14.8236827135926,13.7349941187306,
132.011308130338)) ;
#114732=CARTESIAN_POINT('Ctrl Pts',(-14.8192110157222,13.4462938086935,
131.964998461715)) ;
#114733=CARTESIAN_POINT('Ctrl Pts',(-14.8397608257614,13.1586524064852,
131.992109164985)) ;
#114734=CARTESIAN_POINT('Ctrl Pts',(-14.8852506544382,12.8863235925418,
132.091631205511)) ;
#114735=CARTESIAN_POINT('Ctrl Pts',(-14.952306886852,12.6553854575325,132.254505839022)) ;
#114736=CARTESIAN_POINT('Ctrl Pts',(-15.036993538522,12.4787538591612,132.468885463633)) ;
#114737=CARTESIAN_POINT('Ctrl Pts',(-15.1351325127102,12.3688114822916,
132.722256615459)) ;
#114738=CARTESIAN_POINT('Ctrl Pts',(-15.2387002100067,12.3354319136936,
132.991765834986)) ;
#114739=CARTESIAN_POINT('Ctrl Pts',(-15.3419020299315,12.3792576310417,
133.260178529464)) ;
#114740=CARTESIAN_POINT('Ctrl Pts',(-15.4385746866519,12.4988398999205,
133.509304414363)) ;
#114741=CARTESIAN_POINT('Ctrl Pts',(-15.5211785051019,12.6835118512005,
133.71760539492)) ;
#114742=CARTESIAN_POINT('Ctrl Pts',(-15.585614912484,12.9214923912795,133.872725040323)) ;
#114743=CARTESIAN_POINT('Ctrl Pts',(-15.6276593796861,13.1954916424955,
133.96242929729)) ;
#114744=CARTESIAN_POINT('Ctrl Pts',(-15.6450448286836,13.4865485670219,
133.980012149667)) ;
#114745=CARTESIAN_POINT('Ctrl Pts',(-15.6370948847114,13.772471589557,133.923647448758)) ;
#114746=CARTESIAN_POINT('Ctrl Pts',(-15.6054576941134,14.0322259092952,
133.798239163953)) ;
#114747=CARTESIAN_POINT('Ctrl Pts',(-15.5528532090993,14.2496185339524,
133.611440842472)) ;
#114748=CARTESIAN_POINT('Ctrl Pts',(-15.483617346609,14.4079186586772,133.375986031408)) ;
#114749=CARTESIAN_POINT('Ctrl Pts',(-15.4040148005417,14.495128940057,133.110405781656)) ;
#114750=CARTESIAN_POINT('Ctrl Pts',(-15.3198980850125,14.5060206783235,
132.831544484233)) ;
#114751=CARTESIAN_POINT('Ctrl Pts',(-15.2380342056834,14.4388851972431,
132.55918054693)) ;
#114752=CARTESIAN_POINT('Ctrl Pts',(-15.1654389797841,14.2990479598781,
132.313981427395)) ;
#114753=CARTESIAN_POINT('Ctrl Pts',(-15.107816605712,14.096277092635,132.112499036057)) ;
#114754=CARTESIAN_POINT('Ctrl Pts',(-15.0701124492741,13.8463552274942,
131.969338122834)) ;
#114755=CARTESIAN_POINT('Ctrl Pts',(-15.05554407707,13.5643762793268,131.893541407323)) ;
#114756=CARTESIAN_POINT('Ctrl Pts',(-15.0659585050918,13.2747380866486,
131.891020251149)) ;
#114757=CARTESIAN_POINT('Ctrl Pts',(-15.101446630055,12.9934296976024,131.961474427387)) ;
#114758=CARTESIAN_POINT('Ctrl Pts',(-15.1601039100246,12.7438068041656,
132.099715492444)) ;
#114759=CARTESIAN_POINT('Ctrl Pts',(-15.2384724882155,12.5426943442427,
132.295520501906)) ;
#114760=CARTESIAN_POINT('Ctrl Pts',(-15.3316626347415,12.4046936236787,
132.534630966333)) ;
#114761=CARTESIAN_POINT('Ctrl Pts',(-15.4337983976848,12.3396331759052,
132.799852893319)) ;
#114762=CARTESIAN_POINT('Ctrl Pts',(-15.5380451833256,12.3522550875064,
133.071297592341)) ;
#114763=CARTESIAN_POINT('Ctrl Pts',(-15.6378149553019,12.441158614988,133.329684714748)) ;
#114764=CARTESIAN_POINT('Ctrl Pts',(-15.7271824288003,12.6013769713038,
133.55749869446)) ;
#114765=CARTESIAN_POINT('Ctrl Pts',(-15.799387164279,12.819071640269,133.735430014399)) ;
#114766=CARTESIAN_POINT('Ctrl Pts',(-15.8509954325536,13.0807346140254,
133.853055281245)) ;
#114767=CARTESIAN_POINT('Ctrl Pts',(-15.8785701981475,13.3675408612144,
133.900413861765)) ;
#114768=CARTESIAN_POINT('Ctrl Pts',(-15.880950069095,13.6570979280699,133.874320504545)) ;
#114769=CARTESIAN_POINT('Ctrl Pts',(-15.8584614917164,13.9319893911641,
133.775308859387)) ;
#114770=CARTESIAN_POINT('Ctrl Pts',(-15.8140300794619,14.1676085258846,
133.612576918087)) ;
#114771=CARTESIAN_POINT('Ctrl Pts',(-15.7508365618172,14.3519029604138,
133.394745430706)) ;
#114772=CARTESIAN_POINT('Ctrl Pts',(-15.6747542377325,14.4687263868581,
133.139424327783)) ;
#114773=CARTESIAN_POINT('Ctrl Pts',(-15.5916310901521,14.5110206744739,
132.86348513324)) ;
#114774=CARTESIAN_POINT('Ctrl Pts',(-15.5082277554707,14.4754839101951,
132.586740900539)) ;
#114775=CARTESIAN_POINT('Ctrl Pts',(-15.4310148106346,14.3641243881349,
132.327975519891)) ;
#114776=CARTESIAN_POINT('Ctrl Pts',(-15.366796148105,14.1859981150162,132.10732571318)) ;
#114777=CARTESIAN_POINT('Ctrl Pts',(-15.3203690301936,13.9527739629267,
131.938549874937)) ;
#114778=CARTESIAN_POINT('Ctrl Pts',(-15.2960642034895,13.6818171869407,
131.83443758756)) ;
#114779=CARTESIAN_POINT('Ctrl Pts',(-15.2962284106988,13.3923456599437,
131.801803057666)) ;
#114780=CARTESIAN_POINT('Ctrl Pts',(-15.3217088635482,13.1044625348289,
131.843052348479)) ;
#114781=CARTESIAN_POINT('Ctrl Pts',(-15.3712895624886,12.8400820200563,
131.954780479996)) ;
#114782=CARTESIAN_POINT('Ctrl Pts',(-15.4421215709794,12.6174283224968,
132.128595071256)) ;
#114783=CARTESIAN_POINT('Ctrl Pts',(-15.5300656767636,12.4521814963559,
132.352341736955)) ;
#114784=CARTESIAN_POINT('Ctrl Pts',(-15.6293654089259,12.3567835155047,
132.609283754024)) ;
#114785=CARTESIAN_POINT('Ctrl Pts',(-15.7333497867975,12.3377092271658,
132.880009523703)) ;
#114786=CARTESIAN_POINT('Ctrl Pts',(-15.8360089773108,12.3962076032604,
133.146742886939)) ;
#114787=CARTESIAN_POINT('Ctrl Pts',(-15.930453723468,12.5290432373042,133.389409066584)) ;
#114788=CARTESIAN_POINT('Ctrl Pts',(-16.009869584066,12.7244085230837,133.588441629327)) ;
#114789=CARTESIAN_POINT('Ctrl Pts',(-16.0704566796156,12.9709500550387,
133.732258312717)) ;
#114790=CARTESIAN_POINT('Ctrl Pts',(-16.1079755146477,13.2494402817627,
133.808760193825)) ;
#114791=CARTESIAN_POINT('Ctrl Pts',(-16.1205567949924,13.5418967084717,
133.812230503726)) ;
#114792=CARTESIAN_POINT('Ctrl Pts',(-16.1080660019669,13.8230883914708,
133.742789063125)) ;
#114793=CARTESIAN_POINT('Ctrl Pts',(-16.0720612901439,14.0775910910953,
133.604421793909)) ;
#114794=CARTESIAN_POINT('Ctrl Pts',(-16.016031312662,14.2842118886259,133.407692540579)) ;
#114795=CARTESIAN_POINT('Ctrl Pts',(-15.9444811188164,14.4299775435325,
133.165534218954)) ;
#114796=CARTESIAN_POINT('Ctrl Pts',(-15.8629277653847,14.503331032243,132.894001914259)) ;
#114797=CARTESIAN_POINT('Ctrl Pts',(-15.7793496289803,14.4992417837061,
132.616952244808)) ;
#114798=CARTESIAN_POINT('Ctrl Pts',(-15.6984734089822,14.4177939822546,
132.347381532007)) ;
#114799=CARTESIAN_POINT('Ctrl Pts',(-15.6283650852396,14.2650806147523,
132.109470216545)) ;
#114800=CARTESIAN_POINT('Ctrl Pts',(-15.5743268050137,14.0529681509037,
131.918590385591)) ;
#114801=CARTESIAN_POINT('Ctrl Pts',(-15.5406403700371,13.7955270319932,
131.787101135372)) ;
#114802=CARTESIAN_POINT('Ctrl Pts',(-15.5306638256876,13.5095709535078,
131.724666349948)) ;
#114803=CARTESIAN_POINT('Ctrl Pts',(-15.5460171831695,13.2189036520177,
131.736403340103)) ;
#114804=CARTESIAN_POINT('Ctrl Pts',(-15.5859137154081,12.9437120966298,
131.819943466577)) ;
#114805=CARTESIAN_POINT('Ctrl Pts',(-15.6485475179313,12.7018113312773,
131.969792071976)) ;
#114806=CARTESIAN_POINT('Ctrl Pts',(-15.7301725881226,12.5115374792667,
132.175093619939)) ;
#114807=CARTESIAN_POINT('Ctrl Pts',(-15.8255194984171,12.3865362509785,
132.420501324227)) ;
#114808=CARTESIAN_POINT('Ctrl Pts',(-15.9289904176059,12.3360647683775,
132.689500393083)) ;
#114809=CARTESIAN_POINT('Ctrl Pts',(-16.0322109432962,12.3630945002041,
132.958176956719)) ;
#114810=CARTESIAN_POINT('Ctrl Pts',(-16.1310535797055,12.4665769548229,
133.213630713827)) ;
#114811=CARTESIAN_POINT('Ctrl Pts',(-16.2171162898203,12.637873730405,133.432016347732)) ;
#114812=CARTESIAN_POINT('Ctrl Pts',(-16.2861070614099,12.8661806742055,
133.600365416687)) ;
#114813=CARTESIAN_POINT('Ctrl Pts',(-16.3331577984964,13.1333277515124,
133.704775971435)) ;
#114814=CARTESIAN_POINT('Ctrl Pts',(-16.3560616077762,13.4221934836715,
133.738517459493)) ;
#114815=CARTESIAN_POINT('Ctrl Pts',(-16.3536937500244,13.7107571318464,
133.698487549138)) ;
#114816=CARTESIAN_POINT('Ctrl Pts',(-16.3267795290435,13.9798563780996,
133.58659147111)) ;
#114817=CARTESIAN_POINT('Ctrl Pts',(-16.2784408821239,14.2070905580459,
133.412375341533)) ;
#114818=CARTESIAN_POINT('Ctrl Pts',(-16.2125397227886,14.3790287482914,
133.186748864503)) ;
#114819=CARTESIAN_POINT('Ctrl Pts',(-16.1346594708171,14.4826462514907,
132.926162382995)) ;
#114820=CARTESIAN_POINT('Ctrl Pts',(-16.0504302213959,14.5101765749395,
132.646782279628)) ;
#114821=CARTESIAN_POINT('Ctrl Pts',(-15.9682674268405,14.4602521093363,
132.373878730922)) ;
#114822=CARTESIAN_POINT('Ctrl Pts',(-15.892694390541,14.3349863303821,132.119771873462)) ;
#114823=CARTESIAN_POINT('Ctrl Pts',(-15.8317129503708,14.1459036519263,
131.908681279387)) ;
#114824=CARTESIAN_POINT('Ctrl Pts',(-15.7891216920241,13.9042674567381,
131.751109063095)) ;
#114825=CARTESIAN_POINT('Ctrl Pts',(-15.7692741641614,13.6274934121279,
131.659929127433)) ;
#114826=CARTESIAN_POINT('Ctrl Pts',(-15.774240842792,13.3375401227482,131.641402457855)) ;
#114827=CARTESIAN_POINT('Ctrl Pts',(-15.8042482653973,13.0529656397982,
131.695949415826)) ;
#114828=CARTESIAN_POINT('Ctrl Pts',(-15.8584516986935,12.793542004979,131.820979830249)) ;
#114829=CARTESIAN_POINT('Ctrl Pts',(-15.9326864597706,12.5815361452067,
132.004842248444)) ;
#114830=CARTESIAN_POINT('Ctrl Pts',(-16.0230837910625,12.4287258471182,
132.235797836759)) ;
#114831=CARTESIAN_POINT('Ctrl Pts',(-16.1240643432101,12.3470719994747,
132.497574210549)) ;
#114832=CARTESIAN_POINT('Ctrl Pts',(-16.2285925774014,12.3430683223392,
132.769776197563)) ;
#114833=CARTESIAN_POINT('Ctrl Pts',(-16.3294552263757,12.4155936091128,
133.031491197843)) ;
#114834=CARTESIAN_POINT('Ctrl Pts',(-16.42158697565,12.5608875783812,133.267432939441)) ;
#114835=CARTESIAN_POINT('Ctrl Pts',(-16.4979791687381,12.7672957855937,
133.457539227448)) ;
#114836=CARTESIAN_POINT('Ctrl Pts',(-16.5545469684218,13.0219896288371,
133.589546147221)) ;
#114837=CARTESIAN_POINT('Ctrl Pts',(-16.5873216769804,13.3035436342973,
133.652289558074)) ;
#114838=CARTESIAN_POINT('Ctrl Pts',(-16.5952372158022,13.5948422510341,
133.642264450776)) ;
#114839=CARTESIAN_POINT('Ctrl Pts',(-16.5781262828345,13.8739529691167,
133.559117325056)) ;
#114840=CARTESIAN_POINT('Ctrl Pts',(-16.5380768677347,14.1203174233417,
133.409012301568)) ;
#114841=CARTESIAN_POINT('Ctrl Pts',(-16.4787184094645,14.3167168643634,
133.20251930448)) ;
#114842=CARTESIAN_POINT('Ctrl Pts',(-16.4048795075091,14.4494066861711,
132.953678390524)) ;
#114843=CARTESIAN_POINT('Ctrl Pts',(-16.3225697948458,14.5084702688582,
132.680063070833)) ;
#114844=CARTESIAN_POINT('Ctrl Pts',(-16.2386731326133,14.489700746972,132.401879914645)) ;
#114845=CARTESIAN_POINT('Ctrl Pts',(-16.159666302226,14.3946106074975,132.13794942029)) ;
#114846=CARTESIAN_POINT('Ctrl Pts',(-16.0919372674924,14.2294635345246,
131.906906848158)) ;
#114847=CARTESIAN_POINT('Ctrl Pts',(-16.0414142644033,14.0073333887475,
131.726263966149)) ;
#114848=CARTESIAN_POINT('Ctrl Pts',(-16.0120005571222,13.7435828448799,
131.607279354952)) ;
#114849=CARTESIAN_POINT('Ctrl Pts',(-16.0067413555039,13.454824745877,131.558621231445)) ;
#114850=CARTESIAN_POINT('Ctrl Pts',(-16.0266816029947,13.1663898496403,
131.58388276017)) ;
#114851=CARTESIAN_POINT('Ctrl Pts',(-16.071174096646,12.8948251888563,131.680693404511)) ;
#114852=CARTESIAN_POINT('Ctrl Pts',(-16.1378143759152,12.6613614393991,
131.842219614895)) ;
#114853=CARTESIAN_POINT('Ctrl Pts',(-16.2222899580583,12.4827884864443,
132.055914031115)) ;
#114854=CARTESIAN_POINT('Ctrl Pts',(-16.3195947643377,12.3713198999723,
132.307032186213)) ;
#114855=CARTESIAN_POINT('Ctrl Pts',(-16.42316155049,12.3351536539427,132.576506572357)) ;
#114856=CARTESIAN_POINT('Ctrl Pts',(-16.5269587087536,12.3771106003778,
132.846499102918)) ;
#114857=CARTESIAN_POINT('Ctrl Pts',(-16.6232634802675,12.493746042562,133.094781650953)) ;
#114858=CARTESIAN_POINT('Ctrl Pts',(-16.7066715515362,12.6767291405437,
133.30534152523)) ;
#114859=CARTESIAN_POINT('Ctrl Pts',(-16.7719969184263,12.9147362953278,
133.462888792416)) ;
#114860=CARTESIAN_POINT('Ctrl Pts',(-16.8145117924752,13.1870897175325,
133.554081812245)) ;
#114861=CARTESIAN_POINT('Ctrl Pts',(-16.832664410647,13.4771402294594,133.573993886311)) ;
#114862=CARTESIAN_POINT('Ctrl Pts',(-16.8255195547471,13.7642376991577,
133.519905575425)) ;
#114863=CARTESIAN_POINT('Ctrl Pts',(-16.7943070458963,14.0261140050281,
133.395578546783)) ;
#114864=CARTESIAN_POINT('Ctrl Pts',(-16.7424882598997,14.2437566095146,
133.211251228587)) ;
#114865=CARTESIAN_POINT('Ctrl Pts',(-16.6736113908412,14.4043004510961,
132.976804095223)) ;
#114866=CARTESIAN_POINT('Ctrl Pts',(-16.5942186823598,14.4936451763547,
132.711836822872)) ;
#114867=CARTESIAN_POINT('Ctrl Pts',(-16.5101466580755,14.5067755223083,
132.433108081231)) ;
#114868=CARTESIAN_POINT('Ctrl Pts',(-16.4282410882398,14.4421251633059,
132.160681842967)) ;
#114869=CARTESIAN_POINT('Ctrl Pts',(-16.3551632521983,14.3039891726026,
131.914003956164)) ;
#114870=CARTESIAN_POINT('Ctrl Pts',(-16.2972497108617,14.1040922169467,
131.711842779145)) ;
#114871=CARTESIAN_POINT('Ctrl Pts',(-16.2585983326173,13.8535852347893,
131.565668552377)) ;
#114872=CARTESIAN_POINT('Ctrl Pts',(-16.243420453165,13.5730952435811,131.488208101679)) ;
#114873=CARTESIAN_POINT('Ctrl Pts',(-16.2531006198612,13.2829861782011,
131.483481649537)) ;
#114874=CARTESIAN_POINT('Ctrl Pts',(-16.2877661805878,13.0017737284941,
131.551621835108)) ;
#114875=CARTESIAN_POINT('Ctrl Pts',(-16.3459738367156,12.7500890797144,
131.688431825914)) ;
#114876=CARTESIAN_POINT('Ctrl Pts',(-16.4238184818004,12.5475577998432,
131.882729415997)) ;
#114877=CARTESIAN_POINT('Ctrl Pts',(-16.5167586194788,12.4075652478031,
132.121078295711)) ;
#114878=CARTESIAN_POINT('Ctrl Pts',(-16.6183907518262,12.3405227377109,
132.384938789592)) ;
#114879=CARTESIAN_POINT('Ctrl Pts',(-16.7229364475564,12.3506975715296,
132.657173213167)) ;
#114880=CARTESIAN_POINT('Ctrl Pts',(-16.8232859030364,12.438177489278,132.917122022405)) ;
#114881=CARTESIAN_POINT('Ctrl Pts',(-16.9125712124386,12.5958827964123,
133.1448620791)) ;
#114882=CARTESIAN_POINT('Ctrl Pts',(-16.9854582743437,12.8123887822574,
133.324729525533)) ;
#114883=CARTESIAN_POINT('Ctrl Pts',(-17.037709893631,13.0732934241726,133.444215844693)) ;
#114884=CARTESIAN_POINT('Ctrl Pts',(-17.0659638164382,13.3601444544887,
133.493509177191)) ;
#114885=CARTESIAN_POINT('Ctrl Pts',(-17.0689675284249,13.6487324697402,
133.469363185352)) ;
#114886=CARTESIAN_POINT('Ctrl Pts',(-17.0474035047278,13.9231969052117,
133.37321432911)) ;
#114887=CARTESIAN_POINT('Ctrl Pts',(-17.0033733673897,14.1616648845749,
133.211459633651)) ;
#114888=CARTESIAN_POINT('Ctrl Pts',(-16.9406158991401,14.3474885130478,
132.994912465869)) ;
#114889=CARTESIAN_POINT('Ctrl Pts',(-16.864876505793,14.4664584587802,132.740606759249)) ;
#114890=CARTESIAN_POINT('Ctrl Pts',(-16.7814776117931,14.5109046603937,
132.463712586271)) ;
#114891=CARTESIAN_POINT('Ctrl Pts',(-16.6983907346783,14.477538406395,132.188050973166)) ;
#114892=CARTESIAN_POINT('Ctrl Pts',(-16.6207705482251,14.3681997132881,
131.928042842248)) ;
#114893=CARTESIAN_POINT('Ctrl Pts',(-16.5561356079281,14.19161807787,131.706168442298)) ;
#114894=CARTESIAN_POINT('Ctrl Pts',(-16.5092308734292,13.9603524956053,
131.536079167786)) ;
#114895=CARTESIAN_POINT('Ctrl Pts',(-16.4841796106604,13.6895220911817,
131.429699941359)) ;
#114896=CARTESIAN_POINT('Ctrl Pts',(-16.4836919093705,13.4007319641459,
131.395211960917)) ;
#114897=CARTESIAN_POINT('Ctrl Pts',(-16.5082964988508,13.1132078283894,
131.433992211526)) ;
#114898=CARTESIAN_POINT('Ctrl Pts',(-16.5574784700436,12.8466068578935,
131.544388229293)) ;
#114899=CARTESIAN_POINT('Ctrl Pts',(-16.6273997075169,12.6236984730367,
131.715716955648)) ;
#114900=CARTESIAN_POINT('Ctrl Pts',(-16.7150468521775,12.4561011970055,
131.938529922164)) ;
#114901=CARTESIAN_POINT('Ctrl Pts',(-16.8139682824648,12.3585968124196,
132.194412407875)) ;
#114902=CARTESIAN_POINT('Ctrl Pts',(-16.9182265147246,12.3371246735504,
132.465833558649)) ;
#114903=CARTESIAN_POINT('Ctrl Pts',(-17.0209026074425,12.3935413485491,
132.732653318412)) ;
#114904=CARTESIAN_POINT('Ctrl Pts',(-17.1153756443262,12.5236723848828,
132.975519307564)) ;
#114905=CARTESIAN_POINT('Ctrl Pts',(-17.1956555914022,12.7179304240541,
133.176947444366)) ;
#114906=CARTESIAN_POINT('Ctrl Pts',(-17.2569924030211,12.9643000603806,
133.322838842009)) ;
#114907=CARTESIAN_POINT('Ctrl Pts',(-17.2949538933717,13.2410161239663,
133.400773057716)) ;
#114908=CARTESIAN_POINT('Ctrl Pts',(-17.3083412632257,13.5320326358814,
133.40675253041)) ;
#114909=CARTESIAN_POINT('Ctrl Pts',(-17.2965889183178,13.8151976332958,
133.339306952295)) ;
#114910=CARTESIAN_POINT('Ctrl Pts',(-17.2611712342104,14.070965110173,133.202631251777)) ;
#114911=CARTESIAN_POINT('Ctrl Pts',(-17.2055219190199,14.2795161854134,
133.006946181317)) ;
#114912=CARTESIAN_POINT('Ctrl Pts',(-17.1344526197165,14.4266233568165,
132.766264881813)) ;
#114913=CARTESIAN_POINT('Ctrl Pts',(-17.0535835623515,14.5021444966585,
132.496922447555)) ;
#114914=CARTESIAN_POINT('Ctrl Pts',(-16.9693534559784,14.5004799279669,
132.217713549754)) ;
#114915=CARTESIAN_POINT('Ctrl Pts',(-16.8885085804287,14.4210758361391,
131.948320350664)) ;
#114916=CARTESIAN_POINT('Ctrl Pts',(-16.818249196986,14.2711637356508,131.710095463003)) ;
#114917=CARTESIAN_POINT('Ctrl Pts',(-16.7633840110066,14.0600320259714,
131.516677712646)) ;
#114918=CARTESIAN_POINT('Ctrl Pts',(-16.729034656478,13.8025046463563,131.383125760343)) ;
#114919=CARTESIAN_POINT('Ctrl Pts',(-16.7184105236858,13.5194350300881,
131.319077858953)) ;
#114920=CARTESIAN_POINT('Ctrl Pts',(-16.7329082611137,13.227929848522,131.328230796269)) ;
#114921=CARTESIAN_POINT('Ctrl Pts',(-16.7721540100418,12.9514279979351,
131.409809044102)) ;
#114922=CARTESIAN_POINT('Ctrl Pts',(-16.834426980546,12.7076270254922,131.558495828173)) ;
#114923=CARTESIAN_POINT('Ctrl Pts',(-16.9152315370478,12.5164543914562,
131.761543944961)) ;
#114924=CARTESIAN_POINT('Ctrl Pts',(-17.0104958015721,12.3891143889345,
132.006622580848)) ;
#114925=CARTESIAN_POINT('Ctrl Pts',(-17.1132917121907,12.3364756158918,
132.273826383176)) ;
#114926=CARTESIAN_POINT('Ctrl Pts',(-17.2173332534644,12.3612642231578,
132.54465957405)) ;
#114927=CARTESIAN_POINT('Ctrl Pts',(-17.3163641429157,12.4629838840005,
132.800676032605)) ;
#114928=CARTESIAN_POINT('Ctrl Pts',(-17.4026407183266,12.6321971699934,
133.01975282772)) ;
#114929=CARTESIAN_POINT('Ctrl Pts',(-17.472100457449,12.8584558798932,133.189548524182)) ;
#114930=CARTESIAN_POINT('Ctrl Pts',(-17.5200564206003,13.1261648647243,
133.296424663186)) ;
#114931=CARTESIAN_POINT('Ctrl Pts',(-17.5435329958318,13.4141234552309,
133.331916813786)) ;
#114932=CARTESIAN_POINT('Ctrl Pts',(-17.5418705107985,13.7023852342343,
133.294006470842)) ;
#114933=CARTESIAN_POINT('Ctrl Pts',(-17.515866367185,13.9714212012371,133.184910655295)) ;
#114934=CARTESIAN_POINT('Ctrl Pts',(-17.4677121548387,14.202020081249,133.01095053406)) ;
#114935=CARTESIAN_POINT('Ctrl Pts',(-17.4023716167183,14.3750071736422,
132.787065724901)) ;
#114936=CARTESIAN_POINT('Ctrl Pts',(-17.3247668097447,14.4806351346196,
132.527282453733)) ;
#114937=CARTESIAN_POINT('Ctrl Pts',(-17.2410054869792,14.5105855297535,
132.24943004058)) ;
#114938=CARTESIAN_POINT('Ctrl Pts',(-17.1581501091636,14.4625550657111,
131.974268906069)) ;
#114939=CARTESIAN_POINT('Ctrl Pts',(-17.0827332780509,14.3400369417443,
131.720826863696)) ;
#114940=CARTESIAN_POINT('Ctrl Pts',(-17.0209888868574,14.1521957535254,
131.507380128005)) ;
#114941=CARTESIAN_POINT('Ctrl Pts',(-16.9778207788142,13.9116489154345,
131.348115653949)) ;
#114942=CARTESIAN_POINT('Ctrl Pts',(-16.9572990580186,13.6358544266559,
131.25499330384)) ;
#114943=CARTESIAN_POINT('Ctrl Pts',(-16.9615071381463,13.3459427675745,
131.23424300822)) ;
#114944=CARTESIAN_POINT('Ctrl Pts',(-16.9909211180614,13.0604649745041,
131.286996740778)) ;
#114945=CARTESIAN_POINT('Ctrl Pts',(-17.0441007990242,12.8015143832803,
131.409241549806)) ;
#114946=CARTESIAN_POINT('Ctrl Pts',(-17.1180304186239,12.586871423154,131.592073079015)) ;
#114947=CARTESIAN_POINT('Ctrl Pts',(-17.2080500636742,12.4323032180318,
131.821934768459)) ;
#114948=CARTESIAN_POINT('Ctrl Pts',(-17.3084611337155,12.348604012381,132.082157360211)) ;
#114949=CARTESIAN_POINT('Ctrl Pts',(-17.4130111461555,12.3418345254331,
132.3544143668)) ;
#114950=CARTESIAN_POINT('Ctrl Pts',(-17.5146765749007,12.4127257697425,
132.618266949295)) ;
#114951=CARTESIAN_POINT('Ctrl Pts',(-17.606721170884,12.5554430365515,132.854114383774)) ;
#114952=CARTESIAN_POINT('Ctrl Pts',(-17.6839111619126,12.7608029240068,
133.046442139626)) ;
#114953=CARTESIAN_POINT('Ctrl Pts',(-17.7410331806284,13.0143079229722,
133.180091411217)) ;
#114954=CARTESIAN_POINT('Ctrl Pts',(-17.7745360164768,13.2953661026702,
133.244952941826)) ;
#114955=CARTESIAN_POINT('Ctrl Pts',(-17.7831520054483,13.587499191953,133.236886150184)) ;
#114956=CARTESIAN_POINT('Ctrl Pts',(-17.7666348632763,13.8669338626205,
133.155497022517)) ;
#114957=CARTESIAN_POINT('Ctrl Pts',(-17.7273863718362,14.1134263503453,
133.007875421063)) ;
#114958=CARTESIAN_POINT('Ctrl Pts',(-17.6683893078491,14.3121780897716,
132.802342611055)) ;
#114959=CARTESIAN_POINT('Ctrl Pts',(-17.5946147982464,14.4470050265316,
132.553591742459)) ;
#114960=CARTESIAN_POINT('Ctrl Pts',(-17.5125911040324,14.5078086325279,
132.280874384855)) ;
#114961=CARTESIAN_POINT('Ctrl Pts',(-17.4289255794743,14.4913412737729,
132.003473976216)) ;
#114962=CARTESIAN_POINT('Ctrl Pts',(-17.3497030184291,14.3985299043882,
131.738923406222)) ;
#114963=CARTESIAN_POINT('Ctrl Pts',(-17.2814947859058,14.2353764928408,
131.506472748856)) ;
#114964=CARTESIAN_POINT('Ctrl Pts',(-17.2301833982271,14.0132824388172,
131.32333677435)) ;
#114965=CARTESIAN_POINT('Ctrl Pts',(-17.2003726149901,13.751770584179,131.203370984278)) ;
#114966=CARTESIAN_POINT('Ctrl Pts',(-17.1942692410409,13.4639004603942,
131.15229798358)) ;
#114967=CARTESIAN_POINT('Ctrl Pts',(-17.2136563233809,13.1736259559936,
131.175755585428)) ;
#114968=CARTESIAN_POINT('Ctrl Pts',(-17.2572199771084,12.9029494351804,
131.270058586451)) ;
#114969=CARTESIAN_POINT('Ctrl Pts',(-17.3234518657098,12.6670694829694,
131.430263375814)) ;
#114970=CARTESIAN_POINT('Ctrl Pts',(-17.4076950363158,12.4867414535482,
131.643224441991)) ;
#114971=CARTESIAN_POINT('Ctrl Pts',(-17.5042594533731,12.3736046950475,
131.892333562312)) ;
#114972=CARTESIAN_POINT('Ctrl Pts',(-17.6083225797878,12.3351061359291,
132.163067552705)) ;
#114973=CARTESIAN_POINT('Ctrl Pts',(-17.7115102747659,12.3747297412366,
132.431506046747)) ;
#114974=CARTESIAN_POINT('Ctrl Pts',(-17.80835655534,12.4890530273647,132.681306942846)) ;
#114975=CARTESIAN_POINT('Ctrl Pts',(-17.8927139370083,12.6718473822343,
132.894413198474)) ;
#114976=CARTESIAN_POINT('Ctrl Pts',(-17.9581348743092,12.9071471042355,
133.05245843071)) ;
#114977=CARTESIAN_POINT('Ctrl Pts',(-18.0014489044881,13.1791583633753,
133.145922177929)) ;
#114978=CARTESIAN_POINT('Ctrl Pts',(-18.020261151911,13.4685703303894,133.16781609884)) ;
#114979=CARTESIAN_POINT('Ctrl Pts',(-18.0138792132709,13.7556865610863,
133.115998787948)) ;
#114980=CARTESIAN_POINT('Ctrl Pts',(-17.9834392562243,14.0184520779736,
132.993960277943)) ;
#114981=CARTESIAN_POINT('Ctrl Pts',(-17.9319093006337,14.2386835545227,
132.810307624848)) ;
#114982=CARTESIAN_POINT('Ctrl Pts',(-17.8634196060343,14.4009245247973,
132.577005577925)) ;
#114983=CARTESIAN_POINT('Ctrl Pts',(-17.7839956342627,14.4923209079493,
132.311848278652)) ;
#114984=CARTESIAN_POINT('Ctrl Pts',(-17.7003715420016,14.5074993821674,
132.034597515729)) ;
#114985=CARTESIAN_POINT('Ctrl Pts',(-17.6179715693461,14.4446391320812,
131.760580504429)) ;
#114986=CARTESIAN_POINT('Ctrl Pts',(-17.5449472629492,14.309013886893,131.514230915999)) ;
#114987=CARTESIAN_POINT('Ctrl Pts',(-17.4863929079662,14.1104149351794,
131.310125649846)) ;
#114988=CARTESIAN_POINT('Ctrl Pts',(-17.4472233098488,13.8614588559076,
131.162498832848)) ;
#114989=CARTESIAN_POINT('Ctrl Pts',(-17.4312869960412,13.5819687002437,
131.082859767227)) ;
#114990=CARTESIAN_POINT('Ctrl Pts',(-17.4402797073093,13.2906279013141,
131.075985151787)) ;
#114991=CARTESIAN_POINT('Ctrl Pts',(-17.4743143198391,13.009243305788,131.142317233284)) ;
#114992=CARTESIAN_POINT('Ctrl Pts',(-17.5315517099284,12.7575168112921,
131.276452625469)) ;
#114993=CARTESIAN_POINT('Ctrl Pts',(-17.6091410096472,12.5525240138587,
131.469879021206)) ;
#114994=CARTESIAN_POINT('Ctrl Pts',(-17.7014737885802,12.4108770336832,
131.706544893167)) ;
#114995=CARTESIAN_POINT('Ctrl Pts',(-17.8032831969416,12.3412909140522,
131.97080490142)) ;
#114996=CARTESIAN_POINT('Ctrl Pts',(-17.9077079735701,12.3493861735078,
132.242732393973)) ;
#114997=CARTESIAN_POINT('Ctrl Pts',(-18.0080021312736,12.4342727909203,
132.502613425746)) ;
#114998=CARTESIAN_POINT('Ctrl Pts',(-18.097851259794,12.5900489009072,132.731956223757)) ;
#114999=CARTESIAN_POINT('Ctrl Pts',(-18.1714811565311,12.8056265995217,
132.913906681068)) ;
#115000=CARTESIAN_POINT('Ctrl Pts',(-18.2242791522083,13.0653848746049,
133.035014327401)) ;
#115001=CARTESIAN_POINT('Ctrl Pts',(-18.2532373491338,13.3504851063388,
133.086511791274)) ;
#115002=CARTESIAN_POINT('Ctrl Pts',(-18.2570176970517,13.6412798147236,
133.064399324168)) ;
#115003=CARTESIAN_POINT('Ctrl Pts',(-18.2361288879767,13.915548156852,132.970331104728)) ;
#115004=CARTESIAN_POINT('Ctrl Pts',(-18.1927521468012,14.1552942040558,
132.810491998612)) ;
#115005=CARTESIAN_POINT('Ctrl Pts',(-18.1304889717146,14.3429101935435,
132.595396822877)) ;
#115006=CARTESIAN_POINT('Ctrl Pts',(-18.0549535994053,14.4639893047867,
132.341644352442)) ;
#115007=CARTESIAN_POINT('Ctrl Pts',(-17.9720169774795,14.5107279953385,
132.066239556179)) ;
#115008=CARTESIAN_POINT('Ctrl Pts',(-17.88839874123,14.4794893752074,131.788842595817)) ;
#115009=CARTESIAN_POINT('Ctrl Pts',(-17.8108656194136,14.3727211578977,
131.529246532274)) ;
#115010=CARTESIAN_POINT('Ctrl Pts',(-17.7456151211965,14.1977799584113,
131.305501822006)) ;
#115011=CARTESIAN_POINT('Ctrl Pts',(-17.6981151394564,13.9680803032242,
131.13369579038)) ;
#115012=CARTESIAN_POINT('Ctrl Pts',(-17.6723054333923,13.6967826933105,
131.024941140418)) ;
#115013=CARTESIAN_POINT('Ctrl Pts',(-17.6711447708163,13.4094043760888,
130.98862536116)) ;
#115014=CARTESIAN_POINT('Ctrl Pts',(-17.6950445630246,13.1212039321583,
131.025303143358)) ;
#115015=CARTESIAN_POINT('Ctrl Pts',(-17.74333311896,12.8546896237207,131.133221894845)) ;
#115016=CARTESIAN_POINT('Ctrl Pts',(-17.81282756458,12.6293810356165,131.303196900116)) ;
#115017=CARTESIAN_POINT('Ctrl Pts',(-17.9005194706817,12.4594635396626,
131.525988684649)) ;
#115018=CARTESIAN_POINT('Ctrl Pts',(-17.9986989569018,12.3604529302704,
131.779876218196)) ;
#115019=CARTESIAN_POINT('Ctrl Pts',(-18.1032340963646,12.3366695079855,
132.05199660503)) ;
#115020=CARTESIAN_POINT('Ctrl Pts',(-18.2056125319901,12.3907630606801,
132.318086056791)) ;
#115021=CARTESIAN_POINT('Ctrl Pts',(-18.300613364825,12.5187717527639,132.562441868016)) ;
#115022=CARTESIAN_POINT('Ctrl Pts',(-18.3816465085652,12.7125553045139,
132.765918032423)) ;
#115023=CARTESIAN_POINT('Ctrl Pts',(-18.4429853099616,12.9551208485313,
132.912159665352)) ;
#115024=CARTESIAN_POINT('Ctrl Pts',(-18.4820336765163,13.2325620060974,
132.993078593711)) ;
#115025=CARTESIAN_POINT('Ctrl Pts',(-18.496084383933,13.5243419796884,133.00090515124)) ;
#115026=CARTESIAN_POINT('Ctrl Pts',(-18.4850639350324,13.8069926528057,
132.935714610325)) ;
#115027=CARTESIAN_POINT('Ctrl Pts',(-18.4503367662865,14.0639000199269,
132.801056058483)) ;
#115028=CARTESIAN_POINT('Ctrl Pts',(-18.3952268191814,14.2741558930926,
132.606941700926)) ;
#115029=CARTESIAN_POINT('Ctrl Pts',(-18.3243680288223,14.4234615625839,
132.366801537788)) ;
#115030=CARTESIAN_POINT('Ctrl Pts',(-18.2437816042926,14.5011170686614,
132.098327447916)) ;
#115031=CARTESIAN_POINT('Ctrl Pts',(-18.1592384984199,14.5013614779113,
131.81807310291)) ;
#115032=CARTESIAN_POINT('Ctrl Pts',(-18.0789307375107,14.4249956630962,
131.550560960519)) ;
#115033=CARTESIAN_POINT('Ctrl Pts',(-18.0076541118125,14.2760171565871,
131.309082565097)) ;
#115034=CARTESIAN_POINT('Ctrl Pts',(-17.9524899575172,14.0665442400002,
131.114862544505)) ;
#115035=CARTESIAN_POINT('Ctrl Pts',(-17.9175014310239,13.8110528410318,
130.979547647309)) ;
#115036=CARTESIAN_POINT('Ctrl Pts',(-17.9061688391216,13.5262786463887,
130.913174372637)) ;
#115037=CARTESIAN_POINT('Ctrl Pts',(-17.919877948496,13.2368369901033,130.920277108179)) ;
#115038=CARTESIAN_POINT('Ctrl Pts',(-17.9586197277239,12.9583255903659,
131.000212959745)) ;
#115039=CARTESIAN_POINT('Ctrl Pts',(-18.0199083066583,12.7145800096232,
131.146219952724)) ;
#115040=CARTESIAN_POINT('Ctrl Pts',(-18.1009974511921,12.5201730384604,
131.349794172582)) ;
#115041=CARTESIAN_POINT('Ctrl Pts',(-18.1949562384929,12.392297716127,131.59141902566)) ;
#115042=CARTESIAN_POINT('Ctrl Pts',(-18.2981754606917,12.3368042043637,
131.859663996403)) ;
#115043=CARTESIAN_POINT('Ctrl Pts',(-18.4019398290045,12.3594079574846,
132.129799825424)) ;
#115044=CARTESIAN_POINT('Ctrl Pts',(-18.5013383418749,12.4588426243277,
132.386856715267)) ;
#115045=CARTESIAN_POINT('Ctrl Pts',(-18.5881323912535,12.6263832935465,
132.607414342136)) ;
#115046=CARTESIAN_POINT('Ctrl Pts',(-18.6581587702516,12.8513078071139,
132.778854814353)) ;
#115047=CARTESIAN_POINT('Ctrl Pts',(-18.7067345904951,13.1175341941134,
132.887608467018)) ;
#115048=CARTESIAN_POINT('Ctrl Pts',(-18.731003412201,13.4059954970849,132.925314381533)) ;
#115049=CARTESIAN_POINT('Ctrl Pts',(-18.7300968071152,13.6942419645787,
132.889656262388)) ;
#115050=CARTESIAN_POINT('Ctrl Pts',(-18.7044541735128,13.9656571359195,
132.781395875164)) ;
#115051=CARTESIAN_POINT('Ctrl Pts',(-18.6575265026644,14.1945698215837,
132.611470543872)) ;
#115052=CARTESIAN_POINT('Ctrl Pts',(-18.5922406519204,14.3711224528334,
132.387486886082)) ;
#115053=CARTESIAN_POINT('Ctrl Pts',(-18.5149037393986,14.4785950091488,
132.128508392993)) ;
#115054=CARTESIAN_POINT('Ctrl Pts',(-18.4311371510558,14.5108133112394,
131.850601957705)) ;
#115055=CARTESIAN_POINT('Ctrl Pts',(-18.3483146549276,14.4650394200622,
131.575598992863)) ;
#115056=CARTESIAN_POINT('Ctrl Pts',(-18.2726066198908,14.3446919400874,
131.321313280288)) ;
#115057=CARTESIAN_POINT('Ctrl Pts',(-18.2103307361537,14.1586507898245,
131.106307024848)) ;
#115058=CARTESIAN_POINT('Ctrl Pts',(-18.1664432390162,13.9182142591253,
130.944795156692)) ;
#115059=CARTESIAN_POINT('Ctrl Pts',(-18.1453636366719,13.6446894301756,
130.850233747273)) ;
#115060=CARTESIAN_POINT('Ctrl Pts',(-18.1488348343508,13.3538163555555,
130.82719813754)) ;
#115061=CARTESIAN_POINT('Ctrl Pts',(-18.1774811245967,13.0687529323482,
130.877811758373)) ;
#115062=CARTESIAN_POINT('Ctrl Pts',(-18.2300437642224,12.8084025711039,
130.998208929724)) ;
#115063=CARTESIAN_POINT('Ctrl Pts',(-18.3034001053734,12.5923662507696,
131.179384620874)) ;
#115064=CARTESIAN_POINT('Ctrl Pts',(-18.3931634370597,12.4355966936421,
131.408445657945)) ;
#115065=CARTESIAN_POINT('Ctrl Pts',(-18.4935575860177,12.3498834173245,
131.668562849344)) ;
#115066=CARTESIAN_POINT('Ctrl Pts',(-18.5975530541275,12.3409542808635,
131.939369081028)) ;
#115067=CARTESIAN_POINT('Ctrl Pts',(-18.6994673351223,12.4093757248112,
132.203931136602)) ;
#115068=CARTESIAN_POINT('Ctrl Pts',(-18.7921201529756,12.5505196315372,
132.441467645947)) ;
#115069=CARTESIAN_POINT('Ctrl Pts',(-18.8697017731338,12.7541803006072,
132.634971878383)) ;
#115070=CARTESIAN_POINT('Ctrl Pts',(-18.9273307484839,13.0055267425044,
132.770220733639)) ;
#115071=CARTESIAN_POINT('Ctrl Pts',(-18.9617100390982,13.2870724884799,
132.83751270461)) ;
#115072=CARTESIAN_POINT('Ctrl Pts',(-18.9710255677151,13.5781354317469,
132.831615285865)) ;
#115073=CARTESIAN_POINT('Ctrl Pts',(-18.9553578084607,13.8583662507443,
132.752702523973)) ;
#115074=CARTESIAN_POINT('Ctrl Pts',(-18.9165383575917,14.1072755060793,
132.606171710367)) ;
#115075=CARTESIAN_POINT('Ctrl Pts',(-18.8581587772242,14.3069765889331,
132.4025330216)) ;
#115076=CARTESIAN_POINT('Ctrl Pts',(-18.7850681968336,14.443614067786,132.155907192059)) ;
#115077=CARTESIAN_POINT('Ctrl Pts',(-18.702941141321,14.5071928082345,131.882773592227)) ;
#115078=CARTESIAN_POINT('Ctrl Pts',(-18.6190408117616,14.4928945220509,
131.604612881179)) ;
#115079=CARTESIAN_POINT('Ctrl Pts',(-18.5396187459799,14.4021254936154,
131.339485656911)) ;
#115080=CARTESIAN_POINT('Ctrl Pts',(-18.4711933901986,14.2413770477371,
131.106496569037)) ;
#115081=CARTESIAN_POINT('Ctrl Pts',(-18.4192605637911,14.0210258594474,
130.921552581758)) ;
#115082=CARTESIAN_POINT('Ctrl Pts',(-18.3886405960536,13.7594508415378,
130.799092122936)) ;
#115083=CARTESIAN_POINT('Ctrl Pts',(-18.381928462571,13.4716753030503,130.746210031867)) ;
#115084=CARTESIAN_POINT('Ctrl Pts',(-18.4004216312574,13.18278007244,130.767242888151)) ;
#115085=CARTESIAN_POINT('Ctrl Pts',(-18.4435339670258,12.9097866347109,
130.860039653288)) ;
#115086=CARTESIAN_POINT('Ctrl Pts',(-18.5088204983959,12.6739761120234,
131.017674750893)) ;
#115087=CARTESIAN_POINT('Ctrl Pts',(-18.5926770612546,12.4911376353209,
131.229439455072)) ;
#115088=CARTESIAN_POINT('Ctrl Pts',(-18.6895108158381,12.3755758788311,
131.479159592622)) ;
#115089=CARTESIAN_POINT('Ctrl Pts',(-18.7928542788589,12.3352662329562,
131.747989657394)) ;
#115090=CARTESIAN_POINT('Ctrl Pts',(-18.8962659376777,12.3722006143293,
132.017051741353)) ;
#115091=CARTESIAN_POINT('Ctrl Pts',(-18.9940984306609,12.4858118722087,
132.26946955847)) ;
#115092=CARTESIAN_POINT('Ctrl Pts',(-19.0779483654093,12.6649628027199,
132.481462828409)) ;
#115093=CARTESIAN_POINT('Ctrl Pts',(-19.144324386781,12.8995424291904,132.64216747859)) ;
#115094=CARTESIAN_POINT('Ctrl Pts',(-19.1882893988472,13.1707489990253,
132.73754255469)) ;
#115095=CARTESIAN_POINT('Ctrl Pts',(-19.2078747746244,13.4602465419289,
132.76165779285)) ;
#115096=CARTESIAN_POINT('Ctrl Pts',(-19.2021695943243,13.7479094104328,
132.711797460233)) ;
#115097=CARTESIAN_POINT('Ctrl Pts',(-19.1724541288044,14.0110933638022,
132.591943088721)) ;
#115098=CARTESIAN_POINT('Ctrl Pts',(-19.1214789970609,14.2330195298938,
132.409891780119)) ;
#115099=CARTESIAN_POINT('Ctrl Pts',(-19.0533824116154,14.397056415232,132.177734508543)) ;
#115100=CARTESIAN_POINT('Ctrl Pts',(-18.9744610193818,14.4906410938832,
131.914150162339)) ;
#115101=CARTESIAN_POINT('Ctrl Pts',(-18.890345578861,14.5080280130628,131.635247249356)) ;
#115102=CARTESIAN_POINT('Ctrl Pts',(-18.8085392860132,14.4480725424633,
131.363277720596)) ;
#115103=CARTESIAN_POINT('Ctrl Pts',(-18.7346273925197,14.3139470607326,
131.114108989611)) ;
#115104=CARTESIAN_POINT('Ctrl Pts',(-18.6756142626322,14.1169437524237,
130.908679443903)) ;
#115105=CARTESIAN_POINT('Ctrl Pts',(-18.6357563526766,13.8684682048696,
130.758950982595)) ;
#115106=CARTESIAN_POINT('Ctrl Pts',(-18.6192189361488,13.5907243651,130.677694418299)) ;
#115107=CARTESIAN_POINT('Ctrl Pts',(-18.6274186795787,13.2994062522709,
130.668497076563)) ;
#115108=CARTESIAN_POINT('Ctrl Pts',(-18.6607053713449,13.0173302811176,
130.732637587237)) ;
#115109=CARTESIAN_POINT('Ctrl Pts',(-18.7175745221499,12.7634586998748,
130.865557336184)) ;
#115110=CARTESIAN_POINT('Ctrl Pts',(-18.7946062779487,12.5574053612187,
131.057405473283)) ;
#115111=CARTESIAN_POINT('Ctrl Pts',(-18.8863176363417,12.4141338116398,
131.292346024062)) ;
#115112=CARTESIAN_POINT('Ctrl Pts',(-18.9880396659882,12.342233208706,131.556318246303)) ;
#115113=CARTESIAN_POINT('Ctrl Pts',(-19.092367557879,12.3479816385131,131.828001920729)) ;
#115114=CARTESIAN_POINT('Ctrl Pts',(-19.1930265312653,12.4308508598937,
132.088893600864)) ;
#115115=CARTESIAN_POINT('Ctrl Pts',(-19.2830355733598,12.5841342714032,
132.318802233278)) ;
#115116=CARTESIAN_POINT('Ctrl Pts',(-19.3575448753726,12.7991564308112,
132.503166321675)) ;
#115117=CARTESIAN_POINT('Ctrl Pts',(-19.410786935153,13.0569999610756,132.625693509338)) ;
#115118=CARTESIAN_POINT('Ctrl Pts',(-19.4405356262244,13.3421921034464,
132.679428679679)) ;
#115119=CARTESIAN_POINT('Ctrl Pts',(-19.4450790880921,13.6321454574867,
132.659662972591)) ;
#115120=CARTESIAN_POINT('Ctrl Pts',(-19.4247875387373,13.9089725412032,
132.567125349093)) ;
#115121=CARTESIAN_POINT('Ctrl Pts',(-19.381825668748,14.1498188340954,132.408476398238)) ;
#115122=CARTESIAN_POINT('Ctrl Pts',(-19.3204518279194,14.3379335225619,
132.196198119276)) ;
#115123=CARTESIAN_POINT('Ctrl Pts',(-19.2450347897687,14.4615825769609,
131.942693860373)) ;
#115124=CARTESIAN_POINT('Ctrl Pts',(-19.162267963524,14.5104718339952,131.667809535155)) ;
#115125=CARTESIAN_POINT('Ctrl Pts',(-19.0783524563333,14.4813917081873,
131.389457000585)) ;
#115126=CARTESIAN_POINT('Ctrl Pts',(-19.0006162859046,14.3764101476522,
131.129272642533)) ;
#115127=CARTESIAN_POINT('Ctrl Pts',(-18.9351626104612,14.2041613001764,
130.905077291113)) ;
#115128=CARTESIAN_POINT('Ctrl Pts',(-18.8868641696125,13.9743839791119,
130.730738018104)) ;
#115129=CARTESIAN_POINT('Ctrl Pts',(-18.8605695212481,13.7063210401926,
130.620861352139)) ;
#115130=CARTESIAN_POINT('Ctrl Pts',(-18.8586114405782,13.416701167449,130.581917827711)) ;
#115131=CARTESIAN_POINT('Ctrl Pts',(-18.8818454285258,13.1291677758352,
130.616763647551)) ;
#115132=CARTESIAN_POINT('Ctrl Pts',(-18.9294289009308,12.86171027905,130.722620411742)) ;
#115133=CARTESIAN_POINT('Ctrl Pts',(-18.9984336324713,12.6350478480017,
130.891152728659)) ;
#115134=CARTESIAN_POINT('Ctrl Pts',(-19.0852684560724,12.4638699665219,
131.111590594525)) ;
#115135=CARTESIAN_POINT('Ctrl Pts',(-19.1836902605787,12.3621126869917,
131.366013493841)) ;
#115136=CARTESIAN_POINT('Ctrl Pts',(-19.2880034593845,12.336288293437,131.637540200635)) ;
#115137=CARTESIAN_POINT('Ctrl Pts',(-19.3907293591919,12.3882079133966,
131.9045787098)) ;
#115138=CARTESIAN_POINT('Ctrl Pts',(-19.4861202999562,12.5148240028862,
132.150020522081)) ;
#115139=CARTESIAN_POINT('Ctrl Pts',(-19.566984502277,12.7050812653244,132.353293437429)) ;
#115140=CARTESIAN_POINT('Ctrl Pts',(-19.6294717703468,12.9482677220772,
132.502618790391)) ;
#115141=CARTESIAN_POINT('Ctrl Pts',(-19.6689768655333,13.2238578222556,
132.585025535771)) ;
#115142=CARTESIAN_POINT('Ctrl Pts',(-19.6838357324499,13.5162932448957,
132.595118812429)) ;
#115143=CARTESIAN_POINT('Ctrl Pts',(-19.6735197937544,13.799165239793,132.532024333921)) ;
#115144=CARTESIAN_POINT('Ctrl Pts',(-19.6392454600331,14.0580267764743,
132.398557205212)) ;
#115145=CARTESIAN_POINT('Ctrl Pts',(-19.5848869196862,14.2686028129511,
132.206807442572)) ;
#115146=CARTESIAN_POINT('Ctrl Pts',(-19.5145008411043,14.4199618502008,
131.968069495771)) ;
#115147=CARTESIAN_POINT('Ctrl Pts',(-19.4340220268986,14.4998958219189,
131.699871465245)) ;
#115148=CARTESIAN_POINT('Ctrl Pts',(-19.3495759662661,14.5025664794371,
131.419941342377)) ;
#115149=CARTESIAN_POINT('Ctrl Pts',(-19.2688627445457,14.4280652825415,
131.151146889785)) ;
#115150=CARTESIAN_POINT('Ctrl Pts',(-19.197514432747,14.2819177513075,130.909621465088)) ;
#115151=CARTESIAN_POINT('Ctrl Pts',(-19.1413921728409,14.0723877227319,
130.712339919469)) ;
#115152=CARTESIAN_POINT('Ctrl Pts',(-19.1060584048045,13.8191595273478,
130.576195818314)) ;
#115153=CARTESIAN_POINT('Ctrl Pts',(-19.0939136018658,13.5356702848312,
130.507524027747)) ;
#115154=CARTESIAN_POINT('Ctrl Pts',(-19.1068958007053,13.2451626614465,
130.512392184105)) ;
#115155=CARTESIAN_POINT('Ctrl Pts',(-19.1449564065195,12.9658959397094,
130.5903314269)) ;
#115156=CARTESIAN_POINT('Ctrl Pts',(-19.2057189790489,12.720867949973,130.73477557543)) ;
#115157=CARTESIAN_POINT('Ctrl Pts',(-19.2858400354675,12.5256178596935,
130.935699785553)) ;
#115158=CARTESIAN_POINT('Ctrl Pts',(-19.3800402811628,12.3947249390078,
131.177818876414)) ;
#115159=CARTESIAN_POINT('Ctrl Pts',(-19.4831200353959,12.3373274128747,
131.445666380565)) ;
#115160=CARTESIAN_POINT('Ctrl Pts',(-19.5867485454506,12.3577351376061,
131.715460652154)) ;
#115161=CARTESIAN_POINT('Ctrl Pts',(-19.6862131801358,12.4546492514378,
131.972779675498)) ;
#115162=CARTESIAN_POINT('Ctrl Pts',(-19.7738286134021,12.6210676591383,
132.195587853881)) ;
#115163=CARTESIAN_POINT('Ctrl Pts',(-19.8442902702029,12.8446766854148,
132.368316433847)) ;
#115164=CARTESIAN_POINT('Ctrl Pts',(-19.8933608798738,13.108808163257,132.478653710118)) ;
#115165=CARTESIAN_POINT('Ctrl Pts',(-19.9184859283659,13.3979062620311,
132.518747291947)) ;
#115166=CARTESIAN_POINT('Ctrl Pts',(-19.9181983031023,13.6859097607706,
132.484944374893)) ;
#115167=CARTESIAN_POINT('Ctrl Pts',(-19.8935840118438,13.9567565280856,
132.379898432991)) ;
#115168=CARTESIAN_POINT('Ctrl Pts',(-19.8465997978561,14.1899349125241,
132.209373856163)) ;
#115169=CARTESIAN_POINT('Ctrl Pts',(-19.7823820361551,14.3662692626876,
131.988864508273)) ;
#115170=CARTESIAN_POINT('Ctrl Pts',(-19.7048377925854,14.4768289979695,
131.729048105592)) ;
#115171=CARTESIAN_POINT('Ctrl Pts',(-19.621356858463,14.5109207090365,131.452070562692)) ;
#115172=CARTESIAN_POINT('Ctrl Pts',(-19.5383256537918,14.4673589954117,
131.176412965102)) ;
#115173=CARTESIAN_POINT('Ctrl Pts',(-19.462343360731,14.3490298117359,130.921339630599)) ;
#115174=CARTESIAN_POINT('Ctrl Pts',(-19.399598094763,14.1643442573792,130.70492417211)) ;
#115175=CARTESIAN_POINT('Ctrl Pts',(-19.3553585530389,13.9269540764464,
130.542614298548)) ;
#115176=CARTESIAN_POINT('Ctrl Pts',(-19.3333939719036,13.6529087066834,
130.44529695513)) ;
#115177=CARTESIAN_POINT('Ctrl Pts',(-19.3361541913265,13.3625040426011,
130.420224634067)) ;
#115178=CARTESIAN_POINT('Ctrl Pts',(-19.3641172961552,13.0764917625792,
130.468781137817)) ;
#115179=CARTESIAN_POINT('Ctrl Pts',(-19.4160399610195,12.8152457852602,
130.587319851219)) ;
#115180=CARTESIAN_POINT('Ctrl Pts',(-19.4888652574942,12.5977360848388,
130.766942106929)) ;
#115181=CARTESIAN_POINT('Ctrl Pts',(-19.5781388686584,12.4392301767845,
130.994608862376)) ;
#115182=CARTESIAN_POINT('Ctrl Pts',(-19.6782931891438,12.3513755992719,
131.254028736787)) ;
#115183=CARTESIAN_POINT('Ctrl Pts',(-19.7822229405507,12.3399316332142,
131.524661009902)) ;
#115184=CARTESIAN_POINT('Ctrl Pts',(-19.88504344773,12.4070554351268,131.791616350641)) ;
#115185=CARTESIAN_POINT('Ctrl Pts',(-19.9771610745846,12.5451369869361,
132.027897931008)) ;
#115186=CARTESIAN_POINT('Ctrl Pts',(-20.0556173721215,12.7477726868892,
132.223821692675)) ;
#115187=CARTESIAN_POINT('Ctrl Pts',(-20.1137903255926,12.9979367372735,
132.360683275234)) ;
#115188=CARTESIAN_POINT('Ctrl Pts',(-20.1489013724765,13.2792370978739,
132.430071631305)) ;
#115189=CARTESIAN_POINT('Ctrl Pts',(-20.1588787384282,13.5701580555343,
132.426125674529)) ;
#115190=CARTESIAN_POINT('Ctrl Pts',(-20.143937682242,13.8505377724051,132.349389311992)) ;
#115191=CARTESIAN_POINT('Ctrl Pts',(-20.1057318059421,14.1007512372239,
132.20463305785)) ;
#115192=CARTESIAN_POINT('Ctrl Pts',(-20.0478354950526,14.3021715583994,
132.002395149785)) ;
#115193=CARTESIAN_POINT('Ctrl Pts',(-19.9748500391882,14.4410638226486,
131.755979394128)) ;
#115194=CARTESIAN_POINT('Ctrl Pts',(-19.892940104349,14.506420576945,131.483512074612)) ;
#115195=CARTESIAN_POINT('Ctrl Pts',(-19.8092678890523,14.4944296739133,
131.206120710523)) ;
#115196=CARTESIAN_POINT('Ctrl Pts',(-19.7294350859359,14.4055611915821,
130.939713797808)) ;
#115197=CARTESIAN_POINT('Ctrl Pts',(-19.66081208133,14.2469875620131,130.706232624641)) ;
#115198=CARTESIAN_POINT('Ctrl Pts',(-19.6083158027718,14.0284942715184,
130.519673218377)) ;
#115199=CARTESIAN_POINT('Ctrl Pts',(-19.5769557514165,13.7670074742828,
130.394940588624)) ;
#115200=CARTESIAN_POINT('Ctrl Pts',(-19.5695668686991,13.4805781215048,
130.340191561689)) ;
#115201=CARTESIAN_POINT('Ctrl Pts',(-19.5872696261961,13.1913388058783,
130.358899107894)) ;
#115202=CARTESIAN_POINT('Ctrl Pts',(-19.6297522740938,12.9172330933754,
130.449814911348)) ;
#115203=CARTESIAN_POINT('Ctrl Pts',(-19.6944389773908,12.6799728703758,
130.60569175476)) ;
#115204=CARTESIAN_POINT('Ctrl Pts',(-19.7782230780513,12.4949910418975,
130.817115688087)) ;
#115205=CARTESIAN_POINT('Ctrl Pts',(-19.8739923402946,12.3781840447206,
131.063992159593)) ;
#115206=CARTESIAN_POINT('Ctrl Pts',(-19.9780674608701,12.3352411023339,
131.33468497079)) ;
#115207=CARTESIAN_POINT('Ctrl Pts',(-20.0810744379286,12.3701183957634,
131.602725123913)) ;
#115208=CARTESIAN_POINT('Ctrl Pts',(-20.179252895713,12.4815908370187,131.85612905703)) ;
#115209=CARTESIAN_POINT('Ctrl Pts',(-20.2634570739637,12.6586744463426,
132.069206441814)) ;
#115210=CARTESIAN_POINT('Ctrl Pts',(-20.3305901520664,12.8927064505131,
132.232014267973)) ;
#115211=CARTESIAN_POINT('Ctrl Pts',(-20.3750331233153,13.1615895986342,
132.328969789793)) ;
#115212=CARTESIAN_POINT('Ctrl Pts',(-20.3954965997089,13.4527337961883,
132.355428882089)) ;
#115213=CARTESIAN_POINT('Ctrl Pts',(-20.3904573045894,13.7397606263225,
132.307631593907)) ;
#115214=CARTESIAN_POINT('Ctrl Pts',(-20.3613437715797,14.0044956878458,
132.189457679076)) ;
#115215=CARTESIAN_POINT('Ctrl Pts',(-20.3110168045734,14.2270717047825,
132.009394785638)) ;
#115216=CARTESIAN_POINT('Ctrl Pts',(-20.2436381751946,14.3928428531141,
131.779444891534)) ;
#115217=CARTESIAN_POINT('Ctrl Pts',(-20.164336633125,14.4891679896536,131.51449038135)) ;
#115218=CARTESIAN_POINT('Ctrl Pts',(-20.0809111882638,14.5086708936273,
131.237865647246)) ;
#115219=CARTESIAN_POINT('Ctrl Pts',(-19.9983950566067,14.4507091204102,
130.963592375788)) ;
#115220=CARTESIAN_POINT('Ctrl Pts',(-19.9244190141413,14.318823465338,130.714351089596)) ;
#115221=CARTESIAN_POINT('Ctrl Pts',(-19.8648700988791,14.1234067424229,
130.507330724768)) ;
#115222=CARTESIAN_POINT('Ctrl Pts',(-19.8245161746179,13.8772496577341,
130.356293737963)) ;
#115223=CARTESIAN_POINT('Ctrl Pts',(-19.8070957881005,13.5994498547175,
130.272359938913)) ;
#115224=CARTESIAN_POINT('Ctrl Pts',(-19.8146864693653,13.3067289539218,
130.261220009531)) ;
#115225=CARTESIAN_POINT('Ctrl Pts',(-19.8471784531872,13.025513208076,130.323196727465)) ;
#115226=CARTESIAN_POINT('Ctrl Pts',(-19.9032180692331,12.7708776887036,
130.453754380472)) ;
#115227=CARTESIAN_POINT('Ctrl Pts',(-19.9797679754465,12.5628412979246,
130.644157296538)) ;
#115228=CARTESIAN_POINT('Ctrl Pts',(-20.0712997390683,12.4171764122364,
130.878502714501)) ;
#115229=CARTESIAN_POINT('Ctrl Pts',(-20.173220666744,12.3431378359771,131.142938313351)) ;
#115230=CARTESIAN_POINT('Ctrl Pts',(-20.2769543623743,12.3467434972734,
131.413078047708)) ;
#115231=CARTESIAN_POINT('Ctrl Pts',(-20.3779474556413,12.4272274658185,
131.674911921515)) ;
#115232=CARTESIAN_POINT('Ctrl Pts',(-20.4684824931614,12.5790158149027,
131.906293765199)) ;
#115233=CARTESIAN_POINT('Ctrl Pts',(-20.5433178346082,12.7916687829571,
132.091724629749)) ;
#115234=CARTESIAN_POINT('Ctrl Pts',(-20.59747019779,13.0498138992039,132.216737279054)) ;
#115235=CARTESIAN_POINT('Ctrl Pts',(-20.6277539698486,13.3331756720239,
132.272199599018)) ;
#115236=CARTESIAN_POINT('Ctrl Pts',(-20.63310319697,13.6238935345468,132.254712776567)) ;
#115237=CARTESIAN_POINT('Ctrl Pts',(-20.6135004102223,13.9010885274901,
132.164225860573)) ;
#115238=CARTESIAN_POINT('Ctrl Pts',(-20.5712628793398,14.1432054793993,
132.007719764268)) ;
#115239=CARTESIAN_POINT('Ctrl Pts',(-20.5099062183509,14.3341070280144,
131.795269476235)) ;
#115240=CARTESIAN_POINT('Ctrl Pts',(-20.4352339689786,14.4587991787124,
131.544150012527)) ;
#115241=CARTESIAN_POINT('Ctrl Pts',(-20.3525489079931,14.5101605081857,
131.269477291802)) ;
#115242=CARTESIAN_POINT('Ctrl Pts',(-20.2687361872864,14.4834097576633,
130.991492371573)) ;
#115243=CARTESIAN_POINT('Ctrl Pts',(-20.1906756501309,14.380986704451,130.730363509583)) ;
#115244=CARTESIAN_POINT('Ctrl Pts',(-20.1243569260148,14.2089571607828,
130.503381990289)) ;
#115245=CARTESIAN_POINT('Ctrl Pts',(-20.0759333865454,13.9828180453883,
130.329004955831)) ;
#115246=CARTESIAN_POINT('Ctrl Pts',(-20.0486953445985,13.7132629209954,
130.216063933579)) ;
#115247=CARTESIAN_POINT('Ctrl Pts',(-20.0461136758052,13.42583764063,130.175529664949)) ;
#115248=CARTESIAN_POINT('Ctrl Pts',(-20.0685766436055,13.1374631065902,
130.208056459246)) ;
#115249=CARTESIAN_POINT('Ctrl Pts',(-20.1154485813734,12.8691197006536,
130.31184888817)) ;
#115250=CARTESIAN_POINT('Ctrl Pts',(-20.1842161886027,12.6403113443668,
130.479551228157)) ;
#115251=CARTESIAN_POINT('Ctrl Pts',(-20.2699974667944,12.468420702256,130.697148821309)) ;
#115252=CARTESIAN_POINT('Ctrl Pts',(-20.368777345651,12.3638000217504,130.952399609198)) ;
#115253=CARTESIAN_POINT('Ctrl Pts',(-20.4724837589939,12.3359859144704,
131.22233281641)) ;
#115254=CARTESIAN_POINT('Ctrl Pts',(-20.5755189014966,12.3855342690204,
131.490214378318)) ;
#115255=CARTESIAN_POINT('Ctrl Pts',(-20.6710370148352,12.5097023136888,
131.736103980719)) ;
#115256=CARTESIAN_POINT('Ctrl Pts',(-20.7526999022241,12.6987169895182,
131.941597617443)) ;
#115257=CARTESIAN_POINT('Ctrl Pts',(-20.8159200282362,12.9413958856346,
132.092978431002)) ;
#115258=CARTESIAN_POINT('Ctrl Pts',(-20.8560148207953,13.2164083911014,
132.177101494275)) ;
#115259=CARTESIAN_POINT('Ctrl Pts',(-20.8715568106971,13.5077476116907,
132.18930496735)) ;
#115260=CARTESIAN_POINT('Ctrl Pts',(-20.8618791478333,13.7917084995172,
132.127994218716)) ;
#115261=CARTESIAN_POINT('Ctrl Pts',(-20.8285666993428,14.0497089633418,
131.997596945122)) ;
#115262=CARTESIAN_POINT('Ctrl Pts',(-20.7745879228126,14.2632250030891,
131.806787903495)) ;
#115263=CARTESIAN_POINT('Ctrl Pts',(-20.7043311974277,14.4168537708596,
131.568328459368)) ;
#115264=CARTESIAN_POINT('Ctrl Pts',(-20.6239603167272,14.4987598986465,
131.300415425815)) ;
#115265=CARTESIAN_POINT('Ctrl Pts',(-20.539754785129,14.5035045718472,131.021276419093)) ;
#115266=CARTESIAN_POINT('Ctrl Pts',(-20.4588117616689,14.4313229997249,
130.751803459987)) ;
#115267=CARTESIAN_POINT('Ctrl Pts',(-20.3868956375626,14.286096674379,130.508478859911)) ;
#115268=CARTESIAN_POINT('Ctrl Pts',(-20.3308554449234,14.0806888556304,
130.311826279916)) ;
#115269=CARTESIAN_POINT('Ctrl Pts',(-20.2944696102375,13.8265805447723,
130.172317712221)) ;
#115270=CARTESIAN_POINT('Ctrl Pts',(-20.2817095072984,13.5441879409374,
130.101929815543)) ;
#115271=CARTESIAN_POINT('Ctrl Pts',(-20.2939970046262,13.2530370689606,
130.104694604891)) ;
#115272=CARTESIAN_POINT('Ctrl Pts',(-20.3312192505214,12.9741114175935,
130.18030810907)) ;
#115273=CARTESIAN_POINT('Ctrl Pts',(-20.391477731723,12.7272119216586,130.323195480133)) ;
#115274=CARTESIAN_POINT('Ctrl Pts',(-20.4710215017653,12.5305677659782,
130.522476172394)) ;
#115275=CARTESIAN_POINT('Ctrl Pts',(-20.5648765077218,12.3976028767503,
130.763584707341)) ;
#115276=CARTESIAN_POINT('Ctrl Pts',(-20.6677354645716,12.3378877564715,
131.030810858964)) ;
#115277=CARTESIAN_POINT('Ctrl Pts',(-20.771610142133,12.3561146457162,131.301258410359)) ;
#115278=CARTESIAN_POINT('Ctrl Pts',(-20.8710140356471,12.4504996091204,
131.558507272223)) ;
#115279=CARTESIAN_POINT('Ctrl Pts',(-20.9591976245712,12.6151918179393,
131.782920165643)) ;
#115280=CARTESIAN_POINT('Ctrl Pts',(-21.0301909969835,12.8367627956422,
131.957264907826)) ;
#115281=CARTESIAN_POINT('Ctrl Pts',(-21.0802720431719,13.102471284239,132.070248175628)) ;
#115282=CARTESIAN_POINT('Ctrl Pts',(-21.1058128562322,13.388098474674,132.11192368682)) ;
#115283=CARTESIAN_POINT('Ctrl Pts',(-21.1063578527298,13.6786302634614,
132.08028850925)) ;
#115284=CARTESIAN_POINT('Ctrl Pts',(-21.0823275663731,13.9495118019851,
131.977027551482)) ;
#115285=CARTESIAN_POINT('Ctrl Pts',(-21.0362217842379,14.1831630717315,
131.809216673534)) ;
#115286=CARTESIAN_POINT('Ctrl Pts',(-20.9721884045855,14.3622887251467,
131.589091305906)) ;
#115287=CARTESIAN_POINT('Ctrl Pts',(-20.8947792880245,14.4748192529362,
131.32962547702)) ;
#115288=CARTESIAN_POINT('Ctrl Pts',(-20.8116749026299,14.5109473630978,
131.053861074448)) ;
#115289=CARTESIAN_POINT('Ctrl Pts',(-20.7286272549608,14.46989386631,130.778195045776)) ;
#115290=CARTESIAN_POINT('Ctrl Pts',(-20.6522431108941,14.3536144736526,
130.521907930923)) ;
#115291=CARTESIAN_POINT('Ctrl Pts',(-20.5889583813436,14.17062113719,130.303892930056)) ;
#115292=CARTESIAN_POINT('Ctrl Pts',(-20.5440524129988,13.933736573907,130.13953810035)) ;
#115293=CARTESIAN_POINT('Ctrl Pts',(-20.5214975045223,13.6617104442443,
130.040649083481)) ;
#115294=CARTESIAN_POINT('Ctrl Pts',(-20.5235105668905,13.3701432171844,
130.013237741548)) ;
#115295=CARTESIAN_POINT('Ctrl Pts',(-20.5508607538459,13.0839501475181,
130.0600249237)) ;
#115296=CARTESIAN_POINT('Ctrl Pts',(-20.6019342296123,12.8226369063403,
130.176200002378)) ;
#115297=CARTESIAN_POINT('Ctrl Pts',(-20.674162245095,12.6036153158418,130.354083975274)) ;
#115298=CARTESIAN_POINT('Ctrl Pts',(-20.7628382753172,12.4432239429731,
130.580060592785)) ;
#115299=CARTESIAN_POINT('Ctrl Pts',(-20.8633579914741,12.3525997513282,
130.840351394468)) ;
#115300=CARTESIAN_POINT('Ctrl Pts',(-20.9671168641114,12.3393903655815,
131.110528978872)) ;
#115301=CARTESIAN_POINT('Ctrl Pts',(-21.0694306011919,12.403468098602,131.376231401918)) ;
#115302=CARTESIAN_POINT('Ctrl Pts',(-21.1627219404933,12.5405072085783,
131.615661785443)) ;
#115303=CARTESIAN_POINT('Ctrl Pts',(-21.2416127937835,12.7420005519616,
131.812839172161)) ;
#115304=CARTESIAN_POINT('Ctrl Pts',(-21.3001704333997,12.9900801149227,
131.950949061272)) ;
#115305=CARTESIAN_POINT('Ctrl Pts',(-21.3360159038547,13.2708158721555,
132.022475029764)) ;
#115306=CARTESIAN_POINT('Ctrl Pts',(-21.3467250085586,13.5613604134334,
132.020708203514)) ;
#115307=CARTESIAN_POINT('Ctrl Pts',(-21.332530072888,13.8428560081929,131.946099675255)) ;
#115308=CARTESIAN_POINT('Ctrl Pts',(-21.2946880005883,14.0951246502648,
131.802259522002)) ;
#115309=CARTESIAN_POINT('Ctrl Pts',(-21.2376357521135,14.2968154125605,
131.602698948677)) ;
#115310=CARTESIAN_POINT('Ctrl Pts',(-21.164806246768,14.4382062812648,131.356634806151)) ;
#115311=CARTESIAN_POINT('Ctrl Pts',(-21.0832408338308,14.5055713938207,
131.085254319312)) ;
#115312=CARTESIAN_POINT('Ctrl Pts',(-20.9994162423038,14.4957941932041,
130.807360837672)) ;
#115313=CARTESIAN_POINT('Ctrl Pts',(-20.9195959138854,14.4095662340998,
130.541102349046)) ;
#115314=CARTESIAN_POINT('Ctrl Pts',(-20.8500186277359,14.2515335127425,
130.304558118666)) ;
#115315=CARTESIAN_POINT('Ctrl Pts',(-20.7972486154139,14.0347236874785,
130.11728882556)) ;
#115316=CARTESIAN_POINT('Ctrl Pts',(-20.7653613268004,13.7751700114088,
129.991129528377)) ;
#115317=CARTESIAN_POINT('Ctrl Pts',(-20.7571817990629,13.489555102194,129.934113768398)) ;
#115318=CARTESIAN_POINT('Ctrl Pts',(-20.7742556911792,13.1989624545804,
129.950844344899)) ;
#115319=CARTESIAN_POINT('Ctrl Pts',(-20.8159809707414,12.9245155762064,
130.03960916018)) ;
#115320=CARTESIAN_POINT('Ctrl Pts',(-20.8805367450398,12.6850932088169,
130.194926855194)) ;
#115321=CARTESIAN_POINT('Ctrl Pts',(-20.9626356003938,12.5007200500438,
130.401901459438)) ;
#115322=CARTESIAN_POINT('Ctrl Pts',(-21.0591957946408,12.3802348015134,
130.650687618331)) ;
#115323=CARTESIAN_POINT('Ctrl Pts',(-21.1622370545661,12.3354177830535,
130.918672003733)) ;
#115324=CARTESIAN_POINT('Ctrl Pts',(-21.2662887681593,12.3682931650198,
131.189443526458)) ;
#115325=CARTESIAN_POINT('Ctrl Pts',(-21.3637199956931,12.4764500222757,
131.44102792815)) ;
#115326=CARTESIAN_POINT('Ctrl Pts',(-21.4490683123423,12.6527561756398,
131.657189302748)) ;
#115327=CARTESIAN_POINT('Ctrl Pts',(-21.5164968590452,12.8841372675975,
131.821041651181)) ;
#115328=CARTESIAN_POINT('Ctrl Pts',(-21.5620729321248,13.1550291136418,
131.920951331736)) ;
#115329=CARTESIAN_POINT('Ctrl Pts',(-21.5829990360394,13.4437302360126,
131.949026741888)) ;
#115330=CARTESIAN_POINT('Ctrl Pts',(-21.5787261653874,13.7319393007276,
131.903366364301)) ;
#115331=CARTESIAN_POINT('Ctrl Pts',(-21.5503975227815,13.9965481623833,
131.787623344815)) ;
#115332=CARTESIAN_POINT('Ctrl Pts',(-21.5005342471165,14.2215298170475,
131.608800269925)) ;
#115333=CARTESIAN_POINT('Ctrl Pts',(-21.4333938850247,14.3891483272759,
131.379489123203)) ;
#115334=CARTESIAN_POINT('Ctrl Pts',(-21.3548735774567,14.4871687024338,
131.117033634355)) ;
#115335=CARTESIAN_POINT('Ctrl Pts',(-21.2709428978837,14.5093408079897,
130.838711318976)) ;
#115336=CARTESIAN_POINT('Ctrl Pts',(-21.1882422406468,14.4530254583256,
130.563868416307)) ;
#115337=CARTESIAN_POINT('Ctrl Pts',(-21.1143270880585,14.3240305585518,
130.31499305445)) ;
#115338=CARTESIAN_POINT('Ctrl Pts',(-21.0539688868397,14.1290979717854,
130.105410602035)) ;
#115339=CARTESIAN_POINT('Ctrl Pts',(-21.0132069302916,13.8855604155571,
129.953378103653)) ;
#115340=CARTESIAN_POINT('Ctrl Pts',(-20.9950030451873,13.6058416707122,
129.866845755651)) ;
#115341=CARTESIAN_POINT('Ctrl Pts',(-21.0018793397198,13.3160021377259,
129.853947611582)) ;
#115342=CARTESIAN_POINT('Ctrl Pts',(-21.0337293398582,13.0326886676077,
129.913868033499)) ;
#115343=CARTESIAN_POINT('Ctrl Pts',(-21.0893772116349,12.7766372190837,
130.043216529831)) ;
#115344=CARTESIAN_POINT('Ctrl Pts',(-21.1653161877122,12.5676698161814,
130.231901557219)) ;
#115345=CARTESIAN_POINT('Ctrl Pts',(-21.2561790285771,12.4206517790888,
130.464404545457)) ;
#115346=CARTESIAN_POINT('Ctrl Pts',(-21.3575675366688,12.3443150505119,
130.727387699059)) ;
#115347=CARTESIAN_POINT('Ctrl Pts',(-21.4618210845223,12.3454567433165,
130.998884337509)) ;
#115348=CARTESIAN_POINT('Ctrl Pts',(-21.5631430702427,12.4241540146565,
131.261630006307)) ;
#115349=CARTESIAN_POINT('Ctrl Pts',(-21.6537810155053,12.5736454649868,
131.493407152973)) ;
#115350=CARTESIAN_POINT('Ctrl Pts',(-21.7290950924145,12.7844244258342,
131.680270904741)) ;
#115351=CARTESIAN_POINT('Ctrl Pts',(-21.7839298109933,13.041264478038,131.807295952736)) ;
#115352=CARTESIAN_POINT('Ctrl Pts',(-21.8150448539116,13.3250313838274,
131.865081031141)) ;
#115353=CARTESIAN_POINT('Ctrl Pts',(-21.8210632536644,13.6156492492809,
131.849571033927)) ;
#115354=CARTESIAN_POINT('Ctrl Pts',(-21.8022545212773,13.8929002803611,
131.761487721122)) ;
#115355=CARTESIAN_POINT('Ctrl Pts',(-21.7605924585031,14.1366366428793,
131.606614879296)) ;
#115356=CARTESIAN_POINT('Ctrl Pts',(-21.6999698317163,14.3287833833703,
131.396421302764)) ;
#115357=CARTESIAN_POINT('Ctrl Pts',(-21.6253197774301,14.4563288342089,
131.145218098165)) ;
#115358=CARTESIAN_POINT('Ctrl Pts',(-21.5425945750513,14.5097636463918,
130.870367772935)) ;
#115359=CARTESIAN_POINT('Ctrl Pts',(-21.4589621479375,14.4852491819093,
130.593003563587)) ;
#115360=CARTESIAN_POINT('Ctrl Pts',(-21.380714091029,14.385213180382,130.331360934625)) ;
#115361=CARTESIAN_POINT('Ctrl Pts',(-21.3138290434139,14.2148994362801,
130.102677640231)) ;
#115362=CARTESIAN_POINT('Ctrl Pts',(-21.264802027938,13.9895605141043,129.92646714371)) ;
#115363=CARTESIAN_POINT('Ctrl Pts',(-21.2370048320792,13.7226496289756,
129.812102485109)) ;
#115364=CARTESIAN_POINT('Ctrl Pts',(-21.2336042417307,13.4342098859693,
129.769013814372)) ;
#115365=CARTESIAN_POINT('Ctrl Pts',(-21.2553236046358,13.1458182759752,
129.799407215841)) ;
#115366=CARTESIAN_POINT('Ctrl Pts',(-21.3016988392798,12.8759127132536,
129.901648132077)) ;
#115367=CARTESIAN_POINT('Ctrl Pts',(-21.3694669987003,12.6468868556867,
130.066623481143)) ;
#115368=CARTESIAN_POINT('Ctrl Pts',(-21.4553373193102,12.4721832296684,
130.284273605613)) ;
#115369=CARTESIAN_POINT('Ctrl Pts',(-21.5530256217249,12.3661739274481,
130.536616813639)) ;
#115370=CARTESIAN_POINT('Ctrl Pts',(-21.6575177270796,12.3355863385396,
130.808562220896)) ;
#115371=CARTESIAN_POINT('Ctrl Pts',(-21.7604456918656,12.3831198658751,
131.076206190241)) ;
#115372=CARTESIAN_POINT('Ctrl Pts',(-21.8563696469902,12.5053833023315,
131.323242388746)) ;
#115373=CARTESIAN_POINT('Ctrl Pts',(-21.9382966693068,12.6923270702948,
131.529584453516)) ;
#115374=CARTESIAN_POINT('Ctrl Pts',(-22.0021645015312,12.9335865705139,
131.682862448256)) ;
#115375=CARTESIAN_POINT('Ctrl Pts',(-22.0430213128192,13.2085814539572,
131.769129801508)) ;
#115376=CARTESIAN_POINT('Ctrl Pts',(-22.0592352836556,13.4990557588074,
131.783380739882)) ;
#115377=CARTESIAN_POINT('Ctrl Pts',(-22.0503004073671,13.7836907462661,
131.724216167399)) ;
#115378=CARTESIAN_POINT('Ctrl Pts',(-22.0176371901026,14.0427281414566,
131.595717480909)) ;
#115379=CARTESIAN_POINT('Ctrl Pts',(-21.9641995370827,14.2577309750281,
131.406490661624)) ;
#115380=CARTESIAN_POINT('Ctrl Pts',(-21.8944782363852,14.4131664617501,
131.169654967239)) ;
#115381=CARTESIAN_POINT('Ctrl Pts',(-21.8141620072022,14.4973755702956,
130.901832610092)) ;
#115382=CARTESIAN_POINT('Ctrl Pts',(-21.7303937720881,14.5046724130054,
130.624142862364)) ;
#115383=CARTESIAN_POINT('Ctrl Pts',(-21.6486693225774,14.4343111747756,
130.352140919931)) ;
#115384=CARTESIAN_POINT('Ctrl Pts',(-21.5766530687314,14.2913904033354,
130.108640611113)) ;
#115385=CARTESIAN_POINT('Ctrl Pts',(-21.5199914526865,14.0872940403586,
129.910112364196)) ;
#115386=CARTESIAN_POINT('Ctrl Pts',(-21.4830382408884,13.8349907742835,
129.769035274606)) ;
#115387=CARTESIAN_POINT('Ctrl Pts',(-21.4694985396213,13.5522018199285,
129.696252361388)) ;
#115388=CARTESIAN_POINT('Ctrl Pts',(-21.4810885813508,13.2611771320633,
129.697002826515)) ;
#115389=CARTESIAN_POINT('Ctrl Pts',(-21.5176805732444,12.9814107201437,
129.770743949859)) ;
#115390=CARTESIAN_POINT('Ctrl Pts',(-21.5771191123903,12.7341369610279,
129.911345858839)) ;
#115391=CARTESIAN_POINT('Ctrl Pts',(-21.6563209788842,12.535166216503,130.109544290444)) ;
#115392=CARTESIAN_POINT('Ctrl Pts',(-21.7502713534583,12.4000170891871,
130.350799701057)) ;
#115393=CARTESIAN_POINT('Ctrl Pts',(-21.8524815344102,12.3385941106561,
130.616296707476)) ;
#115394=CARTESIAN_POINT('Ctrl Pts',(-21.9565712501459,12.3545286685026,
130.887315313701)) ;
#115395=CARTESIAN_POINT('Ctrl Pts',(-22.0562577481496,12.4469846430608,
131.14537139149)) ;
#115396=CARTESIAN_POINT('Ctrl Pts',(-22.1449360417052,12.6102579412087,
131.371180205731)) ;
#115397=CARTESIAN_POINT('Ctrl Pts',(-22.2161370464207,12.8296977311719,
131.546256445573)) ;
#115398=CARTESIAN_POINT('Ctrl Pts',(-22.2667592690025,13.0929763552362,
131.660982603106)) ;
#115399=CARTESIAN_POINT('Ctrl Pts',(-22.2932535098378,13.3798715107165,
131.705248169509)) ;
#115400=CARTESIAN_POINT('Ctrl Pts',(-22.2944576782056,13.6705227535771,
131.675549761758)) ;
#115401=CARTESIAN_POINT('Ctrl Pts',(-22.2711545117995,13.9421700423004,
131.57442408932)) ;
#115402=CARTESIAN_POINT('Ctrl Pts',(-22.2253820822901,14.1780191011813,
131.407446635602)) ;
#115403=CARTESIAN_POINT('Ctrl Pts',(-22.1619741826909,14.3579768124892,
131.189272795754)) ;
#115404=CARTESIAN_POINT('Ctrl Pts',(-22.0850483275451,14.4725057553617,
130.931291857228)) ;
#115405=CARTESIAN_POINT('Ctrl Pts',(-22.0018889458697,14.5110248787396,
130.655306915796)) ;
#115406=CARTESIAN_POINT('Ctrl Pts',(-21.9186831269904,14.4721191969269,
130.37915685792)) ;
#115407=CARTESIAN_POINT('Ctrl Pts',(-21.8419983594231,14.3577454336847,
130.121978165508)) ;
#115408=CARTESIAN_POINT('Ctrl Pts',(-21.7784559689967,14.1770688666527,
129.90331119887)) ;
#115409=CARTESIAN_POINT('Ctrl Pts',(-21.7328730623761,13.9416997327419,
129.73698112711)) ;
#115410=CARTESIAN_POINT('Ctrl Pts',(-21.7095937547817,13.6694104353782,
129.635852457523)) ;
#115411=CARTESIAN_POINT('Ctrl Pts',(-21.7108544164153,13.3798585935035,
129.60644988842)) ;
#115412=CARTESIAN_POINT('Ctrl Pts',(-21.7373587408651,13.0927640382574,
129.650717582232)) ;
#115413=CARTESIAN_POINT('Ctrl Pts',(-21.7879727694938,12.8294542733058,
129.765423278)) ;
#115414=CARTESIAN_POINT('Ctrl Pts',(-21.8596572059499,12.6090080043084,
129.941724810289)) ;
#115415=CARTESIAN_POINT('Ctrl Pts',(-21.9481186483126,12.4466659582347,
130.167016290758)) ;
#115416=CARTESIAN_POINT('Ctrl Pts',(-22.0478029406896,12.3544265354386,
130.425067159699)) ;
#115417=CARTESIAN_POINT('Ctrl Pts',(-22.1517530143636,12.338485550426,130.695728652991)) ;
#115418=CARTESIAN_POINT('Ctrl Pts',(-22.2547791723717,12.4009576070215,
130.963329774343)) ;
#115419=CARTESIAN_POINT('Ctrl Pts',(-22.3479076849026,12.5356622675021,
131.202441690569)) ;
#115420=CARTESIAN_POINT('Ctrl Pts',(-22.427039674185,12.7342792931547,131.400473047047)) ;
#115421=CARTESIAN_POINT('Ctrl Pts',(-22.4865817751364,12.9822470405306,
131.541298758196)) ;
#115422=CARTESIAN_POINT('Ctrl Pts',(-22.5231351067208,13.2626104241267,
131.614868935857)) ;
#115423=CARTESIAN_POINT('Ctrl Pts',(-22.5345613145019,13.5537330357078,
131.615129217148)) ;
#115424=CARTESIAN_POINT('Ctrl Pts',(-22.5210072175352,13.8350780443648,
131.542464925158)) ;
#115425=CARTESIAN_POINT('Ctrl Pts',(-22.4841282635127,14.0872562376869,
131.401629162015)) ;
#115426=CARTESIAN_POINT('Ctrl Pts',(-22.4271936380161,14.2922552735091,
131.202157542)) ;
#115427=CARTESIAN_POINT('Ctrl Pts',(-22.3548468095764,14.4349645919609,
130.957589374496)) ;
#115428=CARTESIAN_POINT('Ctrl Pts',(-22.2738049730186,14.5045540577175,
130.687866104784)) ;
#115429=CARTESIAN_POINT('Ctrl Pts',(-22.1896316409164,14.4973581396257,
130.408831550043)) ;
#115430=CARTESIAN_POINT('Ctrl Pts',(-22.1093343470203,14.4126016842873,
130.14105358009)) ;
#115431=CARTESIAN_POINT('Ctrl Pts',(-22.0399356599868,14.2578370889756,
129.905309744937)) ;
#115432=CARTESIAN_POINT('Ctrl Pts',(-21.9863765422796,14.0423606370671,
129.715650705837)) ;
#115433=CARTESIAN_POINT('Ctrl Pts',(-21.9537345461485,13.7833430848993,
129.58722594006)) ;
#115434=CARTESIAN_POINT('Ctrl Pts',(-21.9448743026681,13.4972454461382,
129.528113894271)) ;
#115435=CARTESIAN_POINT('Ctrl Pts',(-21.9611494569257,13.2077137971034,
129.542654652447)) ;
#115436=CARTESIAN_POINT('Ctrl Pts',(-22.002288346979,12.9318531124,129.629618831657)) ;
#115437=CARTESIAN_POINT('Ctrl Pts',(-22.0658546135328,12.6922552108513,
129.782222524194)) ;
#115438=CARTESIAN_POINT('Ctrl Pts',(-22.1480419825475,12.504666487009,129.989213929092)) ;
#115439=CARTESIAN_POINT('Ctrl Pts',(-22.2443302147763,12.3825157199122,
130.237218364436)) ;
#115440=CARTESIAN_POINT('Ctrl Pts',(-22.3470392380216,12.3357140444497,
130.504298662281)) ;
#115441=CARTESIAN_POINT('Ctrl Pts',(-22.4509464733217,12.3660679541908,
130.774724556597)) ;
#115442=CARTESIAN_POINT('Ctrl Pts',(-22.549161413923,12.4727573812884,131.028420389511)) ;
#115443=CARTESIAN_POINT('Ctrl Pts',(-22.6347030566716,12.6471452986828,
131.245220928735)) ;
#115444=CARTESIAN_POINT('Ctrl Pts',(-22.7025433269035,12.8766362181276,
131.410346416835)) ;
#115445=CARTESIAN_POINT('Ctrl Pts',(-22.7487814948906,13.1457609561308,
131.512289397035)) ;
#115446=CARTESIAN_POINT('Ctrl Pts',(-22.7705721874272,13.436208516762,131.542656742186)) ;
#115447=CARTESIAN_POINT('Ctrl Pts',(-22.7669909559281,13.7232902020091,
131.499187113643)) ;
#115448=CARTESIAN_POINT('Ctrl Pts',(-22.739314974999,13.9896012284326,131.385259077282)) ;
#115449=CARTESIAN_POINT('Ctrl Pts',(-22.6899563353196,14.2159296230216,
131.207905951156)) ;
#115450=CARTESIAN_POINT('Ctrl Pts',(-22.6233672864789,14.3851342144556,
130.980263042488)) ;
#115451=CARTESIAN_POINT('Ctrl Pts',(-22.5449702570784,14.4854516976048,
130.718115056966)) ;
#115452=CARTESIAN_POINT('Ctrl Pts',(-22.461265093064,14.5096986607512,130.440515127017)) ;
#115453=CARTESIAN_POINT('Ctrl Pts',(-22.378621004999,14.4561737731647,130.165930931039)) ;
#115454=CARTESIAN_POINT('Ctrl Pts',(-22.3039082628437,14.3282785458503,
129.914502352423)) ;
#115455=CARTESIAN_POINT('Ctrl Pts',(-22.2434277952934,14.1363003864466,
129.704779792514)) ;
#115456=CARTESIAN_POINT('Ctrl Pts',(-22.2017896977858,13.8924839857025,
129.549971716453)) ;
#115457=CARTESIAN_POINT('Ctrl Pts',(-22.1830205641406,13.6154602436594,
129.462035111654)) ;
#115458=CARTESIAN_POINT('Ctrl Pts',(-22.1890712067793,13.3244466531158,
129.446574293387)) ;
#115459=CARTESIAN_POINT('Ctrl Pts',(-22.2202555636145,13.0407282159145,
129.504562629151)) ;
#115460=CARTESIAN_POINT('Ctrl Pts',(-22.2750211321796,12.7843965627726,
129.631442703902)) ;
#115461=CARTESIAN_POINT('Ctrl Pts',(-22.3503429335631,12.5734338880589,
129.818316417424)) ;
#115462=CARTESIAN_POINT('Ctrl Pts',(-22.4414173268538,12.4236459559127,
130.051229799352)) ;
#115463=CARTESIAN_POINT('Ctrl Pts',(-22.5421394962141,12.3455712635568,
130.312426708327)) ;
#115464=CARTESIAN_POINT('Ctrl Pts',(-22.6467265172187,12.3443023671055,
130.584788395612)) ;
#115465=CARTESIAN_POINT('Ctrl Pts',(-22.7481657330948,12.420933178294,130.847899857883)) ;
#115466=CARTESIAN_POINT('Ctrl Pts',(-22.8392055009209,12.5684896870098,
131.080841902066)) ;
#115467=CARTESIAN_POINT('Ctrl Pts',(-22.9152137261507,12.7783872300958,
131.269645560269)) ;
#115468=CARTESIAN_POINT('Ctrl Pts',(-22.9705402435953,13.0341435528073,
131.398130661038)) ;
#115469=CARTESIAN_POINT('Ctrl Pts',(-23.0022377817911,13.3161552682329,
131.457761074721)) ;
#115470=CARTESIAN_POINT('Ctrl Pts',(-23.009059140071,13.6077102167408,131.444501189894)) ;
#115471=CARTESIAN_POINT('Ctrl Pts',(-22.9907943770449,13.8863966863271,
131.357908893058)) ;
#115472=CARTESIAN_POINT('Ctrl Pts',(-22.9497275238959,14.1306963082603,
131.204837242028)) ;
#115473=CARTESIAN_POINT('Ctrl Pts',(-22.8897860606364,14.3238933046915,
130.996741057129)) ;
#115474=CARTESIAN_POINT('Ctrl Pts',(-22.8155047276147,14.4535137780173,
130.746625113997)) ;
#115475=CARTESIAN_POINT('Ctrl Pts',(-22.7328983548189,14.5094099168095,
130.47211370142)) ;
#115476=CARTESIAN_POINT('Ctrl Pts',(-22.6487340748289,14.4867701673882,
130.193005786419)) ;
#115477=CARTESIAN_POINT('Ctrl Pts',(-22.5707021703194,14.3890643828725,
129.932173416396)) ;
#115478=CARTESIAN_POINT('Ctrl Pts',(-22.5034195621283,14.2211869107964,
129.70237977909)) ;
#115479=CARTESIAN_POINT('Ctrl Pts',(-22.4535961395973,13.9958858020985,
129.523655290175)) ;
#115480=CARTESIAN_POINT('Ctrl Pts',(-22.4253306349521,13.7314793548645,
129.40812642471)) ;
#115481=CARTESIAN_POINT('Ctrl Pts',(-22.4210875175899,13.4423639400344,
129.362455182987)) ;
#115482=CARTESIAN_POINT('Ctrl Pts',(-22.4422895478426,13.1530743203904,
129.391256495026)) ;
#115483=CARTESIAN_POINT('Ctrl Pts',(-22.487580667877,12.8842566111771,129.490582827144)) ;
#115484=CARTESIAN_POINT('Ctrl Pts',(-22.5552977498778,12.6519995362001,
129.655140460866)) ;
#115485=CARTESIAN_POINT('Ctrl Pts',(-22.6402716313289,12.4766942436469,
129.870371614395)) ;
#115486=CARTESIAN_POINT('Ctrl Pts',(-22.7378885944903,12.3681120678918,
130.122423877062)) ;
#115487=CARTESIAN_POINT('Ctrl Pts',(-22.8423855341256,12.3353450096833,
130.394363079284)) ;
#115488=CARTESIAN_POINT('Ctrl Pts',(-22.9455053804218,12.3808789292608,
130.66253674151)) ;
#115489=CARTESIAN_POINT('Ctrl Pts',(-23.0414119491019,12.5006496739186,
130.90963712832)) ;
#115490=CARTESIAN_POINT('Ctrl Pts',(-23.1239874820464,12.6862348924807,
131.117800379368)) ;
#115491=CARTESIAN_POINT('Ctrl Pts',(-23.1882404954987,12.9253055289241,
131.272326344278)) ;
#115492=CARTESIAN_POINT('Ctrl Pts',(-23.2299054869804,13.1996774467986,
131.360925356354)) ;
#115493=CARTESIAN_POINT('Ctrl Pts',(-23.2469197712831,13.4900583198245,
131.37750845876)) ;
#115494=CARTESIAN_POINT('Ctrl Pts',(-23.2386702442009,13.7765694769724,
131.320183787516)) ;
#115495=CARTESIAN_POINT('Ctrl Pts',(-23.2064532063664,14.036835662277,131.192930360202)) ;
#115496=CARTESIAN_POINT('Ctrl Pts',(-23.1537890318512,14.2522894974628,
131.006121661116)) ;
#115497=CARTESIAN_POINT('Ctrl Pts',(-23.0841408392017,14.410142650821,130.769355953609)) ;
#115498=CARTESIAN_POINT('Ctrl Pts',(-23.0044224542759,14.4959011359271,
130.503451200898)) ;
#115499=CARTESIAN_POINT('Ctrl Pts',(-22.9205051252153,14.5055615596735,
130.225254015656)) ;
#115500=CARTESIAN_POINT('Ctrl Pts',(-22.8387642579551,14.4373879166647,
129.953265322989)) ;
#115501=CARTESIAN_POINT('Ctrl Pts',(-22.7664377143828,14.2968056087925,
129.708895562602)) ;
#115502=CARTESIAN_POINT('Ctrl Pts',(-22.7090205846332,14.0934340145334,
129.508020332236)) ;
#115503=CARTESIAN_POINT('Ctrl Pts',(-22.6715788423865,13.8423638114029,
129.365551179356)) ;
#115504=CARTESIAN_POINT('Ctrl Pts',(-22.6573294356865,13.5615577206812,
129.290854833297)) ;
#115505=CARTESIAN_POINT('Ctrl Pts',(-22.6681862864359,13.2694348944804,
129.289338191419)) ;
#115506=CARTESIAN_POINT('Ctrl Pts',(-22.7039617574597,12.9897647818979,
129.360785289403)) ;
#115507=CARTESIAN_POINT('Ctrl Pts',(-22.7629534424542,12.7403852471457,
129.499963464368)) ;
#115508=CARTESIAN_POINT('Ctrl Pts',(-22.8415892215112,12.5401778472151,
129.696554511139)) ;
#115509=CARTESIAN_POINT('Ctrl Pts',(-22.9348979213409,12.4032538731495,
129.936029182917)) ;
#115510=CARTESIAN_POINT('Ctrl Pts',(-23.0370685674519,12.3392654765734,
130.201366375023)) ;
#115511=CARTESIAN_POINT('Ctrl Pts',(-23.141478431911,12.3529795705707,130.473233214815)) ;
#115512=CARTESIAN_POINT('Ctrl Pts',(-23.2412861780916,12.44341496887,130.731668708428)) ;
#115513=CARTESIAN_POINT('Ctrl Pts',(-23.330047912579,12.6038142404483,130.957868037024)) ;
#115514=CARTESIAN_POINT('Ctrl Pts',(-23.4023245485338,12.8232746698558,
131.135851245433)) ;
#115515=CARTESIAN_POINT('Ctrl Pts',(-23.4533693512746,13.0848674095602,
131.251920028465)) ;
#115516=CARTESIAN_POINT('Ctrl Pts',(-23.4806176034136,13.3712340427374,
131.298395105942)) ;
#115517=CARTESIAN_POINT('Ctrl Pts',(-23.4825810779044,13.6620670155129,
131.270922868641)) ;
#115518=CARTESIAN_POINT('Ctrl Pts',(-23.4599091408466,13.9347879219274,
131.171598398464)) ;
#115519=CARTESIAN_POINT('Ctrl Pts',(-23.4149763968351,14.1711547034761,
131.007212926626)) ;
#115520=CARTESIAN_POINT('Ctrl Pts',(-23.3516961209413,14.3538985958079,
130.789228498426)) ;
#115521=CARTESIAN_POINT('Ctrl Pts',(-23.2754093744269,14.4699515410886,
130.533273425003)) ;
#115522=CARTESIAN_POINT('Ctrl Pts',(-23.1921867842084,14.511011729743,130.257027506385)) ;
#115523=CARTESIAN_POINT('Ctrl Pts',(-23.1089561500767,14.4745400421894,
129.980842840064)) ;
#115524=CARTESIAN_POINT('Ctrl Pts',(-23.031552894356,14.3614974996119,129.721369859714)) ;
#115525=CARTESIAN_POINT('Ctrl Pts',(-22.9678477580129,14.1829580277845,
129.502345220066)) ;
#115526=CARTESIAN_POINT('Ctrl Pts',(-22.9216856506781,13.9492404929465,
129.334353763701)) ;
#115527=CARTESIAN_POINT('Ctrl Pts',(-22.8977300159152,13.6775800982586,
129.231228230102)) ;
#115528=CARTESIAN_POINT('Ctrl Pts',(-22.8981933527482,13.3886494635436,
129.19954520776)) ;
#115529=CARTESIAN_POINT('Ctrl Pts',(-22.9242400045738,13.0993478015478,
129.242254988579)) ;
#115530=CARTESIAN_POINT('Ctrl Pts',(-22.9739037222349,12.8369458310676,
129.354415199943)) ;
#115531=CARTESIAN_POINT('Ctrl Pts',(-23.0453252131747,12.6140529768099,
129.529801908795)) ;
#115532=CARTESIAN_POINT('Ctrl Pts',(-23.1330410816671,12.4507323341902,
129.753058144926)) ;
#115533=CARTESIAN_POINT('Ctrl Pts',(-23.2324941335687,12.3558899306528,
130.010420059215)) ;
#115534=CARTESIAN_POINT('Ctrl Pts',(-23.3371521212107,12.3380969081111,
130.282910607247)) ;
#115535=CARTESIAN_POINT('Ctrl Pts',(-23.4390406262999,12.3976016694818,
130.547608591386)) ;
#115536=CARTESIAN_POINT('Ctrl Pts',(-23.5331839274626,12.530583824708,130.789474316628)) ;
#115537=CARTESIAN_POINT('Ctrl Pts',(-23.6129508354768,12.7283490506027,
130.989275182951)) ;
#115538=CARTESIAN_POINT('Ctrl Pts',(-23.6728864226876,12.9742771227128,
131.13136588872)) ;
#115539=CARTESIAN_POINT('Ctrl Pts',(-23.71018774412,13.2539376227601,131.207121504005)) ;
#115540=CARTESIAN_POINT('Ctrl Pts',(-23.7223865299285,13.5450903335013,
131.209633661058)) ;
#115541=CARTESIAN_POINT('Ctrl Pts',(-23.7094914718236,13.8275787514848,
131.138820807372)) ;
#115542=CARTESIAN_POINT('Ctrl Pts',(-23.6732974807833,14.080619519853,131.000028693289)) ;
#115543=CARTESIAN_POINT('Ctrl Pts',(-23.616590785082,14.2877392133105,130.801091824847)) ;
#115544=CARTESIAN_POINT('Ctrl Pts',(-23.5452916636683,14.431213841156,130.559896288173)) ;
#115545=CARTESIAN_POINT('Ctrl Pts',(-23.4637700924587,14.5038738166411,
130.288489711948)) ;
#115546=CARTESIAN_POINT('Ctrl Pts',(-23.3797591259085,14.4984557576167,
130.010000564517)) ;
#115547=CARTESIAN_POINT('Ctrl Pts',(-23.2994671912968,14.4164646825051,
129.742342495005)) ;
#115548=CARTESIAN_POINT('Ctrl Pts',(-23.2292002172557,14.2622140461571,
129.503806387235)) ;
#115549=CARTESIAN_POINT('Ctrl Pts',(-23.1755337197615,14.0497489487789,
129.314087251754)) ;
#115550=CARTESIAN_POINT('Ctrl Pts',(-23.1420903990703,13.7905258352839,
129.183151437944)) ;
#115551=CARTESIAN_POINT('Ctrl Pts',(-23.1325295042077,13.506486494377,129.12218848079)) ;
#115552=CARTESIAN_POINT('Ctrl Pts',(-23.1482921851681,13.2142515667239,
129.134926916223)) ;
#115553=CARTESIAN_POINT('Ctrl Pts',(-23.188353413262,12.9406232851689,129.219102820939)) ;
#115554=CARTESIAN_POINT('Ctrl Pts',(-23.2515823582444,12.6982138740687,
129.370525672368)) ;
#115555=CARTESIAN_POINT('Ctrl Pts',(-23.3330631497147,12.5096112048297,
129.575565311669)) ;
#115556=CARTESIAN_POINT('Ctrl Pts',(-23.4290906890084,12.3850648620669,
129.822774700949)) ;
#115557=CARTESIAN_POINT('Ctrl Pts',(-23.531784997696,12.3359713268051,130.089781167871)) ;
#115558=CARTESIAN_POINT('Ctrl Pts',(-23.6357879798494,12.3641515700291,
130.360476235555)) ;
#115559=CARTESIAN_POINT('Ctrl Pts',(-23.7340953356143,12.4683944776065,
130.614508785511)) ;
#115560=CARTESIAN_POINT('Ctrl Pts',(-23.8203211365081,12.6414744910879,
130.833207334208)) ;
#115561=CARTESIAN_POINT('Ctrl Pts',(-23.8886881736005,12.8692739707259,
130.99991574651)) ;
#115562=CARTESIAN_POINT('Ctrl Pts',(-23.9357467861378,13.1394382839076,
131.104034823546)) ;
#115563=CARTESIAN_POINT('Ctrl Pts',(-23.9579774455155,13.4257125423889,
131.136139167156)) ;
#115564=CARTESIAN_POINT('Ctrl Pts',(-23.9552750237727,13.7153678926771,
131.094978168242)) ;
#115565=CARTESIAN_POINT('Ctrl Pts',(-23.9282090173285,13.9823826092166,
130.982854215722)) ;
#115566=CARTESIAN_POINT('Ctrl Pts',(-23.8793697422226,14.210351268189,130.806979650137)) ;
#115567=CARTESIAN_POINT('Ctrl Pts',(-23.8133153702057,14.3810373513132,
130.58096078673)) ;
#115568=CARTESIAN_POINT('Ctrl Pts',(-23.735209224892,14.4835203874639,130.319669563206)) ;
#115569=CARTESIAN_POINT('Ctrl Pts',(-23.6515414522142,14.5102051470099,
130.042171972968)) ;
#115570=CARTESIAN_POINT('Ctrl Pts',(-23.5684272969825,14.4584272467564,
129.766068717826)) ;
#115571=CARTESIAN_POINT('Ctrl Pts',(-23.4938231437372,14.3332271538461,
129.515148015428)) ;
#115572=CARTESIAN_POINT('Ctrl Pts',(-23.4326135115301,14.1422679027751,
129.303162687106)) ;
#115573=CARTESIAN_POINT('Ctrl Pts',(-23.3905185584406,13.9003526545792,
129.147122527455)) ;
#115574=CARTESIAN_POINT('Ctrl Pts',(-23.3709966570516,13.6237176044633,
129.056941792442)) ;
#115575=CARTESIAN_POINT('Ctrl Pts',(-23.3763211847102,13.3329588361478,
129.039378660403)) ;
#115576=CARTESIAN_POINT('Ctrl Pts',(-23.4068246825045,13.0482791472687,
129.095326134194)) ;
#115577=CARTESIAN_POINT('Ctrl Pts',(-23.4611218639704,12.7905984211716,
129.220781957599)) ;
#115578=CARTESIAN_POINT('Ctrl Pts',(-23.5355417145057,12.5792074314873,
129.405190030391)) ;
#115579=CARTESIAN_POINT('Ctrl Pts',(-23.6262276903051,12.4271420328258,
129.636951252849)) ;
#115580=CARTESIAN_POINT('Ctrl Pts',(-23.72702713312,12.3466854620337,129.898286196702)) ;
#115581=CARTESIAN_POINT('Ctrl Pts',(-23.8314987159718,12.3433384451733,
130.170343083653)) ;
#115582=CARTESIAN_POINT('Ctrl Pts',(-23.9327910170219,12.417256873973,130.433143999051)) ;
#115583=CARTESIAN_POINT('Ctrl Pts',(-24.0245736232509,12.5633304568432,
130.668126155051)) ;
#115584=CARTESIAN_POINT('Ctrl Pts',(-24.1008197720403,12.7708593905581,
130.857750684135)) ;
#115585=CARTESIAN_POINT('Ctrl Pts',(-24.1569294635632,13.025326349885,130.988518737243)) ;
#115586=CARTESIAN_POINT('Ctrl Pts',(-24.1894985627988,13.3082178025067,
131.05053265747)) ;
#115587=CARTESIAN_POINT('Ctrl Pts',(-24.196965740994,13.5990344955289,131.039249671657)) ;
#115588=CARTESIAN_POINT('Ctrl Pts',(-24.1795877670942,13.8774216043795,
130.955375021049)) ;
#115589=CARTESIAN_POINT('Ctrl Pts',(-24.1390939585473,14.1239848990119,
130.803863087357)) ;
#115590=CARTESIAN_POINT('Ctrl Pts',(-24.0794901932382,14.3192776170792,
130.596679031769)) ;
#115591=CARTESIAN_POINT('Ctrl Pts',(-24.0055352361048,14.4507732360595,
130.347522670003)) ;
#115592=CARTESIAN_POINT('Ctrl Pts',(-23.9233178114793,14.5087792678555,
130.074243320989)) ;
#115593=CARTESIAN_POINT('Ctrl Pts',(-23.8391129704671,14.4887238336712,
129.795024289797)) ;
#115594=CARTESIAN_POINT('Ctrl Pts',(-23.7605064372372,14.3928285084541,
129.532382450158)) ;
#115595=CARTESIAN_POINT('Ctrl Pts',(-23.6928180061624,14.2263682040696,
129.30137255382)) ;
#115596=CARTESIAN_POINT('Ctrl Pts',(-23.6426620351328,14.0038696460673,
129.121863214626)) ;
#115597=CARTESIAN_POINT('Ctrl Pts',(-23.613563581647,13.7389372008462,129.003713269081)) ;
#115598=CARTESIAN_POINT('Ctrl Pts',(-23.6086509708226,13.4518073715824,
128.956278206236)) ;
#115599=CARTESIAN_POINT('Ctrl Pts',(-23.6290105898186,13.1616327439453,
128.982551634326)) ;
#115600=CARTESIAN_POINT('Ctrl Pts',(-23.6739522585566,12.8906304372966,
129.080681338749)) ;
#115601=CARTESIAN_POINT('Ctrl Pts',(-23.7407279250101,12.6585325321797,
129.242687250476)) ;
#115602=CARTESIAN_POINT('Ctrl Pts',(-23.8252467089156,12.4808578746759,
129.456558276985)) ;
#115603=CARTESIAN_POINT('Ctrl Pts',(-23.9234212908845,12.369794968941,129.709975426016)) ;
#115604=CARTESIAN_POINT('Ctrl Pts',(-24.0266916219991,12.3353140243209,
129.978700782335)) ;
#115605=CARTESIAN_POINT('Ctrl Pts',(-24.1303332495694,12.3783402005982,
130.248268071055)) ;
#115606=CARTESIAN_POINT('Ctrl Pts',(-24.2265146825975,12.4961137906607,
130.496181048475)) ;
#115607=CARTESIAN_POINT('Ctrl Pts',(-24.3096595921357,12.6800956082709,
130.705970404282)) ;
#115608=CARTESIAN_POINT('Ctrl Pts',(-24.3745179631744,12.9180877152906,
130.862244767084)) ;
#115609=CARTESIAN_POINT('Ctrl Pts',(-24.4167847945233,13.1911275173993,
130.952669619891)) ;
#115610=CARTESIAN_POINT('Ctrl Pts',(-24.4345812423772,13.4815072415882,
130.971518185869)) ;
#115611=CARTESIAN_POINT('Ctrl Pts',(-24.4270213519574,13.7684314308885,
130.916204524826)) ;
#115612=CARTESIAN_POINT('Ctrl Pts',(-24.3956514842814,14.029076308477,130.791530690429)) ;
#115613=CARTESIAN_POINT('Ctrl Pts',(-24.343165506001,14.2473093926041,130.605025756878)) ;
#115614=CARTESIAN_POINT('Ctrl Pts',(-24.2745743047042,14.4057091519906,
130.371660986809)) ;
#115615=CARTESIAN_POINT('Ctrl Pts',(-24.1945925450092,14.4946178708306,
130.104760579953)) ;
#115616=CARTESIAN_POINT('Ctrl Pts',(-24.11071512251,14.5063975208026,129.826695894897)) ;
#115617=CARTESIAN_POINT('Ctrl Pts',(-24.0286060386776,14.4401278585609,
129.553540640394)) ;
#115618=CARTESIAN_POINT('Ctrl Pts',(-23.9562423178897,14.3020001323071,
129.309200756072)) ;
#115619=CARTESIAN_POINT('Ctrl Pts',(-23.8982704981956,14.100380875427,129.106698871819)) ;
#115620=CARTESIAN_POINT('Ctrl Pts',(-23.8601423404147,13.8504602239821,
128.962217821069)) ;
#115621=CARTESIAN_POINT('Ctrl Pts',(-23.8451537683981,13.5690360496352,
128.88522225926)) ;
#115622=CARTESIAN_POINT('Ctrl Pts',(-23.85536903869,13.277347744237,128.881881865911)) ;
#115623=CARTESIAN_POINT('Ctrl Pts',(-23.8903250024146,12.9978265767653,
128.951024979183)) ;
#115624=CARTESIAN_POINT('Ctrl Pts',(-23.9487275671782,12.747023860199,129.088449649182)) ;
#115625=CARTESIAN_POINT('Ctrl Pts',(-24.0267536508702,12.5453431667421,
129.283298823089)) ;
#115626=CARTESIAN_POINT('Ctrl Pts',(-24.1198629233628,12.4062333259034,
129.52213584094)) ;
#115627=CARTESIAN_POINT('Ctrl Pts',(-24.2215666079949,12.3400677949455,
129.786207600519)) ;
#115628=CARTESIAN_POINT('Ctrl Pts',(-24.3264846884265,12.3515722965719,
130.059403729799)) ;
#115629=CARTESIAN_POINT('Ctrl Pts',(-24.4261565993231,12.4396025465946,
130.317564726088)) ;
#115630=CARTESIAN_POINT('Ctrl Pts',(-24.515504520949,12.5983879462257,130.545404926639)) ;
#115631=CARTESIAN_POINT('Ctrl Pts',(-24.5881171815504,12.8155081778463,
130.724487254865)) ;
#115632=CARTESIAN_POINT('Ctrl Pts',(-24.6401896035301,13.0777480891852,
130.8433438272)) ;
#115633=CARTESIAN_POINT('Ctrl Pts',(-24.6679851185762,13.3640007134148,
130.891395810982)) ;
#115634=CARTESIAN_POINT('Ctrl Pts',(-24.6706717433523,13.6530970190172,
130.866255003353)) ;
#115635=CARTESIAN_POINT('Ctrl Pts',(-24.6486810155768,13.9274410550996,
130.768823051012)) ;
#115636=CARTESIAN_POINT('Ctrl Pts',(-24.6043588117149,14.1649405448642,
130.60624558075)) ;
#115637=CARTESIAN_POINT('Ctrl Pts',(-24.5413708101056,14.3499176915205,
130.389027795027)) ;
#115638=CARTESIAN_POINT('Ctrl Pts',(-24.4653494690363,14.4676736740884,
130.133852904625)) ;
#115639=CARTESIAN_POINT('Ctrl Pts',(-24.3825873013246,14.5109849198275,
129.859094894237)) ;
#115640=CARTESIAN_POINT('Ctrl Pts',(-24.2987925768636,14.4763368011369,
129.58106163939)) ;
#115641=CARTESIAN_POINT('Ctrl Pts',(-24.2217612201684,14.3664425274482,
129.322969701944)) ;
#115642=CARTESIAN_POINT('Ctrl Pts',(-24.1570057110458,14.1882602546085,
129.100578369949)) ;
#115643=CARTESIAN_POINT('Ctrl Pts',(-24.1105157071068,13.9563928712726,
128.931742068379)) ;
#115644=CARTESIAN_POINT('Ctrl Pts',(-24.0858458393616,13.6856075071528,
128.826527819527)) ;
#115645=CARTESIAN_POINT('Ctrl Pts',(-24.0856539585114,13.3967978155194,
128.792918629269)) ;
#115646=CARTESIAN_POINT('Ctrl Pts',(-24.1107926076059,13.1083772147109,
128.833125740032)) ;
#115647=CARTESIAN_POINT('Ctrl Pts',(-24.1600137825134,12.8436201216384,
128.943820657913)) ;
#115648=CARTESIAN_POINT('Ctrl Pts',(-24.2308058798189,12.6197329650473,
129.117423409396)) ;
#115649=CARTESIAN_POINT('Ctrl Pts',(-24.3182751718309,12.4541610182818,
129.339893353894)) ;
#115650=CARTESIAN_POINT('Ctrl Pts',(-24.4176896908462,12.3575181073951,
129.59708909666)) ;
#115651=CARTESIAN_POINT('Ctrl Pts',(-24.5213942641841,12.337407534574,129.86708474398)) ;
#115652=CARTESIAN_POINT('Ctrl Pts',(-24.6242611097352,12.3950240477661,
130.134369464736)) ;
#115653=CARTESIAN_POINT('Ctrl Pts',(-24.7182893080511,12.5255974682326,
130.376052536827)) ;
#115654=CARTESIAN_POINT('Ctrl Pts',(-24.7987860343519,12.7221236513144,
130.577891266987)) ;
#115655=CARTESIAN_POINT('Ctrl Pts',(-24.8592668458931,12.966643820031,130.721612719223)) ;
#115656=CARTESIAN_POINT('Ctrl Pts',(-24.8973477603996,13.2467842966359,
130.799514303858)) ;
#115657=CARTESIAN_POINT('Ctrl Pts',(-24.9101357439362,13.5364084867458,
130.803917200582)) ;
#115658=CARTESIAN_POINT('Ctrl Pts',(-24.8980433329888,13.819301352246,130.735470391269)) ;
#115659=CARTESIAN_POINT('Ctrl Pts',(-24.8624508729161,14.0737430594077,
130.598397208659)) ;
#115660=CARTESIAN_POINT('Ctrl Pts',(-24.8063650001413,14.2823383256047,
130.401314654759)) ;
#115661=CARTESIAN_POINT('Ctrl Pts',(-24.7352153152331,14.4280819786068,
130.160457808913)) ;
#115662=CARTESIAN_POINT('Ctrl Pts',(-24.654277110767,14.5027907188546,129.890917785084)) ;
#115663=CARTESIAN_POINT('Ctrl Pts',(-24.569599491767,14.4996009182714,129.610218523976)) ;
#115664=CARTESIAN_POINT('Ctrl Pts',(-24.4895659727805,14.4198435135005,
129.343494691889)) ;
#115665=CARTESIAN_POINT('Ctrl Pts',(-24.4190126879205,14.2682255575811,
129.104196361098)) ;
#115666=CARTESIAN_POINT('Ctrl Pts',(-24.364598178107,14.0566692320112,128.91218100257)) ;
#115667=CARTESIAN_POINT('Ctrl Pts',(-24.3305009683015,13.7984046917339,
128.779328284604)) ;
#115668=CARTESIAN_POINT('Ctrl Pts',(-24.3202768420663,13.5146255183712,
128.716401612773)) ;
#115669=CARTESIAN_POINT('Ctrl Pts',(-24.3351461344103,13.22379017507,128.726708255358)) ;
#115670=CARTESIAN_POINT('Ctrl Pts',(-24.3747056074861,12.9476430099182,
128.809207275973)) ;
#115671=CARTESIAN_POINT('Ctrl Pts',(-24.4373988447194,12.7041858709694,
128.959075140171)) ;
#115672=CARTESIAN_POINT('Ctrl Pts',(-24.5182754986541,12.5142908380612,
129.162405255088)) ;
#115673=CARTESIAN_POINT('Ctrl Pts',(-24.6137660742652,12.3877724329813,
129.408115006488)) ;
#115674=CARTESIAN_POINT('Ctrl Pts',(-24.7167971690515,12.3361912043238,
129.675956387308)) ;
#115675=CARTESIAN_POINT('Ctrl Pts',(-24.8208049085079,12.3624798224069,
129.946681899111)) ;
#115676=CARTESIAN_POINT('Ctrl Pts',(-24.9189695732058,12.4640688022784,
130.200435824458)) ;
#115677=CARTESIAN_POINT('Ctrl Pts',(-25.005956640633,12.6358046245907,130.421244636591)) ;
#115678=CARTESIAN_POINT('Ctrl Pts',(-25.0747012664645,12.862048858162,130.589103084132)) ;
#115679=CARTESIAN_POINT('Ctrl Pts',(-25.1223375525266,13.1294243703739,
130.69512008432)) ;
#115680=CARTESIAN_POINT('Ctrl Pts',(-25.1455445896858,13.419127554444,130.729642616116)) ;
#115681=CARTESIAN_POINT('Ctrl Pts',(-25.1435152363736,13.7060585256719,
130.690801967982)) ;
#115682=CARTESIAN_POINT('Ctrl Pts',(-25.1170308827865,13.9758635071568,
130.580144935401)) ;
#115683=CARTESIAN_POINT('Ctrl Pts',(-25.0688142460135,14.2044690811379,
130.40618368144)) ;
#115684=CARTESIAN_POINT('Ctrl Pts',(-25.003123247664,14.3772046466544,130.18118138791)) ;
#115685=CARTESIAN_POINT('Ctrl Pts',(-24.9252844700022,14.4817041640368,
129.920684773534)) ;
#115686=CARTESIAN_POINT('Ctrl Pts',(-24.8415989541778,14.5103977605507,
129.643097336818)) ;
#115687=CARTESIAN_POINT('Ctrl Pts',(-24.7589132492041,14.461387716176,129.368476107022)) ;
#115688=CARTESIAN_POINT('Ctrl Pts',(-24.6835796855055,14.3378670523305,
129.115253926662)) ;
#115689=CARTESIAN_POINT('Ctrl Pts',(-24.6219712562161,14.1487649480966,
128.902143850339)) ;
#115690=CARTESIAN_POINT('Ctrl Pts',(-24.5791815584349,13.9077124472436,
128.744012805924)) ;
#115691=CARTESIAN_POINT('Ctrl Pts',(-24.5590011432879,13.6318349091011,
128.651919455676)) ;
#115692=CARTESIAN_POINT('Ctrl Pts',(-24.5636129562954,13.3411961915081,
128.632272182411)) ;
#115693=CARTESIAN_POINT('Ctrl Pts',(-24.5933692421231,13.0563347009616,
128.686073174335)) ;
#115694=CARTESIAN_POINT('Ctrl Pts',(-24.6470060166101,12.7976622253545,
128.809603060301)) ;
#115695=CARTESIAN_POINT('Ctrl Pts',(-24.7208016129616,12.584625305209,128.992205539617)) ;
#115696=CARTESIAN_POINT('Ctrl Pts',(-24.8118536009071,12.429833286881,129.224781939929)) ;
#115697=CARTESIAN_POINT('Ctrl Pts',(-24.911545430168,12.3481748757021,129.483189757942)) ;
#115698=CARTESIAN_POINT('Ctrl Pts',(-25.0164125625319,12.3422836205948,
129.75626651559)) ;
#115699=CARTESIAN_POINT('Ctrl Pts',(-25.117816306108,12.414162317258,130.019416608038)) ;
#115700=CARTESIAN_POINT('Ctrl Pts',(-25.2100635855326,12.55849168118,130.255714929222)) ;
#115701=CARTESIAN_POINT('Ctrl Pts',(-25.2867433505999,12.7644624942609,
130.446624226534)) ;
#115702=CARTESIAN_POINT('Ctrl Pts',(-25.3433959651672,13.0174115077838,
130.579031809203)) ;
#115703=CARTESIAN_POINT('Ctrl Pts',(-25.3766991434267,13.2998964348547,
130.643172314106)) ;
#115704=CARTESIAN_POINT('Ctrl Pts',(-25.3849027762527,13.5908799629275,
130.634029729427)) ;
#115705=CARTESIAN_POINT('Ctrl Pts',(-25.3681244270798,13.8706960081611,
130.551809717868)) ;
#115706=CARTESIAN_POINT('Ctrl Pts',(-25.3281885696402,14.1180202656557,
130.401959719847)) ;
#115707=CARTESIAN_POINT('Ctrl Pts',(-25.2692654377525,14.3143765894564,
130.196866938718)) ;
#115708=CARTESIAN_POINT('Ctrl Pts',(-25.1954627990625,14.4481660809184,
129.948075722546)) ;
#115709=CARTESIAN_POINT('Ctrl Pts',(-25.1135963031033,14.5080838606745,
129.675906827394)) ;
#115710=CARTESIAN_POINT('Ctrl Pts',(-25.0294161558255,14.4905518531177,
129.396790506061)) ;
#115711=CARTESIAN_POINT('Ctrl Pts',(-24.9503166631056,14.3964092296967,
129.132598410075)) ;
#115712=CARTESIAN_POINT('Ctrl Pts',(-24.8824484698929,14.232304987228,128.901173407916)) ;
#115713=CARTESIAN_POINT('Ctrl Pts',(-24.831656485841,14.0113006854444,128.719789796304)) ;
#115714=CARTESIAN_POINT('Ctrl Pts',(-24.8018618709668,13.7469853282518,
128.599564702445)) ;
#115715=CARTESIAN_POINT('Ctrl Pts',(-24.7961937055128,13.4601451324146,
128.54991646717)) ;
#115716=CARTESIAN_POINT('Ctrl Pts',(-24.8160226315964,13.1687003200991,
128.574510511953)) ;
#115717=CARTESIAN_POINT('Ctrl Pts',(-24.859902739483,12.8989650919222,128.669805113981)) ;
#115718=CARTESIAN_POINT('Ctrl Pts',(-24.9266168659618,12.6635916504989,
128.831356633498)) ;
#115719=CARTESIAN_POINT('Ctrl Pts',(-25.0103639202873,12.485239800862,129.043133485935)) ;
#115720=CARTESIAN_POINT('Ctrl Pts',(-25.1082951885594,12.3719259500599,
129.295815313463)) ;
#115721=CARTESIAN_POINT('Ctrl Pts',(-25.2113378058678,12.3351771032852,
129.563924734244)) ;
#115722=CARTESIAN_POINT('Ctrl Pts',(-25.3153987713946,12.3762351050997,
129.834608633564)) ;
#115723=CARTESIAN_POINT('Ctrl Pts',(-25.4113691303234,12.4911992435135,
130.082089209234)) ;
#115724=CARTESIAN_POINT('Ctrl Pts',(-25.4955318190917,12.6745749260732,
130.29463045715)) ;
#115725=CARTESIAN_POINT('Ctrl Pts',(-25.560704508805,12.9105841176317,130.451940846143)) ;
#115726=CARTESIAN_POINT('Ctrl Pts',(-25.6037591586016,13.1834575472762,
130.544589177351)) ;
#115727=CARTESIAN_POINT('Ctrl Pts',(-25.6221540731369,13.4728172007292,
130.565280977399)) ;
#115728=CARTESIAN_POINT('Ctrl Pts',(-25.6154890774634,13.7593252111675,
130.512691578256)) ;
#115729=CARTESIAN_POINT('Ctrl Pts',(-25.5845017414514,14.0229111380707,
130.388875573167)) ;
#115730=CARTESIAN_POINT('Ctrl Pts',(-25.5329646548234,14.2409568530166,
130.205405121793)) ;
#115731=CARTESIAN_POINT('Ctrl Pts',(-25.4643492210366,14.4024702596202,
129.971739445436)) ;
#115732=CARTESIAN_POINT('Ctrl Pts',(-25.3848249850593,14.4930252918819,
129.706290426526)) ;
#115733=CARTESIAN_POINT('Ctrl Pts',(-25.3009346998094,14.5071138077779,
129.428162516891)) ;
#115734=CARTESIAN_POINT('Ctrl Pts',(-25.2189936227422,14.4434722304718,
129.155638517111)) ;
#115735=CARTESIAN_POINT('Ctrl Pts',(-25.1460018098747,14.3072991508372,
128.909365963459)) ;
#115736=CARTESIAN_POINT('Ctrl Pts',(-25.0872927957611,14.1061281755834,
128.704547183538)) ;
#115737=CARTESIAN_POINT('Ctrl Pts',(-25.0487858755379,13.8584458365122,
128.559117426276)) ;
#115738=CARTESIAN_POINT('Ctrl Pts',(-25.0330304801592,13.5782527615593,
128.479942965013)) ;
#115739=CARTESIAN_POINT('Ctrl Pts',(-25.0424542208566,13.2862405830432,
128.474252693863)) ;
#115740=CARTESIAN_POINT('Ctrl Pts',(-25.0767412324267,13.0054673407222,
128.541371132674)) ;
#115741=CARTESIAN_POINT('Ctrl Pts',(-25.1348051000407,12.7527978446706,
128.67768872235)) ;
#115742=CARTESIAN_POINT('Ctrl Pts',(-25.2119030388808,12.5507722085017,
128.870018404504)) ;
#115743=CARTESIAN_POINT('Ctrl Pts',(-25.3047050008252,12.4092693590586,
129.107923829017)) ;
#115744=CARTESIAN_POINT('Ctrl Pts',(-25.406443595545,12.3409406073707,129.37203421041)) ;
#115745=CARTESIAN_POINT('Ctrl Pts',(-25.5110390200225,12.3499819194409,
129.644402105975)) ;
#115746=CARTESIAN_POINT('Ctrl Pts',(-25.6114390222507,12.4363532158425,
129.904516274518)) ;
#115747=CARTESIAN_POINT('Ctrl Pts',(-25.7007310200177,12.5925663631045,
130.132357144071)) ;
#115748=CARTESIAN_POINT('Ctrl Pts',(-25.7740950725506,12.8085170384963,
130.313559518156)) ;
#115749=CARTESIAN_POINT('Ctrl Pts',(-25.8267351162025,13.0694866152918,
130.434112913458)) ;
#115750=CARTESIAN_POINT('Ctrl Pts',(-25.8553312907165,13.3550371201656,
130.48453070364)) ;
#115751=CARTESIAN_POINT('Ctrl Pts',(-25.8586885366147,13.6462143005165,
130.461126760816)) ;
#115752=CARTESIAN_POINT('Ctrl Pts',(-25.837444412916,13.9195287631536,130.366084906634)) ;
#115753=CARTESIAN_POINT('Ctrl Pts',(-25.7937488394422,14.1586150899391,
130.205310735235)) ;
#115754=CARTESIAN_POINT('Ctrl Pts',(-25.7313611315605,14.3449689837057,
129.989913913384)) ;
#115755=CARTESIAN_POINT('Ctrl Pts',(-25.6556964572195,14.465239738532,129.735783996914)) ;
#115756=CARTESIAN_POINT('Ctrl Pts',(-25.5723964230934,14.5107689866746,
129.459195604095)) ;
#115757=CARTESIAN_POINT('Ctrl Pts',(-25.4893174125801,14.4787461978325,
129.183580822489)) ;
#115758=CARTESIAN_POINT('Ctrl Pts',(-25.4113051186338,14.3700644324197,
128.922314853824)) ;
#115759=CARTESIAN_POINT('Ctrl Pts',(-25.3465909420863,14.1946408166751,
128.700275185896)) ;
#115760=CARTESIAN_POINT('Ctrl Pts',(-25.299369271165,13.963907732595,128.529234819729)) ;
#115761=CARTESIAN_POINT('Ctrl Pts',(-25.2739922523,13.6940409321305,128.421969041019)) ;
#115762=CARTESIAN_POINT('Ctrl Pts',(-25.2731534451911,13.4043243937501,
128.386332734542)) ;
#115763=CARTESIAN_POINT('Ctrl Pts',(-25.2973628386527,13.1175424358185,
128.424062655725)) ;
#115764=CARTESIAN_POINT('Ctrl Pts',(-25.3462006392316,12.8501254079525,
128.533419495547)) ;
#115765=CARTESIAN_POINT('Ctrl Pts',(-25.4160919098287,12.6260375389968,
128.704569775621)) ;
#115766=CARTESIAN_POINT('Ctrl Pts',(-25.5032418915579,12.4581545252769,
128.926046604269)) ;
#115767=CARTESIAN_POINT('Ctrl Pts',(-25.6021785519615,12.3594525497003,
129.181922681907)) ;
#115768=CARTESIAN_POINT('Ctrl Pts',(-25.7061730224389,12.3367944069397,
129.452652747223)) ;
#115769=CARTESIAN_POINT('Ctrl Pts',(-25.8094492173163,12.3925085409291,
129.721047874811)) ;
#115770=CARTESIAN_POINT('Ctrl Pts',(-25.9037624326914,12.5213898755188,
129.963557213451)) ;
#115771=CARTESIAN_POINT('Ctrl Pts',(-25.9844805178092,12.7155724021421,
130.166157205425)) ;
#115772=CARTESIAN_POINT('Ctrl Pts',(-26.0456691934443,12.9595220676015,
130.311865673155)) ;
#115773=CARTESIAN_POINT('Ctrl Pts',(-26.0842093042236,13.2367788940881,
130.391368626224)) ;
#115774=CARTESIAN_POINT('Ctrl Pts',(-26.0979544525776,13.5277643625836,
130.39839898417)) ;
#115775=CARTESIAN_POINT('Ctrl Pts',(-26.0864824258526,13.8120453761231,
130.331665108325)) ;
#115776=CARTESIAN_POINT('Ctrl Pts',(-26.05142082645,14.0676654739834,130.196112404188)) ;
#115777=CARTESIAN_POINT('Ctrl Pts',(-25.9959721958356,14.2771419928287,
130.000979869832)) ;
#115778=CARTESIAN_POINT('Ctrl Pts',(-25.9251922030581,14.425031880978,129.761195796767)) ;
#115779=CARTESIAN_POINT('Ctrl Pts',(-25.8440763649555,14.5017260060049,
129.490996412094)) ;
#115780=CARTESIAN_POINT('Ctrl Pts',(-25.7603662435499,14.5010099059246,
129.213512691512)) ;
#115781=CARTESIAN_POINT('Ctrl Pts',(-25.6794136560246,14.4231233705973,
128.943812915352)) ;
#115782=CARTESIAN_POINT('Ctrl Pts',(-25.6086694413268,14.2735700722065,
128.704038175328)) ;
#115783=CARTESIAN_POINT('Ctrl Pts',(-25.5536232001884,14.0631260843178,
128.510103402269)) ;
#115784=CARTESIAN_POINT('Ctrl Pts',(-25.5190005221295,13.8068513237717,
128.37583898455)) ;
#115785=CARTESIAN_POINT('Ctrl Pts',(-25.5079988886962,13.5229068768556,
128.310556815572)) ;
#115786=CARTESIAN_POINT('Ctrl Pts',(-25.522136912891,13.2323185296325,128.31877011903)) ;
#115787=CARTESIAN_POINT('Ctrl Pts',(-25.5609778387885,12.955462422634,128.399168054502)) ;
#115788=CARTESIAN_POINT('Ctrl Pts',(-25.622981897995,12.7108337306576,128.547046303102)) ;
#115789=CARTESIAN_POINT('Ctrl Pts',(-25.7035387876594,12.5189036902296,
128.749376462235)) ;
#115790=CARTESIAN_POINT('Ctrl Pts',(-25.7983973245378,12.3906586207823,
128.993347141695)) ;
#115791=CARTESIAN_POINT('Ctrl Pts',(-25.9014394205249,12.3366531336248,
129.261165642822)) ;
#115792=CARTESIAN_POINT('Ctrl Pts',(-26.0053503635526,12.360297772879,129.531671267842)) ;
#115793=CARTESIAN_POINT('Ctrl Pts',(-26.1046179703446,12.4609988515391,
129.788341417843)) ;
#115794=CARTESIAN_POINT('Ctrl Pts',(-26.1910706407531,12.6291274638668,
130.0079564874)) ;
#115795=CARTESIAN_POINT('Ctrl Pts',(-26.2610067862353,12.8555169755094,
130.179031109569)) ;
#115796=CARTESIAN_POINT('Ctrl Pts',(-26.3090567054831,13.1215885522129,
130.286335393292)) ;
#115797=CARTESIAN_POINT('Ctrl Pts',(-26.3329796835872,13.4096083938423,
130.323096945283)) ;
#115798=CARTESIAN_POINT('Ctrl Pts',(-26.3317340747676,13.698212942693,130.286391172774)) ;
#115799=CARTESIAN_POINT('Ctrl Pts',(-26.3058007346478,13.9691452295141,
130.177299627734)) ;
#115800=CARTESIAN_POINT('Ctrl Pts',(-26.2583066398341,14.1982918407705,
130.005562251346)) ;
#115801=CARTESIAN_POINT('Ctrl Pts',(-26.1931751350795,14.3728095621698,
129.782233989023)) ;
#115802=CARTESIAN_POINT('Ctrl Pts',(-26.1155255616385,14.479662285758,129.522250222093)) ;
#115803=CARTESIAN_POINT('Ctrl Pts',(-26.0318486038747,14.5107460879228,
129.244664158376)) ;
#115804=CARTESIAN_POINT('Ctrl Pts',(-25.9488165487381,14.4636147982726,
128.968932999966)) ;
#115805=CARTESIAN_POINT('Ctrl Pts',(-25.8735146658894,14.3427084720644,
128.715956195703)) ;
#115806=CARTESIAN_POINT('Ctrl Pts',(-25.811125852612,14.1545214106307,128.500410033898)) ;
#115807=CARTESIAN_POINT('Ctrl Pts',(-25.767859635489,13.914665784431,128.340908123874)) ;
#115808=CARTESIAN_POINT('Ctrl Pts',(-25.7470531048229,13.6405172708492,
128.247102795506)) ;
#115809=CARTESIAN_POINT('Ctrl Pts',(-25.7508957888745,13.3501102818962,
128.225215226321)) ;
#115810=CARTESIAN_POINT('Ctrl Pts',(-25.7797927372613,13.0651843315454,
128.276561420719)) ;
#115811=CARTESIAN_POINT('Ctrl Pts',(-25.8330708547357,12.80388772374,128.398847085602)) ;
#115812=CARTESIAN_POINT('Ctrl Pts',(-25.9063371941856,12.5899465270377,
128.579947959411)) ;
#115813=CARTESIAN_POINT('Ctrl Pts',(-25.9963126660368,12.4339563210189,
128.809607064104)) ;
#115814=CARTESIAN_POINT('Ctrl Pts',(-26.0966203558645,12.3491846989202,
129.069534053189)) ;
#115815=CARTESIAN_POINT('Ctrl Pts',(-26.2015343109458,12.3415474281895,
129.342731765695)) ;
#115816=CARTESIAN_POINT('Ctrl Pts',(-26.3027211617629,12.4110292201394,
129.60537279447)) ;
#115817=CARTESIAN_POINT('Ctrl Pts',(-26.3953588574291,12.5533605448057,
129.842803792173)) ;
#115818=CARTESIAN_POINT('Ctrl Pts',(-26.4724658228993,12.7574391512257,
130.035002583383)) ;
#115819=CARTESIAN_POINT('Ctrl Pts',(-26.5299060950814,13.0095817126533,
130.169659341123)) ;
#115820=CARTESIAN_POINT('Ctrl Pts',(-26.5639504532064,13.2928226801242,
130.235818361087)) ;
#115821=CARTESIAN_POINT('Ctrl Pts',(-26.5727935985865,13.5820119966617,
130.228755567199)) ;
#115822=CARTESIAN_POINT('Ctrl Pts',(-26.5567072828717,13.8633229249982,
130.148453208055)) ;
#115823=CARTESIAN_POINT('Ctrl Pts',(-26.5174678494182,14.1112602779132,
130.000718041267)) ;
#115824=CARTESIAN_POINT('Ctrl Pts',(-26.4589493371831,14.3095521754014,
129.79675027408)) ;
#115825=CARTESIAN_POINT('Ctrl Pts',(-26.3857504408749,14.4451057235358,
129.549834730436)) ;
#115826=CARTESIAN_POINT('Ctrl Pts',(-26.3033581527554,14.5076745769451,
129.275854508276)) ;
#115827=CARTESIAN_POINT('Ctrl Pts',(-26.2193621817028,14.4918702514085,
128.997365975633)) ;
#115828=CARTESIAN_POINT('Ctrl Pts',(-26.1403227598029,14.4001695900989,
128.733462893607)) ;
#115829=CARTESIAN_POINT('Ctrl Pts',(-26.0720785017029,14.238339270588,128.500982256028)) ;
#115830=CARTESIAN_POINT('Ctrl Pts',(-26.0205445494064,14.0178457541506,
128.317291271494)) ;
#115831=CARTESIAN_POINT('Ctrl Pts',(-25.9901309545097,13.7549024704848,
128.195319458128)) ;
#115832=CARTESIAN_POINT('Ctrl Pts',(-25.9838907425677,13.4669383655623,
128.143823454231)) ;
#115833=CARTESIAN_POINT('Ctrl Pts',(-26.002625472959,13.1792878389568,128.165694781332)) ;
#115834=CARTESIAN_POINT('Ctrl Pts',(-26.0462578585361,12.9054935275296,
128.259864888277)) ;
#115835=CARTESIAN_POINT('Ctrl Pts',(-26.1117838862911,12.6708451835732,
128.418257412013)) ;
#115836=CARTESIAN_POINT('Ctrl Pts',(-26.1958394673662,12.4890109361581,
128.630614971608)) ;
#115837=CARTESIAN_POINT('Ctrl Pts',(-26.292450313642,12.3747427440592,128.879802823841)) ;
#115838=CARTESIAN_POINT('Ctrl Pts',(-26.3961466629634,12.335118127865,129.149563628382)) ;
#115839=CARTESIAN_POINT('Ctrl Pts',(-26.4997927945682,12.3735357257966,
129.41921706946)) ;
#115840=CARTESIAN_POINT('Ctrl Pts',(-26.5970562066531,12.4876827050984,
129.670119063763)) ;
#115841=CARTESIAN_POINT('Ctrl Pts',(-26.6809623236233,12.668143871092,129.882175659137)) ;
#115842=CARTESIAN_POINT('Ctrl Pts',(-26.7469567383412,12.9033827829949,
130.041784506141)) ;
#115843=CARTESIAN_POINT('Ctrl Pts',(-26.7905248136644,13.1743601664502,
130.136070712378)) ;
#115844=CARTESIAN_POINT('Ctrl Pts',(-26.8098089341939,13.4644840041335,
130.159245371207)) ;
#115845=CARTESIAN_POINT('Ctrl Pts',(-26.8037407483827,13.7518155739233,
130.108342116625)) ;
#115846=CARTESIAN_POINT('Ctrl Pts',(-26.7736744947239,14.0147480425275,
129.987433665233)) ;
#115847=CARTESIAN_POINT('Ctrl Pts',(-26.7224117937105,14.2359322469135,
129.804543108639)) ;
#115848=CARTESIAN_POINT('Ctrl Pts',(-26.6540459121311,14.3990328419962,
129.571575856472)) ;
#115849=CARTESIAN_POINT('Ctrl Pts',(-26.5752101350165,14.4913721211862,
129.308326055989)) ;
#115850=CARTESIAN_POINT('Ctrl Pts',(-26.4908765753451,14.5077030613306,
129.028705274742)) ;
#115851=CARTESIAN_POINT('Ctrl Pts',(-26.4092296365473,14.4466726935246,
128.757236988289)) ;
#115852=CARTESIAN_POINT('Ctrl Pts',(-26.3352722351391,14.3110620977678,
128.507833953029)) ;
#115853=CARTESIAN_POINT('Ctrl Pts',(-26.2766889458892,14.1132680684101,
128.303711145387)) ;
#115854=CARTESIAN_POINT('Ctrl Pts',(-26.2372639174626,13.8656264960883,
128.15541845975)) ;
#115855=CARTESIAN_POINT('Ctrl Pts',(-26.2209130537975,13.5853317318957,
128.074439710367)) ;
#115856=CARTESIAN_POINT('Ctrl Pts',(-26.2296856924358,13.2939513094312,
128.066914197785)) ;
#115857=CARTESIAN_POINT('Ctrl Pts',(-26.2631798636915,13.0136081090702,
128.131828211089)) ;
#115858=CARTESIAN_POINT('Ctrl Pts',(-26.3203316415523,12.7604084565328,
128.265584239078)) ;
#115859=CARTESIAN_POINT('Ctrl Pts',(-26.397246993967,12.5556140537718,128.457218817256)) ;
#115860=CARTESIAN_POINT('Ctrl Pts',(-26.4898764488098,12.412162783817,128.694571316763)) ;
#115861=CARTESIAN_POINT('Ctrl Pts',(-26.5911530122536,12.3419224833159,
128.957426665658)) ;
#115862=CARTESIAN_POINT('Ctrl Pts',(-26.6956543409951,12.3485705631489,
129.229554057824)) ;
#115863=CARTESIAN_POINT('Ctrl Pts',(-26.7962358912617,12.4325162173742,
129.490217635024)) ;
#115864=CARTESIAN_POINT('Ctrl Pts',(-26.8862177213639,12.5872706018155,
129.719968083883)) ;
#115865=CARTESIAN_POINT('Ctrl Pts',(-26.9600298412944,12.8016741765326,
129.902501376654)) ;
#115866=CARTESIAN_POINT('Ctrl Pts',(-27.0132363984096,13.0608926757193,
130.024793668328)) ;
#115867=CARTESIAN_POINT('Ctrl Pts',(-27.0426146311277,13.3463627388947,
130.077448217005)) ;
#115868=CARTESIAN_POINT('Ctrl Pts',(-27.0467658686963,13.6367413735624,
130.056476137218)) ;
#115869=CARTESIAN_POINT('Ctrl Pts',(-27.0262045189193,13.912123441329,129.96328026669)) ;
#115870=CARTESIAN_POINT('Ctrl Pts',(-26.9829610646689,14.1528033236638,
129.803766513539)) ;
#115871=CARTESIAN_POINT('Ctrl Pts',(-26.9212047054132,14.3402810134416,
129.590308052972)) ;
#115872=CARTESIAN_POINT('Ctrl Pts',(-26.8459513519056,14.4626257099404,
129.33741374041)) ;
#115873=CARTESIAN_POINT('Ctrl Pts',(-26.7626484303445,14.5106364099982,
129.060769517447)) ;
#115874=CARTESIAN_POINT('Ctrl Pts',(-26.6793325739832,14.4805445966973,
128.784392296914)) ;
#115875=CARTESIAN_POINT('Ctrl Pts',(-26.6015120722546,14.3748126779467,
128.523896403084)) ;
#115876=CARTESIAN_POINT('Ctrl Pts',(-26.5360012381168,14.2005693776624,
128.299367371948)) ;
#115877=CARTESIAN_POINT('Ctrl Pts',(-26.4882466006821,13.9714224956824,
128.126808943075)) ;
#115878=CARTESIAN_POINT('Ctrl Pts',(-26.4621696395529,13.7016038456452,
128.017397936684)) ;
#115879=CARTESIAN_POINT('Ctrl Pts',(-26.4605573044593,13.4137877720204,
127.979694610522)) ;
#115880=CARTESIAN_POINT('Ctrl Pts',(-26.4842037814474,13.1249621059971,
128.015572519599)) ;
#115881=CARTESIAN_POINT('Ctrl Pts',(-26.5319266616535,12.858759801946,128.121953585796)) ;
#115882=CARTESIAN_POINT('Ctrl Pts',(-26.601763218089,12.6311849064932,128.292661018411)) ;
#115883=CARTESIAN_POINT('Ctrl Pts',(-26.6883690358658,12.4620614418067,
128.512623702752)) ;
#115884=CARTESIAN_POINT('Ctrl Pts',(-26.7871596601743,12.3611529243014,
128.768034196029)) ;
#115885=CARTESIAN_POINT('Ctrl Pts',(-26.8908594338048,12.336402737043,129.037980194775)) ;
#115886=CARTESIAN_POINT('Ctrl Pts',(-26.9942677499415,12.3896954767389,
129.30676634427)) ;
#115887=CARTESIAN_POINT('Ctrl Pts',(-27.0891228503658,12.5169545730866,
129.550776904504)) ;
#115888=CARTESIAN_POINT('Ctrl Pts',(-27.170110122641,12.7090014500136,129.754247695197)) ;
#115889=CARTESIAN_POINT('Ctrl Pts',(-27.2319803579197,12.9518209129291,
129.901923479105)) ;
#115890=CARTESIAN_POINT('Ctrl Pts',(-27.2712167263555,13.2283911259786,
129.983462395853)) ;
#115891=CARTESIAN_POINT('Ctrl Pts',(-27.2856848450787,13.5192444476926,
129.992606198651)) ;
#115892=CARTESIAN_POINT('Ctrl Pts',(-27.2749998341,13.8035929406365,129.928231036212)) ;
#115893=CARTESIAN_POINT('Ctrl Pts',(-27.2405107086992,14.0607675161601,
129.794281704174)) ;
#115894=CARTESIAN_POINT('Ctrl Pts',(-27.1859404561386,14.2709776513911,
129.601886944103)) ;
#115895=CARTESIAN_POINT('Ctrl Pts',(-27.1150473623168,14.4220258151157,
129.36152624086)) ;
#115896=CARTESIAN_POINT('Ctrl Pts',(-27.0343785010806,14.5004899933202,
129.09274938976)) ;
#115897=CARTESIAN_POINT('Ctrl Pts',(-26.950535069012,14.5020985766214,128.814815907977)) ;
#115898=CARTESIAN_POINT('Ctrl Pts',(-26.8695870479016,14.426667623352,128.545218407416)) ;
#115899=CARTESIAN_POINT('Ctrl Pts',(-26.798211588555,14.2786158189735,128.303482030973)) ;
#115900=CARTESIAN_POINT('Ctrl Pts',(-26.7426992360049,14.0697690186074,
128.108208750919)) ;
#115901=CARTESIAN_POINT('Ctrl Pts',(-26.7074412852036,13.8142976320865,
127.972057291302)) ;
#115902=CARTESIAN_POINT('Ctrl Pts',(-26.6957645215905,13.5318062075926,
127.904912693824)) ;
#115903=CARTESIAN_POINT('Ctrl Pts',(-26.7091353370237,13.2403761874523,
127.91080130822)) ;
#115904=CARTESIAN_POINT('Ctrl Pts',(-26.74755505738,12.9618561593774,127.989837070354)) ;
#115905=CARTESIAN_POINT('Ctrl Pts',(-26.8086943560285,12.7173263730279,
128.135355225743)) ;
#115906=CARTESIAN_POINT('Ctrl Pts',(-26.8888831517,12.5233446886838,128.33655295725)) ;
#115907=CARTESIAN_POINT('Ctrl Pts',(-26.9835011120047,12.3931312315505,
128.579802503126)) ;
#115908=CARTESIAN_POINT('Ctrl Pts',(-27.0865721816442,12.337075246258,128.847656402371)) ;
#115909=CARTESIAN_POINT('Ctrl Pts',(-27.1901303578273,12.3586764449227,
129.117256451724)) ;
#115910=CARTESIAN_POINT('Ctrl Pts',(-27.2892091804132,12.4563696314589,
129.373537084527)) ;
#115911=CARTESIAN_POINT('Ctrl Pts',(-27.3766437558911,12.6234424170359,
129.595825398964)) ;
#115912=CARTESIAN_POINT('Ctrl Pts',(-27.447072154312,12.8484690314232,129.768349176844)) ;
#115913=CARTESIAN_POINT('Ctrl Pts',(-27.4958104255805,13.1134860607375,
129.877675494575)) ;
#115914=CARTESIAN_POINT('Ctrl Pts',(-27.5204851717528,13.402425050447,129.916492772369)) ;
#115915=CARTESIAN_POINT('Ctrl Pts',(-27.5198611034755,13.6901681944769,
129.881727019293)) ;
#115916=CARTESIAN_POINT('Ctrl Pts',(-27.4947206170695,13.9614083380647,
129.775024765156)) ;
#115917=CARTESIAN_POINT('Ctrl Pts',(-27.4477408524357,14.1924050674132,
129.604730002262)) ;
#115918=CARTESIAN_POINT('Ctrl Pts',(-27.3829916295066,14.3688010159201,
129.382496516221)) ;
#115919=CARTESIAN_POINT('Ctrl Pts',(-27.305567395489,14.4776662097744,129.123157647789)) ;
#115920=CARTESIAN_POINT('Ctrl Pts',(-27.2222300887403,14.5108828480259,
128.84666452346)) ;
#115921=CARTESIAN_POINT('Ctrl Pts',(-27.1390665957671,14.4662997711349,
128.570551673275)) ;
#115922=CARTESIAN_POINT('Ctrl Pts',(-27.063203525044,14.3468724358185,128.315811999268)) ;
#115923=CARTESIAN_POINT('Ctrl Pts',(-27.000726116674,14.161614932188,128.10021376119)) ;
#115924=CARTESIAN_POINT('Ctrl Pts',(-26.9566598775861,13.9230022753498,
127.938326275104)) ;
#115925=CARTESIAN_POINT('Ctrl Pts',(-26.9350826150652,13.6485314062169,
127.842142219284)) ;
#115926=CARTESIAN_POINT('Ctrl Pts',(-26.9382141999983,13.3583011743042,
127.818182839235)) ;
#115927=CARTESIAN_POINT('Ctrl Pts',(-26.9665177873497,13.072504270402,127.867737400507)) ;
#115928=CARTESIAN_POINT('Ctrl Pts',(-27.0188173523961,12.8117566735177,
127.987365016217)) ;
#115929=CARTESIAN_POINT('Ctrl Pts',(-27.0915996802834,12.5955171582893,
128.166977325295)) ;
#115930=CARTESIAN_POINT('Ctrl Pts',(-27.1817271815024,12.4369580568928,
128.396898077135)) ;
#115931=CARTESIAN_POINT('Ctrl Pts',(-27.2813708056134,12.3507869630092,
128.655042348106)) ;
#115932=CARTESIAN_POINT('Ctrl Pts',(-27.3857827418417,12.3404899643528,
128.926923079581)) ;
#115933=CARTESIAN_POINT('Ctrl Pts',(-27.4876541467364,12.4078494476239,
129.191403822402)) ;
#115934=CARTESIAN_POINT('Ctrl Pts',(-27.5807089481865,12.5483871977687,
129.430029656426)) ;
#115935=CARTESIAN_POINT('Ctrl Pts',(-27.6584612758746,12.7513533086917,
129.624045981255)) ;
#115936=CARTESIAN_POINT('Ctrl Pts',(-27.7163134902441,13.001941318222,129.759978308328)) ;
#115937=CARTESIAN_POINT('Ctrl Pts',(-27.7510006841768,13.2828868274063,
129.828206089058)) ;
#115938=CARTESIAN_POINT('Ctrl Pts',(-27.7607078220157,13.5743278631276,
129.823412590067)) ;
#115939=CARTESIAN_POINT('Ctrl Pts',(-27.7452570064132,13.8554587804339,
129.745052642731)) ;
#115940=CARTESIAN_POINT('Ctrl Pts',(-27.7068857846591,14.103739100914,129.599981463497)) ;
#115941=CARTESIAN_POINT('Ctrl Pts',(-27.6487231943859,14.3046990175591,
129.396931127844)) ;
#115942=CARTESIAN_POINT('Ctrl Pts',(-27.5755356695319,14.4424188711516,
129.149922663509)) ;
#115943=CARTESIAN_POINT('Ctrl Pts',(-27.4939933548379,14.5067209234145,
128.878704097542)) ;
#115944=CARTESIAN_POINT('Ctrl Pts',(-27.4097527588653,14.4936392684735,
128.599416389571)) ;
#115945=CARTESIAN_POINT('Ctrl Pts',(-27.3303082230943,14.404006740505,128.334269093954)) ;
#115946=CARTESIAN_POINT('Ctrl Pts',(-27.2614819305869,14.2433942656814,
128.099980444704)) ;
#115947=CARTESIAN_POINT('Ctrl Pts',(-27.2096136486434,14.0252993056693,
127.915456300396)) ;
#115948=CARTESIAN_POINT('Ctrl Pts',(-27.178469556164,13.7626963119846,127.791262873367)) ;
#115949=CARTESIAN_POINT('Ctrl Pts',(-27.1714738989522,13.4766513624265,
127.737736625053)) ;
#115950=CARTESIAN_POINT('Ctrl Pts',(-27.1895561727833,13.1866966293381,
127.757460183878)) ;
#115951=CARTESIAN_POINT('Ctrl Pts',(-27.2326135994264,12.9123106961637,
127.849963433579)) ;
#115952=CARTESIAN_POINT('Ctrl Pts',(-27.2974441217088,12.6769408805555,
128.006390666055)) ;
#115953=CARTESIAN_POINT('Ctrl Pts',(-27.3808130116155,12.4935889535621,
128.216818650803)) ;
#115954=CARTESIAN_POINT('Ctrl Pts',(-27.4776575476475,12.3766908568814,
128.466511171481)) ;
#115955=CARTESIAN_POINT('Ctrl Pts',(-27.5810443505466,12.3352383862452,
128.735442117728)) ;
#115956=CARTESIAN_POINT('Ctrl Pts',(-27.6845420847214,12.3713736006973,
129.004732437811)) ;
#115957=CARTESIAN_POINT('Ctrl Pts',(-27.7818596677854,12.4827590293817,
129.255891826048)) ;
#115958=CARTESIAN_POINT('Ctrl Pts',(-27.8667979944307,12.6627224306716,
129.47073002161)) ;
#115959=CARTESIAN_POINT('Ctrl Pts',(-27.9330076414952,12.8955397849013,
129.631137908056)) ;
#115960=CARTESIAN_POINT('Ctrl Pts',(-27.9774352268445,13.1663558963296,
129.72784335586)) ;
#115961=CARTESIAN_POINT('Ctrl Pts',(-27.9973849513202,13.4563321062043,
129.752958193208)) ;
#115962=CARTESIAN_POINT('Ctrl Pts',(-27.9920646322741,13.74354179735,129.704297361198)) ;
#115963=CARTESIAN_POINT('Ctrl Pts',(-27.9626165416411,14.007863745204,129.585142101985)) ;
#115964=CARTESIAN_POINT('Ctrl Pts',(-27.9119828992553,14.2299792391956,
129.404152786278)) ;
#115965=CARTESIAN_POINT('Ctrl Pts',(-27.844287943155,14.3948659481182,129.173238937185)) ;
#115966=CARTESIAN_POINT('Ctrl Pts',(-27.7651604606475,14.4898740802148,
128.908913740689)) ;
#115967=CARTESIAN_POINT('Ctrl Pts',(-27.681397890891,14.5084149248409,128.631178035807)) ;
#115968=CARTESIAN_POINT('Ctrl Pts',(-27.5990872491488,14.4492459338564,
128.357554758999)) ;
#115969=CARTESIAN_POINT('Ctrl Pts',(-27.5253256223266,14.316609488643,128.108970615685)) ;
#115970=CARTESIAN_POINT('Ctrl Pts',(-27.4659033295799,14.1198900556279,
127.9022461303)) ;
#115971=CARTESIAN_POINT('Ctrl Pts',(-27.42591393932,13.8734079349303,127.752317228327)) ;
#115972=CARTESIAN_POINT('Ctrl Pts',(-27.408865491139,13.5947694158123,127.669409669264)) ;
#115973=CARTESIAN_POINT('Ctrl Pts',(-27.4167455300075,13.3033325180628,
127.659268253717)) ;
#115974=CARTESIAN_POINT('Ctrl Pts',(-27.4497732461264,13.0207084742087,
127.722612022269)) ;
#115975=CARTESIAN_POINT('Ctrl Pts',(-27.5060414733426,12.767628690545,127.853947272495)) ;
#115976=CARTESIAN_POINT('Ctrl Pts',(-27.5826500146593,12.5604751539345,
128.044576460787)) ;
#115977=CARTESIAN_POINT('Ctrl Pts',(-27.6748867687302,12.4152916729436,
128.280805111389)) ;
#115978=CARTESIAN_POINT('Ctrl Pts',(-27.7760048062591,12.3428120631862,
128.543188432493)) ;
#115979=CARTESIAN_POINT('Ctrl Pts',(-27.880802690774,12.3473797413046,128.816094258677)) ;
#115980=CARTESIAN_POINT('Ctrl Pts',(-27.9814814316689,12.4294695368143,
129.077065134186)) ;
#115981=CARTESIAN_POINT('Ctrl Pts',(-28.0714598999934,12.5816148375682,
129.306949475753)) ;
#115982=CARTESIAN_POINT('Ctrl Pts',(-28.1460628162166,12.7949907280796,
129.491697351825)) ;
#115983=CARTESIAN_POINT('Ctrl Pts',(-28.1999915303535,13.054101177031,129.616001192498)) ;
#115984=CARTESIAN_POINT('Ctrl Pts',(-28.2299138854955,13.3386274126212,
129.670307692816)) ;
#115985=CARTESIAN_POINT('Ctrl Pts',(-28.2347775216737,13.6281884734652,
129.651524250556)) ;
#115986=CARTESIAN_POINT('Ctrl Pts',(-28.2149512862949,13.9042249218154,
129.560485972219)) ;
#115987=CARTESIAN_POINT('Ctrl Pts',(-28.1723564864184,14.1463903457502,
129.402858889307)) ;
#115988=CARTESIAN_POINT('Ctrl Pts',(-28.1106708276455,14.3364819716926,
129.189416939951)) ;
#115989=CARTESIAN_POINT('Ctrl Pts',(-28.0360880693673,14.4598817702337,
128.938660433378)) ;
#115990=CARTESIAN_POINT('Ctrl Pts',(-27.953057765994,14.5104486170863,128.662863635966)) ;
#115991=CARTESIAN_POINT('Ctrl Pts',(-27.8692045369708,14.4822486369166,
128.384729130641)) ;
#115992=CARTESIAN_POINT('Ctrl Pts',(-27.791608538637,14.3791733041028,128.125092916574)) ;
#115993=CARTESIAN_POINT('Ctrl Pts',(-27.7253583208721,14.2063740303146,
127.898282623416)) ;
#115994=CARTESIAN_POINT('Ctrl Pts',(-27.6770395587882,13.9777765864427,
127.723995413382)) ;
#115995=CARTESIAN_POINT('Ctrl Pts',(-27.6504229397667,13.7109259499415,
127.613260324166)) ;
#115996=CARTESIAN_POINT('Ctrl Pts',(-27.6480583043497,13.4211174151953,
127.573090826099)) ;
#115997=CARTESIAN_POINT('Ctrl Pts',(-27.6709154004622,13.1336909339448,
127.606862509643)) ;
#115998=CARTESIAN_POINT('Ctrl Pts',(-27.7180057890291,12.8658812639418,
127.711313356748)) ;
#115999=CARTESIAN_POINT('Ctrl Pts',(-27.7873482366324,12.6367690190525,
127.880557040248)) ;
#116000=CARTESIAN_POINT('Ctrl Pts',(-27.8736342999947,12.4658337897599,
128.099554794345)) ;
#116001=CARTESIAN_POINT('Ctrl Pts',(-27.9718311891268,12.3631245211514,
128.353345809671)) ;
#116002=CARTESIAN_POINT('Ctrl Pts',(-28.0756846325717,12.3360466241608,
128.623667434511)) ;
#116003=CARTESIAN_POINT('Ctrl Pts',(-28.1788526517052,12.3868688002356,
128.891874367728)) ;
#116004=CARTESIAN_POINT('Ctrl Pts',(-28.2741388501772,12.5119418325269,
129.137115030646)) ;
#116005=CARTESIAN_POINT('Ctrl Pts',(-28.3556708751438,12.7021783709845,
129.342171425122)) ;
#116006=CARTESIAN_POINT('Ctrl Pts',(-28.4184699311589,12.9449353770794,
129.492398354652)) ;
#116007=CARTESIAN_POINT('Ctrl Pts',(-28.4583084084869,13.2214383784226,
129.575638041553)) ;
#116008=CARTESIAN_POINT('Ctrl Pts',(-28.4734122859081,13.5108147708277,
129.586797648768)) ;
#116009=CARTESIAN_POINT('Ctrl Pts',(-28.4633457731125,13.7968084175674,
129.524085701258)) ;
#116010=CARTESIAN_POINT('Ctrl Pts',(-28.4296187997626,14.0536576083437,
129.392533959943)) ;
#116011=CARTESIAN_POINT('Ctrl Pts',(-28.3754911658076,14.2659120564335,
129.201360310375)) ;
#116012=CARTESIAN_POINT('Ctrl Pts',(-28.3050821824441,14.4185012516542,
128.962475031458)) ;
#116013=CARTESIAN_POINT('Ctrl Pts',(-28.2247264730961,14.4992712221482,
128.694649965742)) ;
#116014=CARTESIAN_POINT('Ctrl Pts',(-28.1405276912772,14.5031360116066,
128.415538484686)) ;
#116015=CARTESIAN_POINT('Ctrl Pts',(-28.059513753469,14.4296202074177,128.145783486771)) ;
#116016=CARTESIAN_POINT('Ctrl Pts',(-27.9880766403289,14.2844131247839,
127.904026806799)) ;
#116017=CARTESIAN_POINT('Ctrl Pts',(-27.9318057397691,14.0764755685082,
127.706412345186)) ;
#116018=CARTESIAN_POINT('Ctrl Pts',(-27.8959845576815,13.8227947339683,
127.568706785711)) ;
#116019=CARTESIAN_POINT('Ctrl Pts',(-27.8835201350609,13.5398702989391,
127.499142873583)) ;
#116020=CARTESIAN_POINT('Ctrl Pts',(-27.8962033555758,13.2487717783427,
127.50306914783)) ;
#116021=CARTESIAN_POINT('Ctrl Pts',(-27.9337544855272,12.9703362151756,
127.579661290793)) ;
#116022=CARTESIAN_POINT('Ctrl Pts',(-27.9942820451289,12.7241092781338,
127.723348072863)) ;
#116023=CARTESIAN_POINT('Ctrl Pts',(-28.0741961867263,12.5279171433205,
127.923656462501)) ;
#116024=CARTESIAN_POINT('Ctrl Pts',(-28.1684346295129,12.3959938665945,
128.165822555878)) ;
#116025=CARTESIAN_POINT('Ctrl Pts',(-28.2708930006534,12.3376260980812,
128.432033363079)) ;
#116026=CARTESIAN_POINT('Ctrl Pts',(-28.3752372703154,12.3570497794023,
128.703694565037)) ;
#116027=CARTESIAN_POINT('Ctrl Pts',(-28.474218780803,12.4525559733436,128.959799081295)) ;
#116028=CARTESIAN_POINT('Ctrl Pts',(-28.5620645646479,12.6176036105847,
129.183295489253)) ;
#116029=CARTESIAN_POINT('Ctrl Pts',(-28.6330705369593,12.8410947019102,
129.357514549927)) ;
#116030=CARTESIAN_POINT('Ctrl Pts',(-28.6825047729054,13.1055203518464,
129.468831178845)) ;
#116031=CARTESIAN_POINT('Ctrl Pts',(-28.7078791143123,13.3928980327512,
129.509831198009)) ;
#116032=CARTESIAN_POINT('Ctrl Pts',(-28.7080000857972,13.6824543649216,
129.477058491295)) ;
#116033=CARTESIAN_POINT('Ctrl Pts',(-28.6836462060832,13.9532692757644,
129.372812982897)) ;
#116034=CARTESIAN_POINT('Ctrl Pts',(-28.637210824604,14.1862511235797,129.204032177995)) ;
#116035=CARTESIAN_POINT('Ctrl Pts',(-28.5729983268859,14.3643962082537,
128.983404490918)) ;
#116036=CARTESIAN_POINT('Ctrl Pts',(-28.4953888433576,14.4759024807437,
128.723329064892)) ;
#116037=CARTESIAN_POINT('Ctrl Pts',(-28.4124155755593,14.5109062464403,
128.448017144722)) ;
#116038=CARTESIAN_POINT('Ctrl Pts',(-28.3292183756258,14.4687351628052,
128.171836440681)) ;
#116039=CARTESIAN_POINT('Ctrl Pts',(-28.2530232843449,14.351243796897,127.916105712843)) ;
#116040=CARTESIAN_POINT('Ctrl Pts',(-28.19012029587,14.1681343550178,127.699312985571)) ;
#116041=CARTESIAN_POINT('Ctrl Pts',(-28.1452447510838,13.9291093552066,
127.534840373785)) ;
#116042=CARTESIAN_POINT('Ctrl Pts',(-28.123183101824,13.6572015399983,127.437471920795)) ;
#116043=CARTESIAN_POINT('Ctrl Pts',(-28.1255814706017,13.3659146668707,
127.411223933066)) ;
#116044=CARTESIAN_POINT('Ctrl Pts',(-28.1531210645832,13.0809591455927,
127.458689441797)) ;
#116045=CARTESIAN_POINT('Ctrl Pts',(-28.2046620168687,12.8188859308948,
127.576087509683)) ;
#116046=CARTESIAN_POINT('Ctrl Pts',(-28.277541817743,12.5999510440463,127.755745614815)) ;
#116047=CARTESIAN_POINT('Ctrl Pts',(-28.3661476402695,12.4414984825018,
127.981641389139)) ;
#116048=CARTESIAN_POINT('Ctrl Pts',(-28.4661327647063,12.3520343108791,
128.240572616874)) ;
#116049=CARTESIAN_POINT('Ctrl Pts',(-28.5708059444941,12.3398054622105,
128.513131254719)) ;
#116050=CARTESIAN_POINT('Ctrl Pts',(-28.6724777538977,12.4047865271677,
128.777144444355)) ;
#116051=CARTESIAN_POINT('Ctrl Pts',(-28.7659001413954,12.5431933869583,
129.016844456436)) ;
#116052=CARTESIAN_POINT('Ctrl Pts',(-28.8442058560459,12.7444965603529,
129.212472342267)) ;
#116053=CARTESIAN_POINT('Ctrl Pts',(-28.9027924661007,12.9945025224571,
129.350476244749)) ;
#116054=CARTESIAN_POINT('Ctrl Pts',(-28.9381575691283,13.2745329094811,
129.420727068277)) ;
#116055=CARTESIAN_POINT('Ctrl Pts',(-28.9485234575593,13.5670626370277,
129.417726861736)) ;
#116056=CARTESIAN_POINT('Ctrl Pts',(-28.933960447473,13.8462370772247,129.342272430857)) ;
#116057=CARTESIAN_POINT('Ctrl Pts',(-28.8959789907869,14.0979241250953,
129.198057982517)) ;
#116058=CARTESIAN_POINT('Ctrl Pts',(-28.838332105253,14.2997383418867,128.996585250886)) ;
#116059=CARTESIAN_POINT('Ctrl Pts',(-28.7657725957652,14.4393312193764,
128.7515156292)) ;
#116060=CARTESIAN_POINT('Ctrl Pts',(-28.6837573347161,14.5060643569228,
128.478659684657)) ;
#116061=CARTESIAN_POINT('Ctrl Pts',(-28.6001080114847,14.4951758782706,
128.201352828122)) ;
#116062=CARTESIAN_POINT('Ctrl Pts',(-28.5200653111137,14.4072623281432,
127.934287968157)) ;
#116063=CARTESIAN_POINT('Ctrl Pts',(-28.4511978062007,14.2495039694875,
127.70007480226)) ;
#116064=CARTESIAN_POINT('Ctrl Pts',(-28.3983753819167,14.0308221258824,
127.512458103752)) ;
#116065=CARTESIAN_POINT('Ctrl Pts',(-28.3669487720982,13.7719100664948,
127.38779922883)) ;
#116066=CARTESIAN_POINT('Ctrl Pts',(-28.3590881011533,13.4847456450531,
127.331550611793)) ;
#116067=CARTESIAN_POINT('Ctrl Pts',(-28.3764285791946,13.1955425031336,
127.349219523261)) ;
#116068=CARTESIAN_POINT('Ctrl Pts',(-28.4187558984065,12.9200552968874,
127.439556443674)) ;
#116069=CARTESIAN_POINT('Ctrl Pts',(-28.4830536897966,12.6831184385928,
127.594396583248)) ;
#116070=CARTESIAN_POINT('Ctrl Pts',(-28.5659931747335,12.4980281206389,
127.803559634745)) ;
#116071=CARTESIAN_POINT('Ctrl Pts',(-28.6623364928729,12.3791543430107,
128.051854714151)) ;
#116072=CARTESIAN_POINT('Ctrl Pts',(-28.7659162180442,12.3353503717386,
128.321248640665)) ;
#116073=CARTESIAN_POINT('Ctrl Pts',(-28.869394759317,12.3691099621928,128.590526992868)) ;
#116074=CARTESIAN_POINT('Ctrl Pts',(-28.9675502196224,12.4795856785055,
128.843913403417)) ;
#116075=CARTESIAN_POINT('Ctrl Pts',(-29.0518027446978,12.6553361009926,
129.057199931773)) ;
#116076=CARTESIAN_POINT('Ctrl Pts',(-29.1192464163454,12.8882259217544,
129.220954123798)) ;
#116077=CARTESIAN_POINT('Ctrl Pts',(-29.1642643498932,13.1581921393272,
129.319406321897)) ;
#116078=CARTESIAN_POINT('Ctrl Pts',(-29.1849604313943,13.4482190387101,
129.34666282445)) ;
#116079=CARTESIAN_POINT('Ctrl Pts',(-29.1803518618151,13.7352663202425,
129.300143313471)) ;
#116080=CARTESIAN_POINT('Ctrl Pts',(-29.1516048942262,14.0004787425337,
129.183043232165)) ;
#116081=CARTESIAN_POINT('Ctrl Pts',(-29.1015568370635,14.2242401467777,
129.003757674716)) ;
#116082=CARTESIAN_POINT('Ctrl Pts',(-29.0339430184054,14.391486003047,128.772934980117)) ;
#116083=CARTESIAN_POINT('Ctrl Pts',(-28.955492652777,14.4880341837757,128.510778479589)) ;
#116084=CARTESIAN_POINT('Ctrl Pts',(-28.8714600975796,14.5089767222778,
128.232121389573)) ;
#116085=CARTESIAN_POINT('Ctrl Pts',(-28.7892529362311,14.4520807364783,
127.958902917957)) ;
#116086=CARTESIAN_POINT('Ctrl Pts',(-28.7150523793816,14.3213934969356,
127.708991446956)) ;
#116087=CARTESIAN_POINT('Ctrl Pts',(-28.6551735760367,14.126427628205,127.500952233118)) ;
#116088=CARTESIAN_POINT('Ctrl Pts',(-28.6144873955634,13.8807880817665,
127.348935930026)) ;
#116089=CARTESIAN_POINT('Ctrl Pts',(-28.5968038371001,13.6022566506269,
127.264117077343)) ;
#116090=CARTESIAN_POINT('Ctrl Pts',(-28.6039330637587,13.3123739575692,
127.251951536785)) ;
#116091=CARTESIAN_POINT('Ctrl Pts',(-28.6361660227389,13.0290004002489,
127.312956120869)) ;
#116092=CARTESIAN_POINT('Ctrl Pts',(-28.6919510174919,12.7741270713226,
127.442792020744)) ;
#116093=CARTESIAN_POINT('Ctrl Pts',(-28.7679989254335,12.5657352250487,
127.631815876347)) ;
#116094=CARTESIAN_POINT('Ctrl Pts',(-28.8594997341221,12.4188762117679,
127.866013266875)) ;
#116095=CARTESIAN_POINT('Ctrl Pts',(-28.9608147014607,12.3438128452305,
128.128841957193)) ;
#116096=CARTESIAN_POINT('Ctrl Pts',(-29.0652267516056,12.3461025205116,
128.400746493264)) ;
#116097=CARTESIAN_POINT('Ctrl Pts',(-29.1661640470906,12.4255735874937,
128.662467769584)) ;
#116098=CARTESIAN_POINT('Ctrl Pts',(-29.2569746802431,12.5765456735502,
128.894620530997)) ;
#116099=CARTESIAN_POINT('Ctrl Pts',(-29.3318567873601,12.7879286592572,
129.080274286269)) ;
#116100=CARTESIAN_POINT('Ctrl Pts',(-29.3863322538626,13.0448054046113,
129.206302436344)) ;
#116101=CARTESIAN_POINT('Ctrl Pts',(-29.4171885363179,13.329756321322,129.26322288733)) ;
#116102=CARTESIAN_POINT('Ctrl Pts',(-29.4227776954555,13.6201107178654,
129.246484513251)) ;
#116103=CARTESIAN_POINT('Ctrl Pts',(-29.4036112081965,13.8967554382586,
129.157379684264)) ;
#116104=CARTESIAN_POINT('Ctrl Pts',(-29.3617661068054,14.1394983367384,
129.002038511481)) ;
#116105=CARTESIAN_POINT('Ctrl Pts',(-29.3006432267773,14.3315001569242,
128.790247960104)) ;
#116106=CARTESIAN_POINT('Ctrl Pts',(-29.2260808954585,14.4575222943013,
128.539420298087)) ;
#116107=CARTESIAN_POINT('Ctrl Pts',(-29.1430912249785,14.5099977938908,
128.263711456409)) ;
#116108=CARTESIAN_POINT('Ctrl Pts',(-29.0596283023754,14.4843800867397,
127.986903750172)) ;
#116109=CARTESIAN_POINT('Ctrl Pts',(-28.9813399566608,14.3828781461486,
127.725057189875)) ;
#116110=CARTESIAN_POINT('Ctrl Pts',(-28.9150542416882,14.212816168216,127.498335145429)) ;
#116111=CARTESIAN_POINT('Ctrl Pts',(-28.8659433323491,13.9854781681749,
127.321666885816)) ;
#116112=CARTESIAN_POINT('Ctrl Pts',(-28.8385949971052,13.7179644909653,
127.2086184725)) ;
#116113=CARTESIAN_POINT('Ctrl Pts',(-28.835583635112,13.4301920376034,127.166758116441)) ;
#116114=CARTESIAN_POINT('Ctrl Pts',(-28.8575789748189,13.1421055633853,
127.197981715462)) ;
#116115=CARTESIAN_POINT('Ctrl Pts',(-28.9045188244626,12.87150128464,127.301728733917)) ;
#116116=CARTESIAN_POINT('Ctrl Pts',(-28.9725684665303,12.6436097991943,
127.46756519262)) ;
#116117=CARTESIAN_POINT('Ctrl Pts',(-29.0586604842472,12.4698498437503,
127.68586545448)) ;
#116118=CARTESIAN_POINT('Ctrl Pts',(-29.1565931939368,12.3651221856613,
127.938894371706)) ;
#116119=CARTESIAN_POINT('Ctrl Pts',(-29.2604850351592,12.335692224637,128.209290972507)) ;
#116120=CARTESIAN_POINT('Ctrl Pts',(-29.3638355952977,12.3844432071478,
128.478011145159)) ;
#116121=CARTESIAN_POINT('Ctrl Pts',(-29.4592358664342,12.5072147901112,
128.723652752499)) ;
#116122=CARTESIAN_POINT('Ctrl Pts',(-29.5413221888135,12.6957550150873,
128.930308953615)) ;
#116123=CARTESIAN_POINT('Ctrl Pts',(-29.6047036187767,12.9372999479051,
129.082233550744)) ;
#116124=CARTESIAN_POINT('Ctrl Pts',(-29.6452182047899,13.2121499543988,
129.167553115)) ;
#116125=CARTESIAN_POINT('Ctrl Pts',(-29.6611042764023,13.5032465104466,
129.180780924663)) ;
#116126=CARTESIAN_POINT('Ctrl Pts',(-29.6518819161121,13.7871080328991,
129.120848156331)) ;
#116127=CARTESIAN_POINT('Ctrl Pts',(-29.6187108954398,14.0469104745439,
128.990694231868)) ;
#116128=CARTESIAN_POINT('Ctrl Pts',(-29.5650955851099,14.2605649124229,
128.801033137001)) ;
#116129=CARTESIAN_POINT('Ctrl Pts',(-29.494870755953,14.4153649488043,128.562594916595)) ;
#116130=CARTESIAN_POINT('Ctrl Pts',(-29.4150387131859,14.4978582783663,
128.296438099207)) ;
#116131=CARTESIAN_POINT('Ctrl Pts',(-29.3308499416307,14.5041773990225,
128.017349602118)) ;
#116132=CARTESIAN_POINT('Ctrl Pts',(-29.2496148451093,14.4329779197685,
127.746941843894)) ;
#116133=CARTESIAN_POINT('Ctrl Pts',(-29.1775262666222,14.2890422314917,
127.503142142852)) ;
#116134=CARTESIAN_POINT('Ctrl Pts',(-29.1208969337368,14.082779433517,127.304531079944)) ;
#116135=CARTESIAN_POINT('Ctrl Pts',(-29.0845225826136,13.8309337098099,
127.165299579887)) ;
#116136=CARTESIAN_POINT('Ctrl Pts',(-29.0713186329842,13.5483120187831,
127.093542785031)) ;
#116137=CARTESIAN_POINT('Ctrl Pts',(-29.083229857648,13.2574777531019,127.095253063998)) ;
#116138=CARTESIAN_POINT('Ctrl Pts',(-29.1201441678816,12.9779697529959,
127.169929814834)) ;
#116139=CARTESIAN_POINT('Ctrl Pts',(-29.1798340071233,12.7311580251373,
127.311268080156)) ;
#116140=CARTESIAN_POINT('Ctrl Pts',(-29.259615046753,12.5323980592304,127.511032300878)) ;
#116141=CARTESIAN_POINT('Ctrl Pts',(-29.3531954363121,12.3989897288854,
127.751398360947)) ;
#116142=CARTESIAN_POINT('Ctrl Pts',(-29.4557047728638,12.3382487603058,
128.017686516644)) ;
#116143=CARTESIAN_POINT('Ctrl Pts',(-29.5597398015999,12.3552058083452,
128.288561847953)) ;
#116144=CARTESIAN_POINT('Ctrl Pts',(-29.6596151268484,12.4490680703867,
128.547063275398)) ;
#116145=CARTESIAN_POINT('Ctrl Pts',(-29.747823539621,12.612854304799,128.771597225379)) ;
#116146=CARTESIAN_POINT('Ctrl Pts',(-29.8189230473542,12.8333918295054,
128.946308444558)) ;
#116147=CARTESIAN_POINT('Ctrl Pts',(-29.8692193933531,13.0975419155814,
129.060046052025)) ;
#116148=CARTESIAN_POINT('Ctrl Pts',(-29.8952825556904,13.3843701567211,
129.103082744144)) ;
#116149=CARTESIAN_POINT('Ctrl Pts',(-29.8961296754756,13.6749248626015,
129.072344167559)) ;
#116150=CARTESIAN_POINT('Ctrl Pts',(-29.872352875635,13.9463602578246,128.969789222471)) ;
#116151=CARTESIAN_POINT('Ctrl Pts',(-29.8267467901644,14.1798324379302,
128.803574285622)) ;
#116152=CARTESIAN_POINT('Ctrl Pts',(-29.762567848699,14.3606302769089,128.582842462436)) ;
#116153=CARTESIAN_POINT('Ctrl Pts',(-29.6859295100925,14.4733618864566,
128.325903972762)) ;
#116154=CARTESIAN_POINT('Ctrl Pts',(-29.6022723165312,14.5110756600993,
128.048275924638)) ;
#116155=CARTESIAN_POINT('Ctrl Pts',(-29.5194444158079,14.4709889009811,
127.773361424165)) ;
#116156=CARTESIAN_POINT('Ctrl Pts',(-29.4427850873383,14.3556941984043,
127.516218240476)) ;
#116157=CARTESIAN_POINT('Ctrl Pts',(-29.379260435332,14.1731666486328,127.297467610204)) ;
#116158=CARTESIAN_POINT('Ctrl Pts',(-29.3342254132114,13.9378584167298,
127.132862710005)) ;
#116159=CARTESIAN_POINT('Ctrl Pts',(-29.3112446912435,13.6656355311939,
127.03265253494)) ;
#116160=CARTESIAN_POINT('Ctrl Pts',(-29.3129312287784,13.3744563081115,
127.004322113587)) ;
#116161=CARTESIAN_POINT('Ctrl Pts',(-29.3398177129572,13.0885611803192,
127.049815834232)) ;
#116162=CARTESIAN_POINT('Ctrl Pts',(-29.3906009924672,12.8263306498725,
127.165093753781)) ;
#116163=CARTESIAN_POINT('Ctrl Pts',(-29.4625594349018,12.6063807769631,
127.342179164998)) ;
#116164=CARTESIAN_POINT('Ctrl Pts',(-29.5513814104012,12.4447492933123,
127.568465791526)) ;
#116165=CARTESIAN_POINT('Ctrl Pts',(-29.6511504516607,12.3535025882306,
127.826777567947)) ;
#116166=CARTESIAN_POINT('Ctrl Pts',(-29.7556083087904,12.3391045054194,
128.098761532225)) ;
#116167=CARTESIAN_POINT('Ctrl Pts',(-29.8574615889439,12.4018104241151,
128.363303066571)) ;
#116168=CARTESIAN_POINT('Ctrl Pts',(-29.9515240336887,12.5389586489687,
128.604752086664)) ;
#116169=CARTESIAN_POINT('Ctrl Pts',(-30.0298895040687,12.7377764458565,
128.800721216607)) ;
#116170=CARTESIAN_POINT('Ctrl Pts',(-30.0891318078393,12.9863019722805,
128.940662639121)) ;
#116171=CARTESIAN_POINT('Ctrl Pts',(-30.1252471064463,13.2660338630659,
129.013066477495)) ;
#116172=CARTESIAN_POINT('Ctrl Pts',(-30.1363860269831,13.5582232268191,
129.012365283493)) ;
#116173=CARTESIAN_POINT('Ctrl Pts',(-30.1224573425596,13.8387404070693,
128.9386660175)) ;
#116174=CARTESIAN_POINT('Ctrl Pts',(-30.0853429984546,14.0904925183414,
128.797147021732)) ;
#116175=CARTESIAN_POINT('Ctrl Pts',(-30.0277590711992,14.2955136011611,
128.595595560232)) ;
#116176=CARTESIAN_POINT('Ctrl Pts',(-29.9558778598522,14.4360006812449,
128.352686763533)) ;
#116177=CARTESIAN_POINT('Ctrl Pts',(-29.8742567679805,14.5051702931602,
128.081056456965)) ;
#116178=CARTESIAN_POINT('Ctrl Pts',(-29.7902969630137,14.4966323764384,
127.802731519334)) ;
#116179=CARTESIAN_POINT('Ctrl Pts',(-29.7100123387406,14.4108291399258,
127.534953213959)) ;
#116180=CARTESIAN_POINT('Ctrl Pts',(-29.6407380446541,14.2547209501546,
127.299525468516)) ;
#116181=CARTESIAN_POINT('Ctrl Pts',(-29.5875888674703,14.0388606089928,
127.111132269111)) ;
#116182=CARTESIAN_POINT('Ctrl Pts',(-29.5552494813085,13.779405578044,126.983595808789)) ;
#116183=CARTESIAN_POINT('Ctrl Pts',(-29.5467692399988,13.4926641580088,
126.925547219345)) ;
#116184=CARTESIAN_POINT('Ctrl Pts',(-29.5633816541989,13.2038302112353,
126.941144586643)) ;
#116185=CARTESIAN_POINT('Ctrl Pts',(-29.6048714410533,12.9280759931688,
127.02910382322)) ;
#116186=CARTESIAN_POINT('Ctrl Pts',(-29.6688506403303,12.6887447492448,
127.182864366148)) ;
#116187=CARTESIAN_POINT('Ctrl Pts',(-29.7513587249347,12.5022966343227,
127.39078364992)) ;
#116188=CARTESIAN_POINT('Ctrl Pts',(-29.8469802454942,12.381763978882,127.637108683278)) ;
#116189=CARTESIAN_POINT('Ctrl Pts',(-29.9508020024135,12.3354318114705,
127.907094928409)) ;
#116190=CARTESIAN_POINT('Ctrl Pts',(-30.0541803012317,12.3672035513488,
128.176131637916)) ;
#116191=CARTESIAN_POINT('Ctrl Pts',(-30.1521106585629,12.474426481286,128.429055203006)) ;
#116192=CARTESIAN_POINT('Ctrl Pts',(-30.2377865470727,12.6503068829769,
128.646124078682)) ;
#116193=CARTESIAN_POINT('Ctrl Pts',(-30.3053907898611,12.8812481424524,
128.810483543534)) ;
#116194=CARTESIAN_POINT('Ctrl Pts',(-30.3510328505262,13.1494231082653,
128.910858646302)) ;
#116195=CARTESIAN_POINT('Ctrl Pts',(-30.3725424728725,13.4405328283774,
128.94033906329)) ;
#116196=CARTESIAN_POINT('Ctrl Pts',(-30.3685945252647,13.7272524095848,
128.895825068985)) ;
#116197=CARTESIAN_POINT('Ctrl Pts',(-30.3405359677795,13.9933197786215,
128.780743464257)) ;
#116198=CARTESIAN_POINT('Ctrl Pts',(-30.2910888155488,14.2183989061991,
128.603235194175)) ;
#116199=CARTESIAN_POINT('Ctrl Pts',(-30.2238484293931,14.3876287517767,
128.373477627282)) ;
#116200=CARTESIAN_POINT('Ctrl Pts',(-30.1457515284424,14.4861870970875,
128.112398717919)) ;
#116201=CARTESIAN_POINT('Ctrl Pts',(-30.0617136501863,14.5095212297327,
127.833700802789)) ;
#116202=CARTESIAN_POINT('Ctrl Pts',(-29.9792786676799,14.4547287275128,
127.559780909732)) ;
#116203=CARTESIAN_POINT('Ctrl Pts',(-29.9048009680584,14.3261105544631,
127.309079981945)) ;
#116204=CARTESIAN_POINT('Ctrl Pts',(-29.844419395189,14.1327425032557,127.099559452458)) ;
#116205=CARTESIAN_POINT('Ctrl Pts',(-29.803152525388,13.8885306001009,126.945876263857)) ;
#116206=CARTESIAN_POINT('Ctrl Pts',(-29.7847767393562,13.6107524410049,
126.859040355574)) ;
#116207=CARTESIAN_POINT('Ctrl Pts',(-29.7910854802672,13.3210542583331,
126.844495484992)) ;
#116208=CARTESIAN_POINT('Ctrl Pts',(-29.8229753868191,13.0351251235983,
126.904244014759)) ;
#116209=CARTESIAN_POINT('Ctrl Pts',(-29.8776744286432,12.7816150209491,
127.031216029816)) ;
#116210=CARTESIAN_POINT('Ctrl Pts',(-29.9534311716552,12.5706518061014,
127.219253692065)) ;
#116211=CARTESIAN_POINT('Ctrl Pts',(-30.0445412838822,12.422091900903,127.452333377032)) ;
#116212=CARTESIAN_POINT('Ctrl Pts',(-30.1457887502779,12.3448083833829,
127.714923612566)) ;
#116213=CARTESIAN_POINT('Ctrl Pts',(-30.250148655895,12.3450375607664,127.986693881587)) ;
#116214=CARTESIAN_POINT('Ctrl Pts',(-30.3511170822601,12.4222140372622,
128.248559607977)) ;
#116215=CARTESIAN_POINT('Ctrl Pts',(-30.4423550067095,12.5713072693593,
128.481942746401)) ;
#116216=CARTESIAN_POINT('Ctrl Pts',(-30.5177968325665,12.7812068465324,
128.669220610782)) ;
#116217=CARTESIAN_POINT('Ctrl Pts',(-30.5730322088188,13.0378486801572,
128.797371634622)) ;
#116218=CARTESIAN_POINT('Ctrl Pts',(-30.6044543099339,13.3220972424203,
128.855977004469)) ;
#116219=CARTESIAN_POINT('Ctrl Pts',(-30.6107589621473,13.6116477161832,
128.841431739069)) ;
#116220=CARTESIAN_POINT('Ctrl Pts',(-30.5922328646922,13.8896343949454,
128.754117840507)) ;
#116221=CARTESIAN_POINT('Ctrl Pts',(-30.5510661396947,14.1329048293709,
128.60084368254)) ;
#116222=CARTESIAN_POINT('Ctrl Pts',(-30.4905361238725,14.3266157424045,
128.390815616408)) ;
#116223=CARTESIAN_POINT('Ctrl Pts',(-30.4160368539188,14.4550271923226,
128.140061981301)) ;
#116224=CARTESIAN_POINT('Ctrl Pts',(-30.333450058965,14.5094869156272,127.865640071397)) ;
#116225=CARTESIAN_POINT('Ctrl Pts',(-30.2498814405861,14.4863255111229,
127.588507289986)) ;
#116226=CARTESIAN_POINT('Ctrl Pts',(-30.1712461824057,14.3868080890416,
127.325605825376)) ;
#116227=CARTESIAN_POINT('Ctrl Pts',(-30.1044933380963,14.2186053771164,
127.097513189475)) ;
#116228=CARTESIAN_POINT('Ctrl Pts',(-30.0547280039428,13.9916146831158,
126.918804037804)) ;
#116229=CARTESIAN_POINT('Ctrl Pts',(-30.0268955041398,13.727139474133,126.804607454992)) ;
#116230=CARTESIAN_POINT('Ctrl Pts',(-30.0231159202939,13.437362164295,126.760227532608)) ;
#116231=CARTESIAN_POINT('Ctrl Pts',(-30.0443922432487,13.1504054531947,
126.789513820971)) ;
#116232=CARTESIAN_POINT('Ctrl Pts',(-30.0906616171445,12.8786465021209,
126.89126693415)) ;
#116233=CARTESIAN_POINT('Ctrl Pts',(-30.157970236125,12.6500332814425,127.055027994723)) ;
#116234=CARTESIAN_POINT('Ctrl Pts',(-30.2434337782595,12.4743183897028,
127.271533917434)) ;
#116235=CARTESIAN_POINT('Ctrl Pts',(-30.3417585829433,12.3668547922141,
127.525488336301)) ;
#116236=CARTESIAN_POINT('Ctrl Pts',(-30.4450821005495,12.335562941567,127.79438563983)) ;
#116237=CARTESIAN_POINT('Ctrl Pts',(-30.5484944936694,12.3817108072099,
128.063306891139)) ;
#116238=CARTESIAN_POINT('Ctrl Pts',(-30.6445980415539,12.502839824897,128.310875860644)) ;
#116239=CARTESIAN_POINT('Ctrl Pts',(-30.7271978616452,12.690351441453,128.518969835721)) ;
#116240=CARTESIAN_POINT('Ctrl Pts',(-30.7907079505213,12.9285059391321,
128.671549365572)) ;
#116241=CARTESIAN_POINT('Ctrl Pts',(-30.832295267727,13.2046731907038,128.75974213921)) ;
#116242=CARTESIAN_POINT('Ctrl Pts',(-30.8487758407748,13.4951333113011,
128.774772845728)) ;
#116243=CARTESIAN_POINT('Ctrl Pts',(-30.8402346447153,13.779501210584,128.716814376005)) ;
#116244=CARTESIAN_POINT('Ctrl Pts',(-30.8078637040687,14.0394108332529,
128.589125311067)) ;
#116245=CARTESIAN_POINT('Ctrl Pts',(-30.7546552751125,14.2552141196343,
128.400557285253)) ;
#116246=CARTESIAN_POINT('Ctrl Pts',(-30.6851696086428,14.4112842226695,
128.164437543065)) ;
#116247=CARTESIAN_POINT('Ctrl Pts',(-30.6053419982904,14.49663037618,127.89819080895)) ;
#116248=CARTESIAN_POINT('Ctrl Pts',(-30.520751800545,14.5049768783044,127.617767628039)) ;
#116249=CARTESIAN_POINT('Ctrl Pts',(-30.4397470692586,14.4360835729073,
127.348190225217)) ;
#116250=CARTESIAN_POINT('Ctrl Pts',(-30.3673932451776,14.2946513922982,
127.103676961857)) ;
#116251=CARTESIAN_POINT('Ctrl Pts',(-30.3101336108046,14.0899140100411,
126.903186984993)) ;
#116252=CARTESIAN_POINT('Ctrl Pts',(-30.2730059348416,13.8386917046902,
126.761684342598)) ;
#116253=CARTESIAN_POINT('Ctrl Pts',(-30.2591454609719,13.5555692125345,
126.687892009024)) ;
#116254=CARTESIAN_POINT('Ctrl Pts',(-30.2703044262027,13.2663901180779,
126.687596604313)) ;
#116255=CARTESIAN_POINT('Ctrl Pts',(-30.3064563015578,12.9858847333076,
126.760012223785)) ;
#116256=CARTESIAN_POINT('Ctrl Pts',(-30.3656808780386,12.7375102459871,
126.899927974495)) ;
#116257=CARTESIAN_POINT('Ctrl Pts',(-30.4446592433479,12.5376376287816,
127.097461701573)) ;
#116258=CARTESIAN_POINT('Ctrl Pts',(-30.5383897496922,12.4015826977934,
127.338092518212)) ;
#116259=CARTESIAN_POINT('Ctrl Pts',(-30.6402554773558,12.3390360902595,
127.602664560348)) ;
#116260=CARTESIAN_POINT('Ctrl Pts',(-30.7445603425615,12.353575403094,127.874253187337)) ;
#116261=CARTESIAN_POINT('Ctrl Pts',(-30.8445423217259,12.445274073871,128.133104829671)) ;
#116262=CARTESIAN_POINT('Ctrl Pts',(-30.9331533396269,12.6067971683827,
128.358841764631)) ;
#116263=CARTESIAN_POINT('Ctrl Pts',(-31.0052235518519,12.8274892534517,
128.536166471027)) ;
#116264=CARTESIAN_POINT('Ctrl Pts',(-31.0557929024469,13.0891408927057,
128.650910668167)) ;
#116265=CARTESIAN_POINT('Ctrl Pts',(-31.0826649707566,13.375740122579,128.696283133412)) ;
#116266=CARTESIAN_POINT('Ctrl Pts',(-31.0842457464183,13.6659116032671,
128.667755109105)) ;
#116267=CARTESIAN_POINT('Ctrl Pts',(-31.0612969342213,13.9383430672958,
128.567621981036)) ;
#116268=CARTESIAN_POINT('Ctrl Pts',(-31.0158421470532,14.1747318786697,
128.401589927848)) ;
#116269=CARTESIAN_POINT('Ctrl Pts',(-30.952741170991,14.3556000224366,128.184334680318)) ;
#116270=CARTESIAN_POINT('Ctrl Pts',(-30.8757148543573,14.4715471852787,
127.925954832144)) ;
#116271=CARTESIAN_POINT('Ctrl Pts',(-30.7926989079768,14.5109306884899,
127.650429154449)) ;
#116272=CARTESIAN_POINT('Ctrl Pts',(-30.7096170404131,14.4734197510009,
127.374712802353)) ;
#116273=CARTESIAN_POINT('Ctrl Pts',(-30.6324207964218,14.3595613312843,
127.115883659408)) ;
#116274=CARTESIAN_POINT('Ctrl Pts',(-30.5687431637558,14.179466171533,126.896825275717)) ;
#116275=CARTESIAN_POINT('Ctrl Pts',(-30.5229949276125,13.9455181185487,
126.730115674649)) ;
#116276=CARTESIAN_POINT('Ctrl Pts',(-30.4993062024708,13.6723045745694,
126.627634301698)) ;
#116277=CARTESIAN_POINT('Ctrl Pts',(-30.5003214317798,13.3834915874396,
126.597593551244)) ;
#116278=CARTESIAN_POINT('Ctrl Pts',(-30.5264493139276,13.0966134068724,
126.640803917263)) ;
#116279=CARTESIAN_POINT('Ctrl Pts',(-30.5766713219404,12.8330521051259,
126.754396922064)) ;
#116280=CARTESIAN_POINT('Ctrl Pts',(-30.6483002280116,12.6112324338377,
126.930439181463)) ;
#116281=CARTESIAN_POINT('Ctrl Pts',(-30.736661695068,12.4482429025448,127.155425447181)) ;
#116282=CARTESIAN_POINT('Ctrl Pts',(-30.8357315528907,12.3553252392396,
127.411846833704)) ;
#116283=CARTESIAN_POINT('Ctrl Pts',(-30.9400335857783,12.3382107107946,
127.683413725756)) ;
#116284=CARTESIAN_POINT('Ctrl Pts',(-31.042636248853,12.3992481458877,127.94994445052)) ;
#116285=CARTESIAN_POINT('Ctrl Pts',(-31.1362393771601,12.5331204758664,
128.190343537901)) ;
#116286=CARTESIAN_POINT('Ctrl Pts',(-31.215635139957,12.7309387918669,128.389145202128)) ;
#116287=CARTESIAN_POINT('Ctrl Pts',(-31.2756357249041,12.9791524410526,
128.53120468286)) ;
#116288=CARTESIAN_POINT('Ctrl Pts',(-31.312400854353,13.2585790598106,128.605475928875)) ;
#116289=CARTESIAN_POINT('Ctrl Pts',(-31.3241836080649,13.5499397896395,
128.606744173026)) ;
#116290=CARTESIAN_POINT('Ctrl Pts',(-31.3110087346716,13.8311712407388,
128.535239748079)) ;
#116291=CARTESIAN_POINT('Ctrl Pts',(-31.2742363093329,14.0848085651835,
128.394579152518)) ;
#116292=CARTESIAN_POINT('Ctrl Pts',(-31.2178679894401,14.2892041446737,
128.196968022278)) ;
#116293=CARTESIAN_POINT('Ctrl Pts',(-31.1457920021485,14.4332159069687,
127.953199131549)) ;
#116294=CARTESIAN_POINT('Ctrl Pts',(-31.064501704361,14.5042073782218,127.682616508337)) ;
#116295=CARTESIAN_POINT('Ctrl Pts',(-30.9803569070733,14.4978850554144,
127.403677198383)) ;
#116296=CARTESIAN_POINT('Ctrl Pts',(-30.9001457048563,14.4145534025925,
127.136236709374)) ;
#116297=CARTESIAN_POINT('Ctrl Pts',(-30.8302915857101,14.2600830965558,
126.899030948309)) ;
#116298=CARTESIAN_POINT('Ctrl Pts',(-30.7766783037662,14.0459659620245,
126.70932486434)) ;
#116299=CARTESIAN_POINT('Ctrl Pts',(-30.7436688177568,13.7875807752627,
126.579828846178)) ;
#116300=CARTESIAN_POINT('Ctrl Pts',(-30.7344309347098,13.5015008973902,
126.519590640979)) ;
#116301=CARTESIAN_POINT('Ctrl Pts',(-30.7503570117774,13.2119712102584,
126.533117195425)) ;
#116302=CARTESIAN_POINT('Ctrl Pts',(-30.7909948356034,12.9363053782512,
126.618694908227)) ;
#116303=CARTESIAN_POINT('Ctrl Pts',(-30.8544313460082,12.6952736602129,
126.770815078882)) ;
#116304=CARTESIAN_POINT('Ctrl Pts',(-30.936259477995,12.507125678723,126.976810991267)) ;
#116305=CARTESIAN_POINT('Ctrl Pts',(-31.0324849838793,12.3837628513247,
127.224594411425)) ;
#116306=CARTESIAN_POINT('Ctrl Pts',(-31.1350680188049,12.3357954087756,
127.491330342941)) ;
#116307=CARTESIAN_POINT('Ctrl Pts',(-31.23935127795,12.3652711251859,127.762742575844)) ;
#116308=CARTESIAN_POINT('Ctrl Pts',(-31.3372466101365,12.4705156806676,
128.015655972246)) ;
#116309=CARTESIAN_POINT('Ctrl Pts',(-31.4231098978925,12.6439184973371,
128.233370607722)) ;
#116310=CARTESIAN_POINT('Ctrl Pts',(-31.4913656157794,12.8730354055636,
128.399662361953)) ;
#116311=CARTESIAN_POINT('Ctrl Pts',(-31.5379531663441,13.1424159445997,
128.502550794473)) ;
#116312=CARTESIAN_POINT('Ctrl Pts',(-31.5599892196137,13.4306391754528,
128.533873702179)) ;
#116313=CARTESIAN_POINT('Ctrl Pts',(-31.5568791607716,13.7191539441457,
128.491638388163)) ;
#116314=CARTESIAN_POINT('Ctrl Pts',(-31.5294551877072,13.9861293896989,
128.378414253767)) ;
#116315=CARTESIAN_POINT('Ctrl Pts',(-31.4804720297221,14.2128684001206,
128.202207341774)) ;
#116316=CARTESIAN_POINT('Ctrl Pts',(-31.4139631417804,14.3833347965248,
127.974731570058)) ;
#116317=CARTESIAN_POINT('Ctrl Pts',(-31.3357239804157,14.4845639099252,
127.713064266216)) ;
#116318=CARTESIAN_POINT('Ctrl Pts',(-31.2519760904658,14.5099092471542,
127.435310311413)) ;
#116319=CARTESIAN_POINT('Ctrl Pts',(-31.169269063561,14.4573341215463,127.160540128222)) ;
#116320=CARTESIAN_POINT('Ctrl Pts',(-31.0944827944426,14.3305258270945,
126.908931141692)) ;
#116321=CARTESIAN_POINT('Ctrl Pts',(-31.0337818947545,14.1393930806654,
126.698567894651)) ;
#116322=CARTESIAN_POINT('Ctrl Pts',(-30.991822622221,13.8963012865058,126.542832684996)) ;
#116323=CARTESIAN_POINT('Ctrl Pts',(-30.9727169093987,13.618527952916,126.453788104164)) ;
#116324=CARTESIAN_POINT('Ctrl Pts',(-30.9784116943508,13.3290638567204,
126.43746201239)) ;
#116325=CARTESIAN_POINT('Ctrl Pts',(-31.0092534744897,13.0445549081066,
126.494384804869)) ;
#116326=CARTESIAN_POINT('Ctrl Pts',(-31.0636975928906,12.7876683953407,
126.620329890945)) ;
#116327=CARTESIAN_POINT('Ctrl Pts',(-31.1390893626737,12.5753843248543,
126.807286162987)) ;
#116328=CARTESIAN_POINT('Ctrl Pts',(-31.2294856731981,12.4255194566962,
127.038405016624)) ;
#116329=CARTESIAN_POINT('Ctrl Pts',(-31.3305520361071,12.3459765628223,
127.300458413669)) ;
#116330=CARTESIAN_POINT('Ctrl Pts',(-31.434776599086,12.3439073333341,127.571874828474)) ;
#116331=CARTESIAN_POINT('Ctrl Pts',(-31.5361216061782,12.4188279963137,
127.834788869403)) ;
#116332=CARTESIAN_POINT('Ctrl Pts',(-31.6280697762185,12.5669347456838,
128.070100154879)) ;
#116333=CARTESIAN_POINT('Ctrl Pts',(-31.7035334984892,12.7740276750078,
128.257653591068)) ;
#116334=CARTESIAN_POINT('Ctrl Pts',(-31.759609829367,13.0302839963835,128.388157305165)) ;
#116335=CARTESIAN_POINT('Ctrl Pts',(-31.7916573927032,13.3133908418281,
128.44867020828)) ;
#116336=CARTESIAN_POINT('Ctrl Pts',(-31.7986966116337,13.603463644202,128.436213818987)) ;
#116337=CARTESIAN_POINT('Ctrl Pts',(-31.7809913371395,13.8813033828735,
128.35140974243)) ;
#116338=CARTESIAN_POINT('Ctrl Pts',(-31.7400851389627,14.1277803353935,
128.198621302036)) ;
#116339=CARTESIAN_POINT('Ctrl Pts',(-31.6800730695565,14.3222499491186,
127.990196055143)) ;
#116340=CARTESIAN_POINT('Ctrl Pts',(-31.6061655491007,14.4521801137134,
127.741284607191)) ;
#116341=CARTESIAN_POINT('Ctrl Pts',(-31.5238300942761,14.5090397013049,
127.467639877269)) ;
#116342=CARTESIAN_POINT('Ctrl Pts',(-31.4398666707468,14.4879536383768,
127.189213876511)) ;
#116343=CARTESIAN_POINT('Ctrl Pts',(-31.3611027665607,14.3907169193799,
126.925998091316)) ;
#116344=CARTESIAN_POINT('Ctrl Pts',(-31.2937040056646,14.2230874926912,
126.695841876849)) ;
#116345=CARTESIAN_POINT('Ctrl Pts',(-31.2439920013192,14.0008521290395,
126.517762290878)) ;
#116346=CARTESIAN_POINT('Ctrl Pts',(-31.2150907661555,13.7343152663338,
126.400042595703)) ;
#116347=CARTESIAN_POINT('Ctrl Pts',(-31.2106083276963,13.4474451530714,
126.353922032443)) ;
#116348=CARTESIAN_POINT('Ctrl Pts',(-31.2313383311631,13.1575373599845,
126.381288702569)) ;
#116349=CARTESIAN_POINT('Ctrl Pts',(-31.2764056532061,12.8878586186382,
126.479905180231)) ;
#116350=CARTESIAN_POINT('Ctrl Pts',(-31.3436059924202,12.6555337160297,
126.643048484565)) ;
#116351=CARTESIAN_POINT('Ctrl Pts',(-31.4286039772841,12.4784852863875,
126.858237182344)) ;
#116352=CARTESIAN_POINT('Ctrl Pts',(-31.5266156330296,12.3688435126028,
127.11128245237)) ;
#116353=CARTESIAN_POINT('Ctrl Pts',(-31.630084559127,12.335379050582,127.380536177025)) ;
#116354=CARTESIAN_POINT('Ctrl Pts',(-31.7333993373061,12.3794309050292,
127.649233966248)) ;
#116355=CARTESIAN_POINT('Ctrl Pts',(-31.8295546512421,12.4979553005814,
127.897051153347)) ;
#116356=CARTESIAN_POINT('Ctrl Pts',(-31.9129345986958,12.6843641512771,
128.107301604166)) ;
#116357=CARTESIAN_POINT('Ctrl Pts',(-31.9769081760024,12.9208195190715,
128.261300839291)) ;
#116358=CARTESIAN_POINT('Ctrl Pts',(-32.0192234596835,13.1965599156971,
128.351576775379)) ;
#116359=CARTESIAN_POINT('Ctrl Pts',(-32.0364080377691,13.4854150034454,
128.36882968244)) ;
#116360=CARTESIAN_POINT('Ctrl Pts',(-32.0286590942519,13.7715245103546,
128.313041033143)) ;
#116361=CARTESIAN_POINT('Ctrl Pts',(-31.9967949405779,14.0329603333754,
128.186757372476)) ;
#116362=CARTESIAN_POINT('Ctrl Pts',(-31.9442598511563,14.2495174070446,
128.000252912401)) ;
#116363=CARTESIAN_POINT('Ctrl Pts',(-31.8752637456382,14.4077221355952,
127.765584521541)) ;
#116364=CARTESIAN_POINT('Ctrl Pts',(-31.7949904880439,14.4954974794661,
127.497773147365)) ;
#116365=CARTESIAN_POINT('Ctrl Pts',(-31.7112118667338,14.5058124227374,
127.220036909701)) ;
#116366=CARTESIAN_POINT('Ctrl Pts',(-31.6295895835472,14.4390540160987,
126.948477953836)) ;
#116367=CARTESIAN_POINT('Ctrl Pts',(-31.5567958768622,14.2988995016989,
126.702614005723)) ;
#116368=CARTESIAN_POINT('Ctrl Pts',(-31.4992152164798,14.0959846822767,
126.501253268444)) ;
#116369=CARTESIAN_POINT('Ctrl Pts',(-31.4616155663629,13.8467238077785,
126.358483470145)) ;
#116370=CARTESIAN_POINT('Ctrl Pts',(-31.4469797675735,13.5651499595772,
126.282529118317)) ;
#116371=CARTESIAN_POINT('Ctrl Pts',(-31.4573898379876,13.2745210705863,
126.279884269193)) ;
#116372=CARTESIAN_POINT('Ctrl Pts',(-31.4929777781403,12.9930481847516,
126.350603500459)) ;
#116373=CARTESIAN_POINT('Ctrl Pts',(-31.5514293278227,12.7442685275202,
126.488355718607)) ;
#116374=CARTESIAN_POINT('Ctrl Pts',(-31.629789771733,12.5428869624623,126.684118709821)) ;
#116375=CARTESIAN_POINT('Ctrl Pts',(-31.7230911251259,12.4047083280592,
126.923514916853)) ;
#116376=CARTESIAN_POINT('Ctrl Pts',(-31.8251196709966,12.3396945526809,
127.188456991403)) ;
#116377=CARTESIAN_POINT('Ctrl Pts',(-31.9293847768492,12.3521469576885,
127.459951466802)) ;
#116378=CARTESIAN_POINT('Ctrl Pts',(-32.0293584096416,12.441314353945,127.718862688757)) ;
#116379=CARTESIAN_POINT('Ctrl Pts',(-32.118508034267,12.6011043288198,127.946125196227)) ;
#116380=CARTESIAN_POINT('Ctrl Pts',(-32.1909463624357,12.8194224397463,
128.124637671274)) ;
#116381=CARTESIAN_POINT('Ctrl Pts',(-32.2424853469496,13.0811434342732,
128.242065843194)) ;
#116382=CARTESIAN_POINT('Ctrl Pts',(-32.2700475124695,13.3679217852881,
128.289393931887)) ;
#116383=CARTESIAN_POINT('Ctrl Pts',(-32.2723234688677,13.6574454003315,
128.262990706036)) ;
#116384=CARTESIAN_POINT('Ctrl Pts',(-32.2501377563472,13.9304218890574,
128.16512094437)) ;
#116385=CARTESIAN_POINT('Ctrl Pts',(-32.2052527136117,14.1686008595605,
128.000705406738)) ;
#116386=CARTESIAN_POINT('Ctrl Pts',(-32.1424368825761,14.3514046814191,
127.78421431945)) ;
#116387=CARTESIAN_POINT('Ctrl Pts',(-32.0661890017219,14.4688537010489,
127.528311842842)) ;
#116388=CARTESIAN_POINT('Ctrl Pts',(-31.9829477124764,14.5110084065472,
127.25198980975)) ;
#116389=CARTESIAN_POINT('Ctrl Pts',(-31.8996523370137,14.4754271659884,
126.975598872173)) ;
#116390=CARTESIAN_POINT('Ctrl Pts',(-31.8224332847297,14.3641624802179,
126.716820698264)) ;
#116391=CARTESIAN_POINT('Ctrl Pts',(-31.7580395500746,14.1852632695012,
126.495546204119)) ;
#116392=CARTESIAN_POINT('Ctrl Pts',(-31.7118161309124,13.9526451401233,
126.327472065972)) ;
#116393=CARTESIAN_POINT('Ctrl Pts',(-31.6875151171821,13.6818447118076,
126.223384381321)) ;
#116394=CARTESIAN_POINT('Ctrl Pts',(-31.6876428707132,13.3926206452482,
126.190673672069)) ;
#116395=CARTESIAN_POINT('Ctrl Pts',(-31.7132303697958,13.1038754923078,
126.232132655585)) ;
#116396=CARTESIAN_POINT('Ctrl Pts',(-31.7626844305404,12.8403836297391,
126.343597807942)) ;
#116397=CARTESIAN_POINT('Ctrl Pts',(-31.833493429736,12.6175434576375,126.517332769775)) ;
#116398=CARTESIAN_POINT('Ctrl Pts',(-31.9215930084005,12.4520178789147,
126.741478574285)) ;
#116399=CARTESIAN_POINT('Ctrl Pts',(-32.0209307914902,12.3567780608222,
126.998523271918)) ;
#116400=CARTESIAN_POINT('Ctrl Pts',(-32.1246416504795,12.3376561109864,
127.268538964137)) ;
#116401=CARTESIAN_POINT('Ctrl Pts',(-32.2275246940126,12.3963494804203,
127.535847716125)) ;
#116402=CARTESIAN_POINT('Ctrl Pts',(-32.3214673626583,12.5282529228556,
127.777238677115)) ;
#116403=CARTESIAN_POINT('Ctrl Pts',(-32.4013423719323,12.7243873042916,
127.977442347176)) ;
#116404=CARTESIAN_POINT('Ctrl Pts',(-32.4619096573449,12.9708923918956,
128.121216797039)) ;
#116405=CARTESIAN_POINT('Ctrl Pts',(-32.4994416556502,13.2502126197918,
128.197659332614)) ;
#116406=CARTESIAN_POINT('Ctrl Pts',(-32.5119978982385,13.5400583828972,
128.201358931735)) ;
#116407=CARTESIAN_POINT('Ctrl Pts',(-32.4994888167825,13.8239338286533,
128.131553230696)) ;
#116408=CARTESIAN_POINT('Ctrl Pts',(-32.4634273595897,14.0777676729547,
127.99308635593)) ;
#116409=CARTESIAN_POINT('Ctrl Pts',(-32.4075028614965,14.2841378500946,
127.796711420429)) ;
#116410=CARTESIAN_POINT('Ctrl Pts',(-32.3359847249591,14.429815657766,127.554661094343)) ;
#116411=CARTESIAN_POINT('Ctrl Pts',(-32.2546028623038,14.5033259168077,
127.283693381333)) ;
#116412=CARTESIAN_POINT('Ctrl Pts',(-32.1704924928081,14.499135115111,127.004877771061)) ;
#116413=CARTESIAN_POINT('Ctrl Pts',(-32.0900191687497,14.4177798325381,
126.736640312097)) ;
#116414=CARTESIAN_POINT('Ctrl Pts',(-32.0200109297833,14.2657377102023,
126.499094130843)) ;
#116415=CARTESIAN_POINT('Ctrl Pts',(-31.9656700623202,14.0527574173429,
126.30717910773)) ;
#116416=CARTESIAN_POINT('Ctrl Pts',(-31.9319934820835,13.7942044324148,
126.175602610685)) ;
#116417=CARTESIAN_POINT('Ctrl Pts',(-31.922152144827,13.509972220369,126.1137676569)) ;
#116418=CARTESIAN_POINT('Ctrl Pts',(-31.9373531303038,13.219834764377,126.12511889965)) ;
#116419=CARTESIAN_POINT('Ctrl Pts',(-31.9773715779164,12.9433154987134,
126.208868906181)) ;
#116420=CARTESIAN_POINT('Ctrl Pts',(-32.0403631928475,12.7008042356819,
126.359640175799)) ;
#116421=CARTESIAN_POINT('Ctrl Pts',(-32.1214625671299,12.5118988342583,
126.563632155226)) ;
#116422=CARTESIAN_POINT('Ctrl Pts',(-32.2168510067031,12.3867144480253,
126.809132213192)) ;
#116423=CARTESIAN_POINT('Ctrl Pts',(-32.3199033888381,12.3359851161897,
127.077044236849)) ;
#116424=CARTESIAN_POINT('Ctrl Pts',(-32.4242222709057,12.3634203970633,
127.348571063411)) ;
#116425=CARTESIAN_POINT('Ctrl Pts',(-32.5223579803355,12.4663876358086,
127.602200216398)) ;
#116426=CARTESIAN_POINT('Ctrl Pts',(-32.6089883742709,12.6389701182042,
127.82200642748)) ;
#116427=CARTESIAN_POINT('Ctrl Pts',(-32.6774297887948,12.8657474577828,
127.988998597794)) ;
#116428=CARTESIAN_POINT('Ctrl Pts',(-32.724805208469,13.1346343436699,128.094136048027)) ;
#116429=CARTESIAN_POINT('Ctrl Pts',(-32.7399114943369,13.3266512177486,
128.116225545094)) ;
#116430=CARTESIAN_POINT('Ctrl Pts',(-32.7433109767759,13.4226801736581,
128.115135559137)) ;
#116431=CARTESIAN_POINT('Ctrl Pts',(-11.3048362387632,13.1734341962953,
133.294175679076)) ;
#116432=CARTESIAN_POINT('Ctrl Pts',(-11.3055397872598,13.1676985117492,
133.295499960923)) ;
#116433=CARTESIAN_POINT('Ctrl Pts',(-11.3170134107587,13.0762045259503,
133.317334845661)) ;
#116434=CARTESIAN_POINT('Ctrl Pts',(-11.3479906245566,12.9034782773047,
133.384852143393)) ;
#116435=CARTESIAN_POINT('Ctrl Pts',(-11.4126663887472,12.6923998391673,
133.540763803588)) ;
#116436=CARTESIAN_POINT('Ctrl Pts',(-11.493631562145,12.5327609209973,133.744177423375)) ;
#116437=CARTESIAN_POINT('Ctrl Pts',(-11.5862892630392,12.4368205813749,
133.981580357227)) ;
#116438=CARTESIAN_POINT('Ctrl Pts',(-11.6832291399257,12.4119420222618,
134.231836866922)) ;
#116439=CARTESIAN_POINT('Ctrl Pts',(-11.78005525905,12.4592681303251,134.481464238848)) ;
#116440=CARTESIAN_POINT('Ctrl Pts',(-11.8693322167585,12.5756589901857,
134.709172628028)) ;
#116441=CARTESIAN_POINT('Ctrl Pts',(-11.9459105506398,12.7528353501054,
134.899733529327)) ;
#116442=CARTESIAN_POINT('Ctrl Pts',(-12.0048397897214,12.9779970726337,
135.038757218061)) ;
#116443=CARTESIAN_POINT('Ctrl Pts',(-12.0426597744358,13.2349353323575,
135.116124740278)) ;
#116444=CARTESIAN_POINT('Ctrl Pts',(-12.0574764879123,13.5051817925228,
135.126317551283)) ;
#116445=CARTESIAN_POINT('Ctrl Pts',(-12.0487533971068,13.7710455478253,
135.067545544702)) ;
#116446=CARTESIAN_POINT('Ctrl Pts',(-12.0181630588652,14.0095405119009,
134.945221836394)) ;
#116447=CARTESIAN_POINT('Ctrl Pts',(-11.9683909050091,14.207375982779,134.766695726132)) ;
#116448=CARTESIAN_POINT('Ctrl Pts',(-11.903769353582,14.3489569036635,134.544805288448)) ;
#116449=CARTESIAN_POINT('Ctrl Pts',(-11.8294467098174,14.4243647348289,
134.294477966775)) ;
#116450=CARTESIAN_POINT('Ctrl Pts',(-11.751885562071,14.4276726167065,134.034782669487)) ;
#116451=CARTESIAN_POINT('Ctrl Pts',(-11.6772862681535,14.3592846174027,
133.783789327162)) ;
#116452=CARTESIAN_POINT('Ctrl Pts',(-11.611513681331,14.2239083327593,133.558547654538)) ;
#116453=CARTESIAN_POINT('Ctrl Pts',(-11.5599948518806,14.0309432296264,
133.374897001415)) ;
#116454=CARTESIAN_POINT('Ctrl Pts',(-11.5272842544717,13.793723337017,133.2461166906)) ;
#116455=CARTESIAN_POINT('Ctrl Pts',(-11.516538548757,13.531837086658,133.181746910791)) ;
#116456=CARTESIAN_POINT('Ctrl Pts',(-11.5289803651642,13.2609089527483,
133.184950619645)) ;
#116457=CARTESIAN_POINT('Ctrl Pts',(-11.5648046980364,13.0011532245151,
133.256394467539)) ;
#116458=CARTESIAN_POINT('Ctrl Pts',(-11.6216466377954,12.7729628061281,
133.389432711134)) ;
#116459=CARTESIAN_POINT('Ctrl Pts',(-11.6968168147813,12.5901802135074,
133.575825804335)) ;
#116460=CARTESIAN_POINT('Ctrl Pts',(-11.7850384827174,12.4676468179757,
133.800475594732)) ;
#116461=CARTESIAN_POINT('Ctrl Pts',(-11.8814377069306,12.4133145081089,
134.04885414273)) ;
#116462=CARTESIAN_POINT('Ctrl Pts',(-11.9787704166135,12.4313808819739,
134.300185342639)) ;
#116463=CARTESIAN_POINT('Ctrl Pts',(-12.0720174352247,12.520660304575,134.539371072293)) ;
#116464=CARTESIAN_POINT('Ctrl Pts',(-12.1542732554476,12.6744195620442,
134.746571867679)) ;
#116465=CARTESIAN_POINT('Ctrl Pts',(-12.2208394898278,12.8815892822748,
134.907929827527)) ;
#116466=CARTESIAN_POINT('Ctrl Pts',(-12.2677283074646,13.1290193057785,
135.011625583399)) ;
#116467=CARTESIAN_POINT('Ctrl Pts',(-12.2918106276939,13.3950772223713,
135.049016578508)) ;
#116468=CARTESIAN_POINT('Ctrl Pts',(-12.2926944047224,13.66434219871,135.018483925566)) ;
#116469=CARTESIAN_POINT('Ctrl Pts',(-12.2706182916445,13.9170737503532,
134.920777667333)) ;
#116470=CARTESIAN_POINT('Ctrl Pts',(-12.2281264946411,14.1334228182709,
134.763559895528)) ;
#116471=CARTESIAN_POINT('Ctrl Pts',(-12.1690356539749,14.2989215662944,
134.557882314795)) ;
#116472=CARTESIAN_POINT('Ctrl Pts',(-12.0980917977181,14.4021434485844,
134.317520347929)) ;
#116473=CARTESIAN_POINT('Ctrl Pts',(-12.0209753725309,14.4351203020035,
134.059037518786)) ;
#116474=CARTESIAN_POINT('Ctrl Pts',(-11.9445266332495,14.3956460292368,
133.802668787202)) ;
#116475=CARTESIAN_POINT('Ctrl Pts',(-11.8742770006212,14.2864256382767,
133.564281364103)) ;
#116476=CARTESIAN_POINT('Ctrl Pts',(-11.8163463282874,14.1149876156061,
133.361875622449)) ;
#116477=CARTESIAN_POINT('Ctrl Pts',(-11.7757287928858,13.8950778859157,
133.210204358206)) ;
#116478=CARTESIAN_POINT('Ctrl Pts',(-11.7556794040892,13.6402949383964,
133.118454428844)) ;
#116479=CARTESIAN_POINT('Ctrl Pts',(-11.7586748594706,13.3700135586503,
133.094045455985)) ;
#116480=CARTESIAN_POINT('Ctrl Pts',(-11.7850940030148,13.1040821018971,
133.138124942152)) ;
#116481=CARTESIAN_POINT('Ctrl Pts',(-11.8337147621843,12.8608604058745,
133.247060692441)) ;
#116482=CARTESIAN_POINT('Ctrl Pts',(-11.9022657738097,12.6570995861258,
133.414051481575)) ;
#116483=CARTESIAN_POINT('Ctrl Pts',(-11.9854697021189,12.5097126273575,
133.624148755478)) ;
#116484=CARTESIAN_POINT('Ctrl Pts',(-12.0792563949215,12.4266925864004,
133.864954668484)) ;
#116485=CARTESIAN_POINT('Ctrl Pts',(-12.1770501733971,12.4153566077392,
134.117516473008)) ;
#116486=CARTESIAN_POINT('Ctrl Pts',(-12.2726562901117,12.4761183331586,
134.363693217074)) ;
#116487=CARTESIAN_POINT('Ctrl Pts',(-12.3599672381387,12.6046109786899,
134.585648111921)) ;
#116488=CARTESIAN_POINT('Ctrl Pts',(-12.4336049342943,12.792032892229,134.767601788144)) ;
#116489=CARTESIAN_POINT('Ctrl Pts',(-12.4887847478915,13.0246459231079,
134.895657747207)) ;
#116490=CARTESIAN_POINT('Ctrl Pts',(-12.5223167102954,13.2849675496699,
134.960574363912)) ;
#116491=CARTESIAN_POINT('Ctrl Pts',(-12.5327426141042,13.5561838423073,
134.957866664727)) ;
#116492=CARTESIAN_POINT('Ctrl Pts',(-12.5197199828827,13.8182129454441,
134.886604960408)) ;
#116493=CARTESIAN_POINT('Ctrl Pts',(-12.4852778576315,14.0504673994418,
134.752981386935)) ;
#116494=CARTESIAN_POINT('Ctrl Pts',(-12.432142512104,14.2392687956967,134.564522703169)) ;
#116495=CARTESIAN_POINT('Ctrl Pts',(-12.3651870124344,14.3686948710642,
134.335789865245)) ;
#116496=CARTESIAN_POINT('Ctrl Pts',(-12.2902985792148,14.4303698610576,
134.084054618578)) ;
#116497=CARTESIAN_POINT('Ctrl Pts',(-12.2126339213949,14.4203874495029,
133.82398885631)) ;
#116498=CARTESIAN_POINT('Ctrl Pts',(-12.138892983068,14.3383234433453,133.5753360581)) ;
#116499=CARTESIAN_POINT('Ctrl Pts',(-12.0755004122428,14.1909247439309,
133.357045112776)) ;
#116500=CARTESIAN_POINT('Ctrl Pts',(-12.0274928686727,13.9894772519221,
133.18381104636)) ;
#116501=CARTESIAN_POINT('Ctrl Pts',(-11.9986969915971,13.7468083909025,
133.066570085229)) ;
#116502=CARTESIAN_POINT('Ctrl Pts',(-11.9921460683351,13.4802543553281,
133.014236646284)) ;
#116503=CARTESIAN_POINT('Ctrl Pts',(-12.0092717413035,13.2092851257182,
133.031023331709)) ;
#116504=CARTESIAN_POINT('Ctrl Pts',(-12.0488941477586,12.956342695595,133.113890140615)) ;
#116505=CARTESIAN_POINT('Ctrl Pts',(-12.1097548196694,12.7340443035837,
133.258436779888)) ;
#116506=CARTESIAN_POINT('Ctrl Pts',(-12.1878735220382,12.5620254475304,
133.453464717486)) ;
#116507=CARTESIAN_POINT('Ctrl Pts',(-12.2776773534867,12.45216345603,133.682848097027)) ;
#116508=CARTESIAN_POINT('Ctrl Pts',(-12.3749985350835,12.4110698281944,
133.933870441482)) ;
#116509=CARTESIAN_POINT('Ctrl Pts',(-12.4722736125084,12.4431134785041,
134.184910270632)) ;
#116510=CARTESIAN_POINT('Ctrl Pts',(-12.5633905416193,12.544720783163,134.418071752808)) ;
#116511=CARTESIAN_POINT('Ctrl Pts',(-12.6432257122409,12.7094608170751,
134.618156747253)) ;
#116512=CARTESIAN_POINT('Ctrl Pts',(-12.7064847924193,12.9261933498066,
134.769723779734)) ;
#116513=CARTESIAN_POINT('Ctrl Pts',(-12.7489848469751,13.1767718308822,
134.860888243943)) ;
#116514=CARTESIAN_POINT('Ctrl Pts',(-12.7689773196155,13.4474343048381,
134.885986597225)) ;
#116515=CARTESIAN_POINT('Ctrl Pts',(-12.7652633609867,13.7143157453809,
134.842086211151)) ;
#116516=CARTESIAN_POINT('Ctrl Pts',(-12.7393471136398,13.9601208806252,
134.733384856506)) ;
#116517=CARTESIAN_POINT('Ctrl Pts',(-12.6931971015378,14.1691500146303,
134.565311032996)) ;
#116518=CARTESIAN_POINT('Ctrl Pts',(-12.6315346459168,14.3234012813758,
134.352162858764)) ;
#116519=CARTESIAN_POINT('Ctrl Pts',(-12.5588878324743,14.4138714388817,
134.10676963584)) ;
#116520=CARTESIAN_POINT('Ctrl Pts',(-12.4816544367157,14.433295070235,133.848083489319)) ;
#116521=CARTESIAN_POINT('Ctrl Pts',(-12.4053524670984,14.3798377067091,
133.59187082097)) ;
#116522=CARTESIAN_POINT('Ctrl Pts',(-12.3374332785635,14.2584887860387,
133.360475482159)) ;
#116523=CARTESIAN_POINT('Ctrl Pts',(-12.2824051002791,14.0772215251275,
133.166601528295)) ;
#116524=CARTESIAN_POINT('Ctrl Pts',(-12.2452321826126,13.847858128252,133.024747347105)) ;
#116525=CARTESIAN_POINT('Ctrl Pts',(-12.2296059826708,13.5896600373134,
132.946061283646)) ;
#116526=CARTESIAN_POINT('Ctrl Pts',(-12.2369463909888,13.3195390353182,
132.934455021102)) ;
#116527=CARTESIAN_POINT('Ctrl Pts',(-12.2677721689925,13.0556171631187,
132.991302288782)) ;
#116528=CARTESIAN_POINT('Ctrl Pts',(-12.3203670457723,12.8189344364704,
133.111861078399)) ;
#116529=CARTESIAN_POINT('Ctrl Pts',(-12.3918779427092,12.6251004110513,
133.287618469956)) ;
#116530=CARTESIAN_POINT('Ctrl Pts',(-12.4777181682038,12.4887479855771,
133.505288390372)) ;
#116531=CARTESIAN_POINT('Ctrl Pts',(-12.5724812251264,12.419067054962,133.749046122386)) ;
#116532=CARTESIAN_POINT('Ctrl Pts',(-12.6706720979256,12.4213699638912,
134.00265513351)) ;
#116533=CARTESIAN_POINT('Ctrl Pts',(-12.7650277550218,12.4953802031986,
134.245230364366)) ;
#116534=CARTESIAN_POINT('Ctrl Pts',(-12.8502559447532,12.6359571478174,
134.46105227128)) ;
#116535=CARTESIAN_POINT('Ctrl Pts',(-12.920636677838,12.8329196540899,134.633528157148)) ;
#116536=CARTESIAN_POINT('Ctrl Pts',(-12.9719270374806,13.0719648930025,
134.750256204096)) ;
#116537=CARTESIAN_POINT('Ctrl Pts',(-13.0012404417528,13.3363496355774,
134.802758227356)) ;
#116538=CARTESIAN_POINT('Ctrl Pts',(-13.0071448579909,13.6070576006529,
134.786864740598)) ;
#116539=CARTESIAN_POINT('Ctrl Pts',(-12.9899370940703,13.8644611285128,
134.703467147797)) ;
#116540=CARTESIAN_POINT('Ctrl Pts',(-12.9516551926093,14.0900772537897,
134.558538596344)) ;
#116541=CARTESIAN_POINT('Ctrl Pts',(-12.8956186659196,14.2682172289019,
134.361685303641)) ;
#116542=CARTESIAN_POINT('Ctrl Pts',(-12.8268821751115,14.3854165946879,
134.127841418099)) ;
#116543=CARTESIAN_POINT('Ctrl Pts',(-12.7507359710591,14.4341663213204,
133.872274094897)) ;
#116544=CARTESIAN_POINT('Ctrl Pts',(-12.6733019917063,14.4102121337139,
133.612860993173)) ;
#116545=CARTESIAN_POINT('Ctrl Pts',(-12.6013206553288,14.3156229192553,
133.369490855547)) ;
#116546=CARTESIAN_POINT('Ctrl Pts',(-12.5403300034414,14.1571117362938,
133.15819579006)) ;
#116547=CARTESIAN_POINT('Ctrl Pts',(-12.4955161110385,13.9459764077607,
132.99415734859)) ;
#116548=CARTESIAN_POINT('Ctrl Pts',(-12.4708094097902,13.6975622322246,
132.888878084011)) ;
#116549=CARTESIAN_POINT('Ctrl Pts',(-12.4686895251068,13.4293974985453,
132.849565965806)) ;
#116550=CARTESIAN_POINT('Ctrl Pts',(-12.4899907029116,13.1610019357677,
132.87870343796)) ;
#116551=CARTESIAN_POINT('Ctrl Pts',(-12.534115379757,12.9105848440385,132.974405179964)) ;
#116552=CARTESIAN_POINT('Ctrl Pts',(-12.5983779539559,12.6976134711112,
133.129031831098)) ;
#116553=CARTESIAN_POINT('Ctrl Pts',(-12.6790326424138,12.5364422844779,
133.331520584852)) ;
#116554=CARTESIAN_POINT('Ctrl Pts',(-12.7709549115279,12.4387732297296,
133.566944783629)) ;
#116555=CARTESIAN_POINT('Ctrl Pts',(-12.8685900163271,12.4116342438892,
133.818970272208)) ;
#116556=CARTESIAN_POINT('Ctrl Pts',(-12.9650394138879,12.4569142353896,
134.067666376452)) ;
#116557=CARTESIAN_POINT('Ctrl Pts',(-13.0547600940725,12.5714751747461,
134.296615286209)) ;
#116558=CARTESIAN_POINT('Ctrl Pts',(-13.1316530817672,12.7468632873084,
134.48814580267)) ;
#116559=CARTESIAN_POINT('Ctrl Pts',(-13.1911572181041,12.9706872458922,
134.628860794572)) ;
#116560=CARTESIAN_POINT('Ctrl Pts',(-13.2296656594081,13.2271704836993,
134.708210769396)) ;
#116561=CARTESIAN_POINT('Ctrl Pts',(-13.2451574771088,13.4971329274745,
134.720396296595)) ;
#116562=CARTESIAN_POINT('Ctrl Pts',(-13.2371292685592,13.7633005024016,
134.663671340864)) ;
#116563=CARTESIAN_POINT('Ctrl Pts',(-13.2072039915708,14.002826770648,134.543298284642)) ;
#116564=CARTESIAN_POINT('Ctrl Pts',(-13.1576917384621,14.2028677119568,
134.365387614197)) ;
#116565=CARTESIAN_POINT('Ctrl Pts',(-13.0936548161381,14.3455611134847,
134.145336236451)) ;
#116566=CARTESIAN_POINT('Ctrl Pts',(-13.0195413649078,14.4231516282667,
133.895616180479)) ;
#116567=CARTESIAN_POINT('Ctrl Pts',(-12.941972170223,14.4286657485207,133.635893474366)) ;
#116568=CARTESIAN_POINT('Ctrl Pts',(-12.8670500417961,14.3621070241951,
133.383882958189)) ;
#116569=CARTESIAN_POINT('Ctrl Pts',(-12.8010036125882,14.2287344049999,
133.157884092812)) ;
#116570=CARTESIAN_POINT('Ctrl Pts',(-12.7488856829864,14.0363062184854,
132.972352197591)) ;
#116571=CARTESIAN_POINT('Ctrl Pts',(-12.7158474360347,13.8023698285734,
132.842926745116)) ;
#116572=CARTESIAN_POINT('Ctrl Pts',(-12.7042635666528,13.538853365046,132.775826591809)) ;
#116573=CARTESIAN_POINT('Ctrl Pts',(-12.7161476495276,13.2684519615159,
132.777472109561)) ;
#116574=CARTESIAN_POINT('Ctrl Pts',(-12.751106729114,13.0087998067706,132.846492569486)) ;
#116575=CARTESIAN_POINT('Ctrl Pts',(-12.807873382857,12.7778891535909,132.979055104978)) ;
#116576=CARTESIAN_POINT('Ctrl Pts',(-12.8820585633444,12.5950174463895,
133.162824352565)) ;
#116577=CARTESIAN_POINT('Ctrl Pts',(-12.9703954300045,12.4700325386615,
133.387640500529)) ;
#116578=CARTESIAN_POINT('Ctrl Pts',(-13.0661153420427,12.4138573770184,
133.634230474633)) ;
#116579=CARTESIAN_POINT('Ctrl Pts',(-13.1643568917053,12.4301864135647,
133.887911381757)) ;
#116580=CARTESIAN_POINT('Ctrl Pts',(-13.2568223360738,12.5166843884807,
134.125173786937)) ;
#116581=CARTESIAN_POINT('Ctrl Pts',(-13.3399856657831,12.6693064636983,
134.334830220743)) ;
#116582=CARTESIAN_POINT('Ctrl Pts',(-13.4068238350571,12.8745470940793,
134.49709490505)) ;
#116583=CARTESIAN_POINT('Ctrl Pts',(-13.4544450063346,13.1212023426986,
134.602896573305)) ;
#116584=CARTESIAN_POINT('Ctrl Pts',(-13.4792271367921,13.3871938876445,
134.642301021761)) ;
#116585=CARTESIAN_POINT('Ctrl Pts',(-13.4807690699808,13.6567281593303,
134.613680601786)) ;
#116586=CARTESIAN_POINT('Ctrl Pts',(-13.4594081480435,13.9097854189498,
134.518129927239)) ;
#116587=CARTESIAN_POINT('Ctrl Pts',(-13.4173442290248,14.1280196349839,
134.362063092164)) ;
#116588=CARTESIAN_POINT('Ctrl Pts',(-13.3587335058981,14.2950456009744,
134.157826230202)) ;
#116589=CARTESIAN_POINT('Ctrl Pts',(-13.2875991149223,14.4005267641298,
133.916709156522)) ;
#116590=CARTESIAN_POINT('Ctrl Pts',(-13.2110834913492,14.4350836720727,
133.660212652327)) ;
#116591=CARTESIAN_POINT('Ctrl Pts',(-13.1344387177937,14.3978038966436,
133.403225607042)) ;
#116592=CARTESIAN_POINT('Ctrl Pts',(-13.0640036054603,14.290575680997,133.164336325255)) ;
#116593=CARTESIAN_POINT('Ctrl Pts',(-13.0056367075179,14.12095115065,132.960667025767)) ;
#116594=CARTESIAN_POINT('Ctrl Pts',(-12.9643797564511,13.9018371946246,
132.807063981847)) ;
#116595=CARTESIAN_POINT('Ctrl Pts',(-12.9437529478308,13.6479071600813,
132.713647362735)) ;
#116596=CARTESIAN_POINT('Ctrl Pts',(-12.9459834540189,13.3785018299636,
132.687089601676)) ;
#116597=CARTESIAN_POINT('Ctrl Pts',(-12.9719279522438,13.1105161592094,
132.729570917894)) ;
#116598=CARTESIAN_POINT('Ctrl Pts',(-13.0197798563459,12.8677237069018,
132.836427718895)) ;
#116599=CARTESIAN_POINT('Ctrl Pts',(-13.0875829119615,12.6628308000804,
133.00130569266)) ;
#116600=CARTESIAN_POINT('Ctrl Pts',(-13.170612266529,12.5130918940735,133.21080218841)) ;
#116601=CARTESIAN_POINT('Ctrl Pts',(-13.2644470385299,12.4280189169956,
133.451662716591)) ;
#116602=CARTESIAN_POINT('Ctrl Pts',(-13.3619248043351,12.4146728594404,
133.703398332785)) ;
#116603=CARTESIAN_POINT('Ctrl Pts',(-13.4579000655806,12.4734182584077,
133.950580622376)) ;
#116604=CARTESIAN_POINT('Ctrl Pts',(-13.5456184208567,12.6005220023049,
134.173675299527)) ;
#116605=CARTESIAN_POINT('Ctrl Pts',(-13.6193388851311,12.7855010880113,
134.35603845551)) ;
#116606=CARTESIAN_POINT('Ctrl Pts',(-13.6752095918886,13.0169859630547,
134.486095608093)) ;
#116607=CARTESIAN_POINT('Ctrl Pts',(-13.7094864157964,13.2774552371681,
134.55310035212)) ;
#116608=CARTESIAN_POINT('Ctrl Pts',(-13.720528633581,13.5483710343065,134.552225521987)) ;
#116609=CARTESIAN_POINT('Ctrl Pts',(-13.7082871445483,13.810085890561,134.483364361746)) ;
#116610=CARTESIAN_POINT('Ctrl Pts',(-13.6743307894067,14.0443619160834,
134.351029938079)) ;
#116611=CARTESIAN_POINT('Ctrl Pts',(-13.6218702674786,14.2339605947032,
134.164668424612)) ;
#116612=CARTESIAN_POINT('Ctrl Pts',(-13.5553037879054,14.3656339160498,
133.937067111739)) ;
#116613=CARTESIAN_POINT('Ctrl Pts',(-13.4801990168619,14.429668532247,133.684537332824)) ;
#116614=CARTESIAN_POINT('Ctrl Pts',(-13.4027282664342,14.4216217933316,
133.425128314253)) ;
#116615=CARTESIAN_POINT('Ctrl Pts',(-13.3290373690102,14.3422174614337,
133.176748800641)) ;
#116616=CARTESIAN_POINT('Ctrl Pts',(-13.2649970207051,14.1963613484393,
132.956451230198)) ;
#116617=CARTESIAN_POINT('Ctrl Pts',(-13.216380386921,13.9958156934089,132.781363475866)) ;
#116618=CARTESIAN_POINT('Ctrl Pts',(-13.1870172083142,13.7540872313105,
132.662471429064)) ;
#116619=CARTESIAN_POINT('Ctrl Pts',(-13.1798006866086,13.4887318703653,
132.608289446469)) ;
#116620=CARTESIAN_POINT('Ctrl Pts',(-13.1961455681105,13.217649057413,132.622802604788)) ;
#116621=CARTESIAN_POINT('Ctrl Pts',(-13.2352634058248,12.9629384688392,
132.704064619144)) ;
#116622=CARTESIAN_POINT('Ctrl Pts',(-13.2957072323222,12.7394456661168,
132.847362756883)) ;
#116623=CARTESIAN_POINT('Ctrl Pts',(-13.3729246066129,12.5666312709512,
133.039944449113)) ;
#116624=CARTESIAN_POINT('Ctrl Pts',(-13.4629469008387,12.4542159420662,
133.26977760258)) ;
#116625=CARTESIAN_POINT('Ctrl Pts',(-13.5596073928236,12.4113528372628,
133.519064068063)) ;
#116626=CARTESIAN_POINT('Ctrl Pts',(-13.6571882769877,12.4409689748371,
133.770921960757)) ;
#116627=CARTESIAN_POINT('Ctrl Pts',(-13.7489524527597,12.5412370844769,
134.005829405415)) ;
#116628=CARTESIAN_POINT('Ctrl Pts',(-13.8289234256402,12.7041353062448,
134.206393920477)) ;
#116629=CARTESIAN_POINT('Ctrl Pts',(-13.8925272076632,12.9183855377871,
134.359123275266)) ;
#116630=CARTESIAN_POINT('Ctrl Pts',(-13.9359235262414,13.1698655592683,
134.4526808629)) ;
#116631=CARTESIAN_POINT('Ctrl Pts',(-13.9564522187295,13.4380609708233,
134.479623940371)) ;
#116632=CARTESIAN_POINT('Ctrl Pts',(-13.9535148154135,13.7071666218626,
134.437760908038)) ;
#116633=CARTESIAN_POINT('Ctrl Pts',(-13.9280836146788,13.9538087956849,
134.330459802866)) ;
#116634=CARTESIAN_POINT('Ctrl Pts',(-13.8826845846232,14.1634526907068,
134.164713123178)) ;
#116635=CARTESIAN_POINT('Ctrl Pts',(-13.8211006600171,14.3201289730171,
133.951628153995)) ;
#116636=CARTESIAN_POINT('Ctrl Pts',(-13.7489996042707,14.4121340863402,
133.707983629453)) ;
#116637=CARTESIAN_POINT('Ctrl Pts',(-13.6715419537195,14.4336855953277,
133.448515884899)) ;
#116638=CARTESIAN_POINT('Ctrl Pts',(-13.5955937037084,14.3827386084068,
133.193555965964)) ;
#116639=CARTESIAN_POINT('Ctrl Pts',(-13.5268624238293,14.2627494800209,
132.959564701033)) ;
#116640=CARTESIAN_POINT('Ctrl Pts',(-13.4713984747695,14.0822577525838,
132.764352915223)) ;
#116641=CARTESIAN_POINT('Ctrl Pts',(-13.4339559473982,13.8561932154224,
132.622014295639)) ;
#116642=CARTESIAN_POINT('Ctrl Pts',(-13.4174952487419,13.5974242945969,
132.540719456061)) ;
#116643=CARTESIAN_POINT('Ctrl Pts',(-13.4241801184799,13.3273252607923,
132.527199302951)) ;
#116644=CARTESIAN_POINT('Ctrl Pts',(-13.4544637530165,13.0622912163539,
132.582375891631)) ;
#116645=CARTESIAN_POINT('Ctrl Pts',(-13.506275683364,12.8256130939751,132.700784905767)) ;
#116646=CARTESIAN_POINT('Ctrl Pts',(-13.5772613807945,12.6301799024571,
132.87500207775)) ;
#116647=CARTESIAN_POINT('Ctrl Pts',(-13.6627580520996,12.4918476681471,
133.091661612145)) ;
#116648=CARTESIAN_POINT('Ctrl Pts',(-13.7577512235869,12.4199209913987,
133.335951670398)) ;
#116649=CARTESIAN_POINT('Ctrl Pts',(-13.8557964795529,12.4204245912294,
133.589185764803)) ;
#116650=CARTESIAN_POINT('Ctrl Pts',(-13.9500806778918,12.4921595921641,
133.831642259008)) ;
#116651=CARTESIAN_POINT('Ctrl Pts',(-14.0357484512663,12.6310172827489,
134.048715775205)) ;
#116652=CARTESIAN_POINT('Ctrl Pts',(-14.106561882642,12.8262646896106,134.222494894414)) ;
#116653=CARTESIAN_POINT('Ctrl Pts',(-14.1585280596083,13.0646913803179,
134.341142107312)) ;
#116654=CARTESIAN_POINT('Ctrl Pts',(-14.1884677945267,13.3278244086872,
134.395572491973)) ;
#116655=CARTESIAN_POINT('Ctrl Pts',(-14.1950850105529,13.5998585157466,
134.381605937844)) ;
#116656=CARTESIAN_POINT('Ctrl Pts',(-14.1785645598048,13.8569826798842,
134.300338480903)) ;
#116657=CARTESIAN_POINT('Ctrl Pts',(-14.1407900933548,14.0842218842957,
134.156820745803)) ;
#116658=CARTESIAN_POINT('Ctrl Pts',(-14.0854221164694,14.2634335835668,
133.962037966108)) ;
#116659=CARTESIAN_POINT('Ctrl Pts',(-14.0165549752706,14.3833954654661,
133.727598260658)) ;
#116660=CARTESIAN_POINT('Ctrl Pts',(-13.9404490568541,14.4336980433791,
133.472126825684)) ;
#116661=CARTESIAN_POINT('Ctrl Pts',(-13.8634700735141,14.4120157811793,
133.214261819804)) ;
#116662=CARTESIAN_POINT('Ctrl Pts',(-13.7910288031297,14.3192946840505,
132.969450563142)) ;
#116663=CARTESIAN_POINT('Ctrl Pts',(-13.7296882371886,14.1625583197416,
132.757157972999)) ;
#116664=CARTESIAN_POINT('Ctrl Pts',(-13.6842292209281,13.9521768872698,
132.591146991905)) ;
#116665=CARTESIAN_POINT('Ctrl Pts',(-13.6590028959702,13.7045477483084,
132.484357602539)) ;
#116666=CARTESIAN_POINT('Ctrl Pts',(-13.6561784444072,13.4377490370904,
132.443119072094)) ;
#116667=CARTESIAN_POINT('Ctrl Pts',(-13.6769260302992,13.1678476255433,
132.470479975427)) ;
#116668=CARTESIAN_POINT('Ctrl Pts',(-13.7202606402325,12.9176590110113,
132.564014027659)) ;
#116669=CARTESIAN_POINT('Ctrl Pts',(-13.7842663792317,12.7025601678247,
132.717748248745)) ;
#116670=CARTESIAN_POINT('Ctrl Pts',(-13.8641216089752,12.5405894739356,
132.9180739667)) ;
#116671=CARTESIAN_POINT('Ctrl Pts',(-13.9560307417598,12.4405287609816,
133.153363600866)) ;
#116672=CARTESIAN_POINT('Ctrl Pts',(-14.0535698736063,12.4114132286229,
133.405122651663)) ;
#116673=CARTESIAN_POINT('Ctrl Pts',(-14.150081341787,12.454644377757,133.654012283986)) ;
#116674=CARTESIAN_POINT('Ctrl Pts',(-14.239925801091,12.5668919625006,133.883394142555)) ;
#116675=CARTESIAN_POINT('Ctrl Pts',(-14.3176379666624,12.7415275985948,
134.077154579645)) ;
#116676=CARTESIAN_POINT('Ctrl Pts',(-14.3775148527287,12.9638992642169,
134.219021942572)) ;
#116677=CARTESIAN_POINT('Ctrl Pts',(-14.416625030145,13.2191082193463,134.300199660408)) ;
#116678=CARTESIAN_POINT('Ctrl Pts',(-14.4328165454319,13.4893534284064,
134.314375207921)) ;
#116679=CARTESIAN_POINT('Ctrl Pts',(-14.4255256959129,13.7553188201862,
134.259890989959)) ;
#116680=CARTESIAN_POINT('Ctrl Pts',(-14.3960306585438,13.9971251061997,
134.140588389539)) ;
#116681=CARTESIAN_POINT('Ctrl Pts',(-14.3471169142548,14.1977811038748,
133.964533561341)) ;
#116682=CARTESIAN_POINT('Ctrl Pts',(-14.2834390765795,14.342451043168,133.745515157142)) ;
#116683=CARTESIAN_POINT('Ctrl Pts',(-14.2092345380845,14.4220642715211,
133.495412056176)) ;
#116684=CARTESIAN_POINT('Ctrl Pts',(-14.132069405725,14.4294491071756,133.237035382782)) ;
#116685=CARTESIAN_POINT('Ctrl Pts',(-14.0570189069592,14.3652072705711,
132.984672203024)) ;
#116686=CARTESIAN_POINT('Ctrl Pts',(-13.9905610685186,14.2335292315096,
132.757432925954)) ;
#116687=CARTESIAN_POINT('Ctrl Pts',(-13.9379853069469,14.0429180682628,
132.570604385206)) ;
#116688=CARTESIAN_POINT('Ctrl Pts',(-13.9042931419094,13.809322141679,132.439170793502)) ;
#116689=CARTESIAN_POINT('Ctrl Pts',(-13.8920413663919,13.5476219044277,
132.370281900748)) ;
#116690=CARTESIAN_POINT('Ctrl Pts',(-13.9033354204781,13.2750712862456,
132.369941141271)) ;
#116691=CARTESIAN_POINT('Ctrl Pts',(-13.9375660928449,13.0163165161328,
132.437013069917)) ;
#116692=CARTESIAN_POINT('Ctrl Pts',(-13.9935170806933,12.7846452326426,
132.567266996895)) ;
#116693=CARTESIAN_POINT('Ctrl Pts',(-14.0674634744735,12.5995256932136,
132.750227603435)) ;
#116694=CARTESIAN_POINT('Ctrl Pts',(-14.1555144396674,12.4726551815389,
132.974201835968)) ;
#116695=CARTESIAN_POINT('Ctrl Pts',(-14.2511648890409,12.4145513483266,
133.220562650021)) ;
#116696=CARTESIAN_POINT('Ctrl Pts',(-14.3489313214769,12.428469046116,133.473033644997)) ;
#116697=CARTESIAN_POINT('Ctrl Pts',(-14.4422211554228,12.5133431382162,
133.712493183629)) ;
#116698=CARTESIAN_POINT('Ctrl Pts',(-14.525697832764,12.664436679697,133.923074942934)) ;
#116699=CARTESIAN_POINT('Ctrl Pts',(-14.5929092045224,12.8679925136389,
134.086485175352)) ;
#116700=CARTESIAN_POINT('Ctrl Pts',(-14.6411040107999,13.1131689974074,
134.19403153726)) ;
#116701=CARTESIAN_POINT('Ctrl Pts',(-14.6666810110784,13.3800002481821,
134.235609154939)) ;
#116702=CARTESIAN_POINT('Ctrl Pts',(-14.6687870768603,13.6495651471469,
134.208652991586)) ;
#116703=CARTESIAN_POINT('Ctrl Pts',(-14.6481856090904,13.9023388794203,
134.115460103099)) ;
#116704=CARTESIAN_POINT('Ctrl Pts',(-14.60655186501,14.122657772282,133.960532567143)) ;
#116705=CARTESIAN_POINT('Ctrl Pts',(-14.5484263911728,14.2908247523975,
133.757774272579)) ;
#116706=CARTESIAN_POINT('Ctrl Pts',(-14.4779478810864,14.3981040608109,
133.518731235387)) ;
#116707=CARTESIAN_POINT('Ctrl Pts',(-14.4009739960646,14.435262692703,133.260657337003)) ;
#116708=CARTESIAN_POINT('Ctrl Pts',(-14.3241585125819,14.3995540237045,
133.003128791361)) ;
#116709=CARTESIAN_POINT('Ctrl Pts',(-14.2538096107005,14.2948938625941,
132.764663780773)) ;
#116710=CARTESIAN_POINT('Ctrl Pts',(-14.1946882431415,14.1259509671256,
132.558599866101)) ;
#116711=CARTESIAN_POINT('Ctrl Pts',(-14.1530855073718,13.908522649266,132.404086330448)) ;
#116712=CARTESIAN_POINT('Ctrl Pts',(-14.1318304371245,13.6557404743469,
132.308879501732)) ;
#116713=CARTESIAN_POINT('Ctrl Pts',(-14.133357452909,13.3866405652258,132.280280185455)) ;
#116714=CARTESIAN_POINT('Ctrl Pts',(-14.1586230794445,13.1181024502092,
132.320757015806)) ;
#116715=CARTESIAN_POINT('Ctrl Pts',(-14.205870750163,12.8743683126388,132.425842572683)) ;
#116716=CARTESIAN_POINT('Ctrl Pts',(-14.273163571627,12.667995764075,132.589221439612)) ;
#116717=CARTESIAN_POINT('Ctrl Pts',(-14.3559649810851,12.5164144284275,
132.798000513578)) ;
#116718=CARTESIAN_POINT('Ctrl Pts',(-14.4492350728485,12.4295970392297,
133.037335011155)) ;
#116719=CARTESIAN_POINT('Ctrl Pts',(-14.5469842766314,12.4140261285354,
133.289756077204)) ;
#116720=CARTESIAN_POINT('Ctrl Pts',(-14.6429502867745,12.4707103016775,
133.536966230591)) ;
#116721=CARTESIAN_POINT('Ctrl Pts',(-14.7309816493984,12.5959067650868,
133.760973594387)) ;
#116722=CARTESIAN_POINT('Ctrl Pts',(-14.8051894304306,12.7791141929297,
133.944779681145)) ;
#116723=CARTESIAN_POINT('Ctrl Pts',(-14.8619602274572,13.0114292224114,
134.07721183711)) ;
#116724=CARTESIAN_POINT('Ctrl Pts',(-14.8965056574982,13.2689898399713,
134.145309850726)) ;
#116725=CARTESIAN_POINT('Ctrl Pts',(-14.9083557189504,13.5409256282928,
134.146659285362)) ;
#116726=CARTESIAN_POINT('Ctrl Pts',(-14.8967214619315,13.8029839862651,
134.079595640576)) ;
#116727=CARTESIAN_POINT('Ctrl Pts',(-14.8633027813701,14.038560788847,133.948790636524)) ;
#116728=CARTESIAN_POINT('Ctrl Pts',(-14.8113056824054,14.2294230403712,
133.763800964968)) ;
#116729=CARTESIAN_POINT('Ctrl Pts',(-14.7451795001818,14.3627051094246,
133.5375393849)) ;
#116730=CARTESIAN_POINT('Ctrl Pts',(-14.6702017629751,14.4288334049426,
133.285362852041)) ;
#116731=CARTESIAN_POINT('Ctrl Pts',(-14.592683156035,14.4228924634038,133.025803055449)) ;
#116732=CARTESIAN_POINT('Ctrl Pts',(-14.5185906675657,14.3451234718206,
132.776153366255)) ;
#116733=CARTESIAN_POINT('Ctrl Pts',(-14.4543104706926,14.2008973362482,
132.555187148786)) ;
#116734=CARTESIAN_POINT('Ctrl Pts',(-14.4053408850151,14.0023960855746,
132.379171294356)) ;
#116735=CARTESIAN_POINT('Ctrl Pts',(-14.3753108185381,13.7610318696562,
132.258251275988)) ;
#116736=CARTESIAN_POINT('Ctrl Pts',(-14.3674916680807,13.4967570532622,
132.202394155313)) ;
#116737=CARTESIAN_POINT('Ctrl Pts',(-14.3830668644292,13.2257686273763,
132.214689433479)) ;
#116738=CARTESIAN_POINT('Ctrl Pts',(-14.4216910972161,12.9695426801037,
132.294399307209)) ;
#116739=CARTESIAN_POINT('Ctrl Pts',(-14.4813916484494,12.7456272140063,
132.435636164476)) ;
#116740=CARTESIAN_POINT('Ctrl Pts',(-14.5581647215385,12.5709695556374,
132.626903642083)) ;
#116741=CARTESIAN_POINT('Ctrl Pts',(-14.6480148950082,12.4565179199043,
132.856192443771)) ;
#116742=CARTESIAN_POINT('Ctrl Pts',(-14.7445907682789,12.4114773768948,
133.105225955903)) ;
#116743=CARTESIAN_POINT('Ctrl Pts',(-14.842595675186,12.4394645441859,133.358192549628)) ;
#116744=CARTESIAN_POINT('Ctrl Pts',(-14.9338942089909,12.5368906975998,
133.592009053689)) ;
#116745=CARTESIAN_POINT('Ctrl Pts',(-15.0149505022409,12.6994727132711,
133.795457044531)) ;
#116746=CARTESIAN_POINT('Ctrl Pts',(-15.0786566558626,12.911284387256,133.948692029528)) ;
#116747=CARTESIAN_POINT('Ctrl Pts',(-15.1229382273336,13.1634090150243,
134.044638248895)) ;
#116748=CARTESIAN_POINT('Ctrl Pts',(-15.1439035555132,13.43009560959,134.073018366311)) ;
#116749=CARTESIAN_POINT('Ctrl Pts',(-15.1418047731794,13.6985487058695,
134.033731705758)) ;
#116750=CARTESIAN_POINT('Ctrl Pts',(-15.1167802714419,13.9480246666546,
133.927350353256)) ;
#116751=CARTESIAN_POINT('Ctrl Pts',(-15.0720912700265,14.1576527817006,
133.763864153658)) ;
#116752=CARTESIAN_POINT('Ctrl Pts',(-15.0109964235137,14.3162850148807,
133.552216483996)) ;
#116753=CARTESIAN_POINT('Ctrl Pts',(-14.9387740010428,14.4106899860489,
133.308061015579)) ;
#116754=CARTESIAN_POINT('Ctrl Pts',(-14.8613476917878,14.4339585124651,
133.048676571636)) ;
#116755=CARTESIAN_POINT('Ctrl Pts',(-14.7856037318579,14.3853107733964,
132.794458393841)) ;
#116756=CARTESIAN_POINT('Ctrl Pts',(-14.7163978676272,14.2669554463922,
132.558995140207)) ;
#116757=CARTESIAN_POINT('Ctrl Pts',(-14.6606048304255,14.0883946272744,
132.362895619543)) ;
#116758=CARTESIAN_POINT('Ctrl Pts',(-14.622541821991,13.8631868173472,132.218696170198)) ;
#116759=CARTESIAN_POINT('Ctrl Pts',(-14.6054425239062,13.6057121370264,
132.135619590578)) ;
#116760=CARTESIAN_POINT('Ctrl Pts',(-14.6114571502439,13.3350529276947,
132.120057688217)) ;
#116761=CARTESIAN_POINT('Ctrl Pts',(-14.6409008769268,13.070755438595,132.172936727227)) ;
#116762=CARTESIAN_POINT('Ctrl Pts',(-14.6921558771164,12.8321487482004,
132.289616780284)) ;
#116763=CARTESIAN_POINT('Ctrl Pts',(-14.7630571786097,12.6344630496442,
132.46342517127)) ;
#116764=CARTESIAN_POINT('Ctrl Pts',(-14.8478315319079,12.4951762287069,
132.678132083268)) ;
#116765=CARTESIAN_POINT('Ctrl Pts',(-14.942435880663,12.4210996304978,132.921347561675)) ;
#116766=CARTESIAN_POINT('Ctrl Pts',(-15.0405912621457,12.4192964067175,
133.174865728553)) ;
#116767=CARTESIAN_POINT('Ctrl Pts',(-15.1352752169109,12.4890491878224,
133.418419532976)) ;
#116768=CARTESIAN_POINT('Ctrl Pts',(-15.2215420412865,12.6268326334366,
133.63712537635)) ;
#116769=CARTESIAN_POINT('Ctrl Pts',(-15.2924017249557,12.819583008208,133.811231474629)) ;
#116770=CARTESIAN_POINT('Ctrl Pts',(-15.3450997694842,13.0571001381562,
133.93198280672)) ;
#116771=CARTESIAN_POINT('Ctrl Pts',(-15.3757107378913,13.3202804831109,
133.988310681278)) ;
#116772=CARTESIAN_POINT('Ctrl Pts',(-15.383035487643,13.5914915741981,133.976525348511)) ;
#116773=CARTESIAN_POINT('Ctrl Pts',(-15.3670672892394,13.8505565623955,
133.896697391881)) ;
#116774=CARTESIAN_POINT('Ctrl Pts',(-15.3300175768013,14.0777828680815,
133.755460891241)) ;
#116775=CARTESIAN_POINT('Ctrl Pts',(-15.2750239975421,14.2590885920228,
133.561696857871)) ;
#116776=CARTESIAN_POINT('Ctrl Pts',(-15.2065269555632,14.3807166711332,
133.328376960357)) ;
#116777=CARTESIAN_POINT('Ctrl Pts',(-15.1306232310638,14.433343609964,133.073523056504)) ;
#116778=CARTESIAN_POINT('Ctrl Pts',(-15.0530845875344,14.4133893696398,
132.813800939999)) ;
#116779=CARTESIAN_POINT('Ctrl Pts',(-14.9808883290291,14.322997838196,132.569914498955)) ;
#116780=CARTESIAN_POINT('Ctrl Pts',(-14.9190772112434,14.1680350352392,
132.356220049076)) ;
#116781=CARTESIAN_POINT('Ctrl Pts',(-14.8731819599279,13.9594348156913,
132.189002061103)) ;
#116782=CARTESIAN_POINT('Ctrl Pts',(-14.8471967295744,13.7128291975183,
132.079998756728)) ;
#116783=CARTESIAN_POINT('Ctrl Pts',(-14.8437841989435,13.4442543437845,
132.036783194096)) ;
#116784=CARTESIAN_POINT('Ctrl Pts',(-14.8636402089109,13.1766944137287,
132.061867124773)) ;
#116785=CARTESIAN_POINT('Ctrl Pts',(-14.9067034374907,12.9234094680339,
132.154300428)) ;
#116786=CARTESIAN_POINT('Ctrl Pts',(-14.9698154804404,12.7086523131788,
132.305653046529)) ;
#116787=CARTESIAN_POINT('Ctrl Pts',(-15.0493208194513,12.5444332770708,
132.504896693896)) ;
#116788=CARTESIAN_POINT('Ctrl Pts',(-15.1413379063356,12.442265427868,132.740384202576)) ;
#116789=CARTESIAN_POINT('Ctrl Pts',(-15.2383898734991,12.4113238221151,
132.990859260472)) ;
#116790=CARTESIAN_POINT('Ctrl Pts',(-15.3350927075092,12.4521999804418,
133.240286707603)) ;
#116791=CARTESIAN_POINT('Ctrl Pts',(-15.4257173250681,12.5635389839908,
133.471744679301)) ;
#116792=CARTESIAN_POINT('Ctrl Pts',(-15.5032411736603,12.7354102486573,
133.665205731719)) ;
#116793=CARTESIAN_POINT('Ctrl Pts',(-15.5638610806042,12.9568497903179,
133.809176375546)) ;
#116794=CARTESIAN_POINT('Ctrl Pts',(-15.6036470774416,13.2117694204113,
133.892283046633)) ;
#116795=CARTESIAN_POINT('Ctrl Pts',(-15.6204942624616,13.4825284434545,
133.908293488513)) ;
#116796=CARTESIAN_POINT('Ctrl Pts',(-15.6137728672592,13.7484828360667,
133.855517701894)) ;
#116797=CARTESIAN_POINT('Ctrl Pts',(-15.5850166523139,13.990067054495,133.738525504946)) ;
#116798=CARTESIAN_POINT('Ctrl Pts',(-15.536763965292,14.1922208547519,133.564439930301)) ;
#116799=CARTESIAN_POINT('Ctrl Pts',(-15.4730487748542,14.3393855053723,
133.34511245468)) ;
#116800=CARTESIAN_POINT('Ctrl Pts',(-15.399695343259,14.42040771759,133.09778751226)) ;
#116801=CARTESIAN_POINT('Ctrl Pts',(-15.3221538787493,14.4304302239803,
132.838134252815)) ;
#116802=CARTESIAN_POINT('Ctrl Pts',(-15.2467193227142,14.3678711876826,
132.58455206021)) ;
#116803=CARTESIAN_POINT('Ctrl Pts',(-15.1799138507876,14.2376928211799,
132.356266335115)) ;
#116804=CARTESIAN_POINT('Ctrl Pts',(-15.1270449347704,14.0489884118596,
132.168670045221)) ;
#116805=CARTESIAN_POINT('Ctrl Pts',(-15.0927077016124,13.8164457415788,
132.035344800608)) ;
#116806=CARTESIAN_POINT('Ctrl Pts',(-15.0799009992238,13.5541090228178,
131.964694386055)) ;
#116807=CARTESIAN_POINT('Ctrl Pts',(-15.0903290157032,13.2846773793449,
131.962212925334)) ;
#116808=CARTESIAN_POINT('Ctrl Pts',(-15.1240864041073,13.0230236388571,
132.02761116478)) ;
#116809=CARTESIAN_POINT('Ctrl Pts',(-15.1793905460716,12.7908728134741,
132.156056831622)) ;
#116810=CARTESIAN_POINT('Ctrl Pts',(-15.2530252671634,12.6038718896903,
132.338032999174)) ;
#116811=CARTESIAN_POINT('Ctrl Pts',(-15.3404395281791,12.4755978547321,
132.560270582577)) ;
#116812=CARTESIAN_POINT('Ctrl Pts',(-15.4361666301176,12.4151865518673,
132.806771124844)) ;
#116813=CARTESIAN_POINT('Ctrl Pts',(-15.5338464527214,12.4270410419496,
133.059031997262)) ;
#116814=CARTESIAN_POINT('Ctrl Pts',(-15.6273514722291,12.5098502218198,
133.299118129625)) ;
#116815=CARTESIAN_POINT('Ctrl Pts',(-15.7111748136664,12.6589865553575,
133.510736241021)) ;
#116816=CARTESIAN_POINT('Ctrl Pts',(-15.7790199467508,12.8615686437882,
133.675932015432)) ;
#116817=CARTESIAN_POINT('Ctrl Pts',(-15.8277028915331,13.1050265779988,
133.785011642684)) ;
#116818=CARTESIAN_POINT('Ctrl Pts',(-15.854027088166,13.3718443264194,133.828716982132)) ;
#116819=CARTESIAN_POINT('Ctrl Pts',(-15.856910626616,13.6411903783996,133.804094970037)) ;
#116820=CARTESIAN_POINT('Ctrl Pts',(-15.8366684723925,13.896863473321,133.711645717659)) ;
#116821=CARTESIAN_POINT('Ctrl Pts',(-15.7960112831063,14.1159779541294,
133.559939274363)) ;
#116822=CARTESIAN_POINT('Ctrl Pts',(-15.737913899012,14.287325692981,133.356994933494)) ;
#116823=CARTESIAN_POINT('Ctrl Pts',(-15.6678321119962,14.3958947357892,
133.119202977711)) ;
#116824=CARTESIAN_POINT('Ctrl Pts',(-15.5912113430045,14.435126510394,132.862258941414)) ;
#116825=CARTESIAN_POINT('Ctrl Pts',(-15.5143394894088,14.4019578679091,
132.604594883037)) ;
#116826=CARTESIAN_POINT('Ctrl Pts',(-15.4432379820011,14.298265208763,132.363682618734)) ;
#116827=CARTESIAN_POINT('Ctrl Pts',(-15.3842287146298,14.1324802055206,
132.158250825652)) ;
#116828=CARTESIAN_POINT('Ctrl Pts',(-15.3417783503285,13.915462828794,132.001092130861)) ;
#116829=CARTESIAN_POINT('Ctrl Pts',(-15.319910313068,13.663371252365,131.904098346542)) ;
#116830=CARTESIAN_POINT('Ctrl Pts',(-15.320806233112,13.3940849584222,131.873601342427)) ;
#116831=CARTESIAN_POINT('Ctrl Pts',(-15.3452532949719,13.1263052968225,
131.911831826463)) ;
#116832=CARTESIAN_POINT('Ctrl Pts',(-15.3921146290371,12.8804158989885,
132.015615977984)) ;
#116833=CARTESIAN_POINT('Ctrl Pts',(-15.4587394301298,12.6733663230833,
132.177140209864)) ;
#116834=CARTESIAN_POINT('Ctrl Pts',(-15.5412767697681,12.5197379443073,
132.385092289547)) ;
#116835=CARTESIAN_POINT('Ctrl Pts',(-15.6343686383594,12.4310982287018,
132.623899504288)) ;
#116836=CARTESIAN_POINT('Ctrl Pts',(-15.7318070432573,12.413462824637,132.875502765111)) ;
#116837=CARTESIAN_POINT('Ctrl Pts',(-15.8280059948747,12.4679867146693,
133.123364071303)) ;
#116838=CARTESIAN_POINT('Ctrl Pts',(-15.916556151159,12.5916525071464,133.348810603495)) ;
#116839=CARTESIAN_POINT('Ctrl Pts',(-15.9911124965925,12.773468390421,133.533647244235)) ;
#116840=CARTESIAN_POINT('Ctrl Pts',(-16.0481519771809,13.0028687582652,
133.667100411234)) ;
#116841=CARTESIAN_POINT('Ctrl Pts',(-16.0837269854642,13.2619623581497,
133.737923863175)) ;
#116842=CARTESIAN_POINT('Ctrl Pts',(-16.0961062506615,13.5340191309755,
133.740804033784)) ;
#116843=CARTESIAN_POINT('Ctrl Pts',(-16.0851567800789,13.7955674320649,
133.675865201536)) ;
#116844=CARTESIAN_POINT('Ctrl Pts',(-16.0523419685841,14.0322612851413,
133.546816470338)) ;
#116845=CARTESIAN_POINT('Ctrl Pts',(-16.0009018123364,14.22438976877,133.363495292219)) ;
#116846=CARTESIAN_POINT('Ctrl Pts',(-15.9350335261451,14.3598900784348,
133.137935317501)) ;
#116847=CARTESIAN_POINT('Ctrl Pts',(-15.859872027803,14.4280176148554,132.885075302892)) ;
#116848=CARTESIAN_POINT('Ctrl Pts',(-15.782828331798,14.4241023882727,132.627114452723)) ;
#116849=CARTESIAN_POINT('Ctrl Pts',(-15.7083163890521,14.3482280503466,
132.376135467847)) ;
#116850=CARTESIAN_POINT('Ctrl Pts',(-15.6438258833221,14.206072490763,132.154635276503)) ;
#116851=CARTESIAN_POINT('Ctrl Pts',(-15.5942900234776,14.008680924911,131.976908199774)) ;
#116852=CARTESIAN_POINT('Ctrl Pts',(-15.5636932851511,13.7691472453329,
131.85444476612)) ;
#116853=CARTESIAN_POINT('Ctrl Pts',(-15.555160472364,13.5031161765621,131.796227500216)) ;
#116854=CARTESIAN_POINT('Ctrl Pts',(-15.5701873565133,13.2327334709729,
131.807010775747)) ;
#116855=CARTESIAN_POINT('Ctrl Pts',(-15.6080409619239,12.9767767271815,
131.884582975432)) ;
#116856=CARTESIAN_POINT('Ctrl Pts',(-15.6670437728799,12.7518157779669,
132.023824499167)) ;
#116857=CARTESIAN_POINT('Ctrl Pts',(-15.743706872708,12.5749030821108,132.214630826275)) ;
#116858=CARTESIAN_POINT('Ctrl Pts',(-15.8331256984323,12.4587258790909,
132.442721035975)) ;
#116859=CARTESIAN_POINT('Ctrl Pts',(-15.9300951754384,12.4118884075951,
132.692727681813)) ;
#116860=CARTESIAN_POINT('Ctrl Pts',(-16.0268131871302,12.4371447896242,
132.942408691455)) ;
#116861=CARTESIAN_POINT('Ctrl Pts',(-16.1194581635705,12.5335140110472,
133.17975745332)) ;
#116862=CARTESIAN_POINT('Ctrl Pts',(-16.2002006821098,12.6929505579163,
133.382601408039)) ;
#116863=CARTESIAN_POINT('Ctrl Pts',(-16.2650587042151,12.9053983605441,
133.538877628518)) ;
#116864=CARTESIAN_POINT('Ctrl Pts',(-16.3094994650075,13.1539498809503,
133.635663755891)) ;
#116865=CARTESIAN_POINT('Ctrl Pts',(-16.3314782918866,13.4226750852024,
133.666703127002)) ;
#116866=CARTESIAN_POINT('Ctrl Pts',(-16.3299479186378,13.6910891488428,
133.629119729191)) ;
#116867=CARTESIAN_POINT('Ctrl Pts',(-16.3055899550518,13.9413684449187,
133.524691151503)) ;
#116868=CARTESIAN_POINT('Ctrl Pts',(-16.2613018501774,14.1526799175884,
133.362307720818)) ;
#116869=CARTESIAN_POINT('Ctrl Pts',(-16.200685666699,14.3125333365339,133.152120048597)) ;
#116870=CARTESIAN_POINT('Ctrl Pts',(-16.1289337339076,14.4088194545048,
132.909435999603)) ;
#116871=CARTESIAN_POINT('Ctrl Pts',(-16.0512902573569,14.4343198922647,
132.649294671372)) ;
#116872=CARTESIAN_POINT('Ctrl Pts',(-15.9755688396631,14.3877722216923,
132.395208079009)) ;
#116873=CARTESIAN_POINT('Ctrl Pts',(-15.905996220698,14.2711471229662,132.158630019206)) ;
#116874=CARTESIAN_POINT('Ctrl Pts',(-15.8499964373459,14.0951743050547,
131.962092155261)) ;
#116875=CARTESIAN_POINT('Ctrl Pts',(-15.8111145068756,13.870335406886,131.815355861608)) ;
#116876=CARTESIAN_POINT('Ctrl Pts',(-15.7933948348918,13.6128359937758,
131.730391952872)) ;
#116877=CARTESIAN_POINT('Ctrl Pts',(-15.798756317796,13.3431053830175,131.71301861056)) ;
#116878=CARTESIAN_POINT('Ctrl Pts',(-15.8274126253614,13.0784070527184,
131.763618606217)) ;
#116879=CARTESIAN_POINT('Ctrl Pts',(-15.8785782774498,12.8371326222925,
131.879774862779)) ;
#116880=CARTESIAN_POINT('Ctrl Pts',(-15.9483653149359,12.6399916348322,
132.050644310464)) ;
#116881=CARTESIAN_POINT('Ctrl Pts',(-16.0331828514141,12.4979353055065,
132.265299850434)) ;
#116882=CARTESIAN_POINT('Ctrl Pts',(-16.1278387494795,12.4220838760127,
132.508600246006)) ;
#116883=CARTESIAN_POINT('Ctrl Pts',(-16.2257839895642,12.4184701174221,
132.761571575606)) ;
#116884=CARTESIAN_POINT('Ctrl Pts',(-16.3203051085462,12.4860424298892,
133.004761298642)) ;
#116885=CARTESIAN_POINT('Ctrl Pts',(-16.4067012578865,12.6212969688775,
133.223947844078)) ;
#116886=CARTESIAN_POINT('Ctrl Pts',(-16.4784451122272,12.8133838986541,
133.400475111834)) ;
#116887=CARTESIAN_POINT('Ctrl Pts',(-16.5317455281392,13.0503648242526,
133.522937144078)) ;
#116888=CARTESIAN_POINT('Ctrl Pts',(-16.562904036609,13.3123036510868,133.58095920928)) ;
#116889=CARTESIAN_POINT('Ctrl Pts',(-16.5709394990535,13.583277796962,133.571284430359)) ;
#116890=CARTESIAN_POINT('Ctrl Pts',(-16.5556961065435,13.8428842825667,
133.493592881486)) ;
#116891=CARTESIAN_POINT('Ctrl Pts',(-16.5191174489348,14.0720012464851,
133.353626853518)) ;
#116892=CARTESIAN_POINT('Ctrl Pts',(-16.4645826787132,14.2546155052048,
133.16122511799)) ;
#116893=CARTESIAN_POINT('Ctrl Pts',(-16.3965867046521,14.3779471220683,
132.929452933279)) ;
#116894=CARTESIAN_POINT('Ctrl Pts',(-16.3207208376577,14.43277854508,132.674661781709)) ;
#116895=CARTESIAN_POINT('Ctrl Pts',(-16.2433872066106,14.415204860474,132.415650965892)) ;
#116896=CARTESIAN_POINT('Ctrl Pts',(-16.1706126792223,14.3266409888288,
132.169926667865)) ;
#116897=CARTESIAN_POINT('Ctrl Pts',(-16.1083393228608,14.1729215219676,
131.954821567221)) ;
#116898=CARTESIAN_POINT('Ctrl Pts',(-16.0620759324473,13.9662155734193,
131.786622134201)) ;
#116899=CARTESIAN_POINT('Ctrl Pts',(-16.0354545331854,13.7208187019913,
131.675794589115)) ;
#116900=CARTESIAN_POINT('Ctrl Pts',(-16.031310568843,13.4521886901424,131.630394366892)) ;
#116901=CARTESIAN_POINT('Ctrl Pts',(-16.0506012298629,13.1838897555981,
131.653758282559)) ;
#116902=CARTESIAN_POINT('Ctrl Pts',(-16.092732570887,12.9313138708941,131.743671378859)) ;
#116903=CARTESIAN_POINT('Ctrl Pts',(-16.1554610604641,12.7142071151624,
131.893770222467)) ;
#116904=CARTESIAN_POINT('Ctrl Pts',(-16.2347719855931,12.548182284736,132.092377316928)) ;
#116905=CARTESIAN_POINT('Ctrl Pts',(-16.3260094928037,12.4445945488069,
132.325771295417)) ;
#116906=CARTESIAN_POINT('Ctrl Pts',(-16.423061481813,12.4110615295413,132.576214245398)) ;
#116907=CARTESIAN_POINT('Ctrl Pts',(-16.5203214945035,12.4502003407784,
132.827110054199)) ;
#116908=CARTESIAN_POINT('Ctrl Pts',(-16.6105992456112,12.558798155004,133.057786090289)) ;
#116909=CARTESIAN_POINT('Ctrl Pts',(-16.6888731564621,12.7290992906361,
133.253347731538)) ;
#116910=CARTESIAN_POINT('Ctrl Pts',(-16.750323465089,12.9505642772134,133.399574934352)) ;
#116911=CARTESIAN_POINT('Ctrl Pts',(-16.7905447407979,13.2039533601212,
133.484067750218)) ;
#116912=CARTESIAN_POINT('Ctrl Pts',(-16.808103774948,13.4737768024146,133.502245809363)) ;
#116913=CARTESIAN_POINT('Ctrl Pts',(-16.8021327956016,13.7408243075777,
133.451586700857)) ;
#116914=CARTESIAN_POINT('Ctrl Pts',(-16.7737748215047,13.984382806197,133.335598519286)) ;
#116915=CARTESIAN_POINT('Ctrl Pts',(-16.7262493219245,14.1867700036955,
133.163813020196)) ;
#116916=CARTESIAN_POINT('Ctrl Pts',(-16.6628687750783,14.3360222992997,
132.945422090007)) ;
#116917=CARTESIAN_POINT('Ctrl Pts',(-16.5897103505964,14.419030482185,132.698666801288)) ;
#116918=CARTESIAN_POINT('Ctrl Pts',(-16.51221019719,14.4311357445316,132.43913622336)) ;
#116919=CARTESIAN_POINT('Ctrl Pts',(-16.4367353245665,14.3708888244175,
132.185495743383)) ;
#116920=CARTESIAN_POINT('Ctrl Pts',(-16.3694821265528,14.242292745065,131.955833156551)) ;
#116921=CARTESIAN_POINT('Ctrl Pts',(-16.3163383080254,14.0562620175223,
131.767605594611)) ;
#116922=CARTESIAN_POINT('Ctrl Pts',(-16.2811251005187,13.8231737937943,
131.631475169058)) ;
#116923=CARTESIAN_POINT('Ctrl Pts',(-16.2677486292964,13.5622217788933,
131.559277105701)) ;
#116924=CARTESIAN_POINT('Ctrl Pts',(-16.2774948188854,13.2923511462151,
131.554743523811)) ;
#116925=CARTESIAN_POINT('Ctrl Pts',(-16.3104849708693,13.0307857162003,
131.617989399722)) ;
#116926=CARTESIAN_POINT('Ctrl Pts',(-16.365373545646,12.7967159869363,131.745103480781)) ;
#116927=CARTESIAN_POINT('Ctrl Pts',(-16.4385204924337,12.6083943270826,
131.925677858349)) ;
#116928=CARTESIAN_POINT('Ctrl Pts',(-16.5257030828109,12.4782667432663,
132.147207427787)) ;
#116929=CARTESIAN_POINT('Ctrl Pts',(-16.6209595515756,12.4160107733854,
132.392442931131)) ;
#116930=CARTESIAN_POINT('Ctrl Pts',(-16.7189196059942,12.425588900326,132.645438963958)) ;
#116931=CARTESIAN_POINT('Ctrl Pts',(-16.812966966938,12.5070742961233,132.886977697143)) ;
#116932=CARTESIAN_POINT('Ctrl Pts',(-16.8967106834322,12.6538727227807,
133.098529303095)) ;
#116933=CARTESIAN_POINT('Ctrl Pts',(-16.965192001625,12.8553498973186,133.265526413072)) ;
#116934=CARTESIAN_POINT('Ctrl Pts',(-17.0144739641916,13.0981033261267,
133.376337583619)) ;
#116935=CARTESIAN_POINT('Ctrl Pts',(-17.0414310098506,13.3649637765944,
133.421842396641)) ;
#116936=CARTESIAN_POINT('Ctrl Pts',(-17.0448923056262,13.6334093866667,
133.3990331273)) ;
#116937=CARTESIAN_POINT('Ctrl Pts',(-17.0255067032329,13.8886868084012,
133.309248012564)) ;
#116938=CARTESIAN_POINT('Ctrl Pts',(-16.9852265152679,14.1104518117265,
133.158447905506)) ;
#116939=CARTESIAN_POINT('Ctrl Pts',(-16.9275341963761,14.2832226170572,
132.956697371245)) ;
#116940=CARTESIAN_POINT('Ctrl Pts',(-16.8577706859408,14.3937886197238,
132.719848790466)) ;
#116941=CARTESIAN_POINT('Ctrl Pts',(-16.78089628133,14.4350213819736,132.462014367155)) ;
#116942=CARTESIAN_POINT('Ctrl Pts',(-16.7043149562872,14.4038716569565,
132.205357182892)) ;
#116943=CARTESIAN_POINT('Ctrl Pts',(-16.6328354464211,14.3020574397598,
131.963287583542)) ;
#116944=CARTESIAN_POINT('Ctrl Pts',(-16.5734391248213,14.1377082667359,
131.756716566826)) ;
#116945=CARTESIAN_POINT('Ctrl Pts',(-16.5305427209279,13.922512079821,131.598336680433)) ;
#116946=CARTESIAN_POINT('Ctrl Pts',(-16.507982405518,13.6705375109782,131.499234166552)) ;
#116947=CARTESIAN_POINT('Ctrl Pts',(-16.5082708749943,13.4018845306058,
131.467013585173)) ;
#116948=CARTESIAN_POINT('Ctrl Pts',(-16.5319013398505,13.1344381767143,
131.502948161611)) ;
#116949=CARTESIAN_POINT('Ctrl Pts',(-16.5783956200005,12.8864833216457,
131.605492726989)) ;
#116950=CARTESIAN_POINT('Ctrl Pts',(-16.6441694983151,12.6791960458196,
131.764705926375)) ;
#116951=CARTESIAN_POINT('Ctrl Pts',(-16.726432219592,12.5233811558849,131.971789575967)) ;
#116952=CARTESIAN_POINT('Ctrl Pts',(-16.819171376903,12.4327816680599,132.209612016199)) ;
#116953=CARTESIAN_POINT('Ctrl Pts',(-16.9168669847768,12.412915954978,132.461862014984)) ;
#116954=CARTESIAN_POINT('Ctrl Pts',(-17.0130810554034,12.4655032606852,
132.709804508519)) ;
#116955=CARTESIAN_POINT('Ctrl Pts',(-17.1016552917455,12.5866528980437,
132.935438549739)) ;
#116956=CARTESIAN_POINT('Ctrl Pts',(-17.1770183654666,12.7674395130523,
133.122503206209)) ;
#116957=CARTESIAN_POINT('Ctrl Pts',(-17.2347578061268,12.996680662144,133.257885737137)) ;
#116958=CARTESIAN_POINT('Ctrl Pts',(-17.2707418868054,13.2541240952596,
133.33004341912)) ;
#116959=CARTESIAN_POINT('Ctrl Pts',(-17.2838680119121,13.5248420441081,
133.335259727289)) ;
#116960=CARTESIAN_POINT('Ctrl Pts',(-17.2736087985316,13.7882270430707,
133.272175979222)) ;
#116961=CARTESIAN_POINT('Ctrl Pts',(-17.2413405150168,14.026098281457,133.144700506367)) ;
#116962=CARTESIAN_POINT('Ctrl Pts',(-17.1902557486675,14.220023125983,132.962349683833)) ;
#116963=CARTESIAN_POINT('Ctrl Pts',(-17.12483319593,14.3567721922805,132.738164016465)) ;
#116964=CARTESIAN_POINT('Ctrl Pts',(-17.0503040398658,14.4269174319569,
132.487342101643)) ;
#116965=CARTESIAN_POINT('Ctrl Pts',(-16.972658858244,14.4252573107259,132.22736950121)) ;
#116966=CARTESIAN_POINT('Ctrl Pts',(-16.8981739750149,14.3512845156984,
131.976555512661)) ;
#116967=CARTESIAN_POINT('Ctrl Pts',(-16.8335398285555,14.2117350890935,
131.754763421916)) ;
#116968=CARTESIAN_POINT('Ctrl Pts',(-16.7832370832045,14.0152549017169,
131.574673760724)) ;
#116969=CARTESIAN_POINT('Ctrl Pts',(-16.7520262621574,13.7756400409677,
131.450290290216)) ;
#116970=CARTESIAN_POINT('Ctrl Pts',(-16.7428846424837,13.512293601297,131.390573199531)) ;
#116971=CARTESIAN_POINT('Ctrl Pts',(-16.7571174189924,13.24113011058,131.398952116168)) ;
#116972=CARTESIAN_POINT('Ctrl Pts',(-16.7943670713977,12.9839533998787,
131.474699240851)) ;
#116973=CARTESIAN_POINT('Ctrl Pts',(-16.8530367769723,12.757224045122,131.612859940048)) ;
#116974=CARTESIAN_POINT('Ctrl Pts',(-16.9289336870903,12.5794741736853,
131.801571530647)) ;
#116975=CARTESIAN_POINT('Ctrl Pts',(-17.0182778782105,12.4611210903509,
132.029356074653)) ;
#116976=CARTESIAN_POINT('Ctrl Pts',(-17.1146160701368,12.4122668276836,
132.277695181808)) ;
#116977=CARTESIAN_POINT('Ctrl Pts',(-17.2121033058066,12.4354395008957,
132.529381521733)) ;
#116978=CARTESIAN_POINT('Ctrl Pts',(-17.3049234321536,12.5301694700227,
132.767254707327)) ;
#116979=CARTESIAN_POINT('Ctrl Pts',(-17.3858637794653,12.6876686468163,
132.970742976347)) ;
#116980=CARTESIAN_POINT('Ctrl Pts',(-17.4511566609569,12.8982124507683,
133.128366185446)) ;
#116981=CARTESIAN_POINT('Ctrl Pts',(-17.4964430877249,13.1472879171854,
133.227443906338)) ;
#116982=CARTESIAN_POINT('Ctrl Pts',(-17.5189530226261,13.4151706330379,
133.260112246192)) ;
#116983=CARTESIAN_POINT('Ctrl Pts',(-17.5180772977572,13.6833052761831,
133.224500236615)) ;
#116984=CARTESIAN_POINT('Ctrl Pts',(-17.494562648909,13.9335262221531,133.122676890144)) ;
#116985=CARTESIAN_POINT('Ctrl Pts',(-17.4504518079917,14.1479664879784,
132.960528520529)) ;
#116986=CARTESIAN_POINT('Ctrl Pts',(-17.3903547316673,14.3087959148104,
132.751961242652)) ;
#116987=CARTESIAN_POINT('Ctrl Pts',(-17.3188588627773,14.4069520206095,
132.510023786694)) ;
#116988=CARTESIAN_POINT('Ctrl Pts',(-17.2416470088105,14.4347039368911,
132.251304094887)) ;
#116989=CARTESIAN_POINT('Ctrl Pts',(-17.1652862735102,14.3899170830749,
131.995115519734)) ;
#116990=CARTESIAN_POINT('Ctrl Pts',(-17.0958542528533,14.2758481997907,
131.759156683175)) ;
#116991=CARTESIAN_POINT('Ctrl Pts',(-17.0391474079491,14.1010294693846,
131.560425945483)) ;
#116992=CARTESIAN_POINT('Ctrl Pts',(-16.9997289321043,13.8772034754541,
131.412115133594)) ;
#116993=CARTESIAN_POINT('Ctrl Pts',(-16.9813814044527,13.6206147826081,
131.325344173753)) ;
#116994=CARTESIAN_POINT('Ctrl Pts',(-16.9860373202625,13.3509222115741,
131.305902124102)) ;
#116995=CARTESIAN_POINT('Ctrl Pts',(-17.0141429076236,13.0853829719641,
131.354833697986)) ;
#116996=CARTESIAN_POINT('Ctrl Pts',(-17.0643516475666,12.8445476848772,
131.468399606912)) ;
#116997=CARTESIAN_POINT('Ctrl Pts',(-17.1338580586174,12.644952930344,131.638309780535)) ;
#116998=CARTESIAN_POINT('Ctrl Pts',(-17.2183241864262,12.5012606918104,
131.851948185352)) ;
#116999=CARTESIAN_POINT('Ctrl Pts',(-17.3124481152622,12.4235056732711,
132.09380438388)) ;
#117000=CARTESIAN_POINT('Ctrl Pts',(-17.4104141135003,12.417318606479,132.346827753117)) ;
#117001=CARTESIAN_POINT('Ctrl Pts',(-17.5056867648447,12.4833714427519,
132.592005351237)) ;
#117002=CARTESIAN_POINT('Ctrl Pts',(-17.5919987183341,12.6162285125256,
132.811106229032)) ;
#117003=CARTESIAN_POINT('Ctrl Pts',(-17.6644873151439,12.8073409623945,
132.989699975671)) ;
#117004=CARTESIAN_POINT('Ctrl Pts',(-17.7183030404906,13.0432164497969,
133.113690694589)) ;
#117005=CARTESIAN_POINT('Ctrl Pts',(-17.7501392643195,13.3046948495717,
133.173683613056)) ;
#117006=CARTESIAN_POINT('Ctrl Pts',(-17.7588282011811,13.5764462618644,
133.165829921335)) ;
#117007=CARTESIAN_POINT('Ctrl Pts',(-17.7441367232311,13.8363549423102,
133.089774039034)) ;
#117008=CARTESIAN_POINT('Ctrl Pts',(-17.7083001328226,14.0655921172455,
132.952119497934)) ;
#117009=CARTESIAN_POINT('Ctrl Pts',(-17.654103302564,14.2503953829721,132.760609433254)) ;
#117010=CARTESIAN_POINT('Ctrl Pts',(-17.5861690172399,14.3757153759899,
132.528919395928)) ;
#117011=CARTESIAN_POINT('Ctrl Pts',(-17.5105676394246,14.4321659861442,
132.274963313804)) ;
#117012=CARTESIAN_POINT('Ctrl Pts',(-17.4334463905001,14.4167343147861,
132.016680455663)) ;
#117013=CARTESIAN_POINT('Ctrl Pts',(-17.3604705956701,14.3302900075088,
131.770378332866)) ;
#117014=CARTESIAN_POINT('Ctrl Pts',(-17.297751311033,14.1784243814557,131.55396233599)) ;
#117015=CARTESIAN_POINT('Ctrl Pts',(-17.2507585604563,13.971750794682,131.38344223631)) ;
#117016=CARTESIAN_POINT('Ctrl Pts',(-17.2237636735663,13.7284357059757,
131.271702420089)) ;
#117017=CARTESIAN_POINT('Ctrl Pts',(-17.2188332794065,13.4606302027768,
131.224056001737)) ;
#117018=CARTESIAN_POINT('Ctrl Pts',(-17.2376137110836,13.190619216966,131.245741417272)) ;
#117019=CARTESIAN_POINT('Ctrl Pts',(-17.2788766995086,12.9388679934988,
131.333323569649)) ;
#117020=CARTESIAN_POINT('Ctrl Pts',(-17.3412285355925,12.7195132188822,
131.482193704822)) ;
#117021=CARTESIAN_POINT('Ctrl Pts',(-17.4203247959701,12.5518557366653,
131.680119292236)) ;
#117022=CARTESIAN_POINT('Ctrl Pts',(-17.5108708872975,12.4467157565619,
131.911647299917)) ;
#117023=CARTESIAN_POINT('Ctrl Pts',(-17.6083887104431,12.4110145774925,
132.163260737684)) ;
#117024=CARTESIAN_POINT('Ctrl Pts',(-17.7050772468256,12.4479828352211,
132.412713479872)) ;
#117025=CARTESIAN_POINT('Ctrl Pts',(-17.7958600990291,12.5544308126574,
132.644801506752)) ;
#117026=CARTESIAN_POINT('Ctrl Pts',(-17.8750216891489,12.7245572127077,
132.842729488612)) ;
#117027=CARTESIAN_POINT('Ctrl Pts',(-17.9365564723328,12.9435039801677,
132.989422242518)) ;
#117028=CARTESIAN_POINT('Ctrl Pts',(-17.9775224282541,13.1965754196772,
133.076026647285)) ;
#117029=CARTESIAN_POINT('Ctrl Pts',(-17.9956939192113,13.4658054148295,
133.09604875014)) ;
#117030=CARTESIAN_POINT('Ctrl Pts',(-17.9904317119844,13.7328709435355,
133.047502469415)) ;
#117031=CARTESIAN_POINT('Ctrl Pts',(-17.9627916507943,13.9772572574738,
132.933643191885)) ;
#117032=CARTESIAN_POINT('Ctrl Pts',(-17.9155381808679,14.1820528886268,
132.762483278514)) ;
#117033=CARTESIAN_POINT('Ctrl Pts',(-17.8525173753685,14.3328843450188,
132.545157295433)) ;
#117034=CARTESIAN_POINT('Ctrl Pts',(-17.7793317704753,14.4178010956835,
132.298223906982)) ;
#117035=CARTESIAN_POINT('Ctrl Pts',(-17.7022445272674,14.4318123970992,
132.040068999793)) ;
#117036=CARTESIAN_POINT('Ctrl Pts',(-17.6263126401448,14.3732303174577,
131.78494696794)) ;
#117037=CARTESIAN_POINT('Ctrl Pts',(-17.5591052998671,14.246970367672,131.555590267811)) ;
#117038=CARTESIAN_POINT('Ctrl Pts',(-17.5053666762276,14.0621465768449,
131.365553019795)) ;
#117039=CARTESIAN_POINT('Ctrl Pts',(-17.4696698326379,13.8305008090445,
131.228071032379)) ;
#117040=CARTESIAN_POINT('Ctrl Pts',(-17.4555867985558,13.5704782336575,
131.153845884403)) ;
#117041=CARTESIAN_POINT('Ctrl Pts',(-17.4646965033118,13.2994607453498,
131.147313037759)) ;
#117042=CARTESIAN_POINT('Ctrl Pts',(-17.4970988814655,13.0377344275702,
131.208876933298)) ;
#117043=CARTESIAN_POINT('Ctrl Pts',(-17.5510813018689,12.8036246677019,
131.333503702802)) ;
#117044=CARTESIAN_POINT('Ctrl Pts',(-17.6239936560219,12.6130123925856,
131.513267510233)) ;
#117045=CARTESIAN_POINT('Ctrl Pts',(-17.7106094314361,12.4813447985494,
131.733232511001)) ;
#117046=CARTESIAN_POINT('Ctrl Pts',(-17.8060337046778,12.4167223946536,
131.978839859878)) ;
#117047=CARTESIAN_POINT('Ctrl Pts',(-17.9038805613539,12.4243655838416,
132.231551517827)) ;
#117048=CARTESIAN_POINT('Ctrl Pts',(-17.9978748431434,12.5034382504578,
132.473028954758)) ;
#117049=CARTESIAN_POINT('Ctrl Pts',(-18.0821443467043,12.6484425830615,
132.686072200411)) ;
#117050=CARTESIAN_POINT('Ctrl Pts',(-18.1513187618018,12.8490571219356,
132.855007023695)) ;
#117051=CARTESIAN_POINT('Ctrl Pts',(-18.2011086603779,13.0907448949446,
132.967327226966)) ;
#117052=CARTESIAN_POINT('Ctrl Pts',(-18.2287179809135,13.3559777711551,
133.014884267935)) ;
#117053=CARTESIAN_POINT('Ctrl Pts',(-18.2329064963071,13.6264772467065,
132.993964165235)) ;
#117054=CARTESIAN_POINT('Ctrl Pts',(-18.2141466812409,13.8815733250424,
132.90611529719)) ;
#117055=CARTESIAN_POINT('Ctrl Pts',(-18.1744739172804,14.1045282295606,
132.757096482705)) ;
#117056=CARTESIAN_POINT('Ctrl Pts',(-18.1172408746865,14.2789670310199,
132.556695647005)) ;
#117057=CARTESIAN_POINT('Ctrl Pts',(-18.0476676879061,14.3914951662386,
132.320360288733)) ;
#117058=CARTESIAN_POINT('Ctrl Pts',(-17.9712198186188,14.4348607606962,
132.063910845682)) ;
#117059=CARTESIAN_POINT('Ctrl Pts',(-17.8941478594852,14.4056890546892,
131.805637282681)) ;
#117060=CARTESIAN_POINT('Ctrl Pts',(-17.8227454815296,14.3062653173801,
131.563950734578)) ;
#117061=CARTESIAN_POINT('Ctrl Pts',(-17.7627779364618,14.1434405254574,
131.355638920096)) ;
#117062=CARTESIAN_POINT('Ctrl Pts',(-17.7193273445083,13.9296996080406,
131.195662221209)) ;
#117063=CARTESIAN_POINT('Ctrl Pts',(-17.6960653225894,13.6772902050266,
131.094350026833)) ;
#117064=CARTESIAN_POINT('Ctrl Pts',(-17.6957248215412,13.4099497148623,
131.060430155186)) ;
#117065=CARTESIAN_POINT('Ctrl Pts',(-17.7187008254136,13.1418739584321,
131.094409308727)) ;
#117066=CARTESIAN_POINT('Ctrl Pts',(-17.7643612609263,12.8939990940818,
131.194650629234)) ;
#117067=CARTESIAN_POINT('Ctrl Pts',(-17.8297406925657,12.6844791174551,
131.352604596309)) ;
#117068=CARTESIAN_POINT('Ctrl Pts',(-17.912048493683,12.5265062887792,131.559667994062)) ;
#117069=CARTESIAN_POINT('Ctrl Pts',(-18.0040939259134,12.4345049990361,
131.795636342437)) ;
#117070=CARTESIAN_POINT('Ctrl Pts',(-18.1020496484601,12.4124896095147,
132.048536521904)) ;
#117071=CARTESIAN_POINT('Ctrl Pts',(-18.1979840618264,12.4629154785975,
132.295801289656)) ;
#117072=CARTESIAN_POINT('Ctrl Pts',(-18.2870505883933,12.5820912201831,
132.5228214314)) ;
#117073=CARTESIAN_POINT('Ctrl Pts',(-18.3631176317433,12.7624371254393,
132.71179031039)) ;
#117074=CARTESIAN_POINT('Ctrl Pts',(-18.4208520067614,12.9881391647597,
132.847502465823)) ;
#117075=CARTESIAN_POINT('Ctrl Pts',(-18.4578512180896,13.2462582186001,
132.922435272868)) ;
#117076=CARTESIAN_POINT('Ctrl Pts',(-18.4715963342929,13.5176870879671,
132.929369118207)) ;
#117077=CARTESIAN_POINT('Ctrl Pts',(-18.4620156422079,13.7805943652363,
132.86838448577)) ;
#117078=CARTESIAN_POINT('Ctrl Pts',(-18.4303896901905,14.0195268693382,
132.742785403874)) ;
#117079=CARTESIAN_POINT('Ctrl Pts',(-18.3798066675688,14.2150384579935,
132.561895383621)) ;
#117080=CARTESIAN_POINT('Ctrl Pts',(-18.3145812893689,14.3538332405852,
132.338211899335)) ;
#117081=CARTESIAN_POINT('Ctrl Pts',(-18.2403139322017,14.4259646788893,
132.088197467506)) ;
#117082=CARTESIAN_POINT('Ctrl Pts',(-18.1623800872695,14.4260802935488,
131.827250512301)) ;
#117083=CARTESIAN_POINT('Ctrl Pts',(-18.0883879084288,14.3549351031628,
131.578187846455)) ;
#117084=CARTESIAN_POINT('Ctrl Pts',(-18.0228131840017,14.2162529727103,
131.353366204512)) ;
#117085=CARTESIAN_POINT('Ctrl Pts',(-17.9722305417751,14.0213157651239,
131.1725299858)) ;
#117086=CARTESIAN_POINT('Ctrl Pts',(-17.9404225452434,13.7835943457729,
131.046506253201)) ;
#117087=CARTESIAN_POINT('Ctrl Pts',(-17.9306274462144,13.5186609566866,
130.984624399545)) ;
#117088=CARTESIAN_POINT('Ctrl Pts',(-17.9441208496999,13.2494163240999,
130.991097001359)) ;
#117089=CARTESIAN_POINT('Ctrl Pts',(-17.9809055295072,12.9903692068144,
131.065315650557)) ;
#117090=CARTESIAN_POINT('Ctrl Pts',(-18.0386552877696,12.7636901200826,
131.200984817336)) ;
#117091=CARTESIAN_POINT('Ctrl Pts',(-18.1148239173405,12.5829314316244,
131.390184918453)) ;
#117092=CARTESIAN_POINT('Ctrl Pts',(-18.2029461040862,12.4640788592141,
131.614759525871)) ;
#117093=CARTESIAN_POINT('Ctrl Pts',(-18.2996827120523,12.4125693600516,
131.864067074982)) ;
#117094=CARTESIAN_POINT('Ctrl Pts',(-18.3969100719483,12.433709410136,132.115106582706)) ;
#117095=CARTESIAN_POINT('Ctrl Pts',(-18.4900732804124,12.5263145122891,
132.353948507972)) ;
#117096=CARTESIAN_POINT('Ctrl Pts',(-18.5714958868613,12.682258725893,132.558814736945)) ;
#117097=CARTESIAN_POINT('Ctrl Pts',(-18.6373162617473,12.8915625393506,
132.717968364611)) ;
#117098=CARTESIAN_POINT('Ctrl Pts',(-18.6831779936634,13.1392602988437,
132.818793451197)) ;
#117099=CARTESIAN_POINT('Ctrl Pts',(-18.7064268279725,13.4076118605944,
132.85351971411)) ;
#117100=CARTESIAN_POINT('Ctrl Pts',(-18.7062530712832,13.6757335665798,
132.820002437843)) ;
#117101=CARTESIAN_POINT('Ctrl Pts',(-18.683078950832,13.9281677275871,132.718953226837)) ;
#117102=CARTESIAN_POINT('Ctrl Pts',(-18.640099263916,14.1410411517753,132.560560995141)) ;
#117103=CARTESIAN_POINT('Ctrl Pts',(-18.5800582899644,14.305185990512,132.35189900218)) ;
#117104=CARTESIAN_POINT('Ctrl Pts',(-18.5088109665702,14.4050577723151,
132.110709800884)) ;
#117105=CARTESIAN_POINT('Ctrl Pts',(-18.4315948961661,14.4349188595374,
131.851939151734)) ;
#117106=CARTESIAN_POINT('Ctrl Pts',(-18.355263243623,14.3922309403959,131.59589764855)) ;
#117107=CARTESIAN_POINT('Ctrl Pts',(-18.2855600543647,14.2801808361509,
131.359153670221)) ;
#117108=CARTESIAN_POINT('Ctrl Pts',(-18.2283588377964,14.1070360328529,
131.158971852626)) ;
#117109=CARTESIAN_POINT('Ctrl Pts',(-18.1882743461536,13.8833119932821,
131.0085695641)) ;
#117110=CARTESIAN_POINT('Ctrl Pts',(-18.1694035223355,13.6288342780485,
130.920460577913)) ;
#117111=CARTESIAN_POINT('Ctrl Pts',(-18.1733769016791,13.3582466690145,
130.898891973089)) ;
#117112=CARTESIAN_POINT('Ctrl Pts',(-18.2007660526155,13.0930922580285,
130.945833159448)) ;
#117113=CARTESIAN_POINT('Ctrl Pts',(-18.2504018512957,12.8509541830077,
131.057680258634)) ;
#117114=CARTESIAN_POINT('Ctrl Pts',(-18.3193746459451,12.6500625833759,
131.226050457482)) ;
#117115=CARTESIAN_POINT('Ctrl Pts',(-18.4036036450366,12.504322047528,131.438944253351)) ;
#117116=CARTESIAN_POINT('Ctrl Pts',(-18.4977132388811,12.4246931678785,
131.680702606203)) ;
#117117=CARTESIAN_POINT('Ctrl Pts',(-18.5951599185754,12.416496187653,131.932378104325)) ;
#117118=CARTESIAN_POINT('Ctrl Pts',(-18.6906647519872,12.4802513742885,
132.178216477564)) ;
#117119=CARTESIAN_POINT('Ctrl Pts',(-18.7775446534296,12.6116452281821,
132.398888779547)) ;
#117120=CARTESIAN_POINT('Ctrl Pts',(-18.8503971402191,12.8011771463769,
132.578577969436)) ;
#117121=CARTESIAN_POINT('Ctrl Pts',(-18.9046822847444,13.0350449035092,
132.704058615265)) ;
#117122=CARTESIAN_POINT('Ctrl Pts',(-18.9373366903773,13.2969779492496,
132.766311743464)) ;
#117123=CARTESIAN_POINT('Ctrl Pts',(-18.9466739392997,13.5677345965553,
132.760477775421)) ;
#117124=CARTESIAN_POINT('Ctrl Pts',(-18.9327727327974,13.8283851031189,
132.686725578769)) ;
#117125=CARTESIAN_POINT('Ctrl Pts',(-18.8973384738624,14.0598713577401,
132.550083801221)) ;
#117126=CARTESIAN_POINT('Ctrl Pts',(-18.8437140744461,14.2455587170749,
132.360336246797)) ;
#117127=CARTESIAN_POINT('Ctrl Pts',(-18.776413111715,14.3725641249717,132.130623413319)) ;
#117128=CARTESIAN_POINT('Ctrl Pts',(-18.7007176017471,14.4315964655583,
131.876278049731)) ;
#117129=CARTESIAN_POINT('Ctrl Pts',(-18.6233791710985,14.4181824327013,
131.617286371407)) ;
#117130=CARTESIAN_POINT('Ctrl Pts',(-18.5502173289885,14.3336378405054,
131.370446907116)) ;
#117131=CARTESIAN_POINT('Ctrl Pts',(-18.4872936427762,14.1840091545094,
131.15352964314)) ;
#117132=CARTESIAN_POINT('Ctrl Pts',(-18.4397223531237,13.9789558731559,
130.981326851861)) ;
#117133=CARTESIAN_POINT('Ctrl Pts',(-18.4119775228567,13.7355808052625,
130.867265425768)) ;
#117134=CARTESIAN_POINT('Ctrl Pts',(-18.4064814941183,13.4678622499821,
130.817935896373)) ;
#117135=CARTESIAN_POINT('Ctrl Pts',(-18.4244263066341,13.1991328428123,
130.83736685991)) ;
#117136=CARTESIAN_POINT('Ctrl Pts',(-18.4652738657257,12.9452257319575,
130.923547616471)) ;
#117137=CARTESIAN_POINT('Ctrl Pts',(-18.5267424147599,12.7259341486132,
131.070029383219)) ;
#117138=CARTESIAN_POINT('Ctrl Pts',(-18.605481008747,12.5559411201038,131.266843153907)) ;
#117139=CARTESIAN_POINT('Ctrl Pts',(-18.6962817397117,12.4485460987932,
131.498939242376)) ;
#117140=CARTESIAN_POINT('Ctrl Pts',(-18.7931264919224,12.4111599413339,
131.748784863318)) ;
#117141=CARTESIAN_POINT('Ctrl Pts',(-18.8900242356404,12.4456278255399,
131.998818087739)) ;
#117142=CARTESIAN_POINT('Ctrl Pts',(-18.9817297898447,12.5514145660075,
132.233337505005)) ;
#117143=CARTESIAN_POINT('Ctrl Pts',(-19.0604119039029,12.7181519497096,
132.430234211347)) ;
#117144=CARTESIAN_POINT('Ctrl Pts',(-19.1228377309179,12.9364297066312,
132.579399304795)) ;
#117145=CARTESIAN_POINT('Ctrl Pts',(-19.1644090080696,13.1887531775189,
132.667781651634)) ;
#117146=CARTESIAN_POINT('Ctrl Pts',(-19.1833003674831,13.4580633206524,
132.689869485556)) ;
#117147=CARTESIAN_POINT('Ctrl Pts',(-19.1786680296816,13.7256377650323,
132.643143208247)) ;
#117148=CARTESIAN_POINT('Ctrl Pts',(-19.1517004243795,13.9704139197111,
132.531316059401)) ;
#117149=CARTESIAN_POINT('Ctrl Pts',(-19.104963335141,14.1767864101741,132.361645187947)) ;
#117150=CARTESIAN_POINT('Ctrl Pts',(-19.042308153427,14.3292888333563,132.145383688225)) ;
#117151=CARTESIAN_POINT('Ctrl Pts',(-18.9695876630287,14.4162418922063,
131.899913807586)) ;
#117152=CARTESIAN_POINT('Ctrl Pts',(-18.892047727718,14.4323070636622,131.640219675188)) ;
#117153=CARTESIAN_POINT('Ctrl Pts',(-18.816661183209,14.3764282690484,131.387003920178)) ;
#117154=CARTESIAN_POINT('Ctrl Pts',(-18.7486327689988,14.2515625943371,
131.155022379996)) ;
#117155=CARTESIAN_POINT('Ctrl Pts',(-18.6944668016159,14.0682229013696,
130.963752671128)) ;
#117156=CARTESIAN_POINT('Ctrl Pts',(-18.6581314611437,13.8370234728167,
130.824314562023)) ;
#117157=CARTESIAN_POINT('Ctrl Pts',(-18.6434859969042,13.5786250860868,
130.748584888107)) ;
#117158=CARTESIAN_POINT('Ctrl Pts',(-18.6518580481978,13.3076278419877,
130.739890903035)) ;
#117159=CARTESIAN_POINT('Ctrl Pts',(-18.6835647729175,13.0452574114126,
130.799415914394)) ;
#117160=CARTESIAN_POINT('Ctrl Pts',(-18.7372078222609,12.809151348438,130.922911372363)) ;
#117161=CARTESIAN_POINT('Ctrl Pts',(-18.8096004840355,12.6175516783773,
131.101207495489)) ;
#117162=CARTESIAN_POINT('Ctrl Pts',(-18.8956363694374,12.4843718423873,
131.319568496696)) ;
#117163=CARTESIAN_POINT('Ctrl Pts',(-18.9909803439723,12.417595884224,131.564908742149)) ;
#117164=CARTESIAN_POINT('Ctrl Pts',(-19.0887365409089,12.4230554793737,
131.817394766854)) ;
#117165=CARTESIAN_POINT('Ctrl Pts',(-19.1830717025105,12.5002516157562,
132.059812929187)) ;
#117166=CARTESIAN_POINT('Ctrl Pts',(-19.2674882263268,12.6429370956148,
132.273384344499)) ;
#117167=CARTESIAN_POINT('Ctrl Pts',(-19.3374842285937,12.8430358914049,
132.444563896966)) ;
#117168=CARTESIAN_POINT('Ctrl Pts',(-19.3876849067688,13.0829430235275,
132.558206408806)) ;
#117169=CARTESIAN_POINT('Ctrl Pts',(-19.4160311708763,13.3482625175679,
132.607844720929)) ;
#117170=CARTESIAN_POINT('Ctrl Pts',(-19.4209271929234,13.6179804749313,
132.589108934737)) ;
#117171=CARTESIAN_POINT('Ctrl Pts',(-19.4027272157972,13.8754577443227,
132.502681343733)) ;
#117172=CARTESIAN_POINT('Ctrl Pts',(-19.3634406682626,14.0994367889634,
132.354768976412)) ;
#117173=CARTESIAN_POINT('Ctrl Pts',(-19.3070300640894,14.2743408092093,
132.156989617184)) ;
#117174=CARTESIAN_POINT('Ctrl Pts',(-19.2375686089438,14.3892596649761,
131.920883182707)) ;
#117175=CARTESIAN_POINT('Ctrl Pts',(-19.1612777685189,14.4346258039945,
131.664916915455)) ;
#117176=CARTESIAN_POINT('Ctrl Pts',(-19.083930799282,14.4074612367265,131.405752807975)) ;
#117177=CARTESIAN_POINT('Ctrl Pts',(-19.0123391520556,14.3096987873791,
131.163518218424)) ;
#117178=CARTESIAN_POINT('Ctrl Pts',(-18.952179149292,14.1493774053066,130.954787077338)) ;
#117179=CARTESIAN_POINT('Ctrl Pts',(-18.9079902596912,13.9355628673905,
130.792452884477)) ;
#117180=CARTESIAN_POINT('Ctrl Pts',(-18.8842705546582,13.6861606086544,
130.6900983053)) ;
#117181=CARTESIAN_POINT('Ctrl Pts',(-18.8831952536651,13.4167352141788,
130.653733612536)) ;
#117182=CARTESIAN_POINT('Ctrl Pts',(-18.9055495545771,13.1492793403457,
130.686009635183)) ;
#117183=CARTESIAN_POINT('Ctrl Pts',(-18.950554370829,12.9005268822979,130.784333466505)) ;
#117184=CARTESIAN_POINT('Ctrl Pts',(-19.0154787069261,12.6897474327515,
130.940945875063)) ;
#117185=CARTESIAN_POINT('Ctrl Pts',(-19.0969861591499,12.5306016381553,
131.145821087892)) ;
#117186=CARTESIAN_POINT('Ctrl Pts',(-19.189260918282,12.4360458908817,131.382286850804)) ;
#117187=CARTESIAN_POINT('Ctrl Pts',(-19.2870091730974,12.412131814103,131.634635629436)) ;
#117188=CARTESIAN_POINT('Ctrl Pts',(-19.3832683990726,12.4605357915181,
131.882783283401)) ;
#117189=CARTESIAN_POINT('Ctrl Pts',(-19.4726990706001,12.5784164167772,
132.110813581549)) ;
#117190=CARTESIAN_POINT('Ctrl Pts',(-19.548603124899,12.75548162504,132.299596599868)) ;
#117191=CARTESIAN_POINT('Ctrl Pts',(-19.6074115970358,12.9817623745855,
132.43817522236)) ;
#117192=CARTESIAN_POINT('Ctrl Pts',(-19.6448326502932,13.2381597682889,
132.514493933174)) ;
#117193=CARTESIAN_POINT('Ctrl Pts',(-19.6593315598521,13.5101991451629,
132.523535679866)) ;
#117194=CARTESIAN_POINT('Ctrl Pts',(-19.6504054949689,13.7733130624052,
132.46450138847)) ;
#117195=CARTESIAN_POINT('Ctrl Pts',(-19.6192034341109,14.0140640637462,
132.340009177099)) ;
#117196=CARTESIAN_POINT('Ctrl Pts',(-19.5693158816681,14.2098744225724,
132.161320346302)) ;
#117197=CARTESIAN_POINT('Ctrl Pts',(-19.504529632498,14.3505801926375,131.938940974337)) ;
#117198=CARTESIAN_POINT('Ctrl Pts',(-19.4303629478852,14.4248316495575,
131.689182334829)) ;
#117199=CARTESIAN_POINT('Ctrl Pts',(-19.3525182361724,14.4272048200234,
131.428536488696)) ;
#117200=CARTESIAN_POINT('Ctrl Pts',(-19.2781506637438,14.3577939953671,
131.178279346935)) ;
#117201=CARTESIAN_POINT('Ctrl Pts',(-19.212505421794,14.2217458175161,130.953414089471)) ;
#117202=CARTESIAN_POINT('Ctrl Pts',(-19.16103693859,14.0267542055663,130.769727449748)) ;
#117203=CARTESIAN_POINT('Ctrl Pts',(-19.1289036146384,13.7911380978429,
130.642932687612)) ;
#117204=CARTESIAN_POINT('Ctrl Pts',(-19.1183510866146,13.5273991680406,
130.578912350849)) ;
#117205=CARTESIAN_POINT('Ctrl Pts',(-19.1311706870696,13.2571617641776,
130.583305514474)) ;
#117206=CARTESIAN_POINT('Ctrl Pts',(-19.1673218801738,12.9974109548792,
130.655666860345)) ;
#117207=CARTESIAN_POINT('Ctrl Pts',(-19.2245830115337,12.7695380249157,
130.789882378042)) ;
#117208=CARTESIAN_POINT('Ctrl Pts',(-19.2998473676005,12.5879937236174,
130.976618888734)) ;
#117209=CARTESIAN_POINT('Ctrl Pts',(-19.3881991229152,12.4663339906868,
131.201653000597)) ;
#117210=CARTESIAN_POINT('Ctrl Pts',(-19.4848060932389,12.41305303315,131.450591800084)) ;
#117211=CARTESIAN_POINT('Ctrl Pts',(-19.5819062292555,12.4321501041493,
131.701314973679)) ;
#117212=CARTESIAN_POINT('Ctrl Pts',(-19.675129897644,12.522410787778,131.940402492585)) ;
#117213=CARTESIAN_POINT('Ctrl Pts',(-19.7573199379753,12.677312203341,132.14736167088)) ;
#117214=CARTESIAN_POINT('Ctrl Pts',(-19.823545048816,12.8853931735732,132.307714185514)) ;
#117215=CARTESIAN_POINT('Ctrl Pts',(-19.8698643346986,13.1311434381669,
132.410014121135)) ;
#117216=CARTESIAN_POINT('Ctrl Pts',(-19.8939118774607,13.4000886870271,
132.446960025135)) ;
#117217=CARTESIAN_POINT('Ctrl Pts',(-19.8943127889844,13.667985481151,132.415168505079)) ;
#117218=CARTESIAN_POINT('Ctrl Pts',(-19.8720904633959,13.9198929118074,
132.317110124028)) ;
#117219=CARTESIAN_POINT('Ctrl Pts',(-19.8290668706825,14.13673316727,132.158155563746)) ;
#117220=CARTESIAN_POINT('Ctrl Pts',(-19.770011609999,14.300676131018,131.952727239332)) ;
#117221=CARTESIAN_POINT('Ctrl Pts',(-19.6985762425733,14.4034182516523,
131.71075647086)) ;
#117222=CARTESIAN_POINT('Ctrl Pts',(-19.6216236920745,14.4350219439221,
131.452850053903)) ;
#117223=CARTESIAN_POINT('Ctrl Pts',(-19.5450987456045,14.3943912099649,
131.196198948101)) ;
#117224=CARTESIAN_POINT('Ctrl Pts',(-19.475140036997,14.2842181242634,130.958722088422)) ;
#117225=CARTESIAN_POINT('Ctrl Pts',(-19.4175029628842,14.11233380319,130.757229002199)) ;
#117226=CARTESIAN_POINT('Ctrl Pts',(-19.3770857737604,13.8914433444145,
130.6060852262)) ;
#117227=CARTESIAN_POINT('Ctrl Pts',(-19.3573954947611,13.6364806192018,
130.515411717742)) ;
#117228=CARTESIAN_POINT('Ctrl Pts',(-19.3607065836319,13.3663281974235,
130.491948631403)) ;
#117229=CARTESIAN_POINT('Ctrl Pts',(-19.3874616050322,13.1002905199636,
130.536976005828)) ;
#117230=CARTESIAN_POINT('Ctrl Pts',(-19.4365018798327,12.8573187097229,
130.647094499789)) ;
#117231=CARTESIAN_POINT('Ctrl Pts',(-19.5049808180712,12.6550559201632,
130.814019899914)) ;
#117232=CARTESIAN_POINT('Ctrl Pts',(-19.5887535982055,12.5076995201524,
131.025617281051)) ;
#117233=CARTESIAN_POINT('Ctrl Pts',(-19.6826402090088,12.4260782231414,
131.266727526869)) ;
#117234=CARTESIAN_POINT('Ctrl Pts',(-19.780025633086,12.4155414284777,131.518242098443)) ;
#117235=CARTESIAN_POINT('Ctrl Pts',(-19.8763791576049,12.4780902528913,
131.766305681798)) ;
#117236=CARTESIAN_POINT('Ctrl Pts',(-19.9627548974109,12.6066343285888,
131.985813699722)) ;
#117237=CARTESIAN_POINT('Ctrl Pts',(-20.0364241953336,12.7952135376049,
132.167753376354)) ;
#117238=CARTESIAN_POINT('Ctrl Pts',(-20.0912151052384,13.0279818005268,
132.294735120035)) ;
#117239=CARTESIAN_POINT('Ctrl Pts',(-20.1245512603828,13.2896873731217,
132.358938550464)) ;
#117240=CARTESIAN_POINT('Ctrl Pts',(-20.1345039282667,13.5603127148141,
132.354920444132)) ;
#117241=CARTESIAN_POINT('Ctrl Pts',(-20.1212776955433,13.8211026709328,
132.283193531999)) ;
#117242=CARTESIAN_POINT('Ctrl Pts',(-20.0864145211484,14.0538031496825,
132.148202189386)) ;
#117243=CARTESIAN_POINT('Ctrl Pts',(-20.0332397566341,14.2410907162982,
131.959757160238)) ;
#117244=CARTESIAN_POINT('Ctrl Pts',(-19.9660383596576,14.3701940931664,
131.730238162019)) ;
#117245=CARTESIAN_POINT('Ctrl Pts',(-19.8905439086927,14.4308809460844,
131.476512158403)) ;
#117246=CARTESIAN_POINT('Ctrl Pts',(-19.8134151755877,14.4196139003572,
131.218236026987)) ;
#117247=CARTESIAN_POINT('Ctrl Pts',(-19.7398726196564,14.336836882695,130.97020458083)) ;
#117248=CARTESIAN_POINT('Ctrl Pts',(-19.6767629170673,14.1892311561633,
130.752829213023)) ;
#117249=CARTESIAN_POINT('Ctrl Pts',(-19.6286665108586,13.9859053785223,
130.57912299113)) ;
#117250=CARTESIAN_POINT('Ctrl Pts',(-19.6002355231938,13.7426112517957,
130.462946926761)) ;
#117251=CARTESIAN_POINT('Ctrl Pts',(-19.594107429176,13.4761438814329,130.411880995108)) ;
#117252=CARTESIAN_POINT('Ctrl Pts',(-19.6113174094104,13.2070931774866,
130.429149009167)) ;
#117253=CARTESIAN_POINT('Ctrl Pts',(-19.6515803257306,12.9521503928351,
130.513580392613)) ;
#117254=CARTESIAN_POINT('Ctrl Pts',(-19.712491346524,12.7315094289201,130.658427474088)) ;
#117255=CARTESIAN_POINT('Ctrl Pts',(-19.7911656685738,12.55952255891,130.85492439979)) ;
#117256=CARTESIAN_POINT('Ctrl Pts',(-19.8809709738294,12.4509681348577,
131.084378584018)) ;
#117257=CARTESIAN_POINT('Ctrl Pts',(-19.9785025004899,12.4111337654698,
131.335955835968)) ;
#117258=CARTESIAN_POINT('Ctrl Pts',(-20.0750208858797,12.4436883987287,
131.58504110594)) ;
#117259=CARTESIAN_POINT('Ctrl Pts',(-20.1670489406682,12.5474867410868,
131.820478093993)) ;
#117260=CARTESIAN_POINT('Ctrl Pts',(-20.2460595301685,12.7123018104689,
132.018383639864)) ;
#117261=CARTESIAN_POINT('Ctrl Pts',(-20.3091917091409,12.930070804837,132.169503787281)) ;
#117262=CARTESIAN_POINT('Ctrl Pts',(-20.3512037961698,13.1802337484168,
132.259358056901)) ;
#117263=CARTESIAN_POINT('Ctrl Pts',(-20.3709163624956,13.4510759105696,
132.283623543489)) ;
#117264=CARTESIAN_POINT('Ctrl Pts',(-20.3669009496228,13.7180592820174,
132.238817284807)) ;
#117265=CARTESIAN_POINT('Ctrl Pts',(-20.3404947485754,13.9642785857624,
132.128552198951)) ;
#117266=CARTESIAN_POINT('Ctrl Pts',(-20.2943585159327,14.1712561448263,
131.960731543111)) ;
#117267=CARTESIAN_POINT('Ctrl Pts',(-20.2323687223324,14.3253724982605,
131.74652385602)) ;
#117268=CARTESIAN_POINT('Ctrl Pts',(-20.1592998865513,14.4148742496936,
131.499776720627)) ;
#117269=CARTESIAN_POINT('Ctrl Pts',(-20.0823960426978,14.4329087927554,
131.24220329871)) ;
#117270=CARTESIAN_POINT('Ctrl Pts',(-20.0063538704039,14.3788838662948,
130.986842165717)) ;
#117271=CARTESIAN_POINT('Ctrl Pts',(-19.9382630997815,14.2561020385484,
130.75479330686)) ;
#117272=CARTESIAN_POINT('Ctrl Pts',(-19.8835990530441,14.0742378905462,
130.562042928093)) ;
#117273=CARTESIAN_POINT('Ctrl Pts',(-19.8467989799249,13.8451951074059,
130.421387675447)) ;
#117274=CARTESIAN_POINT('Ctrl Pts',(-19.8313341159971,13.5867436924812,
130.343166472382)) ;
#117275=CARTESIAN_POINT('Ctrl Pts',(-19.8391431535007,13.3144406104729,
130.332664419117)) ;
#117276=CARTESIAN_POINT('Ctrl Pts',(-19.8701070003036,13.0528697153062,
130.390177046887)) ;
#117277=CARTESIAN_POINT('Ctrl Pts',(-19.922977018825,12.8160519673843,130.511475471805)) ;
#117278=CARTESIAN_POINT('Ctrl Pts',(-19.9949224006439,12.6226066577663,
130.688427360909)) ;
#117279=CARTESIAN_POINT('Ctrl Pts',(-20.0807929883206,12.4871997727771,
130.906234994754)) ;
#117280=CARTESIAN_POINT('Ctrl Pts',(-20.1763248041148,12.4184347906441,
131.152006317102)) ;
#117281=CARTESIAN_POINT('Ctrl Pts',(-20.2735243410858,12.421900095689,131.403058055158)) ;
#117282=CARTESIAN_POINT('Ctrl Pts',(-20.3681714156429,12.4968773890891,
131.646353538918)) ;
#117283=CARTESIAN_POINT('Ctrl Pts',(-20.453078884326,12.6381725134135,131.861295773607)) ;
#117284=CARTESIAN_POINT('Ctrl Pts',(-20.5233761153413,12.8360676034159,
132.033469623726)) ;
#117285=CARTESIAN_POINT('Ctrl Pts',(-20.5744273993862,13.0762564614049,
132.149423205006)) ;
#117286=CARTESIAN_POINT('Ctrl Pts',(-20.6032682080112,13.3398739353009,
132.200670249098)) ;
#117287=CARTESIAN_POINT('Ctrl Pts',(-20.6089153558675,13.6103042607725,
132.184053731351)) ;
#117288=CARTESIAN_POINT('Ctrl Pts',(-20.5913552359384,13.8681248638129,
132.0995339823)) ;
#117289=CARTESIAN_POINT('Ctrl Pts',(-20.5527417289415,14.0932870641316,
131.953614612924)) ;
#117290=CARTESIAN_POINT('Ctrl Pts',(-20.4963514522557,14.2707836154913,
131.755672439689)) ;
#117291=CARTESIAN_POINT('Ctrl Pts',(-20.4275781234429,14.3866738270234,
131.521785274535)) ;
#117292=CARTESIAN_POINT('Ctrl Pts',(-20.3513635050219,14.4343395634598,
131.266014418455)) ;
#117293=CARTESIAN_POINT('Ctrl Pts',(-20.2741102846849,14.4093417232231,
131.007191524153)) ;
#117294=CARTESIAN_POINT('Ctrl Pts',(-20.2022164359657,14.3139583409208,
130.764077181119)) ;
#117295=CARTESIAN_POINT('Ctrl Pts',(-20.1412573441085,14.1538396198972,
130.552752557387)) ;
#117296=CARTESIAN_POINT('Ctrl Pts',(-20.0969445519394,13.9434082159672,
130.390384097063)) ;
#117297=CARTESIAN_POINT('Ctrl Pts',(-20.0723542788181,13.6926166151685,
130.285177903961)) ;
#117298=CARTESIAN_POINT('Ctrl Pts',(-20.0706938890781,13.4252309496683,
130.247334933765)) ;
#117299=CARTESIAN_POINT('Ctrl Pts',(-20.092332751845,13.1569924841194,130.277454300474)) ;
#117300=CARTESIAN_POINT('Ctrl Pts',(-20.1366756135325,12.907415746913,130.373858632925)) ;
#117301=CARTESIAN_POINT('Ctrl Pts',(-20.2013825642992,12.6946405642384,
130.529698727295)) ;
#117302=CARTESIAN_POINT('Ctrl Pts',(-20.2819050644324,12.5348309351463,
130.731934046482)) ;
#117303=CARTESIAN_POINT('Ctrl Pts',(-20.3745177661893,12.4376124732534,
130.969168887914)) ;
#117304=CARTESIAN_POINT('Ctrl Pts',(-20.4716979393396,12.411847051202,131.220037230897)) ;
#117305=CARTESIAN_POINT('Ctrl Pts',(-20.5682462895583,12.4580456459642,
131.468969166317)) ;
#117306=CARTESIAN_POINT('Ctrl Pts',(-20.6577938331677,12.5736491008617,
131.697417164121)) ;
#117307=CARTESIAN_POINT('Ctrl Pts',(-20.7344433492042,12.7495591345061,
131.888265424488)) ;
#117308=CARTESIAN_POINT('Ctrl Pts',(-20.7939354209719,12.9753683217391,
132.028755611113)) ;
#117309=CARTESIAN_POINT('Ctrl Pts',(-20.8319052589719,13.2312289198464,
132.106671123273)) ;
#117310=CARTESIAN_POINT('Ctrl Pts',(-20.8470373803621,13.5022490913223,
132.117677262767)) ;
#117311=CARTESIAN_POINT('Ctrl Pts',(-20.8387067324782,13.7663766429706,
132.060301499346)) ;
#117312=CARTESIAN_POINT('Ctrl Pts',(-20.8083941645055,14.0063275981214,
131.938667665989)) ;
#117313=CARTESIAN_POINT('Ctrl Pts',(-20.7588632031017,14.2048735685629,
131.760851862467)) ;
#117314=CARTESIAN_POINT('Ctrl Pts',(-20.6941991703353,14.3476911545505,
131.538730144757)) ;
#117315=CARTESIAN_POINT('Ctrl Pts',(-20.6201333307794,14.4237776141336,
131.289235795019)) ;
#117316=CARTESIAN_POINT('Ctrl Pts',(-20.5425102852112,14.4280807917519,
131.029325961589)) ;
#117317=CARTESIAN_POINT('Ctrl Pts',(-20.467928775171,14.360827921304,130.778436656629)) ;
#117318=CARTESIAN_POINT('Ctrl Pts',(-20.4017581108605,14.2256361349193,
130.551896055991)) ;
#117319=CARTESIAN_POINT('Ctrl Pts',(-20.3503571718372,14.0344801252662,
130.368795956172)) ;
#117320=CARTESIAN_POINT('Ctrl Pts',(-20.3172512957461,13.7980437562362,
130.238869010308)) ;
#117321=CARTESIAN_POINT('Ctrl Pts',(-20.3061244134585,13.53532438393,130.173252180728)) ;
#117322=CARTESIAN_POINT('Ctrl Pts',(-20.3182993207692,13.2644875678434,
130.175688064952)) ;
#117323=CARTESIAN_POINT('Ctrl Pts',(-20.3536678560636,13.0050530170807,
130.245886392756)) ;
#117324=CARTESIAN_POINT('Ctrl Pts',(-20.410462049302,12.775438141039,130.378653667283)) ;
#117325=CARTESIAN_POINT('Ctrl Pts',(-20.4851886237847,12.5925960963687,
130.563862064022)) ;
#117326=CARTESIAN_POINT('Ctrl Pts',(-20.5732195435502,12.4690082469491,
130.787956911041)) ;
#117327=CARTESIAN_POINT('Ctrl Pts',(-20.6696209731858,12.4135709185057,
131.036318926835)) ;
#117328=CARTESIAN_POINT('Ctrl Pts',(-20.7669518533453,12.4306394810107,
131.287650324526)) ;
#117329=CARTESIAN_POINT('Ctrl Pts',(-20.8601171292825,12.5185474861746,
131.526674543202)) ;
#117330=CARTESIAN_POINT('Ctrl Pts',(-20.942837156887,12.6718439913262,131.73512693663)) ;
#117331=CARTESIAN_POINT('Ctrl Pts',(-21.009555833747,12.8780301439606,131.896984168492)) ;
#117332=CARTESIAN_POINT('Ctrl Pts',(-21.056821363786,13.1252485962165,132.001742572807)) ;
#117333=CARTESIAN_POINT('Ctrl Pts',(-21.0812481855893,13.3909665400584,
132.04016382239)) ;
#117334=CARTESIAN_POINT('Ctrl Pts',(-21.0824288286502,13.6612160877443,
132.010385535498)) ;
#117335=CARTESIAN_POINT('Ctrl Pts',(-21.0607478945341,13.9131568788034,
131.913987653532)) ;
#117336=CARTESIAN_POINT('Ctrl Pts',(-21.0185378959284,14.1304384080089,
131.757557383989)) ;
#117337=CARTESIAN_POINT('Ctrl Pts',(-20.9596569052815,14.2969775137474,
131.552483499945)) ;
#117338=CARTESIAN_POINT('Ctrl Pts',(-20.8883479707721,14.4015522183562,
131.310837907487)) ;
#117339=CARTESIAN_POINT('Ctrl Pts',(-20.811743048276,14.4350500547512,131.054060145774)) ;
#117340=CARTESIAN_POINT('Ctrl Pts',(-20.7352017856346,14.396751965708,130.797400979344)) ;
#117341=CARTESIAN_POINT('Ctrl Pts',(-20.6648700748169,14.2884849239284,
130.558794614213)) ;
#117342=CARTESIAN_POINT('Ctrl Pts',(-20.606731654312,14.1181741044495,130.355813335934)) ;
#117343=CARTESIAN_POINT('Ctrl Pts',(-20.5656967115575,13.8977533675812,
130.202766790401)) ;
#117344=CARTESIAN_POINT('Ctrl Pts',(-20.5454538498325,13.6446685040666,
130.110631870406)) ;
#117345=CARTESIAN_POINT('Ctrl Pts',(-20.5480734369409,13.3734340849695,
130.084992346971)) ;
#117346=CARTESIAN_POINT('Ctrl Pts',(-20.5742578565967,13.1072277425428,
130.128374016336)) ;
#117347=CARTESIAN_POINT('Ctrl Pts',(-20.6225056372082,12.8641926256241,
130.236294496297)) ;
#117348=CARTESIAN_POINT('Ctrl Pts',(-20.6904289274689,12.6605228267135,
130.401603234601)) ;
#117349=CARTESIAN_POINT('Ctrl Pts',(-20.7736447523668,12.5114117943071,
130.611629156176)) ;
#117350=CARTESIAN_POINT('Ctrl Pts',(-20.8678757743497,12.4272142366947,
130.853549028094)) ;
#117351=CARTESIAN_POINT('Ctrl Pts',(-20.9651014565131,12.4150347895705,
131.104641444644)) ;
#117352=CARTESIAN_POINT('Ctrl Pts',(-21.060978957513,12.4747490693336,131.35154192915)) ;
#117353=CARTESIAN_POINT('Ctrl Pts',(-21.1484527801317,12.6023244974168,
131.573977816226)) ;
#117354=CARTESIAN_POINT('Ctrl Pts',(-21.2225268496985,12.7898413054048,
131.757084110712)) ;
#117355=CARTESIAN_POINT('Ctrl Pts',(-21.2776732687232,13.0206705904154,
131.885228927191)) ;
#117356=CARTESIAN_POINT('Ctrl Pts',(-21.3116929767443,13.2818516686094,
131.951421363387)) ;
#117357=CARTESIAN_POINT('Ctrl Pts',(-21.3223256302397,13.5521276503918,
131.949431203066)) ;
#117358=CARTESIAN_POINT('Ctrl Pts',(-21.3097945676816,13.8139567141273,
131.87968328586)) ;
#117359=CARTESIAN_POINT('Ctrl Pts',(-21.2752727495354,14.048569772894,131.745542468365)) ;
#117360=CARTESIAN_POINT('Ctrl Pts',(-21.2228787528856,14.236110064849,131.559589873959)) ;
#117361=CARTESIAN_POINT('Ctrl Pts',(-21.1558243323814,14.3675383495349,
131.330396273337)) ;
#117362=CARTESIAN_POINT('Ctrl Pts',(-21.0806484199029,14.4300942129039,
131.077681198035)) ;
#117363=CARTESIAN_POINT('Ctrl Pts',(-21.0033788252062,14.4208865440108,
130.818936586364)) ;
#117364=CARTESIAN_POINT('Ctrl Pts',(-20.9298451040332,14.3405661595428,
130.571042931108)) ;
#117365=CARTESIAN_POINT('Ctrl Pts',(-20.8658533560393,14.1934623353678,
130.350815526822)) ;
#117366=CARTESIAN_POINT('Ctrl Pts',(-20.8175001319599,13.9917022900947,
130.176448833883)) ;
#117367=CARTESIAN_POINT('Ctrl Pts',(-20.7885759620872,13.7502057571416,
130.058945585873)) ;
#117368=CARTESIAN_POINT('Ctrl Pts',(-20.7817113274138,13.4844948245858,
130.005770974268)) ;
#117369=CARTESIAN_POINT('Ctrl Pts',(-20.7983394804369,13.2141841608485,
130.021199429463)) ;
#117370=CARTESIAN_POINT('Ctrl Pts',(-20.8378966646696,12.9589228600533,
130.103630667804)) ;
#117371=CARTESIAN_POINT('Ctrl Pts',(-20.8986899919378,12.7362703078518,
130.247957265141)) ;
#117372=CARTESIAN_POINT('Ctrl Pts',(-20.9757867279196,12.5648475135275,
130.440319362778)) ;
#117373=CARTESIAN_POINT('Ctrl Pts',(-21.0663368128741,12.452872637983,130.67154841129)) ;
#117374=CARTESIAN_POINT('Ctrl Pts',(-21.1629005182569,12.411294196787,130.920610155833)) ;
#117375=CARTESIAN_POINT('Ctrl Pts',(-21.260397731377,12.4419882066381,131.172234258394)) ;
#117376=CARTESIAN_POINT('Ctrl Pts',(-21.3517237017797,12.5427027858175,
131.405983597941)) ;
#117377=CARTESIAN_POINT('Ctrl Pts',(-21.4318039101064,12.706796402249,131.606755442303)) ;
#117378=CARTESIAN_POINT('Ctrl Pts',(-21.4952071393745,12.9221001593752,
131.758848779645)) ;
#117379=CARTESIAN_POINT('Ctrl Pts',(-21.538280315247,13.1741319900526,131.851446839118)) ;
#117380=CARTESIAN_POINT('Ctrl Pts',(-21.5584177432059,13.4427023276839,
131.877218319414)) ;
#117381=CARTESIAN_POINT('Ctrl Pts',(-21.5551172048958,13.7107857008536,
131.834398380484)) ;
#117382=CARTESIAN_POINT('Ctrl Pts',(-21.5294381391568,13.9568883020333,
131.726395472109)) ;
#117383=CARTESIAN_POINT('Ctrl Pts',(-21.483735439408,14.1661036589884,131.559726534066)) ;
#117384=CARTESIAN_POINT('Ctrl Pts',(-21.4219683482731,14.3219384877272,
131.346112125423)) ;
#117385=CARTESIAN_POINT('Ctrl Pts',(-21.3496214859993,14.4130180667709,
131.10169089437)) ;
#117386=CARTESIAN_POINT('Ctrl Pts',(-21.2722521429854,14.4335349377785,
130.842535969221)) ;
#117387=CARTESIAN_POINT('Ctrl Pts',(-21.1960388298333,14.3810414591398,
130.586644305319)) ;
#117388=CARTESIAN_POINT('Ctrl Pts',(-21.1280003928797,14.2609491563611,
130.354936375839)) ;
#117389=CARTESIAN_POINT('Ctrl Pts',(-21.0725876584999,14.0795345145358,
130.159800933147)) ;
#117390=CARTESIAN_POINT('Ctrl Pts',(-21.035403480221,13.8529285433275,130.018220066341)) ;
#117391=CARTESIAN_POINT('Ctrl Pts',(-21.01921653569,13.5926909018936,129.937579732469)) ;
#117392=CARTESIAN_POINT('Ctrl Pts',(-21.0263535490702,13.3230679904021,
129.925443216821)) ;
#117393=CARTESIAN_POINT('Ctrl Pts',(-21.056724206518,13.0595446516906,129.981042089682)) ;
#117394=CARTESIAN_POINT('Ctrl Pts',(-21.1092312885458,12.821409078981,130.101215513039)) ;
#117395=CARTESIAN_POINT('Ctrl Pts',(-21.1806069334904,12.6270968771254,
130.276569849838)) ;
#117396=CARTESIAN_POINT('Ctrl Pts',(-21.2658529230612,12.4904302575877,
130.492664537939)) ;
#117397=CARTESIAN_POINT('Ctrl Pts',(-21.3608874562241,12.4195264376518,
130.737086059353)) ;
#117398=CARTESIAN_POINT('Ctrl Pts',(-21.4585744347889,12.4206997747971,
130.989400021545)) ;
#117399=CARTESIAN_POINT('Ctrl Pts',(-21.5535287966605,12.4940150849619,
131.233544186021)) ;
#117400=CARTESIAN_POINT('Ctrl Pts',(-21.6385302946146,12.6331733496192,
131.448855787369)) ;
#117401=CARTESIAN_POINT('Ctrl Pts',(-21.7092724630891,12.8293255236082,
131.622363791874)) ;
#117402=CARTESIAN_POINT('Ctrl Pts',(-21.7609583754883,13.0683011169746,
131.740190348621)) ;
#117403=CARTESIAN_POINT('Ctrl Pts',(-21.7905747827233,13.3322965961088,
131.793597517871)) ;
#117404=CARTESIAN_POINT('Ctrl Pts',(-21.7968440357838,13.6026348428664,
131.77882032904)) ;
#117405=CARTESIAN_POINT('Ctrl Pts',(-21.7800208228364,13.8605087628932,
131.69653724068)) ;
#117406=CARTESIAN_POINT('Ctrl Pts',(-21.741943453815,14.0871783650871,131.55213623212)) ;
#117407=CARTESIAN_POINT('Ctrl Pts',(-21.68623340069,14.2658343770077,131.356293575374)) ;
#117408=CARTESIAN_POINT('Ctrl Pts',(-21.6174834581691,14.3843789391541,
131.122326149126)) ;
#117409=CARTESIAN_POINT('Ctrl Pts',(-21.5412324446713,14.4339734241572,
130.866388632503)) ;
#117410=CARTESIAN_POINT('Ctrl Pts',(-21.4641445421631,14.4110559361857,
130.608142700945)) ;
#117411=CARTESIAN_POINT('Ctrl Pts',(-21.3920751414043,14.3178925144465,
130.364549551773)) ;
#117412=CARTESIAN_POINT('Ctrl Pts',(-21.3305900015809,14.1593686690055,
130.151640808334)) ;
#117413=CARTESIAN_POINT('Ctrl Pts',(-21.28571730329,13.9496805388889,129.987566165016)) ;
#117414=CARTESIAN_POINT('Ctrl Pts',(-21.2606021210969,13.7013470012748,
129.881036373736)) ;
#117415=CARTESIAN_POINT('Ctrl Pts',(-21.2581837575686,13.4330164706509,
129.840817045843)) ;
#117416=CARTESIAN_POINT('Ctrl Pts',(-21.2791303522906,13.1647607659068,
129.868952988127)) ;
#117417=CARTESIAN_POINT('Ctrl Pts',(-21.3230136561864,12.9137311953691,
129.963914319132)) ;
#117418=CARTESIAN_POINT('Ctrl Pts',(-21.3867869705194,12.7007529765594,
130.11721967487)) ;
#117419=CARTESIAN_POINT('Ctrl Pts',(-21.4673969827414,12.5383275950027,
130.31950305487)) ;
#117420=CARTESIAN_POINT('Ctrl Pts',(-21.5589884850291,12.4398166155699,
130.554035906025)) ;
#117421=CARTESIAN_POINT('Ctrl Pts',(-21.6569056837699,12.4114725014285,
130.806774281656)) ;
#117422=CARTESIAN_POINT('Ctrl Pts',(-21.7533528899772,12.4557968837197,
131.05548625053)) ;
#117423=CARTESIAN_POINT('Ctrl Pts',(-21.8432789043905,12.5696290703402,
131.285000886597)) ;
#117424=CARTESIAN_POINT('Ctrl Pts',(-21.9201726688622,12.7436129145437,
131.476639481316)) ;
#117425=CARTESIAN_POINT('Ctrl Pts',(-21.9802672632297,12.9681021997866,
131.618894855905)) ;
#117426=CARTESIAN_POINT('Ctrl Pts',(-22.0189477125869,13.2239470656193,
131.698804483607)) ;
#117427=CARTESIAN_POINT('Ctrl Pts',(-22.0347032747222,13.4941632022952,
131.711716289731)) ;
#117428=CARTESIAN_POINT('Ctrl Pts',(-22.0270640928502,13.7589185594046,
131.656336781611)) ;
#117429=CARTESIAN_POINT('Ctrl Pts',(-21.9973553870793,13.999834830615,131.536469000517)) ;
#117430=CARTESIAN_POINT('Ctrl Pts',(-21.9483276850161,14.1997645777198,
131.360124808153)) ;
#117431=CARTESIAN_POINT('Ctrl Pts',(-21.8841603470841,14.3442636718176,
131.13951370011)) ;
#117432=CARTESIAN_POINT('Ctrl Pts',(-21.8101465753952,14.4224928178984,
130.890102479285)) ;
#117433=CARTESIAN_POINT('Ctrl Pts',(-21.7329264414407,14.429171124512,130.631541457606)) ;
#117434=CARTESIAN_POINT('Ctrl Pts',(-21.6576229271443,14.3636109202534,
130.378296756051)) ;
#117435=CARTESIAN_POINT('Ctrl Pts',(-21.5913563328133,14.2305642022342,
130.151592715176)) ;
#117436=CARTESIAN_POINT('Ctrl Pts',(-21.5393783348571,14.0406276478755,
129.966746548751)) ;
#117437=CARTESIAN_POINT('Ctrl Pts',(-21.5057424380608,13.8058700767644,
129.83536020891)) ;
#117438=CARTESIAN_POINT('Ctrl Pts',(-21.4938927574469,13.5427809263485,
129.767514290558)) ;
#117439=CARTESIAN_POINT('Ctrl Pts',(-21.5054182379161,13.2720606343581,
129.768076155216)) ;
#117440=CARTESIAN_POINT('Ctrl Pts',(-21.5402011630011,13.0118430008048,
129.836532518463)) ;
#117441=CARTESIAN_POINT('Ctrl Pts',(-21.5962302154441,12.7818788914411,
129.967174419834)) ;
#117442=CARTESIAN_POINT('Ctrl Pts',(-21.670640798543,12.5968717145733,130.151376252176)) ;
#117443=CARTESIAN_POINT('Ctrl Pts',(-21.7587635661607,12.471251749294,130.375607689773)) ;
#117444=CARTESIAN_POINT('Ctrl Pts',(-21.8545581424731,12.4142248024153,
130.62236302727)) ;
#117445=CARTESIAN_POINT('Ctrl Pts',(-21.9520906421161,12.4291610280905,
130.874226280264)) ;
#117446=CARTESIAN_POINT('Ctrl Pts',(-22.0455195215998,12.5152749264354,
131.114002208116)) ;
#117447=CARTESIAN_POINT('Ctrl Pts',(-22.1287010469112,12.6672522037425,
131.323753516195)) ;
#117448=CARTESIAN_POINT('Ctrl Pts',(-22.1956105072192,12.8714563204239,
131.4862930258)) ;
#117449=CARTESIAN_POINT('Ctrl Pts',(-22.243376326576,13.1164156174602,131.592674877965)) ;
#117450=CARTESIAN_POINT('Ctrl Pts',(-22.2686940144247,13.3833143441499,
131.633503423445)) ;
#117451=CARTESIAN_POINT('Ctrl Pts',(-22.2704874915353,13.6536761481919,
131.605526541394)) ;
#117452=CARTESIAN_POINT('Ctrl Pts',(-22.24948244657,13.9063303510439,131.511114286094)) ;
#117453=CARTESIAN_POINT('Ctrl Pts',(-22.20758512911,14.125656517117,131.355457053907)) ;
#117454=CARTESIAN_POINT('Ctrl Pts',(-22.1492829761526,14.2929703980627,
131.152198443017)) ;
#117455=CARTESIAN_POINT('Ctrl Pts',(-22.0784214005424,14.3994043116304,
130.911932860175)) ;
#117456=CARTESIAN_POINT('Ctrl Pts',(-22.0017663750558,14.4351253202173,
130.654948854145)) ;
#117457=CARTESIAN_POINT('Ctrl Pts',(-21.9250783887851,14.3988243960317,
130.397839099872)) ;
#117458=CARTESIAN_POINT('Ctrl Pts',(-21.8544672752435,14.2923293352694,
130.158403148621)) ;
#117459=CARTESIAN_POINT('Ctrl Pts',(-21.796086879611,14.1241731264117,129.95481572673)) ;
#117460=CARTESIAN_POINT('Ctrl Pts',(-21.7544221874796,13.9051614113411,
129.799931790305)) ;
#117461=CARTESIAN_POINT('Ctrl Pts',(-21.7335082685694,13.6518311651615,
129.705713043414)) ;
#117462=CARTESIAN_POINT('Ctrl Pts',(-21.7354233483292,13.3824709073359,
129.678222201939)) ;
#117463=CARTESIAN_POINT('Ctrl Pts',(-21.7608220827505,13.1154253755206,
129.719260176606)) ;
#117464=CARTESIAN_POINT('Ctrl Pts',(-21.8086454011538,12.870532700791,129.825813473863)) ;
#117465=CARTESIAN_POINT('Ctrl Pts',(-21.8760630288498,12.6655371324335,
129.98965053552)) ;
#117466=CARTESIAN_POINT('Ctrl Pts',(-21.9590806571557,12.5146112693424,
130.199039203273)) ;
#117467=CARTESIAN_POINT('Ctrl Pts',(-22.0525303154173,12.4289102076434,
130.438877066077)) ;
#117468=CARTESIAN_POINT('Ctrl Pts',(-22.1499357478845,12.4141896647539,
130.690419940938)) ;
#117469=CARTESIAN_POINT('Ctrl Pts',(-22.2464800920588,12.4724108271044,
130.939085979188)) ;
#117470=CARTESIAN_POINT('Ctrl Pts',(-22.3337993299092,12.5978141623982,
131.161227476013)) ;
#117471=CARTESIAN_POINT('Ctrl Pts',(-22.4080948789666,12.7826551138703,
131.345130318457)) ;
#117472=CARTESIAN_POINT('Ctrl Pts',(-22.4641606542721,13.013381389437,131.47580076802)) ;
#117473=CARTESIAN_POINT('Ctrl Pts',(-22.4988395076517,13.2742167666549,
131.543895101829)) ;
#117474=CARTESIAN_POINT('Ctrl Pts',(-22.5101407381888,13.5450313802589,
131.543790291758)) ;
#117475=CARTESIAN_POINT('Ctrl Pts',(-22.4982044056219,13.8067210995316,
131.475851915162)) ;
#117476=CARTESIAN_POINT('Ctrl Pts',(-22.4645746319177,14.0412512155271,
131.34450786244)) ;
#117477=CARTESIAN_POINT('Ctrl Pts',(-22.4122950867002,14.2318696546287,
131.158634956438)) ;
#117478=CARTESIAN_POINT('Ctrl Pts',(-22.3456877419971,14.3645252689238,
130.930833330674)) ;
#117479=CARTESIAN_POINT('Ctrl Pts',(-22.2709959410269,14.4291513639763,
130.679660185262)) ;
#117480=CARTESIAN_POINT('Ctrl Pts',(-22.1934041314825,14.4223448397237,
130.419851989127)) ;
#117481=CARTESIAN_POINT('Ctrl Pts',(-22.1194291252965,14.3433928726762,
130.170543084568)) ;
#117482=CARTESIAN_POINT('Ctrl Pts',(-22.0555971430006,14.1993298116068,
129.951061058198)) ;
#117483=CARTESIAN_POINT('Ctrl Pts',(-22.0065113703687,13.9988091287191,
129.774469836655)) ;
#117484=CARTESIAN_POINT('Ctrl Pts',(-21.9768862871608,13.7578102679721,
129.654858267008)) ;
#117485=CARTESIAN_POINT('Ctrl Pts',(-21.96939073113,13.491649195449,129.59973283208)) ;
#117486=CARTESIAN_POINT('Ctrl Pts',(-21.9852726561706,13.2223244098795,
129.613124864141)) ;
#117487=CARTESIAN_POINT('Ctrl Pts',(-22.0242864346578,12.96574693319,129.693881033276)) ;
#117488=CARTESIAN_POINT('Ctrl Pts',(-22.0841556386316,12.7429297081588,
129.835684633343)) ;
#117489=CARTESIAN_POINT('Ctrl Pts',(-22.1613403500013,12.5685157395234,
130.028061959146)) ;
#117490=CARTESIAN_POINT('Ctrl Pts',(-22.2516375164601,12.4549912739037,
130.258564915234)) ;
#117491=CARTESIAN_POINT('Ctrl Pts',(-22.3478911325682,12.4115665134561,
130.506787270611)) ;
#117492=CARTESIAN_POINT('Ctrl Pts',(-22.4452527950756,12.439915366976,130.758091824848)) ;
#117493=CARTESIAN_POINT('Ctrl Pts',(-22.5373117307679,12.5392662703676,
130.993804347961)) ;
#117494=CARTESIAN_POINT('Ctrl Pts',(-22.617570466028,12.7015765318143,131.195172124663)) ;
#117495=CARTESIAN_POINT('Ctrl Pts',(-22.6813553440246,12.9151235355211,
131.348450745226)) ;
#117496=CARTESIAN_POINT('Ctrl Pts',(-22.7250421972977,13.1655123701317,
131.442940664013)) ;
#117497=CARTESIAN_POINT('Ctrl Pts',(-22.7459884427464,13.435707308921,131.47084115714)) ;
#117498=CARTESIAN_POINT('Ctrl Pts',(-22.7433276408327,13.7027427336547,
131.430060345605)) ;
#117499=CARTESIAN_POINT('Ctrl Pts',(-22.7182573822089,13.9504288164231,
131.323744309634)) ;
#117500=CARTESIAN_POINT('Ctrl Pts',(-22.6730240374832,14.1608970885181,
131.158442255366)) ;
#117501=CARTESIAN_POINT('Ctrl Pts',(-22.6117684050325,14.3182076506529,
130.946379659081)) ;
#117502=CARTESIAN_POINT('Ctrl Pts',(-22.5395371501238,14.4114239636762,
130.702243522924)) ;
#117503=CARTESIAN_POINT('Ctrl Pts',(-22.4623760563283,14.43387114395,130.443760543668)) ;
#117504=CARTESIAN_POINT('Ctrl Pts',(-22.3862131332903,14.3839736485786,
130.188109535788)) ;
#117505=CARTESIAN_POINT('Ctrl Pts',(-22.3174374178138,14.2649034164715,
129.95402457402)) ;
#117506=CARTESIAN_POINT('Ctrl Pts',(-22.2619059919946,14.0862373803975,
129.758759467005)) ;
#117507=CARTESIAN_POINT('Ctrl Pts',(-22.2239114025602,13.8593710344565,
129.614595036615)) ;
#117508=CARTESIAN_POINT('Ctrl Pts',(-22.2071929927876,13.6016402973256,
129.532649135829)) ;
#117509=CARTESIAN_POINT('Ctrl Pts',(-22.2135652103266,13.3309242141033,
129.518127722561)) ;
#117510=CARTESIAN_POINT('Ctrl Pts',(-22.2433163399307,13.0670234319289,
129.571929224673)) ;
#117511=CARTESIAN_POINT('Ctrl Pts',(-22.2950002229724,12.828626261272,129.689806885452)) ;
#117512=CARTESIAN_POINT('Ctrl Pts',(-22.365802048165,12.6324569777035,129.863476559603)) ;
#117513=CARTESIAN_POINT('Ctrl Pts',(-22.4512496266196,12.4932134027072,
130.079952535297)) ;
#117514=CARTESIAN_POINT('Ctrl Pts',(-22.5456609744461,12.4206918298189,
130.322713874521)) ;
#117515=CARTESIAN_POINT('Ctrl Pts',(-22.643660846344,12.4196226590599,130.575832766512)) ;
#117516=CARTESIAN_POINT('Ctrl Pts',(-22.7387240475708,12.4910154498675,
130.820318212751)) ;
#117517=CARTESIAN_POINT('Ctrl Pts',(-22.8240998486431,12.6283739089441,
131.036714320096)) ;
#117518=CARTESIAN_POINT('Ctrl Pts',(-22.8954898572855,12.8237068444054,
131.212026952757)) ;
#117519=CARTESIAN_POINT('Ctrl Pts',(-22.9476329864119,13.0616748025397,
131.331212538775)) ;
#117520=CARTESIAN_POINT('Ctrl Pts',(-22.9777884983749,13.3240381252934,
131.386338288127)) ;
#117521=CARTESIAN_POINT('Ctrl Pts',(-22.984806720309,13.5952492770895,131.37365349371)) ;
#117522=CARTESIAN_POINT('Ctrl Pts',(-22.9684914873927,13.8544594163448,
131.292756287018)) ;
#117523=CARTESIAN_POINT('Ctrl Pts',(-22.9309664261002,14.081653901287,131.150031141549)) ;
#117524=CARTESIAN_POINT('Ctrl Pts',(-22.8758875876101,14.2612879476329,
130.956139962611)) ;
#117525=CARTESIAN_POINT('Ctrl Pts',(-22.807480111904,14.38176341734,130.723183101685)) ;
#117526=CARTESIAN_POINT('Ctrl Pts',(-22.7313394071239,14.4336477337376,
130.467559606026)) ;
#117527=CARTESIAN_POINT('Ctrl Pts',(-22.6537605132197,14.4124734002023,
130.207689335907)) ;
#117528=CARTESIAN_POINT('Ctrl Pts',(-22.5818879901239,14.3214777532126,
129.964850139128)) ;
#117529=CARTESIAN_POINT('Ctrl Pts',(-22.5200315465699,14.1652192668134,
129.750907755924)) ;
#117530=CARTESIAN_POINT('Ctrl Pts',(-22.4744220607307,13.9555650448247,
129.584493284428)) ;
#117531=CARTESIAN_POINT('Ctrl Pts',(-22.4488665968957,13.7095599731385,
129.476881160954)) ;
#117532=CARTESIAN_POINT('Ctrl Pts',(-22.4456673420391,13.4405995134717,
129.434259316074)) ;
#117533=CARTESIAN_POINT('Ctrl Pts',(-22.466134692506,13.1715077445613,129.460914435123)) ;
#117534=CARTESIAN_POINT('Ctrl Pts',(-22.5090044012617,12.9214880531583,
129.553167187894)) ;
#117535=CARTESIAN_POINT('Ctrl Pts',(-22.5727363504163,12.7055052901806,
129.706083200255)) ;
#117536=CARTESIAN_POINT('Ctrl Pts',(-22.6525084041682,12.542519660956,129.906118446746)) ;
#117537=CARTESIAN_POINT('Ctrl Pts',(-22.7440355247971,12.4416160246637,
130.140380677478)) ;
#117538=CARTESIAN_POINT('Ctrl Pts',(-22.8419577727742,12.4112449651492,
130.393113475988)) ;
#117539=CARTESIAN_POINT('Ctrl Pts',(-22.9385842532159,12.4537097184138,
130.642318308563)) ;
#117540=CARTESIAN_POINT('Ctrl Pts',(-23.0284918398332,12.5652232692769,
130.871894090839)) ;
#117541=CARTESIAN_POINT('Ctrl Pts',(-23.1059904833147,12.7379440024603,
131.065226412408)) ;
#117542=CARTESIAN_POINT('Ctrl Pts',(-23.1664409525888,12.9603974208925,
131.208644145665)) ;
#117543=CARTESIAN_POINT('Ctrl Pts',(-23.2058738661695,13.2156634379738,
131.290722671192)) ;
#117544=CARTESIAN_POINT('Ctrl Pts',(-23.2223740608505,13.4857933225146,
131.305803982737)) ;
#117545=CARTESIAN_POINT('Ctrl Pts',(-23.2153757035201,13.7522945834018,
131.252134307635)) ;
#117546=CARTESIAN_POINT('Ctrl Pts',(-23.1860831994402,13.9943543864371,
131.133424212874)) ;
#117547=CARTESIAN_POINT('Ctrl Pts',(-23.1377716895793,14.1947045665703,
130.959330792338)) ;
#117548=CARTESIAN_POINT('Ctrl Pts',(-23.0736751781071,14.341452901732,130.738783006091)) ;
#117549=CARTESIAN_POINT('Ctrl Pts',(-23.0002138225239,14.4211242912775,
130.491156682117)) ;
#117550=CARTESIAN_POINT('Ctrl Pts',(-22.9228562469191,14.4300014441918,
130.232122262372)) ;
#117551=CARTESIAN_POINT('Ctrl Pts',(-22.8475359109816,14.3664766103849,
129.978889630727)) ;
#117552=CARTESIAN_POINT('Ctrl Pts',(-22.7809795595032,14.2356053057405,
129.751376119369)) ;
#117553=CARTESIAN_POINT('Ctrl Pts',(-22.7283015195165,14.0463421699273,
129.564345016875)) ;
#117554=CARTESIAN_POINT('Ctrl Pts',(-22.6942101862441,13.8127313116574,
129.431663289963)) ;
#117555=CARTESIAN_POINT('Ctrl Pts',(-22.6816965286036,13.5514862656321,
129.362037523503)) ;
#117556=CARTESIAN_POINT('Ctrl Pts',(-22.6925426421092,13.2797432937496,
129.360489515288)) ;
#117557=CARTESIAN_POINT('Ctrl Pts',(-22.7265639166718,13.0196142656872,
129.426812143923)) ;
#117558=CARTESIAN_POINT('Ctrl Pts',(-22.7821800145146,12.7876902930479,
129.556129340797)) ;
#117559=CARTESIAN_POINT('Ctrl Pts',(-22.8560631060446,12.601531820227,129.738836537011)) ;
#117560=CARTESIAN_POINT('Ctrl Pts',(-22.9435871387763,12.4742597851615,
129.961412674426)) ;
#117561=CARTESIAN_POINT('Ctrl Pts',(-23.0393462544556,12.4148459828286,
130.208020099455)) ;
#117562=CARTESIAN_POINT('Ctrl Pts',(-23.1371787911307,12.4277167902933,
130.460672834474)) ;
#117563=CARTESIAN_POINT('Ctrl Pts',(-23.230720242296,12.5119511239392,130.700802831838)) ;
#117564=CARTESIAN_POINT('Ctrl Pts',(-23.3139766894554,12.6612550507726,
130.910919767823)) ;
#117565=CARTESIAN_POINT('Ctrl Pts',(-23.3818918394962,12.8654797343675,
131.076161928415)) ;
#117566=CARTESIAN_POINT('Ctrl Pts',(-23.4300486843934,13.1088715380583,
131.183794226756)) ;
#117567=CARTESIAN_POINT('Ctrl Pts',(-23.4560676914534,13.3752798477322,
131.226678355845)) ;
#117568=CARTESIAN_POINT('Ctrl Pts',(-23.4585672304719,13.6458119714847,
131.200772103874)) ;
#117569=CARTESIAN_POINT('Ctrl Pts',(-23.4381500504978,13.8994657965604,
131.108034372121)) ;
#117570=CARTESIAN_POINT('Ctrl Pts',(-23.3970305648326,14.1192748903921,
130.954788430871)) ;
#117571=CARTESIAN_POINT('Ctrl Pts',(-23.3388505991546,14.289180306213,130.75170335035)) ;
#117572=CARTESIAN_POINT('Ctrl Pts',(-23.2685796505926,14.3970324953059,
130.513322005132)) ;
#117573=CARTESIAN_POINT('Ctrl Pts',(-23.1918669872229,14.4351164743851,
130.256093295235)) ;
#117574=CARTESIAN_POINT('Ctrl Pts',(-23.1151547683793,14.4010787676098,
129.99895063463)) ;
#117575=CARTESIAN_POINT('Ctrl Pts',(-23.0438797487147,14.2958209234975,
129.757379843871)) ;
#117576=CARTESIAN_POINT('Ctrl Pts',(-22.9853452749484,14.1296521766069,
129.553460069811)) ;
#117577=CARTESIAN_POINT('Ctrl Pts',(-22.9431411507693,13.9121761436852,
129.397030923481)) ;
#117578=CARTESIAN_POINT('Ctrl Pts',(-22.9215986259908,13.659430364987,129.300954719031)) ;
#117579=CARTESIAN_POINT('Ctrl Pts',(-22.9227710010657,13.3906473352246,
129.271342984019)) ;
#117580=CARTESIAN_POINT('Ctrl Pts',(-22.9477490187839,13.12154860475,129.310931003686)) ;
#117581=CARTESIAN_POINT('Ctrl Pts',(-22.9946832883936,12.8774995309081,
129.415117779417)) ;
#117582=CARTESIAN_POINT('Ctrl Pts',(-23.0618596955509,12.6702279872938,
129.578103482037)) ;
#117583=CARTESIAN_POINT('Ctrl Pts',(-23.1441807626484,12.5183910771853,
129.785600084306)) ;
#117584=CARTESIAN_POINT('Ctrl Pts',(-23.2374158209668,12.4302683284587,
130.024797603841)) ;
#117585=CARTESIAN_POINT('Ctrl Pts',(-23.3354851080601,12.4138255810916,
130.278040824562)) ;
#117586=CARTESIAN_POINT('Ctrl Pts',(-23.4309623901203,12.469284941687,130.524009939854)) ;
#117587=CARTESIAN_POINT('Ctrl Pts',(-23.5192303902685,12.5930867722267,
130.748712365455)) ;
#117588=CARTESIAN_POINT('Ctrl Pts',(-23.5941185443368,12.7771358580158,
130.934261108261)) ;
#117589=CARTESIAN_POINT('Ctrl Pts',(-23.6505481822479,13.0059648630076,
131.066110013963)) ;
#117590=CARTESIAN_POINT('Ctrl Pts',(-23.6859230327796,13.266147051347,131.13623790108)) ;
#117591=CARTESIAN_POINT('Ctrl Pts',(-23.6979431807968,13.536990507266,131.13822821022)) ;
#117592=CARTESIAN_POINT('Ctrl Pts',(-23.686621463364,13.7997447814263,131.072011498558)) ;
#117593=CARTESIAN_POINT('Ctrl Pts',(-23.6536279786408,14.0350782594662,
130.942568905358)) ;
#117594=CARTESIAN_POINT('Ctrl Pts',(-23.6015630359019,14.2276700254763,
130.757191818353)) ;
#117595=CARTESIAN_POINT('Ctrl Pts',(-23.5359237415765,14.3610390583721,
130.532530125429)) ;
#117596=CARTESIAN_POINT('Ctrl Pts',(-23.4607912004887,14.4285213443226,
130.279787586806)) ;
#117597=CARTESIAN_POINT('Ctrl Pts',(-23.3833487009935,14.4233691665642,
130.020486659445)) ;
#117598=CARTESIAN_POINT('Ctrl Pts',(-23.3093760780976,14.3469901017567,
129.771288961701)) ;
#117599=CARTESIAN_POINT('Ctrl Pts',(-23.2447416178351,14.2034040422047,
129.549206908219)) ;
#117600=CARTESIAN_POINT('Ctrl Pts',(-23.1955501320454,14.0056848767319,
129.372560459008)) ;
#117601=CARTESIAN_POINT('Ctrl Pts',(-23.1651831662936,13.7644936141034,
129.250611487081)) ;
#117602=CARTESIAN_POINT('Ctrl Pts',(-23.1570313325639,13.5002464496988,
129.193764768034)) ;
#117603=CARTESIAN_POINT('Ctrl Pts',(-23.17244335945,13.2284058869682,129.205478850498)) ;
#117604=CARTESIAN_POINT('Ctrl Pts',(-23.2104466819188,12.9739038042497,
129.283643071442)) ;
#117605=CARTESIAN_POINT('Ctrl Pts',(-23.2700066779842,12.748470453343,129.424347957769)) ;
#117606=CARTESIAN_POINT('Ctrl Pts',(-23.3465319156382,12.5731123494061,
129.614911120667)) ;
#117607=CARTESIAN_POINT('Ctrl Pts',(-23.4365877316903,12.4573590885892,
129.844675535288)) ;
#117608=CARTESIAN_POINT('Ctrl Pts',(-23.5328287006259,12.4118025442917,
130.092830099102)) ;
#117609=CARTESIAN_POINT('Ctrl Pts',(-23.6302800263178,12.4381298230363,
130.34438605469)) ;
#117610=CARTESIAN_POINT('Ctrl Pts',(-23.7224239211814,12.5352056579817,
130.580413513911)) ;
#117611=CARTESIAN_POINT('Ctrl Pts',(-23.8033213508231,12.6963006078304,
130.783546488431)) ;
#117612=CARTESIAN_POINT('Ctrl Pts',(-23.8675954361833,12.9082756117234,
130.938298311993)) ;
#117613=CARTESIAN_POINT('Ctrl Pts',(-23.9120498738717,13.1596325354774,
131.034809909213)) ;
#117614=CARTESIAN_POINT('Ctrl Pts',(-23.9333960142979,13.4259468867853,
131.06433034029)) ;
#117615=CARTESIAN_POINT('Ctrl Pts',(-23.9315577140667,13.6953761022081,
131.025693667659)) ;
#117616=CARTESIAN_POINT('Ctrl Pts',(-23.9070542170469,13.9437170228922,
130.92105547931)) ;
#117617=CARTESIAN_POINT('Ctrl Pts',(-23.8623046093946,14.1557110770192,
130.757127908261)) ;
#117618=CARTESIAN_POINT('Ctrl Pts',(-23.801544851302,14.3144000142637,130.546576005001)) ;
#117619=CARTESIAN_POINT('Ctrl Pts',(-23.7295838462157,14.4096307818779,
130.303236352713)) ;
#117620=CARTESIAN_POINT('Ctrl Pts',(-23.652457485825,14.4343455417677,130.044847948643)) ;
#117621=CARTESIAN_POINT('Ctrl Pts',(-23.5758603047259,14.3860725443644,
129.78778248944)) ;
#117622=CARTESIAN_POINT('Ctrl Pts',(-23.5071812655722,14.2695097476577,
129.554170604053)) ;
#117623=CARTESIAN_POINT('Ctrl Pts',(-23.4509742936636,14.0917908235827,
129.356799362595)) ;
#117624=CARTESIAN_POINT('Ctrl Pts',(-23.4125523047924,13.8666927964708,
129.211488897753)) ;
#117625=CARTESIAN_POINT('Ctrl Pts',(-23.3951345162908,13.6093229660632,
129.127454830129)) ;
#117626=CARTESIAN_POINT('Ctrl Pts',(-23.4008307641857,13.3388432839998,
129.110977590817)) ;
#117627=CARTESIAN_POINT('Ctrl Pts',(-23.4299496613037,13.0740475195294,
129.162880281939)) ;
#117628=CARTESIAN_POINT('Ctrl Pts',(-23.481199109324,12.8343947236294,129.279432874347)) ;
#117629=CARTESIAN_POINT('Ctrl Pts',(-23.5511581873575,12.6378260096104,
129.450809857318)) ;
#117630=CARTESIAN_POINT('Ctrl Pts',(-23.636245008783,12.496463053358,129.666214477056)) ;
#117631=CARTESIAN_POINT('Ctrl Pts',(-23.7307304012867,12.4217254212934,
129.909104419076)) ;
#117632=CARTESIAN_POINT('Ctrl Pts',(-23.8286224227458,12.4187226067802,
130.161940676462)) ;
#117633=CARTESIAN_POINT('Ctrl Pts',(-23.9235467354779,12.4875916105364,
130.406139022881)) ;
#117634=CARTESIAN_POINT('Ctrl Pts',(-24.0096166464853,12.6235711646796,
130.624432893392)) ;
#117635=CARTESIAN_POINT('Ctrl Pts',(-24.0812256433191,12.8167006668533,
130.800511081773)) ;
#117636=CARTESIAN_POINT('Ctrl Pts',(-24.1340977218945,13.0534699877681,
130.921821215751)) ;
#117637=CARTESIAN_POINT('Ctrl Pts',(-24.1650674975322,13.316652871898,130.979163090976)) ;
#117638=CARTESIAN_POINT('Ctrl Pts',(-24.1726847473952,13.5871780619914,
130.968318503901)) ;
#117639=CARTESIAN_POINT('Ctrl Pts',(-24.1571918674132,13.8461109459276,
130.889950708408)) ;
#117640=CARTESIAN_POINT('Ctrl Pts',(-24.1202020616415,14.0754122507699,
130.748674888431)) ;
#117641=CARTESIAN_POINT('Ctrl Pts',(-24.0654386807843,14.2569964936062,
130.555630868985)) ;
#117642=CARTESIAN_POINT('Ctrl Pts',(-23.9973344144518,14.3792169088182,
130.323565913951)) ;
#117643=CARTESIAN_POINT('Ctrl Pts',(-23.9215531518041,14.4330645733332,
130.069088286981)) ;
#117644=CARTESIAN_POINT('Ctrl Pts',(-23.843935936724,14.4142942248449,129.809113443856)) ;
#117645=CARTESIAN_POINT('Ctrl Pts',(-23.7715313845943,14.3249818846189,
129.564589222325)) ;
#117646=CARTESIAN_POINT('Ctrl Pts',(-23.7092978479596,14.170040968278,129.349514507389)) ;
#117647=CARTESIAN_POINT('Ctrl Pts',(-23.6633746311722,13.9629929132432,
129.182370156649)) ;
#117648=CARTESIAN_POINT('Ctrl Pts',(-23.6370484781814,13.716497262182,129.072318829966)) ;
#117649=CARTESIAN_POINT('Ctrl Pts',(-23.6332221702439,13.4493823964161,
129.028057143487)) ;
#117650=CARTESIAN_POINT('Ctrl Pts',(-23.652907637159,13.1794660173532,129.052361195891)) ;
#117651=CARTESIAN_POINT('Ctrl Pts',(-23.6954564463867,12.9274139550297,
129.14350072815)) ;
#117652=CARTESIAN_POINT('Ctrl Pts',(-23.7583088038747,12.7115777182511,
129.294045622303)) ;
#117653=CARTESIAN_POINT('Ctrl Pts',(-23.8376585992602,12.5463884321844,
129.492816673603)) ;
#117654=CARTESIAN_POINT('Ctrl Pts',(-23.9297100882255,12.4431786925169,
129.728346657304)) ;
#117655=CARTESIAN_POINT('Ctrl Pts',(-24.0264837858184,12.4112124579401,
129.978093638198)) ;
#117656=CARTESIAN_POINT('Ctrl Pts',(-24.1235984898852,12.4513454594276,
130.22859406653)) ;
#117657=CARTESIAN_POINT('Ctrl Pts',(-24.2137616646637,12.5610016830577,
130.458926128585)) ;
#117658=CARTESIAN_POINT('Ctrl Pts',(-24.2917907983411,12.7322315169158,
130.653770957505)) ;
#117659=CARTESIAN_POINT('Ctrl Pts',(-24.3528048425234,12.953682166373,130.798815030454)) ;
#117660=CARTESIAN_POINT('Ctrl Pts',(-24.3927962667222,13.207709520667,130.882592820559)) ;
#117661=CARTESIAN_POINT('Ctrl Pts',(-24.410024457455,13.477838949959,130.899781358164)) ;
#117662=CARTESIAN_POINT('Ctrl Pts',(-24.4036676831234,13.7447249701473,
130.847982315876)) ;
#117663=CARTESIAN_POINT('Ctrl Pts',(-24.375161047068,13.9871378811425,130.731672734363)) ;
#117664=CARTESIAN_POINT('Ctrl Pts',(-24.3270196390184,14.1900736221216,
130.557859433467)) ;
#117665=CARTESIAN_POINT('Ctrl Pts',(-24.2638997897065,14.3373317370972,
130.34047792192)) ;
#117666=CARTESIAN_POINT('Ctrl Pts',(-24.1901979000983,14.4199335161434,
130.091922667675)) ;
#117667=CARTESIAN_POINT('Ctrl Pts',(-24.1128768889176,14.4307824011819,
129.833010984868)) ;
#117668=CARTESIAN_POINT('Ctrl Pts',(-24.0372157103295,14.3690285687369,
129.578691757844)) ;
#117669=CARTESIAN_POINT('Ctrl Pts',(-23.9706215331039,14.240441055026,129.351206228027)) ;
#117670=CARTESIAN_POINT('Ctrl Pts',(-23.9174273385238,14.0528077050883,
129.162661043568)) ;
#117671=CARTESIAN_POINT('Ctrl Pts',(-23.8826973596537,13.8202656328653,
129.028106967362)) ;
#117672=CARTESIAN_POINT('Ctrl Pts',(-23.8694990287969,13.5584446016604,
128.956341170936)) ;
#117673=CARTESIAN_POINT('Ctrl Pts',(-23.8797470733792,13.2871051677591,
128.95309651991)) ;
#117674=CARTESIAN_POINT('Ctrl Pts',(-23.913003929438,13.0271137580964,129.017276092719)) ;
#117675=CARTESIAN_POINT('Ctrl Pts',(-23.9680727824866,12.7938648791111,
129.144962113817)) ;
#117676=CARTESIAN_POINT('Ctrl Pts',(-24.0413879782623,12.6063348860961,
129.32604954485)) ;
#117677=CARTESIAN_POINT('Ctrl Pts',(-24.1287279410253,12.4770288288764,
129.548032891267)) ;
#117678=CARTESIAN_POINT('Ctrl Pts',(-24.224050813435,12.4155889254397,129.793464619769)) ;
#117679=CARTESIAN_POINT('Ctrl Pts',(-24.322359819618,12.4264045620756,130.047353904498)) ;
#117680=CARTESIAN_POINT('Ctrl Pts',(-24.4157726362298,12.5084012335638,
130.287230439798)) ;
#117681=CARTESIAN_POINT('Ctrl Pts',(-24.4995762096403,12.6562045204938,
130.49887414061)) ;
#117682=CARTESIAN_POINT('Ctrl Pts',(-24.5678017919042,12.8582527624523,
130.665140658846)) ;
#117683=CARTESIAN_POINT('Ctrl Pts',(-24.6169191275358,13.1022479915201,
130.775364646435)) ;
#117684=CARTESIAN_POINT('Ctrl Pts',(-24.6434477080034,13.3685510945704,
130.81971558088)) ;
#117685=CARTESIAN_POINT('Ctrl Pts',(-24.6466154461254,13.6374690116671,
130.795980231762)) ;
#117686=CARTESIAN_POINT('Ctrl Pts',(-24.6268337461158,13.8926337185126,
130.70500143045)) ;
#117687=CARTESIAN_POINT('Ctrl Pts',(-24.5862814048627,14.1134973759114,
130.553436720401)) ;
#117688=CARTESIAN_POINT('Ctrl Pts',(-24.5283747688501,14.2854804463777,
130.351062940108)) ;
#117689=CARTESIAN_POINT('Ctrl Pts',(-24.4583502405941,14.3949169663802,
130.113406317305)) ;
#117690=CARTESIAN_POINT('Ctrl Pts',(-24.3820622863036,14.4350950477778,
129.857561187302)) ;
#117691=CARTESIAN_POINT('Ctrl Pts',(-24.3048294246273,14.4027523557503,
129.59869685969)) ;
#117692=CARTESIAN_POINT('Ctrl Pts',(-24.2338934400316,14.3004224268776,
129.358411107523)) ;
#117693=CARTESIAN_POINT('Ctrl Pts',(-24.1743887417905,14.1345848166218,
129.151358775365)) ;
#117694=CARTESIAN_POINT('Ctrl Pts',(-24.1318770833654,13.9188292644318,
128.994144267598)) ;
#117695=CARTESIAN_POINT('Ctrl Pts',(-24.109670314531,13.6668968300226,128.896125378668)) ;
#117696=CARTESIAN_POINT('Ctrl Pts',(-24.1102335611594,13.3982258229591,
128.864722114506)) ;
#117697=CARTESIAN_POINT('Ctrl Pts',(-24.1343637033151,13.1299460140076,
128.901983111348)) ;
#117698=CARTESIAN_POINT('Ctrl Pts',(-24.1808902872214,12.883706046321,129.004806420228)) ;
#117699=CARTESIAN_POINT('Ctrl Pts',(-24.2474801294373,12.6755091493533,
129.166133279341)) ;
#117700=CARTESIAN_POINT('Ctrl Pts',(-24.3295734455692,12.5215778727762,
129.372898584267)) ;
#117701=CARTESIAN_POINT('Ctrl Pts',(-24.4227739567097,12.4317802296238,
129.611941575593)) ;
#117702=CARTESIAN_POINT('Ctrl Pts',(-24.5199503056922,12.4131805085562,
129.862866562425)) ;
#117703=CARTESIAN_POINT('Ctrl Pts',(-24.6163436963673,12.4668842419267,
130.111240618795)) ;
#117704=CARTESIAN_POINT('Ctrl Pts',(-24.7045015836318,12.5884449970434,
130.335774968224)) ;
#117705=CARTESIAN_POINT('Ctrl Pts',(-24.7800708345001,12.7713420307832,
130.523219246622)) ;
#117706=CARTESIAN_POINT('Ctrl Pts',(-24.8370070768286,12.9988617172705,
130.656586079874)) ;
#117707=CARTESIAN_POINT('Ctrl Pts',(-24.8731099788845,13.2594912156624,
130.728709369952)) ;
#117708=CARTESIAN_POINT('Ctrl Pts',(-24.8856748885241,13.528913215532,130.73246060921)) ;
#117709=CARTESIAN_POINT('Ctrl Pts',(-24.8750994611493,13.7920446626032,
130.668445308032)) ;
#117710=CARTESIAN_POINT('Ctrl Pts',(-24.8426663011521,14.0286822474636,
130.540601272058)) ;
#117711=CARTESIAN_POINT('Ctrl Pts',(-24.7911779391248,14.2226476411148,
130.356949256475)) ;
#117712=CARTESIAN_POINT('Ctrl Pts',(-24.7256794891725,14.3581279629795,
130.132601154518)) ;
#117713=CARTESIAN_POINT('Ctrl Pts',(-24.6510859996418,14.4275172103506,
129.881595712007)) ;
#117714=CARTESIAN_POINT('Ctrl Pts',(-24.5730285429095,14.4244373538993,
129.620235686296)) ;
#117715=CARTESIAN_POINT('Ctrl Pts',(-24.4992922348247,14.3501368659966,
129.371907663713)) ;
#117716=CARTESIAN_POINT('Ctrl Pts',(-24.4343894489451,14.2089998659338,
129.149115926751)) ;
#117717=CARTESIAN_POINT('Ctrl Pts',(-24.3845042562601,14.0121252002097,
128.970331894925)) ;
#117718=CARTESIAN_POINT('Ctrl Pts',(-24.3535289344495,13.771824837408,128.846599032895)) ;
#117719=CARTESIAN_POINT('Ctrl Pts',(-24.3447605801122,13.5078187869416,
128.787925053611)) ;
#117720=CARTESIAN_POINT('Ctrl Pts',(-24.3593374965893,13.2372790594901,
128.797377589244)) ;
#117721=CARTESIAN_POINT('Ctrl Pts',(-24.3968788753453,12.9804327969093,
128.873981225353)) ;
#117722=CARTESIAN_POINT('Ctrl Pts',(-24.4559404822289,12.7540239326364,
129.013240141807)) ;
#117723=CARTESIAN_POINT('Ctrl Pts',(-24.531902751001,12.5774627760268,129.202214044801)) ;
#117724=CARTESIAN_POINT('Ctrl Pts',(-24.6214579569672,12.4598743078943,
129.43058501997)) ;
#117725=CARTESIAN_POINT('Ctrl Pts',(-24.7180157878552,12.4120040784052,
129.679516293973)) ;
#117726=CARTESIAN_POINT('Ctrl Pts',(-24.8154715108942,12.4365719244432,
129.931101642148)) ;
#117727=CARTESIAN_POINT('Ctrl Pts',(-24.9074801725979,12.5311793554758,
130.166872263273)) ;
#117728=CARTESIAN_POINT('Ctrl Pts',(-24.98908833934,12.6910252858477,130.371967891418)) ;
#117729=CARTESIAN_POINT('Ctrl Pts',(-25.0537128322214,12.9015545976397,
130.527790346717)) ;
#117730=CARTESIAN_POINT('Ctrl Pts',(-25.0987003896927,13.1503193803916,
130.62606971385)) ;
#117731=CARTESIAN_POINT('Ctrl Pts',(-25.1209633642502,13.4198238208766,
130.657834390399)) ;
#117732=CARTESIAN_POINT('Ctrl Pts',(-25.1197436702009,13.6867201897118,
130.621358969948)) ;
#117733=CARTESIAN_POINT('Ctrl Pts',(-25.0957857760177,13.9376559886512,
130.518082389912)) ;
#117734=CARTESIAN_POINT('Ctrl Pts',(-25.0516131934043,14.15024285779,130.35593488202)) ;
#117735=CARTESIAN_POINT('Ctrl Pts',(-24.9911921923722,14.3108380618515,
130.146327637034)) ;
#117736=CARTESIAN_POINT('Ctrl Pts',(-24.9194794299346,14.4079445273837,
129.903726724708)) ;
#117737=CARTESIAN_POINT('Ctrl Pts',(-24.8423372287212,14.4345276708083,
129.645254031341)) ;
#117738=CARTESIAN_POINT('Ctrl Pts',(-24.7661334231012,14.3888298887491,
129.389568134777)) ;
#117739=CARTESIAN_POINT('Ctrl Pts',(-24.6967794246489,14.2738285073071,
129.153813837603)) ;
#117740=CARTESIAN_POINT('Ctrl Pts',(-24.6402004549822,14.0978368978208,
128.955396136012)) ;
#117741=CARTESIAN_POINT('Ctrl Pts',(-24.6011334207155,13.873540820756,128.808139971139)) ;
#117742=CARTESIAN_POINT('Ctrl Pts',(-24.5831027131497,13.6168751421622,
128.72232648238)) ;
#117743=CARTESIAN_POINT('Ctrl Pts',(-24.588135943568,13.3465065043273,128.703910280374)) ;
#117744=CARTESIAN_POINT('Ctrl Pts',(-24.616558912276,13.0815409163059,128.753816302396)) ;
#117745=CARTESIAN_POINT('Ctrl Pts',(-24.6671939709622,12.8409648020749,
128.868577387027)) ;
#117746=CARTESIAN_POINT('Ctrl Pts',(-24.7365720466203,12.6428641094173,
129.038275126448)) ;
#117747=CARTESIAN_POINT('Ctrl Pts',(-24.822005129513,12.4989647241715,129.254437227158)) ;
#117748=CARTESIAN_POINT('Ctrl Pts',(-24.9154535440393,12.423107716889,129.494606388429)) ;
#117749=CARTESIAN_POINT('Ctrl Pts',(-25.0137167725077,12.4177381354183,
129.748391405694)) ;
#117750=CARTESIAN_POINT('Ctrl Pts',(-25.1087445130681,12.4847094665518,
129.992915516142)) ;
#117751=CARTESIAN_POINT('Ctrl Pts',(-25.1952478577146,12.6190666936061,
130.212434292899)) ;
#117752=CARTESIAN_POINT('Ctrl Pts',(-25.2672601104286,12.8107470171755,
130.389708558821)) ;
#117753=CARTESIAN_POINT('Ctrl Pts',(-25.3206363863023,13.046104708988,130.512545094294)) ;
#117754=CARTESIAN_POINT('Ctrl Pts',(-25.3522895929508,13.3089102809665,
130.571865598048)) ;
#117755=CARTESIAN_POINT('Ctrl Pts',(-25.3605922534063,13.5795916473862,
130.563012299063)) ;
#117756=CARTESIAN_POINT('Ctrl Pts',(-25.3456591401498,13.8398547760041,
130.486182706922)) ;
#117757=CARTESIAN_POINT('Ctrl Pts',(-25.3091876372828,14.0698648400938,
130.346452999807)) ;
#117758=CARTESIAN_POINT('Ctrl Pts',(-25.2550551240209,14.2524395531566,
130.155354875779)) ;
#117759=CARTESIAN_POINT('Ctrl Pts',(-25.1870939300536,14.3767942781604,
129.923628056113)) ;
#117760=CARTESIAN_POINT('Ctrl Pts',(-25.1116370247179,14.4324209526977,
129.670183261114)) ;
#117761=CARTESIAN_POINT('Ctrl Pts',(-25.0340417226102,14.4159981333991,
129.410303004524)) ;
#117762=CARTESIAN_POINT('Ctrl Pts',(-24.9611806568547,14.3283155565982,
129.164334994584)) ;
#117763=CARTESIAN_POINT('Ctrl Pts',(-24.8987771733635,14.1755659528296,
128.948873846864)) ;
#117764=CARTESIAN_POINT('Ctrl Pts',(-24.852262446507,13.9699068567355,128.779985228531)) ;
#117765=CARTESIAN_POINT('Ctrl Pts',(-24.8252895194219,13.7239840394015,
128.668003026794)) ;
#117766=CARTESIAN_POINT('Ctrl Pts',(-24.8207605382176,13.4571373132025,
128.62168264824)) ;
#117767=CARTESIAN_POINT('Ctrl Pts',(-24.8399553561379,13.1860385292999,
128.644424296114)) ;
#117768=CARTESIAN_POINT('Ctrl Pts',(-24.8815110859698,12.9351633483058,
128.73292877833)) ;
#117769=CARTESIAN_POINT('Ctrl Pts',(-24.9443125871162,12.7162804285951,
128.883050489914)) ;
#117770=CARTESIAN_POINT('Ctrl Pts',(-25.0229415062978,12.5504602957499,
129.079875923212)) ;
#117771=CARTESIAN_POINT('Ctrl Pts',(-25.1147675609777,12.445157177056,129.314722815811)) ;
#117772=CARTESIAN_POINT('Ctrl Pts',(-25.2113285559774,12.4110818139133,
129.563897712835)) ;
#117773=CARTESIAN_POINT('Ctrl Pts',(-25.3088356645265,12.4493848627241,
129.815436071975)) ;
#117774=CARTESIAN_POINT('Ctrl Pts',(-25.3987988307639,12.5564279113244,
130.045368057642)) ;
#117775=CARTESIAN_POINT('Ctrl Pts',(-25.4777792677189,12.7270948639173,
130.242770584934)) ;
#117776=CARTESIAN_POINT('Ctrl Pts',(-25.5390833290002,12.9467013244188,
130.388779692745)) ;
#117777=CARTESIAN_POINT('Ctrl Pts',(-25.579809192093,13.2005745310841,130.474625025538)) ;
#117778=CARTESIAN_POINT('Ctrl Pts',(-25.597592152945,13.4697555759231,130.493529148036)) ;
#117779=CARTESIAN_POINT('Ctrl Pts',(-25.5920655494427,13.7362551955502,
130.444265292038)) ;
#117780=CARTESIAN_POINT('Ctrl Pts',(-25.5639199870897,13.9814041489959,
130.328750855533)) ;
#117781=CARTESIAN_POINT('Ctrl Pts',(-25.5166557810706,14.1841666435664,
130.157762612529)) ;
#117782=CARTESIAN_POINT('Ctrl Pts',(-25.4535179771181,14.3343211623714,
129.940098533994)) ;
#117783=CARTESIAN_POINT('Ctrl Pts',(-25.3802391406752,14.418455096693,129.692893970139)) ;
#117784=CARTESIAN_POINT('Ctrl Pts',(-25.3029064752514,14.4314520041057,
129.433922593139)) ;
#117785=CARTESIAN_POINT('Ctrl Pts',(-25.227398337514,14.3721435581282,129.180190901468)) ;
#117786=CARTESIAN_POINT('Ctrl Pts',(-25.1602216705886,14.2453739060394,
128.950905918899)) ;
#117787=CARTESIAN_POINT('Ctrl Pts',(-25.1063450402745,14.0581567741166,
128.760203803333)) ;
#117788=CARTESIAN_POINT('Ctrl Pts',(-25.0712590260961,13.8276969055429,
128.624767412558)) ;
#117789=CARTESIAN_POINT('Ctrl Pts',(-25.0573457795135,13.5670204809412,
128.550974352564)) ;
#117790=CARTESIAN_POINT('Ctrl Pts',(-25.0668582109147,13.2953787817414,
128.545543170318)) ;
#117791=CARTESIAN_POINT('Ctrl Pts',(-25.0994943187018,13.0342215951602,
128.607838884911)) ;
#117792=CARTESIAN_POINT('Ctrl Pts',(-25.1542507866729,12.7992353621788,
128.734494690188)) ;
#117793=CARTESIAN_POINT('Ctrl Pts',(-25.22669838614,12.6113833751158,128.913239507721)) ;
#117794=CARTESIAN_POINT('Ctrl Pts',(-25.3137534702574,12.4798504311987,
129.13435679031)) ;
#117795=CARTESIAN_POINT('Ctrl Pts',(-25.4091104699422,12.4163978737343,
129.379824853837)) ;
#117796=CARTESIAN_POINT('Ctrl Pts',(-25.50711720003,12.4249214769568,129.632945439815)) ;
#117797=CARTESIAN_POINT('Ctrl Pts',(-25.6012113649615,12.5053755581291,
129.874638598727)) ;
#117798=CARTESIAN_POINT('Ctrl Pts',(-25.6849597712776,12.6507858524343,
130.086285179288)) ;
#117799=CARTESIAN_POINT('Ctrl Pts',(-25.7538861814578,12.8517470379754,
130.254524032593)) ;
#117800=CARTESIAN_POINT('Ctrl Pts',(-25.8035309429625,13.0945613893121,
130.366327420662)) ;
#117801=CARTESIAN_POINT('Ctrl Pts',(-25.8308038778984,13.3602125815229,
130.412879679802)) ;
#117802=CARTESIAN_POINT('Ctrl Pts',(-25.8345999378769,13.6310671509035,
130.390757628165)) ;
#117803=CARTESIAN_POINT('Ctrl Pts',(-25.8155083574025,13.8852753501133,
130.302003918844)) ;
#117804=CARTESIAN_POINT('Ctrl Pts',(-25.7755392118652,14.1076160518456,
130.152115623541)) ;
#117805=CARTESIAN_POINT('Ctrl Pts',(-25.7181892166743,14.2808806548592,
129.951435285494)) ;
#117806=CARTESIAN_POINT('Ctrl Pts',(-25.6484959082951,14.3926567066995,
129.714749299653)) ;
#117807=CARTESIAN_POINT('Ctrl Pts',(-25.5717128930641,14.4348969494453,
129.457198833214)) ;
#117808=CARTESIAN_POINT('Ctrl Pts',(-25.4951381495962,14.4049966963277,
129.20058472654)) ;
#117809=CARTESIAN_POINT('Ctrl Pts',(-25.4232962621115,14.303792887026,128.957344138201)) ;
#117810=CARTESIAN_POINT('Ctrl Pts',(-25.363824625125,14.1405203843961,128.750619307371)) ;
#117811=CARTESIAN_POINT('Ctrl Pts',(-25.3206339986258,13.925819103477,128.591354682337)) ;
#117812=CARTESIAN_POINT('Ctrl Pts',(-25.2977692410781,13.6747404913737,
128.491427879832)) ;
#117813=CARTESIAN_POINT('Ctrl Pts',(-25.2977339239315,13.4052256729127,
128.458138778975)) ;
#117814=CARTESIAN_POINT('Ctrl Pts',(-25.3209945002928,13.1384692552609,
128.493096955899)) ;
#117815=CARTESIAN_POINT('Ctrl Pts',(-25.3671694617792,12.8897551675282,
128.59467494241)) ;
#117816=CARTESIAN_POINT('Ctrl Pts',(-25.4329175346433,12.6813708112152,
128.753721852147)) ;
#117817=CARTESIAN_POINT('Ctrl Pts',(-25.5147153277118,12.5252896551219,
128.959563529951)) ;
#117818=CARTESIAN_POINT('Ctrl Pts',(-25.6074698502328,12.4335762169434,
129.197379956762)) ;
#117819=CARTESIAN_POINT('Ctrl Pts',(-25.7049185069326,12.4126069646067,
129.448987978284)) ;
#117820=CARTESIAN_POINT('Ctrl Pts',(-25.8016946801806,12.4645413585742,
129.698394833031)) ;
#117821=CARTESIAN_POINT('Ctrl Pts',(-25.8901180162125,12.5845282308657,
129.923698284889)) ;
#117822=CARTESIAN_POINT('Ctrl Pts',(-25.965890991119,12.7652450506007,130.111852309267)) ;
#117823=CARTESIAN_POINT('Ctrl Pts',(-26.0234875630242,12.9922346613826,
130.247067297209)) ;
#117824=CARTESIAN_POINT('Ctrl Pts',(-26.0600124784417,13.250181771579,130.32068333464)) ;
#117825=CARTESIAN_POINT('Ctrl Pts',(-26.0734713454908,13.5208712081626,
130.326877389697)) ;
#117826=CARTESIAN_POINT('Ctrl Pts',(-26.0634750774189,13.7852947823376,
130.264454593183)) ;
#117827=CARTESIAN_POINT('Ctrl Pts',(-26.0315363440698,14.0230293048616,
130.13802460234)) ;
#117828=CARTESIAN_POINT('Ctrl Pts',(-25.9806388976771,14.2178153725244,
129.956187274352)) ;
#117829=CARTESIAN_POINT('Ctrl Pts',(-25.915484310865,14.3552930120595,129.732836491923)) ;
#117830=CARTESIAN_POINT('Ctrl Pts',(-25.84072829782,14.4265292407486,129.481215829229)) ;
#117831=CARTESIAN_POINT('Ctrl Pts',(-25.7635624076654,14.4257522410885,
129.222849529606)) ;
#117832=CARTESIAN_POINT('Ctrl Pts',(-25.6889769434919,14.3531912390316,
128.97174979562)) ;
#117833=CARTESIAN_POINT('Ctrl Pts',(-25.6238945066486,14.2139749778386,
128.748514598009)) ;
#117834=CARTESIAN_POINT('Ctrl Pts',(-25.5734229709391,14.0181343967752,
128.567943742831)) ;
#117835=CARTESIAN_POINT('Ctrl Pts',(-25.5419558649472,13.7796846047307,
128.442897581117)) ;
#117836=CARTESIAN_POINT('Ctrl Pts',(-25.532465946712,13.5155236952114,128.38203152979)) ;
#117837=CARTESIAN_POINT('Ctrl Pts',(-25.5463615849931,13.2452127497976,
128.38953676012)) ;
#117838=CARTESIAN_POINT('Ctrl Pts',(-25.5832346236961,12.9877059092876,
128.464185979317)) ;
#117839=CARTESIAN_POINT('Ctrl Pts',(-25.6416547744771,12.7602061146998,
128.601594688484)) ;
#117840=CARTESIAN_POINT('Ctrl Pts',(-25.7173212787246,12.5817513014504,
128.789638745255)) ;
#117841=CARTESIAN_POINT('Ctrl Pts',(-25.8062865385756,12.4625557645347,
129.016393612117)) ;
#117842=CARTESIAN_POINT('Ctrl Pts',(-25.9028561833619,12.4124303731174,
129.265304380517)) ;
#117843=CARTESIAN_POINT('Ctrl Pts',(-26.0002209633361,12.4345388042572,
129.516686941127)) ;
#117844=CARTESIAN_POINT('Ctrl Pts',(-26.0932622644251,12.5283216388457,
129.755168414136)) ;
#117845=CARTESIAN_POINT('Ctrl Pts',(-26.1743660605688,12.6848122289345,
129.95915801482)) ;
#117846=CARTESIAN_POINT('Ctrl Pts',(-26.2401044733367,12.8954782844364,
130.117969955362)) ;
#117847=CARTESIAN_POINT('Ctrl Pts',(-26.2854752226399,13.1430312169486,
130.217447678816)) ;
#117848=CARTESIAN_POINT('Ctrl Pts',(-26.3084010697088,13.4109716006735,
130.251296348672)) ;
#117849=CARTESIAN_POINT('Ctrl Pts',(-26.3079132586112,13.6794257001286,
130.216804302598)) ;
#117850=CARTESIAN_POINT('Ctrl Pts',(-26.2844685673034,13.9314101129575,
130.114982755367)) ;
#117851=CARTESIAN_POINT('Ctrl Pts',(-26.2409654932688,14.1445006499188,
129.954904200554)) ;
#117852=CARTESIAN_POINT('Ctrl Pts',(-26.1810638490843,14.30675364297,129.746853736739)) ;
#117853=CARTESIAN_POINT('Ctrl Pts',(-26.1095277456812,14.4060487021468,
129.504729024047)) ;
#117854=CARTESIAN_POINT('Ctrl Pts',(-26.032393842977,14.4348548844435,129.246256945444)) ;
#117855=CARTESIAN_POINT('Ctrl Pts',(-25.9558698637576,14.3909041683382,
128.989537588897)) ;
#117856=CARTESIAN_POINT('Ctrl Pts',(-25.8865418310219,14.2783347545864,
128.754011972375)) ;
#117857=CARTESIAN_POINT('Ctrl Pts',(-25.8292402720525,14.1031935593991,
128.553327018804)) ;
#117858=CARTESIAN_POINT('Ctrl Pts',(-25.7897294043971,13.8800104934357,
128.404795472586)) ;
#117859=CARTESIAN_POINT('Ctrl Pts',(-25.7711135585255,13.6249527950758,
128.317389710907)) ;
#117860=CARTESIAN_POINT('Ctrl Pts',(-25.775431115054,13.3547990721566,128.296889369296)) ;
#117861=CARTESIAN_POINT('Ctrl Pts',(-25.8030534354026,13.0897727529312,
128.34451204004)) ;
#117862=CARTESIAN_POINT('Ctrl Pts',(-25.8533593061976,12.8467550013015,
128.458114990692)) ;
#117863=CARTESIAN_POINT('Ctrl Pts',(-25.9222441241804,12.6478124741987,
128.626416287819)) ;
#117864=CARTESIAN_POINT('Ctrl Pts',(-26.0066708855511,12.5027972402551,
128.839866149716)) ;
#117865=CARTESIAN_POINT('Ctrl Pts',(-26.100698614946,12.4240443790735,129.08144772251)) ;
#117866=CARTESIAN_POINT('Ctrl Pts',(-26.199005934577,12.4170503512975,129.335345715064)) ;
#117867=CARTESIAN_POINT('Ctrl Pts',(-26.2938294993792,12.4817913528845,
129.579397911555)) ;
#117868=CARTESIAN_POINT('Ctrl Pts',(-26.3806964957364,12.6142900077789,
129.799971178623)) ;
#117869=CARTESIAN_POINT('Ctrl Pts',(-26.4531055700923,12.8042102941726,
129.978446194113)) ;
#117870=CARTESIAN_POINT('Ctrl Pts',(-26.5072159038126,13.0388185676317,
130.10337532566)) ;
#117871=CARTESIAN_POINT('Ctrl Pts',(-26.5395617534597,13.302328429414,130.164572555535)) ;
#117872=CARTESIAN_POINT('Ctrl Pts',(-26.5484551324724,13.5713413202646,
130.157656507272)) ;
#117873=CARTESIAN_POINT('Ctrl Pts',(-26.5341679133082,13.8329961698972,
130.082609782339)) ;
#117874=CARTESIAN_POINT('Ctrl Pts',(-26.4983425431364,14.0635775985236,
129.944847992396)) ;
#117875=CARTESIAN_POINT('Ctrl Pts',(-26.4445874292823,14.2479536598407,
129.754795364822)) ;
#117876=CARTESIAN_POINT('Ctrl Pts',(-26.3771852728711,14.3739504234545,
129.524813623163)) ;
#117877=CARTESIAN_POINT('Ctrl Pts',(-26.3012446932142,14.4320428147267,
129.269680538412)) ;
#117878=CARTESIAN_POINT('Ctrl Pts',(-26.2238185485464,14.4172275166343,
129.010384196713)) ;
#117879=CARTESIAN_POINT('Ctrl Pts',(-26.15101057134,14.3318167265824,128.764684803711)) ;
#117880=CARTESIAN_POINT('Ctrl Pts',(-26.0882559725209,14.1811818661954,
128.548240904809)) ;
#117881=CARTESIAN_POINT('Ctrl Pts',(-26.0410539159268,13.9759968010836,
128.377204526979)) ;
#117882=CARTESIAN_POINT('Ctrl Pts',(-26.0135036934613,13.7313492742168,
128.263597377545)) ;
#117883=CARTESIAN_POINT('Ctrl Pts',(-26.008446515134,13.4634561374574,128.21555732586)) ;
#117884=CARTESIAN_POINT('Ctrl Pts',(-26.0266130110227,13.1958849564785,
128.235768690404)) ;
#117885=CARTESIAN_POINT('Ctrl Pts',(-26.0679474653962,12.9412337113468,
128.323225935666)) ;
#117886=CARTESIAN_POINT('Ctrl Pts',(-26.1296373289063,12.7230235201935,
128.470412014427)) ;
#117887=CARTESIAN_POINT('Ctrl Pts',(-26.2085605635285,12.5539648159992,
128.667776639854)) ;
#117888=CARTESIAN_POINT('Ctrl Pts',(-26.2991512181213,12.4477725871464,
128.899377928494)) ;
#117889=CARTESIAN_POINT('Ctrl Pts',(-26.3963261077533,12.4110238125286,
129.150087833756)) ;
#117890=CARTESIAN_POINT('Ctrl Pts',(-26.4934436652944,12.4468710259381,
129.400669592641)) ;
#117891=CARTESIAN_POINT('Ctrl Pts',(-26.5846169547544,12.5531554017273,
129.633780736787)) ;
#117892=CARTESIAN_POINT('Ctrl Pts',(-26.6633533642397,12.7211113672027,
129.830735256764)) ;
#117893=CARTESIAN_POINT('Ctrl Pts',(-26.7254238754428,12.9400020306265,
129.978881349517)) ;
#117894=CARTESIAN_POINT('Ctrl Pts',(-26.7666245201816,13.1921120605742,
130.066251668361)) ;
#117895=CARTESIAN_POINT('Ctrl Pts',(-26.7852369169418,13.4620045410206,
130.087464045505)) ;
#117896=CARTESIAN_POINT('Ctrl Pts',(-26.7802665924524,13.7292706250682,
130.039767932798)) ;
#117897=CARTESIAN_POINT('Ctrl Pts',(-26.7529733274785,13.9738125834417,
129.926960110945)) ;
#117898=CARTESIAN_POINT('Ctrl Pts',(-26.705968775378,14.1794946936577,129.756508727605)) ;
#117899=CARTESIAN_POINT('Ctrl Pts',(-26.6430636408078,14.3311259021016,
129.539493754098)) ;
#117900=CARTESIAN_POINT('Ctrl Pts',(-26.5704211107655,14.4169205484559,
129.294336057586)) ;
#117901=CARTESIAN_POINT('Ctrl Pts',(-26.4926800660124,14.4320030369242,
129.033973746762)) ;
#117902=CARTESIAN_POINT('Ctrl Pts',(-26.4174411143122,14.3751243958677,
128.781224876368)) ;
#117903=CARTESIAN_POINT('Ctrl Pts',(-26.3493726747927,14.2488768695212,
128.549025048048)) ;
#117904=CARTESIAN_POINT('Ctrl Pts',(-26.295605612608,14.0648019477406,128.35897170667)) ;
#117905=CARTESIAN_POINT('Ctrl Pts',(-26.2596692630275,13.8343789431172,
128.22087036974)) ;
#117906=CARTESIAN_POINT('Ctrl Pts',(-26.2452033860871,13.5736072409061,
128.145398162508)) ;
#117907=CARTESIAN_POINT('Ctrl Pts',(-26.2541085207153,13.3025526358433,
128.138259705612)) ;
#117908=CARTESIAN_POINT('Ctrl Pts',(-26.2860045190759,13.0417946956511,
128.198505035509)) ;
#117909=CARTESIAN_POINT('Ctrl Pts',(-26.3399102327703,12.8063141545274,
128.322778456193)) ;
#117910=CARTESIAN_POINT('Ctrl Pts',(-26.4121917469191,12.6158857625783,
128.50087637384)) ;
#117911=CARTESIAN_POINT('Ctrl Pts',(-26.4990876279591,12.4825397359329,
128.721479595999)) ;
#117912=CARTESIAN_POINT('Ctrl Pts',(-26.5940129888447,12.4173081349344,
128.965781411473)) ;
#117913=CARTESIAN_POINT('Ctrl Pts',(-26.6919317707314,12.4236049843711,
129.218679452647)) ;
#117914=CARTESIAN_POINT('Ctrl Pts',(-26.7861947841509,12.5018025571804,
129.460884921511)) ;
#117915=CARTESIAN_POINT('Ctrl Pts',(-26.8705874596301,12.6458565227928,
129.674307979368)) ;
#117916=CARTESIAN_POINT('Ctrl Pts',(-26.9399304853391,12.8453790155913,
129.843785872194)) ;
#117917=CARTESIAN_POINT('Ctrl Pts',(-26.990100746493,13.0865651955858,129.957208344523)) ;
#117918=CARTESIAN_POINT('Ctrl Pts',(-27.018102279043,13.3521426916341,130.005841189711)) ;
#117919=CARTESIAN_POINT('Ctrl Pts',(-27.02263465622,13.6222556634887,129.985982518834)) ;
#117920=CARTESIAN_POINT('Ctrl Pts',(-27.0041811090057,13.8783882532463,
129.898944093898)) ;
#117921=CARTESIAN_POINT('Ctrl Pts',(-26.9646335695461,14.1022120327878,
129.750227079902)) ;
#117922=CARTESIAN_POINT('Ctrl Pts',(-26.9078686115122,14.2765229338953,
129.551349815167)) ;
#117923=CARTESIAN_POINT('Ctrl Pts',(-26.8385567991512,14.3902286899454,
129.315812307096)) ;
#117924=CARTESIAN_POINT('Ctrl Pts',(-26.7617716565815,14.4347769429382,
129.058208230924)) ;
#117925=CARTESIAN_POINT('Ctrl Pts',(-26.6849778202196,14.4066722645431,
128.800883546346)) ;
#117926=CARTESIAN_POINT('Ctrl Pts',(-26.613309272385,14.3082119147666,128.558359128021)) ;
#117927=CARTESIAN_POINT('Ctrl Pts',(-26.5531000001099,14.1460357865502,
128.349317353602)) ;
#117928=CARTESIAN_POINT('Ctrl Pts',(-26.5094126533137,13.9328084550501,
128.188640550554)) ;
#117929=CARTESIAN_POINT('Ctrl Pts',(-26.4858992546912,13.6817741223337,
128.086718384594)) ;
#117930=CARTESIAN_POINT('Ctrl Pts',(-26.4851402376145,13.4140262375942,
128.051507824856)) ;
#117931=CARTESIAN_POINT('Ctrl Pts',(-26.507882004842,13.1453688529206,128.084742838808)) ;
#117932=CARTESIAN_POINT('Ctrl Pts',(-26.553013805695,12.8977836855868,128.183554680704)) ;
#117933=CARTESIAN_POINT('Ctrl Pts',(-26.6187173976324,12.6861562793818,
128.342188636974)) ;
#117934=CARTESIAN_POINT('Ctrl Pts',(-26.7000075083532,12.5289208756677,
128.546622742812)) ;
#117935=CARTESIAN_POINT('Ctrl Pts',(-26.7926271999993,12.4351549245617,
128.784006318656)) ;
#117936=CARTESIAN_POINT('Ctrl Pts',(-26.8898002619232,12.4122393500749,
129.034886075764)) ;
#117937=CARTESIAN_POINT('Ctrl Pts',(-26.9866994174481,12.4619213661245,
129.284657255046)) ;
#117938=CARTESIAN_POINT('Ctrl Pts',(-27.0756287380429,12.5803996271663,
129.511357053754)) ;
#117939=CARTESIAN_POINT('Ctrl Pts',(-27.1516505419193,12.7591298548141,
129.700322405224)) ;
#117940=CARTESIAN_POINT('Ctrl Pts',(-27.2098817946148,12.9850686452271,
129.837367763896)) ;
#117941=CARTESIAN_POINT('Ctrl Pts',(-27.2470544937516,13.2423776276029,
129.912878159897)) ;
#117942=CARTESIAN_POINT('Ctrl Pts',(-27.2611859668007,13.5129448157843,
129.921038532251)) ;
#117943=CARTESIAN_POINT('Ctrl Pts',(-27.2519206533289,13.77743197275,129.860810679802)) ;
#117944=CARTESIAN_POINT('Ctrl Pts',(-27.2205158418916,14.0166133244865,
129.73587144029)) ;
#117945=CARTESIAN_POINT('Ctrl Pts',(-27.1704319083102,14.2120829890599,
129.556582398162)) ;
#117946=CARTESIAN_POINT('Ctrl Pts',(-27.1051769675512,14.3524988741423,
129.332692223217)) ;
#117947=CARTESIAN_POINT('Ctrl Pts',(-27.0308341297757,14.4253825551606,
129.082395350761)) ;
#117948=CARTESIAN_POINT('Ctrl Pts',(-26.9535452058579,14.4267683079455,
128.823609311485)) ;
#117949=CARTESIAN_POINT('Ctrl Pts',(-26.8789617854659,14.3564920605334,
128.572604483849)) ;
#117950=CARTESIAN_POINT('Ctrl Pts',(-26.8132943369783,14.2186720033249,
128.347542708609)) ;
#117951=CARTESIAN_POINT('Ctrl Pts',(-26.7623884221237,14.024316870989,128.165726044755)) ;
#117952=CARTESIAN_POINT('Ctrl Pts',(-26.7303308114293,13.7866137007774,
128.038923620383)) ;
#117953=CARTESIAN_POINT('Ctrl Pts',(-26.7202102299333,13.5238037993467,
127.976325040153)) ;
#117954=CARTESIAN_POINT('Ctrl Pts',(-26.7333939658771,13.2527086934904,
127.981667146045)) ;
#117955=CARTESIAN_POINT('Ctrl Pts',(-26.7698781643314,12.9936531386933,
128.05504873943)) ;
#117956=CARTESIAN_POINT('Ctrl Pts',(-26.8274902750571,12.7662442453604,
128.190263050934)) ;
#117957=CARTESIAN_POINT('Ctrl Pts',(-26.9028158586766,12.5858801794281,
128.377254060625)) ;
#117958=CARTESIAN_POINT('Ctrl Pts',(-26.9915580162282,12.4648530906934,
128.603338840857)) ;
#117959=CARTESIAN_POINT('Ctrl Pts',(-27.0881560037959,12.4128201898405,
128.852283164429)) ;
#117960=CARTESIAN_POINT('Ctrl Pts',(-27.1851902816751,12.4330274008567,
129.102825190585)) ;
#117961=CARTESIAN_POINT('Ctrl Pts',(-27.2780530128695,12.5240123078526,
129.340946985109)) ;
#117962=CARTESIAN_POINT('Ctrl Pts',(-27.3600745221437,12.6795221093343,
129.547422309088)) ;
#117963=CARTESIAN_POINT('Ctrl Pts',(-27.4262707883137,12.8889213981569,
129.707582915231)) ;
#117964=CARTESIAN_POINT('Ctrl Pts',(-27.4722816893973,13.1354946974878,
129.80894186709)) ;
#117965=CARTESIAN_POINT('Ctrl Pts',(-27.495909604768,13.4042911387148,129.844701076616)) ;
#117966=CARTESIAN_POINT('Ctrl Pts',(-27.4959972441499,13.6719452303359,
129.812014408763)) ;
#117967=CARTESIAN_POINT('Ctrl Pts',(-27.4732881371598,13.9242175359662,
129.712414853415)) ;
#117968=CARTESIAN_POINT('Ctrl Pts',(-27.4302643966516,14.1390288765416,
129.553676677621)) ;
#117969=CARTESIAN_POINT('Ctrl Pts',(-27.3707186087652,14.3030286155002,
129.346643794136)) ;
#117970=CARTESIAN_POINT('Ctrl Pts',(-27.2993922220818,14.4041953321141,
129.105118341883)) ;
#117971=CARTESIAN_POINT('Ctrl Pts',(-27.2225719034685,14.4349854776255,
128.847663054287)) ;
#117972=CARTESIAN_POINT('Ctrl Pts',(-27.1459254586502,14.3934046912769,
128.590588216205)) ;
#117973=CARTESIAN_POINT('Ctrl Pts',(-27.0760780136377,14.2822103213118,
128.353421767456)) ;
#117974=CARTESIAN_POINT('Ctrl Pts',(-27.0186893527385,14.1097942547729,
128.152689099485)) ;
#117975=CARTESIAN_POINT('Ctrl Pts',(-26.9784352679952,13.8877667397205,
128.001937919195)) ;
#117976=CARTESIAN_POINT('Ctrl Pts',(-26.9591052561151,13.6324084843775,
127.912318673804)) ;
#117977=CARTESIAN_POINT('Ctrl Pts',(-26.9627611736166,13.362418602374,127.88989100727)) ;
#117978=CARTESIAN_POINT('Ctrl Pts',(-26.9898328416053,13.0965815355502,
127.935846808179)) ;
#117979=CARTESIAN_POINT('Ctrl Pts',(-27.039223966776,12.8540736750208,128.046978106092)) ;
#117980=CARTESIAN_POINT('Ctrl Pts',(-27.1076603275563,12.6529924848678,
128.213894702152)) ;
#117981=CARTESIAN_POINT('Ctrl Pts',(-27.1922326941678,12.5055874669249,
128.427587444676)) ;
#117982=CARTESIAN_POINT('Ctrl Pts',(-27.285639381657,12.4255318802945,128.667511983218)) ;
#117983=CARTESIAN_POINT('Ctrl Pts',(-27.3834767186371,12.4160627421656,
128.920186580923)) ;
#117984=CARTESIAN_POINT('Ctrl Pts',(-27.4789408405044,12.4788298708389,
129.16594996465)) ;
#117985=CARTESIAN_POINT('Ctrl Pts',(-27.5661966226844,12.6096602147663,
129.387635338008)) ;
#117986=CARTESIAN_POINT('Ctrl Pts',(-27.6392077262574,12.7985461290531,
129.567801300047)) ;
#117987=CARTESIAN_POINT('Ctrl Pts',(-27.6936999893105,13.0317085131987,
129.693918325502)) ;
#117988=CARTESIAN_POINT('Ctrl Pts',(-27.7266401612783,13.2930834714085,
129.757042595518)) ;
#117989=CARTESIAN_POINT('Ctrl Pts',(-27.7363425654746,13.5641923615561,
129.752235268296)) ;
#117990=CARTESIAN_POINT('Ctrl Pts',(-27.7226448073327,13.825680563738,129.678996462907)) ;
#117991=CARTESIAN_POINT('Ctrl Pts',(-27.6876244443127,14.0565822354865,
129.543714023441)) ;
#117992=CARTESIAN_POINT('Ctrl Pts',(-27.6342027276218,14.2434410576494,
129.354513026548)) ;
#117993=CARTESIAN_POINT('Ctrl Pts',(-27.5668135419715,14.3714533294417,
129.124443036194)) ;
#117994=CARTESIAN_POINT('Ctrl Pts',(-27.4916575321869,14.4311593636965,
128.871880546709)) ;
#117995=CARTESIAN_POINT('Ctrl Pts',(-27.4140051961217,14.4188767520017,
128.611838878856)) ;
#117996=CARTESIAN_POINT('Ctrl Pts',(-27.3408213155295,14.3353894135925,
128.364980603773)) ;
#117997=CARTESIAN_POINT('Ctrl Pts',(-27.2775273425459,14.1858866633471,
128.146853314981)) ;
#117998=CARTESIAN_POINT('Ctrl Pts',(-27.2300108576713,13.9829323617686,
127.975041914533)) ;
#117999=CARTESIAN_POINT('Ctrl Pts',(-27.2017828862075,13.7386002363464,
127.859367243912)) ;
#118000=CARTESIAN_POINT('Ctrl Pts',(-27.1960189632252,13.4724911093289,
127.809439215144)) ;
#118001=CARTESIAN_POINT('Ctrl Pts',(-27.2135840337,13.2027754915033,127.827651886763)) ;
#118002=CARTESIAN_POINT('Ctrl Pts',(-27.2543835497371,12.9475729624172,
127.91355918546)) ;
#118003=CARTESIAN_POINT('Ctrl Pts',(-27.3154252564457,12.7286906957619,
128.05891829088)) ;
#118004=CARTESIAN_POINT('Ctrl Pts',(-27.3937085066093,12.5582194265839,
128.254489784026)) ;
#118005=CARTESIAN_POINT('Ctrl Pts',(-27.4845207555076,12.449581474798,128.486560407069)) ;
#118006=CARTESIAN_POINT('Ctrl Pts',(-27.5814065424675,12.4111325027633,
128.736500175583)) ;
#118007=CARTESIAN_POINT('Ctrl Pts',(-27.6783850149472,12.4448573237376,
128.986746017308)) ;
#118008=CARTESIAN_POINT('Ctrl Pts',(-27.7696066911728,12.5485736287012,
129.220097658122)) ;
#118009=CARTESIAN_POINT('Ctrl Pts',(-27.8493079778148,12.7160675413709,
129.419637082268)) ;
#118010=CARTESIAN_POINT('Ctrl Pts',(-27.9115752367297,12.9327061605047,
129.56852821594)) ;
#118011=CARTESIAN_POINT('Ctrl Pts',(-27.9535772039273,13.1846668295447,
129.658147795149)) ;
#118012=CARTESIAN_POINT('Ctrl Pts',(-27.9728087721377,13.454422434914,129.68116470926)) ;
#118013=CARTESIAN_POINT('Ctrl Pts',(-27.9685328637136,13.7215757053134,
129.635554875548)) ;
#118014=CARTESIAN_POINT('Ctrl Pts',(-27.9418155959324,13.9674105502267,
129.524377068385)) ;
#118015=CARTESIAN_POINT('Ctrl Pts',(-27.8953947806625,14.1739595025082,
129.355694529026)) ;
#118016=CARTESIAN_POINT('Ctrl Pts',(-27.833111646103,14.3272528691842,129.140590034414)) ;
#118017=CARTESIAN_POINT('Ctrl Pts',(-27.7602022571812,14.4155297813334,
128.894429525137)) ;
#118018=CARTESIAN_POINT('Ctrl Pts',(-27.6829875719055,14.4326688958934,
128.635821913402)) ;
#118019=CARTESIAN_POINT('Ctrl Pts',(-27.6071356051822,14.3775211091171,
128.381066125451)) ;
#118020=CARTESIAN_POINT('Ctrl Pts',(-27.539243721018,14.2540409956265,128.149629044627)) ;
#118021=CARTESIAN_POINT('Ctrl Pts',(-27.4846991991444,14.0709649077151,
127.957153811199)) ;
#118022=CARTESIAN_POINT('Ctrl Pts',(-27.4482373871036,13.8416200756966,
127.817529893249)) ;
#118023=CARTESIAN_POINT('Ctrl Pts',(-27.4331199621399,13.5823886653328,
127.740263361054)) ;
#118024=CARTESIAN_POINT('Ctrl Pts',(-27.4411948007982,13.3112805522026,
127.730691007012)) ;
#118025=CARTESIAN_POINT('Ctrl Pts',(-27.4726615076401,13.0483998972253,
127.789474656891)) ;
#118026=CARTESIAN_POINT('Ctrl Pts',(-27.5257417126982,12.8130299251434,
127.911496855804)) ;
#118027=CARTESIAN_POINT('Ctrl Pts',(-27.5977403806181,12.6204061484624,
128.088659391279)) ;
#118028=CARTESIAN_POINT('Ctrl Pts',(-27.6842706096557,12.4854479729451,
128.308217781128)) ;
#118029=CARTESIAN_POINT('Ctrl Pts',(-27.7790489564301,12.4181326854097,
128.552081197838)) ;
#118030=CARTESIAN_POINT('Ctrl Pts',(-27.8772458109095,12.4224942327925,
128.805703678812)) ;
#118031=CARTESIAN_POINT('Ctrl Pts',(-27.9715990075916,12.4989652676932,
129.048195975648)) ;
#118032=CARTESIAN_POINT('Ctrl Pts',(-28.0559858430151,12.6405918868476,
129.261745686545)) ;
#118033=CARTESIAN_POINT('Ctrl Pts',(-28.1260668022373,12.8391592679731,
129.433283736594)) ;
#118034=CARTESIAN_POINT('Ctrl Pts',(-28.1769110512927,13.0802458850777,
129.548577043249)) ;
#118035=CARTESIAN_POINT('Ctrl Pts',(-28.2054175915475,13.3449461423443,
129.598747575716)) ;
#118036=CARTESIAN_POINT('Ctrl Pts',(-28.2106105175659,13.6142996015355,
129.58092607558)) ;
#118037=CARTESIAN_POINT('Ctrl Pts',(-28.1928405096762,13.871042063758,129.495894578487)) ;
#118038=CARTESIAN_POINT('Ctrl Pts',(-28.1538963099053,14.0962487888297,
129.348931858615)) ;
#118039=CARTESIAN_POINT('Ctrl Pts',(-28.0972007895565,14.2729913868137,
129.150067416087)) ;
#118040=CARTESIAN_POINT('Ctrl Pts',(-28.0285087313468,14.3876795373717,
128.916519193871)) ;
#118041=CARTESIAN_POINT('Ctrl Pts',(-27.9519756057037,14.4346057861214,
128.659702361539)) ;
#118042=CARTESIAN_POINT('Ctrl Pts',(-27.874685639495,14.4082599511792,128.400740873235)) ;
#118043=CARTESIAN_POINT('Ctrl Pts',(-27.8032210859004,14.3122705937861,
128.159016222046)) ;
#118044=CARTESIAN_POINT('Ctrl Pts',(-27.742326472995,14.1514361884325,127.947851059364)) ;
#118045=CARTESIAN_POINT('Ctrl Pts',(-27.6981161142079,13.938718878438,127.785565576013)) ;
#118046=CARTESIAN_POINT('Ctrl Pts',(-27.6740950339109,13.6904434101565,
127.682412738132)) ;
#118047=CARTESIAN_POINT('Ctrl Pts',(-27.6726425154201,13.4208420564826,
127.644907773527)) ;
#118048=CARTESIAN_POINT('Ctrl Pts',(-27.6946457242154,13.1534853885067,
127.676185027627)) ;
#118049=CARTESIAN_POINT('Ctrl Pts',(-27.7391912414643,12.9044050301422,
127.773201636231)) ;
#118050=CARTESIAN_POINT('Ctrl Pts',(-27.8044358222147,12.6913476051149,
127.930474372812)) ;
#118051=CARTESIAN_POINT('Ctrl Pts',(-27.8854293394204,12.5324269089272,
128.134011207475)) ;
#118052=CARTESIAN_POINT('Ctrl Pts',(-27.9774944389672,12.4369854999087,
128.369889652559)) ;
#118053=CARTESIAN_POINT('Ctrl Pts',(-28.0748121994469,12.4119049756276,
128.621118828358)) ;
#118054=CARTESIAN_POINT('Ctrl Pts',(-28.1714853990872,12.4592885776231,
128.870352685515)) ;
#118055=CARTESIAN_POINT('Ctrl Pts',(-28.2608165469436,12.5757336581161,
129.098197079246)) ;
#118056=CARTESIAN_POINT('Ctrl Pts',(-28.3373453945994,12.7527802479952,
129.288637876852)) ;
#118057=CARTESIAN_POINT('Ctrl Pts',(-28.3964441530546,12.9786617700214,
129.428055264009)) ;
#118058=CARTESIAN_POINT('Ctrl Pts',(-28.434178239495,13.2359087639226,129.50514747171)) ;
#118059=CARTESIAN_POINT('Ctrl Pts',(-28.448897978943,13.5051025506678,129.515184910968)) ;
#118060=CARTESIAN_POINT('Ctrl Pts',(-28.4402109620374,13.7711208061555,
129.456502833988)) ;
#118061=CARTESIAN_POINT('Ctrl Pts',(-28.409511649221,14.0100002848338,129.333795685623)) ;
#118062=CARTESIAN_POINT('Ctrl Pts',(-28.3598408263846,14.2073723791963,
129.1556415538)) ;
#118063=CARTESIAN_POINT('Ctrl Pts',(-28.2950348334462,14.3492225893051,
128.933124083885)) ;
#118064=CARTESIAN_POINT('Ctrl Pts',(-28.2209823020186,14.4242519725476,
128.683712259003)) ;
#118065=CARTESIAN_POINT('Ctrl Pts',(-28.1433654691918,14.4277364692307,
128.423828382397)) ;
#118066=CARTESIAN_POINT('Ctrl Pts',(-28.0687197378844,14.3592420521561,
128.172676590865)) ;
#118067=CARTESIAN_POINT('Ctrl Pts',(-28.0029911633017,14.2240687585133,
127.94759605367)) ;
#118068=CARTESIAN_POINT('Ctrl Pts',(-27.951382030676,14.030558632252,127.763599842461)) ;
#118069=CARTESIAN_POINT('Ctrl Pts',(-27.9187982069096,13.7945207204753,
127.6353514582)) ;
#118070=CARTESIAN_POINT('Ctrl Pts',(-27.9079473566677,13.5313068874669,
127.570501215384)) ;
#118071=CARTESIAN_POINT('Ctrl Pts',(-27.9204903335361,13.2605193044374,
127.574017800966)) ;
#118072=CARTESIAN_POINT('Ctrl Pts',(-27.956164420614,13.0015411948259,127.645126607839)) ;
#118073=CARTESIAN_POINT('Ctrl Pts',(-28.0132085834406,12.7725524549383,
127.778637471497)) ;
#118074=CARTESIAN_POINT('Ctrl Pts',(-28.0882808220234,12.5901314518039,
127.964801388622)) ;
#118075=CARTESIAN_POINT('Ctrl Pts',(-28.1766696377702,12.4675131593939,
128.189879182512)) ;
#118076=CARTESIAN_POINT('Ctrl Pts',(-28.2726948839223,12.4133289167984,
128.437297139227)) ;
#118077=CARTESIAN_POINT('Ctrl Pts',(-28.3704658057419,12.4315113355368,
128.689755862838)) ;
#118078=CARTESIAN_POINT('Ctrl Pts',(-28.4632360481242,12.5204618518985,
128.927715630924)) ;
#118079=CARTESIAN_POINT('Ctrl Pts',(-28.5456402548427,12.6740885345687,
129.135315760515)) ;
#118080=CARTESIAN_POINT('Ctrl Pts',(-28.6123738489482,12.8820605395618,
129.297054080419)) ;
#118081=CARTESIAN_POINT('Ctrl Pts',(-28.6590331122904,13.1280848840325,
129.400264284258)) ;
#118082=CARTESIAN_POINT('Ctrl Pts',(-28.6833089341504,13.3954305340358,
129.438055238725)) ;
#118083=CARTESIAN_POINT('Ctrl Pts',(-28.6840931743626,13.6647721177767,
129.407220114326)) ;
#118084=CARTESIAN_POINT('Ctrl Pts',(-28.6621121847327,13.9166503659834,
129.309906441971)) ;
#118085=CARTESIAN_POINT('Ctrl Pts',(-28.6195959601702,14.1333087838378,
129.152574525308)) ;
#118086=CARTESIAN_POINT('Ctrl Pts',(-28.5605481815634,14.2989356853765,
128.947034341319)) ;
#118087=CARTESIAN_POINT('Ctrl Pts',(-28.4890535847478,14.4025578150193,
128.704822107942)) ;
#118088=CARTESIAN_POINT('Ctrl Pts',(-28.4125691478489,14.4350103975139,
128.448465769779)) ;
#118089=CARTESIAN_POINT('Ctrl Pts',(-28.3358905451254,14.3956728087921,
128.191327603003)) ;
#118090=CARTESIAN_POINT('Ctrl Pts',(-28.2657346269624,14.2862787628231,
127.953238888574)) ;
#118091=CARTESIAN_POINT('Ctrl Pts',(-28.2079489137776,14.1158603656016,
127.751395068649)) ;
#118092=CARTESIAN_POINT('Ctrl Pts',(-28.1669469057147,13.8934485615438,
127.598238076761)) ;
#118093=CARTESIAN_POINT('Ctrl Pts',(-28.1471610978907,13.6404741720686,
127.507517955386)) ;
#118094=CARTESIAN_POINT('Ctrl Pts',(-28.1501382434426,13.3695007769354,
127.482960727044)) ;
#118095=CARTESIAN_POINT('Ctrl Pts',(-28.1764960356968,13.1044457745781,
127.526973882184)) ;
#118096=CARTESIAN_POINT('Ctrl Pts',(-28.225181846566,12.8607040814897,127.636031331103)) ;
#118097=CARTESIAN_POINT('Ctrl Pts',(-28.2937142871452,12.6571155232214,
127.802989653399)) ;
#118098=CARTESIAN_POINT('Ctrl Pts',(-28.3768619488044,12.5098080882698,
128.012940704154)) ;
#118099=CARTESIAN_POINT('Ctrl Pts',(-28.4705911940242,12.4266891682411,
128.253596863206)) ;
#118100=CARTESIAN_POINT('Ctrl Pts',(-28.5686736001448,12.4154229677179,
128.506902117577)) ;
#118101=CARTESIAN_POINT('Ctrl Pts',(-28.6639498164915,12.4759770344289,
128.752232097602)) ;
#118102=CARTESIAN_POINT('Ctrl Pts',(-28.7515478234264,12.6048251808736,
128.974917562034)) ;
#118103=CARTESIAN_POINT('Ctrl Pts',(-28.8250741000503,12.7921644823966,
129.156583452211)) ;
#118104=CARTESIAN_POINT('Ctrl Pts',(-28.8802512943592,13.0247861234327,
129.284627554489)) ;
#118105=CARTESIAN_POINT('Ctrl Pts',(-28.9138214071778,13.2853104299406,
129.349634739468)) ;
#118106=CARTESIAN_POINT('Ctrl Pts',(-28.9241393866765,13.5574329936333,
129.346494578339)) ;
#118107=CARTESIAN_POINT('Ctrl Pts',(-28.9112612456758,13.8171020410684,
129.275962093259)) ;
#118108=CARTESIAN_POINT('Ctrl Pts',(-28.8766091041569,14.0511737874882,
129.141473450271)) ;
#118109=CARTESIAN_POINT('Ctrl Pts',(-28.8236655661538,14.2388281318634,
128.953740433956)) ;
#118110=CARTESIAN_POINT('Ctrl Pts',(-28.7568581926641,14.3685838894511,
128.725474314568)) ;
#118111=CARTESIAN_POINT('Ctrl Pts',(-28.6812672811723,14.4305511388163,
128.471385584917)) ;
#118112=CARTESIAN_POINT('Ctrl Pts',(-28.6041593186733,14.4203097552105,
128.213187763723)) ;
#118113=CARTESIAN_POINT('Ctrl Pts',(-28.5304223006701,14.3384208536168,
127.964543460545)) ;
#118114=CARTESIAN_POINT('Ctrl Pts',(-28.4670853954553,14.191573241038,127.746486631087)) ;
#118115=CARTESIAN_POINT('Ctrl Pts',(-28.4186878189402,13.9880715785311,
127.571796076703)) ;
#118116=CARTESIAN_POINT('Ctrl Pts',(-28.3901888562639,13.7471726162761,
127.455689629108)) ;
#118117=CARTESIAN_POINT('Ctrl Pts',(-28.3836245551766,13.4800206998336,
127.403228049252)) ;
#118118=CARTESIAN_POINT('Ctrl Pts',(-28.4004971163095,13.2110031222513,
127.419530052212)) ;
#118119=CARTESIAN_POINT('Ctrl Pts',(-28.4406184078603,12.9547749456752,
127.503422585335)) ;
#118120=CARTESIAN_POINT('Ctrl Pts',(-28.5011655208637,12.7344342581801,
127.647306006591)) ;
#118121=CARTESIAN_POINT('Ctrl Pts',(-28.5790499129694,12.5623453815543,
127.841701802032)) ;
#118122=CARTESIAN_POINT('Ctrl Pts',(-28.6693949565012,12.4518692126569,
128.072474343319)) ;
#118123=CARTESIAN_POINT('Ctrl Pts',(-28.7664627474836,12.4112334904619,
128.322845196979)) ;
#118124=CARTESIAN_POINT('Ctrl Pts',(-28.8634228465911,12.442749147545,128.573081464854)) ;
#118125=CARTESIAN_POINT('Ctrl Pts',(-28.9554286612127,12.5456206803201,
128.808503142631)) ;
#118126=CARTESIAN_POINT('Ctrl Pts',(-29.0344828901899,12.7091960284291,
129.006604080656)) ;
#118127=CARTESIAN_POINT('Ctrl Pts',(-29.0979031643936,12.9259029795746,
129.158604870418)) ;
#118128=CARTESIAN_POINT('Ctrl Pts',(-29.1404537451632,13.1770736190436,
129.249849282073)) ;
#118129=CARTESIAN_POINT('Ctrl Pts',(-29.160380259994,13.446876823357,129.27485767805)) ;
#118130=CARTESIAN_POINT('Ctrl Pts',(-29.1567650507286,13.7138795618443,
129.231240033964)) ;
#118131=CARTESIAN_POINT('Ctrl Pts',(-29.1306997030977,13.9605431609207,
129.121973670097)) ;
#118132=CARTESIAN_POINT('Ctrl Pts',(-29.0848235950521,14.1686235242906,
128.954875473601)) ;
#118133=CARTESIAN_POINT('Ctrl Pts',(-29.0226188426118,14.324111246448,128.739854084484)) ;
#118134=CARTESIAN_POINT('Ctrl Pts',(-28.9503351461501,14.4138215674339,
128.495712046884)) ;
#118135=CARTESIAN_POINT('Ctrl Pts',(-28.8728719219959,14.433194510591,128.236245701094)) ;
#118136=CARTESIAN_POINT('Ctrl Pts',(-28.7971138201711,14.3801615030747,
127.981866628935)) ;
#118137=CARTESIAN_POINT('Ctrl Pts',(-28.7288143739679,14.2584943373808,
127.749193854589)) ;
#118138=CARTESIAN_POINT('Ctrl Pts',(-28.6738445624091,14.0770492595335,
127.555495097218)) ;
#118139=CARTESIAN_POINT('Ctrl Pts',(-28.6367355115923,13.8484876221982,
127.413928530958)) ;
#118140=CARTESIAN_POINT('Ctrl Pts',(-28.6210283832256,13.5893551833119,
127.334883350605)) ;
#118141=CARTESIAN_POINT('Ctrl Pts',(-28.6284008712887,13.3196923685202,
127.323428440679)) ;
#118142=CARTESIAN_POINT('Ctrl Pts',(-28.6591285906283,13.0561135108425,
127.380035823894)) ;
#118143=CARTESIAN_POINT('Ctrl Pts',(-28.7117612730956,12.8190742431854,
127.500662990414)) ;
#118144=CARTESIAN_POINT('Ctrl Pts',(-28.7832377724029,12.6252976951711,
127.676332558911)) ;
#118145=CARTESIAN_POINT('Ctrl Pts',(-28.8690809391331,12.4887797495905,
127.894002489034)) ;
#118146=CARTESIAN_POINT('Ctrl Pts',(-28.9640456085277,12.4190606643947,
128.138280288588)) ;
#118147=CARTESIAN_POINT('Ctrl Pts',(-29.0618810901176,12.4213023126393,
128.390972937899)) ;
#118148=CARTESIAN_POINT('Ctrl Pts',(-29.1564753036058,12.4953371872364,
128.634164403093)) ;
#118149=CARTESIAN_POINT('Ctrl Pts',(-29.2416400202375,12.6358732180601,
128.849823957107)) ;
#118150=CARTESIAN_POINT('Ctrl Pts',(-29.3119790802921,12.8325868641011,
129.022206276767)) ;
#118151=CARTESIAN_POINT('Ctrl Pts',(-29.3633296045166,13.0715961519443,
129.139105648325)) ;
#118152=CARTESIAN_POINT('Ctrl Pts',(-29.3927074261657,13.3366927750057,
129.191707126252)) ;
#118153=CARTESIAN_POINT('Ctrl Pts',(-29.3985768140557,13.606785296831,129.175787373953)) ;
#118154=CARTESIAN_POINT('Ctrl Pts',(-29.3814203497901,13.8640946124835,
129.092554350732)) ;
#118155=CARTESIAN_POINT('Ctrl Pts',(-29.343171418544,14.0898396891215,128.947718536782)) ;
#118156=CARTESIAN_POINT('Ctrl Pts',(-29.2869989434222,14.2683601358406,
128.75038942018)) ;
#118157=CARTESIAN_POINT('Ctrl Pts',(-29.2183282878595,14.3854877046267,
128.516772892733)) ;
#118158=CARTESIAN_POINT('Ctrl Pts',(-29.1418332811828,14.4341894572121,
128.260036672281)) ;
#118159=CARTESIAN_POINT('Ctrl Pts',(-29.0649019264552,14.4102459921106,
128.002309393832)) ;
#118160=CARTESIAN_POINT('Ctrl Pts',(-28.992797144068,14.3157190634071,127.758526648473)) ;
#118161=CARTESIAN_POINT('Ctrl Pts',(-28.9318649553926,14.1574303068782,
127.547443662481)) ;
#118162=CARTESIAN_POINT('Ctrl Pts',(-28.8869190669663,13.9458829151207,
127.382942524456)) ;
#118163=CARTESIAN_POINT('Ctrl Pts',(-28.8622213277086,13.6969896292084,
127.277637199178)) ;
#118164=CARTESIAN_POINT('Ctrl Pts',(-28.8601628813631,13.4292803760991,
127.238560560346)) ;
#118165=CARTESIAN_POINT('Ctrl Pts',(-28.881365510104,13.161309101516,127.267468442087)) ;
#118166=CARTESIAN_POINT('Ctrl Pts',(-28.9257769976233,12.9096301866455,
127.363829449715)) ;
#118167=CARTESIAN_POINT('Ctrl Pts',(-28.9898111411058,12.6977069175332,
127.517935580813)) ;
#118168=CARTESIAN_POINT('Ctrl Pts',(-29.0706272174786,12.5361591830993,
127.720823430246)) ;
#118169=CARTESIAN_POINT('Ctrl Pts',(-29.1624465503808,12.4388403169488,
127.955993565838)) ;
#118170=CARTESIAN_POINT('Ctrl Pts',(-29.2598010006521,12.4115721832676,
128.207292728113)) ;
#118171=CARTESIAN_POINT('Ctrl Pts',(-29.3566445682897,12.457029405049,128.45700426414)) ;
#118172=CARTESIAN_POINT('Ctrl Pts',(-29.4460805763726,12.5713337324556,
128.685222690321)) ;
#118173=CARTESIAN_POINT('Ctrl Pts',(-29.5231255961065,12.7468028195077,
128.877151920439)) ;
#118174=CARTESIAN_POINT('Ctrl Pts',(-29.5827662875995,12.9715572514285,
129.018148836661)) ;
#118175=CARTESIAN_POINT('Ctrl Pts',(-29.621127294111,13.2272670730613,129.097177228825)) ;
#118176=CARTESIAN_POINT('Ctrl Pts',(-29.6365791297085,13.4980618104753,
129.10913652102)) ;
#118177=CARTESIAN_POINT('Ctrl Pts',(-29.6286710531426,13.7620973804226,
129.053043121291)) ;
#118178=CARTESIAN_POINT('Ctrl Pts',(-29.5984934663747,14.0037248374368,
128.931633804845)) ;
#118179=CARTESIAN_POINT('Ctrl Pts',(-29.5492988117199,14.2023999767799,
128.754886608175)) ;
#118180=CARTESIAN_POINT('Ctrl Pts',(-29.4846658524462,14.3463072474208,
128.532783710775)) ;
#118181=CARTESIAN_POINT('Ctrl Pts',(-29.4110973983037,14.422940695718,128.284924483478)) ;
#118182=CARTESIAN_POINT('Ctrl Pts',(-29.3334897330232,14.4287087327574,
128.025061129065)) ;
#118183=CARTESIAN_POINT('Ctrl Pts',(-29.258638100884,14.3623692114808,127.773301149535)) ;
#118184=CARTESIAN_POINT('Ctrl Pts',(-29.1923062200584,14.2283780368313,
127.546318276707)) ;
#118185=CARTESIAN_POINT('Ctrl Pts',(-29.1403623093104,14.0364257268117,
127.361394564376)) ;
#118186=CARTESIAN_POINT('Ctrl Pts',(-29.1072616567678,13.8020945875402,
127.231726399014)) ;
#118187=CARTESIAN_POINT('Ctrl Pts',(-29.0957233925479,13.5391614868317,
127.164835509363)) ;
#118188=CARTESIAN_POINT('Ctrl Pts',(-29.1075472344212,13.2686187848472,
127.166290520158)) ;
#118189=CARTESIAN_POINT('Ctrl Pts',(-29.1426301460642,13.0086420125285,
127.235617273875)) ;
#118190=CARTESIAN_POINT('Ctrl Pts',(-29.1988929035827,12.7791081292504,
127.366944131897)) ;
#118191=CARTESIAN_POINT('Ctrl Pts',(-29.2738449830755,12.5942977815412,
127.552601689651)) ;
#118192=CARTESIAN_POINT('Ctrl Pts',(-29.3616192086889,12.470297081659,127.776006417397)) ;
#118193=CARTESIAN_POINT('Ctrl Pts',(-29.4576937562919,12.4139049910115,
128.023496861741)) ;
#118194=CARTESIAN_POINT('Ctrl Pts',(-29.5551748682929,12.4297924178913,
128.275226478106)) ;
#118195=CARTESIAN_POINT('Ctrl Pts',(-29.6487814577024,12.5172147153485,
128.515415278977)) ;
#118196=CARTESIAN_POINT('Ctrl Pts',(-29.7315236720721,12.6696685432672,
128.723981025361)) ;
#118197=CARTESIAN_POINT('Ctrl Pts',(-29.7983400212672,12.8748935660195,
128.886180011621)) ;
#118198=CARTESIAN_POINT('Ctrl Pts',(-29.8458033561014,13.1206629009233,
128.991641648077)) ;
#118199=CARTESIAN_POINT('Ctrl Pts',(-29.8707194251093,13.3874986726008,
129.031327378694)) ;
#118200=CARTESIAN_POINT('Ctrl Pts',(-29.8721807681616,13.6577700342002,
129.002383109698)) ;
#118201=CARTESIAN_POINT('Ctrl Pts',(-29.8507362629684,13.9102263509794,
128.906641410683)) ;
#118202=CARTESIAN_POINT('Ctrl Pts',(-29.8089880561964,14.1273421319092,
128.751696352259)) ;
#118203=CARTESIAN_POINT('Ctrl Pts',(-29.7499753711012,14.2954362033895,
128.546056522854)) ;
#118204=CARTESIAN_POINT('Ctrl Pts',(-29.6793771471953,14.4001990487277,
128.30676279706)) ;
#118205=CARTESIAN_POINT('Ctrl Pts',(-29.6022634084759,14.4351706370755,
128.048249901816)) ;
#118206=CARTESIAN_POINT('Ctrl Pts',(-29.5259240512111,14.3977719552174,
127.792290143655)) ;
#118207=CARTESIAN_POINT('Ctrl Pts',(-29.4553374749208,14.2904204351337,
127.552887066617)) ;
#118208=CARTESIAN_POINT('Ctrl Pts',(-29.396976625912,14.1205426319521,127.349221263366)) ;
#118209=CARTESIAN_POINT('Ctrl Pts',(-29.3558187577604,13.9015880459834,
127.19594254992)) ;
#118210=CARTESIAN_POINT('Ctrl Pts',(-29.3351815258141,13.6483197880018,
127.102578325798)) ;
#118211=CARTESIAN_POINT('Ctrl Pts',(-29.3374965976238,13.3774460440173,
127.076084018573)) ;
#118212=CARTESIAN_POINT('Ctrl Pts',(-29.3632483250244,13.1115164567619,
127.11826281631)) ;
#118213=CARTESIAN_POINT('Ctrl Pts',(-29.4112273090806,12.8676277943346,
127.225348651307)) ;
#118214=CARTESIAN_POINT('Ctrl Pts',(-29.4789001513316,12.6630942095761,
127.389914697204)) ;
#118215=CARTESIAN_POINT('Ctrl Pts',(-29.5622543716497,12.5128296966432,
127.6002285727)) ;
#118216=CARTESIAN_POINT('Ctrl Pts',(-29.655782504476,12.42805223675,127.840309014045)) ;
#118217=CARTESIAN_POINT('Ctrl Pts',(-29.7536636355645,12.4147676661353,
128.093080631668)) ;
#118218=CARTESIAN_POINT('Ctrl Pts',(-29.8491089640436,12.4732051898518,
128.338902853644)) ;
#118219=CARTESIAN_POINT('Ctrl Pts',(-29.9373051654279,12.6008829742714,
128.563215033879)) ;
#118220=CARTESIAN_POINT('Ctrl Pts',(-30.0108837724074,12.7859099614939,
128.745200476699)) ;
#118221=CARTESIAN_POINT('Ctrl Pts',(-30.0666707267494,13.0171549052487,
128.875047914663)) ;
#118222=CARTESIAN_POINT('Ctrl Pts',(-30.1009396863754,13.277402309204,128.94205811124)) ;
#118223=CARTESIAN_POINT('Ctrl Pts',(-30.1119760819593,13.5492090907174,
128.941057414916)) ;
#118224=CARTESIAN_POINT('Ctrl Pts',(-30.0996900511507,13.8101281640257,
128.872156772245)) ;
#118225=CARTESIAN_POINT('Ctrl Pts',(-30.0658412126364,14.0442615498891,
128.740177177303)) ;
#118226=CARTESIAN_POINT('Ctrl Pts',(-30.0129614418644,14.2348996277818,
128.552367794294)) ;
#118227=CARTESIAN_POINT('Ctrl Pts',(-29.9467812118258,14.365488247491,128.326113063617)) ;
#118228=CARTESIAN_POINT('Ctrl Pts',(-29.8715551104391,14.429722906614,128.073164206403)) ;
#118229=CARTESIAN_POINT('Ctrl Pts',(-29.7941603221603,14.4216680373145,
127.814017409384)) ;
#118230=CARTESIAN_POINT('Ctrl Pts',(-29.7201980568112,14.3417421595957,
127.564708377422)) ;
#118231=CARTESIAN_POINT('Ctrl Pts',(-29.656483010943,14.1964292169101,127.345520658291)) ;
#118232=CARTESIAN_POINT('Ctrl Pts',(-29.6077772460928,13.9955519637573,
127.170107835032)) ;
#118233=CARTESIAN_POINT('Ctrl Pts',(-29.5784336722028,13.7541465447125,
127.051322930281)) ;
#118234=CARTESIAN_POINT('Ctrl Pts',(-29.5712927220666,13.4873871522708,
126.997186762479)) ;
#118235=CARTESIAN_POINT('Ctrl Pts',(-29.5874867790851,13.2187119669683,
127.01156199828)) ;
#118236=CARTESIAN_POINT('Ctrl Pts',(-29.6268275872939,12.9622340924051,
127.093243502757)) ;
#118237=CARTESIAN_POINT('Ctrl Pts',(-29.6870818963363,12.7396655368573,
127.236122661308)) ;
#118238=CARTESIAN_POINT('Ctrl Pts',(-29.7645649139523,12.5663130362906,
127.429362402402)) ;
#118239=CARTESIAN_POINT('Ctrl Pts',(-29.8542359643291,12.4542929852172,
127.658304546946)) ;
#118240=CARTESIAN_POINT('Ctrl Pts',(-29.9515317793415,12.4113060985389,
127.909226798948)) ;
#118241=CARTESIAN_POINT('Ctrl Pts',(-30.0483978993712,12.440972973662,128.159239721085)) ;
#118242=CARTESIAN_POINT('Ctrl Pts',(-30.1401907845487,12.5408195803972,
128.394234115448)) ;
#118243=CARTESIAN_POINT('Ctrl Pts',(-30.2205767778693,12.7045177215447,
128.595849815702)) ;
#118244=CARTESIAN_POINT('Ctrl Pts',(-30.2841435840745,12.9194126862855,
128.748414866231)) ;
#118245=CARTESIAN_POINT('Ctrl Pts',(-30.3272725943575,13.1689179469772,
128.841448687789)) ;
#118246=CARTESIAN_POINT('Ctrl Pts',(-30.3479588136649,13.4397285772897,
128.868523727985)) ;
#118247=CARTESIAN_POINT('Ctrl Pts',(-30.3449564456502,13.7064270482981,
128.82677202049)) ;
#118248=CARTESIAN_POINT('Ctrl Pts',(-30.3195311548179,13.9538862841149,
128.719382880456)) ;
#118249=CARTESIAN_POINT('Ctrl Pts',(-30.2742133985792,14.1631927449857,
128.553937662438)) ;
#118250=CARTESIAN_POINT('Ctrl Pts',(-30.2123564115104,14.3205261030357,
128.33990642058)) ;
#118251=CARTESIAN_POINT('Ctrl Pts',(-30.140400371972,14.4121066368491,128.096766582893)) ;
#118252=CARTESIAN_POINT('Ctrl Pts',(-30.0629325421194,14.4337042758691,
127.837261507592)) ;
#118253=CARTESIAN_POINT('Ctrl Pts',(-29.9869630886905,14.3826278342729,
127.582229125902)) ;
#118254=CARTESIAN_POINT('Ctrl Pts',(-29.9184051994975,14.2628852897391,
127.348821521757)) ;
#118255=CARTESIAN_POINT('Ctrl Pts',(-29.8629677727426,14.0829262304897,
127.15374414379)) ;
#118256=CARTESIAN_POINT('Ctrl Pts',(-29.8253177094435,13.8556922728628,
127.010626598534)) ;
#118257=CARTESIAN_POINT('Ctrl Pts',(-29.8089663723846,13.5972599907668,
126.929704638367)) ;
#118258=CARTESIAN_POINT('Ctrl Pts',(-29.8155751015149,13.3277680057125,
126.91603611238)) ;
#118259=CARTESIAN_POINT('Ctrl Pts',(-29.8459893717069,13.0618110658261,
126.971473920296)) ;
#118260=CARTESIAN_POINT('Ctrl Pts',(-29.8976049223748,12.8260390349159,
127.089438246611)) ;
#118261=CARTESIAN_POINT('Ctrl Pts',(-29.9688137126878,12.6298697180506,
127.264190142746)) ;
#118262=CARTESIAN_POINT('Ctrl Pts',(-30.0542930667686,12.4917687928696,
127.480820902016)) ;
#118263=CARTESIAN_POINT('Ctrl Pts',(-30.1491960832168,12.4199839443985,
127.724877330346)) ;
#118264=CARTESIAN_POINT('Ctrl Pts',(-30.2469829227126,12.4203084099031,
127.977445944159)) ;
#118265=CARTESIAN_POINT('Ctrl Pts',(-30.3416052555647,12.4922084263286,
128.220773062018)) ;
#118266=CARTESIAN_POINT('Ctrl Pts',(-30.4271681599976,12.6309968831691,
128.437577974098)) ;
#118267=CARTESIAN_POINT('Ctrl Pts',(-30.4980284200408,12.8263310850707,
128.611471879481)) ;
#118268=CARTESIAN_POINT('Ctrl Pts',(-30.5500880714894,13.0651227719104,
128.730345775696)) ;
#118269=CARTESIAN_POINT('Ctrl Pts',(-30.5799917287299,13.3295667495973,
128.784515371445)) ;
#118270=CARTESIAN_POINT('Ctrl Pts',(-30.5865246799036,13.5989123639349,
128.770637027271)) ;
#118271=CARTESIAN_POINT('Ctrl Pts',(-30.5699655121301,13.8574710596154,
128.689069047576)) ;
#118272=CARTESIAN_POINT('Ctrl Pts',(-30.5323457648762,14.0837078972677,
128.54615654452)) ;
#118273=CARTESIAN_POINT('Ctrl Pts',(-30.4767238876144,14.2638191910291,
128.350466442062)) ;
#118274=CARTESIAN_POINT('Ctrl Pts',(-30.4081138852739,14.3831695722174,
128.116916906689)) ;
#118275=CARTESIAN_POINT('Ctrl Pts',(-30.3319909445384,14.4337176680091,
127.861377615128)) ;
#118276=CARTESIAN_POINT('Ctrl Pts',(-30.2549612223786,14.4120588735212,
127.603346669515)) ;
#118277=CARTESIAN_POINT('Ctrl Pts',(-30.1825342935614,14.3193773095664,
127.358581367932)) ;
#118278=CARTESIAN_POINT('Ctrl Pts',(-30.1211674273149,14.1628171058123,
127.146222590611)) ;
#118279=CARTESIAN_POINT('Ctrl Pts',(-30.0756155237359,13.9515916314902,
126.979821977845)) ;
#118280=CARTESIAN_POINT('Ctrl Pts',(-30.050461370889,13.705523326728,126.873449550959)) ;
#118281=CARTESIAN_POINT('Ctrl Pts',(-30.047694629407,13.4359481915904,126.832028407442)) ;
#118282=CARTESIAN_POINT('Ctrl Pts',(-30.0682250191869,13.169026252587,126.85913562874)) ;
#118283=CARTESIAN_POINT('Ctrl Pts',(-30.1120139572627,12.916272819337,126.95364273637)) ;
#118284=CARTESIAN_POINT('Ctrl Pts',(-30.1753570929207,12.7036779649805,
127.105819577044)) ;
#118285=CARTESIAN_POINT('Ctrl Pts',(-30.2555879257156,12.5403117624792,
127.30703937934)) ;
#118286=CARTESIAN_POINT('Ctrl Pts',(-30.3477768389897,12.4404489594076,
127.543069245436)) ;
#118287=CARTESIAN_POINT('Ctrl Pts',(-30.4445994007357,12.4114485635984,
127.792975546885)) ;
#118288=CARTESIAN_POINT('Ctrl Pts',(-30.541500222199,12.4544846359496,128.042874784627)) ;
#118289=CARTESIAN_POINT('Ctrl Pts',(-30.6315932064016,12.5672617568272,
128.27288531667)) ;
#118290=CARTESIAN_POINT('Ctrl Pts',(-30.7091172675057,12.7417744672769,
128.466151664717)) ;
#118291=CARTESIAN_POINT('Ctrl Pts',(-30.7688720388517,12.9633750466865,
128.607760924337)) ;
#118292=CARTESIAN_POINT('Ctrl Pts',(-30.8082363281393,13.2203111282886,
128.689459648843)) ;
#118293=CARTESIAN_POINT('Ctrl Pts',(-30.8242398852336,13.4905143177326,
128.703096866433)) ;
#118294=CARTESIAN_POINT('Ctrl Pts',(-30.8169657794985,13.755021596538,128.648839900988)) ;
#118295=CARTESIAN_POINT('Ctrl Pts',(-30.7875298285178,13.9967495673617,
128.529724713065)) ;
#118296=CARTESIAN_POINT('Ctrl Pts',(-30.7387155255935,14.1974242169902,
128.353993085411)) ;
#118297=CARTESIAN_POINT('Ctrl Pts',(-30.6747667553044,14.3425139654286,
128.134048073582)) ;
#118298=CARTESIAN_POINT('Ctrl Pts',(-30.6012043043127,14.4218015795288,
127.886103518124)) ;
#118299=CARTESIAN_POINT('Ctrl Pts',(-30.5232263864792,14.4294553596466,
127.62499654632)) ;
#118300=CARTESIAN_POINT('Ctrl Pts',(-30.4485854643026,14.3652618643662,
127.374009503978)) ;
#118301=CARTESIAN_POINT('Ctrl Pts',(-30.382005194927,14.2335997278837,127.146362312716)) ;
#118302=CARTESIAN_POINT('Ctrl Pts',(-30.3294754572321,14.043065952539,126.959689608292)) ;
#118303=CARTESIAN_POINT('Ctrl Pts',(-30.2956753204816,13.8093139342674,
126.827907583262)) ;
#118304=CARTESIAN_POINT('Ctrl Pts',(-30.2835287824806,13.5459140316558,
126.759122107196)) ;
#118305=CARTESIAN_POINT('Ctrl Pts',(-30.2946484169742,13.2769104618193,
126.75871180703)) ;
#118306=CARTESIAN_POINT('Ctrl Pts',(-30.329022809304,13.0160047166174,126.825934930956)) ;
#118307=CARTESIAN_POINT('Ctrl Pts',(-30.3848542480685,12.7850162006338,
126.95593843375)) ;
#118308=CARTESIAN_POINT('Ctrl Pts',(-30.4590572718797,12.5991696538989,
127.139522132046)) ;
#118309=CARTESIAN_POINT('Ctrl Pts',(-30.5469752382055,12.4727066988936,
127.363172990166)) ;
#118310=CARTESIAN_POINT('Ctrl Pts',(-30.6424477831083,12.4146340125785,
127.609068863606)) ;
#118311=CARTESIAN_POINT('Ctrl Pts',(-30.7401818962368,12.4282724622725,
127.861462595189)) ;
#118312=CARTESIAN_POINT('Ctrl Pts',(-30.8338872261793,12.5136821957653,
128.101978493891)) ;
#118313=CARTESIAN_POINT('Ctrl Pts',(-30.917003754287,12.6640313593757,128.31166457867)) ;
#118314=CARTESIAN_POINT('Ctrl Pts',(-30.9847278681875,12.8694014058608,
128.476293188432)) ;
#118315=CARTESIAN_POINT('Ctrl Pts',(-31.0324410263083,13.1128473164404,
128.582693695894)) ;
#118316=CARTESIAN_POINT('Ctrl Pts',(-31.0581101474431,13.3794713552814,
128.624552035848)) ;
#118317=CARTESIAN_POINT('Ctrl Pts',(-31.0602524783805,13.6493875459495,
128.597664462069)) ;
#118318=CARTESIAN_POINT('Ctrl Pts',(-31.0395778251596,13.9027716733404,
128.504174750462)) ;
#118319=CARTESIAN_POINT('Ctrl Pts',(-30.9979754649405,14.1226003916879,
128.34939664965)) ;
#118320=CARTESIAN_POINT('Ctrl Pts',(-30.9399581342553,14.2907614910249,
128.14699206746)) ;
#118321=CARTESIAN_POINT('Ctrl Pts',(-30.8690051734005,14.3985142710539,
127.906354089039)) ;
#118322=CARTESIAN_POINT('Ctrl Pts',(-30.7924824842021,14.4350393250775,
127.649796923618)) ;
#118323=CARTESIAN_POINT('Ctrl Pts',(-30.7159080944081,14.400035592365,127.393090625893)) ;
#118324=CARTESIAN_POINT('Ctrl Pts',(-30.6448246928201,14.2940192580209,
127.152118703661)) ;
#118325=CARTESIAN_POINT('Ctrl Pts',(-30.5863183815752,14.1264036829356,
126.948167110242)) ;
#118326=CARTESIAN_POINT('Ctrl Pts',(-30.5444975557761,13.9087136150407,
126.792930507996)) ;
#118327=CARTESIAN_POINT('Ctrl Pts',(-30.5232063252145,13.6545233565068,
126.697452847525)) ;
#118328=CARTESIAN_POINT('Ctrl Pts',(-30.524891337216,13.3858501360358,126.669368708623)) ;
#118329=CARTESIAN_POINT('Ctrl Pts',(-30.5499389792202,13.11900556216,126.709423409167)) ;
#118330=CARTESIAN_POINT('Ctrl Pts',(-30.5973969560023,12.8738785752154,
126.81494195181)) ;
#118331=CARTESIAN_POINT('Ctrl Pts',(-30.6647651473232,12.6676054071639,
126.978537542802)) ;
#118332=CARTESIAN_POINT('Ctrl Pts',(-30.7476901186471,12.516077131837,127.187642374558)) ;
#118333=CARTESIAN_POINT('Ctrl Pts',(-30.8405646959683,12.4297444851197,
127.425965717175)) ;
#118334=CARTESIAN_POINT('Ctrl Pts',(-30.9383003022728,12.4139325771417,
127.678350350006)) ;
#118335=CARTESIAN_POINT('Ctrl Pts',(-31.0344472399923,12.4708186129552,
127.926022202956)) ;
#118336=CARTESIAN_POINT('Ctrl Pts',(-31.1222102381147,12.5954480986012,
128.149360733914)) ;
#118337=CARTESIAN_POINT('Ctrl Pts',(-31.1967512804994,12.7795462403225,
128.333980482879)) ;
#118338=CARTESIAN_POINT('Ctrl Pts',(-31.2532458302397,13.0105017874409,
128.4657979126)) ;
#118339=CARTESIAN_POINT('Ctrl Pts',(-31.2881200869954,13.2704658553687,
128.534545422152)) ;
#118340=CARTESIAN_POINT('Ctrl Pts',(-31.2997537261348,13.5415024018121,
128.535378063465)) ;
#118341=CARTESIAN_POINT('Ctrl Pts',(-31.288169122968,13.8030869084645,128.468519236206)) ;
#118342=CARTESIAN_POINT('Ctrl Pts',(-31.254641174514,14.0389746831751,128.337336611109)) ;
#118343=CARTESIAN_POINT('Ctrl Pts',(-31.2028842012387,14.2290323686529,
128.153196437362)) ;
#118344=CARTESIAN_POINT('Ctrl Pts',(-31.1365285056857,14.3629000991712,
127.926138023514)) ;
#118345=CARTESIAN_POINT('Ctrl Pts',(-31.0616081958548,14.4288302625026,
127.67416381072)) ;
#118346=CARTESIAN_POINT('Ctrl Pts',(-30.98404256555,14.422836536164,127.414443978125)) ;
#118347=CARTESIAN_POINT('Ctrl Pts',(-30.9101456342738,14.3452102750607,
127.165449135438)) ;
#118348=CARTESIAN_POINT('Ctrl Pts',(-30.8458926888161,14.2014203774082,
126.944605876018)) ;
#118349=CARTESIAN_POINT('Ctrl Pts',(-30.7967539777331,14.002164262405,126.76797119047)) ;
#118350=CARTESIAN_POINT('Ctrl Pts',(-30.7667868700996,13.7617532002817,
126.64736275973)) ;
#118351=CARTESIAN_POINT('Ctrl Pts',(-30.7589404789089,13.4956080912223,
126.591189468115)) ;
#118352=CARTESIAN_POINT('Ctrl Pts',(-30.7744975468887,13.2262846444733,
126.603638049819)) ;
#118353=CARTESIAN_POINT('Ctrl Pts',(-30.8130435438419,12.9698877409975,
126.683104985907)) ;
#118354=CARTESIAN_POINT('Ctrl Pts',(-30.8727944794778,12.7457364397051,
126.82445862299)) ;
#118355=CARTESIAN_POINT('Ctrl Pts',(-30.9496439744757,12.5708017682082,
127.015910626943)) ;
#118356=CARTESIAN_POINT('Ctrl Pts',(-31.0398838023028,12.456149717707,127.24620830676)) ;
#118357=CARTESIAN_POINT('Ctrl Pts',(-31.1360199136021,12.4116404870963,
127.494111078372)) ;
#118358=CARTESIAN_POINT('Ctrl Pts',(-31.2337338612294,12.4391729305521,
127.746332624112)) ;
#118359=CARTESIAN_POINT('Ctrl Pts',(-31.3254925425336,12.5371797605548,
127.981319248925)) ;
#118360=CARTESIAN_POINT('Ctrl Pts',(-31.4060511368076,12.6985743465351,
128.183537479242)) ;
#118361=CARTESIAN_POINT('Ctrl Pts',(-31.4702234675365,12.9117741381151,
128.337900585384)) ;
#118362=CARTESIAN_POINT('Ctrl Pts',(-31.5142368155557,13.1624013185224,
128.433269095099)) ;
#118363=CARTESIAN_POINT('Ctrl Pts',(-31.5354063774495,13.430527916598,128.462060753588)) ;
#118364=CARTESIAN_POINT('Ctrl Pts',(-31.5331866509304,13.6988963503242,
128.422426334552)) ;
#118365=CARTESIAN_POINT('Ctrl Pts',(-31.5083514057842,13.9472005331235,
128.316764555466)) ;
#118366=CARTESIAN_POINT('Ctrl Pts',(-31.4634662153984,14.1580510542122,
128.152528884923)) ;
#118367=CARTESIAN_POINT('Ctrl Pts',(-31.4022864663549,14.3165352263592,
127.940620929915)) ;
#118368=CARTESIAN_POINT('Ctrl Pts',(-31.3302015606746,14.4105996600904,
127.696931825965)) ;
#118369=CARTESIAN_POINT('Ctrl Pts',(-31.2530012510953,14.4340684661328,
127.438305075934)) ;
#118370=CARTESIAN_POINT('Ctrl Pts',(-31.1767797421025,14.3850544028617,
127.182480796763)) ;
#118371=CARTESIAN_POINT('Ctrl Pts',(-31.1079347894914,14.2669952592305,
126.948227958792)) ;
#118372=CARTESIAN_POINT('Ctrl Pts',(-31.0521981502,14.08911548236,126.752366622373)) ;
#118373=CARTESIAN_POINT('Ctrl Pts',(-31.0139044640317,13.8629229464963,
126.60733955489)) ;
#118374=CARTESIAN_POINT('Ctrl Pts',(-30.996875692622,13.604494449949,126.524362266426)) ;
#118375=CARTESIAN_POINT('Ctrl Pts',(-31.0029129348444,13.3352196406284,
126.509036582526)) ;
#118376=CARTESIAN_POINT('Ctrl Pts',(-31.0323468270102,13.0705830393377,
126.561846564007)) ;
#118377=CARTESIAN_POINT('Ctrl Pts',(-31.0837316199208,12.8316693122143,
126.678854555658)) ;
#118378=CARTESIAN_POINT('Ctrl Pts',(-31.1546013076082,12.6342706901117,
126.852600636445)) ;
#118379=CARTESIAN_POINT('Ctrl Pts',(-31.2394140271486,12.4949548455415,
127.067408352085)) ;
#118380=CARTESIAN_POINT('Ctrl Pts',(-31.334148974029,12.421067631229,127.310966017458)) ;
#118381=CARTESIAN_POINT('Ctrl Pts',(-31.4318092831184,12.4192534681359,
127.563206519924)) ;
#118382=CARTESIAN_POINT('Ctrl Pts',(-31.5267833807971,12.4890550596445,
127.807509458574)) ;
#118383=CARTESIAN_POINT('Ctrl Pts',(-31.6130103693316,12.6269264793826,
128.026107667869)) ;
#118384=CARTESIAN_POINT('Ctrl Pts',(-31.683886847537,12.8196494832229,128.200260557426)) ;
#118385=CARTESIAN_POINT('Ctrl Pts',(-31.7367312073383,13.0580835296679,
128.321322833757)) ;
#118386=CARTESIAN_POINT('Ctrl Pts',(-31.7672152209321,13.321466149626,128.377268196697)) ;
#118387=CARTESIAN_POINT('Ctrl Pts',(-31.7744327469934,13.5912986837364,
128.365332689352)) ;
#118388=CARTESIAN_POINT('Ctrl Pts',(-31.7586348495878,13.8497218506693,
128.286100562908)) ;
#118389=CARTESIAN_POINT('Ctrl Pts',(-31.7212629287116,14.0789422009193,
128.14363667606)) ;
#118390=CARTESIAN_POINT('Ctrl Pts',(-31.6661208521593,14.2597600748466,
127.94943795922)) ;
#118391=CARTESIAN_POINT('Ctrl Pts',(-31.5980586744624,14.3805241466999,
127.717602294976)) ;
#118392=CARTESIAN_POINT('Ctrl Pts',(-31.5221682369762,14.4333051039602,
127.462785155928)) ;
#118393=CARTESIAN_POINT('Ctrl Pts',(-31.444773905692,14.4135763254968,127.203549201476)) ;
#118394=CARTESIAN_POINT('Ctrl Pts',(-31.3722256183231,14.3230160042054,
126.958490867883)) ;
#118395=CARTESIAN_POINT('Ctrl Pts',(-31.3102615819759,14.1669880886898,
126.744210913267)) ;
#118396=CARTESIAN_POINT('Ctrl Pts',(-31.2647484696902,13.9601855279978,
126.578397395436)) ;
#118397=CARTESIAN_POINT('Ctrl Pts',(-31.2386090991305,13.7121979850729,
126.468745833126)) ;
#118398=CARTESIAN_POINT('Ctrl Pts',(-31.2351816147922,13.44532544281,126.425707068262)) ;
#118399=CARTESIAN_POINT('Ctrl Pts',(-31.2552112460232,13.1756579344581,
126.451027766751)) ;
#118400=CARTESIAN_POINT('Ctrl Pts',(-31.2978741375129,12.9248371120238,
126.542620270216)) ;
#118401=CARTESIAN_POINT('Ctrl Pts',(-31.3611235868385,12.7087904185415,
126.694221985858)) ;
#118402=CARTESIAN_POINT('Ctrl Pts',(-31.4409206069476,12.5441839960965,
126.894217297466)) ;
#118403=CARTESIAN_POINT('Ctrl Pts',(-31.5328183036128,12.4422953635853,
127.129402084781)) ;
#118404=CARTESIAN_POINT('Ctrl Pts',(-31.629777727754,12.4112745925655,127.379639841948)) ;
#118405=CARTESIAN_POINT('Ctrl Pts',(-31.7265865855766,12.4523611217467,
127.629332126508)) ;
#118406=CARTESIAN_POINT('Ctrl Pts',(-31.8167258433804,12.5627156193445,
127.859574831218)) ;
#118407=CARTESIAN_POINT('Ctrl Pts',(-31.8949781937964,12.736203215032,128.054846222434)) ;
#118408=CARTESIAN_POINT('Ctrl Pts',(-31.9551628568403,12.9562236735918,
128.197777042418)) ;
#118409=CARTESIAN_POINT('Ctrl Pts',(-31.9952052502965,13.212763202245,128.281413268464)) ;
#118410=CARTESIAN_POINT('Ctrl Pts',(-32.0118603650355,13.4814739437606,
128.297119473937)) ;
#118411=CARTESIAN_POINT('Ctrl Pts',(-32.0053261625225,13.747602021364,128.244879402817)) ;
#118412=CARTESIAN_POINT('Ctrl Pts',(-31.976363124372,13.9907502143909,128.127070663906)) ;
#118413=CARTESIAN_POINT('Ctrl Pts',(-31.9281731309669,14.192126827699,127.953259372413)) ;
#118414=CARTESIAN_POINT('Ctrl Pts',(-31.8646791619465,14.3392030081547,
127.73466416975)) ;
#118415=CARTESIAN_POINT('Ctrl Pts',(-31.7907074399582,14.420750007367,127.485261238863)) ;
#118416=CARTESIAN_POINT('Ctrl Pts',(-31.7134776522141,14.4302362672735,
127.226655866822)) ;
#118417=CARTESIAN_POINT('Ctrl Pts',(-31.6382657139275,14.3680283061645,
126.973823214759)) ;
#118418=CARTESIAN_POINT('Ctrl Pts',(-31.5712774337174,14.237554410734,126.74491844459)) ;
#118419=CARTESIAN_POINT('Ctrl Pts',(-31.5184473639748,14.0487160493496,
126.557435432275)) ;
#118420=CARTESIAN_POINT('Ctrl Pts',(-31.4842054752315,13.8167884864147,
126.424474538241)) ;
#118421=CARTESIAN_POINT('Ctrl Pts',(-31.4713351737196,13.5548285940714,
126.353677668392)) ;
#118422=CARTESIAN_POINT('Ctrl Pts',(-31.4817616498199,13.2844751401064,
126.351080744583)) ;
#118423=CARTESIAN_POINT('Ctrl Pts',(-31.5156125178178,13.0226684871857,
126.416725531107)) ;
#118424=CARTESIAN_POINT('Ctrl Pts',(-31.5707227695967,12.7913020649599,
126.544716939095)) ;
#118425=CARTESIAN_POINT('Ctrl Pts',(-31.6443503598457,12.6040508049077,
126.726654019701)) ;
#118426=CARTESIAN_POINT('Ctrl Pts',(-31.7318689488069,12.4756114262356,
126.949157250561)) ;
#118427=CARTESIAN_POINT('Ctrl Pts',(-31.8274955783218,12.4152434956171,
127.195397643288)) ;
#118428=CARTESIAN_POINT('Ctrl Pts',(-31.9251925407204,12.4269403592131,
127.447704843771)) ;
#118429=CARTESIAN_POINT('Ctrl Pts',(-32.0188886965611,12.5099952735333,
127.688277904106)) ;
#118430=CARTESIAN_POINT('Ctrl Pts',(-32.1025075923148,12.6587328614396,
127.899383697514)) ;
#118431=CARTESIAN_POINT('Ctrl Pts',(-32.1705721069073,12.8618951640278,
128.065119112413)) ;
#118432=CARTESIAN_POINT('Ctrl Pts',(-32.2191904649823,13.1054069389763,
128.174015366068)) ;
#118433=CARTESIAN_POINT('Ctrl Pts',(-32.2455028035797,13.3721986649784,
128.21769238138)) ;
#118434=CARTESIAN_POINT('Ctrl Pts',(-32.2482898332498,13.6415133850086,
128.192782134854)) ;
#118435=CARTESIAN_POINT('Ctrl Pts',(-32.2283241313474,13.8954057097587,
128.101397608046)) ;
#118436=CARTESIAN_POINT('Ctrl Pts',(-32.1872523956957,14.1169004603375,
127.948121743342)) ;
#118437=CARTESIAN_POINT('Ctrl Pts',(-32.1295014317082,14.286862322143,127.74642646493)) ;
#118438=CARTESIAN_POINT('Ctrl Pts',(-32.0592677095131,14.3960130352986,
127.508092927699)) ;
#118439=CARTESIAN_POINT('Ctrl Pts',(-31.9825379384265,14.435114922765,127.250792751949)) ;
#118440=CARTESIAN_POINT('Ctrl Pts',(-31.9057656974593,14.4019052021935,
126.993457606121)) ;
#118441=CARTESIAN_POINT('Ctrl Pts',(-31.8346583979873,14.2983009170395,
126.752533469883)) ;
#118442=CARTESIAN_POINT('Ctrl Pts',(-31.7754887850036,14.1317969214597,
126.546520009402)) ;
#118443=CARTESIAN_POINT('Ctrl Pts',(-31.7332254358825,13.915343377283,126.390014277616)) ;
#118444=CARTESIAN_POINT('Ctrl Pts',(-31.711360602162,13.6633971798664,126.293043315709)) ;
#118445=CARTESIAN_POINT('Ctrl Pts',(-31.7122219084162,13.3943409624926,
126.262475507033)) ;
#118446=CARTESIAN_POINT('Ctrl Pts',(-31.7367708343716,13.1257595222001,
126.300900545406)) ;
#118447=CARTESIAN_POINT('Ctrl Pts',(-31.7835119755956,12.880696500419,126.404440546327)) ;
#118448=CARTESIAN_POINT('Ctrl Pts',(-31.850115664228,12.6734734022958,126.565890689936)) ;
#118449=CARTESIAN_POINT('Ctrl Pts',(-31.9327988513976,12.5195858406816,
126.774213790266)) ;
#118450=CARTESIAN_POINT('Ctrl Pts',(-32.0259263008221,12.4310932858069,
127.013116469777)) ;
#118451=CARTESIAN_POINT('Ctrl Pts',(-32.1231083724527,12.4134132661188,
127.264059856825)) ;
#118452=CARTESIAN_POINT('Ctrl Pts',(-32.2195172413699,12.468118840117,127.512455841876)) ;
#118453=CARTESIAN_POINT('Ctrl Pts',(-32.3075963273976,12.5909169061166,
127.736717735728)) ;
#118454=CARTESIAN_POINT('Ctrl Pts',(-32.3825833685287,12.773448841542,127.922642365176)) ;
#118455=CARTESIAN_POINT('Ctrl Pts',(-32.4396040817083,13.0028153371377,
128.056056344726)) ;
#118456=CARTESIAN_POINT('Ctrl Pts',(-32.4751933014337,13.2626811935882,
128.126823513117)) ;
#118457=CARTESIAN_POINT('Ctrl Pts',(-32.4875431224731,13.5323090949329,
128.129920100657)) ;
#118458=CARTESIAN_POINT('Ctrl Pts',(-32.4765829085235,13.7963542441069,
128.064639049108)) ;
#118459=CARTESIAN_POINT('Ctrl Pts',(-32.4437139481186,14.0324257207359,
127.93549829729)) ;
#118460=CARTESIAN_POINT('Ctrl Pts',(-32.3923709591125,14.2243211070582,
127.752507155027)) ;
#118461=CARTESIAN_POINT('Ctrl Pts',(-32.326532192024,14.3597396565784,127.527047761077)) ;
#118462=CARTESIAN_POINT('Ctrl Pts',(-32.2515288700067,14.4280132025405,
127.274713443137)) ;
#118463=CARTESIAN_POINT('Ctrl Pts',(-32.1739944938922,14.424002708898,127.015108039322)) ;
#118464=CARTESIAN_POINT('Ctrl Pts',(-32.0998540788628,14.3482149181964,
126.765370673455)) ;
#118465=CARTESIAN_POINT('Ctrl Pts',(-32.035455068552,14.2066839719766,126.544210524556)) ;
#118466=CARTESIAN_POINT('Ctrl Pts',(-31.9856410382067,14.0084845387879,
126.365519583357)) ;
#118467=CARTESIAN_POINT('Ctrl Pts',(-31.9550561070796,13.7679164068615,
126.242974606502)) ;
#118468=CARTESIAN_POINT('Ctrl Pts',(-31.9466445164154,13.5034894092934,
126.185316318488)) ;
#118469=CARTESIAN_POINT('Ctrl Pts',(-31.9615283223229,13.2335994760701,
126.195740996152)) ;
#118470=CARTESIAN_POINT('Ctrl Pts',(-31.9994986451266,12.9764076821957,
126.273507891197)) ;
#118471=CARTESIAN_POINT('Ctrl Pts',(-32.0588369991395,12.7508792714819,
126.41360702449)) ;
#118472=CARTESIAN_POINT('Ctrl Pts',(-32.1350060623825,12.5752390770026,
126.603196268328)) ;
#118473=CARTESIAN_POINT('Ctrl Pts',(-32.2244641327029,12.4588915032614,
126.831372157513)) ;
#118474=CARTESIAN_POINT('Ctrl Pts',(-32.3210414704613,12.4118138319928,
127.080368873198)) ;
#118475=CARTESIAN_POINT('Ctrl Pts',(-32.4187885763319,12.4374481797596,
127.332697812372)) ;
#118476=CARTESIAN_POINT('Ctrl Pts',(-32.5107712538563,12.5333386342992,
127.568352341056)) ;
#118477=CARTESIAN_POINT('Ctrl Pts',(-32.5920459321703,12.693967439573,127.772513096516)) ;
#118478=CARTESIAN_POINT('Ctrl Pts',(-32.6563892906433,12.9050030598073,
127.927533769727)) ;
#118479=CARTESIAN_POINT('Ctrl Pts',(-32.7011347368276,13.1551457617761,
128.02498837055)) ;
#118480=CARTESIAN_POINT('Ctrl Pts',(-32.7156355324634,13.3338156180663,
128.045309077602)) ;
#118481=CARTESIAN_POINT('Ctrl Pts',(-32.7190213287863,13.4231220139207,
128.04417910927)) ;
#118482=CARTESIAN_POINT('Ctrl Pts',(-11.3761033793275,13.1734341962953,
133.269779676638)) ;
#118483=CARTESIAN_POINT('Ctrl Pts',(-11.3768069270304,13.1676985193225,
133.271103956166)) ;
#118484=CARTESIAN_POINT('Ctrl Pts',(-11.3882805706462,13.0762043638356,
133.292938899671)) ;
#118485=CARTESIAN_POINT('Ctrl Pts',(-11.4192577565396,12.9034783486566,
133.360456115887)) ;
#118486=CARTESIAN_POINT('Ctrl Pts',(-11.4839335327708,12.6923998158235,
133.516367811255)) ;
#118487=CARTESIAN_POINT('Ctrl Pts',(-11.5648987051196,12.5327609203509,
133.719781427978)) ;
#118488=CARTESIAN_POINT('Ctrl Pts',(-11.6575564098631,12.4368205750072,
133.957184373076)) ;
#118489=CARTESIAN_POINT('Ctrl Pts',(-11.7544962887077,12.4119420230158,
134.20744088849)) ;
#118490=CARTESIAN_POINT('Ctrl Pts',(-11.8513224104514,12.4592681400663,
134.457068268069)) ;
#118491=CARTESIAN_POINT('Ctrl Pts',(-11.9405993691722,12.5756590132109,
134.684776660205)) ;
#118492=CARTESIAN_POINT('Ctrl Pts',(-12.0171777025799,12.7528353886377,
134.875337560121)) ;
#118493=CARTESIAN_POINT('Ctrl Pts',(-12.0761069391572,12.9779971268721,
135.014361241539)) ;
#118494=CARTESIAN_POINT('Ctrl Pts',(-12.1139269193626,13.2349353999384,
135.091728750585)) ;
#118495=CARTESIAN_POINT('Ctrl Pts',(-12.12874362671,13.505181868833,135.101921543684)) ;
#118496=CARTESIAN_POINT('Ctrl Pts',(-12.1200205283876,13.7710456278858,
135.043149515145)) ;
#118497=CARTESIAN_POINT('Ctrl Pts',(-12.0894301826285,14.0095405856191,
134.920825784876)) ;
#118498=CARTESIAN_POINT('Ctrl Pts',(-12.0396580216246,14.2073760437107,
134.742299653733)) ;
#118499=CARTESIAN_POINT('Ctrl Pts',(-11.9750364644313,14.348956944597,134.520409199205)) ;
#118500=CARTESIAN_POINT('Ctrl Pts',(-11.9007138169304,14.4243647503837,
134.270081866618)) ;
#118501=CARTESIAN_POINT('Ctrl Pts',(-11.8231526682833,14.4276726038888,
134.010386566698)) ;
#118502=CARTESIAN_POINT('Ctrl Pts',(-11.7485533763177,14.359284576391,133.759393230076)) ;
#118503=CARTESIAN_POINT('Ctrl Pts',(-11.6827807941158,14.2239082664501,
133.534151570949)) ;
#118504=CARTESIAN_POINT('Ctrl Pts',(-11.6312619715626,14.0309431435162,
133.350500937974)) ;
#118505=CARTESIAN_POINT('Ctrl Pts',(-11.5985513826321,13.7937232390813,
133.221720651928)) ;
#118506=CARTESIAN_POINT('Ctrl Pts',(-11.5878056858426,13.531836984712,133.157350898192)) ;
#118507=CARTESIAN_POINT('Ctrl Pts',(-11.6002475109844,13.2609088557136,
133.160554632561)) ;
#118508=CARTESIAN_POINT('Ctrl Pts',(-11.6360718512436,13.0011531405438,
133.231998502034)) ;
#118509=CARTESIAN_POINT('Ctrl Pts',(-11.6929137966697,12.7729627395585,
133.365036762185)) ;
#118510=CARTESIAN_POINT('Ctrl Pts',(-11.7680839767594,12.590180168645,133.551429864453)) ;
#118511=CARTESIAN_POINT('Ctrl Pts',(-11.856305645623,12.4676467946536,133.776079657559)) ;
#118512=CARTESIAN_POINT('Ctrl Pts',(-11.9527048680969,12.4133145045735,
134.024458200477)) ;
#118513=CARTESIAN_POINT('Ctrl Pts',(-12.0500375750377,12.4313808939379,
134.275789392375)) ;
#118514=CARTESIAN_POINT('Ctrl Pts',(-12.1432845891867,12.5206603265203,
134.514975108993)) ;
#118515=CARTESIAN_POINT('Ctrl Pts',(-12.2255404050775,12.6744195884329,
134.722175891724)) ;
#118516=CARTESIAN_POINT('Ctrl Pts',(-12.2921066353845,12.8815893082003,
134.883533839674)) ;
#118517=CARTESIAN_POINT('Ctrl Pts',(-12.338995449753,13.1290193256912,134.987229585998)) ;
#118518=CARTESIAN_POINT('Ctrl Pts',(-12.3630777682256,13.3950772370959,
135.024620575974)) ;
#118519=CARTESIAN_POINT('Ctrl Pts',(-12.3639615444683,13.664342206485,134.994087920737)) ;
#118520=CARTESIAN_POINT('Ctrl Pts',(-12.3418854317323,13.9170737521182,
134.896381663503)) ;
#118521=CARTESIAN_POINT('Ctrl Pts',(-12.2993936354334,14.1334228172292,
134.739163893756)) ;
#118522=CARTESIAN_POINT('Ctrl Pts',(-12.2403027953976,14.2989215646412,
134.533486314865)) ;
#118523=CARTESIAN_POINT('Ctrl Pts',(-12.1693589392841,14.402143447902,134.293124348418)) ;
#118524=CARTESIAN_POINT('Ctrl Pts',(-12.0922425132794,14.4351203022994,
134.034641516887)) ;
#118525=CARTESIAN_POINT('Ctrl Pts',(-12.0157937728051,14.3956460287634,
133.778272781817)) ;
#118526=CARTESIAN_POINT('Ctrl Pts',(-11.9455441386352,14.2864256341772,
133.539885354215)) ;
#118527=CARTESIAN_POINT('Ctrl Pts',(-11.8876134651553,14.1149876043022,
133.337479609213)) ;
#118528=CARTESIAN_POINT('Ctrl Pts',(-11.8469959298402,13.8950778661998,
133.185808345223)) ;
#118529=CARTESIAN_POINT('Ctrl Pts',(-11.8269465422163,13.6402949079638,
133.094058419286)) ;
#118530=CARTESIAN_POINT('Ctrl Pts',(-11.8299420004692,13.3700135183461,
133.069649454816)) ;
#118531=CARTESIAN_POINT('Ctrl Pts',(-11.8563611483356,13.1040820554216,
133.113728953609)) ;
#118532=CARTESIAN_POINT('Ctrl Pts',(-11.9049819128071,12.8608603578453,
133.222664719387)) ;
#118533=CARTESIAN_POINT('Ctrl Pts',(-11.9735329306437,12.6570995418072,
133.389655526666)) ;
#118534=CARTESIAN_POINT('Ctrl Pts',(-12.0567368640633,12.5097125952048,
133.599752815498)) ;
#118535=CARTESIAN_POINT('Ctrl Pts',(-12.150523561375,12.4266925714705,133.840558741675)) ;
#118536=CARTESIAN_POINT('Ctrl Pts',(-12.2483173423649,12.4153566152999,
134.093120553544)) ;
#118537=CARTESIAN_POINT('Ctrl Pts',(-12.3439234591775,12.4761183658278,
134.339297297897)) ;
#118538=CARTESIAN_POINT('Ctrl Pts',(-12.4312344046572,12.604611036471,134.561252185302)) ;
#118539=CARTESIAN_POINT('Ctrl Pts',(-12.5048720957458,12.7920329725734,
134.743205846723)) ;
#118540=CARTESIAN_POINT('Ctrl Pts',(-12.5600519020243,13.0246460204259,
134.871261784406)) ;
#118541=CARTESIAN_POINT('Ctrl Pts',(-12.5935838556551,13.2849676562724,
134.936178375483)) ;
#118542=CARTESIAN_POINT('Ctrl Pts',(-12.6040097500515,13.5561839498762,
134.933470648802)) ;
#118543=CARTESIAN_POINT('Ctrl Pts',(-12.5909871097811,13.8182130447303,
134.862208918049)) ;
#118544=CARTESIAN_POINT('Ctrl Pts',(-12.5565449767689,14.0504674828932,
134.728585321904)) ;
#118545=CARTESIAN_POINT('Ctrl Pts',(-12.503409625585,14.2392688566164,134.540126621614)) ;
#118546=CARTESIAN_POINT('Ctrl Pts',(-12.4364541228854,14.3686949061628,
134.311393774839)) ;
#118547=CARTESIAN_POINT('Ctrl Pts',(-12.3615656889771,14.4303698699092,
134.059658526159)) ;
#118548=CARTESIAN_POINT('Ctrl Pts',(-12.2839010334425,14.4203874335836,
133.799592770568)) ;
#118549=CARTESIAN_POINT('Ctrl Pts',(-12.210160099743,14.3383234077631,133.550939985876)) ;
#118550=CARTESIAN_POINT('Ctrl Pts',(-12.1467675345913,14.1909246948651,
133.332649057125)) ;
#118551=CARTESIAN_POINT('Ctrl Pts',(-12.0987599970841,13.9894771952072,
133.159415008421)) ;
#118552=CARTESIAN_POINT('Ctrl Pts',(-12.0699641262129,13.746808334038,133.042174065414)) ;
#118553=CARTESIAN_POINT('Ctrl Pts',(-12.0634132082792,13.4802543050363,
132.989840642035)) ;
#118554=CARTESIAN_POINT('Ctrl Pts',(-12.0805388848431,13.2092850864011,
133.006627337963)) ;
#118555=CARTESIAN_POINT('Ctrl Pts',(-12.1201612936325,12.9563426654799,
133.089494153688)) ;
#118556=CARTESIAN_POINT('Ctrl Pts',(-12.1810219658941,12.7340442860679,
133.234040793985)) ;
#118557=CARTESIAN_POINT('Ctrl Pts',(-12.2591406672729,12.5620254392794,
133.429068728692)) ;
#118558=CARTESIAN_POINT('Ctrl Pts',(-12.3489444975325,12.4521634534599,
133.65845210476)) ;
#118559=CARTESIAN_POINT('Ctrl Pts',(-12.4462656769572,12.411069828673,133.909474442869)) ;
#118560=CARTESIAN_POINT('Ctrl Pts',(-12.5435407529999,12.4431134787165,
134.160514267981)) ;
#118561=CARTESIAN_POINT('Ctrl Pts',(-12.6346576814472,12.544720782059,134.393675748219)) ;
#118562=CARTESIAN_POINT('Ctrl Pts',(-12.7144928520191,12.7094608145556,
134.593760742519)) ;
#118563=CARTESIAN_POINT('Ctrl Pts',(-12.7777519327944,12.9261933483464,
134.745327776743)) ;
#118564=CARTESIAN_POINT('Ctrl Pts',(-12.8202519877699,13.176771832056,134.836492242179)) ;
#118565=CARTESIAN_POINT('Ctrl Pts',(-12.8402444603128,13.4474343122789,
134.861590595176)) ;
#118566=CARTESIAN_POINT('Ctrl Pts',(-12.8365305004501,13.7143157583518,
134.817690205497)) ;
#118567=CARTESIAN_POINT('Ctrl Pts',(-12.8106142510612,13.9601208974721,
134.708988844887)) ;
#118568=CARTESIAN_POINT('Ctrl Pts',(-12.7644642354226,14.1691500345588,
134.540915011046)) ;
#118569=CARTESIAN_POINT('Ctrl Pts',(-12.7028017761949,14.3234012984993,
134.327766826278)) ;
#118570=CARTESIAN_POINT('Ctrl Pts',(-12.6301549587558,14.4138714488527,
134.082373591679)) ;
#118571=CARTESIAN_POINT('Ctrl Pts',(-12.5529215600028,14.4332950677581,
133.82368743641)) ;
#118572=CARTESIAN_POINT('Ctrl Pts',(-12.4766195880281,14.3798376866145,
133.567474761174)) ;
#118573=CARTESIAN_POINT('Ctrl Pts',(-12.4087004001394,14.2584887466458,
133.336079424252)) ;
#118574=CARTESIAN_POINT('Ctrl Pts',(-12.3536722242535,14.0772214658074,
133.142205477393)) ;
#118575=CARTESIAN_POINT('Ctrl Pts',(-12.3164993112394,13.8478580499734,
133.000351309794)) ;
#118576=CARTESIAN_POINT('Ctrl Pts',(-12.3008731181985,13.5896599466639,
132.921665266495)) ;
#118577=CARTESIAN_POINT('Ctrl Pts',(-12.3082135346213,13.3195389388511,
132.910059027627)) ;
#118578=CARTESIAN_POINT('Ctrl Pts',(-12.3390393214159,13.0556170681804,
132.966906320988)) ;
#118579=CARTESIAN_POINT('Ctrl Pts',(-12.3916342065595,12.818934352168,133.087465135038)) ;
#118580=CARTESIAN_POINT('Ctrl Pts',(-12.4631451106269,12.6251003449816,
133.263222547425)) ;
#118581=CARTESIAN_POINT('Ctrl Pts',(-12.548985341136,12.4887479439426,133.48089248249)) ;
#118582=CARTESIAN_POINT('Ctrl Pts',(-12.6437484005123,12.4190670413713,
133.724650221671)) ;
#118583=CARTESIAN_POINT('Ctrl Pts',(-12.7419392728048,12.4213699793115,
133.978259231315)) ;
#118584=CARTESIAN_POINT('Ctrl Pts',(-12.836294926695,12.4953802453317,134.220834452806)) ;
#118585=CARTESIAN_POINT('Ctrl Pts',(-12.9215231107959,12.6359572118525,
134.436656343271)) ;
#118586=CARTESIAN_POINT('Ctrl Pts',(-12.9919038366036,12.8329197331058,
134.609132207882)) ;
#118587=CARTESIAN_POINT('Ctrl Pts',(-13.0431941881955,13.0719649791817,
134.725860231311)) ;
#118588=CARTESIAN_POINT('Ctrl Pts',(-13.0725075844949,13.3363497207088,
134.77836223128)) ;
#118589=CARTESIAN_POINT('Ctrl Pts',(-13.0784119937401,13.6070576774105,
134.762468724094)) ;
#118590=CARTESIAN_POINT('Ctrl Pts',(-13.0612042244902,13.8644611915849,
134.679071115725)) ;
#118591=CARTESIAN_POINT('Ctrl Pts',(-13.0229223196548,14.0900773002825,
134.534142554414)) ;
#118592=CARTESIAN_POINT('Ctrl Pts',(-12.9668857918559,14.2682172577694,
134.337289258471)) ;
#118593=CARTESIAN_POINT('Ctrl Pts',(-12.898149301531,14.385416608164,134.10344537434)) ;
#118594=CARTESIAN_POINT('Ctrl Pts',(-12.8220030996413,14.4341663222017,
133.847878057457)) ;
#118595=CARTESIAN_POINT('Ctrl Pts',(-12.7445691235808,14.4102121268538,
133.58846496535)) ;
#118596=CARTESIAN_POINT('Ctrl Pts',(-12.6725877902746,14.3156229092393,
133.345094836696)) ;
#118597=CARTESIAN_POINT('Ctrl Pts',(-12.6115971411473,14.157111727064,133.133799779272)) ;
#118598=CARTESIAN_POINT('Ctrl Pts',(-12.566783250654,13.9459764019392,132.96976134338)) ;
#118599=CARTESIAN_POINT('Ctrl Pts',(-12.5420765503289,13.6975622305703,
132.864482081499)) ;
#118600=CARTESIAN_POINT('Ctrl Pts',(-12.53995666575,13.4293975003276,132.825169963598)) ;
#118601=CARTESIAN_POINT('Ctrl Pts',(-12.5612578432039,13.1610019390536,
132.854307434728)) ;
#118602=CARTESIAN_POINT('Ctrl Pts',(-12.6053825198436,12.910584846224,132.95000917613)) ;
#118603=CARTESIAN_POINT('Ctrl Pts',(-12.6696450944826,12.6976134707592,
133.10463582855)) ;
#118604=CARTESIAN_POINT('Ctrl Pts',(-12.7502997842175,12.536442281865,133.307124586035)) ;
#118605=CARTESIAN_POINT('Ctrl Pts',(-12.8422220552916,12.4387732267397,
133.542548790537)) ;
#118606=CARTESIAN_POINT('Ctrl Pts',(-12.9398571626702,12.4116342438423,
133.794574286652)) ;
#118607=CARTESIAN_POINT('Ctrl Pts',(-13.0363065622486,12.4569142421678,
134.04327039679)) ;
#118608=CARTESIAN_POINT('Ctrl Pts',(-13.1260272439089,12.5714751922183,
134.272219310858)) ;
#118609=CARTESIAN_POINT('Ctrl Pts',(-13.2029202315668,12.7468633179545,
134.463749827211)) ;
#118610=CARTESIAN_POINT('Ctrl Pts',(-13.2624243662056,12.9706872906827,
134.604464814153)) ;
#118611=CARTESIAN_POINT('Ctrl Pts',(-13.3009328039148,13.2271705417113,
134.683814778475)) ;
#118612=CARTESIAN_POINT('Ctrl Pts',(-13.3164246163393,13.4971329945125,
134.69600029026)) ;
#118613=CARTESIAN_POINT('Ctrl Pts',(-13.3083964010065,13.7633005745665,
134.639275314715)) ;
#118614=CARTESIAN_POINT('Ctrl Pts',(-13.2784711170363,14.0028268383939,
134.518902238097)) ;
#118615=CARTESIAN_POINT('Ctrl Pts',(-13.2289588566988,14.2028677697453,
134.340991546535)) ;
#118616=CARTESIAN_POINT('Ctrl Pts',(-13.1649219288007,14.3455611528234,
134.120940152505)) ;
#118617=CARTESIAN_POINT('Ctrl Pts',(-13.0908084734639,14.4231516441217,
133.871220084537)) ;
#118618=CARTESIAN_POINT('Ctrl Pts',(-13.0132392773694,14.428665737009,133.611497374306)) ;
#118619=CARTESIAN_POINT('Ctrl Pts',(-12.9383171503362,14.3621069846461,
133.3594868622)) ;
#118620=CARTESIAN_POINT('Ctrl Pts',(-12.872270725288,14.2287343396627,133.133488008975)) ;
#118621=CARTESIAN_POINT('Ctrl Pts',(-12.8201528022822,14.0363061322534,
132.947956133022)) ;
#118622=CARTESIAN_POINT('Ctrl Pts',(-12.7871145635481,13.8023697285695,
132.818530704553)) ;
#118623=CARTESIAN_POINT('Ctrl Pts',(-12.7755307033747,13.5388532599518,
132.751430578147)) ;
#118624=CARTESIAN_POINT('Ctrl Pts',(-12.7874147952686,13.2684518599204,
132.753076122246)) ;
#118625=CARTESIAN_POINT('Ctrl Pts',(-12.8223738829444,13.0087997166185,
132.822096605802)) ;
#118626=CARTESIAN_POINT('Ctrl Pts',(-12.8791405427355,12.7778890822412,
132.954659158962)) ;
#118627=CARTESIAN_POINT('Ctrl Pts',(-12.9533257274006,12.5950173960976,
133.138428418753)) ;
#118628=CARTESIAN_POINT('Ctrl Pts',(-13.0416625952284,12.4700325121189,
133.363244570128)) ;
#118629=CARTESIAN_POINT('Ctrl Pts',(-13.1373825064978,12.4138573722268,
133.609834541986)) ;
#118630=CARTESIAN_POINT('Ctrl Pts',(-13.2356240525979,12.4301864266095,
133.863515438704)) ;
#118631=CARTESIAN_POINT('Ctrl Pts',(-13.3280894934625,12.5166844150512,
134.100777833648)) ;
#118632=CARTESIAN_POINT('Ctrl Pts',(-13.4112528177748,12.6693064963876,
134.310434251688)) ;
#118633=CARTESIAN_POINT('Ctrl Pts',(-13.4780909825541,12.8745471287187,
134.472698922864)) ;
#118634=CARTESIAN_POINT('Ctrl Pts',(-13.5257121495714,13.1212023718215,
134.578500578674)) ;
#118635=CARTESIAN_POINT('Ctrl Pts',(-13.5504942774336,13.3871939110425,
134.617905019548)) ;
#118636=CARTESIAN_POINT('Ctrl Pts',(-13.5520362091492,13.6567281745513,
134.58928459527)) ;
#118637=CARTESIAN_POINT('Ctrl Pts',(-13.5306752870686,13.9097854264049,
134.493733920305)) ;
#118638=CARTESIAN_POINT('Ctrl Pts',(-13.4886113688084,14.1280196368697,
134.337667087445)) ;
#118639=CARTESIAN_POINT('Ctrl Pts',(-13.4300006465922,14.2950456004005,
134.133430228144)) ;
#118640=CARTESIAN_POINT('Ctrl Pts',(-13.3588662565052,14.4005267631623,
133.89231315706)) ;
#118641=CARTESIAN_POINT('Ctrl Pts',(-13.2823506329123,14.4350836721885,
133.635816652807)) ;
#118642=CARTESIAN_POINT('Ctrl Pts',(-13.205705858747,14.397803897227,133.378829605741)) ;
#118643=CARTESIAN_POINT('Ctrl Pts',(-13.1352707452639,14.2905756800978,
133.139940320595)) ;
#118644=CARTESIAN_POINT('Ctrl Pts',(-13.0769038461577,14.1209511451637,
132.936271017707)) ;
#118645=CARTESIAN_POINT('Ctrl Pts',(-13.0356468946471,13.9018371823522,
132.78266797249)) ;
#118646=CARTESIAN_POINT('Ctrl Pts',(-13.0150200866047,13.6479071387663,
132.689251355067)) ;
#118647=CARTESIAN_POINT('Ctrl Pts',(-13.0172505947305,13.378501800303,132.662693599669)) ;
#118648=CARTESIAN_POINT('Ctrl Pts',(-13.0431950965829,13.1105161208594,
132.705174926483)) ;
#118649=CARTESIAN_POINT('Ctrl Pts',(-13.0910470050457,12.8677236673919,
132.812031740223)) ;
#118650=CARTESIAN_POINT('Ctrl Pts',(-13.1588500660242,12.662830762423,132.976909729655)) ;
#118651=CARTESIAN_POINT('Ctrl Pts',(-13.241879425623,12.513091865374,133.186406240102)) ;
#118652=CARTESIAN_POINT('Ctrl Pts',(-13.335714202403,12.4280189029097,133.427266782244)) ;
#118653=CARTESIAN_POINT('Ctrl Pts',(-13.4331919707127,12.4146728655739,
133.679002405755)) ;
#118654=CARTESIAN_POINT('Ctrl Pts',(-13.529167232764,12.473418288016,133.9261846977)) ;
#118655=CARTESIAN_POINT('Ctrl Pts',(-13.616885586122,12.6005220564223,134.149279369247)) ;
#118656=CARTESIAN_POINT('Ctrl Pts',(-13.6906060457598,12.7855011637684,
134.331642511686)) ;
#118657=CARTESIAN_POINT('Ctrl Pts',(-13.7464767458507,13.0169860566136,
134.461699644794)) ;
#118658=CARTESIAN_POINT('Ctrl Pts',(-13.7807535613475,13.2774553414867,
134.52870436425)) ;
#118659=CARTESIAN_POINT('Ctrl Pts',(-13.7917957698787,13.5483711409958,
134.527829507085)) ;
#118660=CARTESIAN_POINT('Ctrl Pts',(-13.7795542716983,13.8100859907312,
134.458968320121)) ;
#118661=CARTESIAN_POINT('Ctrl Pts',(-13.7455979084497,14.0443620014337,
134.326633872772)) ;
#118662=CARTESIAN_POINT('Ctrl Pts',(-13.6931373802941,14.2339606584883,
134.140272341113)) ;
#118663=CARTESIAN_POINT('Ctrl Pts',(-13.6265708969899,14.3656339537851,
133.912671017341)) ;
#118664=CARTESIAN_POINT('Ctrl Pts',(-13.5514661250035,14.4296685423803,
133.660141235671)) ;
#118665=CARTESIAN_POINT('Ctrl Pts',(-13.4739953762964,14.4216217772437,
133.400732222126)) ;
#118666=CARTESIAN_POINT('Ctrl Pts',(-13.4003044829647,14.3422174229119,
133.152352720469)) ;
#118667=CARTESIAN_POINT('Ctrl Pts',(-13.3362641407276,14.1963612940614,
132.932055167752)) ;
#118668=CARTESIAN_POINT('Ctrl Pts',(-13.2876475135786,13.9958156297376,
132.756967432803)) ;
#118669=CARTESIAN_POINT('Ctrl Pts',(-13.2582843417661,13.7540871657713,
132.638075405849)) ;
#118670=CARTESIAN_POINT('Ctrl Pts',(-13.2510678261576,13.4887318093835,
132.583893441065)) ;
#118671=CARTESIAN_POINT('Ctrl Pts',(-13.2674127122864,13.2176490073036,
132.5984066129)) ;
#118672=CARTESIAN_POINT('Ctrl Pts',(-13.3065305530606,12.9629384302475,
132.679668636195)) ;
#118673=CARTESIAN_POINT('Ctrl Pts',(-13.366974380418,12.739445641898,132.822966776447)) ;
#118674=CARTESIAN_POINT('Ctrl Pts',(-13.4441917545612,12.5666312573546,
133.015548468246)) ;
#118675=CARTESIAN_POINT('Ctrl Pts',(-13.5342140472049,12.4542159373709,
133.245381617091)) ;
#118676=CARTESIAN_POINT('Ctrl Pts',(-13.6308745371879,12.4113528375642,
133.494668076726)) ;
#118677=CARTESIAN_POINT('Ctrl Pts',(-13.7284554191117,12.4409689765868,
133.746525962875)) ;
#118678=CARTESIAN_POINT('Ctrl Pts',(-13.8202195933766,12.5412370849313,
133.981433403131)) ;
#118679=CARTESIAN_POINT('Ctrl Pts',(-13.9001905656391,12.7041353047709,
134.181997916387)) ;
#118680=CARTESIAN_POINT('Ctrl Pts',(-13.9637943476695,12.9183855347654,
134.334727271198)) ;
#118681=CARTESIAN_POINT('Ctrl Pts',(-14.0071906666907,13.1698655571926,
134.428284860126)) ;
#118682=CARTESIAN_POINT('Ctrl Pts',(-14.0277193594189,13.4380609714907,
134.455227938298)) ;
#118683=CARTESIAN_POINT('Ctrl Pts',(-14.0247819555589,13.7071666281258,
134.413364904376)) ;
#118684=CARTESIAN_POINT('Ctrl Pts',(-13.9993507533856,13.95380880599,134.306063795002)) ;
#118685=CARTESIAN_POINT('Ctrl Pts',(-13.9539517208912,14.1634527040787,
134.14031710819)) ;
#118686=CARTESIAN_POINT('Ctrl Pts',(-13.8923677928476,14.3201289862677,
133.927232128965)) ;
#118687=CARTESIAN_POINT('Ctrl Pts',(-13.8202667339251,14.4121340944115,
133.683587595144)) ;
#118688=CARTESIAN_POINT('Ctrl Pts',(-13.742809080042,14.4336855937072,133.424119840857)) ;
#118689=CARTESIAN_POINT('Ctrl Pts',(-13.6668608280909,14.3827385924792,
133.169159916255)) ;
#118690=CARTESIAN_POINT('Ctrl Pts',(-13.5981295475996,14.2627494461532,
132.935168649536)) ;
#118691=CARTESIAN_POINT('Ctrl Pts',(-13.5426656002654,14.0822576993362,
132.739956868766)) ;
#118692=CARTESIAN_POINT('Ctrl Pts',(-13.5052230771177,13.856193146146,132.597618261521)) ;
#118693=CARTESIAN_POINT('Ctrl Pts',(-13.4887623843814,13.5974242111817,
132.516323439236)) ;
#118694=CARTESIAN_POINT('Ctrl Pts',(-13.4954472616452,13.3273251704849,
132.502803308112)) ;
#118695=CARTESIAN_POINT('Ctrl Pts',(-13.5257309046639,13.062291125414,132.55797992157)) ;
#118696=CARTESIAN_POINT('Ctrl Pts',(-13.5775428431027,12.8256130125541,
132.676388959343)) ;
#118697=CARTESIAN_POINT('Ctrl Pts',(-13.6485285477905,12.6301798373562,
132.850606152527)) ;
#118698=CARTESIAN_POINT('Ctrl Pts',(-13.7340252244735,12.4918476261695,
133.067265702632)) ;
#118699=CARTESIAN_POINT('Ctrl Pts',(-13.8290183989182,12.4199209769537,
133.311555769525)) ;
#118700=CARTESIAN_POINT('Ctrl Pts',(-13.9270636548616,12.4204246059211,
133.564789863863)) ;
#118701=CARTESIAN_POINT('Ctrl Pts',(-14.0213478504549,12.492159634428,133.807246350047)) ;
#118702=CARTESIAN_POINT('Ctrl Pts',(-14.1070156184682,12.6310173484571,
134.024319850583)) ;
#118703=CARTESIAN_POINT('Ctrl Pts',(-14.1778290426334,12.8262647723397,
134.198098948728)) ;
#118704=CARTESIAN_POINT('Ctrl Pts',(-14.2297952112719,13.0646914718589,
134.316746137298)) ;
#118705=CARTESIAN_POINT('Ctrl Pts',(-14.259734937754,13.3278245014775,134.371176497314)) ;
#118706=CARTESIAN_POINT('Ctrl Pts',(-14.2663521460769,13.5998586000628,
134.357209920682)) ;
#118707=CARTESIAN_POINT('Ctrl Pts',(-14.2498316891277,13.8569827516154,
134.275942445626)) ;
#118708=CARTESIAN_POINT('Ctrl Pts',(-14.2120572185788,14.0842219381739,
134.132424698552)) ;
#118709=CARTESIAN_POINT('Ctrl Pts',(-14.1566892395711,14.2634336188574,
133.937641912658)) ;
#118710=CARTESIAN_POINT('Ctrl Pts',(-14.0878220989839,14.3833954818559,
133.703202208994)) ;
#118711=CARTESIAN_POINT('Ctrl Pts',(-14.0117161826671,14.433698045123,133.447730780154)) ;
#118712=CARTESIAN_POINT('Ctrl Pts',(-13.9347372020107,14.412015772317,133.189865782114)) ;
#118713=CARTESIAN_POINT('Ctrl Pts',(-13.8622959354617,14.319294669833,132.945054536655)) ;
#118714=CARTESIAN_POINT('Ctrl Pts',(-13.8009553728816,14.16255830471,132.732761956331)) ;
#118715=CARTESIAN_POINT('Ctrl Pts',(-13.7554963594563,13.9521768757504,
132.566750983519)) ;
#118716=CARTESIAN_POINT('Ctrl Pts',(-13.7302700360325,13.7045477413862,
132.459961598635)) ;
#118717=CARTESIAN_POINT('Ctrl Pts',(-13.7274455850892,13.4377490344594,
132.41872307)) ;
#118718=CARTESIAN_POINT('Ctrl Pts',(-13.7481931708221,13.1678476271901,
132.446083972868)) ;
#118719=CARTESIAN_POINT('Ctrl Pts',(-13.7915277802669,12.917659013908,132.539618023673)) ;
#118720=CARTESIAN_POINT('Ctrl Pts',(-13.855533519147,12.7025601696351,132.693352244411)) ;
#118721=CARTESIAN_POINT('Ctrl Pts',(-13.9353887493187,12.5405894739967,
132.893677963618)) ;
#118722=CARTESIAN_POINT('Ctrl Pts',(-14.027297883474,12.4405287595892,133.128967601787)) ;
#118723=CARTESIAN_POINT('Ctrl Pts',(-14.124837017402,12.4114132283242,133.380726658666)) ;
#118724=CARTESIAN_POINT('Ctrl Pts',(-14.2213484874047,12.4546443819082,
133.629616296311)) ;
#118725=CARTESIAN_POINT('Ctrl Pts',(-14.3111929481664,12.5668919742526,
133.858998159138)) ;
#118726=CARTESIAN_POINT('Ctrl Pts',(-14.3889051145816,12.7415276223377,
134.052758598693)) ;
#118727=CARTESIAN_POINT('Ctrl Pts',(-14.4487819994688,12.963899300171,134.194625958176)) ;
#118728=CARTESIAN_POINT('Ctrl Pts',(-14.4878921741366,13.2191082670462,
134.275803667982)) ;
#118729=CARTESIAN_POINT('Ctrl Pts',(-14.5040836850349,13.4893534858843,
134.289979202675)) ;
#118730=CARTESIAN_POINT('Ctrl Pts',(-14.4967928296328,13.7553188833262,
134.235494967527)) ;
#118731=CARTESIAN_POINT('Ctrl Pts',(-14.4672977855729,13.9971251681561,
134.116192347562)) ;
#118732=CARTESIAN_POINT('Ctrl Pts',(-14.4183840345143,14.1977811573069,
133.940137499588)) ;
#118733=CARTESIAN_POINT('Ctrl Pts',(-14.3547061912952,14.3424510805747,
133.721119079194)) ;
#118734=CARTESIAN_POINT('Ctrl Pts',(-14.2805016481878,14.4220642873528,
133.471015964754)) ;
#118735=CARTESIAN_POINT('Ctrl Pts',(-14.2033365143345,14.429449097017,133.212639286996)) ;
#118736=CARTESIAN_POINT('Ctrl Pts',(-14.1282860163884,14.3652072331767,
132.960276109633)) ;
#118737=CARTESIAN_POINT('Ctrl Pts',(-14.0618281815478,14.2335291681656,
132.73303684308)) ;
#118738=CARTESIAN_POINT('Ctrl Pts',(-14.0092524260735,14.0429179829767,
132.546208320143)) ;
#118739=CARTESIAN_POINT('Ctrl Pts',(-13.9755602690746,13.8093220415122,
132.414774751923)) ;
#118740=CARTESIAN_POINT('Ctrl Pts',(-13.9633085026902,13.5476217971459,
132.345885885849)) ;
#118741=CARTESIAN_POINT('Ctrl Pts',(-13.9746025661185,13.2750711815888,
132.345545153662)) ;
#118742=CARTESIAN_POINT('Ctrl Pts',(-14.0088332469759,13.0163164213971,
132.412617107112)) ;
#118743=CARTESIAN_POINT('Ctrl Pts',(-14.064784241679,12.7846451556795,132.542871054114)) ;
#118744=CARTESIAN_POINT('Ctrl Pts',(-14.1387306401708,12.5995256384001,
132.725831674418)) ;
#118745=CARTESIAN_POINT('Ctrl Pts',(-14.2267816071698,12.4726551517152,
132.949805912223)) ;
#118746=CARTESIAN_POINT('Ctrl Pts',(-14.3224320561303,12.4145513421249,
133.19616672507)) ;
#118747=CARTESIAN_POINT('Ctrl Pts',(-14.4201984857976,12.4284690605263,
133.448637711958)) ;
#118748=CARTESIAN_POINT('Ctrl Pts',(-14.5134883154838,12.5133431684666,
133.688097238147)) ;
#118749=CARTESIAN_POINT('Ctrl Pts',(-14.5969649871232,12.6644367182662,
133.898678980795)) ;
#118750=CARTESIAN_POINT('Ctrl Pts',(-14.6641763539161,12.8679925564765,
134.062089198708)) ;
#118751=CARTESIAN_POINT('Ctrl Pts',(-14.7123711551398,13.1131690365504,
134.169635545851)) ;
#118752=CARTESIAN_POINT('Ctrl Pts',(-14.7379481518439,13.3800002802051,
134.211213153089)) ;
#118753=CARTESIAN_POINT('Ctrl Pts',(-14.7400542154875,13.6495651704166,
134.18425698349)) ;
#118754=CARTESIAN_POINT('Ctrl Pts',(-14.7194527468048,13.9023388943094,
134.091064092335)) ;
#118755=CARTESIAN_POINT('Ctrl Pts',(-14.6778190034174,14.1226577783971,
133.936136558405)) ;
#118756=CARTESIAN_POINT('Ctrl Pts',(-14.6196935304185,14.2908247544057,
133.733378266289)) ;
#118757=CARTESIAN_POINT('Ctrl Pts',(-14.5492150216665,14.3981040604,133.494335232995)) ;
#118758=CARTESIAN_POINT('Ctrl Pts',(-14.4722411376038,14.4352626925802,
133.236261337413)) ;
#118759=CARTESIAN_POINT('Ctrl Pts',(-14.3954256541312,14.3995540245642,
132.978732791801)) ;
#118760=CARTESIAN_POINT('Ctrl Pts',(-14.3250767517661,14.2948938638273,
132.740267779799)) ;
#118761=CARTESIAN_POINT('Ctrl Pts',(-14.2659553830164,14.125950965529,132.534203861649)) ;
#118762=CARTESIAN_POINT('Ctrl Pts',(-14.2243526466944,13.9085226432365,
132.379690324383)) ;
#118763=CARTESIAN_POINT('Ctrl Pts',(-14.2030975765256,13.655740461518,132.284483495896)) ;
#118764=CARTESIAN_POINT('Ctrl Pts',(-14.2046245934485,13.3866405451627,
132.255884182945)) ;
#118765=CARTESIAN_POINT('Ctrl Pts',(-14.2298902227146,13.1181024213027,
132.296361021273)) ;
#118766=CARTESIAN_POINT('Ctrl Pts',(-14.2771378969919,12.8743682814219,
132.401446588546)) ;
#118767=CARTESIAN_POINT('Ctrl Pts',(-14.3444307231662,12.6679957327003,
132.564825469235)) ;
#118768=CARTESIAN_POINT('Ctrl Pts',(-14.4272321374204,12.5164144034558,
132.773604557212)) ;
#118769=CARTESIAN_POINT('Ctrl Pts',(-14.5205022334955,12.4295970264179,
133.012939067384)) ;
#118770=CARTESIAN_POINT('Ctrl Pts',(-14.6182514403091,12.4140261333183,
133.265360142286)) ;
#118771=CARTESIAN_POINT('Ctrl Pts',(-14.7142174515708,12.4707103278581,
133.512570298941)) ;
#118772=CARTESIAN_POINT('Ctrl Pts',(-14.8022488129207,12.5959068144279,
133.736577659016)) ;
#118773=CARTESIAN_POINT('Ctrl Pts',(-14.876456590018,12.7791142632462,133.920383734278)) ;
#118774=CARTESIAN_POINT('Ctrl Pts',(-14.9332273811375,13.0114293123004,
134.052815872987)) ;
#118775=CARTESIAN_POINT('Ctrl Pts',(-14.9677728031387,13.2689899400059,
134.120913863117)) ;
#118776=CARTESIAN_POINT('Ctrl Pts',(-14.9796228556439,13.5409257328685,
134.122263271617)) ;
#118777=CARTESIAN_POINT('Ctrl Pts',(-14.9679885894929,13.8029840857302,
134.055199600153)) ;
#118778=CARTESIAN_POINT('Ctrl Pts',(-14.9345699006002,14.0385608749257,
133.924394571764)) ;
#118779=CARTESIAN_POINT('Ctrl Pts',(-14.8825727950335,14.2294231057281,
133.739404880922)) ;
#118780=CARTESIAN_POINT('Ctrl Pts',(-14.816446608533,14.3627051490732,133.513143288359)) ;
#118781=CARTESIAN_POINT('Ctrl Pts',(-14.741468869848,14.428833416405,133.260966751182)) ;
#118782=CARTESIAN_POINT('Ctrl Pts',(-14.6639502642104,14.4228924472986,
133.001406958395)) ;
#118783=CARTESIAN_POINT('Ctrl Pts',(-14.5898577797733,14.3451234315922,
132.75175728098)) ;
#118784=CARTESIAN_POINT('Ctrl Pts',(-14.5255775888799,14.2008972781255,
132.530791080979)) ;
#118785=CARTESIAN_POINT('Ctrl Pts',(-14.4766080099444,14.0023960154245,
132.354775246245)) ;
#118786=CARTESIAN_POINT('Ctrl Pts',(-14.4465779509174,13.761031796391,132.233855249639)) ;
#118787=CARTESIAN_POINT('Ctrl Pts',(-14.4387588071979,13.4967569826491,
132.177998148648)) ;
#118788=CARTESIAN_POINT('Ctrl Pts',(-14.4543340091487,13.2257685669237,
132.19029344318)) ;
#118789=CARTESIAN_POINT('Ctrl Pts',(-14.4929582457325,12.9695426329055,
132.270003328001)) ;
#118790=CARTESIAN_POINT('Ctrl Pts',(-14.5526587987454,12.7456271817385,
132.411240190467)) ;
#118791=CARTESIAN_POINT('Ctrl Pts',(-14.6294318722115,12.5709695365104,
132.602507669175)) ;
#118792=CARTESIAN_POINT('Ctrl Pts',(-14.7192820441727,12.4565179124428,
132.831796466456)) ;
#118793=CARTESIAN_POINT('Ctrl Pts',(-14.8158579152677,12.411477377022,133.080829972233)) ;
#118794=CARTESIAN_POINT('Ctrl Pts',(-14.9138628191828,12.4394645473503,
133.333796557217)) ;
#118795=CARTESIAN_POINT('Ctrl Pts',(-15.0051613513395,12.5368907011572,
133.567613056464)) ;
#118796=CARTESIAN_POINT('Ctrl Pts',(-15.0862176428517,12.6994727139768,
133.771061042229)) ;
#118797=CARTESIAN_POINT('Ctrl Pts',(-15.1499237960889,12.9112843857967,
133.924296026103)) ;
#118798=CARTESIAN_POINT('Ctrl Pts',(-15.1942053675931,13.1634090116609,
134.020242245567)) ;
#118799=CARTESIAN_POINT('Ctrl Pts',(-15.2151706961316,13.4300956070728,
134.048622364032)) ;
#118800=CARTESIAN_POINT('Ctrl Pts',(-15.2130719138631,13.698548706025,134.009335703669)) ;
#118801=CARTESIAN_POINT('Ctrl Pts',(-15.1880474111806,13.948024671753,133.902954348406)) ;
#118802=CARTESIAN_POINT('Ctrl Pts',(-15.1433584082714,14.1576527891806,
133.739468144445)) ;
#118803=CARTESIAN_POINT('Ctrl Pts',(-15.0822635591605,14.3162850237807,
133.527820467193)) ;
#118804=CARTESIAN_POINT('Ctrl Pts',(-15.0100411334749,14.4106899925297,
133.283664989385)) ;
#118805=CARTESIAN_POINT('Ctrl Pts',(-14.9326148210013,14.4339585114454,
133.024280536039)) ;
#118806=CARTESIAN_POINT('Ctrl Pts',(-14.8568708594425,14.3853107611265,
132.770062353486)) ;
#118807=CARTESIAN_POINT('Ctrl Pts',(-14.7876649938724,14.2669554182004,
132.53459909594)) ;
#118808=CARTESIAN_POINT('Ctrl Pts',(-14.7318719578663,14.0883945818005,
132.338499578768)) ;
#118809=CARTESIAN_POINT('Ctrl Pts',(-14.6938089527837,13.8631867563802,
132.194300139215)) ;
#118810=CARTESIAN_POINT('Ctrl Pts',(-14.6767096598151,13.6057120624757,
132.111223574541)) ;
#118811=CARTESIAN_POINT('Ctrl Pts',(-14.6827242929546,13.3350528446723,
132.09566169205)) ;
#118812=CARTESIAN_POINT('Ctrl Pts',(-14.7121680274684,13.0707553542234,
132.148540753936)) ;
#118813=CARTESIAN_POINT('Ctrl Pts',(-14.7634230355336,12.8321486706852,
132.265220829999)) ;
#118814=CARTESIAN_POINT('Ctrl Pts',(-14.8343243445453,12.634462986152,132.439029242949)) ;
#118815=CARTESIAN_POINT('Ctrl Pts',(-14.9190987032166,12.4951761871636,
132.653736170643)) ;
#118816=CARTESIAN_POINT('Ctrl Pts',(-15.0137030553733,12.4210996152358,
132.896951658987)) ;
#118817=CARTESIAN_POINT('Ctrl Pts',(-15.1118584374447,12.4192964203799,
133.150469827584)) ;
#118818=CARTESIAN_POINT('Ctrl Pts',(-15.2065423898953,12.4890492296412,
133.394023625246)) ;
#118819=CARTESIAN_POINT('Ctrl Pts',(-15.2928092091889,12.6268326997912,
133.612729453774)) ;
#118820=CARTESIAN_POINT('Ctrl Pts',(-15.36366888592,12.8195830933143,133.786835531785)) ;
#118821=CARTESIAN_POINT('Ctrl Pts',(-15.4163669219874,13.0571002340723,
133.90758683916)) ;
#118822=CARTESIAN_POINT('Ctrl Pts',(-15.4469778815777,13.3202805814274,
133.963914687961)) ;
#118823=CARTESIAN_POINT('Ctrl Pts',(-15.4543026229993,13.5914916661993,
133.95212933086)) ;
#118824=CARTESIAN_POINT('Ctrl Pts',(-15.4383344177632,13.850556640903,133.87230135427)) ;
#118825=CARTESIAN_POINT('Ctrl Pts',(-15.4012847002577,14.0777829295082,
133.731064838827)) ;
#118826=CARTESIAN_POINT('Ctrl Pts',(-15.3462911182543,14.2590886329476,
133.53730079744)) ;
#118827=CARTESIAN_POINT('Ctrl Pts',(-15.2777940762264,14.3807166913486,
133.303980899783)) ;
#118828=CARTESIAN_POINT('Ctrl Pts',(-15.2018903534353,14.433343612586,133.049127000921)) ;
#118829=CARTESIAN_POINT('Ctrl Pts',(-15.1243517133712,14.4133893592863,
132.789404894538)) ;
#118830=CARTESIAN_POINT('Ctrl Pts',(-15.0521554583449,14.3229978195751,
132.545518463658)) ;
#118831=CARTESIAN_POINT('Ctrl Pts',(-14.9903443446377,14.1680350137977,
132.331824025693)) ;
#118832=CARTESIAN_POINT('Ctrl Pts',(-14.9444490968226,13.9594347962821,
132.164606047946)) ;
#118833=CARTESIAN_POINT('Ctrl Pts',(-14.9184638689497,13.7128291828127,
132.055602750817)) ;
#118834=CARTESIAN_POINT('Ctrl Pts',(-14.9150513396177,13.4442543360426,
132.012387191979)) ;
#118835=CARTESIAN_POINT('Ctrl Pts',(-14.934907349885,13.1766944104108,132.037471123533)) ;
#118836=CARTESIAN_POINT('Ctrl Pts',(-14.9779705778938,12.9234094695572,
132.129904425091)) ;
#118837=CARTESIAN_POINT('Ctrl Pts',(-15.0410826203302,12.7086523153548,
132.281257042121)) ;
#118838=CARTESIAN_POINT('Ctrl Pts',(-15.12058795907,12.5444332786266,132.480500688696)) ;
#118839=CARTESIAN_POINT('Ctrl Pts',(-15.2126050466934,12.4422654276919,
132.715988199535)) ;
#118840=CARTESIAN_POINT('Ctrl Pts',(-15.3096570151281,12.4113238218205,
132.966463261144)) ;
#118841=CARTESIAN_POINT('Ctrl Pts',(-15.4063598506817,12.4521999821779,
133.215890712785)) ;
#118842=CARTESIAN_POINT('Ctrl Pts',(-15.4969844701974,12.5635389919688,
133.447348690198)) ;
#118843=CARTESIAN_POINT('Ctrl Pts',(-15.5745083193793,12.7354102649258,
133.64080974434)) ;
#118844=CARTESIAN_POINT('Ctrl Pts',(-15.6351282259747,12.9568498172893,
133.784780387148)) ;
#118845=CARTESIAN_POINT('Ctrl Pts',(-15.674914220919,13.2117694586679,133.867887052705)) ;
#118846=CARTESIAN_POINT('Ctrl Pts',(-15.6917614023731,13.4825284922973,
133.883897484168)) ;
#118847=CARTESIAN_POINT('Ctrl Pts',(-15.6850400020228,13.7484828909248,
133.83112168251)) ;
#118848=CARTESIAN_POINT('Ctrl Pts',(-15.6562837813056,13.9900671084782,
133.714129468702)) ;
#118849=CARTESIAN_POINT('Ctrl Pts',(-15.6080310880803,14.1922209027102,
133.540043875935)) ;
#118850=CARTESIAN_POINT('Ctrl Pts',(-15.5443158917429,14.3393855403521,
133.320716383079)) ;
#118851=CARTESIAN_POINT('Ctrl Pts',(-15.4709624560433,14.4204077329138,
133.07339142867)) ;
#118852=CARTESIAN_POINT('Ctrl Pts',(-15.3934209892206,14.4304302154213,
132.813738162468)) ;
#118853=CARTESIAN_POINT('Ctrl Pts',(-15.3179864333146,14.367871152587,132.56015597024)) ;
#118854=CARTESIAN_POINT('Ctrl Pts',(-15.2511809644484,14.2376927603017,
132.331870254085)) ;
#118855=CARTESIAN_POINT('Ctrl Pts',(-15.1983120540608,14.0489883287211,
132.144273980636)) ;
#118856=CARTESIAN_POINT('Ctrl Pts',(-15.1639748285967,13.8164456424353,
132.0109487585)) ;
#118857=CARTESIAN_POINT('Ctrl Pts',(-15.1511681352343,13.5541089152985,
131.940298370315)) ;
#118858=CARTESIAN_POINT('Ctrl Pts',(-15.1615961610843,13.2846772722545,
131.937816936968)) ;
#118859=CARTESIAN_POINT('Ctrl Pts',(-15.1953535583714,13.0230235410346,
132.003215202363)) ;
#118860=CARTESIAN_POINT('Ctrl Pts',(-15.2506577077313,12.790872732509,132.13166089081)) ;
#118861=CARTESIAN_POINT('Ctrl Pts',(-15.3242924340642,12.603871831162,132.313637073672)) ;
#118862=CARTESIAN_POINT('Ctrl Pts',(-15.4117066977416,12.4755978216217,
132.535874664851)) ;
#118863=CARTESIAN_POINT('Ctrl Pts',(-15.5074337996065,12.4151865443115,
132.782375206903)) ;
#118864=CARTESIAN_POINT('Ctrl Pts',(-15.6051136198306,12.4270410572104,
133.034636072369)) ;
#118865=CARTESIAN_POINT('Ctrl Pts',(-15.6986186350994,12.5098502555296,
133.274722192349)) ;
#118866=CARTESIAN_POINT('Ctrl Pts',(-15.7824419706046,12.6589866002263,
133.486340286416)) ;
#118867=CARTESIAN_POINT('Ctrl Pts',(-15.8502870980143,12.8615686944882,
133.65153604425)) ;
#118868=CARTESIAN_POINT('Ctrl Pts',(-15.8989700371052,13.1050266274507,
133.760615654876)) ;
#118869=CARTESIAN_POINT('Ctrl Pts',(-15.925294229189,13.3718443687466,133.804320981034)) ;
#118870=CARTESIAN_POINT('Ctrl Pts',(-15.9281777645095,13.6411904118671,
133.779698959797)) ;
#118871=CARTESIAN_POINT('Ctrl Pts',(-15.9079356090688,13.8968634944342,
133.687249703864)) ;
#118872=CARTESIAN_POINT('Ctrl Pts',(-15.8672784194845,14.1159779670334,
133.535543259696)) ;
#118873=CARTESIAN_POINT('Ctrl Pts',(-15.8091810365908,14.287325697854,133.332598922334)) ;
#118874=CARTESIAN_POINT('Ctrl Pts',(-15.7390992509777,14.3958947367542,
133.094806970649)) ;
#118875=CARTESIAN_POINT('Ctrl Pts',(-15.6624784834203,14.4351265100489,
132.837862938543)) ;
#118876=CARTESIAN_POINT('Ctrl Pts',(-15.5856066307678,14.401957868372,132.580198882921)) ;
#118877=CARTESIAN_POINT('Ctrl Pts',(-15.5145051235158,14.2982652104899,
132.339286619073)) ;
#118878=CARTESIAN_POINT('Ctrl Pts',(-15.4554958556116,14.132480207139,132.133854824434)) ;
#118879=CARTESIAN_POINT('Ctrl Pts',(-15.4130454905872,13.915462827869,131.976696127531)) ;
#118880=CARTESIAN_POINT('Ctrl Pts',(-15.3911774530101,13.6633712465324,
131.879702342287)) ;
#118881=CARTESIAN_POINT('Ctrl Pts',(-15.3920733735863,13.3940849462189,
131.849205339726)) ;
#118882=CARTESIAN_POINT('Ctrl Pts',(-15.4165204372103,13.1263052775463,
131.887435828916)) ;
#118883=CARTESIAN_POINT('Ctrl Pts',(-15.4633817742367,12.8804158751522,
131.991219989087)) ;
#118884=CARTESIAN_POINT('Ctrl Pts',(-15.5300065791661,12.6733662983206,
132.152744232175)) ;
#118885=CARTESIAN_POINT('Ctrl Pts',(-15.6125439232497,12.5197379232373,
132.360696324844)) ;
#118886=CARTESIAN_POINT('Ctrl Pts',(-15.705635796009,12.4310982173194,132.599503551761)) ;
#118887=CARTESIAN_POINT('Ctrl Pts',(-15.803074203752,12.4134628281618,132.851106820896)) ;
#118888=CARTESIAN_POINT('Ctrl Pts',(-15.8992731570117,12.4679867371616,
133.098968131885)) ;
#118889=CARTESIAN_POINT('Ctrl Pts',(-15.9878233128369,12.5916525516401,
133.324414662735)) ;
#118890=CARTESIAN_POINT('Ctrl Pts',(-16.062379654878,12.7734684549556,133.509251293565)) ;
#118891=CARTESIAN_POINT('Ctrl Pts',(-16.1194191301887,13.0028688411228,
133.642704445147)) ;
#118892=CARTESIAN_POINT('Ctrl Pts',(-16.1549941311676,13.2619624535534,
133.71352787575)) ;
#118893=CARTESIAN_POINT('Ctrl Pts',(-16.1673733877208,13.5340192322936,
133.716408021107)) ;
#118894=CARTESIAN_POINT('Ctrl Pts',(-16.1564239082465,13.7955675293532,
133.651469162884)) ;
#118895=CARTESIAN_POINT('Ctrl Pts',(-16.1236090883118,14.0322613707932,
133.522420407032)) ;
#118896=CARTESIAN_POINT('Ctrl Pts',(-16.0721689251693,14.224389834904,133.339099208771)) ;
#118897=CARTESIAN_POINT('Ctrl Pts',(-16.0063006341945,14.3598901194567,
133.113539220079)) ;
#118898=CARTESIAN_POINT('Ctrl Pts',(-15.9311391339714,14.4280176273918,
132.860679199975)) ;
#118899=CARTESIAN_POINT('Ctrl Pts',(-15.8540954386379,14.4241023725172,
132.602718351768)) ;
#118900=CARTESIAN_POINT('Ctrl Pts',(-15.7795834996639,14.3482280088461,
132.35173937791)) ;
#118901=CARTESIAN_POINT('Ctrl Pts',(-15.7150929997006,14.2060724290961,
132.130239203412)) ;
#118902=CARTESIAN_POINT('Ctrl Pts',(-15.6655571468787,14.0086808494732,
131.952512147199)) ;
#118903=CARTESIAN_POINT('Ctrl Pts',(-15.6349604163456,13.7691471639152,
131.830048736311)) ;
#118904=CARTESIAN_POINT('Ctrl Pts',(-15.6264276111756,13.5031160987729,
131.771831492658)) ;
#118905=CARTESIAN_POINT('Ctrl Pts',(-15.6414545015548,13.2327334020777,
131.782614786388)) ;
#118906=CARTESIAN_POINT('Ctrl Pts',(-15.6793081117188,12.9767766707072,
131.86018699996)) ;
#118907=CARTESIAN_POINT('Ctrl Pts',(-15.7383109254035,12.7518157375075,
131.999428531665)) ;
#118908=CARTESIAN_POINT('Ctrl Pts',(-15.8149740258483,12.5749030577416,
132.190234860575)) ;
#118909=CARTESIAN_POINT('Ctrl Pts',(-15.9043928505203,12.458725868686,132.418325067201)) ;
#118910=CARTESIAN_POINT('Ctrl Pts',(-16.0013623248274,12.4118884071783,
132.668331705155)) ;
#118911=CARTESIAN_POINT('Ctrl Pts',(-16.0980803345127,12.4371447951342,
132.918012708935)) ;
#118912=CARTESIAN_POINT('Ctrl Pts',(-16.1907253077105,12.5335140178268,
133.155361461328)) ;
#118913=CARTESIAN_POINT('Ctrl Pts',(-16.2714678242786,12.6929505633227,
133.358205410288)) ;
#118914=CARTESIAN_POINT('Ctrl Pts',(-16.3363258449632,12.9053983623053,
133.514481626618)) ;
#118915=CARTESIAN_POINT('Ctrl Pts',(-16.3807666053811,13.1539498796381,
133.611267752896)) ;
#118916=CARTESIAN_POINT('Ctrl Pts',(-16.4027454324204,13.4226750818637,
133.642307124475)) ;
#118917=CARTESIAN_POINT('Ctrl Pts',(-16.401215059512,13.6910891460654,133.604723727658)) ;
#118918=CARTESIAN_POINT('Ctrl Pts',(-16.3768570956532,13.9413684453662,
133.500295149174)) ;
#118919=CARTESIAN_POINT('Ctrl Pts',(-16.332568989847,14.1526799208371,133.337911715767)) ;
#118920=CARTESIAN_POINT('Ctrl Pts',(-16.2719528045487,14.3125333416555,
133.127724038229)) ;
#118921=CARTESIAN_POINT('Ctrl Pts',(-16.2002008694076,14.4088194589569,
132.885039982371)) ;
#118922=CARTESIAN_POINT('Ctrl Pts',(-16.1225573895585,14.4343198918705,
132.624898644505)) ;
#118923=CARTESIAN_POINT('Ctrl Pts',(-16.0468359703471,14.3877722127897,
132.370812047708)) ;
#118924=CARTESIAN_POINT('Ctrl Pts',(-15.9772633495729,14.2711471004472,
132.134233982621)) ;
#118925=CARTESIAN_POINT('Ctrl Pts',(-15.9212635671219,14.0951742684999,
131.937696121308)) ;
#118926=CARTESIAN_POINT('Ctrl Pts',(-15.8823816388333,13.870335354891,131.790959834028)) ;
#118927=CARTESIAN_POINT('Ctrl Pts',(-15.8646619711302,13.612835927565,131.705995937797)) ;
#118928=CARTESIAN_POINT('Ctrl Pts',(-15.8700234600786,13.3431053086278,
131.688622613142)) ;
#118929=CARTESIAN_POINT('Ctrl Pts',(-15.8986797747435,13.0784069754049,
131.739222629538)) ;
#118930=CARTESIAN_POINT('Ctrl Pts',(-15.9498454347427,12.8371325485697,
131.85537890921)) ;
#118931=CARTESIAN_POINT('Ctrl Pts',(-16.019632479177,12.6399915744991,132.026248377193)) ;
#118932=CARTESIAN_POINT('Ctrl Pts',(-16.1044500214334,12.4979352646964,
132.240903934042)) ;
#118933=CARTESIAN_POINT('Ctrl Pts',(-16.1991059233172,12.4220838603556,
132.484204340769)) ;
#118934=CARTESIAN_POINT('Ctrl Pts',(-16.297051164384,12.4184701300548,132.737175673238)) ;
#118935=CARTESIAN_POINT('Ctrl Pts',(-16.3915722814502,12.4860424705287,
132.980365390677)) ;
#118936=CARTESIAN_POINT('Ctrl Pts',(-16.4779684262832,12.6212970350437,
133.199551922946)) ;
#118937=CARTESIAN_POINT('Ctrl Pts',(-16.5497122738182,12.8133839848722,
133.376079170821)) ;
#118938=CARTESIAN_POINT('Ctrl Pts',(-16.6030126812763,13.050364922785,133.498541178369)) ;
#118939=CARTESIAN_POINT('Ctrl Pts',(-16.6341711807537,13.3123037538977,
133.556563217302)) ;
#118940=CARTESIAN_POINT('Ctrl Pts',(-16.6422066343876,13.5832778951352,
133.546888412643)) ;
#118941=CARTESIAN_POINT('Ctrl Pts',(-16.6269632342962,13.8428843681781,
133.469196841622)) ;
#118942=CARTESIAN_POINT('Ctrl Pts',(-16.5903845709853,14.0720013140808,
133.329230796997)) ;
#118943=CARTESIAN_POINT('Ctrl Pts',(-16.5358497973119,14.2546155515289,
133.136829051385)) ;
#118944=CARTESIAN_POINT('Ctrl Pts',(-16.4678538223331,14.3779471461467,
132.905056863993)) ;
#118945=CARTESIAN_POINT('Ctrl Pts',(-16.3919879568045,14.4327785489293,
132.650265716705)) ;
#118946=CARTESIAN_POINT('Ctrl Pts',(-16.3146543287815,14.4152048482771,
132.391254909722)) ;
#118947=CARTESIAN_POINT('Ctrl Pts',(-16.2418798056375,14.3266409658442,
132.145530624094)) ;
#118948=CARTESIAN_POINT('Ctrl Pts',(-16.1796064540115,14.1729214945641,
131.930425537284)) ;
#118949=CARTESIAN_POINT('Ctrl Pts',(-16.1333430675989,13.9662155459552,
131.762226115951)) ;
#118950=CARTESIAN_POINT('Ctrl Pts',(-16.1067216716661,13.7208186783693,
131.65139858059)) ;
#118951=CARTESIAN_POINT('Ctrl Pts',(-16.1025777094809,13.4521886748155,
131.60599836467)) ;
#118952=CARTESIAN_POINT('Ctrl Pts',(-16.1218683713234,13.1838897462868,
131.629362282739)) ;
#118953=CARTESIAN_POINT('Ctrl Pts',(-16.1639997121743,12.9313138678917,
131.719275378533)) ;
#118954=CARTESIAN_POINT('Ctrl Pts',(-16.2267282009721,12.7142071157524,
131.869374219865)) ;
#118955=CARTESIAN_POINT('Ctrl Pts',(-16.3060391253692,12.5481822862925,
132.067981312188)) ;
#118956=CARTESIAN_POINT('Ctrl Pts',(-16.3972766323407,12.4445945495957,
132.301375289978)) ;
#118957=CARTESIAN_POINT('Ctrl Pts',(-16.4943286218477,12.4110615292549,
132.551818241413)) ;
#118958=CARTESIAN_POINT('Ctrl Pts',(-16.5915886358839,12.4502003410622,
132.802714054145)) ;
#118959=CARTESIAN_POINT('Ctrl Pts',(-16.6818663882812,12.5587981584367,
133.033390094002)) ;
#118960=CARTESIAN_POINT('Ctrl Pts',(-16.7601403001768,12.7290992999271,
133.228951738304)) ;
#118961=CARTESIAN_POINT('Ctrl Pts',(-16.8215906092358,12.9505642966122,
133.375178942379)) ;
#118962=CARTESIAN_POINT('Ctrl Pts',(-16.8618118836172,13.2039533885785,
133.459671754367)) ;
#118963=CARTESIAN_POINT('Ctrl Pts',(-16.8793709151704,13.4737768400672,
133.477849805927)) ;
#118964=CARTESIAN_POINT('Ctrl Pts',(-16.8733999316165,13.7408243528461,
133.42719068513)) ;
#118965=CARTESIAN_POINT('Ctrl Pts',(-16.8450419521337,13.9843828533781,
133.311202487825)) ;
#118966=CARTESIAN_POINT('Ctrl Pts',(-16.7975164472383,14.1867700455966,
133.139416973208)) ;
#118967=CARTESIAN_POINT('Ctrl Pts',(-16.7341358946275,14.3360223311849,
132.921026026179)) ;
#118968=CARTESIAN_POINT('Ctrl Pts',(-16.660977465977,14.4190304968155,132.674270725282)) ;
#118969=CARTESIAN_POINT('Ctrl Pts',(-16.5834773099444,14.4311357374112,
132.414740139683)) ;
#118970=CARTESIAN_POINT('Ctrl Pts',(-16.5080024369756,14.3708887924222,
132.161099658697)) ;
#118971=CARTESIAN_POINT('Ctrl Pts',(-16.4407492412971,14.2422926877059,
131.931437078686)) ;
#118972=CARTESIAN_POINT('Ctrl Pts',(-16.3876054278893,14.0562619383273,
131.743209531702)) ;
#118973=CARTESIAN_POINT('Ctrl Pts',(-16.3523922274863,13.8231736969123,
131.607079126901)) ;
#118974=CARTESIAN_POINT('Ctrl Pts',(-16.3390157650434,13.5622216724448,
131.534881089191)) ;
#118975=CARTESIAN_POINT('Ctrl Pts',(-16.3487619639683,13.2923510388066,
131.530347534574)) ;
#118976=CARTESIAN_POINT('Ctrl Pts',(-16.3817521250503,13.0307856163929,
131.593593437063)) ;
#118977=CARTESIAN_POINT('Ctrl Pts',(-16.4366407076592,12.7967159031727,
131.720707541001)) ;
#118978=CARTESIAN_POINT('Ctrl Pts',(-16.5097876602422,12.6083942654361,
131.901281935499)) ;
#118979=CARTESIAN_POINT('Ctrl Pts',(-16.5969702538156,12.4782667075604,
132.122811514274)) ;
#118980=CARTESIAN_POINT('Ctrl Pts',(-16.6922267232362,12.4160107642981,
132.368047019534)) ;
#118981=CARTESIAN_POINT('Ctrl Pts',(-16.7901867754655,12.425588916255,132.621043045965)) ;
#118982=CARTESIAN_POINT('Ctrl Pts',(-16.8842341319186,12.5070743322311,
132.862581766032)) ;
#118983=CARTESIAN_POINT('Ctrl Pts',(-16.967977842745,12.6538727730597,133.074133355427)) ;
#118984=CARTESIAN_POINT('Ctrl Pts',(-17.0364591546495,12.8553499552797,
133.241130447034)) ;
#118985=CARTESIAN_POINT('Ctrl Pts',(-17.0857411108294,13.098103384175,133.351941598924)) ;
#118986=CARTESIAN_POINT('Ctrl Pts',(-17.1126981511373,13.3649638276871,
133.397446396314)) ;
#118987=CARTESIAN_POINT('Ctrl Pts',(-17.116159442986,13.6334094300958,133.374637115501)) ;
#118988=CARTESIAN_POINT('Ctrl Pts',(-17.0967738382637,13.8886868396263,
133.284851993961)) ;
#118989=CARTESIAN_POINT('Ctrl Pts',(-17.056493649699,14.1104518310445,133.134051885151)) ;
#118990=CARTESIAN_POINT('Ctrl Pts',(-16.9988013317732,14.2832226261628,
132.932301353712)) ;
#118991=CARTESIAN_POINT('Ctrl Pts',(-16.9290378227814,14.3937886224781,
132.69545277715)) ;
#118992=CARTESIAN_POINT('Ctrl Pts',(-16.8521634203114,14.4350213815805,
132.437618360093)) ;
#118993=CARTESIAN_POINT('Ctrl Pts',(-16.7755820965094,14.4038716563582,
132.180961179455)) ;
#118994=CARTESIAN_POINT('Ctrl Pts',(-16.7041025877262,14.302057440806,131.938891583268)) ;
#118995=CARTESIAN_POINT('Ctrl Pts',(-16.6447062661467,14.1377082691097,
131.732320566612)) ;
#118996=CARTESIAN_POINT('Ctrl Pts',(-16.6018098618319,13.9225120820519,
131.573940678987)) ;
#118997=CARTESIAN_POINT('Ctrl Pts',(-16.5792495458964,13.6705375102117,
131.474838163571)) ;
#118998=CARTESIAN_POINT('Ctrl Pts',(-16.5795380154602,13.401884525291,131.442617582448)) ;
#118999=CARTESIAN_POINT('Ctrl Pts',(-16.6031684812186,13.1344381659713,
131.478552161521)) ;
#119000=CARTESIAN_POINT('Ctrl Pts',(-16.6496627637314,12.8864833048174,
131.581096733802)) ;
#119001=CARTESIAN_POINT('Ctrl Pts',(-16.7154366448062,12.6791960280418,
131.740309941251)) ;
#119002=CARTESIAN_POINT('Ctrl Pts',(-16.7976993700621,12.5233811391943,
131.947393602466)) ;
#119003=CARTESIAN_POINT('Ctrl Pts',(-16.8904385311137,12.4327816584244,
132.185216053626)) ;
#119004=CARTESIAN_POINT('Ctrl Pts',(-16.9881341422106,12.4129159573699,
132.437466061827)) ;
#119005=CARTESIAN_POINT('Ctrl Pts',(-17.0843482146644,12.4655032796393,
132.685408560699)) ;
#119006=CARTESIAN_POINT('Ctrl Pts',(-17.172922450877,12.5866529362795,132.911042601542)) ;
#119007=CARTESIAN_POINT('Ctrl Pts',(-17.2482855222662,12.7674395708452,
133.098107251199)) ;
#119008=CARTESIAN_POINT('Ctrl Pts',(-17.3060249584729,12.9966807390071,
133.233489769117)) ;
#119009=CARTESIAN_POINT('Ctrl Pts',(-17.3420090323852,13.2541241840609,
133.305647431334)) ;
#119010=CARTESIAN_POINT('Ctrl Pts',(-17.3551351495104,13.5248421394856,
133.310863716187)) ;
#119011=CARTESIAN_POINT('Ctrl Pts',(-17.3448759274726,13.7882271369091,
133.247779942829)) ;
#119012=CARTESIAN_POINT('Ctrl Pts',(-17.3126076355024,14.0260983655197,
133.120304445274)) ;
#119013=CARTESIAN_POINT('Ctrl Pts',(-17.2615228620159,14.2200231919602,
132.93795360189)) ;
#119014=CARTESIAN_POINT('Ctrl Pts',(-17.1961003041983,14.356772234067,132.713767919682)) ;
#119015=CARTESIAN_POINT('Ctrl Pts',(-17.1215711456038,14.4269174457709,
132.462945997468)) ;
#119016=CARTESIAN_POINT('Ctrl Pts',(-17.0439259643199,14.4252572954794,
132.202973398023)) ;
#119017=CARTESIAN_POINT('Ctrl Pts',(-16.9694410843738,14.3512844735739,
131.952159419064)) ;
#119018=CARTESIAN_POINT('Ctrl Pts',(-16.9048069433037,14.2117350246389,
131.730367344063)) ;
#119019=CARTESIAN_POINT('Ctrl Pts',(-16.8545042052513,14.0152548216542,
131.550277704192)) ;
#119020=CARTESIAN_POINT('Ctrl Pts',(-16.8232933924181,13.7756399540023,
131.425894257679)) ;
#119021=CARTESIAN_POINT('Ctrl Pts',(-16.8141517807368,13.5122935142519,
131.366177190341)) ;
#119022=CARTESIAN_POINT('Ctrl Pts',(-16.8283845644128,13.241130032097,131.374556127916)) ;
#119023=CARTESIAN_POINT('Ctrl Pts',(-16.8656342224088,12.9839533345939,
131.450303268931)) ;
#119024=CARTESIAN_POINT('Ctrl Pts',(-16.9243039312876,12.7572239976212,
131.58846397778)) ;
#119025=CARTESIAN_POINT('Ctrl Pts',(-17.0002008430187,12.5794741431288,
131.777175573092)) ;
#119026=CARTESIAN_POINT('Ctrl Pts',(-17.089545033272,12.4611210765961,132.004960114565)) ;
#119027=CARTESIAN_POINT('Ctrl Pts',(-17.1858832231545,12.4122668265322,
132.253299215749)) ;
#119028=CARTESIAN_POINT('Ctrl Pts',(-17.2833704558394,12.4354395083141,
132.504985546955)) ;
#119029=CARTESIAN_POINT('Ctrl Pts',(-17.3761905784988,12.5301694803305,
132.742858721776)) ;
#119030=CARTESIAN_POINT('Ctrl Pts',(-17.4571309233802,12.6876686572945,
132.946346983697)) ;
#119031=CARTESIAN_POINT('Ctrl Pts',(-17.5224238027242,12.8982124580512,
133.103970186522)) ;
#119032=CARTESIAN_POINT('Ctrl Pts',(-17.5677102283566,13.1472879194742,
133.203047904097)) ;
#119033=CARTESIAN_POINT('Ctrl Pts',(-17.5902201631136,13.4151706318018,
133.23571624353)) ;
#119034=CARTESIAN_POINT('Ctrl Pts',(-17.5893444385462,13.6833052731468,
133.200104234833)) ;
#119035=CARTESIAN_POINT('Ctrl Pts',(-17.5658297900368,13.9335262194554,
133.098280889353)) ;
#119036=CARTESIAN_POINT('Ctrl Pts',(-17.5217189486775,14.1479664880633,
132.936132518446)) ;
#119037=CARTESIAN_POINT('Ctrl Pts',(-17.4616218712877,14.3087959168501,
132.727565237457)) ;
#119038=CARTESIAN_POINT('Ctrl Pts',(-17.3901260006563,14.4069520231813,
132.485627776412)) ;
#119039=CARTESIAN_POINT('Ctrl Pts',(-17.3129141442959,14.4347039370495,
132.226908077612)) ;
#119040=CARTESIAN_POINT('Ctrl Pts',(-17.2365534068234,14.3899170768859,
131.970719496114)) ;
#119041=CARTESIAN_POINT('Ctrl Pts',(-17.1671213847056,14.2758481834518,
131.734760655287)) ;
#119042=CARTESIAN_POINT('Ctrl Pts',(-17.110414539759,14.1010294405417,131.536029917471)) ;
#119043=CARTESIAN_POINT('Ctrl Pts',(-17.070996065358,13.8772034323747,131.3877191098)) ;
#119044=CARTESIAN_POINT('Ctrl Pts',(-17.0526485411338,13.6206147260663,
131.300948159971)) ;
#119045=CARTESIAN_POINT('Ctrl Pts',(-17.0573044621097,13.3509221462812,
131.281506125412)) ;
#119046=CARTESIAN_POINT('Ctrl Pts',(-17.0854100559566,13.0853829020601,
131.330437718243)) ;
#119047=CARTESIAN_POINT('Ctrl Pts',(-17.1356188030015,12.8445476179022,
131.444003647915)) ;
#119048=CARTESIAN_POINT('Ctrl Pts',(-17.2051252209905,12.6449528736105,
131.613913841807)) ;
#119049=CARTESIAN_POINT('Ctrl Pts',(-17.2895913546192,12.501260652652,131.827552263625)) ;
#119050=CARTESIAN_POINT('Ctrl Pts',(-17.3837152874089,12.423505657414,132.069408473703)) ;
#119051=CARTESIAN_POINT('Ctrl Pts',(-17.4816812872353,12.4173186176401,
132.32243184758)) ;
#119052=CARTESIAN_POINT('Ctrl Pts',(-17.576953937296,12.4833714818954,132.56760944195)) ;
#119053=CARTESIAN_POINT('Ctrl Pts',(-17.6632658867121,12.6162285773946,
132.786710307845)) ;
#119054=CARTESIAN_POINT('Ctrl Pts',(-17.7357544770908,12.8073410485065,
132.965304035698)) ;
#119055=CARTESIAN_POINT('Ctrl Pts',(-17.7895701941442,13.0432165498209,
133.089294730388)) ;
#119056=CARTESIAN_POINT('Ctrl Pts',(-17.8214064088599,13.3046949553566,
133.149287622234)) ;
#119057=CARTESIAN_POINT('Ctrl Pts',(-17.8300953365612,13.5764463640802,
133.141433903753)) ;
#119058=CARTESIAN_POINT('Ctrl Pts',(-17.8154038505538,13.8363550328947,
133.065377997914)) ;
#119059=CARTESIAN_POINT('Ctrl Pts',(-17.7795672536449,14.0655921907836,
132.927723437825)) ;
#119060=CARTESIAN_POINT('Ctrl Pts',(-17.725370419326,14.2503954340108,132.736213361284)) ;
#119061=CARTESIAN_POINT('Ctrl Pts',(-17.6574361327673,14.3757154030236,
132.504523320352)) ;
#119062=CARTESIAN_POINT('Ctrl Pts',(-17.5818347558726,14.4321659912553,
132.250567240917)) ;
#119063=CARTESIAN_POINT('Ctrl Pts',(-17.5047135094807,14.4167343012476,
131.992284390174)) ;
#119064=CARTESIAN_POINT('Ctrl Pts',(-17.4317377190015,14.3302899803119,
131.745982280086)) ;
#119065=CARTESIAN_POINT('Ctrl Pts',(-17.3690184396363,14.1784243472653,
131.529566298611)) ;
#119066=CARTESIAN_POINT('Ctrl Pts',(-17.3220256941153,13.9717507603948,
131.3590462137)) ;
#119067=CARTESIAN_POINT('Ctrl Pts',(-17.2950308109835,13.7284356730931,
131.247306408457)) ;
#119068=CARTESIAN_POINT('Ctrl Pts',(-17.2901004199583,13.4606301780327,
131.199659999263)) ;
#119069=CARTESIAN_POINT('Ctrl Pts',(-17.3088808530583,13.1906192009326,
131.221345418955)) ;
#119070=CARTESIAN_POINT('Ctrl Pts',(-17.3501438419449,12.9388679840775,
131.30892757268)) ;
#119071=CARTESIAN_POINT('Ctrl Pts',(-17.4124956771912,12.7195132163599,
131.457797705406)) ;
#119072=CARTESIAN_POINT('Ctrl Pts',(-17.4915919365344,12.5518557369755,
131.655723289798)) ;
#119073=CARTESIAN_POINT('Ctrl Pts',(-17.582138027078,12.4467157573859,131.88725129519)) ;
#119074=CARTESIAN_POINT('Ctrl Pts',(-17.6796558499135,12.4110145774445,
132.138864732051)) ;
#119075=CARTESIAN_POINT('Ctrl Pts',(-17.7763443868199,12.4479828345384,
132.388317475769)) ;
#119076=CARTESIAN_POINT('Ctrl Pts',(-17.8671272399962,12.5544308128886,
132.620405505491)) ;
#119077=CARTESIAN_POINT('Ctrl Pts',(-17.9462888315339,12.7245572177545,
132.818333491493)) ;
#119078=CARTESIAN_POINT('Ctrl Pts',(-18.0078236151475,12.9435039918997,
132.965026246654)) ;
#119079=CARTESIAN_POINT('Ctrl Pts',(-18.0487895704932,13.1965754394182,
133.051630649739)) ;
#119080=CARTESIAN_POINT('Ctrl Pts',(-18.0669610596337,13.465805442607,133.071652747287)) ;
#119081=CARTESIAN_POINT('Ctrl Pts',(-18.0616988491559,13.7328709787398,
133.023106457066)) ;
#119082=CARTESIAN_POINT('Ctrl Pts',(-18.0340587835222,13.9772572958127,
132.909247166554)) ;
#119083=CARTESIAN_POINT('Ctrl Pts',(-17.9868053084932,14.1820529249742,
132.738087238278)) ;
#119084=CARTESIAN_POINT('Ctrl Pts',(-17.9237844975308,14.3328843736513,
132.520761239238)) ;
#119085=CARTESIAN_POINT('Ctrl Pts',(-17.8505988882096,14.417801109475,132.273827837852)) ;
#119086=CARTESIAN_POINT('Ctrl Pts',(-17.773511642618,14.4318123913692,132.0156729237)) ;
#119087=CARTESIAN_POINT('Ctrl Pts',(-17.6975797543095,14.373230288219,131.760550888382)) ;
#119088=CARTESIAN_POINT('Ctrl Pts',(-17.6303724161098,14.2469703146016,
131.531194194324)) ;
#119089=CARTESIAN_POINT('Ctrl Pts',(-17.5766337968563,14.062146501963,131.34115695912)) ;
#119090=CARTESIAN_POINT('Ctrl Pts',(-17.5409369598325,13.8305007160398,
131.203674990885)) ;
#119091=CARTESIAN_POINT('Ctrl Pts',(-17.5268539340979,13.5704781299009,
131.129449867294)) ;
#119092=CARTESIAN_POINT('Ctrl Pts',(-17.5359636480712,13.299460638904,131.122917047577)) ;
#119093=CARTESIAN_POINT('Ctrl Pts',(-17.5683660353675,13.0377343274411,
131.184480969823)) ;
#119094=CARTESIAN_POINT('Ctrl Pts',(-17.6223484639304,12.8036245820339,
131.309107763163)) ;
#119095=CARTESIAN_POINT('Ctrl Pts',(-17.6952608243721,12.6130123285287,
131.488871588966)) ;
#119096=CARTESIAN_POINT('Ctrl Pts',(-17.7818766036407,12.4813447603753,
131.708836600993)) ;
#119097=CARTESIAN_POINT('Ctrl Pts',(-17.8773008779211,12.4167223842582,
131.954443952904)) ;
#119098=CARTESIAN_POINT('Ctrl Pts',(-17.9751477328863,12.42436559993,132.207155605855)) ;
#119099=CARTESIAN_POINT('Ctrl Pts',(-18.0691420106269,12.5034382891946,
132.448633030959)) ;
#119100=CARTESIAN_POINT('Ctrl Pts',(-18.1534115083128,12.6484426384731,
132.661676259449)) ;
#119101=CARTESIAN_POINT('Ctrl Pts',(-18.2225859165493,12.8490571867036,
132.83061106269)) ;
#119102=CARTESIAN_POINT('Ctrl Pts',(-18.2723758082232,13.0907449616811,
132.942931245798)) ;
#119103=CARTESIAN_POINT('Ctrl Pts',(-18.2999851225752,13.3559778335449,
132.990488268703)) ;
#119104=CARTESIAN_POINT('Ctrl Pts',(-18.3041736331466,13.626477299062,132.969568151916)) ;
#119105=CARTESIAN_POINT('Ctrl Pts',(-18.2854138148956,13.8815733654641,
132.881719274568)) ;
#119106=CARTESIAN_POINT('Ctrl Pts',(-18.2457410495779,14.1045282563564,
132.732700456118)) ;
#119107=CARTESIAN_POINT('Ctrl Pts',(-18.1885080075373,14.2789670451528,
132.532299622035)) ;
#119108=CARTESIAN_POINT('Ctrl Pts',(-18.1189348222045,14.3914951714323,
132.295964267991)) ;
#119109=CARTESIAN_POINT('Ctrl Pts',(-18.0424869550482,14.434860760417,132.039514831165)) ;
#119110=CARTESIAN_POINT('Ctrl Pts',(-17.965414998045,14.4056890526457,131.781241274387)) ;
#119111=CARTESIAN_POINT('Ctrl Pts',(-17.8940126216972,14.3062653162723,
131.539554730981)) ;
#119112=CARTESIAN_POINT('Ctrl Pts',(-17.8340450774883,14.1434405265247,
131.331242919008)) ;
#119113=CARTESIAN_POINT('Ctrl Pts',(-17.7905944856401,13.9296996110321,
131.171266220429)) ;
#119114=CARTESIAN_POINT('Ctrl Pts',(-17.7673324632912,13.6772902073351,
131.069954024796)) ;
#119115=CARTESIAN_POINT('Ctrl Pts',(-17.7669919620145,13.4099497148246,
131.036034152482)) ;
#119116=CARTESIAN_POINT('Ctrl Pts',(-17.7899679662138,13.1418739541198,
131.070013306978)) ;
#119117=CARTESIAN_POINT('Ctrl Pts',(-17.8356284031104,12.8939990849847,
131.170254631528)) ;
#119118=CARTESIAN_POINT('Ctrl Pts',(-17.9010078368496,12.6844791056233,
131.328208604738)) ;
#119119=CARTESIAN_POINT('Ctrl Pts',(-17.9833156417732,12.5265062757821,
131.535272013609)) ;
#119120=CARTESIAN_POINT('Ctrl Pts',(-18.0753610768667,12.4345049912951,
131.771240370348)) ;
#119121=CARTESIAN_POINT('Ctrl Pts',(-18.1733168029141,12.4124896110262,
132.024140560041)) ;
#119122=CARTESIAN_POINT('Ctrl Pts',(-18.2692512178841,12.4629154938197,
132.271405332479)) ;
#119123=CARTESIAN_POINT('Ctrl Pts',(-18.3583177450786,12.582091252431,132.498425476056)) ;
#119124=CARTESIAN_POINT('Ctrl Pts',(-18.4343847870178,12.7624371771161,
132.687394350924)) ;
#119125=CARTESIAN_POINT('Ctrl Pts',(-18.4921191579233,12.9881392321824,
132.823106494344)) ;
#119126=CARTESIAN_POINT('Ctrl Pts',(-18.5291183635577,13.2462582998136,
132.898039284755)) ;
#119127=CARTESIAN_POINT('Ctrl Pts',(-18.5428634723026,13.5176871774874,
132.904973108306)) ;
#119128=CARTESIAN_POINT('Ctrl Pts',(-18.533282772069,13.7805944540118,132.843988452066)) ;
#119129=CARTESIAN_POINT('Ctrl Pts',(-18.5016568117638,14.0195269504541,
132.718389345958)) ;
#119130=CARTESIAN_POINT('Ctrl Pts',(-18.4510737818769,14.2150385228552,
132.537499304482)) ;
#119131=CARTESIAN_POINT('Ctrl Pts',(-18.3858483982378,14.3538332825844,
132.313815804307)) ;
#119132=CARTESIAN_POINT('Ctrl Pts',(-18.3115810381023,14.425964693576,132.063801363807)) ;
#119133=CARTESIAN_POINT('Ctrl Pts',(-18.2336471930446,14.4260802790596,
131.802854408235)) ;
#119134=CARTESIAN_POINT('Ctrl Pts',(-18.1596550168565,14.3549350609901,
131.553791750138)) ;
#119135=CARTESIAN_POINT('Ctrl Pts',(-18.0940802977715,14.2162529068252,
131.3289701238)) ;
#119136=CARTESIAN_POINT('Ctrl Pts',(-18.043497662721,14.0213156820109,131.148133926052)) ;
#119137=CARTESIAN_POINT('Ctrl Pts',(-18.0116896745285,13.7835942530776,
131.022110217814)) ;
#119138=CARTESIAN_POINT('Ctrl Pts',(-18.0018945840821,13.5186608640693,
130.96022838923)) ;
#119139=CARTESIAN_POINT('Ctrl Pts',(-18.015387995345,13.2494162372405,130.966701013763)) ;
#119140=CARTESIAN_POINT('Ctrl Pts',(-18.0521726814189,12.9903691341897,
131.040919681268)) ;
#119141=CARTESIAN_POINT('Ctrl Pts',(-18.1099224441214,12.7636900645103,
131.176588861018)) ;
#119142=CARTESIAN_POINT('Ctrl Pts',(-18.1860910752611,12.58293139644,131.365788966717)) ;
#119143=CARTESIAN_POINT('Ctrl Pts',(-18.2742132626293,12.464078841243,131.590363575954)) ;
#119144=CARTESIAN_POINT('Ctrl Pts',(-18.3709498681828,12.4125693581943,
131.839671118017)) ;
#119145=CARTESIAN_POINT('Ctrl Pts',(-18.4681772253489,12.4337094194749,
132.090710617766)) ;
#119146=CARTESIAN_POINT('Ctrl Pts',(-18.5613404295381,12.5263145270348,
132.329552530544)) ;
#119147=CARTESIAN_POINT('Ctrl Pts',(-18.6427630328411,12.6822587422614,
132.534418750328)) ;
#119148=CARTESIAN_POINT('Ctrl Pts',(-18.7085834048123,12.8915625531578,
132.693572369479)) ;
#119149=CARTESIAN_POINT('Ctrl Pts',(-18.7544451348481,13.1392603074742,
132.794397450571)) ;
#119150=CARTESIAN_POINT('Ctrl Pts',(-18.7776939684164,13.4076118636345,
132.829123711321)) ;
#119151=CARTESIAN_POINT('Ctrl Pts',(-18.7775202118103,13.6757335658836,
132.795606435297)) ;
#119152=CARTESIAN_POINT('Ctrl Pts',(-18.7543460918851,13.9281677247044,
132.694557225827)) ;
#119153=CARTESIAN_POINT('Ctrl Pts',(-18.7113664052483,14.1410411495776,
132.536164994947)) ;
#119154=CARTESIAN_POINT('Ctrl Pts',(-18.6513254308885,14.3051859901722,
132.327503000793)) ;
#119155=CARTESIAN_POINT('Ctrl Pts',(-18.5800781063794,14.4050577733478,
132.08631379624)) ;
#119156=CARTESIAN_POINT('Ctrl Pts',(-18.5028620340349,14.4349188598701,
131.827543141422)) ;
#119157=CARTESIAN_POINT('Ctrl Pts',(-18.4265303796658,14.3922309368258,
131.571501632903)) ;
#119158=CARTESIAN_POINT('Ctrl Pts',(-18.3568271888468,14.2801808251174,
131.334757650015)) ;
#119159=CARTESIAN_POINT('Ctrl Pts',(-18.2996259717083,14.1070360117015,
131.134575830755)) ;
#119160=CARTESIAN_POINT('Ctrl Pts',(-18.2595414806214,13.8833119581465,
130.984173543853)) ;
#119161=CARTESIAN_POINT('Ctrl Pts',(-18.2406706595755,13.6288342320535,
130.896064565764)) ;
#119162=CARTESIAN_POINT('Ctrl Pts',(-18.2446440431587,13.3582466127621,
130.874495973325)) ;
#119163=CARTESIAN_POINT('Ctrl Pts',(-18.2720331997506,13.0930921970462,
130.921437176205)) ;
#119164=CARTESIAN_POINT('Ctrl Pts',(-18.3216690049672,12.8509541226963,
131.033284294486)) ;
#119165=CARTESIAN_POINT('Ctrl Pts',(-18.3906418061962,12.650062531176,131.201654512555)) ;
#119166=CARTESIAN_POINT('Ctrl Pts',(-18.4748708111884,12.504322010349,131.414548325661)) ;
#119167=CARTESIAN_POINT('Ctrl Pts',(-18.5689804093053,12.424693152161,131.656306690995)) ;
#119168=CARTESIAN_POINT('Ctrl Pts',(-18.6664270906772,12.4164961973712,
131.907982194017)) ;
#119169=CARTESIAN_POINT('Ctrl Pts',(-18.7619319234567,12.4802514111472,
132.153820565409)) ;
#119170=CARTESIAN_POINT('Ctrl Pts',(-18.8488118214195,12.6116452910191,
132.374492857226)) ;
#119171=CARTESIAN_POINT('Ctrl Pts',(-18.9216643022121,12.8011772311019,
132.554182029598)) ;
#119172=CARTESIAN_POINT('Ctrl Pts',(-18.9759494387784,13.0350450036084,
132.679662652176)) ;
#119173=CARTESIAN_POINT('Ctrl Pts',(-19.008603835286,13.2969780565828,132.741915753718)) ;
#119174=CARTESIAN_POINT('Ctrl Pts',(-19.0179410748661,13.5677347022496,
132.736081758383)) ;
#119175=CARTESIAN_POINT('Ctrl Pts',(-19.0040398597584,13.8283851985519,
132.662329536592)) ;
#119176=CARTESIAN_POINT('Ctrl Pts',(-18.9686055938327,14.0598714357244,
132.525687738623)) ;
#119177=CARTESIAN_POINT('Ctrl Pts',(-18.9149811896249,14.2455587727683,
132.335940170202)) ;
#119178=CARTESIAN_POINT('Ctrl Pts',(-18.8476802246462,14.3725641558704,
132.106227330158)) ;
#119179=CARTESIAN_POINT('Ctrl Pts',(-18.7719847153341,14.4315964719956,
131.851881968485)) ;
#119180=CARTESIAN_POINT('Ctrl Pts',(-18.6946462872458,14.4181824180769,
131.592890297641)) ;
#119181=CARTESIAN_POINT('Ctrl Pts',(-18.6214844495098,14.3336378097198,
131.346050846128)) ;
#119182=CARTESIAN_POINT('Ctrl Pts',(-18.558560768651,14.1840091136267,131.12913359779)) ;
#119183=CARTESIAN_POINT('Ctrl Pts',(-18.5109894847597,13.9789558298509,
130.956930823342)) ;
#119184=CARTESIAN_POINT('Ctrl Pts',(-18.4832446592943,13.735580763414,130.842869411275)) ;
#119185=CARTESIAN_POINT('Ctrl Pts',(-18.4777486344568,13.4678622164134,
130.793539893276)) ;
#119186=CARTESIAN_POINT('Ctrl Pts',(-18.495693449302,13.1991328170732,130.812970863617)) ;
#119187=CARTESIAN_POINT('Ctrl Pts',(-18.5365410093149,12.9452257159657,
130.89915162287)) ;
#119188=CARTESIAN_POINT('Ctrl Pts',(-18.5980095580789,12.7259341405257,
131.045633388828)) ;
#119189=CARTESIAN_POINT('Ctrl Pts',(-18.6767481508151,12.5559411179341,
131.242447155862)) ;
#119190=CARTESIAN_POINT('Ctrl Pts',(-18.7675488804155,12.4485460989971,
131.474543240346)) ;
#119191=CARTESIAN_POINT('Ctrl Pts',(-18.864393631756,12.411159941536,131.724388858746)) ;
#119192=CARTESIAN_POINT('Ctrl Pts',(-18.9612913750933,12.4456278245902,
131.974422082055)) ;
#119193=CARTESIAN_POINT('Ctrl Pts',(-19.0529969299443,12.5514145649144,
132.208941501209)) ;
#119194=CARTESIAN_POINT('Ctrl Pts',(-19.1316790447807,12.7181519501975,
132.405838209825)) ;
#119195=CARTESIAN_POINT('Ctrl Pts',(-19.1941048725885,12.9364297118054,
132.555003305589)) ;
#119196=CARTESIAN_POINT('Ctrl Pts',(-19.2356761496976,13.1887531889945,
132.643385652304)) ;
#119197=CARTESIAN_POINT('Ctrl Pts',(-19.2545675080689,13.4580633394379,
132.665473483181)) ;
#119198=CARTESIAN_POINT('Ctrl Pts',(-19.2499351678231,13.7256377913563,
132.618747198731)) ;
#119199=CARTESIAN_POINT('Ctrl Pts',(-19.222967559006,13.9704139495142,132.506920039618)) ;
#119200=CARTESIAN_POINT('Ctrl Pts',(-19.1762304653284,14.1767864400758,
132.337249155195)) ;
#119201=CARTESIAN_POINT('Ctrl Pts',(-19.1135752785484,14.3292888579234,
132.120987640675)) ;
#119202=CARTESIAN_POINT('Ctrl Pts',(-19.0408547841555,14.4162419047305,
131.875517748366)) ;
#119203=CARTESIAN_POINT('Ctrl Pts',(-18.9633148456444,14.4323070590761,
131.615823606619)) ;
#119204=CARTESIAN_POINT('Ctrl Pts',(-18.8879283003201,14.3764282439281,
131.362607849227)) ;
#119205=CARTESIAN_POINT('Ctrl Pts',(-18.8198998869481,14.2515625460975,
131.130626311494)) ;
#119206=CARTESIAN_POINT('Ctrl Pts',(-18.7657339233337,14.0682228318719,
130.939356613635)) ;
#119207=CARTESIAN_POINT('Ctrl Pts',(-18.7293985887039,13.8370233843303,
130.799918521597)) ;
#119208=CARTESIAN_POINT('Ctrl Pts',(-18.714753132366,13.5786249866576,130.724188870764)) ;
#119209=CARTESIAN_POINT('Ctrl Pts',(-18.7231251925275,13.3076277382397,
130.715494911597)) ;
#119210=CARTESIAN_POINT('Ctrl Pts',(-18.7548319263464,13.0452573122607,
130.775019949537)) ;
#119211=CARTESIAN_POINT('Ctrl Pts',(-18.8084749840881,12.8091512622852,
130.89851543204)) ;
#119212=CARTESIAN_POINT('Ctrl Pts',(-18.8808676525224,12.617551612867,131.076811574621)) ;
#119213=CARTESIAN_POINT('Ctrl Pts',(-18.966903542301,12.4843718023618,131.295172588613)) ;
#119214=CARTESIAN_POINT('Ctrl Pts',(-19.0622475184182,12.4175958724791,
131.540512838689)) ;
#119215=CARTESIAN_POINT('Ctrl Pts',(-19.1600037141583,12.4230554954089,
131.792998859898)) ;
#119216=CARTESIAN_POINT('Ctrl Pts',(-19.2543388718931,12.5002516562104,
132.035417010935)) ;
#119217=CARTESIAN_POINT('Ctrl Pts',(-19.338755390033,12.6429371553798,132.248988409665)) ;
#119218=CARTESIAN_POINT('Ctrl Pts',(-19.4087513849138,12.8430359620073,
132.420167940555)) ;
#119219=CARTESIAN_POINT('Ctrl Pts',(-19.4589520558227,13.0829430987805,
132.533810431169)) ;
#119220=CARTESIAN_POINT('Ctrl Pts',(-19.4872983129428,13.348262589156,132.58344872288)) ;
#119221=CARTESIAN_POINT('Ctrl Pts',(-19.4921943292312,13.617980538018,132.564712919865)) ;
#119222=CARTESIAN_POINT('Ctrl Pts',(-19.4739943482068,13.8754577927148,
132.478285317474)) ;
#119223=CARTESIAN_POINT('Ctrl Pts',(-19.4347077988006,14.0994368224178,
132.330372944685)) ;
#119224=CARTESIAN_POINT('Ctrl Pts',(-19.3782971940941,14.2743408293056,
132.132593583898)) ;
#119225=CARTESIAN_POINT('Ctrl Pts',(-19.3088357404323,14.3892596729095,
131.896487153757)) ;
#119226=CARTESIAN_POINT('Ctrl Pts',(-19.2325449021963,14.4346258040112,
131.640520892899)) ;
#119227=CARTESIAN_POINT('Ctrl Pts',(-19.1551979357679,14.4074612330324,
131.381356793623)) ;
#119228=CARTESIAN_POINT('Ctrl Pts',(-19.083606290679,14.3096987835835,131.139122210316)) ;
#119229=CARTESIAN_POINT('Ctrl Pts',(-19.0234462893368,14.1493774031888,
130.930391073382)) ;
#119230=CARTESIAN_POINT('Ctrl Pts',(-18.9792574006034,13.935562868649,130.768056883055)) ;
#119231=CARTESIAN_POINT('Ctrl Pts',(-18.9555376955123,13.6861606118435,
130.665702303709)) ;
#119232=CARTESIAN_POINT('Ctrl Pts',(-18.954462394183,13.4167352169348,130.629337609962)) ;
#119233=CARTESIAN_POINT('Ctrl Pts',(-18.9768166950085,13.1492793406519,
130.661613632357)) ;
#119234=CARTESIAN_POINT('Ctrl Pts',(-19.0218215119309,12.9005268787558,
130.759937465637)) ;
#119235=CARTESIAN_POINT('Ctrl Pts',(-19.0867458494723,12.6897474261303,
130.916549878415)) ;
#119236=CARTESIAN_POINT('Ctrl Pts',(-19.1682533043497,12.5306016297354,
131.121425098996)) ;
#119237=CARTESIAN_POINT('Ctrl Pts',(-19.260528066382,12.4360458848473,131.35789087038)) ;
#119238=CARTESIAN_POINT('Ctrl Pts',(-19.3582763243507,12.412131814889,131.610239658224)) ;
#119239=CARTESIAN_POINT('Ctrl Pts',(-19.4545355523176,12.4605358033904,
131.858387318007)) ;
#119240=CARTESIAN_POINT('Ctrl Pts',(-19.5439662249688,12.5784164440372,
132.086417619438)) ;
#119241=CARTESIAN_POINT('Ctrl Pts',(-19.6198702779238,12.7554816677878,
132.275200633831)) ;
#119242=CARTESIAN_POINT('Ctrl Pts',(-19.6786787472394,12.981762434369,132.413779248081)) ;
#119243=CARTESIAN_POINT('Ctrl Pts',(-19.7160997954442,13.2381598405705,
132.490097944135)) ;
#119244=CARTESIAN_POINT('Ctrl Pts',(-19.7305986983189,13.5101992275675,
132.499139671301)) ;
#119245=CARTESIAN_POINT('Ctrl Pts',(-19.7216726258315,13.7733131452284,
132.440105357691)) ;
#119246=CARTESIAN_POINT('Ctrl Pts',(-19.6904705567742,14.0140641414936,
132.315613122368)) ;
#119247=CARTESIAN_POINT('Ctrl Pts',(-19.6405829973198,14.2098744851872,
132.136924271088)) ;
#119248=CARTESIAN_POINT('Ctrl Pts',(-19.5757967424892,14.350580234219,131.914544882587)) ;
#119249=CARTESIAN_POINT('Ctrl Pts',(-19.5016300544753,14.424831664933,131.664786233143)) ;
#119250=CARTESIAN_POINT('Ctrl Pts',(-19.4237853420446,14.4272048065726,
131.404140384913)) ;
#119251=CARTESIAN_POINT('Ctrl Pts',(-19.3494177718881,14.3577939538396,
131.15388324979)) ;
#119252=CARTESIAN_POINT('Ctrl Pts',(-19.2837725347632,14.2217457510102,
130.929018006421)) ;
#119253=CARTESIAN_POINT('Ctrl Pts',(-19.2323040587634,14.0267541205093,
130.745331387743)) ;
#119254=CARTESIAN_POINT('Ctrl Pts',(-19.2001707430858,13.7911380012518,
130.618536649777)) ;
#119255=CARTESIAN_POINT('Ctrl Pts',(-19.1896182239787,13.5273990690374,
130.554516339063)) ;
#119256=CARTESIAN_POINT('Ctrl Pts',(-19.2024378328386,13.2571616705375,
130.55890952724)) ;
#119257=CARTESIAN_POINT('Ctrl Pts',(-19.2385890329441,12.9974108749585,
130.631270893564)) ;
#119258=CARTESIAN_POINT('Ctrl Pts',(-19.2958501694243,12.7695379625925,
130.76548642622)) ;
#119259=CARTESIAN_POINT('Ctrl Pts',(-19.3711145282568,12.5879936819102,
130.952222944991)) ;
#119260=CARTESIAN_POINT('Ctrl Pts',(-19.4594662841901,12.4663339694794,
131.177257058661)) ;
#119261=CARTESIAN_POINT('Ctrl Pts',(-19.5560732523899,12.4130530302768,
131.426195851942)) ;
#119262=CARTESIAN_POINT('Ctrl Pts',(-19.6531733858751,12.4321501151392,
131.676919018143)) ;
#119263=CARTESIAN_POINT('Ctrl Pts',(-19.7463970498452,12.5224108071959,
131.916006524141)) ;
#119264=CARTESIAN_POINT('Ctrl Pts',(-19.8285870860188,12.6773122255345,
132.122965690291)) ;
#119265=CARTESIAN_POINT('Ctrl Pts',(-19.8948121933427,12.8853931942508,
132.283318194652)) ;
#119266=CARTESIAN_POINT('Ctrl Pts',(-19.9411314766599,13.1311434549155,
132.385618122778)) ;
#119267=CARTESIAN_POINT('Ctrl Pts',(-19.965179017902,13.4000886960601,132.422564022338)) ;
#119268=CARTESIAN_POINT('Ctrl Pts',(-19.9655799290756,13.6679854854521,
132.390772501259)) ;
#119269=CARTESIAN_POINT('Ctrl Pts',(-19.9433576038818,13.9198929114768,
132.292714121361)) ;
#119270=CARTESIAN_POINT('Ctrl Pts',(-19.9003340118905,14.1367331650745,
132.133759563188)) ;
#119271=CARTESIAN_POINT('Ctrl Pts',(-19.8412787515206,14.3006761293965,
131.928331239691)) ;
#119272=CARTESIAN_POINT('Ctrl Pts',(-19.7698433836344,14.4034182515294,
131.686360469873)) ;
#119273=CARTESIAN_POINT('Ctrl Pts',(-19.6928908319003,14.4350219442823,
131.428454049308)) ;
#119274=CARTESIAN_POINT('Ctrl Pts',(-19.6163658838612,14.3943912084008,
131.171802938922)) ;
#119275=CARTESIAN_POINT('Ctrl Pts',(-19.5464071737182,14.2842181176635,
130.934326074757)) ;
#119276=CARTESIAN_POINT('Ctrl Pts',(-19.4887700986895,14.1123337883522,
130.732832985859)) ;
#119277=CARTESIAN_POINT('Ctrl Pts',(-19.4483529098591,13.8914433195642,
130.581689210717)) ;
#119278=CARTESIAN_POINT('Ctrl Pts',(-19.4286626325355,13.6364805830374,
130.491015707154)) ;
#119279=CARTESIAN_POINT('Ctrl Pts',(-19.4319737247805,13.3663281514523,
130.467552630673)) ;
#119280=CARTESIAN_POINT('Ctrl Pts',(-19.4587287510164,13.1002904677936,
130.512580019223)) ;
#119281=CARTESIAN_POINT('Ctrl Pts',(-19.5077690316902,12.857318656671,130.622698530342)) ;
#119282=CARTESIAN_POINT('Ctrl Pts',(-19.5762479760817,12.6550558730351,
130.789623948442)) ;
#119283=CARTESIAN_POINT('Ctrl Pts',(-19.660020761891,12.5076994857307,131.001221346156)) ;
#119284=CARTESIAN_POINT('Ctrl Pts',(-19.7539073771051,12.4260782078646,
131.24233160486)) ;
#119285=CARTESIAN_POINT('Ctrl Pts',(-19.8512928032056,12.415541436623,131.493846182344)) ;
#119286=CARTESIAN_POINT('Ctrl Pts',(-19.9476463280343,12.4780902877727,
131.741909766604)) ;
#119287=CARTESIAN_POINT('Ctrl Pts',(-20.0340220644824,12.6066343882026,
131.961417774719)) ;
#119288=CARTESIAN_POINT('Ctrl Pts',(-20.1076913571221,12.7952136199714,
132.143357435918)) ;
#119289=CARTESIAN_POINT('Ctrl Pts',(-20.1624822594016,13.027981899229,132.270339157323)) ;
#119290=CARTESIAN_POINT('Ctrl Pts',(-20.1958184055906,13.289687480561,132.334542561591)) ;
#119291=CARTESIAN_POINT('Ctrl Pts',(-20.2057710640606,13.5603128220289,
132.330524427759)) ;
#119292=CARTESIAN_POINT('Ctrl Pts',(-20.1925448224243,13.8211027693198,
132.258797489589)) ;
#119293=CARTESIAN_POINT('Ctrl Pts',(-20.1576816405266,14.0538032313773,
132.123806125058)) ;
#119294=CARTESIAN_POINT('Ctrl Pts',(-20.1045068706167,14.241090775664,131.935361080149)) ;
#119295=CARTESIAN_POINT('Ctrl Pts',(-20.0373054709632,14.3701941266746,
131.705842074109)) ;
#119296=CARTESIAN_POINT('Ctrl Pts',(-19.9618110201247,14.4308809538835,
131.452116070863)) ;
#119297=CARTESIAN_POINT('Ctrl Pts',(-19.884682289029,14.419613884929,131.193839945316)) ;
#119298=CARTESIAN_POINT('Ctrl Pts',(-19.8111397376494,14.336836848792,130.945808512456)) ;
#119299=CARTESIAN_POINT('Ctrl Pts',(-19.7480300404302,14.1892311094166,
130.728433160336)) ;
#119300=CARTESIAN_POINT('Ctrl Pts',(-19.699933640509,13.9859053267194,130.55472695681)) ;
#119301=CARTESIAN_POINT('Ctrl Pts',(-19.6715026585646,13.742611201067,130.438550909152)) ;
#119302=CARTESIAN_POINT('Ctrl Pts',(-19.6653745692253,13.4761438373695,
130.387484991165)) ;
#119303=CARTESIAN_POINT('Ctrl Pts',(-19.682584552737,13.2070931418873,130.404753014799)) ;
#119304=CARTESIAN_POINT('Ctrl Pts',(-19.7228474706637,12.9521503687759,
130.489184402937)) ;
#119305=CARTESIAN_POINT('Ctrl Pts',(-19.7837584916582,12.7315094149766,
130.634031485)) ;
#119306=CARTESIAN_POINT('Ctrl Pts',(-19.8624328122891,12.5595225536488,
130.830528406558)) ;
#119307=CARTESIAN_POINT('Ctrl Pts',(-19.9522381164699,12.4509681334738,
131.059982587645)) ;
#119308=CARTESIAN_POINT('Ctrl Pts',(-20.0497696412485,12.4111337658692,
131.311559834098)) ;
#119309=CARTESIAN_POINT('Ctrl Pts',(-20.1462880258714,12.4436883984276,
131.56064510183)) ;
#119310=CARTESIAN_POINT('Ctrl Pts',(-20.2383160802438,12.547486739405,131.796082088667)) ;
#119311=CARTESIAN_POINT('Ctrl Pts',(-20.3173266702043,12.7123018084608,
131.993987635883)) ;
#119312=CARTESIAN_POINT('Ctrl Pts',(-20.3804588499448,12.9300708055824,
132.145107785543)) ;
#119313=CARTESIAN_POINT('Ctrl Pts',(-20.4224709372142,13.1802337524753,
132.234962055865)) ;
#119314=CARTESIAN_POINT('Ctrl Pts',(-20.442183503171,13.4510759220384,132.259227541376)) ;
#119315=CARTESIAN_POINT('Ctrl Pts',(-20.4381680886622,13.7180592996578,
132.214421277915)) ;
#119316=CARTESIAN_POINT('Ctrl Pts',(-20.4117618848203,13.964278608138,132.104156183895)) ;
#119317=CARTESIAN_POINT('Ctrl Pts',(-20.3656256486064,14.1712561679291,
131.936335517623)) ;
#119318=CARTESIAN_POINT('Ctrl Pts',(-20.3036358508574,14.325372518196,131.722127818412)) ;
#119319=CARTESIAN_POINT('Ctrl Pts',(-20.2305670104494,14.4148742609065,
131.475380669503)) ;
#119320=CARTESIAN_POINT('Ctrl Pts',(-20.1536631641384,14.4329087895001,
131.217807240407)) ;
#119321=CARTESIAN_POINT('Ctrl Pts',(-20.0776209899408,14.3788838445396,
130.962446101852)) ;
#119322=CARTESIAN_POINT('Ctrl Pts',(-20.0095302198618,14.2561019956526,
130.730397244583)) ;
#119323=CARTESIAN_POINT('Ctrl Pts',(-19.9548661761338,14.0742378272797,
130.537646874608)) ;
#119324=CARTESIAN_POINT('Ctrl Pts',(-19.9180661082019,13.8451950259534,
130.396991637115)) ;
#119325=CARTESIAN_POINT('Ctrl Pts',(-19.9026012514215,13.5867435987056,
130.31877045493)) ;
#119326=CARTESIAN_POINT('Ctrl Pts',(-19.9104102974492,13.3144405101765,
130.308268426565)) ;
#119327=CARTESIAN_POINT('Ctrl Pts',(-19.9413741530792,13.0528696187883,
130.365781080122)) ;
#119328=CARTESIAN_POINT('Ctrl Pts',(-19.994244180026,12.8160518820106,130.487079529653)) ;
#119329=CARTESIAN_POINT('Ctrl Pts',(-20.0661895688882,12.6226065915497,
130.664031439332)) ;
#119330=CARTESIAN_POINT('Ctrl Pts',(-20.15206016138,12.4871997315169,130.881839087243)) ;
#119331=CARTESIAN_POINT('Ctrl Pts',(-20.2475919792039,12.4184347778258,
131.127610415521)) ;
#119332=CARTESIAN_POINT('Ctrl Pts',(-20.3447915155676,12.4219001112793,
131.378662151802)) ;
#119333=CARTESIAN_POINT('Ctrl Pts',(-20.4394385866213,12.4968774308013,
131.621957625327)) ;
#119334=CARTESIAN_POINT('Ctrl Pts',(-20.5243460496228,12.6381725760813,
131.83689984342)) ;
#119335=CARTESIAN_POINT('Ctrl Pts',(-20.5946432733037,12.836067679816,132.009073672112)) ;
#119336=CARTESIAN_POINT('Ctrl Pts',(-20.645694549428,13.0762565431926,132.125027230254)) ;
#119337=CARTESIAN_POINT('Ctrl Pts',(-20.6745353505578,13.3398740160854,
132.176274252452)) ;
#119338=CARTESIAN_POINT('Ctrl Pts',(-20.6801824917773,13.6103043330608,
132.159657715316)) ;
#119339=CARTESIAN_POINT('Ctrl Pts',(-20.6626223670688,13.8681249215715,
132.075137952304)) ;
#119340=CARTESIAN_POINT('Ctrl Pts',(-20.6240088572483,14.093287105724,131.929218574679)) ;
#119341=CARTESIAN_POINT('Ctrl Pts',(-20.5676185800388,14.2707836403436,
131.731276399914)) ;
#119342=CARTESIAN_POINT('Ctrl Pts',(-20.4988452517907,14.3866738384329,
131.49738923641)) ;
#119343=CARTESIAN_POINT('Ctrl Pts',(-20.422630635606,14.4343395639672,131.241618386863)) ;
#119344=CARTESIAN_POINT('Ctrl Pts',(-20.3453774182086,14.4093417175208,
130.982795501148)) ;
#119345=CARTESIAN_POINT('Ctrl Pts',(-20.2734835723203,14.3139583331245,
130.739681166384)) ;
#119346=CARTESIAN_POINT('Ctrl Pts',(-20.2125244829768,14.1538396141847,
130.528356549995)) ;
#119347=CARTESIAN_POINT('Ctrl Pts',(-20.1682116920328,13.9434082127298,
130.365988093249)) ;
#119348=CARTESIAN_POINT('Ctrl Pts',(-20.1436214196191,13.6926166165872,
130.260781902215)) ;
#119349=CARTESIAN_POINT('Ctrl Pts',(-20.1419610296582,13.425230952717,130.222938931373)) ;
#119350=CARTESIAN_POINT('Ctrl Pts',(-20.1635998921199,13.1569924871447,
130.253058297191)) ;
#119351=CARTESIAN_POINT('Ctrl Pts',(-20.2079427538387,12.9074157476161,
130.349462629733)) ;
#119352=CARTESIAN_POINT('Ctrl Pts',(-20.2726497055643,12.6946405616374,
130.505302726905)) ;
#119353=CARTESIAN_POINT('Ctrl Pts',(-20.3531722071491,12.5348309308551,
130.707538050332)) ;
#119354=CARTESIAN_POINT('Ctrl Pts',(-20.4457849117443,12.4376124689349,
130.944772900056)) ;
#119355=CARTESIAN_POINT('Ctrl Pts',(-20.5429650872583,12.4118470514465,
131.195641249944)) ;
#119356=CARTESIAN_POINT('Ctrl Pts',(-20.6395134396743,12.4580456544619,
131.444573191783)) ;
#119357=CARTESIAN_POINT('Ctrl Pts',(-20.729060984578,12.5736491216982,131.673021193367)) ;
#119358=CARTESIAN_POINT('Ctrl Pts',(-20.805710500231,12.7495591694402,131.863869452614)) ;
#119359=CARTESIAN_POINT('Ctrl Pts',(-20.8652025700878,12.9753683734727,
132.004359633657)) ;
#119360=CARTESIAN_POINT('Ctrl Pts',(-20.9031724037638,13.2312289838448,
132.082275133185)) ;
#119361=CARTESIAN_POINT('Ctrl Pts',(-20.9183045192812,13.5022491651901,
132.093281255523)) ;
#119362=CARTESIAN_POINT('Ctrl Pts',(-20.9099738643423,13.7663767191028,
132.035905471493)) ;
#119363=CARTESIAN_POINT('Ctrl Pts',(-20.8796612889415,14.0063276697149,
131.914271616436)) ;
#119364=CARTESIAN_POINT('Ctrl Pts',(-20.8301303204373,14.2048736282249,
131.736455792172)) ;
#119365=CARTESIAN_POINT('Ctrl Pts',(-20.7654662816806,14.347691195203,131.514334056963)) ;
#119366=CARTESIAN_POINT('Ctrl Pts',(-20.6914004383808,14.4237776298714,
131.264839696289)) ;
#119367=CARTESIAN_POINT('Ctrl Pts',(-20.6137773916912,14.4280807794616,
131.004929859582)) ;
#119368=CARTESIAN_POINT('Ctrl Pts',(-20.539195883422,14.3608278808949,130.754040559795)) ;
#119369=CARTESIAN_POINT('Ctrl Pts',(-20.4730252235718,14.2256360688744,
130.527499972187)) ;
#119370=CARTESIAN_POINT('Ctrl Pts',(-20.4216242912697,14.0344800390557,
130.344399892003)) ;
#119371=CARTESIAN_POINT('Ctrl Pts',(-20.3885184235804,13.7980436571723,
130.214472970683)) ;
#119372=CARTESIAN_POINT('Ctrl Pts',(-20.377391550382,13.5353242806262,130.148856167655)) ;
#119373=CARTESIAN_POINT('Ctrl Pts',(-20.3895664665377,13.2644874689488,
130.151292077717)) ;
#119374=CARTESIAN_POINT('Ctrl Pts',(-20.424935009537,13.0050529303368,130.22149042803)) ;
#119375=CARTESIAN_POINT('Ctrl Pts',(-20.4817292085783,12.7754380725172,
130.354257719508)) ;
#119376=CARTESIAN_POINT('Ctrl Pts',(-20.5564557866067,12.5925960491714,
130.539466126606)) ;
#119377=CARTESIAN_POINT('Ctrl Pts',(-20.6444867076033,12.4690082220502,
130.763560977221)) ;
#119378=CARTESIAN_POINT('Ctrl Pts',(-20.7408881356029,12.4135709144517,
131.011922988235)) ;
#119379=CARTESIAN_POINT('Ctrl Pts',(-20.8382190130878,12.4306394934732,
131.263254378113)) ;
#119380=CARTESIAN_POINT('Ctrl Pts',(-20.9313842847165,12.518547510187,131.502278584203)) ;
#119381=CARTESIAN_POINT('Ctrl Pts',(-21.0141043074733,12.6718440202401,
131.71073096347)) ;
#119382=CARTESIAN_POINT('Ctrl Pts',(-21.0808229800916,12.8780301734486,
131.87258818294)) ;
#119383=CARTESIAN_POINT('Ctrl Pts',(-21.1280885064397,13.1252486196316,
131.977346576472)) ;
#119384=CARTESIAN_POINT('Ctrl Pts',(-21.1525153261514,13.3909665583226,
132.015767819946)) ;
#119385=CARTESIAN_POINT('Ctrl Pts',(-21.1536959682209,13.6612160977101,
131.985989530158)) ;
#119386=CARTESIAN_POINT('Ctrl Pts',(-21.1320150342008,13.9131568829426,
131.889591648472)) ;
#119387=CARTESIAN_POINT('Ctrl Pts',(-21.0898050363088,14.1304384080909,
131.733161381014)) ;
#119388=CARTESIAN_POINT('Ctrl Pts',(-21.0309240465131,14.2969775123332,
131.528087499457)) ;
#119389=CARTESIAN_POINT('Ctrl Pts',(-20.9596151124055,14.4015522175217,
131.286441908172)) ;
#119390=CARTESIAN_POINT('Ctrl Pts',(-20.8830101894348,14.4350500549688,
131.029664145072)) ;
#119391=CARTESIAN_POINT('Ctrl Pts',(-20.8064689258357,14.3967519657553,
130.773004975845)) ;
#119392=CARTESIAN_POINT('Ctrl Pts',(-20.736137213621,14.288484921225,130.534398606633)) ;
#119393=CARTESIAN_POINT('Ctrl Pts',(-20.6779987919655,14.1181740958946,
130.331417324993)) ;
#119394=CARTESIAN_POINT('Ctrl Pts',(-20.6369638489005,13.897753350153,130.178370778553)) ;
#119395=CARTESIAN_POINT('Ctrl Pts',(-20.6167209882591,13.6446684780805,
130.086235861724)) ;
#119396=CARTESIAN_POINT('Ctrl Pts',(-20.619340577804,13.3734340480479,130.060596345406)) ;
#119397=CARTESIAN_POINT('Ctrl Pts',(-20.6455250015525,13.1072276991085,
130.103978026727)) ;
#119398=CARTESIAN_POINT('Ctrl Pts',(-20.6937727870842,12.8641925809132,
130.211898521061)) ;
#119399=CARTESIAN_POINT('Ctrl Pts',(-20.7616960829119,12.660522785721,130.377207275628)) ;
#119400=CARTESIAN_POINT('Ctrl Pts',(-20.8449119130546,12.511411763425,130.587233212525)) ;
#119401=CARTESIAN_POINT('Ctrl Pts',(-20.9391429401049,12.4272142219304,
130.829153099245)) ;
#119402=CARTESIAN_POINT('Ctrl Pts',(-21.0363686243683,12.4150347964973,
131.08024552193)) ;
#119403=CARTESIAN_POINT('Ctrl Pts',(-21.1322461258614,12.4747491007078,
131.327146007877)) ;
#119404=CARTESIAN_POINT('Ctrl Pts',(-21.2197199461853,12.6023245536218,
131.549581888249)) ;
#119405=CARTESIAN_POINT('Ctrl Pts',(-21.2937940109995,12.7898413846695,
131.732688168851)) ;
#119406=CARTESIAN_POINT('Ctrl Pts',(-21.348940422816,13.0206706862551,131.860832964274)) ;
#119407=CARTESIAN_POINT('Ctrl Pts',(-21.382960122206,13.2818517746603,131.927025375257)) ;
#119408=CARTESIAN_POINT('Ctrl Pts',(-21.3935927663565,13.5521277577084,
131.925035187636)) ;
#119409=CARTESIAN_POINT('Ctrl Pts',(-21.3810616946639,13.813956814144,131.855287243746)) ;
#119410=CARTESIAN_POINT('Ctrl Pts',(-21.3465398686618,14.0485698568868,
131.721146403302)) ;
#119411=CARTESIAN_POINT('Ctrl Pts',(-21.2941458660045,14.2361101273789,
131.535193791347)) ;
#119412=CARTESIAN_POINT('Ctrl Pts',(-21.2270914422676,14.3675383856298,
131.306000181281)) ;
#119413=CARTESIAN_POINT('Ctrl Pts',(-21.1519155292443,14.4300942221494,
131.053285104387)) ;
#119414=CARTESIAN_POINT('Ctrl Pts',(-21.0746459363559,14.4208865281834,
130.794540497998)) ;
#119415=CARTESIAN_POINT('Ctrl Pts',(-21.001112219321,14.3405661224656,130.546646854831)) ;
#119416=CARTESIAN_POINT('Ctrl Pts',(-20.937120477542,14.1934622842168,130.3264194687)) ;
#119417=CARTESIAN_POINT('Ctrl Pts',(-20.8887672599036,13.9917022316215,
130.152052794577)) ;
#119418=CARTESIAN_POINT('Ctrl Pts',(-20.8598430962362,13.7502056970642,
130.034549564694)) ;
#119419=CARTESIAN_POINT('Ctrl Pts',(-20.8529784671607,13.4844947698669,
129.981374969442)) ;
#119420=CARTESIAN_POINT('Ctrl Pts',(-20.8696066243062,13.2141841161546,
129.99680343668)) ;
#119421=CARTESIAN_POINT('Ctrl Pts',(-20.9091638109946,12.9589228275276,
130.079234682195)) ;
#119422=CARTESIAN_POINT('Ctrl Pts',(-20.9699571386437,12.736270288281,130.223561280645)) ;
#119423=CARTESIAN_POINT('Ctrl Pts',(-21.0470538745652,12.5648475025287,
130.415923378106)) ;
#119424=CARTESIAN_POINT('Ctrl Pts',(-21.1376039575189,12.452872634964,130.647152420772)) ;
#119425=CARTESIAN_POINT('Ctrl Pts',(-21.2341676611939,12.4112941971035,
130.896214160326)) ;
#119426=CARTESIAN_POINT('Ctrl Pts',(-21.3316648724746,12.4419882074806,
131.147838257514)) ;
#119427=CARTESIAN_POINT('Ctrl Pts',(-21.4229908419088,12.5427027853094,
131.381587594232)) ;
#119428=CARTESIAN_POINT('Ctrl Pts',(-21.5030710498832,12.7067963999461,
131.582359437564)) ;
#119429=CARTESIAN_POINT('Ctrl Pts',(-21.5664742795253,12.9221001567719,
131.734452775999)) ;
#119430=CARTESIAN_POINT('Ctrl Pts',(-21.6095474559259,13.1741319901515,
131.827050837015)) ;
#119431=CARTESIAN_POINT('Ctrl Pts',(-21.6296848838974,13.44270233198,131.852822317348)) ;
#119432=CARTESIAN_POINT('Ctrl Pts',(-21.6263843446627,13.7107857110311,
131.810002375717)) ;
#119433=CARTESIAN_POINT('Ctrl Pts',(-21.600705277113,13.9568883161136,131.701999462053)) ;
#119434=CARTESIAN_POINT('Ctrl Pts',(-21.5550025744097,14.1661036759461,
131.535330515378)) ;
#119435=CARTESIAN_POINT('Ctrl Pts',(-21.4932354794709,14.3219385035442,
131.321716095624)) ;
#119436=CARTESIAN_POINT('Ctrl Pts',(-21.4208886136072,14.4130180760167,
131.077294854083)) ;
#119437=CARTESIAN_POINT('Ctrl Pts',(-21.3435192673736,14.4335349357277,
130.818139919528)) ;
#119438=CARTESIAN_POINT('Ctrl Pts',(-21.267305951962,14.3810414404785,130.562248249026)) ;
#119439=CARTESIAN_POINT('Ctrl Pts',(-21.1992675154702,14.2609491196068,
130.330540320895)) ;
#119440=CARTESIAN_POINT('Ctrl Pts',(-21.1438547829946,14.0795344573349,
130.135404883766)) ;
#119441=CARTESIAN_POINT('Ctrl Pts',(-21.106670609368,13.8529284696564,129.993824030551)) ;
#119442=CARTESIAN_POINT('Ctrl Pts',(-21.0904836711693,13.5926908131845,
129.913183715177)) ;
#119443=CARTESIAN_POINT('Ctrl Pts',(-21.09762069255,13.3230678960584,129.9010472229)) ;
#119444=CARTESIAN_POINT('Ctrl Pts',(-21.1279913585488,13.0595445585026,
129.956646120741)) ;
#119445=CARTESIAN_POINT('Ctrl Pts',(-21.1804984490399,12.8214089952354,
130.076819568822)) ;
#119446=CARTESIAN_POINT('Ctrl Pts',(-21.2518741011598,12.6270968112276,
130.252173926582)) ;
#119447=CARTESIAN_POINT('Ctrl Pts',(-21.3371200957935,12.4904302156697,
130.468268629472)) ;
#119448=CARTESIAN_POINT('Ctrl Pts',(-21.4321546316194,12.4195264236209,
130.712690158666)) ;
#119449=CARTESIAN_POINT('Ctrl Pts',(-21.5298416099683,12.4206997898043,
130.965004120227)) ;
#119450=CARTESIAN_POINT('Ctrl Pts',(-21.6247959686863,12.4940151271389,
131.20914827549)) ;
#119451=CARTESIAN_POINT('Ctrl Pts',(-21.709797461265,12.6331734144625,131.424459861136)) ;
#119452=CARTESIAN_POINT('Ctrl Pts',(-21.7805396224499,12.829325604419,131.597967844346)) ;
#119453=CARTESIAN_POINT('Ctrl Pts',(-21.8322255266126,13.0683012054675,
131.715794377032)) ;
#119454=CARTESIAN_POINT('Ctrl Pts',(-21.8618419256898,13.332296684324,131.769201522451)) ;
#119455=CARTESIAN_POINT('Ctrl Pts',(-21.868111171437,13.6026349235875,131.754424312256)) ;
#119456=CARTESIAN_POINT('Ctrl Pts',(-21.8512879527441,13.8605088298962,
131.672141207112)) ;
#119457=CARTESIAN_POINT('Ctrl Pts',(-21.8132105801239,14.0871784145907,
131.527740188039)) ;
#119458=CARTESIAN_POINT('Ctrl Pts',(-21.7575005254597,14.2658344085649,
131.331897526796)) ;
#119459=CARTESIAN_POINT('Ctrl Pts',(-21.688750583467,14.3843789538156,131.097930102092)) ;
#119460=CARTESIAN_POINT('Ctrl Pts',(-21.6124995723037,14.4339734253515,
130.841992592288)) ;
#119461=CARTESIAN_POINT('Ctrl Pts',(-21.5354116726094,14.4110559285979,
130.58374666895)) ;
#119462=CARTESIAN_POINT('Ctrl Pts',(-21.4633422750838,14.3178925023023,
130.340153529223)) ;
#119463=CARTESIAN_POINT('Ctrl Pts',(-21.4018571386856,14.159368658012,130.12724479579)) ;
#119464=CARTESIAN_POINT('Ctrl Pts',(-21.3569844423544,13.9496805303502,
129.963170158196)) ;
#119465=CARTESIAN_POINT('Ctrl Pts',(-21.3318692614842,13.7013469975745,
129.856640370781)) ;
#119466=CARTESIAN_POINT('Ctrl Pts',(-21.3294508982289,13.433016471187,129.816421043685)) ;
#119467=CARTESIAN_POINT('Ctrl Pts',(-21.3503974926524,13.1647607687427,
129.844556985097)) ;
#119468=CARTESIAN_POINT('Ctrl Pts',(-21.3942807962129,12.9137311981176,
129.939518315123)) ;
#119469=CARTESIAN_POINT('Ctrl Pts',(-21.4580541106587,12.7007529774686,
130.092823671191)) ;
#119470=CARTESIAN_POINT('Ctrl Pts',(-21.5386641239171,12.5383275935417,
130.295107054219)) ;
#119471=CARTESIAN_POINT('Ctrl Pts',(-21.6302556277388,12.4398166133593,
130.529639909855)) ;
#119472=CARTESIAN_POINT('Ctrl Pts',(-21.7281728291257,12.4114725012227,
130.782378293215)) ;
#119473=CARTESIAN_POINT('Ctrl Pts',(-21.8246200372728,12.4557968893907,
131.031090267756)) ;
#119474=CARTESIAN_POINT('Ctrl Pts',(-21.9145460533065,12.5696290859636,
131.260604908557)) ;
#119475=CARTESIAN_POINT('Ctrl Pts',(-21.9914398177255,12.7436129416571,
131.452243503122)) ;
#119476=CARTESIAN_POINT('Ctrl Pts',(-22.0515344110072,12.9681022420836,
131.594498874539)) ;
#119477=CARTESIAN_POINT('Ctrl Pts',(-22.0902148569532,13.2239471204996,
131.674408492276)) ;
#119478=CARTESIAN_POINT('Ctrl Pts',(-22.1059704140512,13.4941632666535,
131.687320283684)) ;
#119479=CARTESIAN_POINT('Ctrl Pts',(-22.0983312258742,13.7589186275191,
131.631940757146)) ;
#119480=CARTESIAN_POINT('Ctrl Pts',(-22.0686225131946,13.9998348960523,
131.51207295587)) ;
#119481=CARTESIAN_POINT('Ctrl Pts',(-22.0195948042942,14.1997646334102,
131.335728743533)) ;
#119482=CARTESIAN_POINT('Ctrl Pts',(-21.9554274604182,14.3442637107108,
131.115117618126)) ;
#119483=CARTESIAN_POINT('Ctrl Pts',(-21.8814136845686,14.4224928337565,
130.865706385146)) ;
#119484=CARTESIAN_POINT('Ctrl Pts',(-21.8041935492296,14.4291711137562,
130.607145359423)) ;
#119485=CARTESIAN_POINT('Ctrl Pts',(-21.7288900359016,14.3636108814792,
130.353900660696)) ;
#119486=CARTESIAN_POINT('Ctrl Pts',(-21.6626234455838,14.2305641375214,
130.127196631545)) ;
#119487=CARTESIAN_POINT('Ctrl Pts',(-21.610645454006,14.0406275620916,129.942350483753)) ;
#119488=CARTESIAN_POINT('Ctrl Pts',(-21.5770095653815,13.8058699764793,
129.810964167784)) ;
#119489=CARTESIAN_POINT('Ctrl Pts',(-21.5651598939791,13.5427808202944,
129.743118276341)) ;
#119490=CARTESIAN_POINT('Ctrl Pts',(-21.5766853836118,13.2720605312769,
129.743680167768)) ;
#119491=CARTESIAN_POINT('Ctrl Pts',(-21.6114683168991,13.0118429090763,
129.812136554977)) ;
#119492=CARTESIAN_POINT('Ctrl Pts',(-21.6674973759044,12.7818788170933,
129.942778475518)) ;
#119493=CARTESIAN_POINT('Ctrl Pts',(-21.7419079631877,12.5968716626886,
130.126980320084)) ;
#119494=CARTESIAN_POINT('Ctrl Pts',(-21.8300307322548,12.4712517214802,
130.351211761914)) ;
#119495=CARTESIAN_POINT('Ctrl Pts',(-21.9258253078081,12.4142247969978,
130.597967097194)) ;
#119496=CARTESIAN_POINT('Ctrl Pts',(-22.0233578047668,12.4291610418386,
130.849830342346)) ;
#119497=CARTESIAN_POINT('Ctrl Pts',(-22.1167866797565,12.5152749541959,
131.08960625707)) ;
#119498=CARTESIAN_POINT('Ctrl Pts',(-22.1999681996922,12.6672522382755,
131.299357549445)) ;
#119499=CARTESIAN_POINT('Ctrl Pts',(-22.266877655469,12.8714563581182,131.461897045814)) ;
#119500=CARTESIAN_POINT('Ctrl Pts',(-22.3146434703836,13.1164156516164,
131.568278885002)) ;
#119501=CARTESIAN_POINT('Ctrl Pts',(-22.3399611550803,13.3833143712004,
131.609107421274)) ;
#119502=CARTESIAN_POINT('Ctrl Pts',(-22.3417546305339,13.6536761659143,
131.581130534382)) ;
#119503=CARTESIAN_POINT('Ctrl Pts',(-22.3207495851336,13.9063303611245,
131.486718277812)) ;
#119504=CARTESIAN_POINT('Ctrl Pts',(-22.2788522684653,14.1256565202968,
131.331061047938)) ;
#119505=CARTESIAN_POINT('Ctrl Pts',(-22.2205501163383,14.2929703983871,
131.127802439473)) ;
#119506=CARTESIAN_POINT('Ctrl Pts',(-22.1496885418691,14.3994043107509,
130.887536859964)) ;
#119507=CARTESIAN_POINT('Ctrl Pts',(-22.0730335167053,14.4351253202345,
130.630552854878)) ;
#119508=CARTESIAN_POINT('Ctrl Pts',(-21.996345530088,14.3988243968592,130.373443099592)) ;
#119509=CARTESIAN_POINT('Ctrl Pts',(-21.9257344155299,14.2923293351463,
130.134007145371)) ;
#119510=CARTESIAN_POINT('Ctrl Pts',(-21.867354018945,14.1241731231248,129.930419720698)) ;
#119511=CARTESIAN_POINT('Ctrl Pts',(-21.825689326131,13.9051614017352,129.775535782279)) ;
#119512=CARTESIAN_POINT('Ctrl Pts',(-21.8047754075895,13.6518311474299,
129.681317036466)) ;
#119513=CARTESIAN_POINT('Ctrl Pts',(-21.806690488997,13.3824708815404,129.653826199804)) ;
#119514=CARTESIAN_POINT('Ctrl Pts',(-21.8320892264618,13.1154253424266,
129.694864183361)) ;
#119515=CARTESIAN_POINT('Ctrl Pts',(-21.8799125491881,12.870532663978,129.801417493247)) ;
#119516=CARTESIAN_POINT('Ctrl Pts',(-21.9473301818534,12.6655370974074,
129.965254569421)) ;
#119517=CARTESIAN_POINT('Ctrl Pts',(-22.0303478152381,12.5146112418993,
130.174643252011)) ;
#119518=CARTESIAN_POINT('Ctrl Pts',(-22.1237974779465,12.4289101941166,
130.414481127805)) ;
#119519=CARTESIAN_POINT('Ctrl Pts',(-22.22120291299,12.414189670065,130.666024010192)) ;
#119520=CARTESIAN_POINT('Ctrl Pts',(-22.3177472586075,12.4724108557129,
130.914690052658)) ;
#119521=CARTESIAN_POINT('Ctrl Pts',(-22.4050664943516,12.5978142142,131.13683154333)) ;
#119522=CARTESIAN_POINT('Ctrl Pts',(-22.4793620392904,12.7826551877608,
131.320734373742)) ;
#119523=CARTESIAN_POINT('Ctrl Pts',(-22.5354278081203,13.0133814811485,
131.451404804388)) ;
#119524=CARTESIAN_POINT('Ctrl Pts',(-22.5701066532852,13.2742168699271,
131.5194991142)) ;
#119525=CARTESIAN_POINT('Ctrl Pts',(-22.5814078746339,13.5450314863386,
131.519394277287)) ;
#119526=CARTESIAN_POINT('Ctrl Pts',(-22.5694715329342,13.8067211996107,
131.451455874011)) ;
#119527=CARTESIAN_POINT('Ctrl Pts',(-22.5358417510326,14.041251301363,131.320111797343)) ;
#119528=CARTESIAN_POINT('Ctrl Pts',(-22.4835621993957,14.2318697191873,
131.134238872589)) ;
#119529=CARTESIAN_POINT('Ctrl Pts',(-22.4169548508548,14.3645253073145,
130.906437235613)) ;
#119530=CARTESIAN_POINT('Ctrl Pts',(-22.3422630485774,14.4291513748126,
130.655264086382)) ;
#119531=CARTESIAN_POINT('Ctrl Pts',(-22.2646712406155,14.4223448235858,
130.395455894871)) ;
#119532=CARTESIAN_POINT('Ctrl Pts',(-22.1906962386533,14.3433928337176,
130.146147002651)) ;
#119533=CARTESIAN_POINT('Ctrl Pts',(-22.126864261988,14.1993297551337,129.926664992728)) ;
#119534=CARTESIAN_POINT('Ctrl Pts',(-22.0777784963834,13.9988090626419,
129.750073791715)) ;
#119535=CARTESIAN_POINT('Ctrl Pts',(-22.0481534201508,13.7578101990109,
129.630462242444)) ;
#119536=CARTESIAN_POINT('Ctrl Pts',(-22.04065787053,13.4916491318397,129.575336826241)) ;
#119537=CARTESIAN_POINT('Ctrl Pts',(-22.0565398005928,13.2223243547225,
129.588728872974)) ;
#119538=CARTESIAN_POINT('Ctrl Pts',(-22.0955535823169,12.9657468918016,
129.669485051564)) ;
#119539=CARTESIAN_POINT('Ctrl Pts',(-22.1554227877338,12.7429296801426,
129.811288655846)) ;
#119540=CARTESIAN_POINT('Ctrl Pts',(-22.2326074989573,12.5685157240841,
130.003665981222)) ;
#119541=CARTESIAN_POINT('Ctrl Pts',(-22.3229046634719,12.4549912685616,
130.234168931631)) ;
#119542=CARTESIAN_POINT('Ctrl Pts',(-22.4191582779013,12.4115665135432,
130.482391282104)) ;
#119543=CARTESIAN_POINT('Ctrl Pts',(-22.5165199381588,12.4399153694957,
130.733695829769)) ;
#119544=CARTESIAN_POINT('Ctrl Pts',(-22.6085788719043,12.539266271838,130.969408347194)) ;
#119545=CARTESIAN_POINT('Ctrl Pts',(-22.6888376062549,12.7015765311082,
131.170776121239)) ;
#119546=CARTESIAN_POINT('Ctrl Pts',(-22.7526224840521,12.9151235328842,
131.32405474122)) ;
#119547=CARTESIAN_POINT('Ctrl Pts',(-22.7963093376422,13.1655123669942,
131.418544660933)) ;
#119548=CARTESIAN_POINT('Ctrl Pts',(-22.8172555834161,13.4357073087156,
131.44644515501)) ;
#119549=CARTESIAN_POINT('Ctrl Pts',(-22.8145947811972,13.7027427371582,
131.405664342584)) ;
#119550=CARTESIAN_POINT('Ctrl Pts',(-22.7895245214645,13.9504288241065,
131.299348303374)) ;
#119551=CARTESIAN_POINT('Ctrl Pts',(-22.7442911744941,14.1608970997243,
131.134046242548)) ;
#119552=CARTESIAN_POINT('Ctrl Pts',(-22.683035539054,14.3182076621176,130.921983637529)) ;
#119553=CARTESIAN_POINT('Ctrl Pts',(-22.6108042807872,14.4114239711584,
130.677847491563)) ;
#119554=CARTESIAN_POINT('Ctrl Pts',(-22.5336431840969,14.4338711426872,
130.41936450385)) ;
#119555=CARTESIAN_POINT('Ctrl Pts',(-22.4574802588175,14.3839736341,130.163713489423)) ;
#119556=CARTESIAN_POINT('Ctrl Pts',(-22.3887045426789,14.2649033849915,
129.929628525721)) ;
#119557=CARTESIAN_POINT('Ctrl Pts',(-22.3331731185059,14.0862373314476,
129.734363423515)) ;
#119558=CARTESIAN_POINT('Ctrl Pts',(-22.2951785325991,13.8593709680806,
129.59019900343)) ;
#119559=CARTESIAN_POINT('Ctrl Pts',(-22.278460128517,13.6016402175067,129.508253119268)) ;
#119560=CARTESIAN_POINT('Ctrl Pts',(-22.2848323533062,13.3309241263673,
129.493731727179)) ;
#119561=CARTESIAN_POINT('Ctrl Pts',(-22.3145834910505,13.0670233439019,
129.547533253071)) ;
#119562=CARTESIAN_POINT('Ctrl Pts',(-22.3662673822252,12.8286261810775,
129.665410937609)) ;
#119563=CARTESIAN_POINT('Ctrl Pts',(-22.4370692147307,12.6324569131355,
129.839080633123)) ;
#119564=CARTESIAN_POINT('Ctrl Pts',(-22.5225167986892,12.4932133607205,
130.055556624894)) ;
#119565=CARTESIAN_POINT('Ctrl Pts',(-22.6169281495309,12.4206918149119,
130.298317972927)) ;
#119566=CARTESIAN_POINT('Ctrl Pts',(-22.7149280217507,12.4196226732146,
130.551436865858)) ;
#119567=CARTESIAN_POINT('Ctrl Pts',(-22.8099912203035,12.4910154919702,
130.795922304285)) ;
#119568=CARTESIAN_POINT('Ctrl Pts',(-22.8953670162546,12.6283739750249,
131.012318396671)) ;
#119569=CARTESIAN_POINT('Ctrl Pts',(-22.9667570176051,12.8237069279728,
131.18763100803)) ;
#119570=CARTESIAN_POINT('Ctrl Pts',(-23.0189001383716,13.0616748954868,
131.306816569627)) ;
#119571=CARTESIAN_POINT('Ctrl Pts',(-23.0490556418348,13.3240382203917,
131.361942294149)) ;
#119572=CARTESIAN_POINT('Ctrl Pts',(-23.0560738557443,13.5952493651547,
131.349257476289)) ;
#119573=CARTESIAN_POINT('Ctrl Pts',(-23.0397586164554,13.8544594901405,
131.268360250981)) ;
#119574=CARTESIAN_POINT('Ctrl Pts',(-23.0022335507907,14.0816539575776,
131.12563509274)) ;
#119575=CARTESIAN_POINT('Ctrl Pts',(-22.9471547098177,14.2612879852104,
130.931743906549)) ;
#119576=CARTESIAN_POINT('Ctrl Pts',(-22.8787472340573,14.3817634357603,
130.698787045464)) ;
#119577=CARTESIAN_POINT('Ctrl Pts',(-22.8026065314009,14.4336477356996,
130.443163556008)) ;
#119578=CARTESIAN_POINT('Ctrl Pts',(-22.7250276410476,14.4124733910525,
130.183293296263)) ;
#119579=CARTESIAN_POINT('Ctrl Pts',(-22.6531551209299,14.3214777368465,
129.940454108184)) ;
#119580=CARTESIAN_POINT('Ctrl Pts',(-22.5912986814561,14.1652192493521,
129.726511736899)) ;
#119581=CARTESIAN_POINT('Ctrl Pts',(-22.5456891986183,13.9555650304119,
129.560097274171)) ;
#119582=CARTESIAN_POINT('Ctrl Pts',(-22.5201337366245,13.7095599623908,
129.452485156075)) ;
#119583=CARTESIAN_POINT('Ctrl Pts',(-22.5169344827566,13.4405995094296,
129.409863314084)) ;
#119584=CARTESIAN_POINT('Ctrl Pts',(-22.5374018331414,13.1715077447804,
129.436518432893)) ;
#119585=CARTESIAN_POINT('Ctrl Pts',(-22.5802715414608,12.9214880554527,
129.528771184389)) ;
#119586=CARTESIAN_POINT('Ctrl Pts',(-22.6440034901965,12.7055052925361,
129.681687195527)) ;
#119587=CARTESIAN_POINT('Ctrl Pts',(-22.7237755441732,12.5425196617187,
129.881722442674)) ;
#119588=CARTESIAN_POINT('Ctrl Pts',(-22.8153026656991,12.4416160239473,
130.115984676027)) ;
#119589=CARTESIAN_POINT('Ctrl Pts',(-22.9132249157816,12.4112449647392,
130.368717480688)) ;
#119590=CARTESIAN_POINT('Ctrl Pts',(-23.0098513980588,12.4537097217899,
130.617922318624)) ;
#119591=CARTESIAN_POINT('Ctrl Pts',(-23.0997589861042,12.5652232795711,
130.847498105072)) ;
#119592=CARTESIAN_POINT('Ctrl Pts',(-23.177257630143,12.7379440224027,131.040830428269)) ;
#119593=CARTESIAN_POINT('Ctrl Pts',(-23.237708098821,12.960397453185,131.184248159784)) ;
#119594=CARTESIAN_POINT('Ctrl Pts',(-23.2771410099792,13.2156634821883,
131.266326678235)) ;
#119595=CARTESIAN_POINT('Ctrl Pts',(-23.2936412005976,13.4857933764674,
131.281407977912)) ;
#119596=CARTESIAN_POINT('Ctrl Pts',(-23.2866428376385,13.7522946438347,
131.227738286367)) ;
#119597=CARTESIAN_POINT('Ctrl Pts',(-23.2573503270286,13.9943544460531,
131.109028172531)) ;
#119598=CARTESIAN_POINT('Ctrl Pts',(-23.2090388110104,14.1947046175958,
130.934934734007)) ;
#119599=CARTESIAN_POINT('Ctrl Pts',(-23.1449422933138,14.3414529387325,
130.714386929577)) ;
#119600=CARTESIAN_POINT('Ctrl Pts',(-23.071480933739,14.4211243068953,130.466760593943)) ;
#119601=CARTESIAN_POINT('Ctrl Pts',(-22.9941233562367,14.4300014348132,
130.207726168655)) ;
#119602=CARTESIAN_POINT('Ctrl Pts',(-22.9188030207876,14.3664765738552,
129.954493538436)) ;
#119603=CARTESIAN_POINT('Ctrl Pts',(-22.8522466727456,14.235605243378,129.726980037117)) ;
#119604=CARTESIAN_POINT('Ctrl Pts',(-22.7995686386573,14.0463420855303,
129.539948951854)) ;
#119605=CARTESIAN_POINT('Ctrl Pts',(-22.7654773132939,13.8127312117544,
129.407267248046)) ;
#119606=CARTESIAN_POINT('Ctrl Pts',(-22.7529636647336,13.5514861581268,
129.337641508112)) ;
#119607=CARTESIAN_POINT('Ctrl Pts',(-22.7638097876353,13.2797431877816,
129.336093527345)) ;
#119608=CARTESIAN_POINT('Ctrl Pts',(-22.7978310708524,13.0196141695931,
129.402416181262)) ;
#119609=CARTESIAN_POINT('Ctrl Pts',(-22.8534471757938,12.7876902143184,
129.531733398873)) ;
#119610=CARTESIAN_POINT('Ctrl Pts',(-22.9273302721824,12.6015317639528,
129.714440609281)) ;
#119611=CARTESIAN_POINT('Ctrl Pts',(-23.0148543072416,12.4742597537388,
129.937016753495)) ;
#119612=CARTESIAN_POINT('Ctrl Pts',(-23.1106134225891,12.4148459760243,
130.183624177554)) ;
#119613=CARTESIAN_POINT('Ctrl Pts',(-23.2084459565588,12.4277168050886,
130.43627690467)) ;
#119614=CARTESIAN_POINT('Ctrl Pts',(-23.3019874032968,12.5119511552026,
130.676406889101)) ;
#119615=CARTESIAN_POINT('Ctrl Pts',(-23.3852438450899,12.6612550924709,
130.886523809409)) ;
#119616=CARTESIAN_POINT('Ctrl Pts',(-23.4531589894234,12.8654797795072,
131.051765953329)) ;
#119617=CARTESIAN_POINT('Ctrl Pts',(-23.5013158293354,13.1088715817203,
131.159398237107)) ;
#119618=CARTESIAN_POINT('Ctrl Pts',(-23.5273348323144,13.3752798847283,
131.202282354274)) ;
#119619=CARTESIAN_POINT('Ctrl Pts',(-23.5298343688226,13.6458119983222,
131.17637609497)) ;
#119620=CARTESIAN_POINT('Ctrl Pts',(-23.5094171878235,13.899465813918,131.083638360223)) ;
#119621=CARTESIAN_POINT('Ctrl Pts',(-23.4682977024105,14.1192748992269,
130.930392419709)) ;
#119622=CARTESIAN_POINT('Ctrl Pts',(-23.410117737834,14.2891803091472,130.727307342406)) ;
#119623=CARTESIAN_POINT('Ctrl Pts',(-23.3398467906228,14.3970324953894,
130.488926001134)) ;
#119624=CARTESIAN_POINT('Ctrl Pts',(-23.2631341283584,14.4351164741298,
130.231697294466)) ;
#119625=CARTESIAN_POINT('Ctrl Pts',(-23.1864219100301,14.4010787684845,
129.974554635366)) ;
#119626=CARTESIAN_POINT('Ctrl Pts',(-23.1151468899051,14.2958209248288,
129.732983843262)) ;
#119627=CARTESIAN_POINT('Ctrl Pts',(-23.0566124154398,14.129652176779,129.52906406716)) ;
#119628=CARTESIAN_POINT('Ctrl Pts',(-23.0144082905123,13.912176140122,129.372634918644)) ;
#119629=CARTESIAN_POINT('Ctrl Pts',(-22.9928657656156,13.6594303550192,
129.276558713849)) ;
#119630=CARTESIAN_POINT('Ctrl Pts',(-22.9940381415481,13.3906473187371,
129.246946981342)) ;
#119631=CARTESIAN_POINT('Ctrl Pts',(-23.0190161616895,13.1215485791247,
129.286535008088)) ;
#119632=CARTESIAN_POINT('Ctrl Pts',(-23.0659504345269,12.877499502744,129.390721793247)) ;
#119633=CARTESIAN_POINT('Ctrl Pts',(-23.1331268462785,12.6702279580221,
129.553707509289)) ;
#119634=CARTESIAN_POINT('Ctrl Pts',(-23.2154479176507,12.5183910541011,
129.761204124045)) ;
#119635=CARTESIAN_POINT('Ctrl Pts',(-23.3086829803135,12.4302683160369,
130.000401656271)) ;
#119636=CARTESIAN_POINT('Ctrl Pts',(-23.4067522708612,12.4138255854832,
130.253644887084)) ;
#119637=CARTESIAN_POINT('Ctrl Pts',(-23.5022295536224,12.4692849661908,
130.499614004423)) ;
#119638=CARTESIAN_POINT('Ctrl Pts',(-23.590497552906,12.5930868189149,130.724316427498)) ;
#119639=CARTESIAN_POINT('Ctrl Pts',(-23.6653857036061,12.7771359268665,
130.909865160465)) ;
#119640=CARTESIAN_POINT('Ctrl Pts',(-23.7218153355874,13.0059649491312,
131.041714048845)) ;
#119641=CARTESIAN_POINT('Ctrl Pts',(-23.7571901785065,13.2661471501604,
131.111841913724)) ;
#119642=CARTESIAN_POINT('Ctrl Pts',(-23.7692103176648,13.536990610461,131.113832196985)) ;
#119643=CARTESIAN_POINT('Ctrl Pts',(-23.7578885911495,13.7997448803438,
131.04761545879)) ;
#119644=CARTESIAN_POINT('Ctrl Pts',(-23.7248950980706,14.0350783455638,
130.918172841181)) ;
#119645=CARTESIAN_POINT('Ctrl Pts',(-23.6728301485584,14.2276700912271,
130.73279573439)) ;
#119646=CARTESIAN_POINT('Ctrl Pts',(-23.607190849765,14.3610390987627,130.508134028413)) ;
#119647=CARTESIAN_POINT('Ctrl Pts',(-23.5320583070199,14.4285213562849,
130.255391484949)) ;
#119648=CARTESIAN_POINT('Ctrl Pts',(-23.4546158086494,14.4233691506753,
129.996090560874)) ;
#119649=CARTESIAN_POINT('Ctrl Pts',(-23.380643189452,14.3469900608794,129.746892873934)) ;
#119650=CARTESIAN_POINT('Ctrl Pts',(-23.3160087352734,14.2034039826352,
129.524810838225)) ;
#119651=CARTESIAN_POINT('Ctrl Pts',(-23.2668172562997,14.0056848042437,
129.348164408924)) ;
#119652=CARTESIAN_POINT('Ctrl Pts',(-23.2364502982385,13.7644935379873,
129.226215459464)) ;
#119653=CARTESIAN_POINT('Ctrl Pts',(-23.2282984715539,13.5002463759362,
129.169368760998)) ;
#119654=CARTESIAN_POINT('Ctrl Pts',(-23.24371050422,13.2284058241885,129.181082860346)) ;
#119655=CARTESIAN_POINT('Ctrl Pts',(-23.2817138310726,12.9739037522761,
129.259247094097)) ;
#119656=CARTESIAN_POINT('Ctrl Pts',(-23.3412738291248,12.7484704180283,
129.399951986227)) ;
#119657=CARTESIAN_POINT('Ctrl Pts',(-23.4177990674146,12.5731123279677,
129.590515150982)) ;
#119658=CARTESIAN_POINT('Ctrl Pts',(-23.5078548816841,12.45735908031,129.820279560396)) ;
#119659=CARTESIAN_POINT('Ctrl Pts',(-23.604095848768,12.4118025440313,130.068434118801)) ;
#119660=CARTESIAN_POINT('Ctrl Pts',(-23.701547171813,12.4381298273325,130.319990066657)) ;
#119661=CARTESIAN_POINT('Ctrl Pts',(-23.7936910641617,12.5352056627263,
130.556017518531)) ;
#119662=CARTESIAN_POINT('Ctrl Pts',(-23.8745884919989,12.696300610242,130.759150487779)) ;
#119663=CARTESIAN_POINT('Ctrl Pts',(-23.9388625765618,12.9082756113126,
130.913902309013)) ;
#119664=CARTESIAN_POINT('Ctrl Pts',(-23.983317014121,13.1596325323724,131.010413905855)) ;
#119665=CARTESIAN_POINT('Ctrl Pts',(-24.0046631549015,13.4259468835544,
131.039934337967)) ;
#119666=CARTESIAN_POINT('Ctrl Pts',(-24.0028248548074,13.6953761011822,
131.001297665737)) ;
#119667=CARTESIAN_POINT('Ctrl Pts',(-23.9783213573141,13.9437170252716,
130.896659476004)) ;
#119668=CARTESIAN_POINT('Ctrl Pts',(-23.93357174813,14.155711083142,130.73273190048)) ;
#119669=CARTESIAN_POINT('Ctrl Pts',(-23.8728119878527,14.3144000216169,
130.522179990839)) ;
#119670=CARTESIAN_POINT('Ctrl Pts',(-23.8008509799533,14.4096307873655,
130.278840330333)) ;
#119671=CARTESIAN_POINT('Ctrl Pts',(-23.7237246168415,14.4343455413494,
130.020451918313)) ;
#119672=CARTESIAN_POINT('Ctrl Pts',(-23.6471274329311,14.3860725328483,
129.763386450898)) ;
#119673=CARTESIAN_POINT('Ctrl Pts',(-23.5784483932488,14.2695097224109,
129.529774563967)) ;
#119674=CARTESIAN_POINT('Ctrl Pts',(-23.5222414219864,14.0917907818256,
129.332403324397)) ;
#119675=CARTESIAN_POINT('Ctrl Pts',(-23.4838194360288,13.8666927390169,
129.187092868066)) ;
#119676=CARTESIAN_POINT('Ctrl Pts',(-23.4664016523007,13.6093228948058,
129.103058814387)) ;
#119677=CARTESIAN_POINT('Ctrl Pts',(-23.4720979067043,13.3388432041032,
129.086581594088)) ;
#119678=CARTESIAN_POINT('Ctrl Pts',(-23.5012168114343,13.0740474373603,
129.138484307447)) ;
#119679=CARTESIAN_POINT('Ctrl Pts',(-23.5524662673914,12.8343946472962,
129.25503692304)) ;
#119680=CARTESIAN_POINT('Ctrl Pts',(-23.6224253524384,12.6378259475901,
129.4264139265)) ;
#119681=CARTESIAN_POINT('Ctrl Pts',(-23.7075121796353,12.4964630119009,
129.641818563098)) ;
#119682=CARTESIAN_POINT('Ctrl Pts',(-23.8019975756317,12.421725405798,129.884708515321)) ;
#119683=CARTESIAN_POINT('Ctrl Pts',(-23.8998895978672,12.4187226198539,
130.137544774975)) ;
#119684=CARTESIAN_POINT('Ctrl Pts',(-23.9948139084966,12.4875916518615,
130.381743115251)) ;
#119685=CARTESIAN_POINT('Ctrl Pts',(-24.0808838147119,12.6235712310503,
130.600036971764)) ;
#119686=CARTESIAN_POINT('Ctrl Pts',(-24.1524928045672,12.8167007524725,
130.776115139759)) ;
#119687=CARTESIAN_POINT('Ctrl Pts',(-24.2053648747095,13.053470084932,130.897425249101)) ;
#119688=CARTESIAN_POINT('Ctrl Pts',(-24.2363346414086,13.3166529719994,
130.954767098214)) ;
#119689=CARTESIAN_POINT('Ctrl Pts',(-24.2439518827779,13.5871781568045,
130.943922486326)) ;
#119690=CARTESIAN_POINT('Ctrl Pts',(-24.2284589955264,13.8461110281262,
130.865554669598)) ;
#119691=CARTESIAN_POINT('Ctrl Pts',(-24.1914691846138,14.0754123142472,
130.724278834602)) ;
#119692=CARTESIAN_POINT('Ctrl Pts',(-24.1367058007406,14.2569965366052,
130.531234806345)) ;
#119693=CARTESIAN_POINT('Ctrl Pts',(-24.0686015337967,14.3792169308405,
130.299169849526)) ;
#119694=CARTESIAN_POINT('Ctrl Pts',(-23.9928202726193,14.4330645765252,
130.044692226851)) ;
#119695=CARTESIAN_POINT('Ctrl Pts',(-23.9152030610562,14.4142942137405,
129.784717394)) ;
#119696=CARTESIAN_POINT('Ctrl Pts',(-23.8427985126538,14.3249818640555,
129.540193183357)) ;
#119697=CARTESIAN_POINT('Ctrl Pts',(-23.7805649806732,14.1700409450456,
129.325118482017)) ;
#119698=CARTESIAN_POINT('Ctrl Pts',(-23.7346417673261,13.9629928904563,
129.157974141327)) ;
#119699=CARTESIAN_POINT('Ctrl Pts',(-23.7083156172197,13.716497244272,129.04792282307)) ;
#119700=CARTESIAN_POINT('Ctrl Pts',(-23.7044893109021,13.449382384683,129.003661141323)) ;
#119701=CARTESIAN_POINT('Ctrl Pts',(-23.724174778289,13.179466012535,129.027965195106)) ;
#119702=CARTESIAN_POINT('Ctrl Pts',(-23.7667235870963,12.9274139548691,
129.119104726136)) ;
#119703=CARTESIAN_POINT('Ctrl Pts',(-23.8295759439689,12.7115777199899,
129.269649618492)) ;
#119704=CARTESIAN_POINT('Ctrl Pts',(-23.9089257388214,12.5463884339408,
129.468420668235)) ;
#119705=CARTESIAN_POINT('Ctrl Pts',(-24.0009772282109,12.4431786927595,
129.703950653175)) ;
#119706=CARTESIAN_POINT('Ctrl Pts',(-24.0977509267161,12.4112124576001,
129.953697636734)) ;
#119707=CARTESIAN_POINT('Ctrl Pts',(-24.1948656324168,12.4513454606681,
130.20419806984)) ;
#119708=CARTESIAN_POINT('Ctrl Pts',(-24.285028808609,12.5610016888449,130.434530136024)) ;
#119709=CARTESIAN_POINT('Ctrl Pts',(-24.3630579432247,12.7322315301459,
130.629374967685)) ;
#119710=CARTESIAN_POINT('Ctrl Pts',(-24.4240719874066,12.9536821902703,
130.774419040633)) ;
#119711=CARTESIAN_POINT('Ctrl Pts',(-24.4640634099182,13.2077095547012,
130.858196825809)) ;
#119712=CARTESIAN_POINT('Ctrl Pts',(-24.4812915975361,13.4778389937593,
130.875385354315)) ;
#119713=CARTESIAN_POINT('Ctrl Pts',(-24.4749348184018,13.7447250212435,
130.823586297997)) ;
#119714=CARTESIAN_POINT('Ctrl Pts',(-24.4464281767638,13.9871379324524,
130.707276700175)) ;
#119715=CARTESIAN_POINT('Ctrl Pts',(-24.3982867625321,14.1900736683291,
130.53346338122)) ;
#119716=CARTESIAN_POINT('Ctrl Pts',(-24.3351669079392,14.3373317705726,
130.316081854246)) ;
#119717=CARTESIAN_POINT('Ctrl Pts',(-24.2614650136263,14.4199335314477,
130.067526586258)) ;
#119718=CARTESIAN_POINT('Ctrl Pts',(-24.1841440002385,14.4307823932299,
129.808614897003)) ;
#119719=CARTESIAN_POINT('Ctrl Pts',(-24.1084828214291,14.3690285346023,
129.554295669333)) ;
#119720=CARTESIAN_POINT('Ctrl Pts',(-24.041888647281,14.2404409958973,129.326810148506)) ;
#119721=CARTESIAN_POINT('Ctrl Pts',(-23.9886944579791,14.0528076235366,
129.138264979465)) ;
#119722=CARTESIAN_POINT('Ctrl Pts',(-23.953964486593,13.8202655346865,129.003710925122)) ;
#119723=CARTESIAN_POINT('Ctrl Pts',(-23.9407661646502,13.5584444943241,
128.931945154736)) ;
#119724=CARTESIAN_POINT('Ctrl Pts',(-23.951014218669,13.2871050604655,128.928700531277)) ;
#119725=CARTESIAN_POINT('Ctrl Pts',(-23.9842710836601,13.0271136592546,
128.99288013018)) ;
#119726=CARTESIAN_POINT('Ctrl Pts',(-24.0393399443066,12.7938647968009,
129.120566173473)) ;
#119727=CARTESIAN_POINT('Ctrl Pts',(-24.1126551456015,12.6063348260336,
129.301653620629)) ;
#119728=CARTESIAN_POINT('Ctrl Pts',(-24.1999951112264,12.4770287945195,
129.523636975406)) ;
#119729=CARTESIAN_POINT('Ctrl Pts',(-24.2953179840485,12.4155889171301,
129.769068705113)) ;
#119730=CARTESIAN_POINT('Ctrl Pts',(-24.3936269874943,12.4264045775595,
130.022957981845)) ;
#119731=CARTESIAN_POINT('Ctrl Pts',(-24.487039800036,12.5084012682064,130.262834505256)) ;
#119732=CARTESIAN_POINT('Ctrl Pts',(-24.5708433676683,12.6562045678091,
130.474478189188)) ;
#119733=CARTESIAN_POINT('Ctrl Pts',(-24.6390689439144,12.8582528163381,
130.640744689845)) ;
#119734=CARTESIAN_POINT('Ctrl Pts',(-24.688186273424,13.1022480435351,130.75096865955)) ;
#119735=CARTESIAN_POINT('Ctrl Pts',(-24.7147148491463,13.3685511401161,
130.795319580132)) ;
#119736=CARTESIAN_POINT('Ctrl Pts',(-24.7178825838308,13.6374690489365,
130.771584220973)) ;
#119737=CARTESIAN_POINT('Ctrl Pts',(-24.6981008820832,13.8926337439443,
130.680605414583)) ;
#119738=CARTESIAN_POINT('Ctrl Pts',(-24.6575485405634,14.1134973909665,
130.529040703755)) ;
#119739=CARTESIAN_POINT('Ctrl Pts',(-24.5996419056856,14.2854804526752,
130.326666926777)) ;
#119740=CARTESIAN_POINT('Ctrl Pts',(-24.529617378917,14.3949169679371,130.08901030832)) ;
#119741=CARTESIAN_POINT('Ctrl Pts',(-24.4533294260154,14.4350950474159,
129.833165182374)) ;
#119742=CARTESIAN_POINT('Ctrl Pts',(-24.3760965657258,14.4027523558799,
129.574300858813)) ;
#119743=CARTESIAN_POINT('Ctrl Pts',(-24.3051605815314,14.3004224284984,
129.334015107818)) ;
#119744=CARTESIAN_POINT('Ctrl Pts',(-24.2456558829535,14.1345848186711,
129.126962774676)) ;
#119745=CARTESIAN_POINT('Ctrl Pts',(-24.203144223906,13.9188292649382,128.969748265091)) ;
#119746=CARTESIAN_POINT('Ctrl Pts',(-24.1809374546638,13.6668968263447,
128.87172937497)) ;
#119747=CARTESIAN_POINT('Ctrl Pts',(-24.1815007016074,13.3982258139503,
128.840326111729)) ;
#119748=CARTESIAN_POINT('Ctrl Pts',(-24.2056308452266,13.1299459979309,
128.877587112846)) ;
#119749=CARTESIAN_POINT('Ctrl Pts',(-24.2521574317291,12.8837060255956,
128.98041042931)) ;
#119750=CARTESIAN_POINT('Ctrl Pts',(-24.3187472777364,12.6755091265604,
129.141737299498)) ;
#119751=CARTESIAN_POINT('Ctrl Pts',(-24.400840597816,12.5215778534682,129.348502615957)) ;
#119752=CARTESIAN_POINT('Ctrl Pts',(-24.4940411132764,12.4317802187368,
129.587545619902)) ;
#119753=CARTESIAN_POINT('Ctrl Pts',(-24.5912174648574,12.4131805115513,
129.838470614325)) ;
#119754=CARTESIAN_POINT('Ctrl Pts',(-24.6876108574417,12.4668842631246,
130.086844676273)) ;
#119755=CARTESIAN_POINT('Ctrl Pts',(-24.7757687439987,12.5884450381112,
130.311379023635)) ;
#119756=CARTESIAN_POINT('Ctrl Pts',(-24.8513379924622,12.7713420936062,
130.498823295008)) ;
#119757=CARTESIAN_POINT('Ctrl Pts',(-24.9082742295121,12.9988617969997,
130.63219011284)) ;
#119758=CARTESIAN_POINT('Ctrl Pts',(-24.94437712461,13.2594913097142,130.704313382591)) ;
#119759=CARTESIAN_POINT('Ctrl Pts',(-24.9569420258268,13.5289133142041,
130.708064597244)) ;
#119760=CARTESIAN_POINT('Ctrl Pts',(-24.9463665896322,13.7920447587741,
130.644049270301)) ;
#119761=CARTESIAN_POINT('Ctrl Pts',(-24.913933421227,14.028682332542,130.516205209765)) ;
#119762=CARTESIAN_POINT('Ctrl Pts',(-24.8624450520878,14.2226477073875,
130.332553173407)) ;
#119763=CARTESIAN_POINT('Ctrl Pts',(-24.7969465973085,14.358128004445,130.108205057348)) ;
#119764=CARTESIAN_POINT('Ctrl Pts',(-24.722353105465,14.427517223623,129.857199608081)) ;
#119765=CARTESIAN_POINT('Ctrl Pts',(-24.644295649574,14.4244373383238,129.595839584828)) ;
#119766=CARTESIAN_POINT('Ctrl Pts',(-24.5705593446945,14.3501368241958,
129.347511571609)) ;
#119767=CARTESIAN_POINT('Ctrl Pts',(-24.5056565645644,14.2089998029508,
129.124719851443)) ;
#119768=CARTESIAN_POINT('Ctrl Pts',(-24.4557713790485,14.0121251226583,
128.94593584056)) ;
#119769=CARTESIAN_POINT('Ctrl Pts',(-24.4247960653296,13.7718247542597,
128.822203002167)) ;
#119770=CARTESIAN_POINT('Ctrl Pts',(-24.416027718643,13.5078187050463,128.763529045233)) ;
#119771=CARTESIAN_POINT('Ctrl Pts',(-24.4306046417983,13.2372789861246,
128.772981600375)) ;
#119772=CARTESIAN_POINT('Ctrl Pts',(-24.4681460256884,12.9804327366812,
128.849585251481)) ;
#119773=CARTESIAN_POINT('Ctrl Pts',(-24.5272076352715,12.7540238900059,
128.988844175822)) ;
#119774=CARTESIAN_POINT('Ctrl Pts',(-24.6031699054307,12.577462748724,129.177818082868)) ;
#119775=CARTESIAN_POINT('Ctrl Pts',(-24.6927251102051,12.4598742961996,
129.406189054556)) ;
#119776=CARTESIAN_POINT('Ctrl Pts',(-24.7892829387905,12.4120040777539,
129.655120321832)) ;
#119777=CARTESIAN_POINT('Ctrl Pts',(-24.8867386589966,12.4365719304023,
129.906705661731)) ;
#119778=CARTESIAN_POINT('Ctrl Pts',(-24.978747317987,12.5311793642618,130.142476274929)) ;
#119779=CARTESIAN_POINT('Ctrl Pts',(-25.060355481887,12.6910252925006,130.347571894772)) ;
#119780=CARTESIAN_POINT('Ctrl Pts',(-25.1249799734368,12.901554601713,130.503394346182)) ;
#119781=CARTESIAN_POINT('Ctrl Pts',(-25.1699675301259,13.1503193803292,
130.601673711029)) ;
#119782=CARTESIAN_POINT('Ctrl Pts',(-25.1922305047665,13.4198238179189,
130.633438387821)) ;
#119783=CARTESIAN_POINT('Ctrl Pts',(-25.1910108110703,13.6867201864748,
130.596962968401)) ;
#119784=CARTESIAN_POINT('Ctrl Pts',(-25.167052916905,13.9376559874792,130.493686388418)) ;
#119785=CARTESIAN_POINT('Ctrl Pts',(-25.1228803335291,14.1502428596578,
130.331538878298)) ;
#119786=CARTESIAN_POINT('Ctrl Pts',(-25.0624593309472,14.3108380657866,
130.121931628785)) ;
#119787=CARTESIAN_POINT('Ctrl Pts',(-24.9907465662706,14.4079445311136,
129.879330709918)) ;
#119788=CARTESIAN_POINT('Ctrl Pts',(-24.9136043625224,14.4345276707165,
129.620858009147)) ;
#119789=CARTESIAN_POINT('Ctrl Pts',(-24.8374005548157,14.3888298809399,
129.365172106487)) ;
#119790=CARTESIAN_POINT('Ctrl Pts',(-24.7680465549556,14.2738284878411,
129.1294178052)) ;
#119791=CARTESIAN_POINT('Ctrl Pts',(-24.7114675854268,14.0978368640531,
128.931000104012)) ;
#119792=CARTESIAN_POINT('Ctrl Pts',(-24.6724005531575,13.8735407720446,
128.783743944974)) ;
#119793=CARTESIAN_POINT('Ctrl Pts',(-24.6543698495407,13.616875079998,128.697930467751)) ;
#119794=CARTESIAN_POINT('Ctrl Pts',(-24.659403085665,13.3465064329097,128.679514282414)) ;
#119795=CARTESIAN_POINT('Ctrl Pts',(-24.6878260612952,13.0815408414728,
128.729420324657)) ;
#119796=CARTESIAN_POINT('Ctrl Pts',(-24.7384611274853,12.8409647311381,
128.844181431209)) ;
#119797=CARTESIAN_POINT('Ctrl Pts',(-24.8078392099398,12.642864050615,129.013879190485)) ;
#119798=CARTESIAN_POINT('Ctrl Pts',(-24.8932722991771,12.498964683589,129.230041309728)) ;
#119799=CARTESIAN_POINT('Ctrl Pts',(-24.9867207169967,12.4231077011215,
129.47021048062)) ;
#119800=CARTESIAN_POINT('Ctrl Pts',(-25.0849839469443,12.4177381472718,
129.723995502206)) ;
#119801=CARTESIAN_POINT('Ctrl Pts',(-25.180011685858,12.4847095066073,129.968519607844)) ;
#119802=CARTESIAN_POINT('Ctrl Pts',(-25.2665150261769,12.6190667593984,
130.188038371959)) ;
#119803=CARTESIAN_POINT('Ctrl Pts',(-25.338527272186,12.8107471033722,130.365312618294)) ;
#119804=CARTESIAN_POINT('Ctrl Pts',(-25.3919035397376,13.0461048084143,
130.488149129457)) ;
#119805=CARTESIAN_POINT('Ctrl Pts',(-25.4235567372588,13.3089103849839,
130.547469606547)) ;
#119806=CARTESIAN_POINT('Ctrl Pts',(-25.431859388785,13.5795917474079,130.538616281477)) ;
#119807=CARTESIAN_POINT('Ctrl Pts',(-25.416926267712,13.839854863598,130.461786666502)) ;
#119808=CARTESIAN_POINT('Ctrl Pts',(-25.380454759044,14.069864909241,130.322056942441)) ;
#119809=CARTESIAN_POINT('Ctrl Pts',(-25.3263222418805,14.2524396014981,
130.130958807015)) ;
#119810=CARTESIAN_POINT('Ctrl Pts',(-25.2583610468973,14.3767943035019,
129.899231984381)) ;
#119811=CARTESIAN_POINT('Ctrl Pts',(-25.1829041424142,14.4324209572319,
129.645787191873)) ;
#119812=CARTESIAN_POINT('Ctrl Pts',(-25.105308843592,14.4159981206257,129.385906944881)) ;
#119813=CARTESIAN_POINT('Ctrl Pts',(-25.0324477821256,14.3283155320889,
129.13993894747)) ;
#119814=CARTESIAN_POINT('Ctrl Pts',(-24.9700443034682,14.1755659228116,
128.924477813871)) ;
#119815=CARTESIAN_POINT('Ctrl Pts',(-24.9235295808672,13.969906825541,128.75558920797)) ;
#119816=CARTESIAN_POINT('Ctrl Pts',(-24.8965566575616,13.7239840128541,
128.643607017274)) ;
#119817=CARTESIAN_POINT('Ctrl Pts',(-24.8920276788171,13.4571372933653,
128.597286645905)) ;
#119818=CARTESIAN_POINT('Ctrl Pts',(-24.9112224977238,13.1860385186985,
128.620028296661)) ;
#119819=CARTESIAN_POINT('Ctrl Pts',(-24.9527782276845,12.9351633427926,
128.708532779253)) ;
#119820=CARTESIAN_POINT('Ctrl Pts',(-25.0155797279094,12.716280428453,128.858654488145)) ;
#119821=CARTESIAN_POINT('Ctrl Pts',(-25.0942086463885,12.5504602967878,
129.055479919391)) ;
#119822=CARTESIAN_POINT('Ctrl Pts',(-25.1860347004579,12.4451571780271,
129.290326810206)) ;
#119823=CARTESIAN_POINT('Ctrl Pts',(-25.2825956957081,12.4110818136484,
129.539501707962)) ;
#119824=CARTESIAN_POINT('Ctrl Pts',(-25.3801028054309,12.4493848627275,
129.791040070531)) ;
#119825=CARTESIAN_POINT('Ctrl Pts',(-25.4700659725975,12.556427913144,130.020972058912)) ;
#119826=CARTESIAN_POINT('Ctrl Pts',(-25.5490464109895,12.7270948717805,
130.218374590402)) ;
#119827=CARTESIAN_POINT('Ctrl Pts',(-25.6103504725284,12.9467013402175,
130.364383698966)) ;
#119828=CARTESIAN_POINT('Ctrl Pts',(-25.651076334731,13.2005745563337,130.450229029158)) ;
#119829=CARTESIAN_POINT('Ctrl Pts',(-25.6688592932256,13.4697556094875,
130.46913314477)) ;
#119830=CARTESIAN_POINT('Ctrl Pts',(-25.6633326860655,13.7362552359381,
130.419869278086)) ;
#119831=CARTESIAN_POINT('Ctrl Pts',(-25.6351871184438,13.9814041933257,
130.30435482619)) ;
#119832=CARTESIAN_POINT('Ctrl Pts',(-25.5879229073729,14.1841666830384,
130.133366568428)) ;
#119833=CARTESIAN_POINT('Ctrl Pts',(-25.5247850978363,14.3343211929266,
129.91570247358)) ;
#119834=CARTESIAN_POINT('Ctrl Pts',(-25.4515062569338,14.4184551111194,
129.668497896698)) ;
#119835=CARTESIAN_POINT('Ctrl Pts',(-25.3741735889697,14.4314519975607,
129.409526512277)) ;
#119836=CARTESIAN_POINT('Ctrl Pts',(-25.2986654507318,14.3721435273992,
129.155794819144)) ;
#119837=CARTESIAN_POINT('Ctrl Pts',(-25.2314887860347,14.2453738509882,
128.926509843084)) ;
#119838=CARTESIAN_POINT('Ctrl Pts',(-25.177612160251,14.0581566958374,128.735807740753)) ;
#119839=CARTESIAN_POINT('Ctrl Pts',(-25.1425261531772,13.8276968106527,
128.600371370732)) ;
#119840=CARTESIAN_POINT('Ctrl Pts',(-25.1286129151028,13.5670203755234,
128.526578335593)) ;
#119841=CARTESIAN_POINT('Ctrl Pts',(-25.1381253558712,13.2953786744785,
128.521147180712)) ;
#119842=CARTESIAN_POINT('Ctrl Pts',(-25.1707614727794,13.0342214950179,
128.58344292195)) ;
#119843=CARTESIAN_POINT('Ctrl Pts',(-25.2255179487015,12.7992352777049,
128.710098750454)) ;
#119844=CARTESIAN_POINT('Ctrl Pts',(-25.2979655542483,12.6113833120471,
128.888843585747)) ;
#119845=CARTESIAN_POINT('Ctrl Pts',(-25.3850206418746,12.4798503942449,
129.109960878586)) ;
#119846=CARTESIAN_POINT('Ctrl Pts',(-25.4803776423451,12.416397864002,129.355428944409)) ;
#119847=CARTESIAN_POINT('Ctrl Pts',(-25.5783843703953,12.4249214929509,
129.608549524434)) ;
#119848=CARTESIAN_POINT('Ctrl Pts',(-25.672478530963,12.5053755952326,129.850242670599)) ;
#119849=CARTESIAN_POINT('Ctrl Pts',(-25.756226931752,12.6507859052006,130.061889235013)) ;
#119850=CARTESIAN_POINT('Ctrl Pts',(-25.8251533352949,12.8517470992337,
130.230128068929)) ;
#119851=CARTESIAN_POINT('Ctrl Pts',(-25.8747980900926,13.0945614507412,
130.341931437405)) ;
#119852=CARTESIAN_POINT('Ctrl Pts',(-25.9020710193289,13.3602126376938,
130.388483679895)) ;
#119853=CARTESIAN_POINT('Ctrl Pts',(-25.9058670751018,13.6310671963869,
130.366361615972)) ;
#119854=CARTESIAN_POINT('Ctrl Pts',(-25.8867754919466,13.8852753848623,
130.277607898819)) ;
#119855=CARTESIAN_POINT('Ctrl Pts',(-25.846806345492,14.1076160740045,130.127719600837)) ;
#119856=CARTESIAN_POINT('Ctrl Pts',(-25.7894563509561,14.2808806662079,
129.927039264704)) ;
#119857=CARTESIAN_POINT('Ctrl Pts',(-25.7197630440978,14.3926567103846,
129.690353283305)) ;
#119858=CARTESIAN_POINT('Ctrl Pts',(-25.6429800311209,14.4348969491125,
129.432802823452)) ;
#119859=CARTESIAN_POINT('Ctrl Pts',(-25.5664052890858,14.4049966950683,
129.176188720963)) ;
#119860=CARTESIAN_POINT('Ctrl Pts',(-25.4945634031681,14.3037928875116,
128.932948137202)) ;
#119861=CARTESIAN_POINT('Ctrl Pts',(-25.435091766399,14.1405203865162,128.726223307007)) ;
#119862=CARTESIAN_POINT('Ctrl Pts',(-25.3919011396787,13.9258191062473,
128.566958681327)) ;
#119863=CARTESIAN_POINT('Ctrl Pts',(-25.3690363816211,13.6747404924344,
128.467031877332)) ;
#119864=CARTESIAN_POINT('Ctrl Pts',(-25.3690010643952,13.4052256695436,
128.433742776243)) ;
#119865=CARTESIAN_POINT('Ctrl Pts',(-25.3922616413952,13.1384692475265,
128.468700955033)) ;
#119866=CARTESIAN_POINT('Ctrl Pts',(-25.4384366048813,12.8897551535746,
128.570278947386)) ;
#119867=CARTESIAN_POINT('Ctrl Pts',(-25.5041846804616,12.6813707953234,
128.729325865057)) ;
#119868=CARTESIAN_POINT('Ctrl Pts',(-25.585982476974,12.5252896402636,128.935167552922)) ;
#119869=CARTESIAN_POINT('Ctrl Pts',(-25.6787370032368,12.4335762079788,
129.172983990663)) ;
#119870=CARTESIAN_POINT('Ctrl Pts',(-25.7761856628954,12.4126069664436,
129.424592020829)) ;
#119871=CARTESIAN_POINT('Ctrl Pts',(-25.8729618386419,12.4645413764585,
129.673998882875)) ;
#119872=CARTESIAN_POINT('Ctrl Pts',(-25.9613851744278,12.5845282668637,
129.899302334015)) ;
#119873=CARTESIAN_POINT('Ctrl Pts',(-26.0371581474449,12.7652451064021,
130.087456352873)) ;
#119874=CARTESIAN_POINT('Ctrl Pts',(-26.0947547148825,12.9922347341953,
130.222671327764)) ;
#119875=CARTESIAN_POINT('Ctrl Pts',(-26.1312796240102,13.2501818574091,
130.296287346821)) ;
#119876=CARTESIAN_POINT('Ctrl Pts',(-26.1447384833071,13.5208713010695,
130.302481379232)) ;
#119877=CARTESIAN_POINT('Ctrl Pts',(-26.1347422066459,13.7852948748941,
130.240058557626)) ;
#119878=CARTESIAN_POINT('Ctrl Pts',(-26.1028034649425,14.0230293879869,
130.113628542378)) ;
#119879=CARTESIAN_POINT('Ctrl Pts',(-26.0519060113355,14.2178154382897,
129.931791193316)) ;
#119880=CARTESIAN_POINT('Ctrl Pts',(-25.9867514193326,14.3552930540828,
129.708440395722)) ;
#119881=CARTESIAN_POINT('Ctrl Pts',(-25.9119954035665,14.4265292549101,
129.456819725079)) ;
#119882=CARTESIAN_POINT('Ctrl Pts',(-25.834829513542,14.425752226316,129.198453425837)) ;
#119883=CARTESIAN_POINT('Ctrl Pts',(-25.7602440523618,14.3531911968223,
128.947353700595)) ;
#119884=CARTESIAN_POINT('Ctrl Pts',(-25.6951616209711,14.2139749127786,
128.724118518912)) ;
#119885=CARTESIAN_POINT('Ctrl Pts',(-25.6446900925232,14.0181343155111,
128.543547684947)) ;
#119886=CARTESIAN_POINT('Ctrl Pts',(-25.6132229947609,13.7796845152241,
128.418501547274)) ;
#119887=CARTESIAN_POINT('Ctrl Pts',(-25.6037330848021,13.5155236059082,
128.357635520124)) ;
#119888=CARTESIAN_POINT('Ctrl Pts',(-25.617628730475,13.245212667821,128.365140772047)) ;
#119889=CARTESIAN_POINT('Ctrl Pts',(-25.6545017751569,12.987705840382,128.439790008711)) ;
#119890=CARTESIAN_POINT('Ctrl Pts',(-25.7129219295576,12.7602060641004,
128.577198728452)) ;
#119891=CARTESIAN_POINT('Ctrl Pts',(-25.7885884356989,12.5817512683668,
128.765242790756)) ;
#119892=CARTESIAN_POINT('Ctrl Pts',(-25.877553695151,12.4625557490256,128.991997656452)) ;
#119893=CARTESIAN_POINT('Ctrl Pts',(-25.9741233376341,12.4124303716615,
129.240908418124)) ;
#119894=CARTESIAN_POINT('Ctrl Pts',(-26.0714881147419,12.4345388124725,
129.49229097036)) ;
#119895=CARTESIAN_POINT('Ctrl Pts',(-26.164529411831,12.5283216508309,129.730772431684)) ;
#119896=CARTESIAN_POINT('Ctrl Pts',(-26.2456332053162,12.6848122418478,
129.934762024602)) ;
#119897=CARTESIAN_POINT('Ctrl Pts',(-26.3113716154821,12.8954782936503,
130.093573957543)) ;
#119898=CARTESIAN_POINT('Ctrl Pts',(-26.3567423635182,13.1430312218348,
130.193051677295)) ;
#119899=CARTESIAN_POINT('Ctrl Pts',(-26.3796682101619,13.4109716011332,
130.22690034591)) ;
#119900=CARTESIAN_POINT('Ctrl Pts',(-26.379180399323,13.6794256976715,130.192408300591)) ;
#119901=CARTESIAN_POINT('Ctrl Pts',(-26.355735708432,13.9314101100325,130.090586754578)) ;
#119902=CARTESIAN_POINT('Ctrl Pts',(-26.3122326343032,14.1445006487741,
129.930508199489)) ;
#119903=CARTESIAN_POINT('Ctrl Pts',(-26.2523309894027,14.3067536437968,
129.722457733583)) ;
#119904=CARTESIAN_POINT('Ctrl Pts',(-26.180794884382,14.406048704081,129.480333016166)) ;
#119905=CARTESIAN_POINT('Ctrl Pts',(-26.103660979524,14.4348548847552,129.221860931271)) ;
#119906=CARTESIAN_POINT('Ctrl Pts',(-26.027136998052,14.3909041630567,128.965141568143)) ;
#119907=CARTESIAN_POINT('Ctrl Pts',(-25.9578089641216,14.2783347408893,
128.729615948131)) ;
#119908=CARTESIAN_POINT('Ctrl Pts',(-25.9005074043686,14.1031935326512,
128.528930992271)) ;
#119909=CARTESIAN_POINT('Ctrl Pts',(-25.8609965381137,13.8800104531449,
128.380399450144)) ;
#119910=CARTESIAN_POINT('Ctrl Pts',(-25.8423806954271,13.6249527431351,
128.29299369777)) ;
#119911=CARTESIAN_POINT('Ctrl Pts',(-25.8466982567422,13.3547990106838,
128.272493370141)) ;
#119912=CARTESIAN_POINT('Ctrl Pts',(-25.8743205831141,13.0897726871477,
128.320116058481)) ;
#119913=CARTESIAN_POINT('Ctrl Pts',(-25.9246264611834,12.8467549358408,
128.433719030383)) ;
#119914=CARTESIAN_POINT('Ctrl Pts',(-25.9935112856203,12.6478124194814,
128.602020346365)) ;
#119915=CARTESIAN_POINT('Ctrl Pts',(-26.0779380529408,12.5027972017395,
128.815470225642)) ;
#119916=CARTESIAN_POINT('Ctrl Pts',(-26.171965786403,12.4240443631204,129.057051810318)) ;
#119917=CARTESIAN_POINT('Ctrl Pts',(-26.2702731079583,12.4170503620235,
129.310949808494)) ;
#119918=CARTESIAN_POINT('Ctrl Pts',(-26.3650966714635,12.4817913910706,
129.555002001196)) ;
#119919=CARTESIAN_POINT('Ctrl Pts',(-26.45196366406,12.6142900720352,129.775575257278)) ;
#119920=CARTESIAN_POINT('Ctrl Pts',(-26.5243727321012,12.8042103797361,
129.95405025432)) ;
#119921=CARTESIAN_POINT('Ctrl Pts',(-26.578483057693,13.0388186679886,130.078979362122)) ;
#119922=CARTESIAN_POINT('Ctrl Pts',(-26.6108288981163,13.3023285356057,
130.140176565052)) ;
#119923=CARTESIAN_POINT('Ctrl Pts',(-26.6197222679655,13.5713414244093,
130.13326049002)) ;
#119924=CARTESIAN_POINT('Ctrl Pts',(-26.6054350404599,13.8329962624196,
130.05821374072)) ;
#119925=CARTESIAN_POINT('Ctrl Pts',(-26.5696096637515,14.0635776732595,
129.920451931681)) ;
#119926=CARTESIAN_POINT('Ctrl Pts',(-26.5158545454307,14.2479537129057,
129.730399291059)) ;
#119927=CARTESIAN_POINT('Ctrl Pts',(-26.4484523870756,14.3739504524616,
129.500417543721)) ;
#119928=CARTESIAN_POINT('Ctrl Pts',(-26.3725118085867,14.4320428202114,
129.245284462382)) ;
#119929=CARTESIAN_POINT('Ctrl Pts',(-26.2950856667936,14.4172275028747,
128.985988129081)) ;
#119930=CARTESIAN_POINT('Ctrl Pts',(-26.2222776936055,14.3318166981341,
128.740288747817)) ;
#119931=CARTESIAN_POINT('Ctrl Pts',(-26.1595230999705,14.1811818293068,
128.52384486406)) ;
#119932=CARTESIAN_POINT('Ctrl Pts',(-26.1123210485869,13.9759967622757,
128.352808501451)) ;
#119933=CARTESIAN_POINT('Ctrl Pts',(-26.084770830645,13.7313492386451,128.239201365232)) ;
#119934=CARTESIAN_POINT('Ctrl Pts',(-26.0797136555551,13.4634561102099,
128.191161323004)) ;
#119935=CARTESIAN_POINT('Ctrl Pts',(-26.0978801533651,13.195884935421,128.211372693161)) ;
#119936=CARTESIAN_POINT('Ctrl Pts',(-26.1392146081528,12.9412337002998,
128.298829939633)) ;
#119937=CARTESIAN_POINT('Ctrl Pts',(-26.2009044712201,12.7230235152343,
128.4460160171)) ;
#119938=CARTESIAN_POINT('Ctrl Pts',(-26.2798277046628,12.5539648154296,
128.643380639081)) ;
#119939=CARTESIAN_POINT('Ctrl Pts',(-26.3704183582616,12.4477725877379,
128.874981924817)) ;
#119940=CARTESIAN_POINT('Ctrl Pts',(-26.4675932472334,12.4110238126212,
129.125691828151)) ;
#119941=CARTESIAN_POINT('Ctrl Pts',(-26.56471080497,12.4468710250015,129.376273587607)) ;
#119942=CARTESIAN_POINT('Ctrl Pts',(-26.6558840954224,12.553155401547,129.609384734652)) ;
#119943=CARTESIAN_POINT('Ctrl Pts',(-26.7346205058782,12.7211113699614,
129.806339257464)) ;
#119944=CARTESIAN_POINT('Ctrl Pts',(-26.7966910177754,12.9400020395614,
129.954485352245)) ;
#119945=CARTESIAN_POINT('Ctrl Pts',(-26.8378916621286,13.1921120762229,
130.041855669963)) ;
#119946=CARTESIAN_POINT('Ctrl Pts',(-26.8565040574598,13.4620045651565,
130.063068042932)) ;
#119947=CARTESIAN_POINT('Ctrl Pts',(-26.8515337300207,13.7292706567068,
130.015371921608)) ;
#119948=CARTESIAN_POINT('Ctrl Pts',(-26.8242404610039,13.9738126182776,
129.902564087945)) ;
#119949=CARTESIAN_POINT('Ctrl Pts',(-26.7772359040396,14.1794947275424,
129.732112690396)) ;
#119950=CARTESIAN_POINT('Ctrl Pts',(-26.7143307640667,14.3311259291818,
129.515097701107)) ;
#119951=CARTESIAN_POINT('Ctrl Pts',(-26.6416882302053,14.4169205617397,
129.269939993438)) ;
#119952=CARTESIAN_POINT('Ctrl Pts',(-26.5639471821135,14.4320030315974,
129.009577672861)) ;
#119953=CARTESIAN_POINT('Ctrl Pts',(-26.4887082299279,14.3751243687379,
128.756828801049)) ;
#119954=CARTESIAN_POINT('Ctrl Pts',(-26.4206397914384,14.2488768179311,
128.524628975738)) ;
#119955=CARTESIAN_POINT('Ctrl Pts',(-26.3668727336172,14.0648018746923,
128.334575647107)) ;
#119956=CARTESIAN_POINT('Ctrl Pts',(-26.3309363903451,13.8343788522074,
128.196474328605)) ;
#119957=CARTESIAN_POINT('Ctrl Pts',(-26.3164705215498,13.5736071381831,
128.121002145167)) ;
#119958=CARTESIAN_POINT('Ctrl Pts',(-26.3253756653385,13.3025525300613,
128.113863715032)) ;
#119959=CARTESIAN_POINT('Ctrl Pts',(-26.3572716727716,13.0417945957582,
128.174109071432)) ;
#119960=CARTESIAN_POINT('Ctrl Pts',(-26.4111773947375,12.8063140685278,
128.298382516279)) ;
#119961=CARTESIAN_POINT('Ctrl Pts',(-26.4834589153869,12.6158856975737,
128.476480452916)) ;
#119962=CARTESIAN_POINT('Ctrl Pts',(-26.570354800423,12.4825396970198,128.697083686748)) ;
#119963=CARTESIAN_POINT('Ctrl Pts',(-26.6652801627027,12.4173081237828,
128.941385506295)) ;
#119964=CARTESIAN_POINT('Ctrl Pts',(-26.7631989430957,12.423605000428,129.194283543105)) ;
#119965=CARTESIAN_POINT('Ctrl Pts',(-26.8574619524539,12.5018025966581,
129.436489000106)) ;
#119966=CARTESIAN_POINT('Ctrl Pts',(-26.9418546221037,12.6458565798938,
129.649912040933)) ;
#119967=CARTESIAN_POINT('Ctrl Pts',(-27.0111976409268,12.8453790833706,
129.819389913643)) ;
#119968=CARTESIAN_POINT('Ctrl Pts',(-27.061367894877,13.0865652662194,129.932812364929)) ;
#119969=CARTESIAN_POINT('Ctrl Pts',(-27.089369420874,13.3521427577607,129.981445190974)) ;
#119970=CARTESIAN_POINT('Ctrl Pts',(-27.0939017928513,13.6222557202932,
129.961586504907)) ;
#119971=CARTESIAN_POINT('Ctrl Pts',(-27.0754482421394,13.8783882969557,
129.874548069754)) ;
#119972=CARTESIAN_POINT('Ctrl Pts',(-27.0359007012441,14.1022120618795,
129.725831051564)) ;
#119973=CARTESIAN_POINT('Ctrl Pts',(-26.9791357431868,14.2765229506337,
129.52695378676)) ;
#119974=CARTESIAN_POINT('Ctrl Pts',(-26.909823932067,14.3902286964009,129.291416282315)) ;
#119975=CARTESIAN_POINT('Ctrl Pts',(-26.8330387921819,14.4347769427253,
129.033812213985)) ;
#119976=CARTESIAN_POINT('Ctrl Pts',(-26.7562449577674,14.4066722617846,
128.776487535096)) ;
#119977=CARTESIAN_POINT('Ctrl Pts',(-26.6845764119764,14.3082119125381,
128.533963122741)) ;
#119978=CARTESIAN_POINT('Ctrl Pts',(-26.6243671408649,14.1460357867196,
128.324921351722)) ;
#119979=CARTESIAN_POINT('Ctrl Pts',(-26.5806797943847,13.9328084574968,
128.164244549597)) ;
#119980=CARTESIAN_POINT('Ctrl Pts',(-26.5571663955051,13.681774125451,128.062322382885)) ;
#119981=CARTESIAN_POINT('Ctrl Pts',(-26.5564073780867,13.414026239165,128.027111822149)) ;
#119982=CARTESIAN_POINT('Ctrl Pts',(-26.5791491455037,13.1453688505525,
128.060346836654)) ;
#119983=CARTESIAN_POINT('Ctrl Pts',(-26.6242809472691,12.8977836793382,
128.159158681216)) ;
#119984=CARTESIAN_POINT('Ctrl Pts',(-26.6899845415361,12.6861562687701,
128.317792644291)) ;
#119985=CARTESIAN_POINT('Ctrl Pts',(-26.7712746549743,12.5289208649723,
128.522226758068)) ;
#119986=CARTESIAN_POINT('Ctrl Pts',(-26.863894350046,12.4351549173609,128.759610343918)) ;
#119987=CARTESIAN_POINT('Ctrl Pts',(-26.9610674145653,12.41223935111,129.010490108608)) ;
#119988=CARTESIAN_POINT('Ctrl Pts',(-27.0579665728015,12.4619213802628,
129.260261295811)) ;
#119989=CARTESIAN_POINT('Ctrl Pts',(-27.1468958938683,12.5803996576492,
129.486961095898)) ;
#119990=CARTESIAN_POINT('Ctrl Pts',(-27.2229176963561,12.7591299029993,
129.675926443311)) ;
#119991=CARTESIAN_POINT('Ctrl Pts',(-27.281148945456,12.9850687098392,129.81297179148)) ;
#119992=CARTESIAN_POINT('Ctrl Pts',(-27.3183216390964,13.2423777054139,
129.888482171424)) ;
#119993=CARTESIAN_POINT('Ctrl Pts',(-27.33245310508,13.5129449016412,129.896642523138)) ;
#119994=CARTESIAN_POINT('Ctrl Pts',(-27.3231877835587,13.7774320597186,
129.836414647175)) ;
#119995=CARTESIAN_POINT('Ctrl Pts',(-27.2917829639029,14.0166134042629,
129.711475383655)) ;
#119996=CARTESIAN_POINT('Ctrl Pts',(-27.2416990232453,14.2120830530507,
129.532186320855)) ;
#119997=CARTESIAN_POINT('Ctrl Pts',(-27.1764440767512,14.352498916215,129.308296129156)) ;
#119998=CARTESIAN_POINT('Ctrl Pts',(-27.1021012358692,14.4253825701344,
129.057999247625)) ;
#119999=CARTESIAN_POINT('Ctrl Pts',(-27.0248123116318,14.426768294094,128.799213207415)) ;
#120000=CARTESIAN_POINT('Ctrl Pts',(-26.950228893693,14.3564920185828,128.548208386946)) ;
#120001=CARTESIAN_POINT('Ctrl Pts',(-26.8845614503941,14.2186719371757,
128.323146626863)) ;
#120002=CARTESIAN_POINT('Ctrl Pts',(-26.8336555426971,14.024316786925,128.141329983919)) ;
#120003=CARTESIAN_POINT('Ctrl Pts',(-26.801597940401,13.7866136068205,128.01452758408)) ;
#120004=CARTESIAN_POINT('Ctrl Pts',(-26.7914773675253,13.5238037033397,
127.951929029032)) ;
#120005=CARTESIAN_POINT('Ctrl Pts',(-26.8046611115732,13.2527086042196,
127.957271158598)) ;
#120006=CARTESIAN_POINT('Ctrl Pts',(-26.8411453165669,12.9936530632693,
128.030652771087)) ;
#120007=CARTESIAN_POINT('Ctrl Pts',(-26.8987574318875,12.7662441874236,
128.165867096014)) ;
#120008=CARTESIAN_POINT('Ctrl Pts',(-26.9740830180008,12.5858801409006,
128.352858112991)) ;
#120009=CARTESIAN_POINT('Ctrl Pts',(-27.0628251755867,12.4648530718858,
128.578942893323)) ;
#120010=CARTESIAN_POINT('Ctrl Pts',(-27.1594231609068,12.4128201875619,
128.827887210328)) ;
#120011=CARTESIAN_POINT('Ctrl Pts',(-27.2564574363076,12.4330274107103,
129.078429229244)) ;
#120012=CARTESIAN_POINT('Ctrl Pts',(-27.3493201635517,12.524012324909,129.316551012229)) ;
#120013=CARTESIAN_POINT('Ctrl Pts',(-27.4313416689702,12.6795221282536,
129.523026324944)) ;
#120014=CARTESIAN_POINT('Ctrl Pts',(-27.4975379318319,12.8889214141028,
129.683186921422)) ;
#120015=CARTESIAN_POINT('Ctrl Pts',(-27.5435488308571,13.1354947089828,
129.784545867269)) ;
#120016=CARTESIAN_POINT('Ctrl Pts',(-27.5671767452064,13.4042911436029,
129.82030507381)) ;
#120017=CARTESIAN_POINT('Ctrl Pts',(-27.5672643845209,13.6719452313923,
129.787618405761)) ;
#120018=CARTESIAN_POINT('Ctrl Pts',(-27.5445552780615,13.9242175336792,
129.688018851963)) ;
#120019=CARTESIAN_POINT('Ctrl Pts',(-27.5015315379868,14.1390288741834,
129.529280677435)) ;
#120020=CARTESIAN_POINT('Ctrl Pts',(-27.4419857500411,14.3030286144717,
129.322247793777)) ;
#120021=CARTESIAN_POINT('Ctrl Pts',(-27.3706593624215,14.4041953326341,
129.080722338789)) ;
#120022=CARTESIAN_POINT('Ctrl Pts',(-27.2938390424101,14.4349854779899,
128.823267047109)) ;
#120023=CARTESIAN_POINT('Ctrl Pts',(-27.2171925956617,14.3934046886661,
128.566192203389)) ;
#120024=CARTESIAN_POINT('Ctrl Pts',(-27.147345149048,14.2822103121525,128.329025749962)) ;
#120025=CARTESIAN_POINT('Ctrl Pts',(-27.0899564874658,14.1097942363152,
128.128293079995)) ;
#120026=CARTESIAN_POINT('Ctrl Pts',(-27.0497024032013,13.8877667094565,
127.977541901105)) ;
#120027=CARTESIAN_POINT('Ctrl Pts',(-27.0303723935246,13.6324084420419,
127.88792266215)) ;
#120028=CARTESIAN_POINT('Ctrl Pts',(-27.0340283149476,13.3624185504467,
127.865495007072)) ;
#120029=CARTESIAN_POINT('Ctrl Pts',(-27.0610999882633,13.0965814778885,
127.911450823542)) ;
#120030=CARTESIAN_POINT('Ctrl Pts',(-27.1104911197653,12.8540736174815,
128.022582139951)) ;
#120031=CARTESIAN_POINT('Ctrl Pts',(-27.1789274866825,12.652992435015,128.189498753939)) ;
#120032=CARTESIAN_POINT('Ctrl Pts',(-27.263499859652,12.5055874303856,128.403191515036)) ;
#120033=CARTESIAN_POINT('Ctrl Pts',(-27.3569065509663,12.4255318647486,
128.643116064752)) ;
#120034=CARTESIAN_POINT('Ctrl Pts',(-27.4547438900964,12.4160627512278,
128.895790668738)) ;
#120035=CARTESIAN_POINT('Ctrl Pts',(-27.5502080114701,12.4788299066414,
129.141554051022)) ;
#120036=CARTESIAN_POINT('Ctrl Pts',(-27.6374637904928,12.6096602766835,
129.363239415158)) ;
#120037=CARTESIAN_POINT('Ctrl Pts',(-27.710474888215,12.7985462130252,129.543405360105)) ;
#120038=CARTESIAN_POINT('Ctrl Pts',(-27.7649671434383,13.031708612879,129.669522362687)) ;
#120039=CARTESIAN_POINT('Ctrl Pts',(-27.7979073063491,13.293083578928,129.732646606245)) ;
#120040=CARTESIAN_POINT('Ctrl Pts',(-27.8076097011333,13.5641924680593,
129.727839251528)) ;
#120041=CARTESIAN_POINT('Ctrl Pts',(-27.7939119342835,13.8256806601297,
129.6546004207)) ;
#120042=CARTESIAN_POINT('Ctrl Pts',(-27.7588915640264,14.0565823152587,
129.519317960093)) ;
#120043=CARTESIAN_POINT('Ctrl Pts',(-27.7054698422737,14.2434411149003,
129.330116948414)) ;
#120044=CARTESIAN_POINT('Ctrl Pts',(-27.6380806543802,14.3714533613372,
129.100046951507)) ;
#120045=CARTESIAN_POINT('Ctrl Pts',(-27.5629246445623,14.4311593709141,
128.847484461924)) ;
#120046=CARTESIAN_POINT('Ctrl Pts',(-27.4852723112633,14.4188767370812,
128.587442802152)) ;
#120047=CARTESIAN_POINT('Ctrl Pts',(-27.4120884349404,14.3353893813971,
128.340584539541)) ;
#120048=CARTESIAN_POINT('Ctrl Pts',(-27.3487944677133,14.1858866209329,
128.122457267565)) ;
#120049=CARTESIAN_POINT('Ctrl Pts',(-27.3012779883249,13.9829323143578,
127.950645883144)) ;
#120050=CARTESIAN_POINT('Ctrl Pts',(-27.2730500223035,13.7386001915966,
127.834971228421)) ;
#120051=CARTESIAN_POINT('Ctrl Pts',(-27.2672861034049,13.472491070878,127.785043211583)) ;
#120052=CARTESIAN_POINT('Ctrl Pts',(-27.284851176658,13.2027754622607,127.803255891318)) ;
#120053=CARTESIAN_POINT('Ctrl Pts',(-27.3256506936343,12.9475729445581,
127.889163192759)) ;
#120054=CARTESIAN_POINT('Ctrl Pts',(-27.3866924004005,12.7286906854066,
128.034522298347)) ;
#120055=CARTESIAN_POINT('Ctrl Pts',(-27.4649756495311,12.5582194228626,
128.230093788475)) ;
#120056=CARTESIAN_POINT('Ctrl Pts',(-27.5557878968131,12.4495814745878,
128.462164406796)) ;
#120057=CARTESIAN_POINT('Ctrl Pts',(-27.6526736826316,12.4111325030014,
128.712104171976)) ;
#120058=CARTESIAN_POINT('Ctrl Pts',(-27.7496521545279,12.4448573230465,
128.962350011997)) ;
#120059=CARTESIAN_POINT('Ctrl Pts',(-27.8408738308629,12.5485736269638,
129.19570165313)) ;
#120060=CARTESIAN_POINT('Ctrl Pts',(-27.9205751184065,12.7160675409956,
129.39524107991)) ;
#120061=CARTESIAN_POINT('Ctrl Pts',(-27.9828423779555,12.9327061634172,
129.544132215434)) ;
#120062=CARTESIAN_POINT('Ctrl Pts',(-28.0248443453271,13.1846668378338,
129.633751795151)) ;
#120063=CARTESIAN_POINT('Ctrl Pts',(-28.0440759127581,13.4544224505961,
129.656768706986)) ;
#120064=CARTESIAN_POINT('Ctrl Pts',(-28.0398000022802,13.7215757277082,
129.611158867274)) ;
#120065=CARTESIAN_POINT('Ctrl Pts',(-28.0130827312133,13.9674105771419,
129.499981050513)) ;
#120066=CARTESIAN_POINT('Ctrl Pts',(-27.9666619118937,14.173959529566,129.331298499324)) ;
#120067=CARTESIAN_POINT('Ctrl Pts',(-27.9043787727222,14.3272528917974,
129.116193991239)) ;
#120068=CARTESIAN_POINT('Ctrl Pts',(-27.8314693794371,14.4155297933765,
128.870033469215)) ;
#120069=CARTESIAN_POINT('Ctrl Pts',(-27.7542546913223,14.4326688919931,
128.611425849187)) ;
#120070=CARTESIAN_POINT('Ctrl Pts',(-27.6784027230996,14.3775210851954,
128.356670056856)) ;
#120071=CARTESIAN_POINT('Ctrl Pts',(-27.6105108398773,14.2540409497735,
128.125232978784)) ;
#120072=CARTESIAN_POINT('Ctrl Pts',(-27.5559663213141,14.0709648404294,
127.932757755026)) ;
#120073=CARTESIAN_POINT('Ctrl Pts',(-27.5195045149598,13.8416199904244,
127.793133853687)) ;
#120074=CARTESIAN_POINT('Ctrl Pts',(-27.504387097539,13.582388567831,127.715867343528)) ;
#120075=CARTESIAN_POINT('Ctrl Pts',(-27.512461944946,13.3112804497714,127.706295015043)) ;
#120076=CARTESIAN_POINT('Ctrl Pts',(-27.5439286608517,13.0483997987315,
127.765078691399)) ;
#120077=CARTESIAN_POINT('Ctrl Pts',(-27.5970088742453,12.8130298392026,
127.887100914663)) ;
#120078=CARTESIAN_POINT('Ctrl Pts',(-27.6690075490512,12.6204060823588,
128.064263470253)) ;
#120079=CARTESIAN_POINT('Ctrl Pts',(-27.7555377826022,12.4854479324355,
128.283821873288)) ;
#120080=CARTESIAN_POINT('Ctrl Pts',(-27.8503161312509,12.4181326730335,
128.527685295473)) ;
#120081=CARTESIAN_POINT('Ctrl Pts',(-27.9485129845829,12.4224942487035,
128.781307773095)) ;
#120082=CARTESIAN_POINT('Ctrl Pts',(-28.0428661775056,12.4989653084942,
129.023800058949)) ;
#120083=CARTESIAN_POINT('Ctrl Pts',(-28.1272530074145,12.6405919477357,
129.237349753736)) ;
#120084=CARTESIAN_POINT('Ctrl Pts',(-28.1973339593537,12.8391593414189,
129.408887782509)) ;
#120085=CARTESIAN_POINT('Ctrl Pts',(-28.2481782006358,13.080245962358,129.524181066457)) ;
#120086=CARTESIAN_POINT('Ctrl Pts',(-28.2766847337897,13.3449462168028,
129.57435157818)) ;
#120087=CARTESIAN_POINT('Ctrl Pts',(-28.2818776537657,13.6142996681917,
129.556530060392)) ;
#120088=CARTESIAN_POINT('Ctrl Pts',(-28.2641076414484,13.8710421169928,
129.471498550365)) ;
#120089=CARTESIAN_POINT('Ctrl Pts',(-28.2251634394076,14.0962488257935,
129.324535823862)) ;
#120090=CARTESIAN_POINT('Ctrl Pts',(-28.1684679190227,14.2729914081674,
129.125671381229)) ;
#120091=CARTESIAN_POINT('Ctrl Pts',(-28.0997758612644,14.38767954712,128.892123160332)) ;
#120092=CARTESIAN_POINT('Ctrl Pts',(-28.0232427382542,14.4346057861831,
128.63530633569)) ;
#120093=CARTESIAN_POINT('Ctrl Pts',(-27.9459527748653,14.4082599468392,
128.376344855625)) ;
#120094=CARTESIAN_POINT('Ctrl Pts',(-27.8744882234117,14.3122705880149,
128.13462021069)) ;
#120095=CARTESIAN_POINT('Ctrl Pts',(-27.8135936127414,14.151436185241,127.923455054537)) ;
#120096=CARTESIAN_POINT('Ctrl Pts',(-27.7693832548727,13.9387188784377,
127.761169573869)) ;
#120097=CARTESIAN_POINT('Ctrl Pts',(-27.7453621747428,13.6904434125759,
127.658016736476)) ;
#120098=CARTESIAN_POINT('Ctrl Pts',(-27.7439096559699,13.4208420598601,
127.620511771047)) ;
#120099=CARTESIAN_POINT('Ctrl Pts',(-27.7659128645592,13.1534853902676,
127.651789024545)) ;
#120100=CARTESIAN_POINT('Ctrl Pts',(-27.8104583821031,12.9044050288982,
127.748805634011)) ;
#120101=CARTESIAN_POINT('Ctrl Pts',(-27.8757029644118,12.6913475994885,
127.906078375144)) ;
#120102=CARTESIAN_POINT('Ctrl Pts',(-27.9566964837822,12.5324269019675,
128.109615216131)) ;
#120103=CARTESIAN_POINT('Ctrl Pts',(-28.0487615859234,12.4369854947191,
128.345493668793)) ;
#120104=CARTESIAN_POINT('Ctrl Pts',(-28.1460793490075,12.4119049760396,
128.596722852201)) ;
#120105=CARTESIAN_POINT('Ctrl Pts',(-28.2427525510562,12.459288588066,128.845956716394)) ;
#120106=CARTESIAN_POINT('Ctrl Pts',(-28.3320836999319,12.5757336822765,
129.073801113102)) ;
#120107=CARTESIAN_POINT('Ctrl Pts',(-28.4086125469476,12.7527802879128,
129.264241908838)) ;
#120108=CARTESIAN_POINT('Ctrl Pts',(-28.4677113029093,12.9786618268138,
129.403659288711)) ;
#120109=CARTESIAN_POINT('Ctrl Pts',(-28.5054453845473,13.2359088344013,
129.480751482382)) ;
#120110=CARTESIAN_POINT('Ctrl Pts',(-28.5201651176751,13.5051026285248,
129.490788903178)) ;
#120111=CARTESIAN_POINT('Ctrl Pts',(-28.511478093157,13.7711208876962,129.43210680396)) ;
#120112=CARTESIAN_POINT('Ctrl Pts',(-28.4807787726203,14.0100003599807,
129.309399633042)) ;
#120113=CARTESIAN_POINT('Ctrl Pts',(-28.4311079427157,14.2073724408212,
129.131245480571)) ;
#120114=CARTESIAN_POINT('Ctrl Pts',(-28.3663019439018,14.3492226306733,
128.908727993492)) ;
#120115=CARTESIAN_POINT('Ctrl Pts',(-28.2922494089841,14.4242519881516,
128.659316158414)) ;
#120116=CARTESIAN_POINT('Ctrl Pts',(-28.2146325752778,14.4277364563771,
128.399432279239)) ;
#120117=CARTESIAN_POINT('Ctrl Pts',(-28.1399868460076,14.3592420110673,
128.148280493659)) ;
#120118=CARTESIAN_POINT('Ctrl Pts',(-28.0742582761007,14.2240686922171,
127.923199970122)) ;
#120119=CARTESIAN_POINT('Ctrl Pts',(-28.0226491504683,14.0305585465179,
127.739203779342)) ;
#120120=CARTESIAN_POINT('Ctrl Pts',(-27.9900653350808,13.7945206228156,
127.610955419559)) ;
#120121=CARTESIAN_POINT('Ctrl Pts',(-27.9792144938345,13.5313067865741,
127.546105203021)) ;
#120122=CARTESIAN_POINT('Ctrl Pts',(-27.9917574792818,13.2605192088026,
127.549621813665)) ;
#120123=CARTESIAN_POINT('Ctrl Pts',(-28.0274315736986,13.0015411116714,
127.620730641976)) ;
#120124=CARTESIAN_POINT('Ctrl Pts',(-28.0844757419312,12.7725523899085,
127.754241521427)) ;
#120125=CARTESIAN_POINT('Ctrl Pts',(-28.1595479835507,12.5901314079498,
127.940405447423)) ;
#120126=CARTESIAN_POINT('Ctrl Pts',(-28.2479367999414,12.4675131368497,
128.165483243194)) ;
#120127=CARTESIAN_POINT('Ctrl Pts',(-28.3439620446915,12.4133289133512,
128.412901195813)) ;
#120128=CARTESIAN_POINT('Ctrl Pts',(-28.441732963266,12.4315113469885,128.665359909944)) ;
#120129=CARTESIAN_POINT('Ctrl Pts',(-28.5345032017863,12.5204618731953,
128.903319666748)) ;
#120130=CARTESIAN_POINT('Ctrl Pts',(-28.6169074040931,12.6740885600686,
129.110919783452)) ;
#120131=CARTESIAN_POINT('Ctrl Pts',(-28.6836409940969,12.8820605633652,
129.272658091374)) ;
#120132=CARTESIAN_POINT('Ctrl Pts',(-28.7303002545427,13.1280849033747,
129.375868286751)) ;
#120133=CARTESIAN_POINT('Ctrl Pts',(-28.7545760746282,13.3954305468035,
129.413659236035)) ;
#120134=CARTESIAN_POINT('Ctrl Pts',(-28.755360314267,13.6647721239679,129.38282410996)) ;
#120135=CARTESIAN_POINT('Ctrl Pts',(-28.7333793249386,13.9166503672092,
129.285510438486)) ;
#120136=CARTESIAN_POINT('Ctrl Pts',(-28.6908631010797,14.1333087824096,
129.128178523878)) ;
#120137=CARTESIAN_POINT('Ctrl Pts',(-28.631815323096,14.2989356836214,128.92263834171)) ;
#120138=CARTESIAN_POINT('Ctrl Pts',(-28.5603207260596,14.4025578145927,
128.680426107688)) ;
#120139=CARTESIAN_POINT('Ctrl Pts',(-28.4838362884011,14.435010397795,128.424069767306)) ;
#120140=CARTESIAN_POINT('Ctrl Pts',(-28.4071576842928,14.3956728080676,
128.166931596484)) ;
#120141=CARTESIAN_POINT('Ctrl Pts',(-28.3370017645789,14.2862787578303,
127.928842877525)) ;
#120142=CARTESIAN_POINT('Ctrl Pts',(-28.2792160505065,14.1158603541274,
127.726999055007)) ;
#120143=CARTESIAN_POINT('Ctrl Pts',(-28.2382140420626,13.8934485383183,
127.573842062006)) ;
#120144=CARTESIAN_POINT('Ctrl Pts',(-28.2184282359382,13.6404741399982,
127.483121945596)) ;
#120145=CARTESIAN_POINT('Ctrl Pts',(-28.2214053844835,13.3695007340468,
127.458564725998)) ;
#120146=CARTESIAN_POINT('Ctrl Pts',(-28.2477631811765,13.1044457267252,
127.502577894106)) ;
#120147=CARTESIAN_POINT('Ctrl Pts',(-28.2964489975592,12.860704031683,127.611635359131)) ;
#120148=CARTESIAN_POINT('Ctrl Pts',(-28.3649814444321,12.6571154777524,
127.778593699813)) ;
#120149=CARTESIAN_POINT('Ctrl Pts',(-28.4481291111947,12.5098080554844,
127.988544765476)) ;
#120150=CARTESIAN_POINT('Ctrl Pts',(-28.5418583608862,12.4266891530237,
128.229200937591)) ;
#120151=CARTESIAN_POINT('Ctrl Pts',(-28.6399407697042,12.4154229755217,
128.482506199842)) ;
#120152=CARTESIAN_POINT('Ctrl Pts',(-28.7352169858173,12.4759770673935,
128.727836179184)) ;
#120153=CARTESIAN_POINT('Ctrl Pts',(-28.8228149902792,12.6048252394354,
128.950521636392)) ;
#120154=CARTESIAN_POINT('Ctrl Pts',(-28.8963412616457,12.7921645634063,
129.132187511211)) ;
#120155=CARTESIAN_POINT('Ctrl Pts',(-28.9515184485553,13.0247862212583,
129.260231591874)) ;
#120156=CARTESIAN_POINT('Ctrl Pts',(-28.9850885525312,13.2853105369572,
129.32523875102)) ;
#120157=CARTESIAN_POINT('Ctrl Pts',(-28.9954065225807,13.5574331010645,
129.322098562288)) ;
#120158=CARTESIAN_POINT('Ctrl Pts',(-28.9825283726118,13.8171021403353,
129.25156605101)) ;
#120159=CARTESIAN_POINT('Ctrl Pts',(-28.9478762234082,14.0511738702826,
129.117077385573)) ;
#120160=CARTESIAN_POINT('Ctrl Pts',(-28.8949326798189,14.2388281925165,
128.929344352938)) ;
#120161=CARTESIAN_POINT('Ctrl Pts',(-28.828125303218,14.3685839243643,128.701078224462)) ;
#120162=CARTESIAN_POINT('Ctrl Pts',(-28.7525343917434,14.430551147229,128.446989494862)) ;
#120163=CARTESIAN_POINT('Ctrl Pts',(-28.6754264311018,14.4203097396042,
128.188791679093)) ;
#120164=CARTESIAN_POINT('Ctrl Pts',(-28.601689417703,14.3384208186475,127.940147389365)) ;
#120165=CARTESIAN_POINT('Ctrl Pts',(-28.5383525180067,14.191573192343,127.722090576029)) ;
#120166=CARTESIAN_POINT('Ctrl Pts',(-28.4899549480932,13.9880715249732,
127.54740004093)) ;
#120167=CARTESIAN_POINT('Ctrl Pts',(-28.461455990991,13.74717256078,127.431293609618)) ;
#120168=CARTESIAN_POINT('Ctrl Pts',(-28.4548916951247,13.4800206517718,
127.378832045014)) ;
#120169=CARTESIAN_POINT('Ctrl Pts',(-28.4717642598864,13.2110030826081,
127.395134058574)) ;
#120170=CARTESIAN_POINT('Ctrl Pts',(-28.5118855531922,12.9547749192264,
127.479026596824)) ;
#120171=CARTESIAN_POINT('Ctrl Pts',(-28.5724326667241,12.7344342414435,
127.622910019624)) ;
#120172=CARTESIAN_POINT('Ctrl Pts',(-28.650317058003,12.56234537382,127.817305812651)) ;
#120173=CARTESIAN_POINT('Ctrl Pts',(-28.74066209986,12.4518692107331,128.048078349045)) ;
#120174=CARTESIAN_POINT('Ctrl Pts',(-28.8377298890326,12.4112334908308,
128.298449197418)) ;
#120175=CARTESIAN_POINT('Ctrl Pts',(-28.9346899869299,12.4427491476605,
128.548685461757)) ;
#120176=CARTESIAN_POINT('Ctrl Pts',(-29.026695800843,12.5456206788136,128.784107137465)) ;
#120177=CARTESIAN_POINT('Ctrl Pts',(-29.1057500300418,12.7091960260598,
128.982208076137)) ;
#120178=CARTESIAN_POINT('Ctrl Pts',(-29.1691703048475,12.9259029784642,
129.134208867658)) ;
#120179=CARTESIAN_POINT('Ctrl Pts',(-29.2117208860627,13.1770736213742,
129.225453280615)) ;
#120180=CARTESIAN_POINT('Ctrl Pts',(-29.2316474006686,13.4468768316793,
129.250461675935)) ;
#120181=CARTESIAN_POINT('Ctrl Pts',(-29.2280321901409,13.7138795758086,
129.206844028161)) ;
#120182=CARTESIAN_POINT('Ctrl Pts',(-29.2019668400944,13.9605431797111,
129.097577657237)) ;
#120183=CARTESIAN_POINT('Ctrl Pts',(-29.1560907287724,14.1686235448508,
128.93047945117)) ;
#120184=CARTESIAN_POINT('Ctrl Pts',(-29.0938859718026,14.324111265305,128.715458048821)) ;
#120185=CARTESIAN_POINT('Ctrl Pts',(-29.0216022718212,14.4138215777412,
128.47131600094)) ;
#120186=CARTESIAN_POINT('Ctrl Pts',(-28.944139044341,14.4331945078177,128.211849645434)) ;
#120187=CARTESIAN_POINT('Ctrl Pts',(-28.868380940979,14.3801614828431,127.957470568784)) ;
#120188=CARTESIAN_POINT('Ctrl Pts',(-28.800081494987,14.2584942969663,127.724797795054)) ;
#120189=CARTESIAN_POINT('Ctrl Pts',(-28.745111686049,14.0770491987957,127.53109904534)) ;
#120190=CARTESIAN_POINT('Ctrl Pts',(-28.7080026400916,13.848487543227,127.389532493275)) ;
#120191=CARTESIAN_POINT('Ctrl Pts',(-28.6922955186714,13.5893550911286,
127.310487333215)) ;
#120192=CARTESIAN_POINT('Ctrl Pts',(-28.6996680149708,13.3196922711331,
127.299032447349)) ;
#120193=CARTESIAN_POINT('Ctrl Pts',(-28.7303957431008,13.0561134153821,
127.355639856244)) ;
#120194=CARTESIAN_POINT('Ctrl Pts',(-28.783028433985,12.8190741584449,127.476267047352)) ;
#120195=CARTESIAN_POINT('Ctrl Pts',(-28.8545049403867,12.6252976289265,
127.651936636573)) ;
#120196=CARTESIAN_POINT('Ctrl Pts',(-28.9403481121036,12.4887797079064,
127.869606581264)) ;
#120197=CARTESIAN_POINT('Ctrl Pts',(-29.0353127838495,12.4190606508798,
128.113884387687)) ;
#120198=CARTESIAN_POINT('Ctrl Pts',(-29.1331482649175,12.4213023279721,
128.366577035473)) ;
#120199=CARTESIAN_POINT('Ctrl Pts',(-29.2277424750904,12.4953372291496,
128.609768490982)) ;
#120200=CARTESIAN_POINT('Ctrl Pts',(-29.3129071860777,12.6358732815743,
128.825428028507)) ;
#120201=CARTESIAN_POINT('Ctrl Pts',(-29.3832462389174,12.8325869424309,
128.997810327091)) ;
#120202=CARTESIAN_POINT('Ctrl Pts',(-29.4345967551139,13.0715962372375,
129.114709675196)) ;
#120203=CARTESIAN_POINT('Ctrl Pts',(-29.4639745688401,13.3366928582969,
129.167311129979)) ;
#120204=CARTESIAN_POINT('Ctrl Pts',(-29.4698439499065,13.6067853722367,
129.151391357745)) ;
#120205=CARTESIAN_POINT('Ctrl Pts',(-29.4526874804027,13.8640946743987,
129.068158319223)) ;
#120206=CARTESIAN_POINT('Ctrl Pts',(-29.4144385458815,14.0898397345162,
128.923322495705)) ;
#120207=CARTESIAN_POINT('Ctrl Pts',(-29.3582660699698,14.268360163449,128.725993376795)) ;
#120208=CARTESIAN_POINT('Ctrl Pts',(-29.2895954148743,14.3854877174078,
128.492376850714)) ;
#120209=CARTESIAN_POINT('Ctrl Pts',(-29.2131004108755,14.4341894579408,
128.235640638085)) ;
#120210=CARTESIAN_POINT('Ctrl Pts',(-29.1361690586815,14.4102459856392,
127.977913367037)) ;
#120211=CARTESIAN_POINT('Ctrl Pts',(-29.0640642794503,14.3157190540823,
127.734130630897)) ;
#120212=CARTESIAN_POINT('Ctrl Pts',(-29.0031320933351,14.1574302983803,
127.523047652384)) ;
#120213=CARTESIAN_POINT('Ctrl Pts',(-28.9581862068265,13.9458829104796,
127.358546519961)) ;
#120214=CARTESIAN_POINT('Ctrl Pts',(-28.9334884683389,13.6969896287775,
127.253241196933)) ;
#120215=CARTESIAN_POINT('Ctrl Pts',(-28.9314300219935,13.429280378355,127.214164558102)) ;
#120216=CARTESIAN_POINT('Ctrl Pts',(-28.9526326503617,13.1613091049485,
127.243072438753)) ;
#120217=CARTESIAN_POINT('Ctrl Pts',(-28.997044137834,12.9096301880815,127.339433446245)) ;
#120218=CARTESIAN_POINT('Ctrl Pts',(-29.0610782818279,12.6977069165648,
127.493539578836)) ;
#120219=CARTESIAN_POINT('Ctrl Pts',(-29.1418943597176,12.5361591796786,
127.696427432701)) ;
#120220=CARTESIAN_POINT('Ctrl Pts',(-29.2337136946606,12.4388403136538,
127.931597574254)) ;
#120221=CARTESIAN_POINT('Ctrl Pts',(-29.3310681473004,12.4115721831835,
128.182896743448)) ;
#120222=CARTESIAN_POINT('Ctrl Pts',(-29.4279117173817,12.457029412505,128.432608286614)) ;
#120223=CARTESIAN_POINT('Ctrl Pts',(-29.5173477265947,12.5713337507617,
128.660826716096)) ;
#120224=CARTESIAN_POINT('Ctrl Pts',(-29.5943927463647,12.7468028515201,
128.85275594632)) ;
#120225=CARTESIAN_POINT('Ctrl Pts',(-29.6540334361348,12.9715572990884,
128.993752857509)) ;
#120226=CARTESIAN_POINT('Ctrl Pts',(-29.6923944387496,13.2272671330663,
129.072781238289)) ;
#120227=CARTESIAN_POINT('Ctrl Pts',(-29.7078462688087,13.498061880378,129.084740514306)) ;
#120228=CARTESIAN_POINT('Ctrl Pts',(-29.6999381855932,13.762097452862,129.028647095151)) ;
#120229=CARTESIAN_POINT('Ctrl Pts',(-29.6697605913369,14.0037249073099,
128.907237756829)) ;
#120230=CARTESIAN_POINT('Ctrl Pts',(-29.6205659297938,14.2024000350369,
128.730490540037)) ;
#120231=CARTESIAN_POINT('Ctrl Pts',(-29.5559329643647,14.3463072876563,
128.508387624656)) ;
#120232=CARTESIAN_POINT('Ctrl Pts',(-29.4823645066708,14.4229407115658,
128.260528386984)) ;
#120233=CARTESIAN_POINT('Ctrl Pts',(-29.4047568399833,14.428708721228,128.000665028461)) ;
#120234=CARTESIAN_POINT('Ctrl Pts',(-29.3299052093241,14.3623691718519,
127.748905053254)) ;
#120235=CARTESIAN_POINT('Ctrl Pts',(-29.2635733327006,14.2283779712588,
127.521922192701)) ;
#120236=CARTESIAN_POINT('Ctrl Pts',(-29.2116294286318,14.036425640657,127.336998499882)) ;
#120237=CARTESIAN_POINT('Ctrl Pts',(-29.1785287843388,13.8020944878478,
127.20733035862)) ;
#120238=CARTESIAN_POINT('Ctrl Pts',(-29.1669905292766,13.539161382227,127.140439495721)) ;
#120239=CARTESIAN_POINT('Ctrl Pts',(-29.178814380148,13.2686186839106,127.141894532802)) ;
#120240=CARTESIAN_POINT('Ctrl Pts',(-29.2138972997033,13.008641923509,127.211221309632)) ;
#120241=CARTESIAN_POINT('Ctrl Pts',(-29.2701600634812,12.7791080577395,
127.342548185939)) ;
#120242=CARTESIAN_POINT('Ctrl Pts',(-29.3451121464908,12.594297732826,127.528205753968)) ;
#120243=CARTESIAN_POINT('Ctrl Pts',(-29.4328863736172,12.4702970553751,
127.751610486133)) ;
#120244=CARTESIAN_POINT('Ctrl Pts',(-29.5289609200398,12.4139049863059,
127.999100927029)) ;
#120245=CARTESIAN_POINT('Ctrl Pts',(-29.6264420292929,12.4297924309748,
128.250830535367)) ;
#120246=CARTESIAN_POINT('Ctrl Pts',(-29.7200486139469,12.5172147404821,
128.491019322346)) ;
#120247=CARTESIAN_POINT('Ctrl Pts',(-29.8027908234805,12.6696685741938,
128.699585054602)) ;
#120248=CARTESIAN_POINT('Ctrl Pts',(-29.86960716835,12.8748935986054,128.861784028226)) ;
#120249=CARTESIAN_POINT('Ctrl Pts',(-29.9170704992435,13.1206629289391,
128.96724565317)) ;
#120250=CARTESIAN_POINT('Ctrl Pts',(-29.9419865656854,13.3874986938653,
129.006931376291)) ;
#120251=CARTESIAN_POINT('Ctrl Pts',(-29.9434479075333,13.6577700467963,
128.977987103776)) ;
#120252=CARTESIAN_POINT('Ctrl Pts',(-29.9220034023051,13.9102263569756,
128.882245404659)) ;
#120253=CARTESIAN_POINT('Ctrl Pts',(-29.8802551960757,14.1273421335156,
128.72730034782)) ;
#120254=CARTESIAN_POINT('Ctrl Pts',(-29.8212425120714,14.2954362023137,
128.521660521602)) ;
#120255=CARTESIAN_POINT('Ctrl Pts',(-29.7506442887973,14.4001990478318,
128.282366797653)) ;
#120256=CARTESIAN_POINT('Ctrl Pts',(-29.6735305499138,14.4351706372086,
128.023853901931)) ;
#120257=CARTESIAN_POINT('Ctrl Pts',(-29.5971911919457,14.3977719556556,
127.767894141714)) ;
#120258=CARTESIAN_POINT('Ctrl Pts',(-29.5266046143525,14.2904204336126,
127.52849106087)) ;
#120259=CARTESIAN_POINT('Ctrl Pts',(-29.4682437641198,14.1205426251184,
127.324825254044)) ;
#120260=CARTESIAN_POINT('Ctrl Pts',(-29.4270858956956,13.9015880320261,
127.171546539802)) ;
#120261=CARTESIAN_POINT('Ctrl Pts',(-29.4064486644553,13.6483197654843,
127.078182317743)) ;
#120262=CARTESIAN_POINT('Ctrl Pts',(-29.4087637384098,13.3774460111694,
127.051688016783)) ;
#120263=CARTESIAN_POINT('Ctrl Pts',(-29.4345154694378,13.1115164178379,
127.093866825116)) ;
#120264=CARTESIAN_POINT('Ctrl Pts',(-29.4824944581263,12.8676277530858,
127.200952673646)) ;
#120265=CARTESIAN_POINT('Ctrl Pts',(-29.550167305721,12.6630941709717,127.365518735153)) ;
#120266=CARTESIAN_POINT('Ctrl Pts',(-29.6335215314997,12.5128296668561,
127.575832626601)) ;
#120267=CARTESIAN_POINT('Ctrl Pts',(-29.7270496687932,12.4280522223888,
127.815913080995)) ;
#120268=CARTESIAN_POINT('Ctrl Pts',(-29.8249308027257,12.4147676725694,
128.068684706927)) ;
#120269=CARTESIAN_POINT('Ctrl Pts',(-29.9203761314657,12.4732052197203,
128.314506929665)) ;
#120270=CARTESIAN_POINT('Ctrl Pts',(-30.0085723311821,12.6008830294735,
128.538819105028)) ;
#120271=CARTESIAN_POINT('Ctrl Pts',(-30.0821509332757,12.7859100383565,
128.720804533574)) ;
#120272=CARTESIAN_POINT('Ctrl Pts',(-30.1379378808088,13.0171549996097,
128.850651951648)) ;
#120273=CARTESIAN_POINT('Ctrl Pts',(-30.1722068319512,13.277402414091,128.917662123442)) ;
#120274=CARTESIAN_POINT('Ctrl Pts',(-30.1832432181997,13.549209197848,128.916661399848)) ;
#120275=CARTESIAN_POINT('Ctrl Pts',(-30.170957178296,13.8101282641669,128.847760730607)) ;
#120276=CARTESIAN_POINT('Ctrl Pts',(-30.1371083316874,14.0442616351561,
128.71578111202)) ;
#120277=CARTESIAN_POINT('Ctrl Pts',(-30.0842285549006,14.234899690822,128.527971711439)) ;
#120278=CARTESIAN_POINT('Ctrl Pts',(-30.0180483211186,14.3654882849947,
128.301716969827)) ;
#120279=CARTESIAN_POINT('Ctrl Pts',(-29.9428222189424,14.4297229165876,
128.048768110306)) ;
#120280=CARTESIAN_POINT('Ctrl Pts',(-29.8654274323927,14.4216680213317,
127.789621318339)) ;
#120281=CARTESIAN_POINT('Ctrl Pts',(-29.7914651714803,14.3417421219821,
127.540312299338)) ;
#120282=CARTESIAN_POINT('Ctrl Pts',(-29.7277501313066,14.1964291634702,
127.321124596841)) ;
#120283=CARTESIAN_POINT('Ctrl Pts',(-29.6790443731307,13.9955519017587,
127.14571179308)) ;
#120284=CARTESIAN_POINT('Ctrl Pts',(-29.6497008058792,13.7541464807844,
127.026926907722)) ;
#120285=CARTESIAN_POINT('Ctrl Pts',(-29.6425598616829,13.4873870948836,
126.972790757272)) ;
#120286=CARTESIAN_POINT('Ctrl Pts',(-29.6587539231936,13.2187119173844,
126.987166006195)) ;
#120287=CARTESIAN_POINT('Ctrl Pts',(-29.6980947341361,12.9622340564561,
127.068847518659)) ;
#120288=CARTESIAN_POINT('Ctrl Pts',(-29.7583490440813,12.7396655137431,
127.211726679847)) ;
#120289=CARTESIAN_POINT('Ctrl Pts',(-29.8358320612097,12.5663130240366,
127.404966419517)) ;
#120290=CARTESIAN_POINT('Ctrl Pts',(-29.9255031103164,12.4542929808878,
127.63390856035)) ;
#120291=CARTESIAN_POINT('Ctrl Pts',(-30.0227989228316,12.4113060989113,
127.884830805057)) ;
#120292=CARTESIAN_POINT('Ctrl Pts',(-30.1196650413285,12.4409729751149,
128.134843722716)) ;
#120293=CARTESIAN_POINT('Ctrl Pts',(-30.2114579250078,12.5408195806537,
128.369838112703)) ;
#120294=CARTESIAN_POINT('Ctrl Pts',(-30.2918439177153,12.7045177195062,
128.571453811166)) ;
#120295=CARTESIAN_POINT('Ctrl Pts',(-30.3554107241379,12.9194126835292,
128.72401886233)) ;
#120296=CARTESIAN_POINT('Ctrl Pts',(-30.3985397348488,13.1689179450109,
128.817052685138)) ;
#120297=CARTESIAN_POINT('Ctrl Pts',(-30.4192259543522,13.4397285799231,
128.844127725907)) ;
#120298=CARTESIAN_POINT('Ctrl Pts',(-30.4162235857149,13.706427055275,128.802376016593)) ;
#120299=CARTESIAN_POINT('Ctrl Pts',(-30.390798293272,13.953886295735,128.694986871854)) ;
#120300=CARTESIAN_POINT('Ctrl Pts',(-30.3454805345728,14.1631927592464,
128.529541646648)) ;
#120301=CARTESIAN_POINT('Ctrl Pts',(-30.2836235435482,14.3205261176051,
128.315510393234)) ;
#120302=CARTESIAN_POINT('Ctrl Pts',(-30.2116675009614,14.4121066452954,
128.072370546642)) ;
#120303=CARTESIAN_POINT('Ctrl Pts',(-30.1341996677374,14.4337042741575,
127.812865461492)) ;
#120304=CARTESIAN_POINT('Ctrl Pts',(-30.0582302123766,14.3826278175705,
127.557833074158)) ;
#120305=CARTESIAN_POINT('Ctrl Pts',(-29.9896723229114,14.2628852550259,
127.324425469218)) ;
#120306=CARTESIAN_POINT('Ctrl Pts',(-29.934234898034,14.08292617671,127.129348096737)) ;
#120307=CARTESIAN_POINT('Ctrl Pts',(-29.8965848388362,13.8556922014923,
126.986230563461)) ;
#120308=CARTESIAN_POINT('Ctrl Pts',(-29.8802335079759,13.597259905774,126.905308621401)) ;
#120309=CARTESIAN_POINT('Ctrl Pts',(-29.8868422446893,13.3277679144463,
126.891640117567)) ;
#120310=CARTESIAN_POINT('Ctrl Pts',(-29.9172565235401,13.0618109735796,
126.947077950778)) ;
#120311=CARTESIAN_POINT('Ctrl Pts',(-29.9688720822212,12.826038953014,127.065042300501)) ;
#120312=CARTESIAN_POINT('Ctrl Pts',(-30.040080879908,12.6298696524396,127.239794218177)) ;
#120313=CARTESIAN_POINT('Ctrl Pts',(-30.1255602392865,12.4917687507878,
127.456424992923)) ;
#120314=CARTESIAN_POINT('Ctrl Pts',(-30.2204632585728,12.4199839299598,
127.700481429544)) ;
#120315=CARTESIAN_POINT('Ctrl Pts',(-30.3182500980047,12.4203084245316,
127.95305004317)) ;
#120316=CARTESIAN_POINT('Ctrl Pts',(-30.4128724280061,12.4922084684858,
128.196377152701)) ;
#120317=CARTESIAN_POINT('Ctrl Pts',(-30.49843532704,12.6309969485081,128.41318204901)) ;
#120318=CARTESIAN_POINT('Ctrl Pts',(-30.5692955798566,12.8263311670906,
128.587075933282)) ;
#120319=CARTESIAN_POINT('Ctrl Pts',(-30.6213552229333,13.0651228622206,
128.70594980504)) ;
#120320=CARTESIAN_POINT('Ctrl Pts',(-30.6512588718474,13.3295668395412,
128.760119376466)) ;
#120321=CARTESIAN_POINT('Ctrl Pts',(-30.6577918154966,13.5989124476963,
128.74624101031)) ;
#120322=CARTESIAN_POINT('Ctrl Pts',(-30.6412326417354,13.8574711293399,
128.664673013124)) ;
#120323=CARTESIAN_POINT('Ctrl Pts',(-30.6036128903169,14.0837079504238,
128.521760497902)) ;
#120324=CARTESIAN_POINT('Ctrl Pts',(-30.5479910114117,14.2638192247761,
128.326070390643)) ;
#120325=CARTESIAN_POINT('Ctrl Pts',(-30.4793810094137,14.3831695883009,
128.092520856271)) ;
#120326=CARTESIAN_POINT('Ctrl Pts',(-30.4032580708324,14.4337176696405,
127.836981571003)) ;
#120327=CARTESIAN_POINT('Ctrl Pts',(-30.3262283514109,14.4120588650256,
127.578950633389)) ;
#120328=CARTESIAN_POINT('Ctrl Pts',(-30.2538014263296,14.3193772960994,
127.33418534272)) ;
#120329=CARTESIAN_POINT('Ctrl Pts',(-30.1924345633591,14.162817091715,127.121826574969)) ;
#120330=CARTESIAN_POINT('Ctrl Pts',(-30.1468826625933,13.9515916217657,
126.955425970421)) ;
#120331=CARTESIAN_POINT('Ctrl Pts',(-30.1217285110034,13.7055233203187,
126.849053547207)) ;
#120332=CARTESIAN_POINT('Ctrl Pts',(-30.1189617700997,13.4359481909895,
126.80763240538)) ;
#120333=CARTESIAN_POINT('Ctrl Pts',(-30.1394921596568,13.1690262543573,
126.834739626026)) ;
#120334=CARTESIAN_POINT('Ctrl Pts',(-30.1832810972736,12.9162728223831,
126.929246732316)) ;
#120335=CARTESIAN_POINT('Ctrl Pts',(-30.2466242328709,12.7036779666449,
127.081423572812)) ;
#120336=CARTESIAN_POINT('Ctrl Pts',(-30.3268550662309,12.5403117621087,
127.282643376759)) ;
#120337=CARTESIAN_POINT('Ctrl Pts',(-30.4190439813045,12.4404489575973,
127.518673248112)) ;
#120338=CARTESIAN_POINT('Ctrl Pts',(-30.515866544653,12.4114485633587,127.768579554242)) ;
#120339=CARTESIAN_POINT('Ctrl Pts',(-30.6127673682806,12.4544846403687,
128.018478798306)) ;
#120340=CARTESIAN_POINT('Ctrl Pts',(-30.7028603542064,12.5672617699685,
128.248489335384)) ;
#120341=CARTESIAN_POINT('Ctrl Pts',(-30.7803844158743,12.7417744927464,
128.441755685078)) ;
#120342=CARTESIAN_POINT('Ctrl Pts',(-30.8401391858009,12.9633750836739,
128.583364940552)) ;
#120343=CARTESIAN_POINT('Ctrl Pts',(-30.8795034723959,13.2203111794704,
128.665063657192)) ;
#120344=CARTESIAN_POINT('Ctrl Pts',(-30.8955070246914,13.4905143785451,
128.678700860762)) ;
#120345=CARTESIAN_POINT('Ctrl Pts',(-30.8882329130397,13.7550216610133,
128.624443878034)) ;
#120346=CARTESIAN_POINT('Ctrl Pts',(-30.8587969553298,13.996749630301,128.505328670453)) ;
#120347=CARTESIAN_POINT('Ctrl Pts',(-30.8099826456517,14.1974242710986,
128.32959702307)) ;
#120348=CARTESIAN_POINT('Ctrl Pts',(-30.746033869509,14.342514003419,128.109651994141)) ;
#120349=CARTESIAN_POINT('Ctrl Pts',(-30.6724714145086,14.4218015954934,
127.861707426972)) ;
#120350=CARTESIAN_POINT('Ctrl Pts',(-30.5944934945582,14.4294553492896,
127.600600448985)) ;
#120351=CARTESIAN_POINT('Ctrl Pts',(-30.5198525735962,14.3652618267525,
127.349613410191)) ;
#120352=CARTESIAN_POINT('Ctrl Pts',(-30.4532723078222,14.2335996642439,
127.121966229449)) ;
#120353=CARTESIAN_POINT('Ctrl Pts',(-30.400742576325,14.0430658671341,126.93529354313)) ;
#120354=CARTESIAN_POINT('Ctrl Pts',(-30.3669424476525,13.8093138339715,
126.803511541699)) ;
#120355=CARTESIAN_POINT('Ctrl Pts',(-30.354795918861,13.5459139250659,126.734726092536)) ;
#120356=CARTESIAN_POINT('Ctrl Pts',(-30.3659155625559,13.2769103570782,
126.734315819249)) ;
#120357=CARTESIAN_POINT('Ctrl Pts',(-30.4002899633489,13.0160046226691,
126.801538967899)) ;
#120358=CARTESIAN_POINT('Ctrl Pts',(-30.4561214089056,12.7850161242088,
126.931542490534)) ;
#120359=CARTESIAN_POINT('Ctrl Pts',(-30.5303244371711,12.5991696001074,
127.115126201843)) ;
#120360=CARTESIAN_POINT('Ctrl Pts',(-30.6182424052493,12.4727066695535,
127.338777065082)) ;
#120361=CARTESIAN_POINT('Ctrl Pts',(-30.7137149498342,12.4146340063818,
127.584672937593)) ;
#120362=CARTESIAN_POINT('Ctrl Pts',(-30.8114490602173,12.428272476576,127.837066661156)) ;
#120363=CARTESIAN_POINT('Ctrl Pts',(-30.9051543854586,12.5136822248399,
128.077582546125)) ;
#120364=CARTESIAN_POINT('Ctrl Pts',(-30.9882709083332,12.6640313971838,
128.287268615616)) ;
#120365=CARTESIAN_POINT('Ctrl Pts',(-31.0559950168127,12.8694014453016,
128.451897209542)) ;
#120366=CARTESIAN_POINT('Ctrl Pts',(-31.1037081705792,13.1128473541502,
128.558297704285)) ;
#120367=CARTESIAN_POINT('Ctrl Pts',(-31.1293772881811,13.3794713860966,
128.600156033917)) ;
#120368=CARTESIAN_POINT('Ctrl Pts',(-31.1315196171046,13.6493875676937,
128.573268454256)) ;
#120369=CARTESIAN_POINT('Ctrl Pts',(-31.1108449632028,13.9027716863457,
128.479778740659)) ;
#120370=CARTESIAN_POINT('Ctrl Pts',(-31.0692426036565,14.1226003969304,
128.325000641813)) ;
#120371=CARTESIAN_POINT('Ctrl Pts',(-31.0112252737707,14.2907614924808,
128.122596061958)) ;
#120372=CARTESIAN_POINT('Ctrl Pts',(-30.9402723144273,14.3985142703266,
127.881958087952)) ;
#120373=CARTESIAN_POINT('Ctrl Pts',(-30.8637496257416,14.4350393250072,
127.625400924029)) ;
#120374=CARTESIAN_POINT('Ctrl Pts',(-30.7871752359977,14.4000355933247,
127.368694626451)) ;
#120375=CARTESIAN_POINT('Ctrl Pts',(-30.7160918334904,14.294019258596,127.127722701532)) ;
#120376=CARTESIAN_POINT('Ctrl Pts',(-30.6575855213183,14.1264036808229,
126.923771105405)) ;
#120377=CARTESIAN_POINT('Ctrl Pts',(-30.6157646948906,13.9087136081249,
126.768534501323)) ;
#120378=CARTESIAN_POINT('Ctrl Pts',(-30.5944734643708,13.6545233409047,
126.673056840974)) ;
#120379=CARTESIAN_POINT('Ctrl Pts',(-30.5961584778505,13.3858501132774,
126.644972706391)) ;
#120380=CARTESIAN_POINT('Ctrl Pts',(-30.6212061225492,13.1190055325829,
126.685027414806)) ;
#120381=CARTESIAN_POINT('Ctrl Pts',(-30.6686641032527,12.8738785417747,
126.790545968904)) ;
#120382=CARTESIAN_POINT('Ctrl Pts',(-30.7360322995194,12.6676053740016,
126.954141574344)) ;
#120383=CARTESIAN_POINT('Ctrl Pts',(-30.8189572758642,12.5160771056389,
127.163246420767)) ;
#120384=CARTESIAN_POINT('Ctrl Pts',(-30.9118318570724,12.4297444721253,
127.40156977474)) ;
#120385=CARTESIAN_POINT('Ctrl Pts',(-31.0095674663916,12.4139325819383,
127.653954416377)) ;
#120386=CARTESIAN_POINT('Ctrl Pts',(-31.1057144053207,12.4708186398046,
127.901626272861)) ;
#120387=CARTESIAN_POINT('Ctrl Pts',(-31.1934774018543,12.5954481483175,
128.124964799178)) ;
#120388=CARTESIAN_POINT('Ctrl Pts',(-31.2680184404151,12.7795463119932,
128.309584536972)) ;
#120389=CARTESIAN_POINT('Ctrl Pts',(-31.3245129839954,13.0105018776207,
128.441401948698)) ;
#120390=CARTESIAN_POINT('Ctrl Pts',(-31.359387232688,13.270465957133,128.510149434695)) ;
#120391=CARTESIAN_POINT('Ctrl Pts',(-31.3710208627504,13.5415025070648,
128.510982049493)) ;
#120392=CARTESIAN_POINT('Ctrl Pts',(-31.3594362504754,13.8030870082756,
128.444123195626)) ;
#120393=CARTESIAN_POINT('Ctrl Pts',(-31.3259082937146,14.0389747692379,
128.312940546262)) ;
#120394=CARTESIAN_POINT('Ctrl Pts',(-31.274151313902,14.2290324339817,128.128800353418)) ;
#120395=CARTESIAN_POINT('Ctrl Pts',(-31.2077956141783,14.36290013857,127.901741927386)) ;
#120396=CARTESIAN_POINT('Ctrl Pts',(-31.1328753029658,14.4288302738408,
127.649767710556)) ;
#120397=CARTESIAN_POINT('Ctrl Pts',(-31.0553096740806,14.4228365201876,
127.390047882109)) ;
#120398=CARTESIAN_POINT('Ctrl Pts',(-30.9814127467324,14.3452102352826,
127.141053050896)) ;
#120399=CARTESIAN_POINT('Ctrl Pts',(-30.9171598071708,14.2014203196955,
126.9202098087)) ;
#120400=CARTESIAN_POINT('Ctrl Pts',(-30.8680211029908,14.0021641937243,
126.743575143318)) ;
#120401=CARTESIAN_POINT('Ctrl Pts',(-30.8380540025779,13.761753127779,126.622966733671)) ;
#120402=CARTESIAN_POINT('Ctrl Pts',(-30.8302076181397,13.4956080237515,
126.566793461782)) ;
#120403=CARTESIAN_POINT('Ctrl Pts',(-30.8457646914712,13.2262845852455,
126.57924205912)) ;
#120404=CARTESIAN_POINT('Ctrl Pts',(-30.8843106921691,12.9698876950621,
126.658709006147)) ;
#120405=CARTESIAN_POINT('Ctrl Pts',(-30.944061629397,12.7457364087332,126.80006264788)) ;
#120406=CARTESIAN_POINT('Ctrl Pts',(-31.0209111245848,12.5708017503329,
126.991514652388)) ;
#120407=CARTESIAN_POINT('Ctrl Pts',(-31.1111509504485,12.4561497112336,
127.22181232647)) ;
#120408=CARTESIAN_POINT('Ctrl Pts',(-31.2072870600816,12.4116404870858,
127.469715093214)) ;
#120409=CARTESIAN_POINT('Ctrl Pts',(-31.3050010050222,12.4391729336107,
127.721936631105)) ;
#120410=CARTESIAN_POINT('Ctrl Pts',(-31.3967596844395,12.5371797633224,
127.956923250406)) ;
#120411=CARTESIAN_POINT('Ctrl Pts',(-31.4773182773982,12.6985743471033,
128.159141476881)) ;
#120412=CARTESIAN_POINT('Ctrl Pts',(-31.5414906076439,12.9117741360547,
128.313504581612)) ;
#120413=CARTESIAN_POINT('Ctrl Pts',(-31.585503955842,13.1624013152274,128.408873091849)) ;
#120414=CARTESIAN_POINT('Ctrl Pts',(-31.6066735180883,13.4305279145417,
128.437664751368)) ;
#120415=CARTESIAN_POINT('Ctrl Pts',(-31.6044537914995,13.6988963516455,
128.398030332128)) ;
#120416=CARTESIAN_POINT('Ctrl Pts',(-31.5796185454552,13.9472005386101,
128.292368550419)) ;
#120417=CARTESIAN_POINT('Ctrl Pts',(-31.5347333532356,14.1580510630495,
128.128132874519)) ;
#120418=CARTESIAN_POINT('Ctrl Pts',(-31.4735536013256,14.3165352363587,
127.916224911136)) ;
#120419=CARTESIAN_POINT('Ctrl Pts',(-31.4014686925056,14.4105996668628,
127.672535798014)) ;
#120420=CARTESIAN_POINT('Ctrl Pts',(-31.3242683799976,14.4340684651961,
127.413909039428)) ;
#120421=CARTESIAN_POINT('Ctrl Pts',(-31.2480468687016,14.3850543896185,
127.158084753529)) ;
#120422=CARTESIAN_POINT('Ctrl Pts',(-31.1792019153545,14.2669952300402,
126.923831913409)) ;
#120423=CARTESIAN_POINT('Ctrl Pts',(-31.1234652774576,14.0891154364107,
126.727970581063)) ;
#120424=CARTESIAN_POINT('Ctrl Pts',(-31.085171594464,13.8629228835357,126.582943522854)) ;
#120425=CARTESIAN_POINT('Ctrl Pts',(-31.0681428284109,13.6044943724102,
126.499966250038)) ;
#120426=CARTESIAN_POINT('Ctrl Pts',(-31.0741800776185,13.3352195562946,
126.484640586543)) ;
#120427=CARTESIAN_POINT('Ctrl Pts',(-31.1036139777116,13.0705829535361,
126.537450591183)) ;
#120428=CARTESIAN_POINT('Ctrl Pts',(-31.1549987786636,12.8316692334543,
126.654458606324)) ;
#120429=CARTESIAN_POINT('Ctrl Pts',(-31.2258684738244,12.6342706260099,
126.828204708944)) ;
#120430=CARTESIAN_POINT('Ctrl Pts',(-31.3106811987395,12.4949548036794,
127.043012440284)) ;
#120431=CARTESIAN_POINT('Ctrl Pts',(-31.4054161489351,12.4210676160077,
127.286570115342)) ;
#120432=CARTESIAN_POINT('Ctrl Pts',(-31.5030764584432,12.4192534817676,
127.538810619031)) ;
#120433=CARTESIAN_POINT('Ctrl Pts',(-31.5980505537662,12.4890551014873,
127.783113550799)) ;
#120434=CARTESIAN_POINT('Ctrl Pts',(-31.6842775371184,12.626926545497,128.001711744956)) ;
#120435=CARTESIAN_POINT('Ctrl Pts',(-31.7551540083784,12.8196495679067,
128.175864614223)) ;
#120436=CARTESIAN_POINT('Ctrl Pts',(-31.8079983596213,13.0580836243581,
128.296926865552)) ;
#120437=CARTESIAN_POINT('Ctrl Pts',(-31.8384823645199,13.3214662460235,
128.352872203092)) ;
#120438=CARTESIAN_POINT('Ctrl Pts',(-31.8456998824593,13.5912987745739,
128.340936672021)) ;
#120439=CARTESIAN_POINT('Ctrl Pts',(-31.8299019781677,13.8497219287496,
128.261704525461)) ;
#120440=CARTESIAN_POINT('Ctrl Pts',(-31.7925300527276,14.0789422598233,
128.11924062528)) ;
#120441=CARTESIAN_POINT('Ctrl Pts',(-31.7373879737978,14.2597601138698,
127.925041901496)) ;
#120442=CARTESIAN_POINT('Ctrl Pts',(-31.6693257955755,14.3805241665643,
127.693206235717)) ;
#120443=CARTESIAN_POINT('Ctrl Pts',(-31.5934353598195,14.4333051065353,
127.438389101722)) ;
#120444=CARTESIAN_POINT('Ctrl Pts',(-31.5160410317782,14.4135763153339,
127.179153156744)) ;
#120445=CARTESIAN_POINT('Ctrl Pts',(-31.4434927483479,14.3230159864486,
126.934094834657)) ;
#120446=CARTESIAN_POINT('Ctrl Pts',(-31.3815287161961,14.1669880697449,
126.719814892297)) ;
#120447=CARTESIAN_POINT('Ctrl Pts',(-31.3360156066866,13.9601855092309,
126.554001382575)) ;
#120448=CARTESIAN_POINT('Ctrl Pts',(-31.3098762387133,13.7121979724763,
126.444349827821)) ;
#120449=CARTESIAN_POINT('Ctrl Pts',(-31.3064487554567,13.4453254354835,
126.401311066117)) ;
#120450=CARTESIAN_POINT('Ctrl Pts',(-31.3264783868601,13.1756579328103,
126.42663176511)) ;
#120451=CARTESIAN_POINT('Ctrl Pts',(-31.3691412779122,12.9248371133689,
126.518224267297)) ;
#120452=CARTESIAN_POINT('Ctrl Pts',(-31.4323907266609,12.7087904209721,
126.669825981253)) ;
#120453=CARTESIAN_POINT('Ctrl Pts',(-31.5121877466573,12.5441839973877,
126.869821292532)) ;
#120454=CARTESIAN_POINT('Ctrl Pts',(-31.6040854442531,12.4422953631874,
127.105006082566)) ;
#120455=CARTESIAN_POINT('Ctrl Pts',(-31.7010448696948,12.4112745922159,
127.355243843531)) ;
#120456=CARTESIAN_POINT('Ctrl Pts',(-31.7978537292344,12.4523611240387,
127.604936133107)) ;
#120457=CARTESIAN_POINT('Ctrl Pts',(-31.8879929885489,12.5627156272335,
127.83517884223)) ;
#120458=CARTESIAN_POINT('Ctrl Pts',(-31.9662453401921,12.7362032335438,
128.030450237031)) ;
#120459=CARTESIAN_POINT('Ctrl Pts',(-32.0264300023649,12.9562237014372,
128.17338105447)) ;
#120460=CARTESIAN_POINT('Ctrl Pts',(-32.0664723939883,13.2127632436766,
128.257017275162)) ;
#120461=CARTESIAN_POINT('Ctrl Pts',(-32.0831275048794,13.4814739931662,
128.272723469395)) ;
#120462=CARTESIAN_POINT('Ctrl Pts',(-32.0765932972906,13.7476020769462,
128.220483383446)) ;
#120463=CARTESIAN_POINT('Ctrl Pts',(-32.0476302528579,13.9907502707064,
128.102674626184)) ;
#120464=CARTESIAN_POINT('Ctrl Pts',(-31.9994402533025,14.1921268766281,
127.928863316725)) ;
#120465=CARTESIAN_POINT('Ctrl Pts',(-31.9359462785863,14.3392030436754,
127.710268097422)) ;
#120466=CARTESIAN_POINT('Ctrl Pts',(-31.8619745518175,14.4207500230976,
127.46086515257)) ;
#120467=CARTESIAN_POINT('Ctrl Pts',(-31.7847447622153,14.4302362583739,
127.202259775102)) ;
#120468=CARTESIAN_POINT('Ctrl Pts',(-31.7095328243019,14.368028270843,126.949427124129)) ;
#120469=CARTESIAN_POINT('Ctrl Pts',(-31.6425445471401,14.2375543492764,
126.720522362865)) ;
#120470=CARTESIAN_POINT('Ctrl Pts',(-31.5897144831715,14.0487159657188,
126.533039367418)) ;
#120471=CARTESIAN_POINT('Ctrl Pts',(-31.5554726021897,13.8167883871292,
126.400078496056)) ;
#120472=CARTESIAN_POINT('Ctrl Pts',(-31.542602309707,13.5548284865375,126.329281652584)) ;
#120473=CARTESIAN_POINT('Ctrl Pts',(-31.5530287952121,13.2844750332118,
126.326684756249)) ;
#120474=CARTESIAN_POINT('Ctrl Pts',(-31.5868796720123,13.0226683900031,
126.392329568486)) ;
#120475=CARTESIAN_POINT('Ctrl Pts',(-31.6419899311371,12.7913019843532,
126.520320997934)) ;
#120476=CARTESIAN_POINT('Ctrl Pts',(-31.7156175265643,12.6040507467942,
126.702258093667)) ;
#120477=CARTESIAN_POINT('Ctrl Pts',(-31.8031361180212,12.4756113935465,
126.924761331817)) ;
#120478=CARTESIAN_POINT('Ctrl Pts',(-31.8987627474538,12.415243488117,127.171001724304)) ;
#120479=CARTESIAN_POINT('Ctrl Pts',(-31.9964597074322,12.4269403743014,
127.423308917717)) ;
#120480=CARTESIAN_POINT('Ctrl Pts',(-32.0901558588354,12.5099953063745,
127.663881965089)) ;
#120481=CARTESIAN_POINT('Ctrl Pts',(-32.173774748925,12.6587329054093,127.874987741951)) ;
#120482=CARTESIAN_POINT('Ctrl Pts',(-32.2418392577068,12.8618952127667,
128.040723139875)) ;
#120483=CARTESIAN_POINT('Ctrl Pts',(-32.2904576103093,13.1054069861002,
128.149619377544)) ;
#120484=CARTESIAN_POINT('Ctrl Pts',(-32.316769944543,13.3721987049067,128.193296380107)) ;
#120485=CARTESIAN_POINT('Ctrl Pts',(-32.3195569713661,13.6415134162569,
128.168386125265)) ;
#120486=CARTESIAN_POINT('Ctrl Pts',(-32.299591267985,13.8954057310282,128.077001594138)) ;
#120487=CARTESIAN_POINT('Ctrl Pts',(-32.2585195327027,14.1169004710299,
127.923725730513)) ;
#120488=CARTESIAN_POINT('Ctrl Pts',(-32.2007685695086,14.2868623267828,
127.722030454418)) ;
#120489=CARTESIAN_POINT('Ctrl Pts',(-32.1305348488786,14.396013035847,127.48369692176)) ;
#120490=CARTESIAN_POINT('Ctrl Pts',(-32.0538050791662,14.4351149224746,
127.226396750023)) ;
#120491=CARTESIAN_POINT('Ctrl Pts',(-31.9770328389355,14.4019052027925,
126.969061606347)) ;
#120492=CARTESIAN_POINT('Ctrl Pts',(-31.9059255394677,14.2983009187854,
126.728137470122)) ;
#120493=CARTESIAN_POINT('Ctrl Pts',(-31.846755925753,14.1317969224175,126.522124007505)) ;
#120494=CARTESIAN_POINT('Ctrl Pts',(-31.8044925759672,13.91534337541,126.365618273777)) ;
#120495=CARTESIAN_POINT('Ctrl Pts',(-31.7826277420114,13.6633971728162,
126.268647311183)) ;
#120496=CARTESIAN_POINT('Ctrl Pts',(-31.7834890488768,13.3943409490525,
126.238079504293)) ;
#120497=CARTESIAN_POINT('Ctrl Pts',(-31.8080379768348,13.125759500651,126.276504548515)) ;
#120498=CARTESIAN_POINT('Ctrl Pts',(-31.8547791210711,12.8806964753524,
126.380044558236)) ;
#120499=CARTESIAN_POINT('Ctrl Pts',(-31.921382813645,12.6734733763792,126.541494713359)) ;
#120500=CARTESIAN_POINT('Ctrl Pts',(-32.0040660055355,12.5195858185458,
126.74981782748)) ;
#120501=CARTESIAN_POINT('Ctrl Pts',(-32.0971934592114,12.4310932740595,
126.988720519411)) ;
#120502=CARTESIAN_POINT('Ctrl Pts',(-32.1943755333981,12.4134132696985,
127.239663913926)) ;
#120503=CARTESIAN_POINT('Ctrl Pts',(-32.2907844041067,12.4681188633571,
127.48805990421)) ;
#120504=CARTESIAN_POINT('Ctrl Pts',(-32.3788634891402,12.5909169506631,
127.712321795157)) ;
#120505=CARTESIAN_POINT('Ctrl Pts',(-32.4538505271568,12.7734489072163,
127.898246415507)) ;
#120506=CARTESIAN_POINT('Ctrl Pts',(-32.5108712348923,13.0028154211787,
128.031660379154)) ;
#120507=CARTESIAN_POINT('Ctrl Pts',(-32.5464604471638,13.2626812904981,
128.10242752577)) ;
#120508=CARTESIAN_POINT('Ctrl Pts',(-32.5588102595845,13.5323091961428,
128.105524088133)) ;
#120509=CARTESIAN_POINT('Ctrl Pts',(-32.5478500365599,13.7963543423531,
128.040243010073)) ;
#120510=CARTESIAN_POINT('Ctrl Pts',(-32.5149810677505,14.0324258066149,
127.911102233703)) ;
#120511=CARTESIAN_POINT('Ctrl Pts',(-32.4636380719142,14.2243211732623,
127.728111071488)) ;
#120512=CARTESIAN_POINT('Ctrl Pts',(-32.3977993001216,14.3597396975641,
127.502651663795)) ;
#120513=CARTESIAN_POINT('Ctrl Pts',(-32.3227959762273,14.4280132150894,
127.250317340372)) ;
#120514=CARTESIAN_POINT('Ctrl Pts',(-32.2452616010669,14.4240026931505,
126.990711939345)) ;
#120515=CARTESIAN_POINT('Ctrl Pts',(-32.1711211897067,14.348214877112,126.740974584197)) ;
#120516=CARTESIAN_POINT('Ctrl Pts',(-32.1067221850188,14.2066839106137,
126.519814451723)) ;
#120517=CARTESIAN_POINT('Ctrl Pts',(-32.0569081619447,14.0084844644838,
126.341123531766)) ;
#120518=CARTESIAN_POINT('Ctrl Pts',(-32.0263232386117,13.76791632806,126.218578577679)) ;
#120519=CARTESIAN_POINT('Ctrl Pts',(-32.0179116552026,13.5034893328133,
126.160920310859)) ;
#120520=CARTESIAN_POINT('Ctrl Pts',(-32.0327954673164,13.2335994078643,
126.171345006653)) ;
#120521=CARTESIAN_POINT('Ctrl Pts',(-32.0707657946749,12.976407627843,126.249111915004)) ;
#120522=CARTESIAN_POINT('Ctrl Pts',(-32.1301041508424,12.7508792337382,
126.389211054592)) ;
#120523=CARTESIAN_POINT('Ctrl Pts',(-32.2062732152592,12.5752390532541,
126.578800301858)) ;
#120524=CARTESIAN_POINT('Ctrl Pts',(-32.2957312839852,12.4588914929926,
126.806976186385)) ;
#120525=CARTESIAN_POINT('Ctrl Pts',(-32.392308620738,12.4118138328558,127.055972899133)) ;
#120526=CARTESIAN_POINT('Ctrl Pts',(-32.4900557202676,12.4374481799832,
127.308301819784)) ;
#120527=CARTESIAN_POINT('Ctrl Pts',(-32.5820384027822,12.5333386552095,
127.543956363044)) ;
#120528=CARTESIAN_POINT('Ctrl Pts',(-32.6633130647022,12.6939674039094,
127.748117070613)) ;
#120529=CARTESIAN_POINT('Ctrl Pts',(-32.7276564437716,12.9050031482846,
127.903137803992)) ;
#120530=CARTESIAN_POINT('Ctrl Pts',(-32.7724018637935,13.1551455919413,
128.000592328387)) ;
#120531=CARTESIAN_POINT('Ctrl Pts',(-32.7869026808253,13.3338157805737,
128.020913097943)) ;
#120532=CARTESIAN_POINT('Ctrl Pts',(-32.7902884693506,13.4231220893089,
128.019783106832)) ;
#120533=CARTESIAN_POINT('Ctrl Pts',(-11.4473705198918,13.1734341962953,
133.2453836742)) ;
#120534=CARTESIAN_POINT('Ctrl Pts',(-11.4480740668009,13.1676985268958,
133.24670795141)) ;
#120535=CARTESIAN_POINT('Ctrl Pts',(-11.4595477305337,13.076204201721,133.268542953682)) ;
#120536=CARTESIAN_POINT('Ctrl Pts',(-11.4905248885226,12.9034784200084,
133.336060088381)) ;
#120537=CARTESIAN_POINT('Ctrl Pts',(-11.5552006767944,12.6923997924798,
133.491971818923)) ;
#120538=CARTESIAN_POINT('Ctrl Pts',(-11.6361658480941,12.5327609197045,
133.695385432581)) ;
#120539=CARTESIAN_POINT('Ctrl Pts',(-11.7288235566871,12.4368205686394,
133.932788388924)) ;
#120540=CARTESIAN_POINT('Ctrl Pts',(-11.8257634374896,12.4119420237697,
134.183044910058)) ;
#120541=CARTESIAN_POINT('Ctrl Pts',(-11.9225895618528,12.4592681498074,
134.432672297289)) ;
#120542=CARTESIAN_POINT('Ctrl Pts',(-12.0118665215859,12.575659036236,134.660380692383)) ;
#120543=CARTESIAN_POINT('Ctrl Pts',(-12.0884448545199,12.75283542717,134.850941590915)) ;
#120544=CARTESIAN_POINT('Ctrl Pts',(-12.1473740885929,12.9779971811105,
134.989965265017)) ;
#120545=CARTESIAN_POINT('Ctrl Pts',(-12.1851940642893,13.2349354675193,
135.067332760891)) ;
#120546=CARTESIAN_POINT('Ctrl Pts',(-12.2000107655077,13.5051819451432,
135.077525536086)) ;
#120547=CARTESIAN_POINT('Ctrl Pts',(-12.1912876596684,13.7710457079463,
135.018753485588)) ;
#120548=CARTESIAN_POINT('Ctrl Pts',(-12.1606973063918,14.0095406593372,
134.896429733358)) ;
#120549=CARTESIAN_POINT('Ctrl Pts',(-12.11092513824,14.2073761046424,134.717903581334)) ;
#120550=CARTESIAN_POINT('Ctrl Pts',(-12.0463035752806,14.3489569855306,
134.496013109962)) ;
#120551=CARTESIAN_POINT('Ctrl Pts',(-11.9719809240434,14.4243647659385,
134.24568576646)) ;
#120552=CARTESIAN_POINT('Ctrl Pts',(-11.8944197744956,14.427672591071,133.985990463909)) ;
#120553=CARTESIAN_POINT('Ctrl Pts',(-11.819820484482,14.3592845353793,133.734997132989)) ;
#120554=CARTESIAN_POINT('Ctrl Pts',(-11.7540479069007,14.2239082001409,
133.50975548736)) ;
#120555=CARTESIAN_POINT('Ctrl Pts',(-11.7025290912445,14.0309430574059,
133.326104874534)) ;
#120556=CARTESIAN_POINT('Ctrl Pts',(-11.6698185107926,13.7937231411456,
133.197324613256)) ;
#120557=CARTESIAN_POINT('Ctrl Pts',(-11.6590728229283,13.5318368827659,
133.132954885592)) ;
#120558=CARTESIAN_POINT('Ctrl Pts',(-11.6715146568046,13.260908758679,133.136158645477)) ;
#120559=CARTESIAN_POINT('Ctrl Pts',(-11.7073390044507,13.0011530565724,
133.20760253653)) ;
#120560=CARTESIAN_POINT('Ctrl Pts',(-11.7641809555439,12.7729626729889,
133.340640813236)) ;
#120561=CARTESIAN_POINT('Ctrl Pts',(-11.8393511387376,12.5901801237826,
133.527033924571)) ;
#120562=CARTESIAN_POINT('Ctrl Pts',(-11.9275728085287,12.4676467713314,
133.751683720386)) ;
#120563=CARTESIAN_POINT('Ctrl Pts',(-12.0239720292633,12.413314501038,134.000062258223)) ;
#120564=CARTESIAN_POINT('Ctrl Pts',(-12.121304733462,12.4313809059018,134.251393442111)) ;
#120565=CARTESIAN_POINT('Ctrl Pts',(-12.2145517431487,12.5206603484656,
134.490579145694)) ;
#120566=CARTESIAN_POINT('Ctrl Pts',(-12.2968075547073,12.6744196148216,
134.697779915769)) ;
#120567=CARTESIAN_POINT('Ctrl Pts',(-12.3633737809412,12.8815893341258,
134.85913785182)) ;
#120568=CARTESIAN_POINT('Ctrl Pts',(-12.4102625920414,13.1290193456038,
134.962833588597)) ;
#120569=CARTESIAN_POINT('Ctrl Pts',(-12.4343449087572,13.3950772518204,
135.000224573441)) ;
#120570=CARTESIAN_POINT('Ctrl Pts',(-12.4352286842141,13.6643422142601,
134.969691915908)) ;
#120571=CARTESIAN_POINT('Ctrl Pts',(-12.4131525718201,13.9170737538833,
134.871985659673)) ;
#120572=CARTESIAN_POINT('Ctrl Pts',(-12.3706607762256,14.1334228161875,
134.714767891984)) ;
#120573=CARTESIAN_POINT('Ctrl Pts',(-12.3115699368204,14.2989215629879,
134.509090314935)) ;
#120574=CARTESIAN_POINT('Ctrl Pts',(-12.2406260808501,14.4021434472197,
134.268728348906)) ;
#120575=CARTESIAN_POINT('Ctrl Pts',(-12.1635096540278,14.4351203025954,
134.010245514987)) ;
#120576=CARTESIAN_POINT('Ctrl Pts',(-12.0870609123607,14.3956460282901,
133.753876776433)) ;
#120577=CARTESIAN_POINT('Ctrl Pts',(-12.0168112766492,14.2864256300776,
133.515489344327)) ;
#120578=CARTESIAN_POINT('Ctrl Pts',(-11.9588806020232,14.1149875929984,
133.313083595978)) ;
#120579=CARTESIAN_POINT('Ctrl Pts',(-11.9182630667946,13.8950778464839,
133.16141233224)) ;
#120580=CARTESIAN_POINT('Ctrl Pts',(-11.8982136803435,13.6402948775312,
133.069662409729)) ;
#120581=CARTESIAN_POINT('Ctrl Pts',(-11.9012091414679,13.3700134780419,
133.045253453647)) ;
#120582=CARTESIAN_POINT('Ctrl Pts',(-11.9276282936563,13.1040820089462,
133.089332965067)) ;
#120583=CARTESIAN_POINT('Ctrl Pts',(-11.9762490634299,12.8608603098162,
133.198268746333)) ;
#120584=CARTESIAN_POINT('Ctrl Pts',(-12.0448000874776,12.6570994974887,
133.365259571756)) ;
#120585=CARTESIAN_POINT('Ctrl Pts',(-12.1280040260076,12.509712563052,133.575356875517)) ;
#120586=CARTESIAN_POINT('Ctrl Pts',(-12.2217907278284,12.4266925565407,
133.816162814867)) ;
#120587=CARTESIAN_POINT('Ctrl Pts',(-12.3195845113326,12.4153566228605,
134.06872463408)) ;
#120588=CARTESIAN_POINT('Ctrl Pts',(-12.4151906282434,12.476118398497,134.31490137872)) ;
#120589=CARTESIAN_POINT('Ctrl Pts',(-12.5025015711756,12.6046110942521,
134.536856258684)) ;
#120590=CARTESIAN_POINT('Ctrl Pts',(-12.5761392571973,12.7920330529179,
134.718809905303)) ;
#120591=CARTESIAN_POINT('Ctrl Pts',(-12.6313190561571,13.024646117744,134.846865821606)) ;
#120592=CARTESIAN_POINT('Ctrl Pts',(-12.6648510010149,13.2849677628749,
134.911782387054)) ;
#120593=CARTESIAN_POINT('Ctrl Pts',(-12.6752768859988,13.5561840574451,
134.909074632877)) ;
#120594=CARTESIAN_POINT('Ctrl Pts',(-12.6622542366794,13.8182131440166,
134.83781287569)) ;
#120595=CARTESIAN_POINT('Ctrl Pts',(-12.6278120959063,14.0504675663447,
134.704189256873)) ;
#120596=CARTESIAN_POINT('Ctrl Pts',(-12.5746767390659,14.2392689175362,
134.515730540059)) ;
#120597=CARTESIAN_POINT('Ctrl Pts',(-12.5077212333364,14.3686949412613,
134.286997684432)) ;
#120598=CARTESIAN_POINT('Ctrl Pts',(-12.4328327987394,14.4303698787607,
134.035262433741)) ;
#120599=CARTESIAN_POINT('Ctrl Pts',(-12.3551681454901,14.4203874176643,
133.775196684826)) ;
#120600=CARTESIAN_POINT('Ctrl Pts',(-12.281427216418,14.3383233721809,133.526543913651)) ;
#120601=CARTESIAN_POINT('Ctrl Pts',(-12.2180346569397,14.1909246457993,
133.308253001474)) ;
#120602=CARTESIAN_POINT('Ctrl Pts',(-12.1700271254954,13.9894771384923,
133.135018970481)) ;
#120603=CARTESIAN_POINT('Ctrl Pts',(-12.1412312608287,13.7468082771736,
133.017778045599)) ;
#120604=CARTESIAN_POINT('Ctrl Pts',(-12.1346803482234,13.4802542547444,
132.965444637786)) ;
#120605=CARTESIAN_POINT('Ctrl Pts',(-12.1518060283826,13.2092850470841,
132.982231344216)) ;
#120606=CARTESIAN_POINT('Ctrl Pts',(-12.1914284395064,12.9563426353649,
133.065098166761)) ;
#120607=CARTESIAN_POINT('Ctrl Pts',(-12.2522891121189,12.7340442685521,
133.209644808083)) ;
#120608=CARTESIAN_POINT('Ctrl Pts',(-12.3304078125076,12.5620254310283,
133.404672739898)) ;
#120609=CARTESIAN_POINT('Ctrl Pts',(-12.4202116415783,12.4521634508898,
133.634056112492)) ;
#120610=CARTESIAN_POINT('Ctrl Pts',(-12.517532818831,12.4110698291516,133.885078444257)) ;
#120611=CARTESIAN_POINT('Ctrl Pts',(-12.6148078934914,12.4431134789288,
134.136118265331)) ;
#120612=CARTESIAN_POINT('Ctrl Pts',(-12.7059248212752,12.544720780955,134.36927974363)) ;
#120613=CARTESIAN_POINT('Ctrl Pts',(-12.7857599917973,12.709460812036,134.569364737784)) ;
#120614=CARTESIAN_POINT('Ctrl Pts',(-12.8490190731694,12.9261933468861,
134.720931773752)) ;
#120615=CARTESIAN_POINT('Ctrl Pts',(-12.8915191285647,13.1767718332297,
134.812096240414)) ;
#120616=CARTESIAN_POINT('Ctrl Pts',(-12.9115116010101,13.4474343197197,
134.837194593127)) ;
#120617=CARTESIAN_POINT('Ctrl Pts',(-12.9077976399136,13.7143157713228,
134.793294199843)) ;
#120618=CARTESIAN_POINT('Ctrl Pts',(-12.8818813884825,13.960120914319,134.684592833268)) ;
#120619=CARTESIAN_POINT('Ctrl Pts',(-12.8357313693075,14.1691500544874,
134.516518989096)) ;
#120620=CARTESIAN_POINT('Ctrl Pts',(-12.7740689064731,14.3234013156229,
134.303370793792)) ;
#120621=CARTESIAN_POINT('Ctrl Pts',(-12.7014220850373,14.4138714588237,
134.057977547517)) ;
#120622=CARTESIAN_POINT('Ctrl Pts',(-12.6241886832898,14.4332950652812,
133.799291383501)) ;
#120623=CARTESIAN_POINT('Ctrl Pts',(-12.5478867089577,14.37983766652,133.543078701379)) ;
#120624=CARTESIAN_POINT('Ctrl Pts',(-12.4799675217152,14.2584887072528,
133.311683366343)) ;
#120625=CARTESIAN_POINT('Ctrl Pts',(-12.4249393482279,14.0772214064872,
133.117809426492)) ;
#120626=CARTESIAN_POINT('Ctrl Pts',(-12.3877664398662,13.8478579716949,
132.975955272484)) ;
#120627=CARTESIAN_POINT('Ctrl Pts',(-12.3721402537263,13.5896598560144,
132.897269249345)) ;
#120628=CARTESIAN_POINT('Ctrl Pts',(-12.3794806782538,13.3195388423839,
132.885663034153)) ;
#120629=CARTESIAN_POINT('Ctrl Pts',(-12.4103064738394,13.0556169732422,
132.942510353194)) ;
#120630=CARTESIAN_POINT('Ctrl Pts',(-12.4629013673467,12.8189342678657,
133.063069191677)) ;
#120631=CARTESIAN_POINT('Ctrl Pts',(-12.5344122785446,12.625100278912,133.238826624894)) ;
#120632=CARTESIAN_POINT('Ctrl Pts',(-12.6202525140682,12.4887479023081,
133.456496574608)) ;
#120633=CARTESIAN_POINT('Ctrl Pts',(-12.7150155758981,12.4190670277806,
133.700254320957)) ;
#120634=CARTESIAN_POINT('Ctrl Pts',(-12.8132064476839,12.4213699947317,
133.95386332912)) ;
#120635=CARTESIAN_POINT('Ctrl Pts',(-12.9075620983682,12.4953802874648,
134.196438541246)) ;
#120636=CARTESIAN_POINT('Ctrl Pts',(-12.9927902768386,12.6359572758876,
134.412260415263)) ;
#120637=CARTESIAN_POINT('Ctrl Pts',(-13.0631709953693,12.8329198121217,
134.584736258615)) ;
#120638=CARTESIAN_POINT('Ctrl Pts',(-13.1144613389104,13.0719650653609,
134.701464258526)) ;
#120639=CARTESIAN_POINT('Ctrl Pts',(-13.143774727237,13.3363498058402,134.753966235205)) ;
#120640=CARTESIAN_POINT('Ctrl Pts',(-13.1496791294893,13.6070577541681,
134.738072707591)) ;
#120641=CARTESIAN_POINT('Ctrl Pts',(-13.1324713549101,13.8644612546569,
134.654675083653)) ;
#120642=CARTESIAN_POINT('Ctrl Pts',(-13.0941894467002,14.0900773467752,
134.509746512484)) ;
#120643=CARTESIAN_POINT('Ctrl Pts',(-13.0381529177921,14.2682172866369,
134.3128932133)) ;
#120644=CARTESIAN_POINT('Ctrl Pts',(-12.9694164279505,14.38541662164,134.079049330582)) ;
#120645=CARTESIAN_POINT('Ctrl Pts',(-12.8932702282235,14.4341663230829,
133.823482020016)) ;
#120646=CARTESIAN_POINT('Ctrl Pts',(-12.8158362554554,14.4102121199937,
133.564068937527)) ;
#120647=CARTESIAN_POINT('Ctrl Pts',(-12.7438549252204,14.3156228992233,
133.320698817844)) ;
#120648=CARTESIAN_POINT('Ctrl Pts',(-12.6828642788531,14.1571117178342,
133.109403768484)) ;
#120649=CARTESIAN_POINT('Ctrl Pts',(-12.6380503902695,13.9459763961177,
132.945365338171)) ;
#120650=CARTESIAN_POINT('Ctrl Pts',(-12.6133436908675,13.697562228916,132.840086078986)) ;
#120651=CARTESIAN_POINT('Ctrl Pts',(-12.6112238063931,13.4293975021098,
132.800773961391)) ;
#120652=CARTESIAN_POINT('Ctrl Pts',(-12.6325249834962,13.1610019423395,
132.829911431496)) ;
#120653=CARTESIAN_POINT('Ctrl Pts',(-12.6766496599303,12.9105848484096,
132.925613172297)) ;
#120654=CARTESIAN_POINT('Ctrl Pts',(-12.7409122350092,12.6976134704073,
133.080239826003)) ;
#120655=CARTESIAN_POINT('Ctrl Pts',(-12.8215669260211,12.536442279252,133.282728587217)) ;
#120656=CARTESIAN_POINT('Ctrl Pts',(-12.9134891990553,12.4387732237497,
133.518152797446)) ;
#120657=CARTESIAN_POINT('Ctrl Pts',(-13.0111243090133,12.4116342437955,
133.770178301096)) ;
#120658=CARTESIAN_POINT('Ctrl Pts',(-13.1075737106094,12.4569142489461,
134.018874417128)) ;
#120659=CARTESIAN_POINT('Ctrl Pts',(-13.1972943937453,12.5714752096904,
134.247823335506)) ;
#120660=CARTESIAN_POINT('Ctrl Pts',(-13.2741873813664,12.7468633486005,
134.439353851752)) ;
#120661=CARTESIAN_POINT('Ctrl Pts',(-13.3336915143071,12.9706873354731,
134.580068833733)) ;
#120662=CARTESIAN_POINT('Ctrl Pts',(-13.3721999484215,13.2271705997234,
134.659418787554)) ;
#120663=CARTESIAN_POINT('Ctrl Pts',(-13.3876917555698,13.4971330615505,
134.671604283926)) ;
#120664=CARTESIAN_POINT('Ctrl Pts',(-13.3796635334537,13.7633006467314,
134.614879288565)) ;
#120665=CARTESIAN_POINT('Ctrl Pts',(-13.3497382425018,14.0028269061398,
134.494506191552)) ;
#120666=CARTESIAN_POINT('Ctrl Pts',(-13.3002259749356,14.2028678275338,
134.316595478873)) ;
#120667=CARTESIAN_POINT('Ctrl Pts',(-13.2361890414634,14.3455611921622,
134.09654406856)) ;
#120668=CARTESIAN_POINT('Ctrl Pts',(-13.16207558202,14.4231516599767,133.846823988595)) ;
#120669=CARTESIAN_POINT('Ctrl Pts',(-13.0845063845158,14.4286657254974,
133.587101274246)) ;
#120670=CARTESIAN_POINT('Ctrl Pts',(-13.0095842588762,14.3621069450972,
133.335090766211)) ;
#120671=CARTESIAN_POINT('Ctrl Pts',(-12.9435378379878,14.2287342743254,
133.109091925138)) ;
#120672=CARTESIAN_POINT('Ctrl Pts',(-12.8914199215781,14.0363060460215,
132.923560068454)) ;
#120673=CARTESIAN_POINT('Ctrl Pts',(-12.8583816910615,13.8023696285656,
132.794134663991)) ;
#120674=CARTESIAN_POINT('Ctrl Pts',(-12.8467978400967,13.5388531548576,
132.727034564485)) ;
#120675=CARTESIAN_POINT('Ctrl Pts',(-12.8586819410096,13.268451758325,132.728680134931)) ;
#120676=CARTESIAN_POINT('Ctrl Pts',(-12.8936410367749,13.0087996264663,
132.797700642119)) ;
#120677=CARTESIAN_POINT('Ctrl Pts',(-12.9504077026141,12.7778890108915,
132.930263212947)) ;
#120678=CARTESIAN_POINT('Ctrl Pts',(-13.0245928914567,12.5950173458057,
133.114032484941)) ;
#120679=CARTESIAN_POINT('Ctrl Pts',(-13.1129297604522,12.4700324855763,
133.338848639727)) ;
#120680=CARTESIAN_POINT('Ctrl Pts',(-13.2086496709529,12.4138573674352,
133.58543860934)) ;
#120681=CARTESIAN_POINT('Ctrl Pts',(-13.3068912134905,12.4301864396543,
133.83911949565)) ;
#120682=CARTESIAN_POINT('Ctrl Pts',(-13.3993566508513,12.5166844416216,
134.076381880359)) ;
#120683=CARTESIAN_POINT('Ctrl Pts',(-13.4825199697664,12.6693065290769,
134.286038282632)) ;
#120684=CARTESIAN_POINT('Ctrl Pts',(-13.5493581300511,12.8745471633582,
134.448302940679)) ;
#120685=CARTESIAN_POINT('Ctrl Pts',(-13.5969792928083,13.1212024009445,
134.554104584044)) ;
#120686=CARTESIAN_POINT('Ctrl Pts',(-13.6217614180752,13.3871939344405,
134.593509017336)) ;
#120687=CARTESIAN_POINT('Ctrl Pts',(-13.6233033483175,13.6567281897723,
134.564888588754)) ;
#120688=CARTESIAN_POINT('Ctrl Pts',(-13.6019424260938,13.90978543386,134.469337913371)) ;
#120689=CARTESIAN_POINT('Ctrl Pts',(-13.559878508592,14.1280196387556,134.313271082727)) ;
#120690=CARTESIAN_POINT('Ctrl Pts',(-13.5012677872863,14.2950455998267,
134.109034226085)) ;
#120691=CARTESIAN_POINT('Ctrl Pts',(-13.4301333980882,14.4005267621949,
133.867917157598)) ;
#120692=CARTESIAN_POINT('Ctrl Pts',(-13.3536177744754,14.4350836723043,
133.611420653287)) ;
#120693=CARTESIAN_POINT('Ctrl Pts',(-13.2769729997003,14.3978038978104,
133.354433604439)) ;
#120694=CARTESIAN_POINT('Ctrl Pts',(-13.2065378850675,14.2905756791986,
133.115544315935)) ;
#120695=CARTESIAN_POINT('Ctrl Pts',(-13.1481709847974,14.1209511396773,
132.911875009647)) ;
#120696=CARTESIAN_POINT('Ctrl Pts',(-13.106914032843,13.9018371700798,132.758271963134)) ;
#120697=CARTESIAN_POINT('Ctrl Pts',(-13.0862872253786,13.6479071174512,
132.664855347399)) ;
#120698=CARTESIAN_POINT('Ctrl Pts',(-13.0885177354421,13.3785017706424,
132.638297597662)) ;
#120699=CARTESIAN_POINT('Ctrl Pts',(-13.1144622409219,13.1105160825095,
132.680778935072)) ;
#120700=CARTESIAN_POINT('Ctrl Pts',(-13.1623141537455,12.867723627882,132.787635761551)) ;
#120701=CARTESIAN_POINT('Ctrl Pts',(-13.230117220087,12.6628307247657,132.952513766649)) ;
#120702=CARTESIAN_POINT('Ctrl Pts',(-13.313146584717,12.5130918366744,133.162010291795)) ;
#120703=CARTESIAN_POINT('Ctrl Pts',(-13.4069813662761,12.4280188888238,
133.402870847898)) ;
#120704=CARTESIAN_POINT('Ctrl Pts',(-13.5044591370903,12.4146728717073,
133.654606478724)) ;
#120705=CARTESIAN_POINT('Ctrl Pts',(-13.6004343999475,12.4734183176243,
133.901788773024)) ;
#120706=CARTESIAN_POINT('Ctrl Pts',(-13.6881527513873,12.6005221105397,
134.124883438968)) ;
#120707=CARTESIAN_POINT('Ctrl Pts',(-13.7618732063886,12.7855012395254,
134.307246567862)) ;
#120708=CARTESIAN_POINT('Ctrl Pts',(-13.8177438998128,13.0169861501724,
134.437303681495)) ;
#120709=CARTESIAN_POINT('Ctrl Pts',(-13.8520207068986,13.2774554458054,
134.50430837638)) ;
#120710=CARTESIAN_POINT('Ctrl Pts',(-13.8630629061763,13.548371247685,134.503433492184)) ;
#120711=CARTESIAN_POINT('Ctrl Pts',(-13.8508213988482,13.8100860909014,
134.434572278497)) ;
#120712=CARTESIAN_POINT('Ctrl Pts',(-13.8168650274927,14.0443620867839,
134.302237807465)) ;
#120713=CARTESIAN_POINT('Ctrl Pts',(-13.7644044931097,14.2339607222734,
134.115876257614)) ;
#120714=CARTESIAN_POINT('Ctrl Pts',(-13.6978380060744,14.3656339915205,
133.888274922942)) ;
#120715=CARTESIAN_POINT('Ctrl Pts',(-13.622733233145,14.4296685525136,133.635745138518)) ;
#120716=CARTESIAN_POINT('Ctrl Pts',(-13.5452624861586,14.4216217611559,
133.37633613)) ;
#120717=CARTESIAN_POINT('Ctrl Pts',(-13.4715715969191,14.3422173843901,
133.127956640297)) ;
#120718=CARTESIAN_POINT('Ctrl Pts',(-13.4075312607501,14.1963612396834,
132.907659105306)) ;
#120719=CARTESIAN_POINT('Ctrl Pts',(-13.3589146402362,13.9958155660663,
132.73257138974)) ;
#120720=CARTESIAN_POINT('Ctrl Pts',(-13.329551475218,13.754087100232,132.613679382634)) ;
#120721=CARTESIAN_POINT('Ctrl Pts',(-13.3223349657066,13.4887317484018,
132.559497435662)) ;
#120722=CARTESIAN_POINT('Ctrl Pts',(-13.3386798564622,13.2176489571942,
132.574010621013)) ;
#120723=CARTESIAN_POINT('Ctrl Pts',(-13.3777977002964,12.9629383916558,
132.655272653247)) ;
#120724=CARTESIAN_POINT('Ctrl Pts',(-13.4382415285139,12.7394456176792,
132.798570796011)) ;
#120725=CARTESIAN_POINT('Ctrl Pts',(-13.5154589025096,12.5666312437579,
132.991152487379)) ;
#120726=CARTESIAN_POINT('Ctrl Pts',(-13.605481193571,12.4542159326756,133.220985631602)) ;
#120727=CARTESIAN_POINT('Ctrl Pts',(-13.7021416815521,12.4113528378657,
133.470272085389)) ;
#120728=CARTESIAN_POINT('Ctrl Pts',(-13.7997225612357,12.4409689783365,
133.722129964994)) ;
#120729=CARTESIAN_POINT('Ctrl Pts',(-13.8914867339935,12.5412370853856,
133.957037400847)) ;
#120730=CARTESIAN_POINT('Ctrl Pts',(-13.971457705638,12.7041353032971,134.157601912298)) ;
#120731=CARTESIAN_POINT('Ctrl Pts',(-14.0350614876758,12.9183855317437,
134.31033126713)) ;
#120732=CARTESIAN_POINT('Ctrl Pts',(-14.0784578071401,13.1698655551169,
134.403888857352)) ;
#120733=CARTESIAN_POINT('Ctrl Pts',(-14.0989865001082,13.4380609721582,
134.430831936226)) ;
#120734=CARTESIAN_POINT('Ctrl Pts',(-14.0960490957043,13.707166634389,134.388968900715)) ;
#120735=CARTESIAN_POINT('Ctrl Pts',(-14.0706178920924,13.9538088162951,
134.281667787138)) ;
#120736=CARTESIAN_POINT('Ctrl Pts',(-14.0252188571593,14.1634527174507,
134.115921093202)) ;
#120737=CARTESIAN_POINT('Ctrl Pts',(-13.963634925678,14.3201289995184,133.902836103935)) ;
#120738=CARTESIAN_POINT('Ctrl Pts',(-13.8915338635795,14.4121341024828,
133.659191560836)) ;
#120739=CARTESIAN_POINT('Ctrl Pts',(-13.8140762063645,14.4336855920868,
133.399723796815)) ;
#120740=CARTESIAN_POINT('Ctrl Pts',(-13.7381279524733,14.3827385765516,
133.144763866546)) ;
#120741=CARTESIAN_POINT('Ctrl Pts',(-13.66939667137,14.2627494122855,132.910772598038)) ;
#120742=CARTESIAN_POINT('Ctrl Pts',(-13.6139327257614,14.0822576460886,
132.71556082231)) ;
#120743=CARTESIAN_POINT('Ctrl Pts',(-13.5764902068372,13.8561930768697,
132.573222227403)) ;
#120744=CARTESIAN_POINT('Ctrl Pts',(-13.5600295200209,13.5974241277666,
132.491927422412)) ;
#120745=CARTESIAN_POINT('Ctrl Pts',(-13.5667144048106,13.3273250801774,
132.478407313272)) ;
#120746=CARTESIAN_POINT('Ctrl Pts',(-13.5969980563113,13.0622910344741,
132.533583951509)) ;
#120747=CARTESIAN_POINT('Ctrl Pts',(-13.6488100028414,12.8256129311331,
132.651993012919)) ;
#120748=CARTESIAN_POINT('Ctrl Pts',(-13.7197957147865,12.6301797722552,
132.826210227303)) ;
#120749=CARTESIAN_POINT('Ctrl Pts',(-13.8052923968474,12.491847584192,133.042869793119)) ;
#120750=CARTESIAN_POINT('Ctrl Pts',(-13.9002855742496,12.4199209625087,
133.287159868651)) ;
#120751=CARTESIAN_POINT('Ctrl Pts',(-13.9983308301703,12.4204246206127,
133.540393962923)) ;
#120752=CARTESIAN_POINT('Ctrl Pts',(-14.0926150230179,12.4921596766918,
133.782850441087)) ;
#120753=CARTESIAN_POINT('Ctrl Pts',(-14.1782827856701,12.6310174141653,
133.999923925961)) ;
#120754=CARTESIAN_POINT('Ctrl Pts',(-14.2490962026249,12.8262648550687,
134.173703003042)) ;
#120755=CARTESIAN_POINT('Ctrl Pts',(-14.3010623629354,13.0646915634,134.292350167285)) ;
#120756=CARTESIAN_POINT('Ctrl Pts',(-14.3310020809812,13.3278245942677,
134.346780502656)) ;
#120757=CARTESIAN_POINT('Ctrl Pts',(-14.3376192816008,13.599858684379,134.33281390352)) ;
#120758=CARTESIAN_POINT('Ctrl Pts',(-14.3210988184506,13.8569828233467,
134.25154641035)) ;
#120759=CARTESIAN_POINT('Ctrl Pts',(-14.2833243438028,14.0842219920521,
134.108028651301)) ;
#120760=CARTESIAN_POINT('Ctrl Pts',(-14.2279563626728,14.263433654148,133.913245859207)) ;
#120761=CARTESIAN_POINT('Ctrl Pts',(-14.1590892226973,14.3833954982456,
133.67880615733)) ;
#120762=CARTESIAN_POINT('Ctrl Pts',(-14.08298330848,14.4336980468668,133.423334734623)) ;
#120763=CARTESIAN_POINT('Ctrl Pts',(-14.0060043305073,14.4120157634547,
133.165469744423)) ;
#120764=CARTESIAN_POINT('Ctrl Pts',(-13.9335630677938,14.3192946556154,
132.920658510169)) ;
#120765=CARTESIAN_POINT('Ctrl Pts',(-13.8722225085746,14.1625582896785,
132.708365939663)) ;
#120766=CARTESIAN_POINT('Ctrl Pts',(-13.8267634979844,13.9521768642311,
132.542354975134)) ;
#120767=CARTESIAN_POINT('Ctrl Pts',(-13.8015371760947,13.7045477344639,
132.43556559473)) ;
#120768=CARTESIAN_POINT('Ctrl Pts',(-13.7987127257712,13.4377490318283,
132.394327067906)) ;
#120769=CARTESIAN_POINT('Ctrl Pts',(-13.819460311345,13.1678476288368,132.421687970309)) ;
#120770=CARTESIAN_POINT('Ctrl Pts',(-13.8627949203012,12.9176590168047,
132.515222019688)) ;
#120771=CARTESIAN_POINT('Ctrl Pts',(-13.9268006590622,12.7025601714455,
132.668956240077)) ;
#120772=CARTESIAN_POINT('Ctrl Pts',(-14.0066558896622,12.5405894740577,
132.869281960535)) ;
#120773=CARTESIAN_POINT('Ctrl Pts',(-14.0985650251881,12.4405287581968,
133.104571602708)) ;
#120774=CARTESIAN_POINT('Ctrl Pts',(-14.1961041611978,12.4114132280254,
133.356330665668)) ;
#120775=CARTESIAN_POINT('Ctrl Pts',(-14.2926156330225,12.4546443860593,
133.605220308635)) ;
#120776=CARTESIAN_POINT('Ctrl Pts',(-14.3824600952418,12.5668919860046,
133.834602175721)) ;
#120777=CARTESIAN_POINT('Ctrl Pts',(-14.4601722625008,12.7415276460806,
134.028362617741)) ;
#120778=CARTESIAN_POINT('Ctrl Pts',(-14.520049146209,12.9638993361252,134.170229973779)) ;
#120779=CARTESIAN_POINT('Ctrl Pts',(-14.5591593181283,13.2191083147461,
134.251407675557)) ;
#120780=CARTESIAN_POINT('Ctrl Pts',(-14.575350824638,13.4893535433623,134.265583197429)) ;
#120781=CARTESIAN_POINT('Ctrl Pts',(-14.5680599633527,13.7553189464662,
134.211098945095)) ;
#120782=CARTESIAN_POINT('Ctrl Pts',(-14.5385649126019,13.9971252301126,
134.091796305584)) ;
#120783=CARTESIAN_POINT('Ctrl Pts',(-14.4896511547738,14.197781210739,133.915741437835)) ;
#120784=CARTESIAN_POINT('Ctrl Pts',(-14.4259733060109,14.3424511179814,
133.696723001246)) ;
#120785=CARTESIAN_POINT('Ctrl Pts',(-14.351768758291,14.4220643031845,133.446619873331)) ;
#120786=CARTESIAN_POINT('Ctrl Pts',(-14.274603622944,14.4294490868584,133.18824319121)) ;
#120787=CARTESIAN_POINT('Ctrl Pts',(-14.1995531258177,14.3652071957823,
132.935880016242)) ;
#120788=CARTESIAN_POINT('Ctrl Pts',(-14.1330952945771,14.2335291048216,
132.708640760205)) ;
#120789=CARTESIAN_POINT('Ctrl Pts',(-14.0805195452,14.0429178976906,132.52181225508)) ;
#120790=CARTESIAN_POINT('Ctrl Pts',(-14.0468273962399,13.8093219413454,
132.390378710343)) ;
#120791=CARTESIAN_POINT('Ctrl Pts',(-14.0345756389885,13.547621689864,132.321489870949)) ;
#120792=CARTESIAN_POINT('Ctrl Pts',(-14.045869711759,13.275071076932,132.321149166054)) ;
#120793=CARTESIAN_POINT('Ctrl Pts',(-14.0801004011068,13.0163163266613,
132.388221144306)) ;
#120794=CARTESIAN_POINT('Ctrl Pts',(-14.1360514026648,12.7846450787164,
132.518475111333)) ;
#120795=CARTESIAN_POINT('Ctrl Pts',(-14.209997805868,12.5995255835865,132.7014357454)) ;
#120796=CARTESIAN_POINT('Ctrl Pts',(-14.2980487746721,12.4726551218916,
132.925409988479)) ;
#120797=CARTESIAN_POINT('Ctrl Pts',(-14.3936992232197,12.4145513359232,
133.171770800119)) ;
#120798=CARTESIAN_POINT('Ctrl Pts',(-14.4914656501182,12.4284690749365,
133.424241778918)) ;
#120799=CARTESIAN_POINT('Ctrl Pts',(-14.5847554755448,12.513343198717,133.663701292664)) ;
#120800=CARTESIAN_POINT('Ctrl Pts',(-14.6682321414824,12.6644367568353,
133.874283018656)) ;
#120801=CARTESIAN_POINT('Ctrl Pts',(-14.7354435033099,12.8679925993142,
134.037693222063)) ;
#120802=CARTESIAN_POINT('Ctrl Pts',(-14.7836382994798,13.1131690756933,
134.145239554443)) ;
#120803=CARTESIAN_POINT('Ctrl Pts',(-14.8092152926094,13.380000312228,134.186817151239)) ;
#120804=CARTESIAN_POINT('Ctrl Pts',(-14.8113213541148,13.6495651936862,
134.159860975393)) ;
#120805=CARTESIAN_POINT('Ctrl Pts',(-14.7907198845191,13.9023389091985,
134.066668081572)) ;
#120806=CARTESIAN_POINT('Ctrl Pts',(-14.7490861418248,14.1226577845122,
133.911740549666)) ;
#120807=CARTESIAN_POINT('Ctrl Pts',(-14.6909606696642,14.2908247564139,
133.708982259999)) ;
#120808=CARTESIAN_POINT('Ctrl Pts',(-14.6204821622466,14.398104059989,133.469939230604)) ;
#120809=CARTESIAN_POINT('Ctrl Pts',(-14.5435082791429,14.4352626924574,
133.211865337823)) ;
#120810=CARTESIAN_POINT('Ctrl Pts',(-14.4666927956805,14.3995540254238,
132.95433679224)) ;
#120811=CARTESIAN_POINT('Ctrl Pts',(-14.3963438928318,14.2948938650605,
132.715871778826)) ;
#120812=CARTESIAN_POINT('Ctrl Pts',(-14.3372225228914,14.1259509639325,
132.509807857198)) ;
#120813=CARTESIAN_POINT('Ctrl Pts',(-14.2956197860169,13.9085226372069,
132.355294318318)) ;
#120814=CARTESIAN_POINT('Ctrl Pts',(-14.2743647159268,13.6557404486892,
132.26008749006)) ;
#120815=CARTESIAN_POINT('Ctrl Pts',(-14.2758917339881,13.3866405250996,
132.231488180435)) ;
#120816=CARTESIAN_POINT('Ctrl Pts',(-14.3011573659847,13.1181023923962,
132.271965026739)) ;
#120817=CARTESIAN_POINT('Ctrl Pts',(-14.3484050438208,12.8743682502049,
132.377050604409)) ;
#120818=CARTESIAN_POINT('Ctrl Pts',(-14.4156978747053,12.6679957013257,
132.540429498857)) ;
#120819=CARTESIAN_POINT('Ctrl Pts',(-14.4984992937558,12.5164143784842,
132.749208600845)) ;
#120820=CARTESIAN_POINT('Ctrl Pts',(-14.5917693941425,12.4295970136061,
132.988543123613)) ;
#120821=CARTESIAN_POINT('Ctrl Pts',(-14.6895186039868,12.4140261381013,
133.240964207369)) ;
#120822=CARTESIAN_POINT('Ctrl Pts',(-14.7854846163672,12.4707103540387,
133.488174367292)) ;
#120823=CARTESIAN_POINT('Ctrl Pts',(-14.8735159764431,12.595906863769,133.712181723645)) ;
#120824=CARTESIAN_POINT('Ctrl Pts',(-14.9477237496053,12.7791143335627,
133.895987787412)) ;
#120825=CARTESIAN_POINT('Ctrl Pts',(-15.0044945348177,13.0114294021893,
134.028419908865)) ;
#120826=CARTESIAN_POINT('Ctrl Pts',(-15.0390399487791,13.2689900400404,
134.096517875508)) ;
#120827=CARTESIAN_POINT('Ctrl Pts',(-15.0508899923374,13.5409258374442,
134.097867257872)) ;
#120828=CARTESIAN_POINT('Ctrl Pts',(-15.0392557170542,13.8029841851952,
134.030803559731)) ;
#120829=CARTESIAN_POINT('Ctrl Pts',(-15.0058370198303,14.0385609610044,
133.899998507003)) ;
#120830=CARTESIAN_POINT('Ctrl Pts',(-14.9538399076615,14.229423171085,133.715008796875)) ;
#120831=CARTESIAN_POINT('Ctrl Pts',(-14.8877137168842,14.3627051887218,
133.488747191819)) ;
#120832=CARTESIAN_POINT('Ctrl Pts',(-14.8127359767209,14.4288334278673,
133.236570650323)) ;
#120833=CARTESIAN_POINT('Ctrl Pts',(-14.7352173723857,14.4228924311934,
132.97701086134)) ;
#120834=CARTESIAN_POINT('Ctrl Pts',(-14.6611248919809,14.3451233913639,
132.727361195705)) ;
#120835=CARTESIAN_POINT('Ctrl Pts',(-14.5968447070673,14.2008972200028,
132.506395013173)) ;
#120836=CARTESIAN_POINT('Ctrl Pts',(-14.5478751348737,14.0023959452744,
132.330379198133)) ;
#120837=CARTESIAN_POINT('Ctrl Pts',(-14.5178450832966,13.7610317231258,
132.209459223291)) ;
#120838=CARTESIAN_POINT('Ctrl Pts',(-14.5100259463151,13.496756912036,132.153602141983)) ;
#120839=CARTESIAN_POINT('Ctrl Pts',(-14.5256011538682,13.2257685064712,
132.165897452881)) ;
#120840=CARTESIAN_POINT('Ctrl Pts',(-14.5642253942489,12.9695425857073,
132.245607348793)) ;
#120841=CARTESIAN_POINT('Ctrl Pts',(-14.6239259490414,12.7456271494707,
132.386844216458)) ;
#120842=CARTESIAN_POINT('Ctrl Pts',(-14.7006990228845,12.5709695173834,
132.578111696268)) ;
#120843=CARTESIAN_POINT('Ctrl Pts',(-14.7905491933371,12.4565179049814,
132.807400489142)) ;
#120844=CARTESIAN_POINT('Ctrl Pts',(-14.8871250622566,12.4114773771493,
133.056433988563)) ;
#120845=CARTESIAN_POINT('Ctrl Pts',(-14.9851299631796,12.4394645505146,
133.309400564807)) ;
#120846=CARTESIAN_POINT('Ctrl Pts',(-15.0764284936881,12.5368907047146,
133.543217059238)) ;
#120847=CARTESIAN_POINT('Ctrl Pts',(-15.1574847834624,12.6994727146824,
133.746665039927)) ;
#120848=CARTESIAN_POINT('Ctrl Pts',(-15.2211909363152,12.9112843843373,
133.899900022678)) ;
#120849=CARTESIAN_POINT('Ctrl Pts',(-15.2654725078526,13.1634090082974,
133.995846242239)) ;
#120850=CARTESIAN_POINT('Ctrl Pts',(-15.2864378367501,13.4300956045555,
134.024226361752)) ;
#120851=CARTESIAN_POINT('Ctrl Pts',(-15.2843390545469,13.6985487061805,
133.984939701581)) ;
#120852=CARTESIAN_POINT('Ctrl Pts',(-15.2593145509194,13.9480246768514,
133.878558343557)) ;
#120853=CARTESIAN_POINT('Ctrl Pts',(-15.2146255465162,14.1576527966606,
133.715072135231)) ;
#120854=CARTESIAN_POINT('Ctrl Pts',(-15.1535306948074,14.3162850326807,
133.50342445039)) ;
#120855=CARTESIAN_POINT('Ctrl Pts',(-15.0813082659069,14.4106899990105,
133.25926896319)) ;
#120856=CARTESIAN_POINT('Ctrl Pts',(-15.0038819502148,14.4339585104257,
132.999884500443)) ;
#120857=CARTESIAN_POINT('Ctrl Pts',(-14.928137987027,14.3853107488566,132.745666313131)) ;
#120858=CARTESIAN_POINT('Ctrl Pts',(-14.8589321201176,14.2669553900087,
132.510203051672)) ;
#120859=CARTESIAN_POINT('Ctrl Pts',(-14.8031390853071,14.0883945363266,
132.314103537993)) ;
#120860=CARTESIAN_POINT('Ctrl Pts',(-14.7650760835763,13.8631866954131,
132.169904108232)) ;
#120861=CARTESIAN_POINT('Ctrl Pts',(-14.747976795724,13.6057119879249,132.086827558504)) ;
#120862=CARTESIAN_POINT('Ctrl Pts',(-14.7539914356653,13.3350527616499,
132.071265695883)) ;
#120863=CARTESIAN_POINT('Ctrl Pts',(-14.7834351780099,13.0707552698518,
132.124144780644)) ;
#120864=CARTESIAN_POINT('Ctrl Pts',(-14.8346901939508,12.8321485931701,
132.240824879715)) ;
#120865=CARTESIAN_POINT('Ctrl Pts',(-14.9055915104809,12.6344629226598,
132.414633314627)) ;
#120866=CARTESIAN_POINT('Ctrl Pts',(-14.9903658745253,12.4951761456202,
132.629340258018)) ;
#120867=CARTESIAN_POINT('Ctrl Pts',(-15.0849702300836,12.4210995999737,
132.872555756299)) ;
#120868=CARTESIAN_POINT('Ctrl Pts',(-15.1831256127438,12.4192964340424,
133.126073926616)) ;
#120869=CARTESIAN_POINT('Ctrl Pts',(-15.2778095628797,12.4890492714601,
133.369627717516)) ;
#120870=CARTESIAN_POINT('Ctrl Pts',(-15.3640763770914,12.6268327661457,
133.588333531199)) ;
#120871=CARTESIAN_POINT('Ctrl Pts',(-15.4349360468843,12.8195831784206,
133.762439588941)) ;
#120872=CARTESIAN_POINT('Ctrl Pts',(-15.4876340744907,13.0571003299884,
133.883190871599)) ;
#120873=CARTESIAN_POINT('Ctrl Pts',(-15.518245025264,13.320280679744,133.939518694644)) ;
#120874=CARTESIAN_POINT('Ctrl Pts',(-15.5255697583556,13.5914917582005,
133.927733313208)) ;
#120875=CARTESIAN_POINT('Ctrl Pts',(-15.509601546287,13.8505567194106,133.847905316659)) ;
#120876=CARTESIAN_POINT('Ctrl Pts',(-15.472551823714,14.0777829909349,133.706668786412)) ;
#120877=CARTESIAN_POINT('Ctrl Pts',(-15.4175582389666,14.2590886738723,
133.512904737009)) ;
#120878=CARTESIAN_POINT('Ctrl Pts',(-15.3490611968896,14.3807167115641,
133.279584839209)) ;
#120879=CARTESIAN_POINT('Ctrl Pts',(-15.2731574758069,14.433343615208,133.024730945337)) ;
#120880=CARTESIAN_POINT('Ctrl Pts',(-15.1956188392081,14.4133893489329,
132.765008849078)) ;
#120881=CARTESIAN_POINT('Ctrl Pts',(-15.1234225876608,14.3229978009541,
132.521122428361)) ;
#120882=CARTESIAN_POINT('Ctrl Pts',(-15.0616114780319,14.1680349923561,
132.307428002309)) ;
#120883=CARTESIAN_POINT('Ctrl Pts',(-15.0157162337173,13.959434776873,132.140210034788)) ;
#120884=CARTESIAN_POINT('Ctrl Pts',(-14.9897310083251,13.712829168107,132.031206744906)) ;
#120885=CARTESIAN_POINT('Ctrl Pts',(-14.9863184802919,13.4442543283008,
131.987991189862)) ;
#120886=CARTESIAN_POINT('Ctrl Pts',(-15.0061744908591,13.176694407093,132.013075122292)) ;
#120887=CARTESIAN_POINT('Ctrl Pts',(-15.049237718297,12.9234094710806,132.105508422183)) ;
#120888=CARTESIAN_POINT('Ctrl Pts',(-15.11234976022,12.7086523175308,132.256861037713)) ;
#120889=CARTESIAN_POINT('Ctrl Pts',(-15.1918550986888,12.5444332801825,
132.456104683496)) ;
#120890=CARTESIAN_POINT('Ctrl Pts',(-15.2838721870511,12.4422654275157,
132.691592196494)) ;
#120891=CARTESIAN_POINT('Ctrl Pts',(-15.3809241567571,12.4113238215259,
132.942067261817)) ;
#120892=CARTESIAN_POINT('Ctrl Pts',(-15.4776269938542,12.452199983914,133.191494717966)) ;
#120893=CARTESIAN_POINT('Ctrl Pts',(-15.5682516153267,12.5635389999469,
133.422952701096)) ;
#120894=CARTESIAN_POINT('Ctrl Pts',(-15.6457754650984,12.7354102811942,
133.616413756961)) ;
#120895=CARTESIAN_POINT('Ctrl Pts',(-15.7063953713452,12.9568498442606,
133.76038439875)) ;
#120896=CARTESIAN_POINT('Ctrl Pts',(-15.7461813643963,13.2117694969246,
133.843491058777)) ;
#120897=CARTESIAN_POINT('Ctrl Pts',(-15.7630285422846,13.48252854114,133.859501479823)) ;
#120898=CARTESIAN_POINT('Ctrl Pts',(-15.7563071367863,13.748482945783,133.806725663127)) ;
#120899=CARTESIAN_POINT('Ctrl Pts',(-15.7275509102973,13.9900671624614,
133.689733432458)) ;
#120900=CARTESIAN_POINT('Ctrl Pts',(-15.6792982108687,14.1922209506685,
133.515647821569)) ;
#120901=CARTESIAN_POINT('Ctrl Pts',(-15.6155830086315,14.3393855753319,
133.296320311479)) ;
#120902=CARTESIAN_POINT('Ctrl Pts',(-15.5422295688276,14.4204077482377,
133.04899534508)) ;
#120903=CARTESIAN_POINT('Ctrl Pts',(-15.4646880996919,14.4304302068623,
132.789342072121)) ;
#120904=CARTESIAN_POINT('Ctrl Pts',(-15.389253543915,14.3678711174913,132.53575988027)) ;
#120905=CARTESIAN_POINT('Ctrl Pts',(-15.3224480781091,14.2376926994235,
132.307474173055)) ;
#120906=CARTESIAN_POINT('Ctrl Pts',(-15.2695791733511,14.0489882455827,
132.119877916052)) ;
#120907=CARTESIAN_POINT('Ctrl Pts',(-15.2352419555811,13.8164455432918,
131.986552716391)) ;
#120908=CARTESIAN_POINT('Ctrl Pts',(-15.2224352712447,13.5541088077793,
131.915902354574)) ;
#120909=CARTESIAN_POINT('Ctrl Pts',(-15.2328633064654,13.2846771651641,
131.913420948601)) ;
#120910=CARTESIAN_POINT('Ctrl Pts',(-15.2666207126356,13.0230234432121,
131.978819239946)) ;
#120911=CARTESIAN_POINT('Ctrl Pts',(-15.3219248693909,12.7908726515439,
132.107264949997)) ;
#120912=CARTESIAN_POINT('Ctrl Pts',(-15.3955596009651,12.6038717726337,
132.289241148171)) ;
#120913=CARTESIAN_POINT('Ctrl Pts',(-15.4829738673042,12.4755977885113,
132.511478747125)) ;
#120914=CARTESIAN_POINT('Ctrl Pts',(-15.5787009690955,12.4151865367556,
132.757979288962)) ;
#120915=CARTESIAN_POINT('Ctrl Pts',(-15.6763807869398,12.4270410724712,
133.010240147476)) ;
#120916=CARTESIAN_POINT('Ctrl Pts',(-15.7698857979697,12.5098502892393,
133.250326255073)) ;
#120917=CARTESIAN_POINT('Ctrl Pts',(-15.8537091275427,12.6589866450951,
133.46194433181)) ;
#120918=CARTESIAN_POINT('Ctrl Pts',(-15.9215542492779,12.8615687451882,
133.627140073067)) ;
#120919=CARTESIAN_POINT('Ctrl Pts',(-15.9702371826774,13.1050266769027,
133.736219667067)) ;
#120920=CARTESIAN_POINT('Ctrl Pts',(-15.9965613702119,13.3718444110737,
133.779924979936)) ;
#120921=CARTESIAN_POINT('Ctrl Pts',(-15.999444902403,13.6411904453346,133.755302949557)) ;
#120922=CARTESIAN_POINT('Ctrl Pts',(-15.979202745745,13.8968635155474,133.662853690068)) ;
#120923=CARTESIAN_POINT('Ctrl Pts',(-15.9385455558626,14.1159779799374,
133.511147245029)) ;
#120924=CARTESIAN_POINT('Ctrl Pts',(-15.8804481741695,14.2873257027271,
133.308202911175)) ;
#120925=CARTESIAN_POINT('Ctrl Pts',(-15.8103663899591,14.3958947377193,
133.070410963587)) ;
#120926=CARTESIAN_POINT('Ctrl Pts',(-15.733745623836,14.4351265097039,132.813466935671)) ;
#120927=CARTESIAN_POINT('Ctrl Pts',(-15.6568737721267,14.401957868835,132.555802882805)) ;
#120928=CARTESIAN_POINT('Ctrl Pts',(-15.5857722650305,14.2982652122168,
132.314890619411)) ;
#120929=CARTESIAN_POINT('Ctrl Pts',(-15.5267629965934,14.1324802087574,
132.109458823216)) ;
#120930=CARTESIAN_POINT('Ctrl Pts',(-15.484312630846,13.9154628269439,131.9523001242)) ;
#120931=CARTESIAN_POINT('Ctrl Pts',(-15.4624445929521,13.6633712406997,
131.855306338031)) ;
#120932=CARTESIAN_POINT('Ctrl Pts',(-15.4633405140607,13.3940849340156,
131.824809337026)) ;
#120933=CARTESIAN_POINT('Ctrl Pts',(-15.4877875794486,13.1263052582701,
131.863039831368)) ;
#120934=CARTESIAN_POINT('Ctrl Pts',(-15.5346489194363,12.8804158513159,
131.96682400019)) ;
#120935=CARTESIAN_POINT('Ctrl Pts',(-15.6012737282025,12.6733662735578,
132.128348254486)) ;
#120936=CARTESIAN_POINT('Ctrl Pts',(-15.6838110767312,12.5197379021673,
132.336300360141)) ;
#120937=CARTESIAN_POINT('Ctrl Pts',(-15.7769029536586,12.4310982059369,
132.575107599234)) ;
#120938=CARTESIAN_POINT('Ctrl Pts',(-15.8743413642468,12.4134628316865,
132.82671087668)) ;
#120939=CARTESIAN_POINT('Ctrl Pts',(-15.9705403191487,12.4679867596538,
133.074572192467)) ;
#120940=CARTESIAN_POINT('Ctrl Pts',(-16.0590904745147,12.5916525961337,
133.300018721976)) ;
#120941=CARTESIAN_POINT('Ctrl Pts',(-16.1336468131636,12.7734685194903,
133.484855342896)) ;
#120942=CARTESIAN_POINT('Ctrl Pts',(-16.1906862831964,13.0028689239805,
133.61830847906)) ;
#120943=CARTESIAN_POINT('Ctrl Pts',(-16.226261276871,13.261962548957,133.689131888325)) ;
#120944=CARTESIAN_POINT('Ctrl Pts',(-16.2386405247801,13.5340193336117,
133.692012008431)) ;
#120945=CARTESIAN_POINT('Ctrl Pts',(-16.227691036414,13.7955676266414,133.627073124232)) ;
#120946=CARTESIAN_POINT('Ctrl Pts',(-16.1948762080394,14.0322614564451,
133.498024343725)) ;
#120947=CARTESIAN_POINT('Ctrl Pts',(-16.1434360380022,14.2243899010379,
133.314703125322)) ;
#120948=CARTESIAN_POINT('Ctrl Pts',(-16.0775677422439,14.3598901604785,
133.089143122656)) ;
#120949=CARTESIAN_POINT('Ctrl Pts',(-16.0024062401398,14.4280176399282,
132.836283097058)) ;
#120950=CARTESIAN_POINT('Ctrl Pts',(-15.9253625454778,14.4241023567618,
132.578322250813)) ;
#120951=CARTESIAN_POINT('Ctrl Pts',(-15.8508506102757,14.3482279673457,
132.327343287973)) ;
#120952=CARTESIAN_POINT('Ctrl Pts',(-15.786360116079,14.2060723674291,132.105843130321)) ;
#120953=CARTESIAN_POINT('Ctrl Pts',(-15.7368242702798,14.0086807740354,
131.928116094623)) ;
#120954=CARTESIAN_POINT('Ctrl Pts',(-15.7062275475401,13.7691470824975,
131.805652706501)) ;
#120955=CARTESIAN_POINT('Ctrl Pts',(-15.6976947499871,13.5031160209837,
131.7474354851)) ;
#120956=CARTESIAN_POINT('Ctrl Pts',(-15.7127216465963,13.2327333331826,
131.758218797029)) ;
#120957=CARTESIAN_POINT('Ctrl Pts',(-15.7505752615138,12.976776614233,131.835791024487)) ;
#120958=CARTESIAN_POINT('Ctrl Pts',(-15.8095780779271,12.7518156970481,
131.975032564164)) ;
#120959=CARTESIAN_POINT('Ctrl Pts',(-15.8862411789886,12.5749030333723,
132.165838894875)) ;
#120960=CARTESIAN_POINT('Ctrl Pts',(-15.9756600026082,12.4587258582811,
132.393929098427)) ;
#120961=CARTESIAN_POINT('Ctrl Pts',(-16.0726294742164,12.4118884067616,
132.643935728496)) ;
#120962=CARTESIAN_POINT('Ctrl Pts',(-16.1693474818951,12.4371448006442,
132.893616726414)) ;
#120963=CARTESIAN_POINT('Ctrl Pts',(-16.2619924518505,12.5335140246063,
133.130965469335)) ;
#120964=CARTESIAN_POINT('Ctrl Pts',(-16.3427349664474,12.6929505687292,
133.333809412538)) ;
#120965=CARTESIAN_POINT('Ctrl Pts',(-16.4075929857113,12.9053983640665,
133.490085624717)) ;
#120966=CARTESIAN_POINT('Ctrl Pts',(-16.4520337457546,13.1539498783259,
133.586871749901)) ;
#120967=CARTESIAN_POINT('Ctrl Pts',(-16.4740125729542,13.422675078525,133.617911121948)) ;
#120968=CARTESIAN_POINT('Ctrl Pts',(-16.4724822003861,13.691089143288,133.580327726125)) ;
#120969=CARTESIAN_POINT('Ctrl Pts',(-16.4481242362547,13.9413684458137,
133.475899146845)) ;
#120970=CARTESIAN_POINT('Ctrl Pts',(-16.4038361295165,14.1526799240858,
133.313515710715)) ;
#120971=CARTESIAN_POINT('Ctrl Pts',(-16.3432199423983,14.3125333467772,
133.103328027861)) ;
#120972=CARTESIAN_POINT('Ctrl Pts',(-16.2714680049075,14.408819463409,132.860643965138)) ;
#120973=CARTESIAN_POINT('Ctrl Pts',(-16.1938245217602,14.4343198914763,
132.600502617637)) ;
#120974=CARTESIAN_POINT('Ctrl Pts',(-16.1181031010312,14.3877722038871,
132.346416016408)) ;
#120975=CARTESIAN_POINT('Ctrl Pts',(-16.0485304784478,14.2711470779282,
132.109837946035)) ;
#120976=CARTESIAN_POINT('Ctrl Pts',(-15.9925306968979,14.0951742319451,
131.913300087355)) ;
#120977=CARTESIAN_POINT('Ctrl Pts',(-15.953648770791,13.870335302896,131.766563806448)) ;
#120978=CARTESIAN_POINT('Ctrl Pts',(-15.9359291073685,13.6128358613542,
131.681599922722)) ;
#120979=CARTESIAN_POINT('Ctrl Pts',(-15.9412906023611,13.3431052342381,
131.664226615723)) ;
#120980=CARTESIAN_POINT('Ctrl Pts',(-15.9699469241256,13.0784068980914,
131.71482665286)) ;
#120981=CARTESIAN_POINT('Ctrl Pts',(-16.0211125920356,12.8371324748468,
131.830982955641)) ;
#120982=CARTESIAN_POINT('Ctrl Pts',(-16.0908996434181,12.639991514166,132.001852443921)) ;
#120983=CARTESIAN_POINT('Ctrl Pts',(-16.1757171914526,12.4979352238862,
132.21650801765)) ;
#120984=CARTESIAN_POINT('Ctrl Pts',(-16.2703730971549,12.4220838446985,
132.459808435532)) ;
#120985=CARTESIAN_POINT('Ctrl Pts',(-16.3683183392038,12.4184701426874,
132.712779770869)) ;
#120986=CARTESIAN_POINT('Ctrl Pts',(-16.4628394543541,12.4860425111682,
132.955969482712)) ;
#120987=CARTESIAN_POINT('Ctrl Pts',(-16.5492355946798,12.62129710121,133.175156001814)) ;
#120988=CARTESIAN_POINT('Ctrl Pts',(-16.6209794354091,12.8133840710904,
133.351683229808)) ;
#120989=CARTESIAN_POINT('Ctrl Pts',(-16.6742798344133,13.0503650213175,
133.474145212659)) ;
#120990=CARTESIAN_POINT('Ctrl Pts',(-16.7054383248983,13.3123038567085,
133.532167225324)) ;
#120991=CARTESIAN_POINT('Ctrl Pts',(-16.7134737697217,13.5832779933084,
133.522492394927)) ;
#120992=CARTESIAN_POINT('Ctrl Pts',(-16.6982303620489,13.8428844537896,
133.444800801758)) ;
#120993=CARTESIAN_POINT('Ctrl Pts',(-16.6616516930359,14.0720013816764,
133.304834740476)) ;
#120994=CARTESIAN_POINT('Ctrl Pts',(-16.6071169159106,14.2546155978529,
133.11243298478)) ;
#120995=CARTESIAN_POINT('Ctrl Pts',(-16.5391209400141,14.3779471702252,
132.880660794707)) ;
#120996=CARTESIAN_POINT('Ctrl Pts',(-16.4632550759513,14.4327785527786,
132.625869651701)) ;
#120997=CARTESIAN_POINT('Ctrl Pts',(-16.3859214509523,14.4152048360803,
132.366858853552)) ;
#120998=CARTESIAN_POINT('Ctrl Pts',(-16.3131469320527,14.3266409428597,
132.121134580323)) ;
#120999=CARTESIAN_POINT('Ctrl Pts',(-16.2508735851622,14.1729214671605,
131.906029507347)) ;
#121000=CARTESIAN_POINT('Ctrl Pts',(-16.2046102027505,13.9662155184911,
131.737830097701)) ;
#121001=CARTESIAN_POINT('Ctrl Pts',(-16.1779888101469,13.7208186547473,
131.627002572066)) ;
#121002=CARTESIAN_POINT('Ctrl Pts',(-16.1738448501189,13.4521886594885,
131.581602362447)) ;
#121003=CARTESIAN_POINT('Ctrl Pts',(-16.1931355127838,13.1838897369756,
131.604966282919)) ;
#121004=CARTESIAN_POINT('Ctrl Pts',(-16.2352668534616,12.9313138648893,
131.694879378208)) ;
#121005=CARTESIAN_POINT('Ctrl Pts',(-16.2979953414801,12.7142071163423,
131.844978217263)) ;
#121006=CARTESIAN_POINT('Ctrl Pts',(-16.3773062651453,12.5481822878489,
132.043585307447)) ;
#121007=CARTESIAN_POINT('Ctrl Pts',(-16.4685437718777,12.4445945503844,
132.27697928454)) ;
#121008=CARTESIAN_POINT('Ctrl Pts',(-16.5655957618824,12.4110615289685,
132.527422237429)) ;
#121009=CARTESIAN_POINT('Ctrl Pts',(-16.6628557772642,12.4502003413461,
132.778318054091)) ;
#121010=CARTESIAN_POINT('Ctrl Pts',(-16.7531335309511,12.5587981618695,
133.008994097715)) ;
#121011=CARTESIAN_POINT('Ctrl Pts',(-16.8314074438916,12.7290993092181,
133.20455574507)) ;
#121012=CARTESIAN_POINT('Ctrl Pts',(-16.8928577533825,12.950564316011,133.350782950407)) ;
#121013=CARTESIAN_POINT('Ctrl Pts',(-16.9330790264365,13.2039534170359,
133.435275758517)) ;
#121014=CARTESIAN_POINT('Ctrl Pts',(-16.9506380553928,13.4737768777198,
133.45345380249)) ;
#121015=CARTESIAN_POINT('Ctrl Pts',(-16.9446670676314,13.7408243981145,
133.402794669402)) ;
#121016=CARTESIAN_POINT('Ctrl Pts',(-16.9163090827626,13.9843829005592,
133.286806456363)) ;
#121017=CARTESIAN_POINT('Ctrl Pts',(-16.8687835725521,14.1867700874977,
133.115020926219)) ;
#121018=CARTESIAN_POINT('Ctrl Pts',(-16.8054030141767,14.3360223630702,
132.896629962351)) ;
#121019=CARTESIAN_POINT('Ctrl Pts',(-16.7322445813577,14.4190305114461,
132.649874649277)) ;
#121020=CARTESIAN_POINT('Ctrl Pts',(-16.6547444226988,14.4311357302908,
132.390344056005)) ;
#121021=CARTESIAN_POINT('Ctrl Pts',(-16.5792695493848,14.3708887604269,
132.136703574011)) ;
#121022=CARTESIAN_POINT('Ctrl Pts',(-16.5120163560413,14.2422926303469,
131.907041000821)) ;
#121023=CARTESIAN_POINT('Ctrl Pts',(-16.4588725477531,14.0562618591324,
131.718813468793)) ;
#121024=CARTESIAN_POINT('Ctrl Pts',(-16.4236593544539,13.8231736000303,
131.582683084744)) ;
#121025=CARTESIAN_POINT('Ctrl Pts',(-16.4102829007904,13.5622215659962,
131.510485072681)) ;
#121026=CARTESIAN_POINT('Ctrl Pts',(-16.4200291090512,13.2923509313982,
131.505951545336)) ;
#121027=CARTESIAN_POINT('Ctrl Pts',(-16.4530192792313,13.0307855165856,
131.569197474403)) ;
#121028=CARTESIAN_POINT('Ctrl Pts',(-16.5079078696725,12.796715819409,131.696311601221)) ;
#121029=CARTESIAN_POINT('Ctrl Pts',(-16.5810548280508,12.6083942037896,
131.876886012649)) ;
#121030=CARTESIAN_POINT('Ctrl Pts',(-16.6682374248203,12.4782666718545,
132.098415600761)) ;
#121031=CARTESIAN_POINT('Ctrl Pts',(-16.7634938948967,12.4160107552107,
132.343651107937)) ;
#121032=CARTESIAN_POINT('Ctrl Pts',(-16.8614539449369,12.4255889321841,
132.596647127972)) ;
#121033=CARTESIAN_POINT('Ctrl Pts',(-16.9555012968993,12.5070743683389,
132.838185834921)) ;
#121034=CARTESIAN_POINT('Ctrl Pts',(-17.0392450020579,12.6538728233386,
133.049737407758)) ;
#121035=CARTESIAN_POINT('Ctrl Pts',(-17.107726307674,12.8553500132408,133.216734480995)) ;
#121036=CARTESIAN_POINT('Ctrl Pts',(-17.1570082574672,13.0981034422233,
133.327545614228)) ;
#121037=CARTESIAN_POINT('Ctrl Pts',(-17.183965292424,13.3649638787798,133.373050395986)) ;
#121038=CARTESIAN_POINT('Ctrl Pts',(-17.1874265803459,13.633409473525,133.350241103702)) ;
#121039=CARTESIAN_POINT('Ctrl Pts',(-17.1680409732944,13.8886868708514,
133.260455975359)) ;
#121040=CARTESIAN_POINT('Ctrl Pts',(-17.12776078413,14.1104518503625,133.109655864797)) ;
#121041=CARTESIAN_POINT('Ctrl Pts',(-17.0700684671704,14.2832226352683,
132.90790533618)) ;
#121042=CARTESIAN_POINT('Ctrl Pts',(-17.0003049596219,14.3937886252325,
132.671056763834)) ;
#121043=CARTESIAN_POINT('Ctrl Pts',(-16.9234305592928,14.4350213811874,
132.413222353031)) ;
#121044=CARTESIAN_POINT('Ctrl Pts',(-16.8468492367316,14.4038716557598,
132.156565176017)) ;
#121045=CARTESIAN_POINT('Ctrl Pts',(-16.7753697290314,14.3020574418522,
131.914495582995)) ;
#121046=CARTESIAN_POINT('Ctrl Pts',(-16.7159734074721,14.1377082714835,
131.707924566398)) ;
#121047=CARTESIAN_POINT('Ctrl Pts',(-16.6730770027358,13.9225120842828,
131.549544677542)) ;
#121048=CARTESIAN_POINT('Ctrl Pts',(-16.6505166862748,13.6705375094453,
131.45044216059)) ;
#121049=CARTESIAN_POINT('Ctrl Pts',(-16.6508051559261,13.4018845199762,
131.418221579722)) ;
#121050=CARTESIAN_POINT('Ctrl Pts',(-16.6744356225866,13.1344381552283,
131.454156161431)) ;
#121051=CARTESIAN_POINT('Ctrl Pts',(-16.7209299074623,12.8864832879891,
131.556700740614)) ;
#121052=CARTESIAN_POINT('Ctrl Pts',(-16.7867037912973,12.679196010264,131.715913956127)) ;
#121053=CARTESIAN_POINT('Ctrl Pts',(-16.8689665205321,12.5233811225036,
131.922997628966)) ;
#121054=CARTESIAN_POINT('Ctrl Pts',(-16.9617056853245,12.4327816487888,
132.160820091053)) ;
#121055=CARTESIAN_POINT('Ctrl Pts',(-17.0594012996445,12.4129159597619,
132.41307010867)) ;
#121056=CARTESIAN_POINT('Ctrl Pts',(-17.1556153739254,12.4655032985934,
132.66101261288)) ;
#121057=CARTESIAN_POINT('Ctrl Pts',(-17.2441896100086,12.5866529745153,
132.886646653344)) ;
#121058=CARTESIAN_POINT('Ctrl Pts',(-17.3195526790658,12.767439628638,133.073711296189)) ;
#121059=CARTESIAN_POINT('Ctrl Pts',(-17.377292110819,12.9966808158701,133.209093801097)) ;
#121060=CARTESIAN_POINT('Ctrl Pts',(-17.4132761779649,13.2541242728622,
133.281251443548)) ;
#121061=CARTESIAN_POINT('Ctrl Pts',(-17.4264022871086,13.524842234863,133.286467705085)) ;
#121062=CARTESIAN_POINT('Ctrl Pts',(-17.4161430564136,13.7882272307475,
133.223383906437)) ;
#121063=CARTESIAN_POINT('Ctrl Pts',(-17.383874755988,14.0260984495824,133.095908384181)) ;
#121064=CARTESIAN_POINT('Ctrl Pts',(-17.3327899753643,14.2200232579374,
132.913557519948)) ;
#121065=CARTESIAN_POINT('Ctrl Pts',(-17.2673674124666,14.3567722758536,
132.6893718229)) ;
#121066=CARTESIAN_POINT('Ctrl Pts',(-17.1928382513417,14.4269174595849,
132.438549893294)) ;
#121067=CARTESIAN_POINT('Ctrl Pts',(-17.1151930703958,14.4252572802329,
132.178577294835)) ;
#121068=CARTESIAN_POINT('Ctrl Pts',(-17.0407081937327,14.3512844314495,
131.927763325467)) ;
#121069=CARTESIAN_POINT('Ctrl Pts',(-16.9760740580518,14.2117349601844,
131.705971266209)) ;
#121070=CARTESIAN_POINT('Ctrl Pts',(-16.9257713272981,14.0152547415916,
131.52588164766)) ;
#121071=CARTESIAN_POINT('Ctrl Pts',(-16.8945605226789,13.7756398670369,
131.401498225142)) ;
#121072=CARTESIAN_POINT('Ctrl Pts',(-16.88541891899,13.5122934272068,131.341781181152)) ;
#121073=CARTESIAN_POINT('Ctrl Pts',(-16.8996517098331,13.2411299536141,
131.350160139664)) ;
#121074=CARTESIAN_POINT('Ctrl Pts',(-16.9369013734199,12.9839532693091,
131.425907297011)) ;
#121075=CARTESIAN_POINT('Ctrl Pts',(-16.9955710856029,12.7572239501203,
131.564068015513)) ;
#121076=CARTESIAN_POINT('Ctrl Pts',(-17.071467998947,12.5794741125724,131.752779615537)) ;
#121077=CARTESIAN_POINT('Ctrl Pts',(-17.1608121883335,12.4611210628414,
131.980564154477)) ;
#121078=CARTESIAN_POINT('Ctrl Pts',(-17.2571503761721,12.4122668253808,
132.228903249691)) ;
#121079=CARTESIAN_POINT('Ctrl Pts',(-17.3546376058722,12.4354395157324,
132.480589572177)) ;
#121080=CARTESIAN_POINT('Ctrl Pts',(-17.4474577248439,12.5301694906382,
132.718462736226)) ;
#121081=CARTESIAN_POINT('Ctrl Pts',(-17.528398067295,12.6876686677728,132.921950991047)) ;
#121082=CARTESIAN_POINT('Ctrl Pts',(-17.5936909444915,12.898212465334,133.079574187598)) ;
#121083=CARTESIAN_POINT('Ctrl Pts',(-17.6389773689883,13.1472879217631,
133.178651901856)) ;
#121084=CARTESIAN_POINT('Ctrl Pts',(-17.6614873036012,13.4151706305656,
133.211320240868)) ;
#121085=CARTESIAN_POINT('Ctrl Pts',(-17.6606115793353,13.6833052701105,
133.175708233052)) ;
#121086=CARTESIAN_POINT('Ctrl Pts',(-17.6370969311646,13.9335262167577,
133.073884888561)) ;
#121087=CARTESIAN_POINT('Ctrl Pts',(-17.5929860893633,14.1479664881483,
132.911736516363)) ;
#121088=CARTESIAN_POINT('Ctrl Pts',(-17.5328890109081,14.3087959188899,
132.703169232262)) ;
#121089=CARTESIAN_POINT('Ctrl Pts',(-17.4613931385352,14.4069520257531,
132.461231766129)) ;
#121090=CARTESIAN_POINT('Ctrl Pts',(-17.3841812797812,14.434703937208,132.202512060337)) ;
#121091=CARTESIAN_POINT('Ctrl Pts',(-17.3078205401366,14.3899170706969,
131.946323472494)) ;
#121092=CARTESIAN_POINT('Ctrl Pts',(-17.2383885165578,14.275848167113,131.710364627399)) ;
#121093=CARTESIAN_POINT('Ctrl Pts',(-17.1816816715689,14.1010294116989,
131.511633889459)) ;
#121094=CARTESIAN_POINT('Ctrl Pts',(-17.1422631986116,13.8772033892953,
131.363323086006)) ;
#121095=CARTESIAN_POINT('Ctrl Pts',(-17.1239156778148,13.6206146695245,
131.276552146189)) ;
#121096=CARTESIAN_POINT('Ctrl Pts',(-17.128571603957,13.3509220809883,131.257110126722)) ;
#121097=CARTESIAN_POINT('Ctrl Pts',(-17.1566772042895,13.0853828321562,
131.306041738499)) ;
#121098=CARTESIAN_POINT('Ctrl Pts',(-17.2068859584364,12.8445475509271,
131.419607688918)) ;
#121099=CARTESIAN_POINT('Ctrl Pts',(-17.2763923833637,12.6449528168769,
131.589517903078)) ;
#121100=CARTESIAN_POINT('Ctrl Pts',(-17.3608585228123,12.5012606134937,
131.803156341898)) ;
#121101=CARTESIAN_POINT('Ctrl Pts',(-17.4549824595557,12.4235056415569,
132.045012563526)) ;
#121102=CARTESIAN_POINT('Ctrl Pts',(-17.5529484609703,12.4173186288012,
132.298035942043)) ;
#121103=CARTESIAN_POINT('Ctrl Pts',(-17.6482211097473,12.4833715210388,
132.543213532662)) ;
#121104=CARTESIAN_POINT('Ctrl Pts',(-17.7345330550901,12.6162286422635,
132.762314386659)) ;
#121105=CARTESIAN_POINT('Ctrl Pts',(-17.8070216390377,12.8073411346184,
132.940908095724)) ;
#121106=CARTESIAN_POINT('Ctrl Pts',(-17.8608373477978,13.0432166498449,
133.064898766188)) ;
#121107=CARTESIAN_POINT('Ctrl Pts',(-17.8926735534002,13.3046950611415,
133.124891631411)) ;
#121108=CARTESIAN_POINT('Ctrl Pts',(-17.9013624719413,13.5764464662961,
133.117037886171)) ;
#121109=CARTESIAN_POINT('Ctrl Pts',(-17.8866709778763,13.8363551234792,
133.040981956794)) ;
#121110=CARTESIAN_POINT('Ctrl Pts',(-17.8508343744671,14.0655922643217,
132.903327377715)) ;
#121111=CARTESIAN_POINT('Ctrl Pts',(-17.7966375360881,14.2503954850495,
132.711817289313)) ;
#121112=CARTESIAN_POINT('Ctrl Pts',(-17.7287032482948,14.3757154300573,
132.480127244775)) ;
#121113=CARTESIAN_POINT('Ctrl Pts',(-17.6531018723206,14.4321659963664,
132.226171168029)) ;
#121114=CARTESIAN_POINT('Ctrl Pts',(-17.5759806284613,14.416734287709,131.967888324685)) ;
#121115=CARTESIAN_POINT('Ctrl Pts',(-17.503004842333,14.330289953115,131.721586227307)) ;
#121116=CARTESIAN_POINT('Ctrl Pts',(-17.4402855682396,14.1784243130749,
131.505170261232)) ;
#121117=CARTESIAN_POINT('Ctrl Pts',(-17.3932928277742,13.9717507261075,
131.33465019109)) ;
#121118=CARTESIAN_POINT('Ctrl Pts',(-17.3662979484006,13.7284356402105,
131.222910396826)) ;
#121119=CARTESIAN_POINT('Ctrl Pts',(-17.3613675605102,13.4606301532886,
131.175263996789)) ;
#121120=CARTESIAN_POINT('Ctrl Pts',(-17.3801479950331,13.1906191848992,
131.196949420637)) ;
#121121=CARTESIAN_POINT('Ctrl Pts',(-17.4214109843812,12.9388679746563,
131.28453157571)) ;
#121122=CARTESIAN_POINT('Ctrl Pts',(-17.4837628187899,12.7195132138376,
131.43340170599)) ;
#121123=CARTESIAN_POINT('Ctrl Pts',(-17.5628590770987,12.5518557372857,
131.631327287361)) ;
#121124=CARTESIAN_POINT('Ctrl Pts',(-17.6534051668585,12.4467157582098,
131.862855290462)) ;
#121125=CARTESIAN_POINT('Ctrl Pts',(-17.750922989384,12.4110145773966,132.114468726418)) ;
#121126=CARTESIAN_POINT('Ctrl Pts',(-17.8476115268141,12.4479828338558,
132.363921471666)) ;
#121127=CARTESIAN_POINT('Ctrl Pts',(-17.9383943809633,12.5544308131199,
132.596009504229)) ;
#121128=CARTESIAN_POINT('Ctrl Pts',(-18.0175559739188,12.7245572228014,
132.793937494374)) ;
#121129=CARTESIAN_POINT('Ctrl Pts',(-18.0790907579623,12.9435040036317,
132.940630250791)) ;
#121130=CARTESIAN_POINT('Ctrl Pts',(-18.1200567127323,13.1965754591591,
133.027234652194)) ;
#121131=CARTESIAN_POINT('Ctrl Pts',(-18.1382282000561,13.4658054703846,
133.047256744435)) ;
#121132=CARTESIAN_POINT('Ctrl Pts',(-18.1329659863274,13.732871013944,132.998710444717)) ;
#121133=CARTESIAN_POINT('Ctrl Pts',(-18.10532591625,13.9772573341515,132.884851141224)) ;
#121134=CARTESIAN_POINT('Ctrl Pts',(-18.0580724361184,14.1820529613216,
132.713691198042)) ;
#121135=CARTESIAN_POINT('Ctrl Pts',(-17.9950516196932,14.3328844022839,
132.496365183043)) ;
#121136=CARTESIAN_POINT('Ctrl Pts',(-17.9218660059439,14.4178011232664,
132.249431768721)) ;
#121137=CARTESIAN_POINT('Ctrl Pts',(-17.8447787579686,14.4318123856393,
131.991276847606)) ;
#121138=CARTESIAN_POINT('Ctrl Pts',(-17.7688468684742,14.3732302589804,
131.736154808824)) ;
#121139=CARTESIAN_POINT('Ctrl Pts',(-17.7016395323525,14.2469702615313,
131.506798120837)) ;
#121140=CARTESIAN_POINT('Ctrl Pts',(-17.6479009174849,14.062146427081,131.316760898445)) ;
#121141=CARTESIAN_POINT('Ctrl Pts',(-17.6122040870272,13.8305006230351,
131.179278949391)) ;
#121142=CARTESIAN_POINT('Ctrl Pts',(-17.59812106964,13.5704780261443,131.105053850186)) ;
#121143=CARTESIAN_POINT('Ctrl Pts',(-17.6072307928306,13.2994605324582,
131.098521057394)) ;
#121144=CARTESIAN_POINT('Ctrl Pts',(-17.6396331892695,13.037734227312,131.160085006349)) ;
#121145=CARTESIAN_POINT('Ctrl Pts',(-17.6936156259918,12.803624496366,131.284711823525)) ;
#121146=CARTESIAN_POINT('Ctrl Pts',(-17.7665279927222,12.6130122644718,
131.464475667698)) ;
#121147=CARTESIAN_POINT('Ctrl Pts',(-17.8531437758454,12.4813447222013,
131.684440690985)) ;
#121148=CARTESIAN_POINT('Ctrl Pts',(-17.9485680511644,12.4167223738628,
131.930048045931)) ;
#121149=CARTESIAN_POINT('Ctrl Pts',(-18.0464149044187,12.4243656160183,
132.182759693883)) ;
#121150=CARTESIAN_POINT('Ctrl Pts',(-18.1404091781105,12.5034383279314,
132.424237107159)) ;
#121151=CARTESIAN_POINT('Ctrl Pts',(-18.2246786699213,12.6484426938847,
132.637280318487)) ;
#121152=CARTESIAN_POINT('Ctrl Pts',(-18.2938530712968,12.8490572514717,
132.806215101685)) ;
#121153=CARTESIAN_POINT('Ctrl Pts',(-18.3436429560685,13.0907450284177,
132.91853526463)) ;
#121154=CARTESIAN_POINT('Ctrl Pts',(-18.371252264237,13.3559778959346,132.966092269471)) ;
#121155=CARTESIAN_POINT('Ctrl Pts',(-18.3754407699862,13.6264773514175,
132.945172138598)) ;
#121156=CARTESIAN_POINT('Ctrl Pts',(-18.3566809485503,13.8815734058857,
132.857323251945)) ;
#121157=CARTESIAN_POINT('Ctrl Pts',(-18.3170081818755,14.1045282831523,
132.708304429531)) ;
#121158=CARTESIAN_POINT('Ctrl Pts',(-18.2597751403882,14.2789670592856,
132.507903597064)) ;
#121159=CARTESIAN_POINT('Ctrl Pts',(-18.1902019565029,14.391495176626,132.271568247248)) ;
#121160=CARTESIAN_POINT('Ctrl Pts',(-18.1137540914775,14.4348607601378,
132.015118816648)) ;
#121161=CARTESIAN_POINT('Ctrl Pts',(-18.0366821366047,14.4056890506022,
131.756845266094)) ;
#121162=CARTESIAN_POINT('Ctrl Pts',(-17.9652797618649,14.3062653151645,
131.515158727385)) ;
#121163=CARTESIAN_POINT('Ctrl Pts',(-17.9053122185148,14.143440527592,131.306846917921)) ;
#121164=CARTESIAN_POINT('Ctrl Pts',(-17.8618616267719,13.9296996140236,
131.14687021965)) ;
#121165=CARTESIAN_POINT('Ctrl Pts',(-17.8385996039929,13.6772902096435,
131.04555802276)) ;
#121166=CARTESIAN_POINT('Ctrl Pts',(-17.8382591024878,13.409949714787,131.011638149779)) ;
#121167=CARTESIAN_POINT('Ctrl Pts',(-17.8612351070141,13.1418739498075,
131.04561730523)) ;
#121168=CARTESIAN_POINT('Ctrl Pts',(-17.9068955452945,12.8939990758876,
131.145858633822)) ;
#121169=CARTESIAN_POINT('Ctrl Pts',(-17.9722749811336,12.6844790937915,
131.303812613166)) ;
#121170=CARTESIAN_POINT('Ctrl Pts',(-18.0545827898634,12.5265062627849,
131.510876033157)) ;
#121171=CARTESIAN_POINT('Ctrl Pts',(-18.1466282278198,12.4345049835541,
131.746844398259)) ;
#121172=CARTESIAN_POINT('Ctrl Pts',(-18.2445839573682,12.4124896125378,
131.999744598179)) ;
#121173=CARTESIAN_POINT('Ctrl Pts',(-18.3405183739417,12.4629155090419,
132.247009375301)) ;
#121174=CARTESIAN_POINT('Ctrl Pts',(-18.4295849017639,12.5820912846789,
132.474029520711)) ;
#121175=CARTESIAN_POINT('Ctrl Pts',(-18.5056519422923,12.762437228793,132.662998391459)) ;
#121176=CARTESIAN_POINT('Ctrl Pts',(-18.5633863090852,12.9881392996051,
132.798710522865)) ;
#121177=CARTESIAN_POINT('Ctrl Pts',(-18.6003855090257,13.2462583810271,
132.873643296643)) ;
#121178=CARTESIAN_POINT('Ctrl Pts',(-18.6141306103123,13.5176872670076,
132.880577098406)) ;
#121179=CARTESIAN_POINT('Ctrl Pts',(-18.6045499019302,13.7805945427873,
132.819592418361)) ;
#121180=CARTESIAN_POINT('Ctrl Pts',(-18.5729239333371,14.0195270315699,
132.693993288043)) ;
#121181=CARTESIAN_POINT('Ctrl Pts',(-18.522340896185,14.215038587717,132.513103225343)) ;
#121182=CARTESIAN_POINT('Ctrl Pts',(-18.4571155071067,14.3538333245836,
132.289419709278)) ;
#121183=CARTESIAN_POINT('Ctrl Pts',(-18.3828481440028,14.4259647082628,
132.039405260107)) ;
#121184=CARTESIAN_POINT('Ctrl Pts',(-18.3049142988197,14.4260802645705,
131.778458304169)) ;
#121185=CARTESIAN_POINT('Ctrl Pts',(-18.2309221252842,14.3549350188174,
131.529395653821)) ;
#121186=CARTESIAN_POINT('Ctrl Pts',(-18.1653474115413,14.2162528409401,
131.304574043089)) ;
#121187=CARTESIAN_POINT('Ctrl Pts',(-18.1147647836669,14.0213155988979,
131.123737866304)) ;
#121188=CARTESIAN_POINT('Ctrl Pts',(-18.0829568038137,13.7835941603823,
130.997714182427)) ;
#121189=CARTESIAN_POINT('Ctrl Pts',(-18.0731617219499,13.5186607714519,
130.935832378915)) ;
#121190=CARTESIAN_POINT('Ctrl Pts',(-18.08665514099,13.2494161503812,130.942305026168)) ;
#121191=CARTESIAN_POINT('Ctrl Pts',(-18.1234398333306,12.990369061565,131.01652371198)) ;
#121192=CARTESIAN_POINT('Ctrl Pts',(-18.1811896004733,12.763690008938,131.1521929047)) ;
#121193=CARTESIAN_POINT('Ctrl Pts',(-18.2573582331817,12.5829313612557,
131.341393014982)) ;
#121194=CARTESIAN_POINT('Ctrl Pts',(-18.3454804211725,12.4640788232719,
131.565967626037)) ;
#121195=CARTESIAN_POINT('Ctrl Pts',(-18.4422170243134,12.4125693563369,
131.815275161053)) ;
#121196=CARTESIAN_POINT('Ctrl Pts',(-18.5394443787495,12.4337094288139,
132.066314652827)) ;
#121197=CARTESIAN_POINT('Ctrl Pts',(-18.6326075786638,12.5263145417804,
132.305156553116)) ;
#121198=CARTESIAN_POINT('Ctrl Pts',(-18.7140301788209,12.6822587586298,
132.51002276371)) ;
#121199=CARTESIAN_POINT('Ctrl Pts',(-18.7798505478773,12.891562566965,132.669176374346)) ;
#121200=CARTESIAN_POINT('Ctrl Pts',(-18.8257122760329,13.1392603161048,
132.770001449946)) ;
#121201=CARTESIAN_POINT('Ctrl Pts',(-18.8489611088603,13.4076118666746,
132.804727708531)) ;
#121202=CARTESIAN_POINT('Ctrl Pts',(-18.8487873523375,13.6757335651874,
132.77121043275)) ;
#121203=CARTESIAN_POINT('Ctrl Pts',(-18.8256132329382,13.9281677218218,
132.670161224817)) ;
#121204=CARTESIAN_POINT('Ctrl Pts',(-18.7826335465806,14.1410411473799,
132.511768994752)) ;
#121205=CARTESIAN_POINT('Ctrl Pts',(-18.7225925718125,14.3051859898324,
132.303106999407)) ;
#121206=CARTESIAN_POINT('Ctrl Pts',(-18.6513452461886,14.4050577743806,
132.061917791597)) ;
#121207=CARTESIAN_POINT('Ctrl Pts',(-18.5741291719038,14.4349188602028,
131.80314713111)) ;
#121208=CARTESIAN_POINT('Ctrl Pts',(-18.4977975157086,14.3922309332557,
131.547105617257)) ;
#121209=CARTESIAN_POINT('Ctrl Pts',(-18.4280943233288,14.280180814084,131.310361629809)) ;
#121210=CARTESIAN_POINT('Ctrl Pts',(-18.3708931056203,14.1070359905501,
131.110179808883)) ;
#121211=CARTESIAN_POINT('Ctrl Pts',(-18.3308086150891,13.8833119230109,
130.959777523606)) ;
#121212=CARTESIAN_POINT('Ctrl Pts',(-18.3119377968156,13.6288341860585,
130.871668553615)) ;
#121213=CARTESIAN_POINT('Ctrl Pts',(-18.3159111846383,13.3582465565096,
130.850099973561)) ;
#121214=CARTESIAN_POINT('Ctrl Pts',(-18.3433003468858,13.0930921360638,
130.897041192962)) ;
#121215=CARTESIAN_POINT('Ctrl Pts',(-18.3929361586387,12.8509540623848,
131.008888330338)) ;
#121216=CARTESIAN_POINT('Ctrl Pts',(-18.4619089664474,12.6500624789761,
131.177258567627)) ;
#121217=CARTESIAN_POINT('Ctrl Pts',(-18.5461379773402,12.5043219731701,
131.390152397971)) ;
#121218=CARTESIAN_POINT('Ctrl Pts',(-18.6402475797295,12.4246931364435,
131.631910775786)) ;
#121219=CARTESIAN_POINT('Ctrl Pts',(-18.7376942627791,12.4164962070895,
131.883586283708)) ;
#121220=CARTESIAN_POINT('Ctrl Pts',(-18.8331990949263,12.480251448006,132.129424653254)) ;
#121221=CARTESIAN_POINT('Ctrl Pts',(-18.9200789894093,12.6116453538561,
132.350096934906)) ;
#121222=CARTESIAN_POINT('Ctrl Pts',(-18.9929314642051,12.8011773158268,
132.529786089759)) ;
#121223=CARTESIAN_POINT('Ctrl Pts',(-19.0472165928124,13.0350451037076,
132.655266689086)) ;
#121224=CARTESIAN_POINT('Ctrl Pts',(-19.0798709801947,13.296978163916,132.717519763971)) ;
#121225=CARTESIAN_POINT('Ctrl Pts',(-19.0892082104324,13.567734807944,132.711685741346)) ;
#121226=CARTESIAN_POINT('Ctrl Pts',(-19.0753069867193,13.8283852939848,
132.637933494416)) ;
#121227=CARTESIAN_POINT('Ctrl Pts',(-19.0398727138031,14.0598715137087,
132.501291676026)) ;
#121228=CARTESIAN_POINT('Ctrl Pts',(-18.9862483048037,14.2455588284616,
132.311544093607)) ;
#121229=CARTESIAN_POINT('Ctrl Pts',(-18.9189473375773,14.372564186769,132.081831246997)) ;
#121230=CARTESIAN_POINT('Ctrl Pts',(-18.8432518289211,14.4315964784329,
131.82748588724)) ;
#121231=CARTESIAN_POINT('Ctrl Pts',(-18.765913403393,14.4181824034525,131.568494223874)) ;
#121232=CARTESIAN_POINT('Ctrl Pts',(-18.692751570031,14.3336377789342,131.321654785139)) ;
#121233=CARTESIAN_POINT('Ctrl Pts',(-18.6298278945258,14.1840090727439,
131.10473755244)) ;
#121234=CARTESIAN_POINT('Ctrl Pts',(-18.5822566163956,13.9789557865459,
130.932534794822)) ;
#121235=CARTESIAN_POINT('Ctrl Pts',(-18.5545117957318,13.7355807215654,
130.818473396782)) ;
#121236=CARTESIAN_POINT('Ctrl Pts',(-18.5490157747953,13.4678621828446,
130.769143890178)) ;
#121237=CARTESIAN_POINT('Ctrl Pts',(-18.56696059197,13.1991327913341,130.788574867325)) ;
#121238=CARTESIAN_POINT('Ctrl Pts',(-18.6078081529041,12.945225699974,130.874755629269)) ;
#121239=CARTESIAN_POINT('Ctrl Pts',(-18.6692767013979,12.7259341324381,
131.021237394438)) ;
#121240=CARTESIAN_POINT('Ctrl Pts',(-18.7480152928831,12.5559411157644,
131.218051157817)) ;
#121241=CARTESIAN_POINT('Ctrl Pts',(-18.8388160211192,12.448546099201,131.450147238315)) ;
#121242=CARTESIAN_POINT('Ctrl Pts',(-18.9356607715897,12.4111599417381,
131.699992854173)) ;
#121243=CARTESIAN_POINT('Ctrl Pts',(-19.0325585145463,12.4456278236405,
131.95002607637)) ;
#121244=CARTESIAN_POINT('Ctrl Pts',(-19.1242640700438,12.5514145638213,
132.184545497414)) ;
#121245=CARTESIAN_POINT('Ctrl Pts',(-19.2029461856585,12.7181519506854,
132.381442208303)) ;
#121246=CARTESIAN_POINT('Ctrl Pts',(-19.265372014259,12.9364297169796,132.530607306383)) ;
#121247=CARTESIAN_POINT('Ctrl Pts',(-19.3069432913256,13.18875320047,132.618989652973)) ;
#121248=CARTESIAN_POINT('Ctrl Pts',(-19.3258346486548,13.4580633582235,
132.641077480806)) ;
#121249=CARTESIAN_POINT('Ctrl Pts',(-19.3212023059647,13.7256378176803,
132.594351189216)) ;
#121250=CARTESIAN_POINT('Ctrl Pts',(-19.2942346936325,13.9704139793173,
132.482524019834)) ;
#121251=CARTESIAN_POINT('Ctrl Pts',(-19.2474975955159,14.1767864699774,
132.312853122444)) ;
#121252=CARTESIAN_POINT('Ctrl Pts',(-19.1848424036697,14.3292888824905,
132.096591593124)) ;
#121253=CARTESIAN_POINT('Ctrl Pts',(-19.1121219052823,14.4162419172546,
131.851121689147)) ;
#121254=CARTESIAN_POINT('Ctrl Pts',(-19.0345819635708,14.4323070544899,
131.59142753805)) ;
#121255=CARTESIAN_POINT('Ctrl Pts',(-18.9591954174312,14.3764282188079,
131.338211778277)) ;
#121256=CARTESIAN_POINT('Ctrl Pts',(-18.8911670048974,14.2515624978579,
131.106230242992)) ;
#121257=CARTESIAN_POINT('Ctrl Pts',(-18.8370010450514,14.0682227623741,
130.914960556141)) ;
#121258=CARTESIAN_POINT('Ctrl Pts',(-18.800665716264,13.8370232958438,130.775522481171)) ;
#121259=CARTESIAN_POINT('Ctrl Pts',(-18.7860202678278,13.5786248872284,
130.699792853421)) ;
#121260=CARTESIAN_POINT('Ctrl Pts',(-18.7943923368573,13.3076276344917,
130.69109892016)) ;
#121261=CARTESIAN_POINT('Ctrl Pts',(-18.8260990797752,13.0452572131087,
130.75062398468)) ;
#121262=CARTESIAN_POINT('Ctrl Pts',(-18.8797421459153,12.8091511761324,
130.874119491717)) ;
#121263=CARTESIAN_POINT('Ctrl Pts',(-18.9521348210093,12.6175515473568,
131.052415653752)) ;
#121264=CARTESIAN_POINT('Ctrl Pts',(-19.0381707151645,12.4843717623364,
131.27077668053)) ;
#121265=CARTESIAN_POINT('Ctrl Pts',(-19.1335146928641,12.4175958607342,
131.516116935228)) ;
#121266=CARTESIAN_POINT('Ctrl Pts',(-19.2312708874078,12.423055511444,131.768602952943)) ;
#121267=CARTESIAN_POINT('Ctrl Pts',(-19.3256060412756,12.5002516966647,
132.011021092683)) ;
#121268=CARTESIAN_POINT('Ctrl Pts',(-19.4100225537391,12.6429372151447,
132.22459247483)) ;
#121269=CARTESIAN_POINT('Ctrl Pts',(-19.4800185412338,12.8430360326097,
132.395771984144)) ;
#121270=CARTESIAN_POINT('Ctrl Pts',(-19.5302192048766,13.0829431740334,
132.509414453532)) ;
#121271=CARTESIAN_POINT('Ctrl Pts',(-19.5585654550094,13.3482626607442,
132.55905272483)) ;
#121272=CARTESIAN_POINT('Ctrl Pts',(-19.563461465539,13.6179806011048,132.540316904992)) ;
#121273=CARTESIAN_POINT('Ctrl Pts',(-19.5452614806164,13.875457841107,132.453889291214)) ;
#121274=CARTESIAN_POINT('Ctrl Pts',(-19.5059749293386,14.0994368558722,
132.305976912958)) ;
#121275=CARTESIAN_POINT('Ctrl Pts',(-19.4495643240987,14.2743408494019,
132.108197550613)) ;
#121276=CARTESIAN_POINT('Ctrl Pts',(-19.3801028719207,14.3892596808428,
131.872091124806)) ;
#121277=CARTESIAN_POINT('Ctrl Pts',(-19.3038120358737,14.4346258040279,
131.616124870343)) ;
#121278=CARTESIAN_POINT('Ctrl Pts',(-19.2264650722539,14.4074612293383,
131.356960779271)) ;
#121279=CARTESIAN_POINT('Ctrl Pts',(-19.1548734293025,14.309698779788,131.114726202209)) ;
#121280=CARTESIAN_POINT('Ctrl Pts',(-19.0947134293815,14.149377401071,130.905995069427)) ;
#121281=CARTESIAN_POINT('Ctrl Pts',(-19.0505245415155,13.9355628699076,
130.743660881634)) ;
#121282=CARTESIAN_POINT('Ctrl Pts',(-19.0268048363665,13.6861606150325,
130.641306302118)) ;
#121283=CARTESIAN_POINT('Ctrl Pts',(-19.0257295347008,13.4167352196909,
130.604941607389)) ;
#121284=CARTESIAN_POINT('Ctrl Pts',(-19.04808383544,13.1492793409581,130.637217629532)) ;
#121285=CARTESIAN_POINT('Ctrl Pts',(-19.0930886530328,12.9005268752137,
130.73554146477)) ;
#121286=CARTESIAN_POINT('Ctrl Pts',(-19.1580129920185,12.6897474195092,
130.892153881767)) ;
#121287=CARTESIAN_POINT('Ctrl Pts',(-19.2395204495496,12.5306016213155,
131.0970291101)) ;
#121288=CARTESIAN_POINT('Ctrl Pts',(-19.3317952144819,12.4360458788129,
131.333494889956)) ;
#121289=CARTESIAN_POINT('Ctrl Pts',(-19.4295434756039,12.412131815675,131.585843687012)) ;
#121290=CARTESIAN_POINT('Ctrl Pts',(-19.5258027055626,12.4605358152628,
131.833991352613)) ;
#121291=CARTESIAN_POINT('Ctrl Pts',(-19.6152333793376,12.5784164712972,
132.062021657327)) ;
#121292=CARTESIAN_POINT('Ctrl Pts',(-19.6911374309485,12.7554817105356,
132.250804667793)) ;
#121293=CARTESIAN_POINT('Ctrl Pts',(-19.7499458974431,12.9817624941524,
132.389383273802)) ;
#121294=CARTESIAN_POINT('Ctrl Pts',(-19.7873669405952,13.238159912852,132.465701955096)) ;
#121295=CARTESIAN_POINT('Ctrl Pts',(-19.8018658367857,13.5101993099721,
132.474743662736)) ;
#121296=CARTESIAN_POINT('Ctrl Pts',(-19.7929397566941,13.7733132280516,
132.415709326912)) ;
#121297=CARTESIAN_POINT('Ctrl Pts',(-19.7617376794374,14.014064219241,132.291217067636)) ;
#121298=CARTESIAN_POINT('Ctrl Pts',(-19.7118501129715,14.209874547802,132.112528195874)) ;
#121299=CARTESIAN_POINT('Ctrl Pts',(-19.6470638524804,14.3505802758006,
131.890148790837)) ;
#121300=CARTESIAN_POINT('Ctrl Pts',(-19.5728971610653,14.4248316803085,
131.640390131458)) ;
#121301=CARTESIAN_POINT('Ctrl Pts',(-19.4950524479168,14.4272047931218,
131.379744281131)) ;
#121302=CARTESIAN_POINT('Ctrl Pts',(-19.4206848800324,14.3577939123121,
131.129487152645)) ;
#121303=CARTESIAN_POINT('Ctrl Pts',(-19.3550396477323,14.2217456845042,
130.904621923371)) ;
#121304=CARTESIAN_POINT('Ctrl Pts',(-19.3035711789367,14.0267540354523,
130.720935325739)) ;
#121305=CARTESIAN_POINT('Ctrl Pts',(-19.2714378715331,13.7911379046606,
130.594140611943)) ;
#121306=CARTESIAN_POINT('Ctrl Pts',(-19.2608853613429,13.5273989700341,
130.530120327277)) ;
#121307=CARTESIAN_POINT('Ctrl Pts',(-19.2737049786075,13.2571615768974,
130.534513540007)) ;
#121308=CARTESIAN_POINT('Ctrl Pts',(-19.3098561857145,12.9974107950377,
130.606874926784)) ;
#121309=CARTESIAN_POINT('Ctrl Pts',(-19.3671173273149,12.7695379002692,
130.741090474397)) ;
#121310=CARTESIAN_POINT('Ctrl Pts',(-19.4423816889131,12.5879936402029,
130.927827001247)) ;
#121311=CARTESIAN_POINT('Ctrl Pts',(-19.5307334454651,12.4663339482719,
131.152861116724)) ;
#121312=CARTESIAN_POINT('Ctrl Pts',(-19.6273404115409,12.4130530274037,
131.401799903801)) ;
#121313=CARTESIAN_POINT('Ctrl Pts',(-19.7244405424946,12.4321501261291,
131.652523062607)) ;
#121314=CARTESIAN_POINT('Ctrl Pts',(-19.8176642020463,12.5224108266138,
131.891610555698)) ;
#121315=CARTESIAN_POINT('Ctrl Pts',(-19.8998542340623,12.677312247728,132.098569709702)) ;
#121316=CARTESIAN_POINT('Ctrl Pts',(-19.9660793378694,12.8853932149283,
132.258922203789)) ;
#121317=CARTESIAN_POINT('Ctrl Pts',(-20.0123986186212,13.1311434716641,
132.361222124421)) ;
#121318=CARTESIAN_POINT('Ctrl Pts',(-20.0364461583432,13.400088705093,132.398168019541)) ;
#121319=CARTESIAN_POINT('Ctrl Pts',(-20.0368470691668,13.6679854897532,
132.366376497439)) ;
#121320=CARTESIAN_POINT('Ctrl Pts',(-20.0146247443677,13.9198929111463,
132.268318118694)) ;
#121321=CARTESIAN_POINT('Ctrl Pts',(-19.9716011530985,14.1367331628791,
132.109363562631)) ;
#121322=CARTESIAN_POINT('Ctrl Pts',(-19.9125458930421,14.300676127775,131.903935240049)) ;
#121323=CARTESIAN_POINT('Ctrl Pts',(-19.8411105246955,14.4034182514066,
131.661964468887)) ;
#121324=CARTESIAN_POINT('Ctrl Pts',(-19.764157971726,14.4350219446425,131.404058044713)) ;
#121325=CARTESIAN_POINT('Ctrl Pts',(-19.687633022118,14.3943912068368,131.147406929743)) ;
#121326=CARTESIAN_POINT('Ctrl Pts',(-19.6176743104395,14.2842181110636,
130.909930061093)) ;
#121327=CARTESIAN_POINT('Ctrl Pts',(-19.5600372344949,14.1123337735145,
130.708436969519)) ;
#121328=CARTESIAN_POINT('Ctrl Pts',(-19.5196200459579,13.8914432947139,
130.557293195234)) ;
#121329=CARTESIAN_POINT('Ctrl Pts',(-19.4999297703099,13.6364805468731,
130.466619696567)) ;
#121330=CARTESIAN_POINT('Ctrl Pts',(-19.5032408659291,13.3663281054811,
130.443156629942)) ;
#121331=CARTESIAN_POINT('Ctrl Pts',(-19.5299958970005,13.1002904156236,
130.488184032619)) ;
#121332=CARTESIAN_POINT('Ctrl Pts',(-19.5790361835478,12.8573186036191,
130.598302560895)) ;
#121333=CARTESIAN_POINT('Ctrl Pts',(-19.6475151340922,12.655055825907,130.765227996969)) ;
#121334=CARTESIAN_POINT('Ctrl Pts',(-19.7312879255764,12.5076994513089,
130.976825411261)) ;
#121335=CARTESIAN_POINT('Ctrl Pts',(-19.8251745452015,12.4260781925878,
131.217935682851)) ;
#121336=CARTESIAN_POINT('Ctrl Pts',(-19.9225599733253,12.4155414447684,
131.469450266245)) ;
#121337=CARTESIAN_POINT('Ctrl Pts',(-20.0189134984637,12.478090322654,131.71751385141)) ;
#121338=CARTESIAN_POINT('Ctrl Pts',(-20.1052892315539,12.6066344478164,
131.937021849716)) ;
#121339=CARTESIAN_POINT('Ctrl Pts',(-20.1789585189106,12.7952137023379,
132.118961495482)) ;
#121340=CARTESIAN_POINT('Ctrl Pts',(-20.2337494135648,13.0279819979312,
132.245943194612)) ;
#121341=CARTESIAN_POINT('Ctrl Pts',(-20.2670855507984,13.2896875880003,
132.310146572719)) ;
#121342=CARTESIAN_POINT('Ctrl Pts',(-20.2770381998546,13.5603129292438,
132.306128411386)) ;
#121343=CARTESIAN_POINT('Ctrl Pts',(-20.2638119493052,13.8211028677067,
132.234401447179)) ;
#121344=CARTESIAN_POINT('Ctrl Pts',(-20.2289487599049,14.053803313072,132.099410060731)) ;
#121345=CARTESIAN_POINT('Ctrl Pts',(-20.1757739845993,14.2410908350298,
131.910965000059)) ;
#121346=CARTESIAN_POINT('Ctrl Pts',(-20.1085725822687,14.3701941601828,
131.681445986199)) ;
#121347=CARTESIAN_POINT('Ctrl Pts',(-20.0330781315566,14.4308809616827,
131.427719983322)) ;
#121348=CARTESIAN_POINT('Ctrl Pts',(-19.9559494024703,14.4196138695008,
131.169443863645)) ;
#121349=CARTESIAN_POINT('Ctrl Pts',(-19.8824068556425,14.3368368148889,
130.921412444081)) ;
#121350=CARTESIAN_POINT('Ctrl Pts',(-19.8192971637931,14.1892310626699,
130.704037107648)) ;
#121351=CARTESIAN_POINT('Ctrl Pts',(-19.7712007701594,13.9859052749166,
130.53033092249)) ;
#121352=CARTESIAN_POINT('Ctrl Pts',(-19.7427697939353,13.7426111503383,
130.414154891542)) ;
#121353=CARTESIAN_POINT('Ctrl Pts',(-19.7366417092746,13.4761437933061,
130.363088987223)) ;
#121354=CARTESIAN_POINT('Ctrl Pts',(-19.7538516960635,13.207093106288,130.38035702043)) ;
#121355=CARTESIAN_POINT('Ctrl Pts',(-19.7941146155968,12.9521503447167,
130.464788413262)) ;
#121356=CARTESIAN_POINT('Ctrl Pts',(-19.8550256367924,12.7315094010331,
130.609635495912)) ;
#121357=CARTESIAN_POINT('Ctrl Pts',(-19.9336999560045,12.5595225483876,
130.806132413325)) ;
#121358=CARTESIAN_POINT('Ctrl Pts',(-20.0235052591104,12.4509681320899,
131.035586591273)) ;
#121359=CARTESIAN_POINT('Ctrl Pts',(-20.1210367820071,12.4111337662686,
131.287163832228)) ;
#121360=CARTESIAN_POINT('Ctrl Pts',(-20.2175551658632,12.4436883981266,
131.536249097719)) ;
#121361=CARTESIAN_POINT('Ctrl Pts',(-20.3095832198193,12.5474867377232,
131.771686083341)) ;
#121362=CARTESIAN_POINT('Ctrl Pts',(-20.3885938102402,12.7123018064528,
131.969591631901)) ;
#121363=CARTESIAN_POINT('Ctrl Pts',(-20.4517259907487,12.9300708063277,
132.120711783805)) ;
#121364=CARTESIAN_POINT('Ctrl Pts',(-20.4937380782586,13.1802337565337,
132.21056605483)) ;
#121365=CARTESIAN_POINT('Ctrl Pts',(-20.5134506438464,13.4510759335073,
132.234831539263)) ;
#121366=CARTESIAN_POINT('Ctrl Pts',(-20.5094352277015,13.7180593172982,
132.190025271022)) ;
#121367=CARTESIAN_POINT('Ctrl Pts',(-20.4830290210652,13.9642786305136,
132.079760168839)) ;
#121368=CARTESIAN_POINT('Ctrl Pts',(-20.43689278128,14.1712561910319,131.911939492134)) ;
#121369=CARTESIAN_POINT('Ctrl Pts',(-20.3749029793823,14.3253725381315,
131.697731780804)) ;
#121370=CARTESIAN_POINT('Ctrl Pts',(-20.3018341343474,14.4148742721194,
131.450984618379)) ;
#121371=CARTESIAN_POINT('Ctrl Pts',(-20.2249302855789,14.4329087862449,
131.193411182104)) ;
#121372=CARTESIAN_POINT('Ctrl Pts',(-20.1488881094776,14.3788838227845,
130.938050037987)) ;
#121373=CARTESIAN_POINT('Ctrl Pts',(-20.080797339942,14.2561019527568,130.706001182306)) ;
#121374=CARTESIAN_POINT('Ctrl Pts',(-20.0261332992237,14.0742377640131,
130.513250821122)) ;
#121375=CARTESIAN_POINT('Ctrl Pts',(-19.9893332364788,13.8451949445008,
130.372595598783)) ;
#121376=CARTESIAN_POINT('Ctrl Pts',(-19.973868386846,13.58674350493,130.294374437478)) ;
#121377=CARTESIAN_POINT('Ctrl Pts',(-19.9816774413976,13.3144404098801,
130.283872434014)) ;
#121378=CARTESIAN_POINT('Ctrl Pts',(-20.0126413058548,13.0528695222705,
130.341385113357)) ;
#121379=CARTESIAN_POINT('Ctrl Pts',(-20.065511341227,12.8160517966369,130.4626835875)) ;
#121380=CARTESIAN_POINT('Ctrl Pts',(-20.1374567371324,12.6226065253332,
130.639635517755)) ;
#121381=CARTESIAN_POINT('Ctrl Pts',(-20.2233273344394,12.4871996902566,
130.857443179732)) ;
#121382=CARTESIAN_POINT('Ctrl Pts',(-20.318859154293,12.4184347650075,131.103214513939)) ;
#121383=CARTESIAN_POINT('Ctrl Pts',(-20.4160586900493,12.4219001268695,
131.354266248446)) ;
#121384=CARTESIAN_POINT('Ctrl Pts',(-20.5107057575997,12.4968774725135,
131.597561711737)) ;
#121385=CARTESIAN_POINT('Ctrl Pts',(-20.5956132149196,12.6381726387492,
131.812503913232)) ;
#121386=CARTESIAN_POINT('Ctrl Pts',(-20.6659104312661,12.8360677562161,
131.984677720499)) ;
#121387=CARTESIAN_POINT('Ctrl Pts',(-20.7169616994697,13.0762566249802,
132.100631255503)) ;
#121388=CARTESIAN_POINT('Ctrl Pts',(-20.7458024931045,13.3398740968699,
132.151878255805)) ;
#121389=CARTESIAN_POINT('Ctrl Pts',(-20.7514496276872,13.6103044053491,
132.135261699282)) ;
#121390=CARTESIAN_POINT('Ctrl Pts',(-20.7338894981992,13.86812497933,132.050741922307)) ;
#121391=CARTESIAN_POINT('Ctrl Pts',(-20.6952759855552,14.0932871473164,
131.904822536434)) ;
#121392=CARTESIAN_POINT('Ctrl Pts',(-20.6388857078219,14.2707836651958,
131.706880360139)) ;
#121393=CARTESIAN_POINT('Ctrl Pts',(-20.5701123801385,14.3866738498425,
131.472993198284)) ;
#121394=CARTESIAN_POINT('Ctrl Pts',(-20.4938977661901,14.4343395644747,
131.21722235527)) ;
#121395=CARTESIAN_POINT('Ctrl Pts',(-20.4166445517324,14.4093417118186,
130.958399478142)) ;
#121396=CARTESIAN_POINT('Ctrl Pts',(-20.344750708675,14.3139583253282,130.715285151649)) ;
#121397=CARTESIAN_POINT('Ctrl Pts',(-20.283791621845,14.1538396084722,130.503960542603)) ;
#121398=CARTESIAN_POINT('Ctrl Pts',(-20.2394788321261,13.9434082094923,
130.341592089435)) ;
#121399=CARTESIAN_POINT('Ctrl Pts',(-20.2148885604201,13.6926166180059,
130.236385900469)) ;
#121400=CARTESIAN_POINT('Ctrl Pts',(-20.2132281702384,13.4252309557657,
130.198542928982)) ;
#121401=CARTESIAN_POINT('Ctrl Pts',(-20.2348670323948,13.15699249017,130.228662293908)) ;
#121402=CARTESIAN_POINT('Ctrl Pts',(-20.2792098941449,12.9074157483193,
130.325066626541)) ;
#121403=CARTESIAN_POINT('Ctrl Pts',(-20.3439168468294,12.6946405590363,
130.480906726514)) ;
#121404=CARTESIAN_POINT('Ctrl Pts',(-20.4244393498658,12.5348309265639,
130.683142054182)) ;
#121405=CARTESIAN_POINT('Ctrl Pts',(-20.5170520572993,12.4376124646164,
130.920376912197)) ;
#121406=CARTESIAN_POINT('Ctrl Pts',(-20.614232235177,12.411847051691,131.17124526899)) ;
#121407=CARTESIAN_POINT('Ctrl Pts',(-20.7107805897904,12.4580456629596,
131.420177217248)) ;
#121408=CARTESIAN_POINT('Ctrl Pts',(-20.8003281359883,12.5736491425348,
131.648625222613)) ;
#121409=CARTESIAN_POINT('Ctrl Pts',(-20.8769776512577,12.7495592043743,
131.839473480739)) ;
#121410=CARTESIAN_POINT('Ctrl Pts',(-20.9364697192037,12.9753684252062,
131.979963656201)) ;
#121411=CARTESIAN_POINT('Ctrl Pts',(-20.9744395485556,13.2312290478431,
132.057879143097)) ;
#121412=CARTESIAN_POINT('Ctrl Pts',(-20.9895716582003,13.5022492390578,
132.068885248279)) ;
#121413=CARTESIAN_POINT('Ctrl Pts',(-20.9812409962063,13.766376795235,132.011509443639)) ;
#121414=CARTESIAN_POINT('Ctrl Pts',(-20.9509284133775,14.0063277413084,
131.889875566884)) ;
#121415=CARTESIAN_POINT('Ctrl Pts',(-20.901397437773,14.2048736878869,131.712059721878)) ;
#121416=CARTESIAN_POINT('Ctrl Pts',(-20.8367333930258,14.3476912358554,
131.489937969168)) ;
#121417=CARTESIAN_POINT('Ctrl Pts',(-20.7626675459821,14.4237776456092,
131.240443597558)) ;
#121418=CARTESIAN_POINT('Ctrl Pts',(-20.6850444981711,14.4280807671714,
130.980533757575)) ;
#121419=CARTESIAN_POINT('Ctrl Pts',(-20.6104629916729,14.3608278404858,
130.729644462962)) ;
#121420=CARTESIAN_POINT('Ctrl Pts',(-20.5442923362831,14.2256360028295,
130.503103888384)) ;
#121421=CARTESIAN_POINT('Ctrl Pts',(-20.4928914107022,14.0344799528452,
130.320003827834)) ;
#121422=CARTESIAN_POINT('Ctrl Pts',(-20.4597855514147,13.7980435581084,
130.190076931057)) ;
#121423=CARTESIAN_POINT('Ctrl Pts',(-20.4486586873055,13.5353241773225,
130.124460154582)) ;
#121424=CARTESIAN_POINT('Ctrl Pts',(-20.4608336123062,13.2644873700543,
130.126896090482)) ;
#121425=CARTESIAN_POINT('Ctrl Pts',(-20.4962021630104,13.0050528435928,
130.197094463303)) ;
#121426=CARTESIAN_POINT('Ctrl Pts',(-20.5529963678547,12.7754380039954,
130.329861771733)) ;
#121427=CARTESIAN_POINT('Ctrl Pts',(-20.6277229494288,12.592596001974,130.515070189189)) ;
#121428=CARTESIAN_POINT('Ctrl Pts',(-20.7157538716564,12.4690081971512,
130.7391650434)) ;
#121429=CARTESIAN_POINT('Ctrl Pts',(-20.81215529802,12.4135709103977,130.987527049635)) ;
#121430=CARTESIAN_POINT('Ctrl Pts',(-20.9094861728303,12.4306395059357,
131.238858431699)) ;
#121431=CARTESIAN_POINT('Ctrl Pts',(-21.0026514401505,12.5185475341995,
131.477882625203)) ;
#121432=CARTESIAN_POINT('Ctrl Pts',(-21.0853714580596,12.671844049154,131.686334990309)) ;
#121433=CARTESIAN_POINT('Ctrl Pts',(-21.1520901264361,12.8780302029366,
131.848192197388)) ;
#121434=CARTESIAN_POINT('Ctrl Pts',(-21.1993556490934,13.1252486430467,
131.952950580138)) ;
#121435=CARTESIAN_POINT('Ctrl Pts',(-21.2237824667136,13.3909665765868,
131.991371817502)) ;
#121436=CARTESIAN_POINT('Ctrl Pts',(-21.2249631077916,13.6612161076759,
131.961593524817)) ;
#121437=CARTESIAN_POINT('Ctrl Pts',(-21.2032821738675,13.9131568870817,
131.865195643412)) ;
#121438=CARTESIAN_POINT('Ctrl Pts',(-21.1610721766892,14.130438408173,131.708765378038)) ;
#121439=CARTESIAN_POINT('Ctrl Pts',(-21.1021911877447,14.2969775109189,
131.503691498968)) ;
#121440=CARTESIAN_POINT('Ctrl Pts',(-21.0308822540389,14.4015522166871,
131.262045908857)) ;
#121441=CARTESIAN_POINT('Ctrl Pts',(-20.9542773305936,14.4350500551864,
131.005268144371)) ;
#121442=CARTESIAN_POINT('Ctrl Pts',(-20.8777360660368,14.3967519658026,
130.748608972346)) ;
#121443=CARTESIAN_POINT('Ctrl Pts',(-20.8074043524251,14.2884849185217,
130.510002599054)) ;
#121444=CARTESIAN_POINT('Ctrl Pts',(-20.749265929619,14.1181740873397,130.307021314052)) ;
#121445=CARTESIAN_POINT('Ctrl Pts',(-20.7082309862435,13.8977533327247,
130.153974766705)) ;
#121446=CARTESIAN_POINT('Ctrl Pts',(-20.6879881266858,13.6446684520944,
130.061839853042)) ;
#121447=CARTESIAN_POINT('Ctrl Pts',(-20.6906077186671,13.3734340111263,
130.036200343841)) ;
#121448=CARTESIAN_POINT('Ctrl Pts',(-20.7167921465083,13.1072276556743,
130.079582037118)) ;
#121449=CARTESIAN_POINT('Ctrl Pts',(-20.7650399369603,12.8641925362022,
130.187502545825)) ;
#121450=CARTESIAN_POINT('Ctrl Pts',(-20.832963238355,12.6605227447286,130.352811316655)) ;
#121451=CARTESIAN_POINT('Ctrl Pts',(-20.9161790737425,12.511411732543,130.562837268873)) ;
#121452=CARTESIAN_POINT('Ctrl Pts',(-21.0104101058601,12.4272142071662,
130.804757170397)) ;
#121453=CARTESIAN_POINT('Ctrl Pts',(-21.1076357922236,12.415034803424,131.055849599217)) ;
#121454=CARTESIAN_POINT('Ctrl Pts',(-21.2035132942098,12.474749132082,131.302750086604)) ;
#121455=CARTESIAN_POINT('Ctrl Pts',(-21.2909871122389,12.6023246098268,
131.525185960272)) ;
#121456=CARTESIAN_POINT('Ctrl Pts',(-21.3650611723006,12.7898414639342,
131.708292226991)) ;
#121457=CARTESIAN_POINT('Ctrl Pts',(-21.4202075769088,13.0206707820948,
131.836437001356)) ;
#121458=CARTESIAN_POINT('Ctrl Pts',(-21.4542272676677,13.2818518807112,
131.902629387126)) ;
#121459=CARTESIAN_POINT('Ctrl Pts',(-21.4648599024733,13.552127865025,131.900639172206)) ;
#121460=CARTESIAN_POINT('Ctrl Pts',(-21.4523288216463,13.8139569141608,
131.830891201632)) ;
#121461=CARTESIAN_POINT('Ctrl Pts',(-21.4178069877882,14.0485699408796,
131.696750338238)) ;
#121462=CARTESIAN_POINT('Ctrl Pts',(-21.3654129791233,14.2361101899088,
131.510797708734)) ;
#121463=CARTESIAN_POINT('Ctrl Pts',(-21.2983585521537,14.3675384217247,
131.281604089224)) ;
#121464=CARTESIAN_POINT('Ctrl Pts',(-21.2231826385857,14.4300942313948,
131.028889010739)) ;
#121465=CARTESIAN_POINT('Ctrl Pts',(-21.1459130475057,14.420886512356,130.770144409633)) ;
#121466=CARTESIAN_POINT('Ctrl Pts',(-21.0723793346089,14.3405660853883,
130.522250778554)) ;
#121467=CARTESIAN_POINT('Ctrl Pts',(-21.0083875990447,14.1934622330658,
130.302023410579)) ;
#121468=CARTESIAN_POINT('Ctrl Pts',(-20.9600343878473,13.9917021731483,
130.127656755271)) ;
#121469=CARTESIAN_POINT('Ctrl Pts',(-20.9311102303853,13.7502056369867,
130.010153543516)) ;
#121470=CARTESIAN_POINT('Ctrl Pts',(-20.9242456069076,13.4844947151479,
129.956978964617)) ;
#121471=CARTESIAN_POINT('Ctrl Pts',(-20.9408737681755,13.2141840714607,
129.972407443897)) ;
#121472=CARTESIAN_POINT('Ctrl Pts',(-20.9804309573197,12.958922795002,130.054838696586)) ;
#121473=CARTESIAN_POINT('Ctrl Pts',(-21.0412242853496,12.7362702687102,
130.199165296148)) ;
#121474=CARTESIAN_POINT('Ctrl Pts',(-21.1183210212108,12.5648474915298,
130.391527393433)) ;
#121475=CARTESIAN_POINT('Ctrl Pts',(-21.2088711021638,12.452872631945,130.622756430255)) ;
#121476=CARTESIAN_POINT('Ctrl Pts',(-21.305434804131,12.41129419742,130.87181816482)) ;
#121477=CARTESIAN_POINT('Ctrl Pts',(-21.4029320135723,12.4419882083232,
131.123442256635)) ;
#121478=CARTESIAN_POINT('Ctrl Pts',(-21.494257982038,12.5427027848013,131.357191590523)) ;
#121479=CARTESIAN_POINT('Ctrl Pts',(-21.57433818966,12.7067963976432,131.557963432826)) ;
#121480=CARTESIAN_POINT('Ctrl Pts',(-21.637741419676,12.9221001541686,131.710056772353)) ;
#121481=CARTESIAN_POINT('Ctrl Pts',(-21.6808145966047,13.1741319902504,
131.802654834912)) ;
#121482=CARTESIAN_POINT('Ctrl Pts',(-21.7009520245888,13.4427023362762,
131.828426315282)) ;
#121483=CARTESIAN_POINT('Ctrl Pts',(-21.6976514844297,13.7107857212086,
131.78560637095)) ;
#121484=CARTESIAN_POINT('Ctrl Pts',(-21.6719724150692,13.956888330194,131.677603451996)) ;
#121485=CARTESIAN_POINT('Ctrl Pts',(-21.6262697094113,14.1661036929037,
131.51093449669)) ;
#121486=CARTESIAN_POINT('Ctrl Pts',(-21.5645026106687,14.3219385193613,
131.297320065824)) ;
#121487=CARTESIAN_POINT('Ctrl Pts',(-21.4921557412151,14.4130180852625,
131.052898813796)) ;
#121488=CARTESIAN_POINT('Ctrl Pts',(-21.4147863917618,14.4335349336769,
130.793743869836)) ;
#121489=CARTESIAN_POINT('Ctrl Pts',(-21.3385730740908,14.3810414218173,
130.537852192733)) ;
#121490=CARTESIAN_POINT('Ctrl Pts',(-21.2705346380607,14.2609490828525,
130.306144265951)) ;
#121491=CARTESIAN_POINT('Ctrl Pts',(-21.2151219074894,14.079534400134,130.111008834385)) ;
#121492=CARTESIAN_POINT('Ctrl Pts',(-21.177937738515,13.8529283959852,129.96942799476)) ;
#121493=CARTESIAN_POINT('Ctrl Pts',(-21.1617508066486,13.5926907244754,
129.888787697885)) ;
#121494=CARTESIAN_POINT('Ctrl Pts',(-21.1688878360298,13.3230678017147,
129.87665122898)) ;
#121495=CARTESIAN_POINT('Ctrl Pts',(-21.1992585105796,13.0595444653147,
129.9322501518)) ;
#121496=CARTESIAN_POINT('Ctrl Pts',(-21.251765609534,12.8214089114898,130.052423624605)) ;
#121497=CARTESIAN_POINT('Ctrl Pts',(-21.3231412688293,12.6270967453298,
130.227778003325)) ;
#121498=CARTESIAN_POINT('Ctrl Pts',(-21.4083872685259,12.4904301737517,
130.443872721006)) ;
#121499=CARTESIAN_POINT('Ctrl Pts',(-21.5034218070146,12.41952640959,130.688294257978)) ;
#121500=CARTESIAN_POINT('Ctrl Pts',(-21.6011087851476,12.4206998048116,
130.940608218909)) ;
#121501=CARTESIAN_POINT('Ctrl Pts',(-21.696063140712,12.4940151693159,131.18475236496)) ;
#121502=CARTESIAN_POINT('Ctrl Pts',(-21.7810646279155,12.6331734793058,
131.400063934903)) ;
#121503=CARTESIAN_POINT('Ctrl Pts',(-21.8518067818107,12.8293256852298,
131.573571896818)) ;
#121504=CARTESIAN_POINT('Ctrl Pts',(-21.9034926777369,13.0683012939604,
131.691398405443)) ;
#121505=CARTESIAN_POINT('Ctrl Pts',(-21.9331090686563,13.3322967725392,
131.74480552703)) ;
#121506=CARTESIAN_POINT('Ctrl Pts',(-21.9393783070901,13.6026350043085,
131.730028295471)) ;
#121507=CARTESIAN_POINT('Ctrl Pts',(-21.9225550826518,13.8605088968992,
131.647745173543)) ;
#121508=CARTESIAN_POINT('Ctrl Pts',(-21.8844777064328,14.0871784640944,
131.503344143957)) ;
#121509=CARTESIAN_POINT('Ctrl Pts',(-21.8287676502295,14.265834440122,131.307501478219)) ;
#121510=CARTESIAN_POINT('Ctrl Pts',(-21.760017708765,14.3843789684771,131.073534055057)) ;
#121511=CARTESIAN_POINT('Ctrl Pts',(-21.6837666999361,14.4339734265458,
130.817596552073)) ;
#121512=CARTESIAN_POINT('Ctrl Pts',(-21.6066788030557,14.4110559210102,
130.559350636955)) ;
#121513=CARTESIAN_POINT('Ctrl Pts',(-21.5346094087633,14.3178924901581,
130.315757506672)) ;
#121514=CARTESIAN_POINT('Ctrl Pts',(-21.4731242757902,14.1593686470185,
130.102848783246)) ;
#121515=CARTESIAN_POINT('Ctrl Pts',(-21.4282515814187,13.9496805218115,
129.938774151377)) ;
#121516=CARTESIAN_POINT('Ctrl Pts',(-21.4031364018714,13.7013469938743,
129.832244367826)) ;
#121517=CARTESIAN_POINT('Ctrl Pts',(-21.4007180388891,13.4330164717232,
129.792025041528)) ;
#121518=CARTESIAN_POINT('Ctrl Pts',(-21.4216646330142,13.1647607715786,
129.820160982068)) ;
#121519=CARTESIAN_POINT('Ctrl Pts',(-21.4655479362394,12.9137312008662,
129.915122311114)) ;
#121520=CARTESIAN_POINT('Ctrl Pts',(-21.529321250798,12.7007529783777,130.068427667511)) ;
#121521=CARTESIAN_POINT('Ctrl Pts',(-21.6099312650928,12.5383275920807,
130.270711053567)) ;
#121522=CARTESIAN_POINT('Ctrl Pts',(-21.7015227704485,12.4398166111486,
130.505243913684)) ;
#121523=CARTESIAN_POINT('Ctrl Pts',(-21.7994399744814,12.4114725010168,
130.757982304775)) ;
#121524=CARTESIAN_POINT('Ctrl Pts',(-21.8958871845684,12.4557968950616,
131.006694284982)) ;
#121525=CARTESIAN_POINT('Ctrl Pts',(-21.9858132022225,12.569629101587,131.236208930516)) ;
#121526=CARTESIAN_POINT('Ctrl Pts',(-22.0627069665889,12.7436129687706,
131.427847524928)) ;
#121527=CARTESIAN_POINT('Ctrl Pts',(-22.1228015587848,12.9681022843807,
131.570102893173)) ;
#121528=CARTESIAN_POINT('Ctrl Pts',(-22.1614820013196,13.2239471753799,
131.650012500945)) ;
#121529=CARTESIAN_POINT('Ctrl Pts',(-22.1772375533801,13.4941633310118,
131.662924277638)) ;
#121530=CARTESIAN_POINT('Ctrl Pts',(-22.1695983588983,13.7589186956337,
131.607544732681)) ;
#121531=CARTESIAN_POINT('Ctrl Pts',(-22.1398896393099,13.9998349614895,
131.487676911223)) ;
#121532=CARTESIAN_POINT('Ctrl Pts',(-22.0908619235723,14.1997646891006,
131.311332678912)) ;
#121533=CARTESIAN_POINT('Ctrl Pts',(-22.0266945737524,14.344263749604,131.090721536142)) ;
#121534=CARTESIAN_POINT('Ctrl Pts',(-21.952680793742,14.4224928496146,130.841310291008)) ;
#121535=CARTESIAN_POINT('Ctrl Pts',(-21.8754606570184,14.4291711030004,
130.58274926124)) ;
#121536=CARTESIAN_POINT('Ctrl Pts',(-21.8001571446588,14.3636108427049,
130.329504565342)) ;
#121537=CARTESIAN_POINT('Ctrl Pts',(-21.7338905583542,14.2305640728087,
130.102800547914)) ;
#121538=CARTESIAN_POINT('Ctrl Pts',(-21.6819125731549,14.0406274763076,
129.917954418755)) ;
#121539=CARTESIAN_POINT('Ctrl Pts',(-21.6482766927022,13.8058698761943,
129.786568126659)) ;
#121540=CARTESIAN_POINT('Ctrl Pts',(-21.6364270305114,13.5427807142404,
129.718722262125)) ;
#121541=CARTESIAN_POINT('Ctrl Pts',(-21.6479525293074,13.2720604281958,
129.719284180321)) ;
#121542=CARTESIAN_POINT('Ctrl Pts',(-21.6827354707971,13.0118428173477,
129.787740591491)) ;
#121543=CARTESIAN_POINT('Ctrl Pts',(-21.7387645363647,12.7818787427455,
129.918382531202)) ;
#121544=CARTESIAN_POINT('Ctrl Pts',(-21.8131751278323,12.5968716108038,
130.102584387991)) ;
#121545=CARTESIAN_POINT('Ctrl Pts',(-21.9012978983489,12.4712516936664,
130.326815834056)) ;
#121546=CARTESIAN_POINT('Ctrl Pts',(-21.9970924731431,12.4142247915804,
130.573571167119)) ;
#121547=CARTESIAN_POINT('Ctrl Pts',(-22.0946249674174,12.4291610555867,
130.825434404428)) ;
#121548=CARTESIAN_POINT('Ctrl Pts',(-22.1880538379132,12.5152749819563,
131.065210306025)) ;
#121549=CARTESIAN_POINT('Ctrl Pts',(-22.2712353524733,12.6672522728085,
131.274961582696)) ;
#121550=CARTESIAN_POINT('Ctrl Pts',(-22.3381448037188,12.8714563958125,
131.437501065827)) ;
#121551=CARTESIAN_POINT('Ctrl Pts',(-22.3859106141911,13.1164156857726,
131.543882892038)) ;
#121552=CARTESIAN_POINT('Ctrl Pts',(-22.4112282957359,13.3833143982509,
131.584711419103)) ;
#121553=CARTESIAN_POINT('Ctrl Pts',(-22.4130217695324,13.6536761836367,
131.55673452737)) ;
#121554=CARTESIAN_POINT('Ctrl Pts',(-22.3920167236971,13.9063303712051,
131.462322269529)) ;
#121555=CARTESIAN_POINT('Ctrl Pts',(-22.3501194078207,14.1256565234766,
131.306665041968)) ;
#121556=CARTESIAN_POINT('Ctrl Pts',(-22.2918172565239,14.2929703987116,
131.103406435929)) ;
#121557=CARTESIAN_POINT('Ctrl Pts',(-22.2209556831958,14.3994043098715,
130.863140859753)) ;
#121558=CARTESIAN_POINT('Ctrl Pts',(-22.1443006583547,14.4351253202518,
130.60615685561)) ;
#121559=CARTESIAN_POINT('Ctrl Pts',(-22.0676126713909,14.3988243976867,
130.349047099311)) ;
#121560=CARTESIAN_POINT('Ctrl Pts',(-21.9970015558164,14.2923293350233,
130.109611142122)) ;
#121561=CARTESIAN_POINT('Ctrl Pts',(-21.9386211582789,14.1241731198379,
129.906023714666)) ;
#121562=CARTESIAN_POINT('Ctrl Pts',(-21.8969564647824,13.9051613921294,
129.751139774253)) ;
#121563=CARTESIAN_POINT('Ctrl Pts',(-21.8760425466096,13.6518311296983,
129.656921029517)) ;
#121564=CARTESIAN_POINT('Ctrl Pts',(-21.8779576296647,13.382470855745,129.629430197668)) ;
#121565=CARTESIAN_POINT('Ctrl Pts',(-21.903356370173,13.1154253093326,129.670468190117)) ;
#121566=CARTESIAN_POINT('Ctrl Pts',(-21.9511796972224,12.870532627165,129.777021512631)) ;
#121567=CARTESIAN_POINT('Ctrl Pts',(-22.018597334857,12.6655370623813,129.940858603322)) ;
#121568=CARTESIAN_POINT('Ctrl Pts',(-22.1016149733205,12.5146112144562,
130.150247300748)) ;
#121569=CARTESIAN_POINT('Ctrl Pts',(-22.1950646404757,12.4289101805898,
130.390085189532)) ;
#121570=CARTESIAN_POINT('Ctrl Pts',(-22.2924700780955,12.414189675376,130.641628079446)) ;
#121571=CARTESIAN_POINT('Ctrl Pts',(-22.3890144251563,12.4724108843215,
130.890294126128)) ;
#121572=CARTESIAN_POINT('Ctrl Pts',(-22.4763336587939,12.5978142660017,
131.112435610646)) ;
#121573=CARTESIAN_POINT('Ctrl Pts',(-22.5506291996143,12.7826552616513,
131.296338429027)) ;
#121574=CARTESIAN_POINT('Ctrl Pts',(-22.6066949619686,13.0133815728599,
131.427008840756)) ;
#121575=CARTESIAN_POINT('Ctrl Pts',(-22.6413737989187,13.2742169731993,
131.495103126571)) ;
#121576=CARTESIAN_POINT('Ctrl Pts',(-22.652675011079,13.5450315924184,131.494998262817)) ;
#121577=CARTESIAN_POINT('Ctrl Pts',(-22.6407386602464,13.8067212996898,
131.427059832861)) ;
#121578=CARTESIAN_POINT('Ctrl Pts',(-22.6071088701475,14.041251387199,131.295715732246)) ;
#121579=CARTESIAN_POINT('Ctrl Pts',(-22.5548293120912,14.2318697837458,
131.109842788739)) ;
#121580=CARTESIAN_POINT('Ctrl Pts',(-22.4882219597125,14.3645253457052,
130.882041140552)) ;
#121581=CARTESIAN_POINT('Ctrl Pts',(-22.4135301561278,14.4291513856489,
130.630867987503)) ;
#121582=CARTESIAN_POINT('Ctrl Pts',(-22.3359383497484,14.4223448074479,
130.371059800614)) ;
#121583=CARTESIAN_POINT('Ctrl Pts',(-22.2619633520101,14.3433927947591,
130.121750920733)) ;
#121584=CARTESIAN_POINT('Ctrl Pts',(-22.1981313809753,14.1993296986607,
129.902268927259)) ;
#121585=CARTESIAN_POINT('Ctrl Pts',(-22.1490456223981,13.9988089965648,
129.725677746774)) ;
#121586=CARTESIAN_POINT('Ctrl Pts',(-22.1194205531409,13.7578101300497,
129.60606621788)) ;
#121587=CARTESIAN_POINT('Ctrl Pts',(-22.1119250099299,13.4916490682303,
129.550940820402)) ;
#121588=CARTESIAN_POINT('Ctrl Pts',(-22.1278069450151,13.2223242995655,
129.564332881806)) ;
#121589=CARTESIAN_POINT('Ctrl Pts',(-22.166820729976,12.9657468504133,129.645089069852)) ;
#121590=CARTESIAN_POINT('Ctrl Pts',(-22.2266899368361,12.7429296521264,
129.78689267835)) ;
#121591=CARTESIAN_POINT('Ctrl Pts',(-22.3038746479134,12.5685157086448,
129.979270003299)) ;
#121592=CARTESIAN_POINT('Ctrl Pts',(-22.3941718104836,12.4549912632195,
130.209772948028)) ;
#121593=CARTESIAN_POINT('Ctrl Pts',(-22.4904254232344,12.4115665136302,
130.457995293597)) ;
#121594=CARTESIAN_POINT('Ctrl Pts',(-22.5877870812419,12.4399153720153,
130.709299834689)) ;
#121595=CARTESIAN_POINT('Ctrl Pts',(-22.6798460130406,12.5392662733084,
130.945012346427)) ;
#121596=CARTESIAN_POINT('Ctrl Pts',(-22.7601047464817,12.7015765304021,
131.146380117816)) ;
#121597=CARTESIAN_POINT('Ctrl Pts',(-22.8238896240796,12.9151235302472,
131.299658737214)) ;
#121598=CARTESIAN_POINT('Ctrl Pts',(-22.8675764779866,13.1655123638567,
131.394148657853)) ;
#121599=CARTESIAN_POINT('Ctrl Pts',(-22.8885227240857,13.4357073085102,
131.42204915288)) ;
#121600=CARTESIAN_POINT('Ctrl Pts',(-22.8858619215617,13.7027427406616,
131.381268339562)) ;
#121601=CARTESIAN_POINT('Ctrl Pts',(-22.8607916607201,13.9504288317899,
131.274952297113)) ;
#121602=CARTESIAN_POINT('Ctrl Pts',(-22.815558311505,14.1608971109305,131.109650229729)) ;
#121603=CARTESIAN_POINT('Ctrl Pts',(-22.7543026730754,14.3182076735822,
130.897587615978)) ;
#121604=CARTESIAN_POINT('Ctrl Pts',(-22.6820714114506,14.4114239786406,
130.653451460202)) ;
#121605=CARTESIAN_POINT('Ctrl Pts',(-22.6049103118654,14.4338711414245,
130.394968464032)) ;
#121606=CARTESIAN_POINT('Ctrl Pts',(-22.5287473843446,14.3839736196214,
130.139317443058)) ;
#121607=CARTESIAN_POINT('Ctrl Pts',(-22.459971667544,14.2649033535115,129.905232477421)) ;
#121608=CARTESIAN_POINT('Ctrl Pts',(-22.4044402450173,14.0862372824977,
129.709967380025)) ;
#121609=CARTESIAN_POINT('Ctrl Pts',(-22.3664456626379,13.8593709017047,
129.565802970245)) ;
#121610=CARTESIAN_POINT('Ctrl Pts',(-22.3497272642463,13.6016401376878,
129.483857102706)) ;
#121611=CARTESIAN_POINT('Ctrl Pts',(-22.3560994962859,13.3309240386314,
129.469335731797)) ;
#121612=CARTESIAN_POINT('Ctrl Pts',(-22.3858506421703,13.0670232558749,
129.523137281469)) ;
#121613=CARTESIAN_POINT('Ctrl Pts',(-22.4375345414781,12.828626100883,129.641014989765)) ;
#121614=CARTESIAN_POINT('Ctrl Pts',(-22.5083363812964,12.6324568485675,
129.814684706642)) ;
#121615=CARTESIAN_POINT('Ctrl Pts',(-22.5937839707588,12.4932133187338,
130.031160714492)) ;
#121616=CARTESIAN_POINT('Ctrl Pts',(-22.6881953246157,12.4206918000049,
130.273922071333)) ;
#121617=CARTESIAN_POINT('Ctrl Pts',(-22.7861951971573,12.4196226873693,
130.527040965204)) ;
#121618=CARTESIAN_POINT('Ctrl Pts',(-22.8812583930361,12.491015534073,130.77152639582)) ;
#121619=CARTESIAN_POINT('Ctrl Pts',(-22.9666341838661,12.6283740411058,
130.987922473245)) ;
#121620=CARTESIAN_POINT('Ctrl Pts',(-23.0380241779246,12.8237070115403,
131.163235063303)) ;
#121621=CARTESIAN_POINT('Ctrl Pts',(-23.0901672903314,13.061674988434,131.282420600478)) ;
#121622=CARTESIAN_POINT('Ctrl Pts',(-23.1203227852946,13.32403831549,131.33754630017)) ;
#121623=CARTESIAN_POINT('Ctrl Pts',(-23.1273409911795,13.5952494532198,
131.324861458868)) ;
#121624=CARTESIAN_POINT('Ctrl Pts',(-23.1110257455182,13.8544595639362,
131.243964214945)) ;
#121625=CARTESIAN_POINT('Ctrl Pts',(-23.0735006754812,14.0816540138682,
131.101239043931)) ;
#121626=CARTESIAN_POINT('Ctrl Pts',(-23.0184218320253,14.2612880227879,
130.907347850486)) ;
#121627=CARTESIAN_POINT('Ctrl Pts',(-22.9500143562106,14.3817634541805,
130.674390989242)) ;
#121628=CARTESIAN_POINT('Ctrl Pts',(-22.8738736556778,14.4336477376616,
130.418767505991)) ;
#121629=CARTESIAN_POINT('Ctrl Pts',(-22.7962947688756,14.4124733819028,
130.158897256619)) ;
#121630=CARTESIAN_POINT('Ctrl Pts',(-22.7244222517359,14.3214777204803,
129.916058077239)) ;
#121631=CARTESIAN_POINT('Ctrl Pts',(-22.6625658163423,14.1652192318908,
129.702115717874)) ;
#121632=CARTESIAN_POINT('Ctrl Pts',(-22.616956336506,13.955565015999,129.535701263914)) ;
#121633=CARTESIAN_POINT('Ctrl Pts',(-22.5914008763533,13.709559951643,129.428089151197)) ;
#121634=CARTESIAN_POINT('Ctrl Pts',(-22.5882016234741,13.4405995053874,
129.385467312093)) ;
#121635=CARTESIAN_POINT('Ctrl Pts',(-22.6086689737768,13.1715077449996,
129.412122430663)) ;
#121636=CARTESIAN_POINT('Ctrl Pts',(-22.6515386816599,12.9214880577471,
129.504375180884)) ;
#121637=CARTESIAN_POINT('Ctrl Pts',(-22.7152706299767,12.7055052948916,
129.657291190798)) ;
#121638=CARTESIAN_POINT('Ctrl Pts',(-22.7950426841781,12.5425196624815,
129.857326438602)) ;
#121639=CARTESIAN_POINT('Ctrl Pts',(-22.8865698066011,12.4416160232308,
130.091588674576)) ;
#121640=CARTESIAN_POINT('Ctrl Pts',(-22.984492058789,12.4112449643292,130.344321485387)) ;
#121641=CARTESIAN_POINT('Ctrl Pts',(-23.0811185429017,12.4537097251659,
130.593526328685)) ;
#121642=CARTESIAN_POINT('Ctrl Pts',(-23.1710261323751,12.5652232898652,
130.823102119305)) ;
#121643=CARTESIAN_POINT('Ctrl Pts',(-23.2485247769713,12.7379440423451,
131.01643444413)) ;
#121644=CARTESIAN_POINT('Ctrl Pts',(-23.3089752450533,12.9603974854775,
131.159852173904)) ;
#121645=CARTESIAN_POINT('Ctrl Pts',(-23.348408153789,13.2156635264027,131.241930685278)) ;
#121646=CARTESIAN_POINT('Ctrl Pts',(-23.3649083403446,13.4857934304202,
131.257011973087)) ;
#121647=CARTESIAN_POINT('Ctrl Pts',(-23.357909971757,13.7522947042676,131.203342265099)) ;
#121648=CARTESIAN_POINT('Ctrl Pts',(-23.328617454617,13.9943545056691,131.084632132187)) ;
#121649=CARTESIAN_POINT('Ctrl Pts',(-23.2803059324415,14.1947046686213,
130.910538675676)) ;
#121650=CARTESIAN_POINT('Ctrl Pts',(-23.2162094085204,14.341452975733,130.689990853063)) ;
#121651=CARTESIAN_POINT('Ctrl Pts',(-23.142748044954,14.4211243225131,130.442364505768)) ;
#121652=CARTESIAN_POINT('Ctrl Pts',(-23.0653904655543,14.4300014254347,
130.183330074937)) ;
#121653=CARTESIAN_POINT('Ctrl Pts',(-22.9900701305937,14.3664765373256,
129.930097446145)) ;
#121654=CARTESIAN_POINT('Ctrl Pts',(-22.923513785988,14.2356051810154,129.702583954865)) ;
#121655=CARTESIAN_POINT('Ctrl Pts',(-22.8708357577981,14.0463420011333,
129.515552886833)) ;
#121656=CARTESIAN_POINT('Ctrl Pts',(-22.8367444403438,13.8127311118514,
129.382871206129)) ;
#121657=CARTESIAN_POINT('Ctrl Pts',(-22.8242308008636,13.5514860506215,
129.313245492721)) ;
#121658=CARTESIAN_POINT('Ctrl Pts',(-22.8350769331615,13.2797430818136,
129.311697539403)) ;
#121659=CARTESIAN_POINT('Ctrl Pts',(-22.869098225033,13.0196140734991,129.378020218601)) ;
#121660=CARTESIAN_POINT('Ctrl Pts',(-22.9247143370731,12.7876901355889,
129.507337456949)) ;
#121661=CARTESIAN_POINT('Ctrl Pts',(-22.9985974383203,12.6015317076786,
129.69004468155)) ;
#121662=CARTESIAN_POINT('Ctrl Pts',(-23.086121475707,12.474259722316,129.912620832564)) ;
#121663=CARTESIAN_POINT('Ctrl Pts',(-23.1818805907226,12.41484596922,130.159228255654)) ;
#121664=CARTESIAN_POINT('Ctrl Pts',(-23.2797131219869,12.4277168198839,
130.411880974866)) ;
#121665=CARTESIAN_POINT('Ctrl Pts',(-23.3732545642975,12.511951186466,130.652010946363)) ;
#121666=CARTESIAN_POINT('Ctrl Pts',(-23.4565110007243,12.6612551341691,
130.862127850995)) ;
#121667=CARTESIAN_POINT('Ctrl Pts',(-23.5244261393507,12.8654798246469,
131.027369978243)) ;
#121668=CARTESIAN_POINT('Ctrl Pts',(-23.5725829742774,13.1088716253824,
131.135002247458)) ;
#121669=CARTESIAN_POINT('Ctrl Pts',(-23.5986019731753,13.3752799217244,
131.177886352702)) ;
#121670=CARTESIAN_POINT('Ctrl Pts',(-23.6011015071733,13.6458120251598,
131.151980086065)) ;
#121671=CARTESIAN_POINT('Ctrl Pts',(-23.5806843251492,13.8994658312756,
131.059242348324)) ;
#121672=CARTESIAN_POINT('Ctrl Pts',(-23.5395648399883,14.1192749080617,
130.905996408547)) ;
#121673=CARTESIAN_POINT('Ctrl Pts',(-23.4813848765133,14.2891803120814,
130.702911334462)) ;
#121674=CARTESIAN_POINT('Ctrl Pts',(-23.4111139306529,14.3970324954729,
130.464529997136)) ;
#121675=CARTESIAN_POINT('Ctrl Pts',(-23.3344012694939,14.4351164738745,
130.207301293697)) ;
#121676=CARTESIAN_POINT('Ctrl Pts',(-23.2576890516809,14.4010787693592,
129.950158636102)) ;
#121677=CARTESIAN_POINT('Ctrl Pts',(-23.1864140310954,14.2958209261601,
129.708587842653)) ;
#121678=CARTESIAN_POINT('Ctrl Pts',(-23.1278795559311,14.1296521769512,
129.504668064509)) ;
#121679=CARTESIAN_POINT('Ctrl Pts',(-23.0856754302554,13.9121761365587,
129.348238913807)) ;
#121680=CARTESIAN_POINT('Ctrl Pts',(-23.0641329052405,13.6594303450515,
129.252162708667)) ;
#121681=CARTESIAN_POINT('Ctrl Pts',(-23.0653052820305,13.3906473022496,
129.222550978665)) ;
#121682=CARTESIAN_POINT('Ctrl Pts',(-23.090283304595,13.1215485534994,129.26213901249)) ;
#121683=CARTESIAN_POINT('Ctrl Pts',(-23.1372175806603,12.8774994745799,
129.366325807078)) ;
#121684=CARTESIAN_POINT('Ctrl Pts',(-23.204393997006,12.6702279287505,129.52931153654)) ;
#121685=CARTESIAN_POINT('Ctrl Pts',(-23.2867150726529,12.5183910310168,
129.736808163785)) ;
#121686=CARTESIAN_POINT('Ctrl Pts',(-23.3799501396602,12.4302683036152,
129.976005708702)) ;
#121687=CARTESIAN_POINT('Ctrl Pts',(-23.4780194336623,12.4138255898749,
130.229248949606)) ;
#121688=CARTESIAN_POINT('Ctrl Pts',(-23.5734967171244,12.4692849906945,
130.475218068993)) ;
#121689=CARTESIAN_POINT('Ctrl Pts',(-23.6617647155434,12.593086865603,130.699920489542)) ;
#121690=CARTESIAN_POINT('Ctrl Pts',(-23.7366528628754,12.7771359957172,
130.88546921267)) ;
#121691=CARTESIAN_POINT('Ctrl Pts',(-23.7930824889268,13.0059650352549,
131.017318083727)) ;
#121692=CARTESIAN_POINT('Ctrl Pts',(-23.8284573242334,13.2661472489738,
131.087445926367)) ;
#121693=CARTESIAN_POINT('Ctrl Pts',(-23.8404774545327,13.5369907136561,
131.089436183749)) ;
#121694=CARTESIAN_POINT('Ctrl Pts',(-23.829155718935,13.7997449792612,131.023219419023)) ;
#121695=CARTESIAN_POINT('Ctrl Pts',(-23.7961622175003,14.0350784316614,
130.893776777003)) ;
#121696=CARTESIAN_POINT('Ctrl Pts',(-23.7440972612148,14.2276701569779,
130.708399650426)) ;
#121697=CARTESIAN_POINT('Ctrl Pts',(-23.6784579579534,14.3610391391533,
130.483737931397)) ;
#121698=CARTESIAN_POINT('Ctrl Pts',(-23.6033254135512,14.4285213682471,
130.230995383092)) ;
#121699=CARTESIAN_POINT('Ctrl Pts',(-23.5258829163053,14.4233691347863,
129.971694462302)) ;
#121700=CARTESIAN_POINT('Ctrl Pts',(-23.4519103008065,14.3469900200021,
129.722496786167)) ;
#121701=CARTESIAN_POINT('Ctrl Pts',(-23.3872758527117,14.2034039230656,
129.50041476823)) ;
#121702=CARTESIAN_POINT('Ctrl Pts',(-23.3380843805541,14.0056847317555,
129.323768358841)) ;
#121703=CARTESIAN_POINT('Ctrl Pts',(-23.3077174301833,13.7644934618712,
129.201819431847)) ;
#121704=CARTESIAN_POINT('Ctrl Pts',(-23.2995656105439,13.5002463021735,
129.144972753961)) ;
#121705=CARTESIAN_POINT('Ctrl Pts',(-23.31497764899,13.2284057614088,129.156686870194)) ;
#121706=CARTESIAN_POINT('Ctrl Pts',(-23.3529809802264,12.9739037003026,
129.234851116751)) ;
#121707=CARTESIAN_POINT('Ctrl Pts',(-23.4125409802653,12.7484703827135,
129.375556014686)) ;
#121708=CARTESIAN_POINT('Ctrl Pts',(-23.489066219191,12.5731123065293,129.566119181298)) ;
#121709=CARTESIAN_POINT('Ctrl Pts',(-23.5791220316779,12.4573590720307,
129.795883585505)) ;
#121710=CARTESIAN_POINT('Ctrl Pts',(-23.6753629969101,12.4118025437708,
130.044038138499)) ;
#121711=CARTESIAN_POINT('Ctrl Pts',(-23.7728143173082,12.4381298316287,
130.295594078623)) ;
#121712=CARTESIAN_POINT('Ctrl Pts',(-23.8649582071419,12.5352056674708,
130.53162152315)) ;
#121713=CARTESIAN_POINT('Ctrl Pts',(-23.9458556331746,12.6963006126537,
130.734754487128)) ;
#121714=CARTESIAN_POINT('Ctrl Pts',(-24.0101297169403,12.9082756109017,
130.889506306032)) ;
#121715=CARTESIAN_POINT('Ctrl Pts',(-24.0545841543703,13.1596325292673,
130.986017902497)) ;
#121716=CARTESIAN_POINT('Ctrl Pts',(-24.0759302955051,13.4259468803236,
131.015538335644)) ;
#121717=CARTESIAN_POINT('Ctrl Pts',(-24.0740919955481,13.6953761001562,
130.976901663814)) ;
#121718=CARTESIAN_POINT('Ctrl Pts',(-24.0495884975813,13.943717027651,130.872263472699)) ;
#121719=CARTESIAN_POINT('Ctrl Pts',(-24.0048388868655,14.1557110892649,
130.7083358927)) ;
#121720=CARTESIAN_POINT('Ctrl Pts',(-23.9440791244033,14.3144000289701,
130.497783976676)) ;
#121721=CARTESIAN_POINT('Ctrl Pts',(-23.8721181136908,14.4096307928531,
130.254444307952)) ;
#121722=CARTESIAN_POINT('Ctrl Pts',(-23.7949917478579,14.4343455409311,
129.996055887983)) ;
#121723=CARTESIAN_POINT('Ctrl Pts',(-23.7183945611364,14.3860725213322,
129.738990412357)) ;
#121724=CARTESIAN_POINT('Ctrl Pts',(-23.6497155209254,14.269509697164,129.505378523881)) ;
#121725=CARTESIAN_POINT('Ctrl Pts',(-23.5935085503092,14.0917907400684,
129.308007286199)) ;
#121726=CARTESIAN_POINT('Ctrl Pts',(-23.5550865672651,13.8666926815631,
129.162696838379)) ;
#121727=CARTESIAN_POINT('Ctrl Pts',(-23.5376687883105,13.6093228235484,
129.078662798644)) ;
#121728=CARTESIAN_POINT('Ctrl Pts',(-23.5433650492229,13.3388431242067,
129.062185597359)) ;
#121729=CARTESIAN_POINT('Ctrl Pts',(-23.5724839615649,13.0740473551912,
129.114088332955)) ;
#121730=CARTESIAN_POINT('Ctrl Pts',(-23.6237334254588,12.834394570963,129.230640971734)) ;
#121731=CARTESIAN_POINT('Ctrl Pts',(-23.6936925175192,12.6378258855697,
129.402017995682)) ;
#121732=CARTESIAN_POINT('Ctrl Pts',(-23.7787793504876,12.4964629704439,
129.617422649139)) ;
#121733=CARTESIAN_POINT('Ctrl Pts',(-23.8732647499766,12.4217253903026,
129.860312611565)) ;
#121734=CARTESIAN_POINT('Ctrl Pts',(-23.9711567729886,12.4187226329277,
130.113148873488)) ;
#121735=CARTESIAN_POINT('Ctrl Pts',(-24.0660810815152,12.4875916931866,
130.357347207621)) ;
#121736=CARTESIAN_POINT('Ctrl Pts',(-24.1521509829385,12.6235712974209,
130.575641050135)) ;
#121737=CARTESIAN_POINT('Ctrl Pts',(-24.2237599658154,12.8167008380917,
130.751719197744)) ;
#121738=CARTESIAN_POINT('Ctrl Pts',(-24.2766320275245,13.053470182096,130.873029282451)) ;
#121739=CARTESIAN_POINT('Ctrl Pts',(-24.3076017852851,13.3166530721009,
130.930371105452)) ;
#121740=CARTESIAN_POINT('Ctrl Pts',(-24.3152190181606,13.5871782516177,
130.919526468752)) ;
#121741=CARTESIAN_POINT('Ctrl Pts',(-24.2997261236397,13.8461111103248,
130.841158630787)) ;
#121742=CARTESIAN_POINT('Ctrl Pts',(-24.2627363075861,14.0754123777246,
130.699882780774)) ;
#121743=CARTESIAN_POINT('Ctrl Pts',(-24.2079729206968,14.2569965796042,
130.506838743706)) ;
#121744=CARTESIAN_POINT('Ctrl Pts',(-24.1398686531416,14.3792169528627,
130.274773785101)) ;
#121745=CARTESIAN_POINT('Ctrl Pts',(-24.0640873934345,14.4330645797171,
130.020296166721)) ;
#121746=CARTESIAN_POINT('Ctrl Pts',(-23.9864701853882,14.4142942026361,
129.760321344143)) ;
#121747=CARTESIAN_POINT('Ctrl Pts',(-23.9140656407132,14.3249818434921,
129.515797144389)) ;
#121748=CARTESIAN_POINT('Ctrl Pts',(-23.8518321133868,14.1700409218133,
129.300722456645)) ;
#121749=CARTESIAN_POINT('Ctrl Pts',(-23.8059089034799,13.9629928676694,
129.133578126005)) ;
#121750=CARTESIAN_POINT('Ctrl Pts',(-23.7795827562579,13.7164972263621,
129.023526816175)) ;
#121751=CARTESIAN_POINT('Ctrl Pts',(-23.7757564515604,13.4493823729498,
128.97926513916)) ;
#121752=CARTESIAN_POINT('Ctrl Pts',(-23.7954419194189,13.1794660077169,
129.00356919432)) ;
#121753=CARTESIAN_POINT('Ctrl Pts',(-23.8379907278059,12.9274139547086,
129.094708724123)) ;
#121754=CARTESIAN_POINT('Ctrl Pts',(-23.9008430840631,12.7115777217288,
129.24525361468)) ;
#121755=CARTESIAN_POINT('Ctrl Pts',(-23.9801928783826,12.5463884356972,
129.444024662867)) ;
#121756=CARTESIAN_POINT('Ctrl Pts',(-24.0722443681962,12.443178693002,129.679554649046)) ;
#121757=CARTESIAN_POINT('Ctrl Pts',(-24.1690180676137,12.4112124572602,
129.92930163527)) ;
#121758=CARTESIAN_POINT('Ctrl Pts',(-24.2661327749485,12.4513454619086,
130.179802073149)) ;
#121759=CARTESIAN_POINT('Ctrl Pts',(-24.3562959525543,12.5610016946322,
130.410134143463)) ;
#121760=CARTESIAN_POINT('Ctrl Pts',(-24.4343250881083,12.732231543376,130.604978977865)) ;
#121761=CARTESIAN_POINT('Ctrl Pts',(-24.4953391322898,12.9536822141676,
130.750023050811)) ;
#121762=CARTESIAN_POINT('Ctrl Pts',(-24.5353305531141,13.2077095887355,
130.833800831059)) ;
#121763=CARTESIAN_POINT('Ctrl Pts',(-24.5525587376172,13.4778390375596,
130.850989350465)) ;
#121764=CARTESIAN_POINT('Ctrl Pts',(-24.5462019536801,13.7447250723396,
130.799190280117)) ;
#121765=CARTESIAN_POINT('Ctrl Pts',(-24.5176953064597,13.9871379837623,
130.682880665988)) ;
#121766=CARTESIAN_POINT('Ctrl Pts',(-24.4695538860457,14.1900737145365,
130.509067328973)) ;
#121767=CARTESIAN_POINT('Ctrl Pts',(-24.4064340261719,14.3373318040479,
130.291685786572)) ;
#121768=CARTESIAN_POINT('Ctrl Pts',(-24.3327321271544,14.419933546752,130.04313050484)) ;
#121769=CARTESIAN_POINT('Ctrl Pts',(-24.2554111115595,14.4307823852778,
129.784218809138)) ;
#121770=CARTESIAN_POINT('Ctrl Pts',(-24.1797499325286,14.3690285004678,
129.529899580821)) ;
#121771=CARTESIAN_POINT('Ctrl Pts',(-24.1131557614582,14.2404409367686,
129.302414068984)) ;
#121772=CARTESIAN_POINT('Ctrl Pts',(-24.0599615774343,14.0528075419849,
129.113868915362)) ;
#121773=CARTESIAN_POINT('Ctrl Pts',(-24.0252316135323,13.8202654365076,
128.979314882882)) ;
#121774=CARTESIAN_POINT('Ctrl Pts',(-24.0120333005036,13.5584443869878,
128.907549138537)) ;
#121775=CARTESIAN_POINT('Ctrl Pts',(-24.0222813639588,13.2871049531719,
128.904304542644)) ;
#121776=CARTESIAN_POINT('Ctrl Pts',(-24.0555382378822,13.0271135604128,
128.96848416764)) ;
#121777=CARTESIAN_POINT('Ctrl Pts',(-24.1106071061266,12.7938647144907,
129.096170233129)) ;
#121778=CARTESIAN_POINT('Ctrl Pts',(-24.1839223129408,12.6063347659711,
129.277257696409)) ;
#121779=CARTESIAN_POINT('Ctrl Pts',(-24.2712622814274,12.4770287601625,
129.499241059545)) ;
#121780=CARTESIAN_POINT('Ctrl Pts',(-24.366585154662,12.4155889088205,129.744672790457)) ;
#121781=CARTESIAN_POINT('Ctrl Pts',(-24.4648941553705,12.4264045930434,
129.998562059193)) ;
#121782=CARTESIAN_POINT('Ctrl Pts',(-24.5583069638422,12.5084013028489,
130.238438570714)) ;
#121783=CARTESIAN_POINT('Ctrl Pts',(-24.6421105256963,12.6562046151244,
130.450082237767)) ;
#121784=CARTESIAN_POINT('Ctrl Pts',(-24.7103360959245,12.8582528702238,
130.616348720843)) ;
#121785=CARTESIAN_POINT('Ctrl Pts',(-24.7594534193122,13.10224809555,130.726572672664)) ;
#121786=CARTESIAN_POINT('Ctrl Pts',(-24.7859819902892,13.3685511856617,
130.770923579385)) ;
#121787=CARTESIAN_POINT('Ctrl Pts',(-24.7891497215362,13.6374690862059,
130.747188210183)) ;
#121788=CARTESIAN_POINT('Ctrl Pts',(-24.7693680180505,13.8926337693761,
130.656209398717)) ;
#121789=CARTESIAN_POINT('Ctrl Pts',(-24.728815676264,14.1134974060216,130.50464468711)) ;
#121790=CARTESIAN_POINT('Ctrl Pts',(-24.670909042521,14.2854804589728,130.302270913447)) ;
#121791=CARTESIAN_POINT('Ctrl Pts',(-24.60088451724,14.394916969494,130.064614299334)) ;
#121792=CARTESIAN_POINT('Ctrl Pts',(-24.5245965657273,14.435095047054,129.808769177446)) ;
#121793=CARTESIAN_POINT('Ctrl Pts',(-24.4473637068243,14.4027523560096,
129.549904857935)) ;
#121794=CARTESIAN_POINT('Ctrl Pts',(-24.3764277230312,14.3004224301193,
129.309619108113)) ;
#121795=CARTESIAN_POINT('Ctrl Pts',(-24.3169230241164,14.1345848207203,
129.102566773987)) ;
#121796=CARTESIAN_POINT('Ctrl Pts',(-24.2744113644466,13.9188292654447,
128.945352262584)) ;
#121797=CARTESIAN_POINT('Ctrl Pts',(-24.2522045947965,13.6668968226668,
128.847333371272)) ;
#121798=CARTESIAN_POINT('Ctrl Pts',(-24.2527678420555,13.3982258049414,
128.815930108952)) ;
#121799=CARTESIAN_POINT('Ctrl Pts',(-24.276897987138,13.1299459818543,128.853191114343)) ;
#121800=CARTESIAN_POINT('Ctrl Pts',(-24.3234245762368,12.8837060048702,
128.956014438392)) ;
#121801=CARTESIAN_POINT('Ctrl Pts',(-24.3900144260355,12.6755091037675,
129.117341319656)) ;
#121802=CARTESIAN_POINT('Ctrl Pts',(-24.4721077500629,12.5215778341602,
129.324106647647)) ;
#121803=CARTESIAN_POINT('Ctrl Pts',(-24.565308269843,12.4317802078497,129.563149664211)) ;
#121804=CARTESIAN_POINT('Ctrl Pts',(-24.6624846240227,12.4131805145463,
129.814074666226)) ;
#121805=CARTESIAN_POINT('Ctrl Pts',(-24.7588780185162,12.4668842843224,
130.062448733751)) ;
#121806=CARTESIAN_POINT('Ctrl Pts',(-24.8470359043657,12.5884450791791,
130.286983079046)) ;
#121807=CARTESIAN_POINT('Ctrl Pts',(-24.9226051504243,12.7713421564293,
130.474427343393)) ;
#121808=CARTESIAN_POINT('Ctrl Pts',(-24.9795413821956,12.9988618767288,
130.607794145805)) ;
#121809=CARTESIAN_POINT('Ctrl Pts',(-25.0156442703355,13.259491403766,130.679917395231)) ;
#121810=CARTESIAN_POINT('Ctrl Pts',(-25.0282091631295,13.5289134128762,
130.683668585279)) ;
#121811=CARTESIAN_POINT('Ctrl Pts',(-25.0176337181152,13.792044854945,130.619653232571)) ;
#121812=CARTESIAN_POINT('Ctrl Pts',(-24.9852005413018,14.0286824176204,
130.491809147473)) ;
#121813=CARTESIAN_POINT('Ctrl Pts',(-24.9337121650507,14.2226477736602,
130.308157090339)) ;
#121814=CARTESIAN_POINT('Ctrl Pts',(-24.8682137054445,14.3581280459106,
130.083808960179)) ;
#121815=CARTESIAN_POINT('Ctrl Pts',(-24.7936202112881,14.4275172368953,
129.832803504155)) ;
#121816=CARTESIAN_POINT('Ctrl Pts',(-24.7155627562385,14.4244373227483,
129.57144348336)) ;
#121817=CARTESIAN_POINT('Ctrl Pts',(-24.6418264545641,14.3501367823951,
129.323115479504)) ;
#121818=CARTESIAN_POINT('Ctrl Pts',(-24.5769236801836,14.2089997399679,
129.100323776134)) ;
#121819=CARTESIAN_POINT('Ctrl Pts',(-24.5270385018368,14.0121250451069,
128.921539786194)) ;
#121820=CARTESIAN_POINT('Ctrl Pts',(-24.4960631962097,13.7718246711113,
128.797806971439)) ;
#121821=CARTESIAN_POINT('Ctrl Pts',(-24.4872948571739,13.5078186231509,
128.739133036855)) ;
#121822=CARTESIAN_POINT('Ctrl Pts',(-24.5018717870073,13.2372789127591,
128.748585611505)) ;
#121823=CARTESIAN_POINT('Ctrl Pts',(-24.5394131760315,12.980432676453,128.82518927761)) ;
#121824=CARTESIAN_POINT('Ctrl Pts',(-24.5984747883142,12.7540238473754,
128.964448209837)) ;
#121825=CARTESIAN_POINT('Ctrl Pts',(-24.6744370598604,12.5774627214212,
129.153422120935)) ;
#121826=CARTESIAN_POINT('Ctrl Pts',(-24.7639922634429,12.4598742845048,
129.381793089141)) ;
#121827=CARTESIAN_POINT('Ctrl Pts',(-24.8605500897258,12.4120040771025,
129.630724349691)) ;
#121828=CARTESIAN_POINT('Ctrl Pts',(-24.958005807099,12.4365719363613,129.882309681314)) ;
#121829=CARTESIAN_POINT('Ctrl Pts',(-25.050014463376,12.5311793730478,130.118080286586)) ;
#121830=CARTESIAN_POINT('Ctrl Pts',(-25.1316226244339,12.6910252991536,
130.323175898126)) ;
#121831=CARTESIAN_POINT('Ctrl Pts',(-25.1962471146522,12.9015546057863,
130.478998345646)) ;
#121832=CARTESIAN_POINT('Ctrl Pts',(-25.241234670559,13.1503193802668,130.577277708208)) ;
#121833=CARTESIAN_POINT('Ctrl Pts',(-25.2634976452827,13.4198238149612,
130.609042385242)) ;
#121834=CARTESIAN_POINT('Ctrl Pts',(-25.2622779519396,13.6867201832379,
130.572566966855)) ;
#121835=CARTESIAN_POINT('Ctrl Pts',(-25.2383200577923,13.9376559863072,
130.469290386923)) ;
#121836=CARTESIAN_POINT('Ctrl Pts',(-25.1941474736539,14.1502428615257,
130.307142874577)) ;
#121837=CARTESIAN_POINT('Ctrl Pts',(-25.1337264695222,14.3108380697217,
130.097535620536)) ;
#121838=CARTESIAN_POINT('Ctrl Pts',(-25.0620137026065,14.4079445348436,
129.854934695128)) ;
#121839=CARTESIAN_POINT('Ctrl Pts',(-24.9848714963236,14.4345276706247,
129.596461986952)) ;
#121840=CARTESIAN_POINT('Ctrl Pts',(-24.9086676865302,14.3888298731307,
129.340776078196)) ;
#121841=CARTESIAN_POINT('Ctrl Pts',(-24.8393136852622,14.273828468375,129.105021772797)) ;
#121842=CARTESIAN_POINT('Ctrl Pts',(-24.7827347158713,14.0978368302853,
128.906604072011)) ;
#121843=CARTESIAN_POINT('Ctrl Pts',(-24.7436676855994,13.8735407233332,
128.759347918809)) ;
#121844=CARTESIAN_POINT('Ctrl Pts',(-24.7256369859318,13.6168750178338,
128.673534453122)) ;
#121845=CARTESIAN_POINT('Ctrl Pts',(-24.7306702277621,13.346506361492,128.655118284453)) ;
#121846=CARTESIAN_POINT('Ctrl Pts',(-24.7590932103143,13.0815407666398,
128.705024346918)) ;
#121847=CARTESIAN_POINT('Ctrl Pts',(-24.8097282840083,12.8409646602013,
128.819785475391)) ;
#121848=CARTESIAN_POINT('Ctrl Pts',(-24.8791063732593,12.6428639918128,
128.989483254521)) ;
#121849=CARTESIAN_POINT('Ctrl Pts',(-24.9645394688412,12.4989646430065,
129.205645392299)) ;
#121850=CARTESIAN_POINT('Ctrl Pts',(-25.0579878899541,12.4231076853541,
129.445814572811)) ;
#121851=CARTESIAN_POINT('Ctrl Pts',(-25.1562511213808,12.4177381591252,
129.699599598718)) ;
#121852=CARTESIAN_POINT('Ctrl Pts',(-25.2512788586479,12.4847095466627,
129.944123699546)) ;
#121853=CARTESIAN_POINT('Ctrl Pts',(-25.3377821946392,12.6190668251906,
130.163642451019)) ;
#121854=CARTESIAN_POINT('Ctrl Pts',(-25.4097944339434,12.8107471895688,
130.340916677767)) ;
#121855=CARTESIAN_POINT('Ctrl Pts',(-25.4631706931729,13.0461049078406,
130.463753164619)) ;
#121856=CARTESIAN_POINT('Ctrl Pts',(-25.4948238815669,13.3089104890012,
130.523073615046)) ;
#121857=CARTESIAN_POINT('Ctrl Pts',(-25.5031265241636,13.5795918474296,
130.514220263891)) ;
#121858=CARTESIAN_POINT('Ctrl Pts',(-25.4881933952742,13.8398549511919,
130.437390626082)) ;
#121859=CARTESIAN_POINT('Ctrl Pts',(-25.4517218808051,14.0698649783882,
130.297660885074)) ;
#121860=CARTESIAN_POINT('Ctrl Pts',(-25.3975893597401,14.2524396498396,
130.106562738251)) ;
#121861=CARTESIAN_POINT('Ctrl Pts',(-25.329628163741,14.3767943288433,129.874835912649)) ;
#121862=CARTESIAN_POINT('Ctrl Pts',(-25.2541712601105,14.4324209617662,
129.621391122632)) ;
#121863=CARTESIAN_POINT('Ctrl Pts',(-25.1765759645738,14.4159981078524,
129.361510885237)) ;
#121864=CARTESIAN_POINT('Ctrl Pts',(-25.1037149073964,14.3283155075796,
129.115542900356)) ;
#121865=CARTESIAN_POINT('Ctrl Pts',(-25.0413114335729,14.1755658927935,
128.900081780878)) ;
#121866=CARTESIAN_POINT('Ctrl Pts',(-24.9947967152274,13.9699067943466,
128.731193187408)) ;
#121867=CARTESIAN_POINT('Ctrl Pts',(-24.9678237957013,13.7239839863066,
128.619211007753)) ;
#121868=CARTESIAN_POINT('Ctrl Pts',(-24.9632948194165,13.4571372735282,
128.57289064357)) ;
#121869=CARTESIAN_POINT('Ctrl Pts',(-24.9824896393098,13.1860385080971,
128.595632297208)) ;
#121870=CARTESIAN_POINT('Ctrl Pts',(-25.0240453693991,12.9351633372793,
128.684136780175)) ;
#121871=CARTESIAN_POINT('Ctrl Pts',(-25.0868468687025,12.7162804283108,
128.834258486375)) ;
#121872=CARTESIAN_POINT('Ctrl Pts',(-25.1654757864791,12.5504602978257,
129.03108391557)) ;
#121873=CARTESIAN_POINT('Ctrl Pts',(-25.257301839938,12.4451571789981,129.265930804602)) ;
#121874=CARTESIAN_POINT('Ctrl Pts',(-25.3538628354389,12.4110818133835,
129.515105703089)) ;
#121875=CARTESIAN_POINT('Ctrl Pts',(-25.4513699463354,12.4493848627309,
129.766644069087)) ;
#121876=CARTESIAN_POINT('Ctrl Pts',(-25.5413331144309,12.5564279149636,
129.996576060182)) ;
#121877=CARTESIAN_POINT('Ctrl Pts',(-25.62031355426,12.7270948796437,130.19397859587)) ;
#121878=CARTESIAN_POINT('Ctrl Pts',(-25.6816176160566,12.9467013560163,
130.339987705186)) ;
#121879=CARTESIAN_POINT('Ctrl Pts',(-25.7223434773691,13.2005745815833,
130.425833032778)) ;
#121880=CARTESIAN_POINT('Ctrl Pts',(-25.7401264335062,13.4697556430519,
130.444737141503)) ;
#121881=CARTESIAN_POINT('Ctrl Pts',(-25.7345998226882,13.736255276326,130.395473264133)) ;
#121882=CARTESIAN_POINT('Ctrl Pts',(-25.7064542497978,13.9814042376555,
130.279958796847)) ;
#121883=CARTESIAN_POINT('Ctrl Pts',(-25.6591900336752,14.1841667225104,
130.108970524327)) ;
#121884=CARTESIAN_POINT('Ctrl Pts',(-25.5960522185544,14.3343212234818,
129.891306413167)) ;
#121885=CARTESIAN_POINT('Ctrl Pts',(-25.5227733731923,14.4184551255459,
129.644101823257)) ;
#121886=CARTESIAN_POINT('Ctrl Pts',(-25.4454407026881,14.4314519910157,
129.385130431416)) ;
#121887=CARTESIAN_POINT('Ctrl Pts',(-25.3699325639496,14.3721434966701,
129.13139873682)) ;
#121888=CARTESIAN_POINT('Ctrl Pts',(-25.3027559014807,14.245373795937,128.90211376727)) ;
#121889=CARTESIAN_POINT('Ctrl Pts',(-25.2488792802276,14.0581566175582,
128.711411678173)) ;
#121890=CARTESIAN_POINT('Ctrl Pts',(-25.2137932802583,13.8276967157625,
128.575975328907)) ;
#121891=CARTESIAN_POINT('Ctrl Pts',(-25.199880050692,13.5670202701056,128.502182318622)) ;
#121892=CARTESIAN_POINT('Ctrl Pts',(-25.2093925008277,13.2953785672156,
128.496751191105)) ;
#121893=CARTESIAN_POINT('Ctrl Pts',(-25.242028626857,13.0342213948757,128.559046958988)) ;
#121894=CARTESIAN_POINT('Ctrl Pts',(-25.2967851107302,12.799235193231,128.685702810719)) ;
#121895=CARTESIAN_POINT('Ctrl Pts',(-25.3692327223565,12.6113832489784,
128.864447663773)) ;
#121896=CARTESIAN_POINT('Ctrl Pts',(-25.4562878134917,12.4798503572911,
129.085564966862)) ;
#121897=CARTESIAN_POINT('Ctrl Pts',(-25.5516448147479,12.4163978542697,
129.33103303498)) ;
#121898=CARTESIAN_POINT('Ctrl Pts',(-25.6496515407606,12.4249215089451,
129.584153609053)) ;
#121899=CARTESIAN_POINT('Ctrl Pts',(-25.7437456969646,12.505375632336,129.82584674247)) ;
#121900=CARTESIAN_POINT('Ctrl Pts',(-25.8274940922264,12.6507859579669,
130.037493290738)) ;
#121901=CARTESIAN_POINT('Ctrl Pts',(-25.8964204891319,12.8517471604921,
130.205732105265)) ;
#121902=CARTESIAN_POINT('Ctrl Pts',(-25.9460652372226,13.0945615121704,
130.317535454147)) ;
#121903=CARTESIAN_POINT('Ctrl Pts',(-25.9733381607594,13.3602126938648,
130.364087679988)) ;
#121904=CARTESIAN_POINT('Ctrl Pts',(-25.9771342123268,13.6310672418703,
130.341965603779)) ;
#121905=CARTESIAN_POINT('Ctrl Pts',(-25.9580426264907,13.8852754196112,
130.253211878795)) ;
#121906=CARTESIAN_POINT('Ctrl Pts',(-25.9180734791188,14.1076160961634,
130.103323578132)) ;
#121907=CARTESIAN_POINT('Ctrl Pts',(-25.8607234852378,14.2808806775566,
129.902643243913)) ;
#121908=CARTESIAN_POINT('Ctrl Pts',(-25.7910301799006,14.3926567140697,
129.665957266958)) ;
#121909=CARTESIAN_POINT('Ctrl Pts',(-25.7142471691777,14.4348969487797,
129.408406813689)) ;
#121910=CARTESIAN_POINT('Ctrl Pts',(-25.6376724285755,14.4049966938089,
129.151792715386)) ;
#121911=CARTESIAN_POINT('Ctrl Pts',(-25.5658305442248,14.3037928879971,
128.908552136202)) ;
#121912=CARTESIAN_POINT('Ctrl Pts',(-25.506358907673,14.1405203886364,128.701827306642)) ;
#121913=CARTESIAN_POINT('Ctrl Pts',(-25.4631682807316,13.9258191090176,
128.542562680316)) ;
#121914=CARTESIAN_POINT('Ctrl Pts',(-25.4403035221641,13.6747404934951,
128.442635874831)) ;
#121915=CARTESIAN_POINT('Ctrl Pts',(-25.4402682048589,13.4052256661744,
128.409346773511)) ;
#121916=CARTESIAN_POINT('Ctrl Pts',(-25.4635287824975,13.138469239792,128.444304954167)) ;
#121917=CARTESIAN_POINT('Ctrl Pts',(-25.5097037479834,12.8897551396211,
128.545882952362)) ;
#121918=CARTESIAN_POINT('Ctrl Pts',(-25.5754518262798,12.6813707794316,
128.704929877967)) ;
#121919=CARTESIAN_POINT('Ctrl Pts',(-25.6572496262362,12.5252896254052,
128.910771575894)) ;
#121920=CARTESIAN_POINT('Ctrl Pts',(-25.7500041562407,12.4335761990142,
129.148588024565)) ;
#121921=CARTESIAN_POINT('Ctrl Pts',(-25.8474528188583,12.4126069682806,
129.400196063375)) ;
#121922=CARTESIAN_POINT('Ctrl Pts',(-25.9442289971032,12.4645413943428,
129.649602932719)) ;
#121923=CARTESIAN_POINT('Ctrl Pts',(-26.0326523326431,12.5845283028617,
129.87490638314)) ;
#121924=CARTESIAN_POINT('Ctrl Pts',(-26.1084253037707,12.7652451622035,
130.063060396479)) ;
#121925=CARTESIAN_POINT('Ctrl Pts',(-26.1660218667408,12.9922348070079,
130.198275358319)) ;
#121926=CARTESIAN_POINT('Ctrl Pts',(-26.2025467695787,13.2501819432392,
130.271891359002)) ;
#121927=CARTESIAN_POINT('Ctrl Pts',(-26.2160056211235,13.5208713939763,
130.278085368767)) ;
#121928=CARTESIAN_POINT('Ctrl Pts',(-26.206009335873,13.7852949674506,130.21566252207)) ;
#121929=CARTESIAN_POINT('Ctrl Pts',(-26.1740705858152,14.0230294711121,
130.089232482416)) ;
#121930=CARTESIAN_POINT('Ctrl Pts',(-26.1231731249939,14.217815504055,129.907395112279)) ;
#121931=CARTESIAN_POINT('Ctrl Pts',(-26.0580185278002,14.355293096106,129.684044299522)) ;
#121932=CARTESIAN_POINT('Ctrl Pts',(-25.983262509313,14.4265292690715,129.43242362093)) ;
#121933=CARTESIAN_POINT('Ctrl Pts',(-25.9060966194187,14.4257522115435,
129.174057322067)) ;
#121934=CARTESIAN_POINT('Ctrl Pts',(-25.8315111612316,14.353191154613,128.922957605569)) ;
#121935=CARTESIAN_POINT('Ctrl Pts',(-25.7664287352936,14.2139748477186,
128.699722439815)) ;
#121936=CARTESIAN_POINT('Ctrl Pts',(-25.7159572141074,14.0181342342469,
128.519151627063)) ;
#121937=CARTESIAN_POINT('Ctrl Pts',(-25.6844901245746,13.7796844257176,
128.394105513431)) ;
#121938=CARTESIAN_POINT('Ctrl Pts',(-25.6750002228921,13.515523516605,128.333239510458)) ;
#121939=CARTESIAN_POINT('Ctrl Pts',(-25.6888958759568,13.2452125858444,
128.340744783975)) ;
#121940=CARTESIAN_POINT('Ctrl Pts',(-25.7257689266178,12.9877057714763,
128.415394038105)) ;
#121941=CARTESIAN_POINT('Ctrl Pts',(-25.7841890846381,12.760206013501,128.55280276842)) ;
#121942=CARTESIAN_POINT('Ctrl Pts',(-25.8598555926733,12.5817512352831,
128.740846836256)) ;
#121943=CARTESIAN_POINT('Ctrl Pts',(-25.9488208517265,12.4625557335165,
128.967601700787)) ;
#121944=CARTESIAN_POINT('Ctrl Pts',(-26.0453904919063,12.4124303702056,
129.216512455731)) ;
#121945=CARTESIAN_POINT('Ctrl Pts',(-26.1427552661478,12.4345388206878,
129.467894999594)) ;
#121946=CARTESIAN_POINT('Ctrl Pts',(-26.2357965592368,12.5283216628162,
129.706376449232)) ;
#121947=CARTESIAN_POINT('Ctrl Pts',(-26.3169003500636,12.6848122547612,
129.910366034385)) ;
#121948=CARTESIAN_POINT('Ctrl Pts',(-26.3826387576274,12.8954783028643,
130.069177959724)) ;
#121949=CARTESIAN_POINT('Ctrl Pts',(-26.4280095043964,13.143031226721,130.168655675774)) ;
#121950=CARTESIAN_POINT('Ctrl Pts',(-26.450935350615,13.4109716015929,130.202504343147)) ;
#121951=CARTESIAN_POINT('Ctrl Pts',(-26.4504475400349,13.6794256952143,
130.168012298584)) ;
#121952=CARTESIAN_POINT('Ctrl Pts',(-26.4270028495607,13.9314101071075,
130.066190753789)) ;
#121953=CARTESIAN_POINT('Ctrl Pts',(-26.3834997753375,14.1445006476294,
129.906112198424)) ;
#121954=CARTESIAN_POINT('Ctrl Pts',(-26.3235981297211,14.3067536446236,
129.698061730427)) ;
#121955=CARTESIAN_POINT('Ctrl Pts',(-26.2520620230828,14.4060487060152,
129.455937008284)) ;
#121956=CARTESIAN_POINT('Ctrl Pts',(-26.174928116071,14.4348548850669,129.197464917097)) ;
#121957=CARTESIAN_POINT('Ctrl Pts',(-26.0984041323465,14.3909041577753,
128.94074554739)) ;
#121958=CARTESIAN_POINT('Ctrl Pts',(-26.0290760972212,14.2783347271922,
128.705219923887)) ;
#121959=CARTESIAN_POINT('Ctrl Pts',(-25.9717745366847,14.1031935059032,
128.504534965738)) ;
#121960=CARTESIAN_POINT('Ctrl Pts',(-25.9322636718303,13.880010412854,128.356003427703)) ;
#121961=CARTESIAN_POINT('Ctrl Pts',(-25.9136478323287,13.6249526911944,
128.268597684632)) ;
#121962=CARTESIAN_POINT('Ctrl Pts',(-25.9179653984303,13.354798949211,128.248097370987)) ;
#121963=CARTESIAN_POINT('Ctrl Pts',(-25.9455877308256,13.0897726213642,
128.295720076923)) ;
#121964=CARTESIAN_POINT('Ctrl Pts',(-25.9958936161693,12.8467548703801,
128.409323070075)) ;
#121965=CARTESIAN_POINT('Ctrl Pts',(-26.0647784470602,12.6478123647641,
128.57762440491)) ;
#121966=CARTESIAN_POINT('Ctrl Pts',(-26.1492052203305,12.5027971632239,
128.791074301569)) ;
#121967=CARTESIAN_POINT('Ctrl Pts',(-26.2432329578599,12.4240443471672,
129.032655898126)) ;
#121968=CARTESIAN_POINT('Ctrl Pts',(-26.3415402813396,12.4170503727496,
129.286553901924)) ;
#121969=CARTESIAN_POINT('Ctrl Pts',(-26.4363638435478,12.4817914292567,
129.530606090837)) ;
#121970=CARTESIAN_POINT('Ctrl Pts',(-26.5232308323837,12.6142901362916,
129.751179335933)) ;
#121971=CARTESIAN_POINT('Ctrl Pts',(-26.59563989411,12.8042104652996,129.929654314528)) ;
#121972=CARTESIAN_POINT('Ctrl Pts',(-26.6497502115733,13.0388187683455,
130.054583398585)) ;
#121973=CARTESIAN_POINT('Ctrl Pts',(-26.6820960427729,13.3023286417973,
130.115780574569)) ;
#121974=CARTESIAN_POINT('Ctrl Pts',(-26.6909894034587,13.571341528554,130.108864472769)) ;
#121975=CARTESIAN_POINT('Ctrl Pts',(-26.6767021676116,13.8329963549421,
130.0338176991)) ;
#121976=CARTESIAN_POINT('Ctrl Pts',(-26.6408767843664,14.0635777479953,
129.896055870966)) ;
#121977=CARTESIAN_POINT('Ctrl Pts',(-26.5871216615792,14.2479537659708,
129.706003217297)) ;
#121978=CARTESIAN_POINT('Ctrl Pts',(-26.5197195012801,14.3739504814687,
129.476021464279)) ;
#121979=CARTESIAN_POINT('Ctrl Pts',(-26.4437789239592,14.4320428256961,
129.220888386353)) ;
#121980=CARTESIAN_POINT('Ctrl Pts',(-26.3663527850407,14.417227489115,128.961592061449)) ;
#121981=CARTESIAN_POINT('Ctrl Pts',(-26.2935448158709,14.3318166696858,
128.715892691924)) ;
#121982=CARTESIAN_POINT('Ctrl Pts',(-26.23079022742,14.1811817924182,128.499448823311)) ;
#121983=CARTESIAN_POINT('Ctrl Pts',(-26.183588181247,13.9759967234678,128.328412475923)) ;
#121984=CARTESIAN_POINT('Ctrl Pts',(-26.1560379678286,13.7313492030733,
128.214805352919)) ;
#121985=CARTESIAN_POINT('Ctrl Pts',(-26.1509807959761,13.4634560829624,
128.166765320148)) ;
#121986=CARTESIAN_POINT('Ctrl Pts',(-26.1691472957076,13.1958849143636,
128.186976695918)) ;
#121987=CARTESIAN_POINT('Ctrl Pts',(-26.2104817509094,12.9412336892527,
128.274433943599)) ;
#121988=CARTESIAN_POINT('Ctrl Pts',(-26.2721716135339,12.7230235102752,
128.421620019773)) ;
#121989=CARTESIAN_POINT('Ctrl Pts',(-26.3510948457971,12.5539648148601,
128.618984638309)) ;
#121990=CARTESIAN_POINT('Ctrl Pts',(-26.4416854984019,12.4477725883293,
128.850585921141)) ;
#121991=CARTESIAN_POINT('Ctrl Pts',(-26.5388603867134,12.4110238127138,
129.101295822546)) ;
#121992=CARTESIAN_POINT('Ctrl Pts',(-26.6359779446456,12.4468710240649,
129.351877582573)) ;
#121993=CARTESIAN_POINT('Ctrl Pts',(-26.7271512360903,12.5531554013667,
129.584988732517)) ;
#121994=CARTESIAN_POINT('Ctrl Pts',(-26.8058876475167,12.7211113727201,
129.781943258164)) ;
#121995=CARTESIAN_POINT('Ctrl Pts',(-26.867958160108,12.9400020484962,129.930089354973)) ;
#121996=CARTESIAN_POINT('Ctrl Pts',(-26.9091588040755,13.1921120918715,
130.017459671564)) ;
#121997=CARTESIAN_POINT('Ctrl Pts',(-26.9277711979778,13.4620045892925,
130.038672040359)) ;
#121998=CARTESIAN_POINT('Ctrl Pts',(-26.9228008675889,13.7292706883455,
129.990975910418)) ;
#121999=CARTESIAN_POINT('Ctrl Pts',(-26.8955075945293,13.9738126531135,
129.878168064945)) ;
#122000=CARTESIAN_POINT('Ctrl Pts',(-26.8485030327011,14.179494761427,129.707716653188)) ;
#122001=CARTESIAN_POINT('Ctrl Pts',(-26.7855978873256,14.3311259562621,
129.490701648116)) ;
#122002=CARTESIAN_POINT('Ctrl Pts',(-26.7129553496451,14.4169205750236,
129.24554392929)) ;
#122003=CARTESIAN_POINT('Ctrl Pts',(-26.6352142982145,14.4320030262707,
128.98518159896)) ;
#122004=CARTESIAN_POINT('Ctrl Pts',(-26.5599753455434,14.3751243416082,
128.732432725729)) ;
#122005=CARTESIAN_POINT('Ctrl Pts',(-26.491906908084,14.2488767663409,128.500232903427)) ;
#122006=CARTESIAN_POINT('Ctrl Pts',(-26.4381398546264,14.0648018016439,
128.310179587544)) ;
#122007=CARTESIAN_POINT('Ctrl Pts',(-26.4022035176628,13.8343787612975,
128.17207828747)) ;
#122008=CARTESIAN_POINT('Ctrl Pts',(-26.3877376570125,13.57360703546,128.096606127826)) ;
#122009=CARTESIAN_POINT('Ctrl Pts',(-26.3966428099618,13.3025524242793,
128.089467724452)) ;
#122010=CARTESIAN_POINT('Ctrl Pts',(-26.4285388264674,13.0417944958654,
128.149713107354)) ;
#122011=CARTESIAN_POINT('Ctrl Pts',(-26.4824445567047,12.8063139825281,
128.273986576365)) ;
#122012=CARTESIAN_POINT('Ctrl Pts',(-26.5547260838546,12.6158856325691,
128.452084531992)) ;
#122013=CARTESIAN_POINT('Ctrl Pts',(-26.6416219728868,12.4825396581066,
128.672687777498)) ;
#122014=CARTESIAN_POINT('Ctrl Pts',(-26.7365473365606,12.4173081126312,
128.916989601117)) ;
#122015=CARTESIAN_POINT('Ctrl Pts',(-26.8344661154599,12.4236050164849,
129.169887633563)) ;
#122016=CARTESIAN_POINT('Ctrl Pts',(-26.9287291207569,12.5018026361359,
129.4120930787)) ;
#122017=CARTESIAN_POINT('Ctrl Pts',(-27.0131217845774,12.6458566369947,
129.625516102499)) ;
#122018=CARTESIAN_POINT('Ctrl Pts',(-27.0824647965145,12.8453791511498,
129.794993955093)) ;
#122019=CARTESIAN_POINT('Ctrl Pts',(-27.1326350432609,13.0865653368531,
129.908416385334)) ;
#122020=CARTESIAN_POINT('Ctrl Pts',(-27.1606365627051,13.3521428238873,
129.957049192237)) ;
#122021=CARTESIAN_POINT('Ctrl Pts',(-27.1651689294827,13.6222557770976,
129.93719049098)) ;
#122022=CARTESIAN_POINT('Ctrl Pts',(-27.1467153752729,13.878388340665,129.850152045609)) ;
#122023=CARTESIAN_POINT('Ctrl Pts',(-27.1071678329421,14.1022120909712,
129.701435023225)) ;
#122024=CARTESIAN_POINT('Ctrl Pts',(-27.0504028748614,14.2765229673721,
129.502557758353)) ;
#122025=CARTESIAN_POINT('Ctrl Pts',(-26.9810910649829,14.3902287028563,
129.267020257534)) ;
#122026=CARTESIAN_POINT('Ctrl Pts',(-26.9043059277822,14.4347769425123,
129.009416197046)) ;
#122027=CARTESIAN_POINT('Ctrl Pts',(-26.8275120953152,14.406672259026,128.752091523846)) ;
#122028=CARTESIAN_POINT('Ctrl Pts',(-26.7558435515678,14.3082119103095,
128.509567117461)) ;
#122029=CARTESIAN_POINT('Ctrl Pts',(-26.6956342816198,14.146035786889,128.300525349841)) ;
#122030=CARTESIAN_POINT('Ctrl Pts',(-26.6519469354556,13.9328084599434,
128.139848548639)) ;
#122031=CARTESIAN_POINT('Ctrl Pts',(-26.6284335363191,13.6817741285683,
128.037926381176)) ;
#122032=CARTESIAN_POINT('Ctrl Pts',(-26.627674518559,13.4140262407359,128.002715819442)) ;
#122033=CARTESIAN_POINT('Ctrl Pts',(-26.6504162861654,13.1453688481844,
128.035950834501)) ;
#122034=CARTESIAN_POINT('Ctrl Pts',(-26.6955480888432,12.8977836730895,
128.134762681728)) ;
#122035=CARTESIAN_POINT('Ctrl Pts',(-26.7612516854397,12.6861562581584,
128.293396651609)) ;
#122036=CARTESIAN_POINT('Ctrl Pts',(-26.8425418015955,12.5289208542769,
128.497830773323)) ;
#122037=CARTESIAN_POINT('Ctrl Pts',(-26.9351615000927,12.43515491016,128.735214369181)) ;
#122038=CARTESIAN_POINT('Ctrl Pts',(-27.0323345672073,12.4122393521451,
128.986094141453)) ;
#122039=CARTESIAN_POINT('Ctrl Pts',(-27.1292337281549,12.461921394401,129.235865336576)) ;
#122040=CARTESIAN_POINT('Ctrl Pts',(-27.2181630496938,12.5803996881322,
129.462565138042)) ;
#122041=CARTESIAN_POINT('Ctrl Pts',(-27.2941848507928,12.7591299511845,
129.651530481398)) ;
#122042=CARTESIAN_POINT('Ctrl Pts',(-27.3524160962972,12.9850687744513,
129.788575819063)) ;
#122043=CARTESIAN_POINT('Ctrl Pts',(-27.3895887844412,13.2423777832249,
129.864086182952)) ;
#122044=CARTESIAN_POINT('Ctrl Pts',(-27.4037202433593,13.5129449874981,
129.872246514025)) ;
#122045=CARTESIAN_POINT('Ctrl Pts',(-27.3944549137884,13.7774321466873,
129.812018614547)) ;
#122046=CARTESIAN_POINT('Ctrl Pts',(-27.3630500859143,14.0166134840393,
129.687079327019)) ;
#122047=CARTESIAN_POINT('Ctrl Pts',(-27.3129661381804,14.2120831170415,
129.507790243548)) ;
#122048=CARTESIAN_POINT('Ctrl Pts',(-27.2477111859512,14.3524989582878,
129.283900035096)) ;
#122049=CARTESIAN_POINT('Ctrl Pts',(-27.1733683419627,14.4253825851082,
129.033603144489)) ;
#122050=CARTESIAN_POINT('Ctrl Pts',(-27.0960794174057,14.4267682802424,
128.774817103346)) ;
#122051=CARTESIAN_POINT('Ctrl Pts',(-27.0214960019201,14.3564919766321,
128.523812290043)) ;
#122052=CARTESIAN_POINT('Ctrl Pts',(-26.9558285638099,14.2186718710266,
128.298750545118)) ;
#122053=CARTESIAN_POINT('Ctrl Pts',(-26.9049226632705,14.024316702861,128.116933923083)) ;
#122054=CARTESIAN_POINT('Ctrl Pts',(-26.8728650693728,13.7866135128635,
127.990131547778)) ;
#122055=CARTESIAN_POINT('Ctrl Pts',(-26.8627445051173,13.5238036073327,
127.927533017912)) ;
#122056=CARTESIAN_POINT('Ctrl Pts',(-26.8759282572692,13.2527085149488,
127.932875171152)) ;
#122057=CARTESIAN_POINT('Ctrl Pts',(-26.9124124688024,12.9936529878453,
128.006256802744)) ;
#122058=CARTESIAN_POINT('Ctrl Pts',(-26.9700245887179,12.7662441294868,
128.141471141094)) ;
#122059=CARTESIAN_POINT('Ctrl Pts',(-27.0453501773252,12.5858801023732,
128.328462165356)) ;
#122060=CARTESIAN_POINT('Ctrl Pts',(-27.1340923349453,12.4648530530782,
128.554546945788)) ;
#122061=CARTESIAN_POINT('Ctrl Pts',(-27.2306903180176,12.4128201852834,
128.803491256227)) ;
#122062=CARTESIAN_POINT('Ctrl Pts',(-27.3277245909402,12.4330274205639,
129.054033267904)) ;
#122063=CARTESIAN_POINT('Ctrl Pts',(-27.420587314234,12.5240123419654,129.292155039348)) ;
#122064=CARTESIAN_POINT('Ctrl Pts',(-27.5026088157967,12.6795221471728,
129.4986303408)) ;
#122065=CARTESIAN_POINT('Ctrl Pts',(-27.56880507535,12.8889214300487,129.658790927613)) ;
#122066=CARTESIAN_POINT('Ctrl Pts',(-27.614815972317,13.1354947204779,129.760149867447)) ;
#122067=CARTESIAN_POINT('Ctrl Pts',(-27.6384438856448,13.4042911484909,
129.795909071005)) ;
#122068=CARTESIAN_POINT('Ctrl Pts',(-27.638531524892,13.6719452324486,129.763222402758)) ;
#122069=CARTESIAN_POINT('Ctrl Pts',(-27.6158224189632,13.9242175313922,
129.663622850511)) ;
#122070=CARTESIAN_POINT('Ctrl Pts',(-27.572798679322,14.1390288718251,129.504884677249)) ;
#122071=CARTESIAN_POINT('Ctrl Pts',(-27.513252891317,14.3030286134432,129.297851793418)) ;
#122072=CARTESIAN_POINT('Ctrl Pts',(-27.4419265027612,14.404195333154,129.056326335695)) ;
#122073=CARTESIAN_POINT('Ctrl Pts',(-27.3651061813518,14.4349854783543,
128.79887103993)) ;
#122074=CARTESIAN_POINT('Ctrl Pts',(-27.2884597326731,14.3934046860553,
128.541796190572)) ;
#122075=CARTESIAN_POINT('Ctrl Pts',(-27.2186122844583,14.2822103029933,
128.304629732468)) ;
#122076=CARTESIAN_POINT('Ctrl Pts',(-27.1612236221931,14.1097942178576,
128.103897060506)) ;
#122077=CARTESIAN_POINT('Ctrl Pts',(-27.1209695384075,13.8877666791924,
127.953145883014)) ;
#122078=CARTESIAN_POINT('Ctrl Pts',(-27.1016395309341,13.6324083997063,
127.863526650496)) ;
#122079=CARTESIAN_POINT('Ctrl Pts',(-27.1052954562786,13.3624184985193,
127.841099006874)) ;
#122080=CARTESIAN_POINT('Ctrl Pts',(-27.1323671349213,13.0965814202268,
127.887054838906)) ;
#122081=CARTESIAN_POINT('Ctrl Pts',(-27.1817582727546,12.8540735599423,
127.99818617381)) ;
#122082=CARTESIAN_POINT('Ctrl Pts',(-27.2501946458088,12.6529923851621,
128.165102805726)) ;
#122083=CARTESIAN_POINT('Ctrl Pts',(-27.3347670251361,12.5055873938463,
128.378795585395)) ;
#122084=CARTESIAN_POINT('Ctrl Pts',(-27.4281737202757,12.4255318492028,
128.618720146286)) ;
#122085=CARTESIAN_POINT('Ctrl Pts',(-27.5260110615558,12.41606276029,128.871394756553)) ;
#122086=CARTESIAN_POINT('Ctrl Pts',(-27.6214751824357,12.478829942444,129.117158137395)) ;
#122087=CARTESIAN_POINT('Ctrl Pts',(-27.7087309583013,12.6096603386007,
129.338843492308)) ;
#122088=CARTESIAN_POINT('Ctrl Pts',(-27.7817420501725,12.7985462969973,
129.519009420162)) ;
#122089=CARTESIAN_POINT('Ctrl Pts',(-27.8362342975662,13.0317087125592,
129.645126399872)) ;
#122090=CARTESIAN_POINT('Ctrl Pts',(-27.8691744514199,13.2930836864475,
129.708250616972)) ;
#122091=CARTESIAN_POINT('Ctrl Pts',(-27.8788768367921,13.5641925745626,
129.70344323476)) ;
#122092=CARTESIAN_POINT('Ctrl Pts',(-27.8651790612343,13.8256807565213,
129.630204378494)) ;
#122093=CARTESIAN_POINT('Ctrl Pts',(-27.8301586837401,14.0565823950309,
129.494921896745)) ;
#122094=CARTESIAN_POINT('Ctrl Pts',(-27.7767369569256,14.2434411721512,
129.305720870279)) ;
#122095=CARTESIAN_POINT('Ctrl Pts',(-27.7093477667888,14.3714533932326,
129.075650866819)) ;
#122096=CARTESIAN_POINT('Ctrl Pts',(-27.6341917569376,14.4311593781317,
128.823088377139)) ;
#122097=CARTESIAN_POINT('Ctrl Pts',(-27.5565394264049,14.4188767221607,
128.563046725448)) ;
#122098=CARTESIAN_POINT('Ctrl Pts',(-27.4833555543512,14.3353893492018,
128.316188475308)) ;
#122099=CARTESIAN_POINT('Ctrl Pts',(-27.4200615928807,14.1858865785186,
128.098061220149)) ;
#122100=CARTESIAN_POINT('Ctrl Pts',(-27.3725451189786,13.982932266947,127.926249851755)) ;
#122101=CARTESIAN_POINT('Ctrl Pts',(-27.3443171583994,13.7386001468469,
127.81057521293)) ;
#122102=CARTESIAN_POINT('Ctrl Pts',(-27.3385532435846,13.472491032427,127.760647208021)) ;
#122103=CARTESIAN_POINT('Ctrl Pts',(-27.3561183196159,13.2027754330182,
127.778859895872)) ;
#122104=CARTESIAN_POINT('Ctrl Pts',(-27.3969178375316,12.947572926699,127.864767200057)) ;
#122105=CARTESIAN_POINT('Ctrl Pts',(-27.4579595443552,12.7286906750514,
128.010126305813)) ;
#122106=CARTESIAN_POINT('Ctrl Pts',(-27.536242792453,12.5582194191414,128.205697792925)) ;
#122107=CARTESIAN_POINT('Ctrl Pts',(-27.6270550381186,12.4495814743775,
128.437768406524)) ;
#122108=CARTESIAN_POINT('Ctrl Pts',(-27.7239408227956,12.4111325032394,
128.687708168369)) ;
#122109=CARTESIAN_POINT('Ctrl Pts',(-27.8209192941087,12.4448573223553,
128.937954006686)) ;
#122110=CARTESIAN_POINT('Ctrl Pts',(-27.912140970553,12.5485736252265,129.171305648138)) ;
#122111=CARTESIAN_POINT('Ctrl Pts',(-27.9918422589982,12.7160675406203,
129.370845077553)) ;
#122112=CARTESIAN_POINT('Ctrl Pts',(-28.0541095191813,12.9327061663297,
129.519736214929)) ;
#122113=CARTESIAN_POINT('Ctrl Pts',(-28.0961114867268,13.1846668461228,
129.609355795154)) ;
#122114=CARTESIAN_POINT('Ctrl Pts',(-28.1153430533785,13.4544224662781,
129.632372704712)) ;
#122115=CARTESIAN_POINT('Ctrl Pts',(-28.1110671408469,13.7215757501031,
129.586762859001)) ;
#122116=CARTESIAN_POINT('Ctrl Pts',(-28.0843498664941,13.9674106040572,
129.475585032641)) ;
#122117=CARTESIAN_POINT('Ctrl Pts',(-28.037929043125,14.1739595566239,129.306902469622)) ;
#122118=CARTESIAN_POINT('Ctrl Pts',(-27.9756458993413,14.3272529144105,
129.091797948064)) ;
#122119=CARTESIAN_POINT('Ctrl Pts',(-27.902736501693,14.4155298054197,128.845637413294)) ;
#122120=CARTESIAN_POINT('Ctrl Pts',(-27.8255218107392,14.4326688880929,
128.587029784971)) ;
#122121=CARTESIAN_POINT('Ctrl Pts',(-27.7496698410169,14.3775210612736,
128.332273988261)) ;
#122122=CARTESIAN_POINT('Ctrl Pts',(-27.6817779587366,14.2540409039206,
128.10083691294)) ;
#122123=CARTESIAN_POINT('Ctrl Pts',(-27.6272334434837,14.0709647731437,
127.908361698852)) ;
#122124=CARTESIAN_POINT('Ctrl Pts',(-27.590771642816,13.8416199051522,127.768737814126)) ;
#122125=CARTESIAN_POINT('Ctrl Pts',(-27.575654232938,13.5823884703292,127.691471326001)) ;
#122126=CARTESIAN_POINT('Ctrl Pts',(-27.5837290890939,13.3112803473401,
127.681899023074)) ;
#122127=CARTESIAN_POINT('Ctrl Pts',(-27.6151958140633,13.0483997002377,
127.740682725908)) ;
#122128=CARTESIAN_POINT('Ctrl Pts',(-27.6682760357924,12.8130297532618,
127.862704973521)) ;
#122129=CARTESIAN_POINT('Ctrl Pts',(-27.7402747174842,12.6204060162552,
128.039867549227)) ;
#122130=CARTESIAN_POINT('Ctrl Pts',(-27.8268049555487,12.4854478919258,
128.259425965447)) ;
#122131=CARTESIAN_POINT('Ctrl Pts',(-27.9215833060717,12.4181326606572,
128.503289393107)) ;
#122132=CARTESIAN_POINT('Ctrl Pts',(-28.0197801582564,12.4224942646145,
128.756911867378)) ;
#122133=CARTESIAN_POINT('Ctrl Pts',(-28.1141333474196,12.4989653492952,
128.99940414225)) ;
#122134=CARTESIAN_POINT('Ctrl Pts',(-28.1985201718138,12.6405920086238,
129.212953820927)) ;
#122135=CARTESIAN_POINT('Ctrl Pts',(-28.26860111647,12.8391594148647,129.384491828424)) ;
#122136=CARTESIAN_POINT('Ctrl Pts',(-28.3194453499789,13.0802460396382,
129.499785089664)) ;
#122137=CARTESIAN_POINT('Ctrl Pts',(-28.3479518760318,13.3449462912613,
129.549955580643)) ;
#122138=CARTESIAN_POINT('Ctrl Pts',(-28.3531447899655,13.614299734848,129.532134045205)) ;
#122139=CARTESIAN_POINT('Ctrl Pts',(-28.3353747732206,13.8710421702277,
129.447102522243)) ;
#122140=CARTESIAN_POINT('Ctrl Pts',(-28.29643056891,14.0962488627573,129.300139789109)) ;
#122141=CARTESIAN_POINT('Ctrl Pts',(-28.239735048489,14.272991429521,129.10127534637)) ;
#122142=CARTESIAN_POINT('Ctrl Pts',(-28.171042991182,14.3876795568682,128.867727126792)) ;
#122143=CARTESIAN_POINT('Ctrl Pts',(-28.0945098708047,14.4346057862448,
128.610910309842)) ;
#122144=CARTESIAN_POINT('Ctrl Pts',(-28.0172199102355,14.4082599424993,
128.351948838014)) ;
#122145=CARTESIAN_POINT('Ctrl Pts',(-27.945755360923,14.3122705822436,128.110224199333)) ;
#122146=CARTESIAN_POINT('Ctrl Pts',(-27.8848607524878,14.1514361820495,
127.89905904971)) ;
#122147=CARTESIAN_POINT('Ctrl Pts',(-27.8406503955374,13.9387188784373,
127.736773571724)) ;
#122148=CARTESIAN_POINT('Ctrl Pts',(-27.8166293155747,13.6904434149952,
127.63362073482)) ;
#122149=CARTESIAN_POINT('Ctrl Pts',(-27.8151767965197,13.4208420632377,
127.596115768567)) ;
#122150=CARTESIAN_POINT('Ctrl Pts',(-27.8371800049029,13.1534853920285,
127.627393021463)) ;
#122151=CARTESIAN_POINT('Ctrl Pts',(-27.8817255227419,12.9044050276542,
127.724409631791)) ;
#122152=CARTESIAN_POINT('Ctrl Pts',(-27.9469701066089,12.691347593862,127.881682377476)) ;
#122153=CARTESIAN_POINT('Ctrl Pts',(-28.027963628144,12.5324268950077,128.085219224786)) ;
#122154=CARTESIAN_POINT('Ctrl Pts',(-28.1200287328796,12.4369854895294,
128.321097685028)) ;
#122155=CARTESIAN_POINT('Ctrl Pts',(-28.2173464985682,12.4119049764517,
128.572326876044)) ;
#122156=CARTESIAN_POINT('Ctrl Pts',(-28.3140197030252,12.4592885985088,
128.821560747272)) ;
#122157=CARTESIAN_POINT('Ctrl Pts',(-28.4033508529203,12.575733706437,129.049405146958)) ;
#122158=CARTESIAN_POINT('Ctrl Pts',(-28.4798796992957,12.7527803278304,
129.239845940824)) ;
#122159=CARTESIAN_POINT('Ctrl Pts',(-28.5389784527639,12.9786618836061,
129.379263313413)) ;
#122160=CARTESIAN_POINT('Ctrl Pts',(-28.5767125295995,13.2359089048801,
129.456355493055)) ;
#122161=CARTESIAN_POINT('Ctrl Pts',(-28.5914322564073,13.5051027063819,
129.466392895388)) ;
#122162=CARTESIAN_POINT('Ctrl Pts',(-28.5827452242765,13.771120969237,129.407710773932)) ;
#122163=CARTESIAN_POINT('Ctrl Pts',(-28.5520458960196,14.0100004351276,
129.285003580461)) ;
#122164=CARTESIAN_POINT('Ctrl Pts',(-28.5023750590468,14.2073725024461,
129.106849407342)) ;
#122165=CARTESIAN_POINT('Ctrl Pts',(-28.4375690543573,14.3492226720416,
128.884331903099)) ;
#122166=CARTESIAN_POINT('Ctrl Pts',(-28.3635165159496,14.4242520037555,
128.634920057826)) ;
#122167=CARTESIAN_POINT('Ctrl Pts',(-28.2858996813637,14.4277364435235,
128.375036176081)) ;
#122168=CARTESIAN_POINT('Ctrl Pts',(-28.2112539541308,14.3592419699784,
128.123884396452)) ;
#122169=CARTESIAN_POINT('Ctrl Pts',(-28.1455253888997,14.2240686259208,
127.898803886575)) ;
#122170=CARTESIAN_POINT('Ctrl Pts',(-28.0939162702605,14.0305584607837,
127.714807716224)) ;
#122171=CARTESIAN_POINT('Ctrl Pts',(-28.061332463252,13.7945205251559,127.586559380918)) ;
#122172=CARTESIAN_POINT('Ctrl Pts',(-28.0504816310014,13.5313066856814,
127.521709190659)) ;
#122173=CARTESIAN_POINT('Ctrl Pts',(-28.0630246250275,13.2605191131678,
127.525225826364)) ;
#122174=CARTESIAN_POINT('Ctrl Pts',(-28.0986987267832,13.0015410285169,
127.596334676114)) ;
#122175=CARTESIAN_POINT('Ctrl Pts',(-28.1557429004217,12.7725523248786,
127.729845571357)) ;
#122176=CARTESIAN_POINT('Ctrl Pts',(-28.2308151450779,12.5901313640957,
127.916009506223)) ;
#122177=CARTESIAN_POINT('Ctrl Pts',(-28.3192039621127,12.4675131143056,
128.141087303876)) ;
#122178=CARTESIAN_POINT('Ctrl Pts',(-28.4152292054608,12.4133289099041,
128.388505252399)) ;
#122179=CARTESIAN_POINT('Ctrl Pts',(-28.51300012079,12.4315113584402,128.64096395705)) ;
#122180=CARTESIAN_POINT('Ctrl Pts',(-28.6057703554483,12.5204618944922,
128.878923702572)) ;
#122181=CARTESIAN_POINT('Ctrl Pts',(-28.6881745533434,12.6740885855686,
129.086523806388)) ;
#122182=CARTESIAN_POINT('Ctrl Pts',(-28.7549081392456,12.8820605871686,
129.248262102328)) ;
#122183=CARTESIAN_POINT('Ctrl Pts',(-28.8015673967949,13.1280849227168,
129.351472289244)) ;
#122184=CARTESIAN_POINT('Ctrl Pts',(-28.8258432151059,13.3954305595711,
129.389263233344)) ;
#122185=CARTESIAN_POINT('Ctrl Pts',(-28.8266274541713,13.664772130159,129.358428105594)) ;
#122186=CARTESIAN_POINT('Ctrl Pts',(-28.8046464651445,13.916650368435,129.261114435001)) ;
#122187=CARTESIAN_POINT('Ctrl Pts',(-28.7621302419893,14.1333087809813,
129.103782522449)) ;
#122188=CARTESIAN_POINT('Ctrl Pts',(-28.7030824646286,14.2989356818664,
128.898242342101)) ;
#122189=CARTESIAN_POINT('Ctrl Pts',(-28.6315878673714,14.4025578141661,
128.656030107433)) ;
#122190=CARTESIAN_POINT('Ctrl Pts',(-28.5551034289532,14.4350103980761,
128.399673764832)) ;
#122191=CARTESIAN_POINT('Ctrl Pts',(-28.4784248234603,14.3956728073431,
128.142535589966)) ;
#122192=CARTESIAN_POINT('Ctrl Pts',(-28.4082689021954,14.2862787528374,
127.904446866476)) ;
#122193=CARTESIAN_POINT('Ctrl Pts',(-28.3504831872354,14.1158603426533,
127.702603041365)) ;
#122194=CARTESIAN_POINT('Ctrl Pts',(-28.3094811784105,13.8934485150928,
127.549446047251)) ;
#122195=CARTESIAN_POINT('Ctrl Pts',(-28.2896953739857,13.6404741079279,
127.458725935806)) ;
#122196=CARTESIAN_POINT('Ctrl Pts',(-28.2926725255243,13.3695006911583,
127.434168724953)) ;
#122197=CARTESIAN_POINT('Ctrl Pts',(-28.3190303266563,13.1044456788723,
127.478181906027)) ;
#122198=CARTESIAN_POINT('Ctrl Pts',(-28.3677161485524,12.8607039818763,
127.587239387159)) ;
#122199=CARTESIAN_POINT('Ctrl Pts',(-28.436248601719,12.6571154322834,127.754197746226)) ;
#122200=CARTESIAN_POINT('Ctrl Pts',(-28.519396273585,12.509808022699,127.964148826798)) ;
#122201=CARTESIAN_POINT('Ctrl Pts',(-28.6131255277483,12.4266891378063,
128.204805011976)) ;
#122202=CARTESIAN_POINT('Ctrl Pts',(-28.7112079392635,12.4154229833254,
128.458110282106)) ;
#122203=CARTESIAN_POINT('Ctrl Pts',(-28.8064841551431,12.4759771003581,
128.703440260766)) ;
#122204=CARTESIAN_POINT('Ctrl Pts',(-28.894082157132,12.6048252979973,128.92612571075)) ;
#122205=CARTESIAN_POINT('Ctrl Pts',(-28.9676084232411,12.792164644416,129.10779157021)) ;
#122206=CARTESIAN_POINT('Ctrl Pts',(-29.0227856027514,13.0247863190839,
129.235835629259)) ;
#122207=CARTESIAN_POINT('Ctrl Pts',(-29.0563556978844,13.2853106439738,
129.300842762572)) ;
#122208=CARTESIAN_POINT('Ctrl Pts',(-29.066673658485,13.5574332084958,129.297702546237)) ;
#122209=CARTESIAN_POINT('Ctrl Pts',(-29.0537954995477,13.8171022396022,
129.22717000876)) ;
#122210=CARTESIAN_POINT('Ctrl Pts',(-29.0191433426595,14.051173953077,129.092681320874)) ;
#122211=CARTESIAN_POINT('Ctrl Pts',(-28.9661997934839,14.2388282531697,
128.904948271921)) ;
#122212=CARTESIAN_POINT('Ctrl Pts',(-28.8993924137718,14.3685839592775,
128.676682134356)) ;
#122213=CARTESIAN_POINT('Ctrl Pts',(-28.8238015023144,14.4305511556418,
128.422593404806)) ;
#122214=CARTESIAN_POINT('Ctrl Pts',(-28.7466935435304,14.4203097239978,
128.164395594464)) ;
#122215=CARTESIAN_POINT('Ctrl Pts',(-28.6729565347358,14.3384207836783,
127.915751318186)) ;
#122216=CARTESIAN_POINT('Ctrl Pts',(-28.6096196405582,14.1915731436481,
127.697694520971)) ;
#122217=CARTESIAN_POINT('Ctrl Pts',(-28.5612220772461,13.9880714714153,
127.523004005157)) ;
#122218=CARTESIAN_POINT('Ctrl Pts',(-28.5327231257182,13.7471725052838,
127.406897590129)) ;
#122219=CARTESIAN_POINT('Ctrl Pts',(-28.5261588350729,13.4800206037099,
127.354436040776)) ;
#122220=CARTESIAN_POINT('Ctrl Pts',(-28.5430314034632,13.2110030429649,
127.370738064937)) ;
#122221=CARTESIAN_POINT('Ctrl Pts',(-28.5831526985241,12.9547748927777,
127.454630608314)) ;
#122222=CARTESIAN_POINT('Ctrl Pts',(-28.6436998125845,12.7344342247069,
127.598514032658)) ;
#122223=CARTESIAN_POINT('Ctrl Pts',(-28.7215842030367,12.5623453660856,
127.792909823269)) ;
#122224=CARTESIAN_POINT('Ctrl Pts',(-28.8119292432189,12.4518692088092,
128.023682354771)) ;
#122225=CARTESIAN_POINT('Ctrl Pts',(-28.9089970305816,12.4112334911996,
128.274053197857)) ;
#122226=CARTESIAN_POINT('Ctrl Pts',(-29.0059571272688,12.442749147776,128.524289458661)) ;
#122227=CARTESIAN_POINT('Ctrl Pts',(-29.0979629404732,12.5456206773071,
128.759711132298)) ;
#122228=CARTESIAN_POINT('Ctrl Pts',(-29.1770171698936,12.7091960236905,
128.957812071618)) ;
#122229=CARTESIAN_POINT('Ctrl Pts',(-29.2404374453014,12.9259029773537,
129.109812864898)) ;
#122230=CARTESIAN_POINT('Ctrl Pts',(-29.2829880269622,13.1770736237047,
129.201057279156)) ;
#122231=CARTESIAN_POINT('Ctrl Pts',(-29.3029145413432,13.4468768400015,
129.226065673819)) ;
#122232=CARTESIAN_POINT('Ctrl Pts',(-29.2992993295531,13.7138795897728,
129.182448022358)) ;
#122233=CARTESIAN_POINT('Ctrl Pts',(-29.273233977091,13.9605431985016,129.073181644377)) ;
#122234=CARTESIAN_POINT('Ctrl Pts',(-29.2273578624926,14.1686235654109,
128.906083428739)) ;
#122235=CARTESIAN_POINT('Ctrl Pts',(-29.1651531009933,14.324111284162,128.691062013158)) ;
#122236=CARTESIAN_POINT('Ctrl Pts',(-29.0928693974923,14.4138215880485,
128.446919954995)) ;
#122237=CARTESIAN_POINT('Ctrl Pts',(-29.0154061666861,14.4331945050443,
128.187453589773)) ;
#122238=CARTESIAN_POINT('Ctrl Pts',(-28.9396480617869,14.3801614626116,
127.933074508633)) ;
#122239=CARTESIAN_POINT('Ctrl Pts',(-28.871348616006,14.2584942565519,127.70040173552)) ;
#122240=CARTESIAN_POINT('Ctrl Pts',(-28.816378809689,14.0770491380578,127.506702993462)) ;
#122241=CARTESIAN_POINT('Ctrl Pts',(-28.7792697685908,13.8484874642558,
127.365136455592)) ;
#122242=CARTESIAN_POINT('Ctrl Pts',(-28.7635626541173,13.5893549989453,
127.286091315825)) ;
#122243=CARTESIAN_POINT('Ctrl Pts',(-28.7709351586529,13.319692173746,127.274636454019)) ;
#122244=CARTESIAN_POINT('Ctrl Pts',(-28.8016628955735,13.0561133199218,
127.331243888594)) ;
#122245=CARTESIAN_POINT('Ctrl Pts',(-28.8542955948744,12.8190740737043,
127.451871104289)) ;
#122246=CARTESIAN_POINT('Ctrl Pts',(-28.9257721083705,12.6252975626819,
127.627540714235)) ;
#122247=CARTESIAN_POINT('Ctrl Pts',(-29.0116152850741,12.4887796662223,
127.845210673493)) ;
#122248=CARTESIAN_POINT('Ctrl Pts',(-29.1065799591714,12.4190606373648,
128.089488486785)) ;
#122249=CARTESIAN_POINT('Ctrl Pts',(-29.2044154397174,12.4213023433048,
128.342181133046)) ;
#122250=CARTESIAN_POINT('Ctrl Pts',(-29.2990096465751,12.4953372710628,
128.585372578871)) ;
#122251=CARTESIAN_POINT('Ctrl Pts',(-29.3841743519178,12.6358733450884,
128.801032099907)) ;
#122252=CARTESIAN_POINT('Ctrl Pts',(-29.4545133975427,12.8325870207608,
128.973414377414)) ;
#122253=CARTESIAN_POINT('Ctrl Pts',(-29.5058639057111,13.0715963225307,
129.090313702067)) ;
#122254=CARTESIAN_POINT('Ctrl Pts',(-29.5352417115144,13.336692941588,129.142915133705)) ;
#122255=CARTESIAN_POINT('Ctrl Pts',(-29.5411110857573,13.6067854476423,
129.126995341538)) ;
#122256=CARTESIAN_POINT('Ctrl Pts',(-29.5239546110153,13.8640947363139,
129.043762287714)) ;
#122257=CARTESIAN_POINT('Ctrl Pts',(-29.4857056732189,14.089839779911,128.898926454628)) ;
#122258=CARTESIAN_POINT('Ctrl Pts',(-29.4295331965174,14.2683601910573,
128.701597333411)) ;
#122259=CARTESIAN_POINT('Ctrl Pts',(-29.360862541889,14.385487730189,128.467980808694)) ;
#122260=CARTESIAN_POINT('Ctrl Pts',(-29.2843675405681,14.4341894586694,
128.211244603888)) ;
#122261=CARTESIAN_POINT('Ctrl Pts',(-29.2074361909077,14.4102459791679,
127.953517340241)) ;
#122262=CARTESIAN_POINT('Ctrl Pts',(-29.1353314148325,14.3157190447574,
127.709734613321)) ;
#122263=CARTESIAN_POINT('Ctrl Pts',(-29.0743992312775,14.1574302898824,
127.498651642287)) ;
#122264=CARTESIAN_POINT('Ctrl Pts',(-29.0294533466867,13.9458829058386,
127.334150515467)) ;
#122265=CARTESIAN_POINT('Ctrl Pts',(-29.0047556089691,13.6969896283466,
127.228845194687)) ;
#122266=CARTESIAN_POINT('Ctrl Pts',(-29.002697162624,13.4292803806108,127.189768555857)) ;
#122267=CARTESIAN_POINT('Ctrl Pts',(-29.0238997906195,13.1613091083809,
127.21867643542)) ;
#122268=CARTESIAN_POINT('Ctrl Pts',(-29.0683112780447,12.9096301895175,
127.315037442774)) ;
#122269=CARTESIAN_POINT('Ctrl Pts',(-29.1323454225498,12.6977069155964,
127.469143576858)) ;
#122270=CARTESIAN_POINT('Ctrl Pts',(-29.2131615019566,12.536159176258,127.672031435155)) ;
#122271=CARTESIAN_POINT('Ctrl Pts',(-29.3049808389405,12.4388403103588,
127.907201582671)) ;
#122272=CARTESIAN_POINT('Ctrl Pts',(-29.4023352939487,12.4115721830993,
128.158500758783)) ;
#122273=CARTESIAN_POINT('Ctrl Pts',(-29.4991788664738,12.457029419961,128.408212309088)) ;
#122274=CARTESIAN_POINT('Ctrl Pts',(-29.5886148768168,12.5713337690677,
128.636430741871)) ;
#122275=CARTESIAN_POINT('Ctrl Pts',(-29.6656598966229,12.7468028835324,
128.8283599722)) ;
#122276=CARTESIAN_POINT('Ctrl Pts',(-29.72530058467,12.9715573467482,128.969356878356)) ;
#122277=CARTESIAN_POINT('Ctrl Pts',(-29.7636615833883,13.2272671930713,
129.048385247754)) ;
#122278=CARTESIAN_POINT('Ctrl Pts',(-29.7791134079089,13.4980619502807,
129.060344507591)) ;
#122279=CARTESIAN_POINT('Ctrl Pts',(-29.7712053180438,13.7620975253013,
129.004251069011)) ;
#122280=CARTESIAN_POINT('Ctrl Pts',(-29.7410277162991,14.0037249771829,
128.882841708814)) ;
#122281=CARTESIAN_POINT('Ctrl Pts',(-29.6918330478677,14.202400093294,128.706094471898)) ;
#122282=CARTESIAN_POINT('Ctrl Pts',(-29.6272000762833,14.3463073278919,
128.483991538536)) ;
#122283=CARTESIAN_POINT('Ctrl Pts',(-29.5536316150379,14.4229407274136,
128.23613229049)) ;
#122284=CARTESIAN_POINT('Ctrl Pts',(-29.4760239469434,14.4287087096985,
127.976268927856)) ;
#122285=CARTESIAN_POINT('Ctrl Pts',(-29.4011723177642,14.3623691322231,
127.724508956974)) ;
#122286=CARTESIAN_POINT('Ctrl Pts',(-29.3348404453428,14.2283779056864,
127.497526108696)) ;
#122287=CARTESIAN_POINT('Ctrl Pts',(-29.2828965479532,14.0364255545022,
127.312602435389)) ;
#122288=CARTESIAN_POINT('Ctrl Pts',(-29.2497959119098,13.8020943881553,
127.182934318226)) ;
#122289=CARTESIAN_POINT('Ctrl Pts',(-29.2382576660052,13.5391612776222,
127.116043482078)) ;
#122290=CARTESIAN_POINT('Ctrl Pts',(-29.2500815258749,13.268618582974,127.117498545445)) ;
#122291=CARTESIAN_POINT('Ctrl Pts',(-29.2851644533423,13.0086418344895,
127.186825345389)) ;
#122292=CARTESIAN_POINT('Ctrl Pts',(-29.3414272233796,12.7791079862287,
127.318152239982)) ;
#122293=CARTESIAN_POINT('Ctrl Pts',(-29.4163793099061,12.5942976841109,
127.503809818284)) ;
#122294=CARTESIAN_POINT('Ctrl Pts',(-29.5041535385455,12.4702970290912,
127.727214554869)) ;
#122295=CARTESIAN_POINT('Ctrl Pts',(-29.6002280837878,12.4139049816003,
127.974704992316)) ;
#122296=CARTESIAN_POINT('Ctrl Pts',(-29.6977091902929,12.4297924440583,
128.226434592627)) ;
#122297=CARTESIAN_POINT('Ctrl Pts',(-29.7913157701915,12.5172147656158,
128.466623365714)) ;
#122298=CARTESIAN_POINT('Ctrl Pts',(-29.874057974889,12.6696686051205,128.675189083843)) ;
#122299=CARTESIAN_POINT('Ctrl Pts',(-29.9408743154327,12.8748936311913,
128.83738804483)) ;
#122300=CARTESIAN_POINT('Ctrl Pts',(-29.9883376423857,13.1206629569548,
128.942849658263)) ;
#122301=CARTESIAN_POINT('Ctrl Pts',(-30.0132537062615,13.3874987151297,
128.982535373887)) ;
#122302=CARTESIAN_POINT('Ctrl Pts',(-30.0147150469051,13.6577700593923,
128.953591097854)) ;
#122303=CARTESIAN_POINT('Ctrl Pts',(-29.9932705416419,13.9102263629719,
128.857849398636)) ;
#122304=CARTESIAN_POINT('Ctrl Pts',(-29.9515223359549,14.127342135122,128.702904343381)) ;
#122305=CARTESIAN_POINT('Ctrl Pts',(-29.8925096530416,14.2954362012379,
128.49726452035)) ;
#122306=CARTESIAN_POINT('Ctrl Pts',(-29.8219114303992,14.400199046936,128.257970798247)) ;
#122307=CARTESIAN_POINT('Ctrl Pts',(-29.7447976913517,14.4351706373417,
127.999457902045)) ;
#122308=CARTESIAN_POINT('Ctrl Pts',(-29.6684583326803,14.3977719560938,
127.743498139774)) ;
#122309=CARTESIAN_POINT('Ctrl Pts',(-29.5978717537841,14.2904204320916,
127.504095055123)) ;
#122310=CARTESIAN_POINT('Ctrl Pts',(-29.5395109023276,14.1205426182846,
127.300429244723)) ;
#122311=CARTESIAN_POINT('Ctrl Pts',(-29.4983530336309,13.9015880180689,
127.147150529684)) ;
#122312=CARTESIAN_POINT('Ctrl Pts',(-29.4777158030966,13.6483197429669,
127.053786309688)) ;
#122313=CARTESIAN_POINT('Ctrl Pts',(-29.4800308791957,13.3774459783215,
127.027292014993)) ;
#122314=CARTESIAN_POINT('Ctrl Pts',(-29.5057826138513,13.1115163789139,
127.069470833923)) ;
#122315=CARTESIAN_POINT('Ctrl Pts',(-29.553761607172,12.867627711837,127.176556695985)) ;
#122316=CARTESIAN_POINT('Ctrl Pts',(-29.6214344601104,12.6630941323673,
127.341122773102)) ;
#122317=CARTESIAN_POINT('Ctrl Pts',(-29.7047886913497,12.5128296370691,
127.551436680502)) ;
#122318=CARTESIAN_POINT('Ctrl Pts',(-29.7983168331104,12.4280522080275,
127.791517147946)) ;
#122319=CARTESIAN_POINT('Ctrl Pts',(-29.896197969887,12.4147676790035,128.044288782186)) ;
#122320=CARTESIAN_POINT('Ctrl Pts',(-29.9916432988877,12.4732052495888,
128.290111005686)) ;
#122321=CARTESIAN_POINT('Ctrl Pts',(-30.0798394969363,12.6008830846757,
128.514423176177)) ;
#122322=CARTESIAN_POINT('Ctrl Pts',(-30.153418094144,12.7859101152191,128.69640859045)) ;
#122323=CARTESIAN_POINT('Ctrl Pts',(-30.2092050348681,13.0171550939707,
128.826255988633)) ;
#122324=CARTESIAN_POINT('Ctrl Pts',(-30.2434739775271,13.2774025189781,
128.893266135644)) ;
#122325=CARTESIAN_POINT('Ctrl Pts',(-30.2545103544402,13.5492093049786,
128.892265384779)) ;
#122326=CARTESIAN_POINT('Ctrl Pts',(-30.2422243054412,13.8101283643081,
128.823364688969)) ;
#122327=CARTESIAN_POINT('Ctrl Pts',(-30.2083754507383,14.0442617204232,
128.691385046736)) ;
#122328=CARTESIAN_POINT('Ctrl Pts',(-30.1554956679367,14.2348997538622,
128.503575628584)) ;
#122329=CARTESIAN_POINT('Ctrl Pts',(-30.0893154304115,14.3654883224984,
128.277320876037)) ;
#122330=CARTESIAN_POINT('Ctrl Pts',(-30.0140893274458,14.4297229265612,
128.02437201421)) ;
#122331=CARTESIAN_POINT('Ctrl Pts',(-29.9366945426251,14.421668005349,127.765225227294)) ;
#122332=CARTESIAN_POINT('Ctrl Pts',(-29.8627322861493,14.3417420843685,
127.515916221253)) ;
#122333=CARTESIAN_POINT('Ctrl Pts',(-29.7990172516701,14.1964291100303,
127.296728535392)) ;
#122334=CARTESIAN_POINT('Ctrl Pts',(-29.7503115001684,13.9955518397601,
127.121315751128)) ;
#122335=CARTESIAN_POINT('Ctrl Pts',(-29.7209679395557,13.7541464168563,
127.002530885163)) ;
#122336=CARTESIAN_POINT('Ctrl Pts',(-29.7138270012993,13.4873870374965,
126.948394752065)) ;
#122337=CARTESIAN_POINT('Ctrl Pts',(-29.7300210673021,13.2187118678006,
126.962770014111)) ;
#122338=CARTESIAN_POINT('Ctrl Pts',(-29.7693618809783,12.9622340205071,
127.04445153456)) ;
#122339=CARTESIAN_POINT('Ctrl Pts',(-29.8296161918263,12.7396654906289,
127.187330698386)) ;
#122340=CARTESIAN_POINT('Ctrl Pts',(-29.9070992084671,12.5663130117826,
127.380570436631)) ;
#122341=CARTESIAN_POINT('Ctrl Pts',(-29.9967702563037,12.4542929765583,
127.609512573754)) ;
#122342=CARTESIAN_POINT('Ctrl Pts',(-30.0940660663216,12.4113060992836,
127.860434811166)) ;
#122343=CARTESIAN_POINT('Ctrl Pts',(-30.1909321832857,12.4409729765678,
128.110447724348)) ;
#122344=CARTESIAN_POINT('Ctrl Pts',(-30.2827250654669,12.5408195809103,
128.345442109958)) ;
#122345=CARTESIAN_POINT('Ctrl Pts',(-30.3631110575611,12.7045177174677,
128.54705780663)) ;
#122346=CARTESIAN_POINT('Ctrl Pts',(-30.4266778642014,12.919412680773,128.69962285843)) ;
#122347=CARTESIAN_POINT('Ctrl Pts',(-30.4698068753402,13.1689179430447,
128.792656682487)) ;
#122348=CARTESIAN_POINT('Ctrl Pts',(-30.4904930950395,13.4397285825566,
128.819731723829)) ;
#122349=CARTESIAN_POINT('Ctrl Pts',(-30.4874907257796,13.7064270622518,
128.777980012696)) ;
#122350=CARTESIAN_POINT('Ctrl Pts',(-30.4620654317262,13.9538863073551,
128.670590863252)) ;
#122351=CARTESIAN_POINT('Ctrl Pts',(-30.4167476705665,14.163192773507,128.505145630859)) ;
#122352=CARTESIAN_POINT('Ctrl Pts',(-30.3548906755859,14.3205261321744,
128.291114365887)) ;
#122353=CARTESIAN_POINT('Ctrl Pts',(-30.2829346299508,14.4121066537417,
128.047974510391)) ;
#122354=CARTESIAN_POINT('Ctrl Pts',(-30.2054667933554,14.433704272446,127.788469415393)) ;
#122355=CARTESIAN_POINT('Ctrl Pts',(-30.1294973360627,14.3826278008681,
127.533437022415)) ;
#122356=CARTESIAN_POINT('Ctrl Pts',(-30.0609394463252,14.2628852203127,
127.300029416679)) ;
#122357=CARTESIAN_POINT('Ctrl Pts',(-30.0055020233255,14.0829261229302,
127.104952049683)) ;
#122358=CARTESIAN_POINT('Ctrl Pts',(-29.9678519682289,13.8556921301219,
126.961834528388)) ;
#122359=CARTESIAN_POINT('Ctrl Pts',(-29.9515006435671,13.5972598207812,
126.880912604436)) ;
#122360=CARTESIAN_POINT('Ctrl Pts',(-29.9581093878637,13.3277678231801,
126.867244122754)) ;
#122361=CARTESIAN_POINT('Ctrl Pts',(-29.9885236753733,13.061810881333,126.92268198126)) ;
#122362=CARTESIAN_POINT('Ctrl Pts',(-30.0401392420675,12.8260388711121,
127.040646354392)) ;
#122363=CARTESIAN_POINT('Ctrl Pts',(-30.1113480471282,12.6298695868286,
127.215398293609)) ;
#122364=CARTESIAN_POINT('Ctrl Pts',(-30.1968274118044,12.491768708706,127.432029083831)) ;
#122365=CARTESIAN_POINT('Ctrl Pts',(-30.2917304339287,12.4199839155212,
127.676085528742)) ;
#122366=CARTESIAN_POINT('Ctrl Pts',(-30.3895172732968,12.4203084391601,
127.928654142182)) ;
#122367=CARTESIAN_POINT('Ctrl Pts',(-30.4841396004474,12.492208510643,128.171981243385)) ;
#122368=CARTESIAN_POINT('Ctrl Pts',(-30.5697024940823,12.630997013847,128.388786123922)) ;
#122369=CARTESIAN_POINT('Ctrl Pts',(-30.6405627396724,12.8263312491105,
128.562679987083)) ;
#122370=CARTESIAN_POINT('Ctrl Pts',(-30.6926223743772,13.0651229525308,
128.681553834385)) ;
#122371=CARTESIAN_POINT('Ctrl Pts',(-30.7225260149649,13.3295669294852,
128.735723381487)) ;
#122372=CARTESIAN_POINT('Ctrl Pts',(-30.7290589510896,13.5989125314577,
128.72184499335)) ;
#122373=CARTESIAN_POINT('Ctrl Pts',(-30.7124997713408,13.8574711990645,
128.640276978673)) ;
#122374=CARTESIAN_POINT('Ctrl Pts',(-30.6748800157575,14.08370800358,128.497364451285)) ;
#122375=CARTESIAN_POINT('Ctrl Pts',(-30.6192581352089,14.2638192585231,
128.301674339225)) ;
#122376=CARTESIAN_POINT('Ctrl Pts',(-30.5506481335535,14.3831696043844,
128.068124805853)) ;
#122377=CARTESIAN_POINT('Ctrl Pts',(-30.4745251971265,14.4337176712718,
127.812585526878)) ;
#122378=CARTESIAN_POINT('Ctrl Pts',(-30.3974954804431,14.4120588565301,
127.554554597263)) ;
#122379=CARTESIAN_POINT('Ctrl Pts',(-30.3250685590978,14.3193772826324,
127.309789317507)) ;
#122380=CARTESIAN_POINT('Ctrl Pts',(-30.2637016994033,14.1628170776178,
127.097430559327)) ;
#122381=CARTESIAN_POINT('Ctrl Pts',(-30.2181498014506,13.9515916120412,
126.931029962997)) ;
#122382=CARTESIAN_POINT('Ctrl Pts',(-30.1929956511177,13.7055233139094,
126.824657543455)) ;
#122383=CARTESIAN_POINT('Ctrl Pts',(-30.1902289107925,13.4359481903885,
126.783236403317)) ;
#122384=CARTESIAN_POINT('Ctrl Pts',(-30.2107593001267,13.1690262561277,
126.810343623313)) ;
#122385=CARTESIAN_POINT('Ctrl Pts',(-30.2545482372846,12.9162728254293,
126.904850728262)) ;
#122386=CARTESIAN_POINT('Ctrl Pts',(-30.3178913728212,12.7036779683092,
127.057027568581)) ;
#122387=CARTESIAN_POINT('Ctrl Pts',(-30.3981222067462,12.5403117617381,
127.258247374178)) ;
#122388=CARTESIAN_POINT('Ctrl Pts',(-30.4903111236193,12.4404489557871,
127.494277250787)) ;
#122389=CARTESIAN_POINT('Ctrl Pts',(-30.5871336885702,12.4114485631191,
127.744183561599)) ;
#122390=CARTESIAN_POINT('Ctrl Pts',(-30.6840345143622,12.4544846447878,
127.994082811986)) ;
#122391=CARTESIAN_POINT('Ctrl Pts',(-30.7741275020112,12.5672617831098,
128.224093354097)) ;
#122392=CARTESIAN_POINT('Ctrl Pts',(-30.8516515642429,12.741774518216,128.417359705438)) ;
#122393=CARTESIAN_POINT('Ctrl Pts',(-30.9114063327502,12.9633751206612,
128.558968956766)) ;
#122394=CARTESIAN_POINT('Ctrl Pts',(-30.9507706166524,13.2203112306522,
128.64066766554)) ;
#122395=CARTESIAN_POINT('Ctrl Pts',(-30.9667741641491,13.4905144393576,
128.654304855092)) ;
#122396=CARTESIAN_POINT('Ctrl Pts',(-30.9595000465809,13.7550217254887,
128.60004785508)) ;
#122397=CARTESIAN_POINT('Ctrl Pts',(-30.9300640821417,13.9967496932403,
128.480932627841)) ;
#122398=CARTESIAN_POINT('Ctrl Pts',(-30.88124976571,14.1974243252069,128.305200960729)) ;
#122399=CARTESIAN_POINT('Ctrl Pts',(-30.8173009837137,14.3425140414095,
128.0852559147)) ;
#122400=CARTESIAN_POINT('Ctrl Pts',(-30.7437385247045,14.4218016114581,
127.837311335821)) ;
#122401=CARTESIAN_POINT('Ctrl Pts',(-30.6657606026371,14.4294553389326,
127.576204351649)) ;
#122402=CARTESIAN_POINT('Ctrl Pts',(-30.5911196828898,14.3652617891387,
127.325217316403)) ;
#122403=CARTESIAN_POINT('Ctrl Pts',(-30.5245394207173,14.2335996006041,
127.097570146183)) ;
#122404=CARTESIAN_POINT('Ctrl Pts',(-30.4720096954179,14.0430657817291,
126.910897477969)) ;
#122405=CARTESIAN_POINT('Ctrl Pts',(-30.4382095748234,13.8093137336756,
126.779115500136)) ;
#122406=CARTESIAN_POINT('Ctrl Pts',(-30.4260630552414,13.5459138184761,
126.710330077877)) ;
#122407=CARTESIAN_POINT('Ctrl Pts',(-30.4371827081375,13.2769102523372,
126.709919831468)) ;
#122408=CARTESIAN_POINT('Ctrl Pts',(-30.4715571173939,13.0160045287208,
126.777143004842)) ;
#122409=CARTESIAN_POINT('Ctrl Pts',(-30.5273885697427,12.7850160477838,
126.907146547319)) ;
#122410=CARTESIAN_POINT('Ctrl Pts',(-30.6015916024625,12.5991695463159,
127.09073027164)) ;
#122411=CARTESIAN_POINT('Ctrl Pts',(-30.689509572293,12.4727066402134,127.314381139998)) ;
#122412=CARTESIAN_POINT('Ctrl Pts',(-30.78498211656,12.414634000185,127.56027701158)) ;
#122413=CARTESIAN_POINT('Ctrl Pts',(-30.8827162241977,12.4282724908794,
127.812670727123)) ;
#122414=CARTESIAN_POINT('Ctrl Pts',(-30.9764215447378,12.5136822539145,
128.053186598358)) ;
#122415=CARTESIAN_POINT('Ctrl Pts',(-31.0595380623793,12.6640314349918,
128.262872652563)) ;
#122416=CARTESIAN_POINT('Ctrl Pts',(-31.1272621654378,12.8694014847424,
128.427501230652)) ;
#122417=CARTESIAN_POINT('Ctrl Pts',(-31.1749753148501,13.11284739186,128.533901712675)) ;
#122418=CARTESIAN_POINT('Ctrl Pts',(-31.2006444289191,13.3794714169119,
128.575760031987)) ;
#122419=CARTESIAN_POINT('Ctrl Pts',(-31.2027867558287,13.649387589438,128.548872446442)) ;
#122420=CARTESIAN_POINT('Ctrl Pts',(-31.182112101246,13.9027716993511,128.455382730857)) ;
#122421=CARTESIAN_POINT('Ctrl Pts',(-31.1405097423725,14.1226004021729,
128.300604633976)) ;
#122422=CARTESIAN_POINT('Ctrl Pts',(-31.0824924132861,14.2907614939367,
128.098200056456)) ;
#122423=CARTESIAN_POINT('Ctrl Pts',(-31.0115394554541,14.3985142695992,
127.857562086865)) ;
#122424=CARTESIAN_POINT('Ctrl Pts',(-30.9350167672811,14.4350393249369,
127.60100492444)) ;
#122425=CARTESIAN_POINT('Ctrl Pts',(-30.8584423775873,14.4000355942845,
127.344298627008)) ;
#122426=CARTESIAN_POINT('Ctrl Pts',(-30.7873589741607,14.294019259171,127.103326699404)) ;
#122427=CARTESIAN_POINT('Ctrl Pts',(-30.7288526610613,14.1264036787102,
126.899375100568)) ;
#122428=CARTESIAN_POINT('Ctrl Pts',(-30.687031834005,13.908713601209,126.744138494649)) ;
#122429=CARTESIAN_POINT('Ctrl Pts',(-30.665740603527,13.6545233253026,126.648660834423)) ;
#122430=CARTESIAN_POINT('Ctrl Pts',(-30.6674256184851,13.385850090519,126.620576704158)) ;
#122431=CARTESIAN_POINT('Ctrl Pts',(-30.6924732658782,13.1190055030057,
126.660631420444)) ;
#122432=CARTESIAN_POINT('Ctrl Pts',(-30.739931250503,12.8738785083339,126.766149985998)) ;
#122433=CARTESIAN_POINT('Ctrl Pts',(-30.8072994517156,12.6676053408392,
126.929745605886)) ;
#122434=CARTESIAN_POINT('Ctrl Pts',(-30.8902244330813,12.5160770794409,
127.138850466977)) ;
#122435=CARTESIAN_POINT('Ctrl Pts',(-30.9830990181765,12.429744459131,127.377173832304)) ;
#122436=CARTESIAN_POINT('Ctrl Pts',(-31.0808346305105,12.4139325867349,
127.629558482749)) ;
#122437=CARTESIAN_POINT('Ctrl Pts',(-31.1769815706491,12.470818666654,127.877230342766)) ;
#122438=CARTESIAN_POINT('Ctrl Pts',(-31.2647445655939,12.5954481980338,
128.100568864441)) ;
#122439=CARTESIAN_POINT('Ctrl Pts',(-31.3392856003309,12.7795463836638,
128.285188591065)) ;
#122440=CARTESIAN_POINT('Ctrl Pts',(-31.3957801377511,13.0105019678005,
128.417005984796)) ;
#122441=CARTESIAN_POINT('Ctrl Pts',(-31.4306543783806,13.2704660588973,
128.485753447239)) ;
#122442=CARTESIAN_POINT('Ctrl Pts',(-31.442287999366,13.5415026123175,128.48658603552)) ;
#122443=CARTESIAN_POINT('Ctrl Pts',(-31.4307033779827,13.8030871080867,
128.419727155045)) ;
#122444=CARTESIAN_POINT('Ctrl Pts',(-31.3971754129151,14.0389748553007,
128.288544481416)) ;
#122445=CARTESIAN_POINT('Ctrl Pts',(-31.3454184265653,14.2290324993106,
128.104404269474)) ;
#122446=CARTESIAN_POINT('Ctrl Pts',(-31.2790627226709,14.3629001779689,
127.877345831259)) ;
#122447=CARTESIAN_POINT('Ctrl Pts',(-31.2041424100767,14.428830285179,127.625371610393)) ;
#122448=CARTESIAN_POINT('Ctrl Pts',(-31.1265767826112,14.4228365042112,
127.365651786092)) ;
#122449=CARTESIAN_POINT('Ctrl Pts',(-31.052679859191,14.3452101955046,127.116656966355)) ;
#122450=CARTESIAN_POINT('Ctrl Pts',(-30.9884269255255,14.2014202619827,
126.895813741383)) ;
#122451=CARTESIAN_POINT('Ctrl Pts',(-30.9392882282485,14.0021641250436,
126.719179096165)) ;
#122452=CARTESIAN_POINT('Ctrl Pts',(-30.9093211350562,13.7617530552763,
126.598570707612)) ;
#122453=CARTESIAN_POINT('Ctrl Pts',(-30.9014747573705,13.4956079562807,
126.542397455449)) ;
#122454=CARTESIAN_POINT('Ctrl Pts',(-30.9170318360537,13.2262845260177,
126.55484606842)) ;
#122455=CARTESIAN_POINT('Ctrl Pts',(-30.9555778404963,12.9698876491267,
126.634313026387)) ;
#122456=CARTESIAN_POINT('Ctrl Pts',(-31.0153287793161,12.7457363777613,
126.77566667277)) ;
#122457=CARTESIAN_POINT('Ctrl Pts',(-31.0921782746939,12.5708017324576,
126.967118677833)) ;
#122458=CARTESIAN_POINT('Ctrl Pts',(-31.1824180985943,12.4561497047602,
127.197416346179)) ;
#122459=CARTESIAN_POINT('Ctrl Pts',(-31.278554206561,12.4116404870753,127.445319108056)) ;
#122460=CARTESIAN_POINT('Ctrl Pts',(-31.3762681488149,12.4391729366694,
127.697540638099)) ;
#122461=CARTESIAN_POINT('Ctrl Pts',(-31.4680268263453,12.53717976609,127.932527251887)) ;
#122462=CARTESIAN_POINT('Ctrl Pts',(-31.5485854179887,12.6985743476714,
128.13474547452)) ;
#122463=CARTESIAN_POINT('Ctrl Pts',(-31.6127577477514,12.9117741339943,
128.289108577839)) ;
#122464=CARTESIAN_POINT('Ctrl Pts',(-31.6567710961282,13.1624013119324,
128.384477088599)) ;
#122465=CARTESIAN_POINT('Ctrl Pts',(-31.6779406587271,13.4305279124855,
128.413268749148)) ;
#122466=CARTESIAN_POINT('Ctrl Pts',(-31.6757209320686,13.6988963529668,
128.373634329705)) ;
#122467=CARTESIAN_POINT('Ctrl Pts',(-31.6508856851263,13.9472005440968,
128.267972545371)) ;
#122468=CARTESIAN_POINT('Ctrl Pts',(-31.6060004910728,14.1580510718868,
128.103736864114)) ;
#122469=CARTESIAN_POINT('Ctrl Pts',(-31.5448207362963,14.3165352463583,
127.891828892358)) ;
#122470=CARTESIAN_POINT('Ctrl Pts',(-31.4727358243366,14.4105996736352,
127.648139770064)) ;
#122471=CARTESIAN_POINT('Ctrl Pts',(-31.3955355088999,14.4340684642594,
127.389513002923)) ;
#122472=CARTESIAN_POINT('Ctrl Pts',(-31.3193139953007,14.3850543763753,
127.133688710295)) ;
#122473=CARTESIAN_POINT('Ctrl Pts',(-31.2504690412177,14.2669952008499,
126.899435868025)) ;
#122474=CARTESIAN_POINT('Ctrl Pts',(-31.1947324047151,14.0891153904615,
126.703574539752)) ;
#122475=CARTESIAN_POINT('Ctrl Pts',(-31.1564387248963,13.862922820575,126.558547490818)) ;
#122476=CARTESIAN_POINT('Ctrl Pts',(-31.1394099641997,13.6044942948714,
126.47557023365)) ;
#122477=CARTESIAN_POINT('Ctrl Pts',(-31.1454472203925,13.3352194719608,
126.460244590561)) ;
#122478=CARTESIAN_POINT('Ctrl Pts',(-31.1748811284131,13.0705828677346,
126.513054618359)) ;
#122479=CARTESIAN_POINT('Ctrl Pts',(-31.2262659374063,12.8316691546943,
126.630062656991)) ;
#122480=CARTESIAN_POINT('Ctrl Pts',(-31.2971356400406,12.6342705619082,
126.803808781442)) ;
#122481=CARTESIAN_POINT('Ctrl Pts',(-31.3819483703303,12.4949547618174,
127.018616528483)) ;
#122482=CARTESIAN_POINT('Ctrl Pts',(-31.4766833238412,12.4210676007864,
127.262174213226)) ;
#122483=CARTESIAN_POINT('Ctrl Pts',(-31.5743436337679,12.4192534953992,
127.514414718138)) ;
#122484=CARTESIAN_POINT('Ctrl Pts',(-31.6693177267353,12.4890551433301,
127.758717643024)) ;
#122485=CARTESIAN_POINT('Ctrl Pts',(-31.7555447049053,12.6269266116115,
127.977315822043)) ;
#122486=CARTESIAN_POINT('Ctrl Pts',(-31.8264211692197,12.8196496525906,
128.15146867102)) ;
#122487=CARTESIAN_POINT('Ctrl Pts',(-31.8792655119042,13.0580837190484,
128.272530897348)) ;
#122488=CARTESIAN_POINT('Ctrl Pts',(-31.9097495081077,13.3214663424209,
128.328476209486)) ;
#122489=CARTESIAN_POINT('Ctrl Pts',(-31.9169670179251,13.5912988654113,
128.316540654689)) ;
#122490=CARTESIAN_POINT('Ctrl Pts',(-31.9011691067475,13.8497220068298,
128.237308488014)) ;
#122491=CARTESIAN_POINT('Ctrl Pts',(-31.8637971767436,14.0789423187272,
128.0948445745)) ;
#122492=CARTESIAN_POINT('Ctrl Pts',(-31.8086550954363,14.259760152893,127.900645843771)) ;
#122493=CARTESIAN_POINT('Ctrl Pts',(-31.7405929166887,14.3805241864287,
127.668810176457)) ;
#122494=CARTESIAN_POINT('Ctrl Pts',(-31.6647024826629,14.4333051091104,
127.413993047517)) ;
#122495=CARTESIAN_POINT('Ctrl Pts',(-31.5873081578645,14.4135763051709,
127.154757112012)) ;
#122496=CARTESIAN_POINT('Ctrl Pts',(-31.5147598783728,14.3230159686918,
126.909698801431)) ;
#122497=CARTESIAN_POINT('Ctrl Pts',(-31.4527958504163,14.1669880508,126.695418871326)) ;
#122498=CARTESIAN_POINT('Ctrl Pts',(-31.4072827436831,13.960185490464,126.529605369715)) ;
#122499=CARTESIAN_POINT('Ctrl Pts',(-31.381143378296,13.7121979598798,126.419953822516)) ;
#122500=CARTESIAN_POINT('Ctrl Pts',(-31.3777158961212,13.445325428157,126.376915063972)) ;
#122501=CARTESIAN_POINT('Ctrl Pts',(-31.397745527697,13.1756579311624,126.402235763468)) ;
#122502=CARTESIAN_POINT('Ctrl Pts',(-31.4404084183114,12.9248371147139,
126.493828264377)) ;
#122503=CARTESIAN_POINT('Ctrl Pts',(-31.5036578664833,12.7087904234027,
126.645429976648)) ;
#122504=CARTESIAN_POINT('Ctrl Pts',(-31.5834548863671,12.5441839986788,
126.845425287598)) ;
#122505=CARTESIAN_POINT('Ctrl Pts',(-31.6753525848934,12.4422953627895,
127.08061008035)) ;
#122506=CARTESIAN_POINT('Ctrl Pts',(-31.7723120116357,12.4112745918663,
127.330847845115)) ;
#122507=CARTESIAN_POINT('Ctrl Pts',(-31.8691208728923,12.4523611263307,
127.580540139706)) ;
#122508=CARTESIAN_POINT('Ctrl Pts',(-31.9592601337174,12.5627156351226,
127.810782853242)) ;
#122509=CARTESIAN_POINT('Ctrl Pts',(-32.0375124865879,12.7362032520556,
128.006054251628)) ;
#122510=CARTESIAN_POINT('Ctrl Pts',(-32.0976971478895,12.9562237292826,
128.148985066523)) ;
#122511=CARTESIAN_POINT('Ctrl Pts',(-32.13773953768,13.2127632851082,128.232621281861)) ;
#122512=CARTESIAN_POINT('Ctrl Pts',(-32.1543946447233,13.4814740425718,
128.248327464853)) ;
#122513=CARTESIAN_POINT('Ctrl Pts',(-32.1478604320586,13.7476021325284,
128.196087364076)) ;
#122514=CARTESIAN_POINT('Ctrl Pts',(-32.1188973813439,13.9907503270219,
128.078278588462)) ;
#122515=CARTESIAN_POINT('Ctrl Pts',(-32.0707073756381,14.1921269255571,
127.904467261036)) ;
#122516=CARTESIAN_POINT('Ctrl Pts',(-32.0072133952261,14.3392030791961,
127.685872025095)) ;
#122517=CARTESIAN_POINT('Ctrl Pts',(-31.9332416636767,14.4207500388282,
127.436469066278)) ;
#122518=CARTESIAN_POINT('Ctrl Pts',(-31.8560118722166,14.4302362494743,
127.177863683382)) ;
#122519=CARTESIAN_POINT('Ctrl Pts',(-31.7807999346763,14.3680282355215,
126.925031033499)) ;
#122520=CARTESIAN_POINT('Ctrl Pts',(-31.7138116605628,14.2375542878188,
126.69612628114)) ;
#122521=CARTESIAN_POINT('Ctrl Pts',(-31.6609816023683,14.0487158820881,
126.50864330256)) ;
#122522=CARTESIAN_POINT('Ctrl Pts',(-31.6267397291478,13.8167882878437,
126.375682453872)) ;
#122523=CARTESIAN_POINT('Ctrl Pts',(-31.6138694456944,13.5548283790035,
126.304885636777)) ;
#122524=CARTESIAN_POINT('Ctrl Pts',(-31.6242959406042,13.2844749263172,
126.302288767915)) ;
#122525=CARTESIAN_POINT('Ctrl Pts',(-31.6581468262068,13.0226682928204,
126.367933605866)) ;
#122526=CARTESIAN_POINT('Ctrl Pts',(-31.7132570926775,12.7913019037466,
126.495925056773)) ;
#122527=CARTESIAN_POINT('Ctrl Pts',(-31.7868846932829,12.6040506886806,
126.677862167633)) ;
#122528=CARTESIAN_POINT('Ctrl Pts',(-31.8744032872355,12.4756113608574,
126.900365413074)) ;
#122529=CARTESIAN_POINT('Ctrl Pts',(-31.9700299165858,12.4152434806169,
127.14660580532)) ;
#122530=CARTESIAN_POINT('Ctrl Pts',(-32.067726874144,12.4269403893897,127.398912991664)) ;
#122531=CARTESIAN_POINT('Ctrl Pts',(-32.1614230211097,12.5099953392157,
127.639486026072)) ;
#122532=CARTESIAN_POINT('Ctrl Pts',(-32.2450419055353,12.6587329493789,
127.850591786388)) ;
#122533=CARTESIAN_POINT('Ctrl Pts',(-32.3131064085061,12.8618952615055,
128.016327167337)) ;
#122534=CARTESIAN_POINT('Ctrl Pts',(-32.3617247556363,13.105407033224,128.125223389019)) ;
#122535=CARTESIAN_POINT('Ctrl Pts',(-32.3880370855062,13.372198744835,128.168900378835)) ;
#122536=CARTESIAN_POINT('Ctrl Pts',(-32.3908241094825,13.6415134475053,
128.143990115677)) ;
#122537=CARTESIAN_POINT('Ctrl Pts',(-32.3708584046227,13.8954057522976,
128.052605580229)) ;
#122538=CARTESIAN_POINT('Ctrl Pts',(-32.3297866697098,14.1169004817223,
127.899329717684)) ;
#122539=CARTESIAN_POINT('Ctrl Pts',(-32.2720357073091,14.2868623314226,
127.697634443906)) ;
#122540=CARTESIAN_POINT('Ctrl Pts',(-32.2018019882442,14.3960130363954,
127.45930091582)) ;
#122541=CARTESIAN_POINT('Ctrl Pts',(-32.1250722199058,14.4351149221843,
127.202000748098)) ;
#122542=CARTESIAN_POINT('Ctrl Pts',(-32.0482999804116,14.4019052033915,
126.944665606573)) ;
#122543=CARTESIAN_POINT('Ctrl Pts',(-31.9771926809482,14.2983009205314,
126.70374147036)) ;
#122544=CARTESIAN_POINT('Ctrl Pts',(-31.9180230665024,14.1317969233753,
126.497728005608)) ;
#122545=CARTESIAN_POINT('Ctrl Pts',(-31.8757597160519,13.9153433735369,
126.341222269938)) ;
#122546=CARTESIAN_POINT('Ctrl Pts',(-31.8538948818607,13.6633971657659,
126.244251306656)) ;
#122547=CARTESIAN_POINT('Ctrl Pts',(-31.8547561893373,13.3943409356125,
126.213683501552)) ;
#122548=CARTESIAN_POINT('Ctrl Pts',(-31.879305119298,13.125759479102,126.252108551624)) ;
#122549=CARTESIAN_POINT('Ctrl Pts',(-31.9260462665466,12.8806964502858,
126.355648570145)) ;
#122550=CARTESIAN_POINT('Ctrl Pts',(-31.992649963062,12.6734733504626,126.517098736783)) ;
#122551=CARTESIAN_POINT('Ctrl Pts',(-32.0753331596735,12.5195857964099,
126.725421864695)) ;
#122552=CARTESIAN_POINT('Ctrl Pts',(-32.1684606176005,12.431093262312,126.964324569044)) ;
#122553=CARTESIAN_POINT('Ctrl Pts',(-32.2656426943434,12.4134132732782,
127.215267971027)) ;
#122554=CARTESIAN_POINT('Ctrl Pts',(-32.3620515668434,12.4681188865971,
127.463663966544)) ;
#122555=CARTESIAN_POINT('Ctrl Pts',(-32.4501306508827,12.5909169952097,
127.687925854587)) ;
#122556=CARTESIAN_POINT('Ctrl Pts',(-32.5251176857849,12.7734489728906,
127.873850465839)) ;
#122557=CARTESIAN_POINT('Ctrl Pts',(-32.5821383880763,13.0028155052197,
128.007264413582)) ;
#122558=CARTESIAN_POINT('Ctrl Pts',(-32.6177275928939,13.2626813874081,
128.078031538423)) ;
#122559=CARTESIAN_POINT('Ctrl Pts',(-32.6300773966959,13.5323092973528,
128.081128075608)) ;
#122560=CARTESIAN_POINT('Ctrl Pts',(-32.6191171645962,13.7963544405994,
128.015846971038)) ;
#122561=CARTESIAN_POINT('Ctrl Pts',(-32.5862481873824,14.0324258924939,
127.886706170116)) ;
#122562=CARTESIAN_POINT('Ctrl Pts',(-32.5349051847159,14.2243212394665,
127.703714987948)) ;
#122563=CARTESIAN_POINT('Ctrl Pts',(-32.4690664082192,14.3597397385498,
127.478255566514)) ;
#122564=CARTESIAN_POINT('Ctrl Pts',(-32.3940630824478,14.4280132276383,
127.225921237608)) ;
#122565=CARTESIAN_POINT('Ctrl Pts',(-32.3165287082417,14.4240026774031,
126.966315839368)) ;
#122566=CARTESIAN_POINT('Ctrl Pts',(-32.2423883005505,14.3482148360276,
126.716578494938)) ;
#122567=CARTESIAN_POINT('Ctrl Pts',(-32.1779893014855,14.2066838492508,
126.49541837889)) ;
#122568=CARTESIAN_POINT('Ctrl Pts',(-32.1281752856826,14.0084843901798,
126.316727480174)) ;
#122569=CARTESIAN_POINT('Ctrl Pts',(-32.0975903701439,13.7679162492584,
126.194182548856)) ;
#122570=CARTESIAN_POINT('Ctrl Pts',(-32.0891787939898,13.5034892563332,
126.13652430323)) ;
#122571=CARTESIAN_POINT('Ctrl Pts',(-32.1040626123099,13.2335993396584,
126.146949017154)) ;
#122572=CARTESIAN_POINT('Ctrl Pts',(-32.1420329442231,12.9764075734903,
126.224715938811)) ;
#122573=CARTESIAN_POINT('Ctrl Pts',(-32.2013713025453,12.7508791959946,
126.364815084693)) ;
#122574=CARTESIAN_POINT('Ctrl Pts',(-32.2775403681359,12.5752390295055,
126.554404335388)) ;
#122575=CARTESIAN_POINT('Ctrl Pts',(-32.3669984352675,12.4588914827239,
126.782580215258)) ;
#122576=CARTESIAN_POINT('Ctrl Pts',(-32.4635757710145,12.4118138337187,
127.031576925067)) ;
#122577=CARTESIAN_POINT('Ctrl Pts',(-32.5613228642034,12.4374481802068,
127.283905827195)) ;
#122578=CARTESIAN_POINT('Ctrl Pts',(-32.6533055517079,12.5333386761198,
127.519560385033)) ;
#122579=CARTESIAN_POINT('Ctrl Pts',(-32.7345801972341,12.6939673682458,
127.72372104471)) ;
#122580=CARTESIAN_POINT('Ctrl Pts',(-32.7989235968999,12.905003236762,127.878741838257)) ;
#122581=CARTESIAN_POINT('Ctrl Pts',(-32.8436689907595,13.1551454221065,
127.976196286225)) ;
#122582=CARTESIAN_POINT('Ctrl Pts',(-32.8581698291871,13.3338159430811,
127.996517118284)) ;
#122583=CARTESIAN_POINT('Ctrl Pts',(-32.8615556099148,13.423122164697,127.995387104394)) ;
#122584=CARTESIAN_POINT('Ctrl Pts',(-11.4238141454945,13.1551399285885,
133.176569308009)) ;
#122585=CARTESIAN_POINT('Ctrl Pts',(-11.4245530443044,13.1489709760559,
133.177996857566)) ;
#122586=CARTESIAN_POINT('Ctrl Pts',(-11.4366069089063,13.0505875198745,
133.201526775898)) ;
#122587=CARTESIAN_POINT('Ctrl Pts',(-11.4693539332526,12.8648901900081,
133.274214160344)) ;
#122588=CARTESIAN_POINT('Ctrl Pts',(-11.5380924228032,12.637899642759,133.441994108163)) ;
#122589=CARTESIAN_POINT('Ctrl Pts',(-11.6243468898402,12.4661938429578,
133.66085914641)) ;
#122590=CARTESIAN_POINT('Ctrl Pts',(-11.723176143549,12.3629468652583,133.9162908092)) ;
#122591=CARTESIAN_POINT('Ctrl Pts',(-11.8266263732223,12.3360866593215,
134.185565771878)) ;
#122592=CARTESIAN_POINT('Ctrl Pts',(-11.9299575986037,12.3868468010151,
134.454196270192)) ;
#122593=CARTESIAN_POINT('Ctrl Pts',(-12.0251860635232,12.5118616654237,
134.699290577349)) ;
#122594=CARTESIAN_POINT('Ctrl Pts',(-12.1067707542268,12.7022377085439,
134.904476363702)) ;
#122595=CARTESIAN_POINT('Ctrl Pts',(-12.1693898147792,12.9442212424904,
135.054278991416)) ;
#122596=CARTESIAN_POINT('Ctrl Pts',(-12.2093211316432,13.2203923683254,
135.137814270087)) ;
#122597=CARTESIAN_POINT('Ctrl Pts',(-12.2245264343576,13.5109002567873,
135.149142252338)) ;
#122598=CARTESIAN_POINT('Ctrl Pts',(-12.2144214456397,13.7967279051741,
135.086333358288)) ;
#122599=CARTESIAN_POINT('Ctrl Pts',(-12.1808130028206,14.053163616969,134.955192972495)) ;
#122600=CARTESIAN_POINT('Ctrl Pts',(-12.1265747443939,14.2659162320927,
134.763620195857)) ;
#122601=CARTESIAN_POINT('Ctrl Pts',(-12.0563659530723,14.4182156131257,
134.525407960618)) ;
#122602=CARTESIAN_POINT('Ctrl Pts',(-11.9757170636332,14.4993926376335,
134.256600011119)) ;
#122603=CARTESIAN_POINT('Ctrl Pts',(-11.8915786962281,14.5030673759949,
133.977690925007)) ;
#122604=CARTESIAN_POINT('Ctrl Pts',(-11.8106152149464,14.4296657361334,
133.708106117249)) ;
#122605=CARTESIAN_POINT('Ctrl Pts',(-11.7391300458456,14.2842404294125,
133.466176489072)) ;
#122606=CARTESIAN_POINT('Ctrl Pts',(-11.6829581874867,14.0768884033213,
133.268933114529)) ;
#122607=CARTESIAN_POINT('Ctrl Pts',(-11.646996920623,13.8219373708246,133.130656743182)) ;
#122608=CARTESIAN_POINT('Ctrl Pts',(-11.6346497120723,13.5404395793698,
133.061608552357)) ;
#122609=CARTESIAN_POINT('Ctrl Pts',(-11.6472238284623,13.2491901831122,
133.065198744336)) ;
#122610=CARTESIAN_POINT('Ctrl Pts',(-11.6849339883728,12.969918720115,133.142151589187)) ;
#122611=CARTESIAN_POINT('Ctrl Pts',(-11.7452470370939,12.7245501655325,
133.285329855241)) ;
#122612=CARTESIAN_POINT('Ctrl Pts',(-11.8252651009664,12.5279693790049,
133.485884901424)) ;
#122613=CARTESIAN_POINT('Ctrl Pts',(-11.9193252668049,12.3961376577074,
133.727590480155)) ;
#122614=CARTESIAN_POINT('Ctrl Pts',(-12.0221825717366,12.3376103607184,
133.994834780915)) ;
#122615=CARTESIAN_POINT('Ctrl Pts',(-12.1260592524752,12.3569098768634,
134.265282641821)) ;
#122616=CARTESIAN_POINT('Ctrl Pts',(-12.2255494729972,12.4527690637887,
134.522706406723)) ;
#122617=CARTESIAN_POINT('Ctrl Pts',(-12.3132365332066,12.6179594101214,
134.745773282964)) ;
#122618=CARTESIAN_POINT('Ctrl Pts',(-12.3840649431859,12.8405880896203,
134.919582179066)) ;
#122619=CARTESIAN_POINT('Ctrl Pts',(-12.4337419164154,13.1065246819692,
135.03142287103)) ;
#122620=CARTESIAN_POINT('Ctrl Pts',(-12.4589118501879,13.3925179969382,
135.071991071504)) ;
#122621=CARTESIAN_POINT('Ctrl Pts',(-12.4591401291713,13.6819916806813,
135.039543536461)) ;
#122622=CARTESIAN_POINT('Ctrl Pts',(-12.4346814882847,13.953724245336,134.934877287873)) ;
#122623=CARTESIAN_POINT('Ctrl Pts',(-12.388273358954,14.1863734270825,134.7662188792)) ;
#122624=CARTESIAN_POINT('Ctrl Pts',(-12.3240143345099,14.3643807952629,
134.54544367418)) ;
#122625=CARTESIAN_POINT('Ctrl Pts',(-12.2470026289218,14.4754559836596,
134.287355923251)) ;
#122626=CARTESIAN_POINT('Ctrl Pts',(-12.1633433065906,14.5110246745496,
134.009759570375)) ;
#122627=CARTESIAN_POINT('Ctrl Pts',(-12.0803955015974,14.468706357864,133.73440535818)) ;
#122628=CARTESIAN_POINT('Ctrl Pts',(-12.0040990392821,14.3514018733064,
133.478353554825)) ;
#122629=CARTESIAN_POINT('Ctrl Pts',(-11.9410368381369,14.1671964526519,
133.260957267519)) ;
#122630=CARTESIAN_POINT('Ctrl Pts',(-11.8965833260819,13.9308607646815,
133.098080106287)) ;
#122631=CARTESIAN_POINT('Ctrl Pts',(-11.8742320407181,13.6570089391064,
132.999605731374)) ;
#122632=CARTESIAN_POINT('Ctrl Pts',(-11.8766523771408,13.3664658768335,
132.973516684588)) ;
#122633=CARTESIAN_POINT('Ctrl Pts',(-11.9042552122956,13.0805680543038,
133.021054045171)) ;
#122634=CARTESIAN_POINT('Ctrl Pts',(-11.9557279014714,12.8190538509803,
133.138321033065)) ;
#122635=CARTESIAN_POINT('Ctrl Pts',(-12.0286271711589,12.599933753752,133.318014227644)) ;
#122636=CARTESIAN_POINT('Ctrl Pts',(-12.1172930726756,12.4413956885076,
133.544067361959)) ;
#122637=CARTESIAN_POINT('Ctrl Pts',(-12.2173395667587,12.3520377966892,
133.803159801022)) ;
#122638=CARTESIAN_POINT('Ctrl Pts',(-12.3217048099071,12.3397344016033,
134.074918582379)) ;
#122639=CARTESIAN_POINT('Ctrl Pts',(-12.4237285580169,12.4049383820741,
134.339842915822)) ;
#122640=CARTESIAN_POINT('Ctrl Pts',(-12.5168448241173,12.5429636135127,
134.57875667178)) ;
#122641=CARTESIAN_POINT('Ctrl Pts',(-12.5952694191645,12.744355559365,134.774694138797)) ;
#122642=CARTESIAN_POINT('Ctrl Pts',(-12.6538589035849,12.99435234836,134.912710643206)) ;
#122643=CARTESIAN_POINT('Ctrl Pts',(-12.6891834098298,13.2741649900779,
134.982863751975)) ;
#122644=CARTESIAN_POINT('Ctrl Pts',(-12.6996678027026,13.5657204845938,
134.980326914716)) ;
#122645=CARTESIAN_POINT('Ctrl Pts',(-12.6849427514785,13.8474317542271,
134.904091993754)) ;
#122646=CARTESIAN_POINT('Ctrl Pts',(-12.6471924840568,14.0971651338937,
134.760804466809)) ;
#122647=CARTESIAN_POINT('Ctrl Pts',(-12.5893357951143,14.300212406185,134.558553497018)) ;
#122648=CARTESIAN_POINT('Ctrl Pts',(-12.5166162325577,14.439451037695,134.312982315221)) ;
#122649=CARTESIAN_POINT('Ctrl Pts',(-12.4353628774632,14.5058688377535,
134.042653457514)) ;
#122650=CARTESIAN_POINT('Ctrl Pts',(-12.35110971528,14.4952594512815,133.763340940985)) ;
#122651=CARTESIAN_POINT('Ctrl Pts',(-12.2710628646113,14.4071576201155,
133.496266914171)) ;
#122652=CARTESIAN_POINT('Ctrl Pts',(-12.2021338287001,14.2488069359853,
133.261802498077)) ;
#122653=CARTESIAN_POINT('Ctrl Pts',(-12.1497382582167,14.0323324822322,
133.075749850883)) ;
#122654=CARTESIAN_POINT('Ctrl Pts',(-12.1179861315855,13.7715184536488,
132.949872907299)) ;
#122655=CARTESIAN_POINT('Ctrl Pts',(-12.1101419823041,13.4849967549257,
132.893761615134)) ;
#122656=CARTESIAN_POINT('Ctrl Pts',(-12.1277484366407,13.1936953531143,
132.911952789586)) ;
#122657=CARTESIAN_POINT('Ctrl Pts',(-12.1695498192332,12.9217410379526,
133.001184961085)) ;
#122658=CARTESIAN_POINT('Ctrl Pts',(-12.2341785842338,12.6826992816898,
133.156739191655)) ;
#122659=CARTESIAN_POINT('Ctrl Pts',(-12.3173687753878,12.4976839055064,
133.366582282212)) ;
#122660=CARTESIAN_POINT('Ctrl Pts',(-12.4131346667197,12.37947113767,133.613382407111)) ;
#122661=CARTESIAN_POINT('Ctrl Pts',(-12.5169846737337,12.3351744205894,
133.883477168164)) ;
#122662=CARTESIAN_POINT('Ctrl Pts',(-12.620799301784,12.3695012767601,134.153620745015)) ;
#122663=CARTESIAN_POINT('Ctrl Pts',(-12.718006444483,12.4786183713965,134.404573343174)) ;
#122664=CARTESIAN_POINT('Ctrl Pts',(-12.8030921061426,12.6556201650726,
134.619996403116)) ;
#122665=CARTESIAN_POINT('Ctrl Pts',(-12.8703633587299,12.8885376927875,
134.783284046582)) ;
#122666=CARTESIAN_POINT('Ctrl Pts',(-12.9153284854686,13.1578672301346,
134.881649635031)) ;
#122667=CARTESIAN_POINT('Ctrl Pts',(-12.9360932774699,13.4488181207259,
134.909004136217)) ;
#122668=CARTESIAN_POINT('Ctrl Pts',(-12.9313786707726,13.7357351510131,
134.862180593803)) ;
#122669=CARTESIAN_POINT('Ctrl Pts',(-12.902794866539,14.0000244491373,134.745686603675)) ;
#122670=CARTESIAN_POINT('Ctrl Pts',(-12.8524484285654,14.2248064092014,
134.565353916144)) ;
#122671=CARTESIAN_POINT('Ctrl Pts',(-12.7854240568806,14.3907221874245,
134.336542174488)) ;
#122672=CARTESIAN_POINT('Ctrl Pts',(-12.706579030057,14.4880878252355,134.073042339653)) ;
#122673=CARTESIAN_POINT('Ctrl Pts',(-12.6227960155401,14.5090844466389,
133.795223033695)) ;
#122674=CARTESIAN_POINT('Ctrl Pts',(-12.539998525129,14.4517330875411,133.520035240251)) ;
#122675=CARTESIAN_POINT('Ctrl Pts',(-12.4662105878813,14.3213872706393,
133.271495742536)) ;
#122676=CARTESIAN_POINT('Ctrl Pts',(-12.4062689631647,14.1266125068475,
133.063268319006)) ;
#122677=CARTESIAN_POINT('Ctrl Pts',(-12.3655117240341,13.8801112237431,
132.910943391806)) ;
#122678=CARTESIAN_POINT('Ctrl Pts',(-12.3479181290299,13.6025838419119,
132.826510049742)) ;
#122679=CARTESIAN_POINT('Ctrl Pts',(-12.3550115270232,13.3122087049322,
132.814182204973)) ;
#122680=CARTESIAN_POINT('Ctrl Pts',(-12.3873488064402,13.0284663697123,
132.875444965799)) ;
#122681=CARTESIAN_POINT('Ctrl Pts',(-12.4430942234961,12.7739763347418,
133.005207312266)) ;
#122682=CARTESIAN_POINT('Ctrl Pts',(-12.5191788386626,12.5655227594086,
133.194325737859)) ;
#122683=CARTESIAN_POINT('Ctrl Pts',(-12.6106767313811,12.4188417655465,
133.428523192485)) ;
#122684=CARTESIAN_POINT('Ctrl Pts',(-12.7117766054599,12.343819791052,133.690792434329)) ;
#122685=CARTESIAN_POINT('Ctrl Pts',(-12.816567838712,12.3461750188478,133.963682834605)) ;
#122686=CARTESIAN_POINT('Ctrl Pts',(-12.9172505658003,12.4256200301873,
134.224741101302)) ;
#122687=CARTESIAN_POINT('Ctrl Pts',(-13.0081288677706,12.5766361181176,
134.457068472408)) ;
#122688=CARTESIAN_POINT('Ctrl Pts',(-13.0830551204936,12.7882866055861,
134.642823016933)) ;
#122689=CARTESIAN_POINT('Ctrl Pts',(-13.1374659893816,13.0452021106171,
134.768666892341)) ;
#122690=CARTESIAN_POINT('Ctrl Pts',(-13.1682549286523,13.3293878961544,
134.82547934159)) ;
#122691=CARTESIAN_POINT('Ctrl Pts',(-13.173880051194,13.6204037391964,134.808769964606)) ;
#122692=CARTESIAN_POINT('Ctrl Pts',(-13.1546580785961,13.8971497414612,
134.719488338554)) ;
#122693=CARTESIAN_POINT('Ctrl Pts',(-13.1127775878744,14.1397539982186,
134.564047361394)) ;
#122694=CARTESIAN_POINT('Ctrl Pts',(-13.0518026076723,14.3313465280224,
134.352767547066)) ;
#122695=CARTESIAN_POINT('Ctrl Pts',(-12.9771687196265,14.4574458886048,
134.101695813006)) ;
#122696=CARTESIAN_POINT('Ctrl Pts',(-12.8945575156937,14.509972396165,133.827242524673)) ;
#122697=CARTESIAN_POINT('Ctrl Pts',(-12.810549262933,14.4843439557881,133.54862424111)) ;
#122698=CARTESIAN_POINT('Ctrl Pts',(-12.7323948337942,14.3827749210334,
133.287220875815)) ;
#122699=CARTESIAN_POINT('Ctrl Pts',(-12.6660452885251,14.2124739765949,
133.060271073219)) ;
#122700=CARTESIAN_POINT('Ctrl Pts',(-12.617078134981,13.9855789270548,132.88409986354)) ;
#122701=CARTESIAN_POINT('Ctrl Pts',(-12.5897214243873,13.7185805831256,
132.771079224658)) ;
#122702=CARTESIAN_POINT('Ctrl Pts',(-12.5866426015232,13.4303185672317,
132.728965795836)) ;
#122703=CARTESIAN_POINT('Ctrl Pts',(-12.6087424481062,13.1417758390937,
132.760436389614)) ;
#122704=CARTESIAN_POINT('Ctrl Pts',(-12.6553781410414,12.8725286087569,
132.863473470132)) ;
#122705=CARTESIAN_POINT('Ctrl Pts',(-12.7236698746677,12.6435096250976,
133.029870355786)) ;
#122706=CARTESIAN_POINT('Ctrl Pts',(-12.8095900819889,12.470154617103,133.24774107517)) ;
#122707=CARTESIAN_POINT('Ctrl Pts',(-12.9076323750732,12.3650501816311,
133.501043473753)) ;
#122708=CARTESIAN_POINT('Ctrl Pts',(-13.0118238480069,12.3357586673989,
133.77222183819)) ;
#122709=CARTESIAN_POINT('Ctrl Pts',(-13.1147537603917,12.3843195645159,
134.039849230825)) ;
#122710=CARTESIAN_POINT('Ctrl Pts',(-13.2104578166392,12.5073667033233,
134.286277155853)) ;
#122711=CARTESIAN_POINT('Ctrl Pts',(-13.2923817417662,12.695820098274,134.492504363806)) ;
#122712=CARTESIAN_POINT('Ctrl Pts',(-13.3556189438732,12.9363650189031,
134.644124622663)) ;
#122713=CARTESIAN_POINT('Ctrl Pts',(-13.3962896174136,13.2120463476192,
134.729791046471)) ;
#122714=CARTESIAN_POINT('Ctrl Pts',(-13.4122210373586,13.5022482408363,
134.743260767323)) ;
#122715=CARTESIAN_POINT('Ctrl Pts',(-13.4028633875802,13.788401757224,134.682652163882)) ;
#122716=CARTESIAN_POINT('Ctrl Pts',(-13.3699700950396,14.0459452112238,
134.553608753382)) ;
#122717=CARTESIAN_POINT('Ctrl Pts',(-13.3160081710471,14.261068186074,134.362699423646)) ;
#122718=CARTESIAN_POINT('Ctrl Pts',(-13.2464308886998,14.4145624952327,
134.126463196777)) ;
#122719=CARTESIAN_POINT('Ctrl Pts',(-13.1660070259215,14.4980852442795,
133.858308768603)) ;
#122720=CARTESIAN_POINT('Ctrl Pts',(-13.0818602097117,14.5041312509629,
133.579371099685)) ;
#122721=CARTESIAN_POINT('Ctrl Pts',(-13.0005482976357,14.4326961548768,
133.308694344568)) ;
#122722=CARTESIAN_POINT('Ctrl Pts',(-12.9287700664934,14.2894246996344,
133.065951377945)) ;
#122723=CARTESIAN_POINT('Ctrl Pts',(-12.8719513781794,14.0826506129639,
132.86668732997)) ;
#122724=CARTESIAN_POINT('Ctrl Pts',(-12.8356455811312,13.8312289814619,
132.727716504135)) ;
#122725=CARTESIAN_POINT('Ctrl Pts',(-12.8223908350727,13.5479803719868,
132.655735280563)) ;
#122726=CARTESIAN_POINT('Ctrl Pts',(-12.8343672045851,13.257297898438,132.657650391912)) ;
#122727=CARTESIAN_POINT('Ctrl Pts',(-12.8711497724761,12.9781390141801,
132.731997740918)) ;
#122728=CARTESIAN_POINT('Ctrl Pts',(-12.9313756283262,12.7298469956755,
132.874665515828)) ;
#122729=CARTESIAN_POINT('Ctrl Pts',(-13.0103407400145,12.5331717504731,
133.072398199913)) ;
#122730=CARTESIAN_POINT('Ctrl Pts',(-13.104520422701,12.3987049958051,133.314282750599)) ;
#122731=CARTESIAN_POINT('Ctrl Pts',(-13.206651695878,12.3381977038027,133.579601997238)) ;
#122732=CARTESIAN_POINT('Ctrl Pts',(-13.3114979804847,12.3556286047268,
133.852577072708)) ;
#122733=CARTESIAN_POINT('Ctrl Pts',(-13.410155841517,12.4484986932729,134.107929156)) ;
#122734=CARTESIAN_POINT('Ctrl Pts',(-13.4988137139682,12.6124652381156,
134.333636594698)) ;
#122735=CARTESIAN_POINT('Ctrl Pts',(-13.5699367109128,12.833019455732,134.508418387899)) ;
#122736=CARTESIAN_POINT('Ctrl Pts',(-13.6204000704498,13.0981217097557,
134.622522835896)) ;
#122737=CARTESIAN_POINT('Ctrl Pts',(-13.6463216515392,13.3840424084956,
134.665255919507)) ;
#122738=CARTESIAN_POINT('Ctrl Pts',(-13.6472573616294,13.673804350161,134.63486456253)) ;
#122739=CARTESIAN_POINT('Ctrl Pts',(-13.6235693400262,13.9458856599705,
134.532515817835)) ;
#122740=CARTESIAN_POINT('Ctrl Pts',(-13.5776193745675,14.1805609779054,
134.365096818976)) ;
#122741=CARTESIAN_POINT('Ctrl Pts',(-13.513877843915,14.3602096691543,134.145871518623)) ;
#122742=CARTESIAN_POINT('Ctrl Pts',(-13.4366571499825,14.47371465445,133.886974753033)) ;
#122743=CARTESIAN_POINT('Ctrl Pts',(-13.3536493203175,14.5109817362897,
133.611512807046)) ;
#122744=CARTESIAN_POINT('Ctrl Pts',(-13.270489833554,14.4710234549687,133.335494570733)) ;
#122745=CARTESIAN_POINT('Ctrl Pts',(-13.1939950003663,14.3558611737084,
133.078903250233)) ;
#122746=CARTESIAN_POINT('Ctrl Pts',(-13.1304641501164,14.173605953239,132.860148687561)) ;
#122747=CARTESIAN_POINT('Ctrl Pts',(-13.0853217322533,13.9381264570577,
132.695195172933)) ;
#122748=CARTESIAN_POINT('Ctrl Pts',(-13.0623501902045,13.6651920565378,
132.594928970547)) ;
#122749=CARTESIAN_POINT('Ctrl Pts',(-13.0639502382484,13.3755914390975,
132.566529475268)) ;
#122750=CARTESIAN_POINT('Ctrl Pts',(-13.0910376757839,13.0874856739398,
132.612349617676)) ;
#122751=CARTESIAN_POINT('Ctrl Pts',(-13.1416877816723,12.8264336867777,
132.72738070205)) ;
#122752=CARTESIAN_POINT('Ctrl Pts',(-13.2137845958373,12.6060973636301,
132.904801873855)) ;
#122753=CARTESIAN_POINT('Ctrl Pts',(-13.3022604878942,12.4450312815742,
133.130209138199)) ;
#122754=CARTESIAN_POINT('Ctrl Pts',(-13.4023564676707,12.3534665915943,
133.389360301153)) ;
#122755=CARTESIAN_POINT('Ctrl Pts',(-13.5063840325338,12.3390030026154,
133.660229603222)) ;
#122756=CARTESIAN_POINT('Ctrl Pts',(-13.6088026539799,12.4020393022516,
133.926234642771)) ;
#122757=CARTESIAN_POINT('Ctrl Pts',(-13.7023554945417,12.5385712255671,
134.166373386109)) ;
#122758=CARTESIAN_POINT('Ctrl Pts',(-13.7808725717634,12.7373374755761,
134.362748710196)) ;
#122759=CARTESIAN_POINT('Ctrl Pts',(-13.8402040940885,12.9861208763485,
134.502915815351)) ;
#122760=CARTESIAN_POINT('Ctrl Pts',(-13.876327184752,13.2660912868939,134.575313990181)) ;
#122761=CARTESIAN_POINT('Ctrl Pts',(-13.8874746844965,13.5573229974737,
134.57474671631)) ;
#122762=CARTESIAN_POINT('Ctrl Pts',(-13.8735918642489,13.8386954173301,
134.501090795817)) ;
#122763=CARTESIAN_POINT('Ctrl Pts',(-13.8363610091342,14.0906009261112,
134.359190696365)) ;
#122764=CARTESIAN_POINT('Ctrl Pts',(-13.7792326201737,14.2945041038628,
134.159193115425)) ;
#122765=CARTESIAN_POINT('Ctrl Pts',(-13.7069314087024,14.4361574942565,
133.914839142184)) ;
#122766=CARTESIAN_POINT('Ctrl Pts',(-13.6254421725762,14.5051117773277,
133.643658661375)) ;
#122767=CARTESIAN_POINT('Ctrl Pts',(-13.5413998090464,14.4965825882903,
133.36505223233)) ;
#122768=CARTESIAN_POINT('Ctrl Pts',(-13.4614100970346,14.4113394048867,
133.098272224482)) ;
#122769=CARTESIAN_POINT('Ctrl Pts',(-13.3917824494901,14.2546478359796,
132.861652683335)) ;
#122770=CARTESIAN_POINT('Ctrl Pts',(-13.3387306382198,14.0391437504434,
132.673608609)) ;
#122771=CARTESIAN_POINT('Ctrl Pts',(-13.3063690219606,13.7793415261531,
132.545957337206)) ;
#122772=CARTESIAN_POINT('Ctrl Pts',(-13.2978117868869,13.4941094654563,
132.487858778329)) ;
#122773=CARTESIAN_POINT('Ctrl Pts',(-13.3145790512622,13.2026873964626,
132.503605828306)) ;
#122774=CARTESIAN_POINT('Ctrl Pts',(-13.3558347243656,12.9288332689777,
132.591113022334)) ;
#122775=CARTESIAN_POINT('Ctrl Pts',(-13.42001442131,12.6885083227908,132.745324620566)) ;
#122776=CARTESIAN_POINT('Ctrl Pts',(-13.502239679633,12.5026390523848,132.95253565952)) ;
#122777=CARTESIAN_POINT('Ctrl Pts',(-13.5982356435554,12.3816810142256,
133.199819473708)) ;
#122778=CARTESIAN_POINT('Ctrl Pts',(-13.7013793589073,12.3354826601101,
133.4680451402)) ;
#122779=CARTESIAN_POINT('Ctrl Pts',(-13.80552054206,12.3671988695935,133.739067392066)) ;
#122780=CARTESIAN_POINT('Ctrl Pts',(-13.9034200313392,12.4748749590594,
133.991897701478)) ;
#122781=CARTESIAN_POINT('Ctrl Pts',(-13.9886532302031,12.6498955161038,
134.207834562929)) ;
#122782=CARTESIAN_POINT('Ctrl Pts',(-14.0562984562977,12.8801431271714,
134.372370038988)) ;
#122783=CARTESIAN_POINT('Ctrl Pts',(-14.1022223995616,13.1504415256103,
134.473311483202)) ;
#122784=CARTESIAN_POINT('Ctrl Pts',(-14.123569864062,13.4387392039499,134.502646409052)) ;
#122785=CARTESIAN_POINT('Ctrl Pts',(-14.1196852055216,13.7280473627643,
134.458016194927)) ;
#122786=CARTESIAN_POINT('Ctrl Pts',(-14.0916226131084,13.9932362270437,
134.343028102369)) ;
#122787=CARTESIAN_POINT('Ctrl Pts',(-14.0420866562791,14.2186784013421,
134.165196371218)) ;
#122788=CARTESIAN_POINT('Ctrl Pts',(-13.9751431455741,14.3872014595801,
133.936454641031)) ;
#122789=CARTESIAN_POINT('Ctrl Pts',(-13.8968885105808,14.4862165376707,
133.674833892658)) ;
#122790=CARTESIAN_POINT('Ctrl Pts',(-13.8128617180063,14.5095010534955,
133.396175956052)) ;
#122791=CARTESIAN_POINT('Ctrl Pts',(-13.7304497643329,14.4548476370639,
133.12233385827)) ;
#122792=CARTESIAN_POINT('Ctrl Pts',(-13.6557838577664,14.3259645840264,
132.871005987492)) ;
#122793=CARTESIAN_POINT('Ctrl Pts',(-13.5953724007658,14.132023950122,132.661341229371)) ;
#122794=CARTESIAN_POINT('Ctrl Pts',(-13.5543327518314,13.8890686102105,
132.508494471355)) ;
#122795=CARTESIAN_POINT('Ctrl Pts',(-13.5358381663009,13.6109286818878,
132.421258113055)) ;
#122796=CARTESIAN_POINT('Ctrl Pts',(-13.542226996446,13.3205779167508,132.406873150315)) ;
#122797=CARTESIAN_POINT('Ctrl Pts',(-13.5739794264152,13.0356408417454,
132.466340476707)) ;
#122798=CARTESIAN_POINT('Ctrl Pts',(-13.6288864921363,12.7811566928917,
132.593791195391)) ;
#122799=CARTESIAN_POINT('Ctrl Pts',(-13.7044062779157,12.5709849974497,
132.78125363208)) ;
#122800=CARTESIAN_POINT('Ctrl Pts',(-13.7955344981284,12.4221765780121,
133.014364402187)) ;
#122801=CARTESIAN_POINT('Ctrl Pts',(-13.8968781749281,12.3447406523641,
133.277205956951)) ;
#122802=CARTESIAN_POINT('Ctrl Pts',(-14.0015137983245,12.3451621896592,
133.549692248237)) ;
#122803=CARTESIAN_POINT('Ctrl Pts',(-14.1021214510041,12.4221618578868,
133.810621215989)) ;
#122804=CARTESIAN_POINT('Ctrl Pts',(-14.1934712046152,12.5713294888185,
134.04429329116)) ;
#122805=CARTESIAN_POINT('Ctrl Pts',(-14.2688631560375,12.781135912573,134.231447471873)) ;
#122806=CARTESIAN_POINT('Ctrl Pts',(-14.3239990336241,13.0373855963871,
134.359354214164)) ;
#122807=CARTESIAN_POINT('Ctrl Pts',(-14.3554632461864,13.3202249658799,
134.418237999123)) ;
#122808=CARTESIAN_POINT('Ctrl Pts',(-14.3618511494396,13.6126651184226,
134.403601562198)) ;
#122809=CARTESIAN_POINT('Ctrl Pts',(-14.3433707383352,13.8891096825995,
134.316608545591)) ;
#122810=CARTESIAN_POINT('Ctrl Pts',(-14.3020343167185,14.1334577296797,
134.162685402609)) ;
#122811=CARTESIAN_POINT('Ctrl Pts',(-14.2417808956239,14.3262011562841,
133.95363095538)) ;
#122812=CARTESIAN_POINT('Ctrl Pts',(-14.1670021264005,14.4552702569289,
133.701921829577)) ;
#122813=CARTESIAN_POINT('Ctrl Pts',(-14.0844340238259,14.5094659908496,
133.427572654941)) ;
#122814=CARTESIAN_POINT('Ctrl Pts',(-14.0009203738356,14.4862792648155,
133.150618168943)) ;
#122815=CARTESIAN_POINT('Ctrl Pts',(-13.9222696214615,14.3867194046613,
132.887667382131)) ;
#122816=CARTESIAN_POINT('Ctrl Pts',(-13.8555447933731,14.2183273088974,
132.659645946051)) ;
#122817=CARTESIAN_POINT('Ctrl Pts',(-13.8058821838959,13.992244078071,132.481355163551)) ;
#122818=CARTESIAN_POINT('Ctrl Pts',(-13.7779670985824,13.7260908725509,
132.366711198007)) ;
#122819=CARTESIAN_POINT('Ctrl Pts',(-13.7741339235042,13.4392990631296,
132.322525920907)) ;
#122820=CARTESIAN_POINT('Ctrl Pts',(-13.7956345554261,13.1491383959326,
132.352086669861)) ;
#122821=CARTESIAN_POINT('Ctrl Pts',(-13.8414238224562,12.8801381500525,
132.452791421209)) ;
#122822=CARTESIAN_POINT('Ctrl Pts',(-13.9094358836924,12.64883120769,132.618229163413)) ;
#122823=CARTESIAN_POINT('Ctrl Pts',(-13.9945003827061,12.4746173054018,
132.833772527183)) ;
#122824=CARTESIAN_POINT('Ctrl Pts',(-14.092526137208,12.3669410554066,133.086930422302)) ;
#122825=CARTESIAN_POINT('Ctrl Pts',(-14.1966145933381,12.3355244461353,
133.35782177204)) ;
#122826=CARTESIAN_POINT('Ctrl Pts',(-14.2996113408853,12.3818824720289,
133.625656611254)) ;
#122827=CARTESIAN_POINT('Ctrl Pts',(-14.3954499004576,12.5024424639559,
133.872548813345)) ;
#122828=CARTESIAN_POINT('Ctrl Pts',(-14.4782507258047,12.6900860834509,
134.081174564054)) ;
#122829=CARTESIAN_POINT('Ctrl Pts',(-14.5418899408693,12.9290694340201,
134.234032679536)) ;
#122830=CARTESIAN_POINT('Ctrl Pts',(-14.5832089306858,13.2033803581446,
134.32166291928)) ;
#122831=CARTESIAN_POINT('Ctrl Pts',(-14.5998913013211,13.4938855393019,
134.33727238423)) ;
#122832=CARTESIAN_POINT('Ctrl Pts',(-14.5913281946562,13.7798209622441,
134.27907156831)) ;
#122833=CARTESIAN_POINT('Ctrl Pts',(-14.5588933837246,14.0398148496058,
134.151181115851)) ;
#122834=CARTESIAN_POINT('Ctrl Pts',(-14.5055772883064,14.2555982023478,
133.962265861814)) ;
#122835=CARTESIAN_POINT('Ctrl Pts',(-14.4363858406778,14.4112165805385,
133.727140752466)) ;
#122836=CARTESIAN_POINT('Ctrl Pts',(-14.3558616395475,14.4969136071728,
133.458576254405)) ;
#122837=CARTESIAN_POINT('Ctrl Pts',(-14.2721531493714,14.5049696606859,
133.18108471151)) ;
#122838=CARTESIAN_POINT('Ctrl Pts',(-14.1907040785466,14.4360248987559,
132.910029619532)) ;
#122839=CARTESIAN_POINT('Ctrl Pts',(-14.1184830111954,14.2945753095186,
132.665954434727)) ;
#122840=CARTESIAN_POINT('Ctrl Pts',(-14.0611734388472,14.0897547152948,
132.465297187422)) ;
#122841=CARTESIAN_POINT('Ctrl Pts',(-14.0241626277862,13.8386999371902,
132.324168957696)) ;
#122842=CARTESIAN_POINT('Ctrl Pts',(-14.0101940089266,13.557404245294,132.250264713925)) ;
#122843=CARTESIAN_POINT('Ctrl Pts',(-14.0215298956694,13.2644127915957,
132.250046158682)) ;
#122844=CARTESIAN_POINT('Ctrl Pts',(-14.0575338067527,12.9862193835362,
132.322298184115)) ;
#122845=CARTESIAN_POINT('Ctrl Pts',(-14.11688454634,12.7371110279746,132.462483680312)) ;
#122846=CARTESIAN_POINT('Ctrl Pts',(-14.1955901076799,12.5380202146654,
132.659347067288)) ;
#122847=CARTESIAN_POINT('Ctrl Pts',(-14.28946201566,12.4015272035531,132.900325805036)) ;
#122848=CARTESIAN_POINT('Ctrl Pts',(-14.3915176998432,12.3389469979449,
133.165397994997)) ;
#122849=CARTESIAN_POINT('Ctrl Pts',(-14.495856941834,12.3537865285607,133.437069895814)) ;
#122850=CARTESIAN_POINT('Ctrl Pts',(-14.5953958091729,12.4449099781865,
133.694784504948)) ;
#122851=CARTESIAN_POINT('Ctrl Pts',(-14.6843904512869,12.6072328334928,
133.921485691051)) ;
#122852=CARTESIAN_POINT('Ctrl Pts',(-14.7559156143078,12.8259752277409,
134.097497642623)) ;
#122853=CARTESIAN_POINT('Ctrl Pts',(-14.8069969604636,13.0894865992637,
134.213476347008)) ;
#122854=CARTESIAN_POINT('Ctrl Pts',(-14.8337697603498,13.3763086885043,
134.258547210058)) ;
#122855=CARTESIAN_POINT('Ctrl Pts',(-14.8353123618202,13.6661024734113,
134.229945019376)) ;
#122856=CARTESIAN_POINT('Ctrl Pts',(-14.8124440803992,13.9378774690874,
134.130130172042)) ;
#122857=CARTESIAN_POINT('Ctrl Pts',(-14.7669543359677,14.1747933111433,
133.963938244878)) ;
#122858=CARTESIAN_POINT('Ctrl Pts',(-14.7037362321117,14.3556679919274,
133.746303038478)) ;
#122859=CARTESIAN_POINT('Ctrl Pts',(-14.6272249106364,14.4711053285872,
133.489636572354)) ;
#122860=CARTESIAN_POINT('Ctrl Pts',(-14.5437193293295,14.5111709794694,
133.21248187099)) ;
#122861=CARTESIAN_POINT('Ctrl Pts',(-14.4603753611253,14.4729025358904,
132.935881904141)) ;
#122862=CARTESIAN_POINT('Ctrl Pts',(-14.3839774531889,14.3605014207988,
132.679746155635)) ;
#122863=CARTESIAN_POINT('Ctrl Pts',(-14.3196308997706,14.1789799465746,
132.458418098484)) ;
#122864=CARTESIAN_POINT('Ctrl Pts',(-14.2741191671532,13.9453130634453,
132.292485354684)) ;
#122865=CARTESIAN_POINT('Ctrl Pts',(-14.2504732824165,13.6736132719233,
132.190294327821)) ;
#122866=CARTESIAN_POINT('Ctrl Pts',(-14.2513173292015,13.3843416076431,
132.159699879319)) ;
#122867=CARTESIAN_POINT('Ctrl Pts',(-14.2776743807249,13.0956424209517,
132.20336504898)) ;
#122868=CARTESIAN_POINT('Ctrl Pts',(-14.3276746731947,12.8335786861196,
132.31649173796)) ;
#122869=CARTESIAN_POINT('Ctrl Pts',(-14.3992226458396,12.611652190356,132.492301020647)) ;
#122870=CARTESIAN_POINT('Ctrl Pts',(-14.4874521229701,12.4486057551385,
132.716936908001)) ;
#122871=CARTESIAN_POINT('Ctrl Pts',(-14.5869437822239,12.3551665725231,
132.974446240664)) ;
#122872=CARTESIAN_POINT('Ctrl Pts',(-14.6912604023576,12.338311146402,133.246052457304)) ;
#122873=CARTESIAN_POINT('Ctrl Pts',(-14.7936701073007,12.39913191908,133.512086338097)) ;
#122874=CARTESIAN_POINT('Ctrl Pts',(-14.8875591251362,12.5336134533254,
133.753205453511)) ;
#122875=CARTESIAN_POINT('Ctrl Pts',(-14.9666002083636,12.7304748931974,
133.951130887302)) ;
#122876=CARTESIAN_POINT('Ctrl Pts',(-15.0268934696713,12.9801495362985,
134.093853087901)) ;
#122877=CARTESIAN_POINT('Ctrl Pts',(-15.0633119226926,13.2569932871313,
134.1674226943)) ;
#122878=CARTESIAN_POINT('Ctrl Pts',(-15.0753247260425,13.5493203158773,
134.169247540756)) ;
#122879=CARTESIAN_POINT('Ctrl Pts',(-15.0620951374536,13.8310611217576,
134.097523512761)) ;
#122880=CARTESIAN_POINT('Ctrl Pts',(-15.0254414043506,14.0843639820839,
133.957268069224)) ;
#122881=CARTESIAN_POINT('Ctrl Pts',(-14.9688116918277,14.2896245798539,
133.758745314845)) ;
#122882=CARTESIAN_POINT('Ctrl Pts',(-14.8969851728588,14.433006390985,133.515831551673)) ;
#122883=CARTESIAN_POINT('Ctrl Pts',(-14.8156323832822,14.5042107644556,
133.245031813908)) ;
#122884=CARTESIAN_POINT('Ctrl Pts',(-14.7315386625411,14.4979449677576,
132.96626438036)) ;
#122885=CARTESIAN_POINT('Ctrl Pts',(-14.6511153589677,14.4144600975177,
132.698120714996)) ;
#122886=CARTESIAN_POINT('Ctrl Pts',(-14.5812309184614,14.259520873967,132.46078302777)) ;
#122887=CARTESIAN_POINT('Ctrl Pts',(-14.5278024226519,14.0462147796788,
132.271741524007)) ;
#122888=CARTESIAN_POINT('Ctrl Pts',(-14.4947222340059,13.7868051984224,
132.141911296577)) ;
#122889=CARTESIAN_POINT('Ctrl Pts',(-14.4855193570548,13.5027355977882,
132.082011946942)) ;
#122890=CARTESIAN_POINT('Ctrl Pts',(-14.5014599681923,13.2114163358095,
132.095374697993)) ;
#122891=CARTESIAN_POINT('Ctrl Pts',(-14.5421822561904,12.9359342039492,
132.181213543049)) ;
#122892=CARTESIAN_POINT('Ctrl Pts',(-14.6055653322678,12.6951561372944,
132.33320802425)) ;
#122893=CARTESIAN_POINT('Ctrl Pts',(-14.6873122286846,12.5073060889563,
132.539005348311)) ;
#122894=CARTESIAN_POINT('Ctrl Pts',(-14.7831217899283,12.3841592537523,
132.785703089486)) ;
#122895=CARTESIAN_POINT('Ctrl Pts',(-14.8861739591066,12.3356200242118,
133.053655565713)) ;
#122896=CARTESIAN_POINT('Ctrl Pts',(-14.9907676880009,12.3655842342963,
133.325869841831)) ;
#122897=CARTESIAN_POINT('Ctrl Pts',(-15.0881721710896,12.4702048662911,
133.57752343002)) ;
#122898=CARTESIAN_POINT('Ctrl Pts',(-15.1745656232195,12.6448837990351,
133.796562666015)) ;
#122899=CARTESIAN_POINT('Ctrl Pts',(-15.2423252658601,12.8725084203653,
133.96163895876)) ;
#122900=CARTESIAN_POINT('Ctrl Pts',(-15.2891967482421,13.1434988264021,
134.065150989214)) ;
#122901=CARTESIAN_POINT('Ctrl Pts',(-15.3110173033622,13.4301737730148,
134.096029449475)) ;
#122902=CARTESIAN_POINT('Ctrl Pts',(-15.3080372177454,13.718779591721,134.054168270157)) ;
#122903=CARTESIAN_POINT('Ctrl Pts',(-15.2804060867555,13.9870154535706,
133.940172267824)) ;
#122904=CARTESIAN_POINT('Ctrl Pts',(-15.2316377774267,14.2124398495338,
133.764769336654)) ;
#122905=CARTESIAN_POINT('Ctrl Pts',(-15.165220452902,14.3830654639858,133.537573308493)) ;
#122906=CARTESIAN_POINT('Ctrl Pts',(-15.086831973333,14.4846609671348,133.275405165143)) ;
#122907=CARTESIAN_POINT('Ctrl Pts',(-15.0028388335443,14.5097913596576,
132.99683728162)) ;
#122908=CARTESIAN_POINT('Ctrl Pts',(-14.9206500675865,14.4576092834796,
132.723792129969)) ;
#122909=CARTESIAN_POINT('Ctrl Pts',(-14.8454721612017,14.3304830753539,
132.470882970049)) ;
#122910=CARTESIAN_POINT('Ctrl Pts',(-14.7847088609425,14.1386182913456,
132.260264003398)) ;
#122911=CARTESIAN_POINT('Ctrl Pts',(-14.743001227268,13.8965845637284,132.105417644869)) ;
#122912=CARTESIAN_POINT('Ctrl Pts',(-14.7238223056134,13.6198364139058,
132.016265937607)) ;
#122913=CARTESIAN_POINT('Ctrl Pts',(-14.7294887108316,13.3288843077371,
131.999686789623)) ;
#122914=CARTESIAN_POINT('Ctrl Pts',(-14.7603420714365,13.0447398144614,
132.056683740009)) ;
#122915=CARTESIAN_POINT('Ctrl Pts',(-14.8146479427189,12.7881834818384,
132.182276189974)) ;
#122916=CARTESIAN_POINT('Ctrl Pts',(-14.8900730017905,12.5755908845443,
132.369299666731)) ;
#122917=CARTESIAN_POINT('Ctrl Pts',(-14.9804283663031,12.4257573634701,
132.600310180538)) ;
#122918=CARTESIAN_POINT('Ctrl Pts',(-15.081355257857,12.3460112100503,132.861995469573)) ;
#122919=CARTESIAN_POINT('Ctrl Pts',(-15.1861080584628,12.3439532777376,
133.134786433152)) ;
#122920=CARTESIAN_POINT('Ctrl Pts',(-15.2871434627303,12.4188219737117,
133.396894492333)) ;
#122921=CARTESIAN_POINT('Ctrl Pts',(-15.3791342092762,12.5668342389243,
133.632321418082)) ;
#122922=CARTESIAN_POINT('Ctrl Pts',(-15.4545799026391,12.7739567012615,
133.819824457066)) ;
#122923=CARTESIAN_POINT('Ctrl Pts',(-15.5105014700374,13.0292277214245,
133.949992547475)) ;
#122924=CARTESIAN_POINT('Ctrl Pts',(-15.54268567825,13.3121169680532,134.010916269422)) ;
#122925=CARTESIAN_POINT('Ctrl Pts',(-15.5498365649966,13.603671342882,133.998623037179)) ;
#122926=CARTESIAN_POINT('Ctrl Pts',(-15.531946047433,13.8822011658837,133.913179480728)) ;
#122927=CARTESIAN_POINT('Ctrl Pts',(-15.491392435008,14.1265341471654,133.76170716662)) ;
#122928=CARTESIAN_POINT('Ctrl Pts',(-15.431540081892,14.3215277974717,133.553749376831)) ;
#122929=CARTESIAN_POINT('Ctrl Pts',(-15.3571603450366,14.4523872873454,
133.303244580285)) ;
#122930=CARTESIAN_POINT('Ctrl Pts',(-15.2748106437101,14.509081275177,133.029560282638)) ;
#122931=CARTESIAN_POINT('Ctrl Pts',(-15.1906905864766,14.4877530377578,
132.750612125616)) ;
#122932=CARTESIAN_POINT('Ctrl Pts',(-15.1123084559039,14.3906972119634,
132.488655125181)) ;
#122933=CARTESIAN_POINT('Ctrl Pts',(-15.0450774786089,14.2242126836462,
132.259127840119)) ;
#122934=CARTESIAN_POINT('Ctrl Pts',(-14.9949477568096,14.0000453573048,
132.079539850124)) ;
#122935=CARTESIAN_POINT('Ctrl Pts',(-14.9662169923433,13.7349940893193,
131.962516118515)) ;
#122936=CARTESIAN_POINT('Ctrl Pts',(-14.9617452970706,13.4462937932098,
131.916206457482)) ;
#122937=CARTESIAN_POINT('Ctrl Pts',(-14.9822951077096,13.1586523998495,
131.943317162503)) ;
#122938=CARTESIAN_POINT('Ctrl Pts',(-15.0277849352445,12.8863235955885,
132.042839199694)) ;
#122939=CARTESIAN_POINT('Ctrl Pts',(-15.0948411666316,12.6553854618845,
132.205713830206)) ;
#122940=CARTESIAN_POINT('Ctrl Pts',(-15.1795278177596,12.4787538622729,
132.420093453233)) ;
#122941=CARTESIAN_POINT('Ctrl Pts',(-15.2776667934257,12.3688114819393,
132.673464609376)) ;
#122942=CARTESIAN_POINT('Ctrl Pts',(-15.3812344932646,12.3354319131045,
132.942973836331)) ;
#122943=CARTESIAN_POINT('Ctrl Pts',(-15.4844363162764,12.3792576345139,
133.211386539826)) ;
#122944=CARTESIAN_POINT('Ctrl Pts',(-15.5811089769105,12.4988399158766,
133.460512436159)) ;
#122945=CARTESIAN_POINT('Ctrl Pts',(-15.6637127965401,12.6835118837374,
133.668813420161)) ;
#122946=CARTESIAN_POINT('Ctrl Pts',(-15.728149203225,12.9214924452222,133.823933063528)) ;
#122947=CARTESIAN_POINT('Ctrl Pts',(-15.7701936666408,13.1954917190088,
133.913637309434)) ;
#122948=CARTESIAN_POINT('Ctrl Pts',(-15.7875791085066,13.4865486647074,
133.931220140978)) ;
#122949=CARTESIAN_POINT('Ctrl Pts',(-15.7796291542385,13.7724716992733,
133.874855409992)) ;
#122950=CARTESIAN_POINT('Ctrl Pts',(-15.7479919520967,14.0322260172615,
133.749447091464)) ;
#122951=CARTESIAN_POINT('Ctrl Pts',(-15.695387454676,14.249618629869,133.56264873374)) ;
#122952=CARTESIAN_POINT('Ctrl Pts',(-15.6261515803863,14.4079187286369,
133.327193888207)) ;
#122953=CARTESIAN_POINT('Ctrl Pts',(-15.5465490261103,14.4951289707047,
133.061613614476)) ;
#122954=CARTESIAN_POINT('Ctrl Pts',(-15.4624323059552,14.5060206612055,
132.782752303538)) ;
#122955=CARTESIAN_POINT('Ctrl Pts',(-15.3805684268842,14.4388851270518,
132.51038836699)) ;
#122956=CARTESIAN_POINT('Ctrl Pts',(-15.3079732071055,14.2990478381217,
132.265189265335)) ;
#122957=CARTESIAN_POINT('Ctrl Pts',(-15.2503508442927,14.0962769263581,
132.063706906888)) ;
#122958=CARTESIAN_POINT('Ctrl Pts',(-15.2126467032428,13.8463550292072,
131.920546038618)) ;
#122959=CARTESIAN_POINT('Ctrl Pts',(-15.1980783490908,13.5643760642883,
131.844749375842)) ;
#122960=CARTESIAN_POINT('Ctrl Pts',(-15.208492795854,13.2747378724678,131.842228274416)) ;
#122961=CARTESIAN_POINT('Ctrl Pts',(-15.2439809385834,12.9934295019574,
131.912682502554)) ;
#122962=CARTESIAN_POINT('Ctrl Pts',(-15.3026382333439,12.7438066422354,
132.050923610819)) ;
#122963=CARTESIAN_POINT('Ctrl Pts',(-15.3810068220172,12.542694227186,132.246728650902)) ;
#122964=CARTESIAN_POINT('Ctrl Pts',(-15.4741969738666,12.4046935574579,
132.485839130881)) ;
#122965=CARTESIAN_POINT('Ctrl Pts',(-15.5763327366627,12.3396331607935,
132.751061057437)) ;
#122966=CARTESIAN_POINT('Ctrl Pts',(-15.680579517544,12.3522551180279,133.022505742555)) ;
#122967=CARTESIAN_POINT('Ctrl Pts',(-15.7803492810426,12.4411586824075,
133.280892840196)) ;
#122968=CARTESIAN_POINT('Ctrl Pts',(-15.8697167426766,12.6013770610415,
133.508706785249)) ;
#122969=CARTESIAN_POINT('Ctrl Pts',(-15.9419214668062,12.819071741669,133.686638072034)) ;
#122970=CARTESIAN_POINT('Ctrl Pts',(-15.9935297236979,13.0807347129293,
133.804263305628)) ;
#122971=CARTESIAN_POINT('Ctrl Pts',(-16.0211044801934,13.3675409458687,
133.851621859569)) ;
#122972=CARTESIAN_POINT('Ctrl Pts',(-16.0234843448819,13.6570979950049,
133.825528484065)) ;
#122973=CARTESIAN_POINT('Ctrl Pts',(-16.000995765069,13.9319894333905,133.726516831796)) ;
#122974=CARTESIAN_POINT('Ctrl Pts',(-15.9565643522182,14.1676085516927,
133.563784888754)) ;
#122975=CARTESIAN_POINT('Ctrl Pts',(-15.8933708369746,14.3519029701599,
133.345953408387)) ;
#122976=CARTESIAN_POINT('Ctrl Pts',(-15.8172885156954,14.4687263887883,
133.09063231366)) ;
#122977=CARTESIAN_POINT('Ctrl Pts',(-15.7341653709837,14.5110206737837,
132.814693127497)) ;
#122978=CARTESIAN_POINT('Ctrl Pts',(-15.6507620381886,14.475483911121,132.537948900306)) ;
#122979=CARTESIAN_POINT('Ctrl Pts',(-15.5735490936641,14.3641243915887,
132.279183520569)) ;
#122980=CARTESIAN_POINT('Ctrl Pts',(-15.5093304300685,14.185998118253,132.058533710743)) ;
#122981=CARTESIAN_POINT('Ctrl Pts',(-15.462903310711,13.9527739610766,131.889757868276)) ;
#122982=CARTESIAN_POINT('Ctrl Pts',(-15.4385984833737,13.6818171752754,
131.785645579049)) ;
#122983=CARTESIAN_POINT('Ctrl Pts',(-15.4387626916475,13.392345635537,131.753011052265)) ;
#122984=CARTESIAN_POINT('Ctrl Pts',(-15.464243148025,13.1044624962765,131.794260353384)) ;
#122985=CARTESIAN_POINT('Ctrl Pts',(-15.5138238528878,12.8400819723837,
131.905988502202)) ;
#122986=CARTESIAN_POINT('Ctrl Pts',(-15.5846558690521,12.6174282729713,
132.079803115879)) ;
#122987=CARTESIAN_POINT('Ctrl Pts',(-15.6725999837267,12.452181454216,132.303549807549)) ;
#122988=CARTESIAN_POINT('Ctrl Pts',(-15.7718997242251,12.3567834927398,
132.560491848969)) ;
#122989=CARTESIAN_POINT('Ctrl Pts',(-15.875884107787,12.3377092342152,132.831217635272)) ;
#122990=CARTESIAN_POINT('Ctrl Pts',(-15.9785433015848,12.396207648245,133.097951008103)) ;
#122991=CARTESIAN_POINT('Ctrl Pts',(-16.0729880468236,12.5290433262916,
133.340617185065)) ;
#122992=CARTESIAN_POINT('Ctrl Pts',(-16.1524039006371,12.7244086521529,
133.539649727989)) ;
#122993=CARTESIAN_POINT('Ctrl Pts',(-16.2129909856311,12.970950220754,133.683466380543)) ;
#122994=CARTESIAN_POINT('Ctrl Pts',(-16.2505098060545,13.24944047257,133.759968218975)) ;
#122995=CARTESIAN_POINT('Ctrl Pts',(-16.263091069111,13.5418969111079,133.763438478373)) ;
#122996=CARTESIAN_POINT('Ctrl Pts',(-16.250600258302,13.8230885860474,133.693996985821)) ;
#122997=CARTESIAN_POINT('Ctrl Pts',(-16.2145955295992,14.0775912623992,
133.555629667295)) ;
#122998=CARTESIAN_POINT('Ctrl Pts',(-16.1585655383278,14.2842120208938,
133.358900373682)) ;
#122999=CARTESIAN_POINT('Ctrl Pts',(-16.0870153349153,14.4299776255762,
133.11674202411)) ;
#123000=CARTESIAN_POINT('Ctrl Pts',(-16.0054619777215,14.5033310573158,
132.845209708425)) ;
#123001=CARTESIAN_POINT('Ctrl Pts',(-15.9218838426601,14.4992417521952,
132.568160042897)) ;
#123002=CARTESIAN_POINT('Ctrl Pts',(-15.8410076302058,14.4177938992537,
132.298589352133)) ;
#123003=CARTESIAN_POINT('Ctrl Pts',(-15.7708993179965,14.2650804914184,
132.060678070363)) ;
#123004=CARTESIAN_POINT('Ctrl Pts',(-15.7168610518159,14.0529680000281,
131.86979828044)) ;
#123005=CARTESIAN_POINT('Ctrl Pts',(-15.6831746324261,13.7955268691578,
131.738309075754)) ;
#123006=CARTESIAN_POINT('Ctrl Pts',(-15.6731981033107,13.5095707979293,
131.675874334833)) ;
#123007=CARTESIAN_POINT('Ctrl Pts',(-15.6885514732525,13.2189035142274,
131.687611361385)) ;
#123008=CARTESIAN_POINT('Ctrl Pts',(-15.7284480149979,12.9437119836813,
131.771151515632)) ;
#123009=CARTESIAN_POINT('Ctrl Pts',(-15.7910818229785,12.7018112503585,
131.921000136973)) ;
#123010=CARTESIAN_POINT('Ctrl Pts',(-15.8727068944032,12.5115374305282,
132.126301688539)) ;
#123011=CARTESIAN_POINT('Ctrl Pts',(-15.9680538025931,12.3865362301687,
132.371709386679)) ;
#123012=CARTESIAN_POINT('Ctrl Pts',(-16.0715247163839,12.3360647675439,
132.640708439766)) ;
#123013=CARTESIAN_POINT('Ctrl Pts',(-16.174745238061,12.3630945112241,132.909384991678)) ;
#123014=CARTESIAN_POINT('Ctrl Pts',(-16.2735878679855,12.466576968382,133.164838729843)) ;
#123015=CARTESIAN_POINT('Ctrl Pts',(-16.3596505741579,12.6378737412179,
133.38322435223)) ;
#123016=CARTESIAN_POINT('Ctrl Pts',(-16.4286413429061,12.8661806777279,
133.551573412885)) ;
#123017=CARTESIAN_POINT('Ctrl Pts',(-16.4756920792434,13.133327748888,133.655983965445)) ;
#123018=CARTESIAN_POINT('Ctrl Pts',(-16.4985958888438,13.4221934769942,
133.689725454439)) ;
#123019=CARTESIAN_POINT('Ctrl Pts',(-16.4962280317727,13.7107571262916,
133.649695546072)) ;
#123020=CARTESIAN_POINT('Ctrl Pts',(-16.4693138102463,13.9798563789946,
133.537799466451)) ;
#123021=CARTESIAN_POINT('Ctrl Pts',(-16.420975161463,14.2070905645433,133.363583331429)) ;
#123022=CARTESIAN_POINT('Ctrl Pts',(-16.3550739984878,14.3790287585347,
133.137956843767)) ;
#123023=CARTESIAN_POINT('Ctrl Pts',(-16.2771937418169,14.4826462603949,
132.877370348531)) ;
#123024=CARTESIAN_POINT('Ctrl Pts',(-16.1929644857992,14.5101765741511,
132.597990225894)) ;
#123025=CARTESIAN_POINT('Ctrl Pts',(-16.1108016882086,14.4602520915312,
132.325086668321)) ;
#123026=CARTESIAN_POINT('Ctrl Pts',(-16.0352286482908,14.3349862853441,
132.070979800291)) ;
#123027=CARTESIAN_POINT('Ctrl Pts',(-15.9742472099228,14.1459035788167,
131.859889211481)) ;
#123028=CARTESIAN_POINT('Ctrl Pts',(-15.9316559559395,13.9042673527481,
131.702317007935)) ;
#123029=CARTESIAN_POINT('Ctrl Pts',(-15.9118084366381,13.6274932797063,
131.611137097283)) ;
#123030=CARTESIAN_POINT('Ctrl Pts',(-15.9167751273571,13.3375399739688,
131.592610463019)) ;
#123031=CARTESIAN_POINT('Ctrl Pts',(-15.9467825641615,13.0529654851711,
131.647157462469)) ;
#123032=CARTESIAN_POINT('Ctrl Pts',(-16.0009860132793,12.7935418575334,
131.77218792311)) ;
#123033=CARTESIAN_POINT('Ctrl Pts',(-16.0752207882529,12.5815360245405,
131.956050381901)) ;
#123034=CARTESIAN_POINT('Ctrl Pts',(-16.165618131101,12.4287257654979,132.187006003975)) ;
#123035=CARTESIAN_POINT('Ctrl Pts',(-16.2665986908856,12.3470719681604,
132.448782400074)) ;
#123036=CARTESIAN_POINT('Ctrl Pts',(-16.371126927041,12.3430683476044,132.720984392827)) ;
#123037=CARTESIAN_POINT('Ctrl Pts',(-16.4719895721837,12.4155936903918,
132.982699381913)) ;
#123038=CARTESIAN_POINT('Ctrl Pts',(-16.5641213124433,12.5608877107137,
133.218641097177)) ;
#123039=CARTESIAN_POINT('Ctrl Pts',(-16.64051349192,12.76729595803,133.408747345421)) ;
#123040=CARTESIAN_POINT('Ctrl Pts',(-16.6970812746958,13.021989825902,133.540754215802)) ;
#123041=CARTESIAN_POINT('Ctrl Pts',(-16.7298559652697,13.303543839919,133.603497574117)) ;
#123042=CARTESIAN_POINT('Ctrl Pts',(-16.7377714864704,13.5948424473805,
133.593472415343)) ;
#123043=CARTESIAN_POINT('Ctrl Pts',(-16.7206605383398,13.8739531403396,
133.510325245329)) ;
#123044=CARTESIAN_POINT('Ctrl Pts',(-16.6806111118358,14.1203175585331,
133.360220188526)) ;
#123045=CARTESIAN_POINT('Ctrl Pts',(-16.6212526466619,14.3167169570115,
133.15372717127)) ;
#123046=CARTESIAN_POINT('Ctrl Pts',(-16.5474137428711,14.4494067343281,
132.904886251952)) ;
#123047=CARTESIAN_POINT('Ctrl Pts',(-16.4651040331395,14.5084702765568,
132.631270940826)) ;
#123048=CARTESIAN_POINT('Ctrl Pts',(-16.381207376955,14.4897007225782,132.353087802305)) ;
#123049=CARTESIAN_POINT('Ctrl Pts',(-16.3022005550565,14.3946105615284,
132.089157332748)) ;
#123050=CARTESIAN_POINT('Ctrl Pts',(-16.2344715297939,14.2294634797175,
131.858114788284)) ;
#123051=CARTESIAN_POINT('Ctrl Pts',(-16.1839485347065,14.0073333338193,
131.677471929649)) ;
#123052=CARTESIAN_POINT('Ctrl Pts',(-16.1545348340837,13.743582797636,131.558487337903)) ;
#123053=CARTESIAN_POINT('Ctrl Pts',(-16.1492756367797,13.4548247152231,
131.509829227)) ;
#123054=CARTESIAN_POINT('Ctrl Pts',(-16.1692158859155,13.1663898310179,
131.53509076053)) ;
#123055=CARTESIAN_POINT('Ctrl Pts',(-16.2137083792206,12.8948251828515,
131.63190140386)) ;
#123056=CARTESIAN_POINT('Ctrl Pts',(-16.2803486569312,12.661361440579,131.79342760969)) ;
#123057=CARTESIAN_POINT('Ctrl Pts',(-16.3648242376105,12.4827884895572,
132.007122021634)) ;
#123058=CARTESIAN_POINT('Ctrl Pts',(-16.4621290434118,12.3713199015498,
132.258240175335)) ;
#123059=CARTESIAN_POINT('Ctrl Pts',(-16.5656958305595,12.3351536533699,
132.527714564387)) ;
#123060=CARTESIAN_POINT('Ctrl Pts',(-16.6694929915143,12.3771106009455,
132.79770710281)) ;
#123061=CARTESIAN_POINT('Ctrl Pts',(-16.7657977656074,12.4937460494275,
133.04598965838)) ;
#123062=CARTESIAN_POINT('Ctrl Pts',(-16.8492058389657,12.6767291591256,
133.256549538761)) ;
#123063=CARTESIAN_POINT('Ctrl Pts',(-16.9145312067199,12.9147363341255,
133.414096808471)) ;
#123064=CARTESIAN_POINT('Ctrl Pts',(-16.9570460781137,13.1870897744472,
133.505289820544)) ;
#123065=CARTESIAN_POINT('Ctrl Pts',(-16.9751986910918,13.4771403047647,
133.525201879438)) ;
#123066=CARTESIAN_POINT('Ctrl Pts',(-16.968053826777,13.7642377896945,133.47111354397)) ;
#123067=CARTESIAN_POINT('Ctrl Pts',(-16.9368413071542,14.0261140993903,
133.34678648386)) ;
#123068=CARTESIAN_POINT('Ctrl Pts',(-16.8850225105273,14.2437566933168,
133.16245913461)) ;
#123069=CARTESIAN_POINT('Ctrl Pts',(-16.8161456299396,14.4043005148666,
132.928011967567)) ;
#123070=CARTESIAN_POINT('Ctrl Pts',(-16.7367529131212,14.4936452056158,
132.66304467086)) ;
#123071=CARTESIAN_POINT('Ctrl Pts',(-16.6526808835843,14.5067755080675,
132.384315913876)) ;
#123072=CARTESIAN_POINT('Ctrl Pts',(-16.5707753130581,14.4421250993153,
132.111889673594)) ;
#123073=CARTESIAN_POINT('Ctrl Pts',(-16.4976974816868,14.3039890578845,
131.865211800435)) ;
#123074=CARTESIAN_POINT('Ctrl Pts',(-16.4397839505893,14.1040920585568,
131.663050653327)) ;
#123075=CARTESIAN_POINT('Ctrl Pts',(-16.4011325865525,13.8535850410252,
131.516876468062)) ;
#123076=CARTESIAN_POINT('Ctrl Pts',(-16.385954724659,13.573095030684,131.439416068659)) ;
#123077=CARTESIAN_POINT('Ctrl Pts',(-16.395634910027,13.2829859633842,131.434689671062)) ;
#123078=CARTESIAN_POINT('Ctrl Pts',(-16.4303004889498,13.0017735288795,
131.502829909788)) ;
#123079=CARTESIAN_POINT('Ctrl Pts',(-16.4885081607421,12.7500889121872,
131.639639946355)) ;
#123080=CARTESIAN_POINT('Ctrl Pts',(-16.5663528174175,12.5475576765503,
131.833937570297)) ;
#123081=CARTESIAN_POINT('Ctrl Pts',(-16.6592929614882,12.4075651763914,
132.072286468684)) ;
#123082=CARTESIAN_POINT('Ctrl Pts',(-16.7609250951473,12.3405227195362,
132.336146966397)) ;
#123083=CARTESIAN_POINT('Ctrl Pts',(-16.8654707864991,12.3506976033877,
132.608381377182)) ;
#123084=CARTESIAN_POINT('Ctrl Pts',(-16.9658202329978,12.4381775614935,
132.868330160183)) ;
#123085=CARTESIAN_POINT('Ctrl Pts',(-17.0551055310643,12.5958828969702,
133.096070183763)) ;
#123086=CARTESIAN_POINT('Ctrl Pts',(-17.1279925803926,12.8123888981795,
133.275937593456)) ;
#123087=CARTESIAN_POINT('Ctrl Pts',(-17.1802441869066,13.0732935402693,
133.395423875302)) ;
#123088=CARTESIAN_POINT('Ctrl Pts',(-17.2084980990116,13.3601445566741,
133.444717176536)) ;
#123089=CARTESIAN_POINT('Ctrl Pts',(-17.2115018031446,13.6487325565986,
133.420571161755)) ;
#123090=CARTESIAN_POINT('Ctrl Pts',(-17.1899377747894,13.9231969676619,
133.324422291905)) ;
#123091=CARTESIAN_POINT('Ctrl Pts',(-17.1459076362519,14.161664923211,133.162667592942)) ;
#123092=CARTESIAN_POINT('Ctrl Pts',(-17.0831501699344,14.3474885312589,
132.946120430805)) ;
#123093=CARTESIAN_POINT('Ctrl Pts',(-17.0074107794741,14.4664584642889,
132.691814732617)) ;
#123094=CARTESIAN_POINT('Ctrl Pts',(-16.9240118897558,14.5109046596075,
132.414920572147)) ;
#123095=CARTESIAN_POINT('Ctrl Pts',(-16.8409250151227,14.4775384051983,
132.139258966291)) ;
#123096=CARTESIAN_POINT('Ctrl Pts',(-16.7633048308355,14.3681997153804,
131.879250841701)) ;
#123097=CARTESIAN_POINT('Ctrl Pts',(-16.698669890579,14.1916180826176,131.657376441869)) ;
#123098=CARTESIAN_POINT('Ctrl Pts',(-16.6517651552372,13.9603525000671,
131.487287164895)) ;
#123099=CARTESIAN_POINT('Ctrl Pts',(-16.6267138914172,13.6895220896488,
131.380907935397)) ;
#123100=CARTESIAN_POINT('Ctrl Pts',(-16.6262261903022,13.4007319535163,
131.346419955467)) ;
#123101=CARTESIAN_POINT('Ctrl Pts',(-16.6508307815869,13.1132078069033,
131.385200211347)) ;
#123102=CARTESIAN_POINT('Ctrl Pts',(-16.7000127575053,12.846606824237,131.495596242918)) ;
#123103=CARTESIAN_POINT('Ctrl Pts',(-16.7699340004991,12.623698437481,131.6669249854)) ;
#123104=CARTESIAN_POINT('Ctrl Pts',(-16.8575811531176,12.4561011636242,
131.889737975163)) ;
#123105=CARTESIAN_POINT('Ctrl Pts',(-16.9565025908863,12.3585967931485,
132.145620482729)) ;
#123106=CARTESIAN_POINT('Ctrl Pts',(-17.0607608295923,12.3371246783343,
132.417041652335)) ;
#123107=CARTESIAN_POINT('Ctrl Pts',(-17.1634369259646,12.3935413864574,
132.683861422773)) ;
#123108=CARTESIAN_POINT('Ctrl Pts',(-17.2579099625892,12.5236724613545,
132.926727411168)) ;
#123109=CARTESIAN_POINT('Ctrl Pts',(-17.3381899050013,12.7179305396398,
133.128155534346)) ;
#123110=CARTESIAN_POINT('Ctrl Pts',(-17.3995267077133,12.9643002141067,
133.27404690597)) ;
#123111=CARTESIAN_POINT('Ctrl Pts',(-17.4374881845313,13.2410163015689,
133.351981082144)) ;
#123112=CARTESIAN_POINT('Ctrl Pts',(-17.4508755384222,13.5320328266363,
133.357960508206)) ;
#123113=CARTESIAN_POINT('Ctrl Pts',(-17.4391231761998,13.8151978209727,
133.29051487951)) ;
#123114=CARTESIAN_POINT('Ctrl Pts',(-17.4037054751815,14.0709652782984,
133.153839129592)) ;
#123115=CARTESIAN_POINT('Ctrl Pts',(-17.3480561457166,14.2795163173677,
132.958154017432)) ;
#123116=CARTESIAN_POINT('Ctrl Pts',(-17.2769868362532,14.4266234403896,
132.717472688248)) ;
#123117=CARTESIAN_POINT('Ctrl Pts',(-17.1961177738273,14.5021445242865,
132.448130239206)) ;
#123118=CARTESIAN_POINT('Ctrl Pts',(-17.1118876681302,14.5004798974739,
132.16892134338)) ;
#123119=CARTESIAN_POINT('Ctrl Pts',(-17.0310427991464,14.4210757518903,
131.899528163471)) ;
#123120=CARTESIAN_POINT('Ctrl Pts',(-16.9607834264823,14.2711636067417,
131.661303307297)) ;
#123121=CARTESIAN_POINT('Ctrl Pts',(-16.9059182551002,14.0600318658462,
131.467885599582)) ;
#123122=CARTESIAN_POINT('Ctrl Pts',(-16.8715689169995,13.8025044724255,
131.334333695269)) ;
#123123=CARTESIAN_POINT('Ctrl Pts',(-16.8609448001921,13.5194348559979,
131.270285840575)) ;
#123124=CARTESIAN_POINT('Ctrl Pts',(-16.8754425519544,13.2279296915562,
131.279438819765)) ;
#123125=CARTESIAN_POINT('Ctrl Pts',(-16.9146883120641,12.9514278673655,
131.361017100262)) ;
#123126=CARTESIAN_POINT('Ctrl Pts',(-16.9769612891766,12.7076269304905,
131.509703903638)) ;
#123127=CARTESIAN_POINT('Ctrl Pts',(-17.0577658489045,12.5164543303433,
131.712752029851)) ;
#123128=CARTESIAN_POINT('Ctrl Pts',(-17.1530301116951,12.3891143614251,
131.957830660672)) ;
#123129=CARTESIAN_POINT('Ctrl Pts',(-17.255826018226,12.3364756135891,132.22503445106)) ;
#123130=CARTESIAN_POINT('Ctrl Pts',(-17.3598675535299,12.3612642379946,
132.495867624495)) ;
#123131=CARTESIAN_POINT('Ctrl Pts',(-17.4588984356061,12.4629839046161,
132.751884061504)) ;
#123132=CARTESIAN_POINT('Ctrl Pts',(-17.5451750061563,12.6321971909499,
132.97096084242)) ;
#123133=CARTESIAN_POINT('Ctrl Pts',(-17.6146347409835,12.8584558944589,
133.140756526335)) ;
#123134=CARTESIAN_POINT('Ctrl Pts',(-17.6625907018637,13.126164869302,133.247632658704)) ;
#123135=CARTESIAN_POINT('Ctrl Pts',(-17.686067276807,13.4141234527586,133.283124808462)) ;
#123136=CARTESIAN_POINT('Ctrl Pts',(-17.6844047923767,13.7023852281616,
133.24521446728)) ;
#123137=CARTESIAN_POINT('Ctrl Pts',(-17.6584006494406,13.9714211958417,
133.136118653712)) ;
#123138=CARTESIAN_POINT('Ctrl Pts',(-17.6102464362103,14.2020200814189,
132.962158529894)) ;
#123139=CARTESIAN_POINT('Ctrl Pts',(-17.5449058959592,14.3750071777218,
132.73827371451)) ;
#123140=CARTESIAN_POINT('Ctrl Pts',(-17.4673010855026,14.4806351397631,
132.478490433168)) ;
#123141=CARTESIAN_POINT('Ctrl Pts',(-17.3835397579498,14.5105855300703,
132.200638006031)) ;
#123142=CARTESIAN_POINT('Ctrl Pts',(-17.30068437579,14.4625550533332,131.925476858829)) ;
#123143=CARTESIAN_POINT('Ctrl Pts',(-17.2252675417554,14.3400369090667,
131.67203480792)) ;
#123144=CARTESIAN_POINT('Ctrl Pts',(-17.1635231504772,14.1521956958397,
131.458588071982)) ;
#123145=CARTESIAN_POINT('Ctrl Pts',(-17.1203550453216,13.9116488292757,
131.299323606361)) ;
#123146=CARTESIAN_POINT('Ctrl Pts',(-17.0998333313807,13.6358543135724,
131.206201276277)) ;
#123147=CARTESIAN_POINT('Ctrl Pts',(-17.1040414218408,13.3459426369887,
131.18545101084)) ;
#123148=CARTESIAN_POINT('Ctrl Pts',(-17.1334554147273,13.0604648346963,
131.238204781291)) ;
#123149=CARTESIAN_POINT('Ctrl Pts',(-17.186635109894,12.8015142493302,131.360449631812)) ;
#123150=CARTESIAN_POINT('Ctrl Pts',(-17.2605647433702,12.5868713096869,
131.543281201559)) ;
#123151=CARTESIAN_POINT('Ctrl Pts',(-17.3505844000603,12.432303139715,131.773142925006)) ;
#123152=CARTESIAN_POINT('Ctrl Pts',(-17.450995478009,12.3486039806668,132.033365539858)) ;
#123153=CARTESIAN_POINT('Ctrl Pts',(-17.5555454936255,12.3418345477554,
132.305622555726)) ;
#123154=CARTESIAN_POINT('Ctrl Pts',(-17.6572109198033,12.4127258480294,
132.569475130721)) ;
#123155=CARTESIAN_POINT('Ctrl Pts',(-17.74925550764,12.5554431662894,132.805322541401)) ;
#123156=CARTESIAN_POINT('Ctrl Pts',(-17.8264454858064,12.7608030962308,
132.99765025968)) ;
#123157=CARTESIAN_POINT('Ctrl Pts',(-17.8835674879356,13.0143081230203,
133.131299482817)) ;
#123158=CARTESIAN_POINT('Ctrl Pts',(-17.9170703055575,13.29536631424,133.196160960181)) ;
#123159=CARTESIAN_POINT('Ctrl Pts',(-17.9256862762086,13.5874993963847,
133.18809411502)) ;
#123160=CARTESIAN_POINT('Ctrl Pts',(-17.9091691179215,13.8669340437894,
133.106704940277)) ;
#123161=CARTESIAN_POINT('Ctrl Pts',(-17.8699206134807,14.1134264974216,
132.959083300844)) ;
#123162=CARTESIAN_POINT('Ctrl Pts',(-17.8109235413731,14.312178191849,132.753550467114)) ;
#123163=CARTESIAN_POINT('Ctrl Pts',(-17.7371490293014,14.447005080599,132.504799591305)) ;
#123164=CARTESIAN_POINT('Ctrl Pts',(-17.6551253369284,14.50780864275,132.23208223908)) ;
#123165=CARTESIAN_POINT('Ctrl Pts',(-17.5714598174354,14.4913412466958,
131.954681845237)) ;
#123166=CARTESIAN_POINT('Ctrl Pts',(-17.4922372650921,14.3985298499944,
131.690131300663)) ;
#123167=CARTESIAN_POINT('Ctrl Pts',(-17.4240290431123,14.23537642446,131.457680674098)) ;
#123168=CARTESIAN_POINT('Ctrl Pts',(-17.372717665545,14.0132823702427,131.27454472913)) ;
#123169=CARTESIAN_POINT('Ctrl Pts',(-17.3429068898243,13.7517705184138,
131.154578961015)) ;
#123170=CARTESIAN_POINT('Ctrl Pts',(-17.3368035221446,13.4639004109061,
131.103505978631)) ;
#123171=CARTESIAN_POINT('Ctrl Pts',(-17.3561906073303,13.1736259239267,
131.126963588793)) ;
#123172=CARTESIAN_POINT('Ctrl Pts',(-17.399754261981,12.9029494163379,131.221266592512)) ;
#123173=CARTESIAN_POINT('Ctrl Pts',(-17.4659861489072,12.6670694779248,
131.381471376982)) ;
#123174=CARTESIAN_POINT('Ctrl Pts',(-17.5502293174444,12.4867414541686,
131.594432437116)) ;
#123175=CARTESIAN_POINT('Ctrl Pts',(-17.6467937329341,12.3736046966953,
131.843541552857)) ;
#123176=CARTESIAN_POINT('Ctrl Pts',(-17.7508568587286,12.3351061358333,
132.114275541439)) ;
#123177=CARTESIAN_POINT('Ctrl Pts',(-17.8540445547543,12.3747297398712,
132.382714038541)) ;
#123178=CARTESIAN_POINT('Ctrl Pts',(-17.9508908372742,12.4890530278271,
132.632514940323)) ;
#123179=CARTESIAN_POINT('Ctrl Pts',(-18.0352482217783,12.671847392328,132.845621204235)) ;
#123180=CARTESIAN_POINT('Ctrl Pts',(-18.1006691599388,12.9071471276995,
133.003666438983)) ;
#123181=CARTESIAN_POINT('Ctrl Pts',(-18.1439831889663,13.1791584028572,
133.097130182838)) ;
#123182=CARTESIAN_POINT('Ctrl Pts',(-18.1627954327558,13.4685703859445,
133.119024093136)) ;
#123183=CARTESIAN_POINT('Ctrl Pts',(-18.1564134876139,13.7556866314948,
133.067206763249)) ;
#123184=CARTESIAN_POINT('Ctrl Pts',(-18.12597352168,14.0184521546514,132.945168227283)) ;
#123185=CARTESIAN_POINT('Ctrl Pts',(-18.0744435558841,14.2386836272176,
132.761515544376)) ;
#123186=CARTESIAN_POINT('Ctrl Pts',(-18.005953850359,14.4009245820624,132.528213465536)) ;
#123187=CARTESIAN_POINT('Ctrl Pts',(-17.9265298697312,14.4923209355322,
132.263056140391)) ;
#123188=CARTESIAN_POINT('Ctrl Pts',(-17.8429057727029,14.5074993707076,
131.985805363542)) ;
#123189=CARTESIAN_POINT('Ctrl Pts',(-17.7605057976756,14.4446390736038,
131.711788345313)) ;
#123190=CARTESIAN_POINT('Ctrl Pts',(-17.6874814954345,14.3090137807522,
131.465438769024)) ;
#123191=CARTESIAN_POINT('Ctrl Pts',(-17.6289271492235,14.1104147854154,
131.261333528496)) ;
#123192=CARTESIAN_POINT('Ctrl Pts',(-17.5897575642381,13.8614586698981,
131.113706749861)) ;
#123193=CARTESIAN_POINT('Ctrl Pts',(-17.5738212671254,13.5819684927305,
131.034067733009)) ;
#123194=CARTESIAN_POINT('Ctrl Pts',(-17.5828139968281,13.2906276884224,
131.027193171422)) ;
#123195=CARTESIAN_POINT('Ctrl Pts',(-17.616848627643,13.0092431055299,131.093525306334)) ;
#123196=CARTESIAN_POINT('Ctrl Pts',(-17.6740860340513,12.7575166399562,
131.227660746191)) ;
#123197=CARTESIAN_POINT('Ctrl Pts',(-17.7516753463476,12.5525238857448,
131.421087178671)) ;
#123198=CARTESIAN_POINT('Ctrl Pts',(-17.8440081329895,12.4108769573351,
131.657753073151)) ;
#123199=CARTESIAN_POINT('Ctrl Pts',(-17.9458175434282,12.3412908932615,
131.922013087473)) ;
#123200=CARTESIAN_POINT('Ctrl Pts',(-18.0502423166348,12.3493862056845,
132.193940570029)) ;
#123201=CARTESIAN_POINT('Ctrl Pts',(-18.1505364662407,12.434272868394,132.453821578147)) ;
#123202=CARTESIAN_POINT('Ctrl Pts',(-18.240385583011,12.5900490117304,132.683164341833)) ;
#123203=CARTESIAN_POINT('Ctrl Pts',(-18.3140154660262,12.8056267290578,
132.865114759058)) ;
#123204=CARTESIAN_POINT('Ctrl Pts',(-18.366813447899,13.065385008078,132.986222365065)) ;
#123205=CARTESIAN_POINT('Ctrl Pts',(-18.3957716324573,13.3504852311182,
133.03771979281)) ;
#123206=CARTESIAN_POINT('Ctrl Pts',(-18.3995519707308,13.6412799194347,
133.015607297531)) ;
#123207=CARTESIAN_POINT('Ctrl Pts',(-18.3786631552861,13.9155482376954,
132.921539059482)) ;
#123208=CARTESIAN_POINT('Ctrl Pts',(-18.3352864113963,14.1552942576475,
132.761699945438)) ;
#123209=CARTESIAN_POINT('Ctrl Pts',(-18.2730232374163,14.3429102218091,
132.546604772936)) ;
#123210=CARTESIAN_POINT('Ctrl Pts',(-18.1974878680021,14.4639893151741,
132.292852310958)) ;
#123211=CARTESIAN_POINT('Ctrl Pts',(-18.1145512503383,14.5107279947802,
132.017447527145)) ;
#123212=CARTESIAN_POINT('Ctrl Pts',(-18.0309330183496,14.4794893711203,
131.74005057923)) ;
#123213=CARTESIAN_POINT('Ctrl Pts',(-17.9533998997489,14.3727211556821,
131.480454525081)) ;
#123214=CARTESIAN_POINT('Ctrl Pts',(-17.8881494032496,14.1977799605459,
131.256709819831)) ;
#123215=CARTESIAN_POINT('Ctrl Pts',(-17.84064942172,13.9680803092071,131.08490378882)) ;
#123216=CARTESIAN_POINT('Ctrl Pts',(-17.8148397147958,13.6967826979273,
130.976149136345)) ;
#123217=CARTESIAN_POINT('Ctrl Pts',(-17.8136790517629,13.4094043760134,
130.939833355752)) ;
#123218=CARTESIAN_POINT('Ctrl Pts',(-17.8375788446251,13.1212039235338,
130.976511139861)) ;
#123219=CARTESIAN_POINT('Ctrl Pts',(-17.8858674033282,12.8546896055266,
131.084429899433)) ;
#123220=CARTESIAN_POINT('Ctrl Pts',(-17.955361853148,12.6293810119528,131.254404916973)) ;
#123221=CARTESIAN_POINT('Ctrl Pts',(-18.0430537668622,12.4594635136683,
131.477196723744)) ;
#123222=CARTESIAN_POINT('Ctrl Pts',(-18.1412332588082,12.3604529147884,
131.731084274018)) ;
#123223=CARTESIAN_POINT('Ctrl Pts',(-18.2457684052727,12.3366695110087,
132.003204681306)) ;
#123224=CARTESIAN_POINT('Ctrl Pts',(-18.3481468441055,12.3907630911244,
132.269294142436)) ;
#123225=CARTESIAN_POINT('Ctrl Pts',(-18.4431476781956,12.5187718172597,
132.513649957328)) ;
#123226=CARTESIAN_POINT('Ctrl Pts',(-18.5241808191143,12.7125554078675,
132.717126113492)) ;
#123227=CARTESIAN_POINT('Ctrl Pts',(-18.5855196122855,12.9551209833767,
132.863367722393)) ;
#123228=CARTESIAN_POINT('Ctrl Pts',(-18.6245679674523,13.2325621685243,
132.944286617486)) ;
#123229=CARTESIAN_POINT('Ctrl Pts',(-18.6386186599524,13.5243421587289,
132.952113131439)) ;
#123230=CARTESIAN_POINT('Ctrl Pts',(-18.6275981947546,13.8069928303566,
132.886922542916)) ;
#123231=CARTESIAN_POINT('Ctrl Pts',(-18.5928710094331,14.0639001821586,
132.752263942652)) ;
#123232=CARTESIAN_POINT('Ctrl Pts',(-18.5377610477976,14.274156022816,132.558149542648)) ;
#123233=CARTESIAN_POINT('Ctrl Pts',(-18.4669022465602,14.4234616465823,
132.318009347732)) ;
#123234=CARTESIAN_POINT('Ctrl Pts',(-18.3863158160937,14.5011170980349,
132.049535240517)) ;
#123235=CARTESIAN_POINT('Ctrl Pts',(-18.3017727099702,14.501361448933,131.769280894779)) ;
#123236=CARTESIAN_POINT('Ctrl Pts',(-18.2214649543661,14.4249955787507,
131.501768767885)) ;
#123237=CARTESIAN_POINT('Ctrl Pts',(-18.1501883393521,14.2760170248169,
131.260290403675)) ;
#123238=CARTESIAN_POINT('Ctrl Pts',(-18.0950241994089,14.0665440737742,
131.066070425009)) ;
#123239=CARTESIAN_POINT('Ctrl Pts',(-18.0600356895942,13.8110526556412,
130.930755576535)) ;
#123240=CARTESIAN_POINT('Ctrl Pts',(-18.0487031148571,13.5262784611541,
130.864382352007)) ;
#123241=CARTESIAN_POINT('Ctrl Pts',(-18.062412239786,13.2368368163846,130.871485132988)) ;
#123242=CARTESIAN_POINT('Ctrl Pts',(-18.1011540315473,12.9583254451164,
130.951421021167)) ;
#123243=CARTESIAN_POINT('Ctrl Pts',(-18.162442619362,12.7145798984787,131.097428040088)) ;
#123244=CARTESIAN_POINT('Ctrl Pts',(-18.2435317670333,12.5201729680917,
131.301002269112)) ;
#123245=CARTESIAN_POINT('Ctrl Pts',(-18.3374905555791,12.3922976801848,
131.542627125827)) ;
#123246=CARTESIAN_POINT('Ctrl Pts',(-18.4407097729528,12.3368042006491,
131.810872082474)) ;
#123247=CARTESIAN_POINT('Ctrl Pts',(-18.5444741358057,12.3594079761625,
132.081007895545)) ;
#123248=CARTESIAN_POINT('Ctrl Pts',(-18.6438726401263,12.458842653819,132.338064760412)) ;
#123249=CARTESIAN_POINT('Ctrl Pts',(-18.730666683213,12.6263833262832,132.5586223689)) ;
#123250=CARTESIAN_POINT('Ctrl Pts',(-18.8006930563816,12.8513078347283,
132.730062824088)) ;
#123251=CARTESIAN_POINT('Ctrl Pts',(-18.8492688728646,13.1175342113745,
132.838816465767)) ;
#123252=CARTESIAN_POINT('Ctrl Pts',(-18.8735376930888,13.4059955031651,
132.876522375954)) ;
#123253=CARTESIAN_POINT('Ctrl Pts',(-18.8726310881695,13.6942419631863,
132.840864257295)) ;
#123254=CARTESIAN_POINT('Ctrl Pts',(-18.846988455619,13.9656571301542,132.732603873144)) ;
#123255=CARTESIAN_POINT('Ctrl Pts',(-18.800060785329,14.1945698171883,132.562678543483)) ;
#123256=CARTESIAN_POINT('Ctrl Pts',(-18.7347749337685,14.3711224521538,
132.338694883308)) ;
#123257=CARTESIAN_POINT('Ctrl Pts',(-18.657438019017,14.4785950112144,132.079716383706)) ;
#123258=CARTESIAN_POINT('Ctrl Pts',(-18.5736714267936,14.5108133119048,
131.801809937082)) ;
#123259=CARTESIAN_POINT('Ctrl Pts',(-18.4908489270132,14.465039412922,131.52680696157)) ;
#123260=CARTESIAN_POINT('Ctrl Pts',(-18.4151408888549,14.3446919180205,
131.272521239877)) ;
#123261=CARTESIAN_POINT('Ctrl Pts',(-18.3528650039776,14.1586507475217,
131.057514981106)) ;
#123262=CARTESIAN_POINT('Ctrl Pts',(-18.3089775079518,13.9182141888542,
130.896003116198)) ;
#123263=CARTESIAN_POINT('Ctrl Pts',(-18.287897911152,13.6446893381856,130.801441722976)) ;
#123264=CARTESIAN_POINT('Ctrl Pts',(-18.29136911731,13.3538162430507,130.778406138012)) ;
#123265=CARTESIAN_POINT('Ctrl Pts',(-18.320015418867,13.0687528103835,130.829019791888)) ;
#123266=CARTESIAN_POINT('Ctrl Pts',(-18.3725780715655,12.808402450481,130.949417001428)) ;
#123267=CARTESIAN_POINT('Ctrl Pts',(-18.4459344258757,12.5923661463697,
131.130592731019)) ;
#123268=CARTESIAN_POINT('Ctrl Pts',(-18.5356977693632,12.4355966192842,
131.359653802566)) ;
#123269=CARTESIAN_POINT('Ctrl Pts',(-18.6360919268662,12.3498833858894,
131.619771018926)) ;
#123270=CARTESIAN_POINT('Ctrl Pts',(-18.7400873983312,12.3409543002999,
131.890577260411)) ;
#123271=CARTESIAN_POINT('Ctrl Pts',(-18.8420016780614,12.4093757985287,
132.155139312292)) ;
#123272=CARTESIAN_POINT('Ctrl Pts',(-18.9346544889553,12.5505197572112,
132.392675801306)) ;
#123273=CARTESIAN_POINT('Ctrl Pts',(-19.0122360971197,12.7541804700571,
132.586179998705)) ;
#123274=CARTESIAN_POINT('Ctrl Pts',(-19.0698650565518,13.0055269427028,
132.721428807461)) ;
#123275=CARTESIAN_POINT('Ctrl Pts',(-19.1042443289156,13.2870727031463,
132.788720725117)) ;
#123276=CARTESIAN_POINT('Ctrl Pts',(-19.1135598388478,13.5781356431356,
132.782823251789)) ;
#123277=CARTESIAN_POINT('Ctrl Pts',(-19.0978920623825,13.8583664416102,
132.70391043962)) ;
#123278=CARTESIAN_POINT('Ctrl Pts',(-19.0590725975324,14.1072756620479,
132.557379585171)) ;
#123279=CARTESIAN_POINT('Ctrl Pts',(-19.0006930075818,14.3069767003197,
132.35374086841)) ;
#123280=CARTESIAN_POINT('Ctrl Pts',(-18.9276024226959,14.4436141295833,
132.107115025737)) ;
#123281=CARTESIAN_POINT('Ctrl Pts',(-18.845475368495,14.5071928211091,131.833981429736)) ;
#123282=CARTESIAN_POINT('Ctrl Pts',(-18.7615750440561,14.4928944928021,
131.555820733646)) ;
#123283=CARTESIAN_POINT('Ctrl Pts',(-18.6821529870225,14.4021254320443,
131.290693534934)) ;
#123284=CARTESIAN_POINT('Ctrl Pts',(-18.6137276419482,14.2413769659717,
131.057704478338)) ;
#123285=CARTESIAN_POINT('Ctrl Pts',(-18.5617948270631,14.0210257728375,
130.872760524719)) ;
#123286=CARTESIAN_POINT('Ctrl Pts',(-18.5311748689287,13.7594507578406,
130.75030009395)) ;
#123287=CARTESIAN_POINT('Ctrl Pts',(-18.524462743248,13.4716752359127,130.697418025673)) ;
#123288=CARTESIAN_POINT('Ctrl Pts',(-18.5429559165933,13.1827800209618,
130.718450895566)) ;
#123289=CARTESIAN_POINT('Ctrl Pts',(-18.5860682542042,12.9097866027274,
130.811247666085)) ;
#123290=CARTESIAN_POINT('Ctrl Pts',(-18.6513547850338,12.6739760958484,
130.968882762111)) ;
#123291=CARTESIAN_POINT('Ctrl Pts',(-18.7352113453907,12.4911376309814,
131.180647458982)) ;
#123292=CARTESIAN_POINT('Ctrl Pts',(-18.8320450972457,12.375575879239,131.430367588562)) ;
#123293=CARTESIAN_POINT('Ctrl Pts',(-18.9353885585262,12.3352662333604,
131.699197648249)) ;
#123294=CARTESIAN_POINT('Ctrl Pts',(-19.0388002165836,12.3722006124299,
131.968259729985)) ;
#123295=CARTESIAN_POINT('Ctrl Pts',(-19.13663271086,12.4858118700224,132.220677550879)) ;
#123296=CARTESIAN_POINT('Ctrl Pts',(-19.2204826471649,12.6649628036957,
132.432670825365)) ;
#123297=CARTESIAN_POINT('Ctrl Pts',(-19.2868586701222,12.8995424395387,
132.593375480178)) ;
#123298=CARTESIAN_POINT('Ctrl Pts',(-19.3308236821031,13.1707490219764,
132.688750556029)) ;
#123299=CARTESIAN_POINT('Ctrl Pts',(-19.3504090557961,13.4602465795,132.7128657881)) ;
#123300=CARTESIAN_POINT('Ctrl Pts',(-19.3447038706074,13.7479094630808,
132.663005441202)) ;
#123301=CARTESIAN_POINT('Ctrl Pts',(-19.3149883980574,14.0110934234083,
132.543151049153)) ;
#123302=CARTESIAN_POINT('Ctrl Pts',(-19.2640132574358,14.233019589697,132.361099714617)) ;
#123303=CARTESIAN_POINT('Ctrl Pts',(-19.1959166618581,14.3970564643661,
132.128942413442)) ;
#123304=CARTESIAN_POINT('Ctrl Pts',(-19.1169952616353,14.4906411189315,
131.865358043899)) ;
#123305=CARTESIAN_POINT('Ctrl Pts',(-19.0328798147139,14.5080280038905,
131.586455112218)) ;
#123306=CARTESIAN_POINT('Ctrl Pts',(-18.9510735202354,14.4480724922228,
131.314485578695)) ;
#123307=CARTESIAN_POINT('Ctrl Pts',(-18.8771616284183,14.3139469642534,
131.065316852607)) ;
#123308=CARTESIAN_POINT('Ctrl Pts',(-18.8181485060677,14.1169436134283,
130.859887328916)) ;
#123309=CARTESIAN_POINT('Ctrl Pts',(-18.7782906077968,13.8684680278967,
130.710158901743)) ;
#123310=CARTESIAN_POINT('Ctrl Pts',(-18.7617532070724,13.5907241662415,
130.628902383612)) ;
#123311=CARTESIAN_POINT('Ctrl Pts',(-18.7699529682382,13.2994060447749,
130.619705093688)) ;
#123312=CARTESIAN_POINT('Ctrl Pts',(-18.8032396782026,13.0173300828137,
130.683845657523)) ;
#123313=CARTESIAN_POINT('Ctrl Pts',(-18.8601088458043,12.7634585275692,
130.816765455538)) ;
#123314=CARTESIAN_POINT('Ctrl Pts',(-18.9371406149224,12.5574052301983,
131.008613631546)) ;
#123315=CARTESIAN_POINT('Ctrl Pts',(-19.0288519820687,12.4141337315889,
131.243554207896)) ;
#123316=CARTESIAN_POINT('Ctrl Pts',(-19.13057401488,12.3422331852162,131.507526439382)) ;
#123317=CARTESIAN_POINT('Ctrl Pts',(-19.2349019043779,12.3479816705834,
131.779210106818)) ;
#123318=CARTESIAN_POINT('Ctrl Pts',(-19.3355608700303,12.4308509408022,
132.04010176436)) ;
#123319=CARTESIAN_POINT('Ctrl Pts',(-19.4255699007721,12.5841343909331,
132.27001036361)) ;
#123320=CARTESIAN_POINT('Ctrl Pts',(-19.5000791880127,12.7991565720161,
132.454374408853)) ;
#123321=CARTESIAN_POINT('Ctrl Pts',(-19.5533212332608,13.0570001115815,
132.576901554063)) ;
#123322=CARTESIAN_POINT('Ctrl Pts',(-19.5830699103574,13.3421922466227,
132.63063668358)) ;
#123323=CARTESIAN_POINT('Ctrl Pts',(-19.5876133607077,13.6321455836602,
132.610870942847)) ;
#123324=CARTESIAN_POINT('Ctrl Pts',(-19.5673218035565,13.9089726379876,
132.518333296573)) ;
#123325=CARTESIAN_POINT('Ctrl Pts',(-19.5243599298239,14.1498189010042,
132.359684334784)) ;
#123326=CARTESIAN_POINT('Ctrl Pts',(-19.4629860879287,14.3379335627546,
132.147406052705)) ;
#123327=CARTESIAN_POINT('Ctrl Pts',(-19.3875690527456,14.4615825928275,
131.893901802472)) ;
#123328=CARTESIAN_POINT('Ctrl Pts',(-19.3048022308788,14.5104718340286,
131.619017490043)) ;
#123329=CARTESIAN_POINT('Ctrl Pts',(-19.2208867293053,14.4813917007992,
131.340664971881)) ;
#123330=CARTESIAN_POINT('Ctrl Pts',(-19.1431505631515,14.376410140061,131.080480626318)) ;
#123331=CARTESIAN_POINT('Ctrl Pts',(-19.0776968905506,14.2041612959408,
130.856285283201)) ;
#123332=CARTESIAN_POINT('Ctrl Pts',(-19.0293984514368,13.974383981629,130.68194601526)) ;
#123333=CARTESIAN_POINT('Ctrl Pts',(-19.0031038029563,13.7063210465707,
130.572069348957)) ;
#123334=CARTESIAN_POINT('Ctrl Pts',(-19.001145721614,13.4167011729611,130.533125822564)) ;
#123335=CARTESIAN_POINT('Ctrl Pts',(-19.0243797093888,13.1291677764475,
130.5679716419)) ;
#123336=CARTESIAN_POINT('Ctrl Pts',(-19.0719631831347,12.8617102719658,
130.673828410007)) ;
#123337=CARTESIAN_POINT('Ctrl Pts',(-19.1409679175638,12.6350478347594,
130.842360735363)) ;
#123338=CARTESIAN_POINT('Ctrl Pts',(-19.2278027464721,12.4638699496821,
131.062798616732)) ;
#123339=CARTESIAN_POINT('Ctrl Pts',(-19.3262245567786,12.3621126749229,
131.317221532993)) ;
#123340=CARTESIAN_POINT('Ctrl Pts',(-19.430537761891,12.336288295009,131.58874825821)) ;
#123341=CARTESIAN_POINT('Ctrl Pts',(-19.5332636656819,12.3882079371413,
131.855786779012)) ;
#123342=CARTESIAN_POINT('Ctrl Pts',(-19.6286546086938,12.5148240574062,
132.101228597858)) ;
#123343=CARTESIAN_POINT('Ctrl Pts',(-19.7095188083265,12.7050813508199,
132.304501505355)) ;
#123344=CARTESIAN_POINT('Ctrl Pts',(-19.7720060707541,12.9482678416441,
132.453826841834)) ;
#123345=CARTESIAN_POINT('Ctrl Pts',(-19.8115111558353,13.2238579668187,
132.536233557694)) ;
#123346=CARTESIAN_POINT('Ctrl Pts',(-19.8263700093836,13.5162934097049,
132.546326795299)) ;
#123347=CARTESIAN_POINT('Ctrl Pts',(-19.8160540554796,13.7991654054394,
132.483232272363)) ;
#123348=CARTESIAN_POINT('Ctrl Pts',(-19.7817797053596,14.0580269319691,
132.349765095749)) ;
#123349=CARTESIAN_POINT('Ctrl Pts',(-19.7274211509896,14.2686029381806,
132.158015292144)) ;
#123350=CARTESIAN_POINT('Ctrl Pts',(-19.6570350610866,14.419961933364,131.919277312271)) ;
#123351=CARTESIAN_POINT('Ctrl Pts',(-19.5765562400787,14.49989585267,131.651079261874)) ;
#123352=CARTESIAN_POINT('Ctrl Pts',(-19.4921101780105,14.5025664525356,
131.371149134813)) ;
#123353=CARTESIAN_POINT('Ctrl Pts',(-19.4113969608343,14.4280651994865,
131.102354695495)) ;
#123354=CARTESIAN_POINT('Ctrl Pts',(-19.3400486586853,14.2819176182956,
130.860829298988)) ;
#123355=CARTESIAN_POINT('Ctrl Pts',(-19.2839264131876,14.0723875526179,
130.663547795459)) ;
#123356=CARTESIAN_POINT('Ctrl Pts',(-19.2485926616992,13.8191593341655,
130.527403742645)) ;
#123357=CARTESIAN_POINT('Ctrl Pts',(-19.2364478765941,13.5356700868247,
130.458732004174)) ;
#123358=CARTESIAN_POINT('Ctrl Pts',(-19.2494300922433,13.2451624741664,
130.463600209638)) ;
#123359=CARTESIAN_POINT('Ctrl Pts',(-19.2874907120602,12.9658957798679,
130.541539493339)) ;
#123360=CARTESIAN_POINT('Ctrl Pts',(-19.3482532948302,12.7208678253265,
130.685983671784)) ;
#123361=CARTESIAN_POINT('Ctrl Pts',(-19.4283743567801,12.5256177762791,
130.886907898066)) ;
#123362=CARTESIAN_POINT('Ctrl Pts',(-19.5225746037128,12.3947248965929,
131.129026992541)) ;
#123363=CARTESIAN_POINT('Ctrl Pts',(-19.6256543536979,12.3373274071284,
131.396874484283)) ;
#123364=CARTESIAN_POINT('Ctrl Pts',(-19.7292828586896,12.3577351595859,
131.666668741082)) ;
#123365=CARTESIAN_POINT('Ctrl Pts',(-19.828747484538,12.4546492902735,131.923987738611)) ;
#123366=CARTESIAN_POINT('Ctrl Pts',(-19.9163629094891,12.6210677035252,
132.146795892703)) ;
#123367=CARTESIAN_POINT('Ctrl Pts',(-19.9868245592564,12.8446767267699,
132.319524452122)) ;
#123368=CARTESIAN_POINT('Ctrl Pts',(-20.0358951637964,13.1088081967542,
132.429861713404)) ;
#123369=CARTESIAN_POINT('Ctrl Pts',(-20.0610202092485,13.3979062800969,
132.469955286352)) ;
#123370=CARTESIAN_POINT('Ctrl Pts',(-20.0607325832847,13.6859097693729,
132.436152367253)) ;
#123371=CARTESIAN_POINT('Ctrl Pts',(-20.0361182928156,13.9567565274245,
132.331106427657)) ;
#123372=CARTESIAN_POINT('Ctrl Pts',(-19.989134080272,14.1899349081331,132.160581855048)) ;
#123373=CARTESIAN_POINT('Ctrl Pts',(-19.9249163191982,14.3662692594446,
131.940072508991)) ;
#123374=CARTESIAN_POINT('Ctrl Pts',(-19.8473720747076,14.4768289977238,
131.680256103619)) ;
#123375=CARTESIAN_POINT('Ctrl Pts',(-19.7638911381145,14.5109207097569,
131.403278553501)) ;
#123376=CARTESIAN_POINT('Ctrl Pts',(-19.6808599303053,14.4673589922836,
131.127620946744)) ;
#123377=CARTESIAN_POINT('Ctrl Pts',(-19.6048776341735,14.3490297985362,
130.87254760327)) ;
#123378=CARTESIAN_POINT('Ctrl Pts',(-19.5421323663737,14.1643442277036,
130.65613213943)) ;
#123379=CARTESIAN_POINT('Ctrl Pts',(-19.4978928252363,13.9269540267458,
130.493822267582)) ;
#123380=CARTESIAN_POINT('Ctrl Pts',(-19.4759282474524,13.6529086343547,
130.396504933955)) ;
#123381=CARTESIAN_POINT('Ctrl Pts',(-19.4786884736238,13.3625039506586,
130.371432632605)) ;
#123382=CARTESIAN_POINT('Ctrl Pts',(-19.5066515881235,13.0764916582392,
130.419989164608)) ;
#123383=CARTESIAN_POINT('Ctrl Pts',(-19.5585742647346,12.8152456791565,
130.538527912325)) ;
#123384=CARTESIAN_POINT('Ctrl Pts',(-19.6313995735152,12.5977359905825,
130.718150203984)) ;
#123385=CARTESIAN_POINT('Ctrl Pts',(-19.7206731960293,12.439230107941,130.945816992587)) ;
#123386=CARTESIAN_POINT('Ctrl Pts',(-19.8208275253365,12.3513755687183,
131.205236892769)) ;
#123387=CARTESIAN_POINT('Ctrl Pts',(-19.9247572807901,12.339931649505,131.475869177705)) ;
#123388=CARTESIAN_POINT('Ctrl Pts',(-20.0275777885888,12.4070555048895,
131.742824520254)) ;
#123389=CARTESIAN_POINT('Ctrl Pts',(-20.1196954087276,12.5451371061637,
131.979106081002)) ;
#123390=CARTESIAN_POINT('Ctrl Pts',(-20.1981516956985,12.7477728516222,
132.175029811803)) ;
#123391=CARTESIAN_POINT('Ctrl Pts',(-20.256324633919,12.9979369346779,132.311891349811)) ;
#123392=CARTESIAN_POINT('Ctrl Pts',(-20.2914356628922,13.2792373127526,
132.38127965356)) ;
#123393=CARTESIAN_POINT('Ctrl Pts',(-20.3014130100161,13.570158269964,132.377333641783)) ;
#123394=CARTESIAN_POINT('Ctrl Pts',(-20.286471936004,13.850537969179,132.300597227172)) ;
#123395=CARTESIAN_POINT('Ctrl Pts',(-20.2482660446986,14.1007514006134,
132.155840929195)) ;
#123396=CARTESIAN_POINT('Ctrl Pts',(-20.1903697230178,14.302171677131,131.953602989605)) ;
#123397=CARTESIAN_POINT('Ctrl Pts',(-20.1173842617992,14.4410638896651,
131.707187218307)) ;
#123398=CARTESIAN_POINT('Ctrl Pts',(-20.0354743272129,14.5064205925433,
131.434719899531)) ;
#123399=CARTESIAN_POINT('Ctrl Pts',(-19.9518021159349,14.4944296430568,
131.157328547181)) ;
#123400=CARTESIAN_POINT('Ctrl Pts',(-19.871969321922,14.405561123776,130.89092166106)) ;
#123401=CARTESIAN_POINT('Ctrl Pts',(-19.8033463280559,14.2469874685197,
130.657440519266)) ;
#123402=CARTESIAN_POINT('Ctrl Pts',(-19.7508500620726,14.0284941679127,
130.470881149737)) ;
#123403=CARTESIAN_POINT('Ctrl Pts',(-19.719490022158,13.7670073728255,130.346148553405)) ;
#123404=CARTESIAN_POINT('Ctrl Pts',(-19.7121011487977,13.480578033378,130.291399553805)) ;
#123405=CARTESIAN_POINT('Ctrl Pts',(-19.7298039128491,13.1913387346796,
130.310107119157)) ;
#123406=CARTESIAN_POINT('Ctrl Pts',(-19.7722865639601,12.9172330452571,
130.401022931997)) ;
#123407=CARTESIAN_POINT('Ctrl Pts',(-19.8369732676592,12.6799728424888,
130.556899776584)) ;
#123408=CARTESIAN_POINT('Ctrl Pts',(-19.920757365482,12.4949910313751,130.768323701621)) ;
#123409=CARTESIAN_POINT('Ctrl Pts',(-20.0165266255756,12.3781840419528,
131.015200166848)) ;
#123410=CARTESIAN_POINT('Ctrl Pts',(-20.1206017423873,12.3352411031327,
131.28589296705)) ;
#123411=CARTESIAN_POINT('Ctrl Pts',(-20.2236087179121,12.3701183951614,
131.553933115692)) ;
#123412=CARTESIAN_POINT('Ctrl Pts',(-20.3217871748641,12.4815908336551,
131.807337046377)) ;
#123413=CARTESIAN_POINT('Ctrl Pts',(-20.4059913540354,12.6586744423265,
132.020414433851)) ;
#123414=CARTESIAN_POINT('Ctrl Pts',(-20.4731244336742,12.8927064520039,
132.183222264498)) ;
#123415=CARTESIAN_POINT('Ctrl Pts',(-20.5175674054042,13.161589606751,132.280177787723)) ;
#123416=CARTESIAN_POINT('Ctrl Pts',(-20.5380308810597,13.452733819126,132.306636877863)) ;
#123417=CARTESIAN_POINT('Ctrl Pts',(-20.5329915826682,13.7397606616034,
132.258839580122)) ;
#123418=CARTESIAN_POINT('Ctrl Pts',(-20.5038780440695,14.0044957325971,
132.140665648964)) ;
#123419=CARTESIAN_POINT('Ctrl Pts',(-20.4535510699206,14.2270717509881,
131.960602734661)) ;
#123420=CARTESIAN_POINT('Ctrl Pts',(-20.3861724322445,14.3928428929851,
131.730652816318)) ;
#123421=CARTESIAN_POINT('Ctrl Pts',(-20.3068708809211,14.4891680120794,
131.465698279101)) ;
#123422=CARTESIAN_POINT('Ctrl Pts',(-20.2234454311449,14.5086708871169,
131.18907353064)) ;
#123423=CARTESIAN_POINT('Ctrl Pts',(-20.1409292956804,14.4507090768999,
130.914800248059)) ;
#123424=CARTESIAN_POINT('Ctrl Pts',(-20.0669532543017,14.3188233795464,
130.665558965042)) ;
#123425=CARTESIAN_POINT('Ctrl Pts',(-20.0074043450587,14.1234066158898,
130.458538617797)) ;
#123426=CARTESIAN_POINT('Ctrl Pts',(-19.9670504311719,13.8772494948289,
130.307501661299)) ;
#123427=CARTESIAN_POINT('Ctrl Pts',(-19.9496300589494,13.5994496671663,
130.223567904008)) ;
#123428=CARTESIAN_POINT('Ctrl Pts',(-19.9572207572621,13.306728753329,130.212428024428)) ;
#123429=CARTESIAN_POINT('Ctrl Pts',(-19.9897127587384,13.0255130150403,
130.274404793934)) ;
#123430=CARTESIAN_POINT('Ctrl Pts',(-20.0457523916351,12.7708775179562,
130.404962496167)) ;
#123431=CARTESIAN_POINT('Ctrl Pts',(-20.122302311935,12.5628411654916,130.595365453384)) ;
#123432=CARTESIAN_POINT('Ctrl Pts',(-20.213834085187,12.4171763297159,130.829710899479)) ;
#123433=CARTESIAN_POINT('Ctrl Pts',(-20.3157550169223,12.3431378103405,
131.094146510188)) ;
#123434=CARTESIAN_POINT('Ctrl Pts',(-20.4194887113378,12.346743528454,131.364286240996)) ;
#123435=CARTESIAN_POINT('Ctrl Pts',(-20.520481797598,12.4272275492429,131.626120094335)) ;
#123436=CARTESIAN_POINT('Ctrl Pts',(-20.611016823755,12.5790159402385,131.857501904824)) ;
#123437=CARTESIAN_POINT('Ctrl Pts',(-20.6858521505329,12.7916689357573,
132.042932726522)) ;
#123438=CARTESIAN_POINT('Ctrl Pts',(-20.7400044978734,13.0498140627792,
132.167945329551)) ;
#123439=CARTESIAN_POINT('Ctrl Pts',(-20.7702882549419,13.3331758335929,
132.223407605724)) ;
#123440=CARTESIAN_POINT('Ctrl Pts',(-20.7756374687898,13.6238936791233,
132.205920744498)) ;
#123441=CARTESIAN_POINT('Ctrl Pts',(-20.7560346724831,13.9010886430072,
132.115433800579)) ;
#123442=CARTESIAN_POINT('Ctrl Pts',(-20.7137971359534,14.1432055625841,
131.958927687778)) ;
#123443=CARTESIAN_POINT('Ctrl Pts',(-20.6524404739172,14.334107077719,131.746477396685)) ;
#123444=CARTESIAN_POINT('Ctrl Pts',(-20.5777682256743,14.4587992015315,
131.495357936276)) ;
#123445=CARTESIAN_POINT('Ctrl Pts',(-20.4950831691612,14.5101605092006,
131.220685228617)) ;
#123446=CARTESIAN_POINT('Ctrl Pts',(-20.4112704543339,14.4834097462587,
130.942700325563)) ;
#123447=CARTESIAN_POINT('Ctrl Pts',(-20.3332099228401,14.3809866888584,
130.681571480112)) ;
#123448=CARTESIAN_POINT('Ctrl Pts',(-20.2668912037514,14.2089571493578,
130.454589975505)) ;
#123449=CARTESIAN_POINT('Ctrl Pts',(-20.218467666732,13.9828180389134,130.280212948204)) ;
#123450=CARTESIAN_POINT('Ctrl Pts',(-20.1912296262005,13.7132629238328,
130.167271930086)) ;
#123451=CARTESIAN_POINT('Ctrl Pts',(-20.1886479569655,13.4258376467274,
130.126737660166)) ;
#123452=CARTESIAN_POINT('Ctrl Pts',(-20.2111109241553,13.1374631126408,
130.159264452679)) ;
#123453=CARTESIAN_POINT('Ctrl Pts',(-20.2579828619858,12.8691197020598,
130.263056881787)) ;
#123454=CARTESIAN_POINT('Ctrl Pts',(-20.3267504711329,12.6403113391648,
130.430759227376)) ;
#123455=CARTESIAN_POINT('Ctrl Pts',(-20.4125317522278,12.4684206936737,
130.648356829009)) ;
#123456=CARTESIAN_POINT('Ctrl Pts',(-20.511311636761,12.3638000131135,130.90360763348)) ;
#123457=CARTESIAN_POINT('Ctrl Pts',(-20.6150180548314,12.3359859149595,
131.173540854503)) ;
#123458=CARTESIAN_POINT('Ctrl Pts',(-20.7180532017287,12.3855342860159,
131.441422429249)) ;
#123459=CARTESIAN_POINT('Ctrl Pts',(-20.8135713176557,12.5097023553619,
131.687312039212)) ;
#123460=CARTESIAN_POINT('Ctrl Pts',(-20.8952342042776,12.6987170593864,
131.892805673695)) ;
#123461=CARTESIAN_POINT('Ctrl Pts',(-20.958454326468,12.9413959891016,132.04418647609)) ;
#123462=CARTESIAN_POINT('Ctrl Pts',(-20.998549110379,13.2164085190981,132.128309514099)) ;
#123463=CARTESIAN_POINT('Ctrl Pts',(-21.0140910885354,13.5077477594262,
132.140512952863)) ;
#123464=CARTESIAN_POINT('Ctrl Pts',(-21.0044134115614,13.7917086517815,
132.07920216301)) ;
#123465=CARTESIAN_POINT('Ctrl Pts',(-20.9711009482148,14.0497091065288,
131.948804846017)) ;
#123466=CARTESIAN_POINT('Ctrl Pts',(-20.9171221574838,14.2632251224131,
131.757995762905)) ;
#123467=CARTESIAN_POINT('Ctrl Pts',(-20.8468654201181,14.4168538521645,
131.51953628378)) ;
#123468=CARTESIAN_POINT('Ctrl Pts',(-20.76649453193,14.498759930122,131.251623228353)) ;
#123469=CARTESIAN_POINT('Ctrl Pts',(-20.6822889980889,14.5035045472666,
130.97248421508)) ;
#123470=CARTESIAN_POINT('Ctrl Pts',(-20.6013459781706,14.4313229189066,
130.703011266321)) ;
#123471=CARTESIAN_POINT('Ctrl Pts',(-20.5294298629852,14.2860965422893,
130.459686692304)) ;
#123472=CARTESIAN_POINT('Ctrl Pts',(-20.4733896837884,14.0806886832094,
130.263034151577)) ;
#123473=CARTESIAN_POINT('Ctrl Pts',(-20.437003865906,13.8265803466444,130.123525632971)) ;
#123474=CARTESIAN_POINT('Ctrl Pts',(-20.4242437811455,13.5441877343299,
130.053137789397)) ;
#123475=CARTESIAN_POINT('Ctrl Pts',(-20.4365312961632,13.2530368711715,
130.055902630421)) ;
#123476=CARTESIAN_POINT('Ctrl Pts',(-20.4737535574682,12.9741112441056,
130.131516179616)) ;
#123477=CARTESIAN_POINT('Ctrl Pts',(-20.5340120502757,12.727211784615,130.274403584584)) ;
#123478=CARTESIAN_POINT('Ctrl Pts',(-20.6135558274094,12.5305676715835,
130.47368429756)) ;
#123479=CARTESIAN_POINT('Ctrl Pts',(-20.7074108358281,12.3976028269524,
130.7147928397)) ;
#123480=CARTESIAN_POINT('Ctrl Pts',(-20.8102697894059,12.3378877483635,
130.982018981764)) ;
#123481=CARTESIAN_POINT('Ctrl Pts',(-20.9141444616179,12.3561146706411,
131.252466517533)) ;
#123482=CARTESIAN_POINT('Ctrl Pts',(-21.013548346515,12.4504996571453,131.509715354224)) ;
#123483=CARTESIAN_POINT('Ctrl Pts',(-21.1017319257438,12.6151918757671,
131.734128219321)) ;
#123484=CARTESIAN_POINT('Ctrl Pts',(-21.1727252896726,12.8367628546182,
131.908472936722)) ;
#123485=CARTESIAN_POINT('Ctrl Pts',(-21.2228063284793,13.1024713310692,
132.02145618296)) ;
#123486=CARTESIAN_POINT('Ctrl Pts',(-21.2483471373565,13.3880985112024,
132.063131681932)) ;
#123487=CARTESIAN_POINT('Ctrl Pts',(-21.2488921318712,13.6786302833929,
132.03149649857)) ;
#123488=CARTESIAN_POINT('Ctrl Pts',(-21.2248618457064,13.9495118102634,
131.928235541362)) ;
#123489=CARTESIAN_POINT('Ctrl Pts',(-21.1787560649986,14.1831630718956,
131.760424667583)) ;
#123490=CARTESIAN_POINT('Ctrl Pts',(-21.1147226870487,14.3622887223182,
131.540299304929)) ;
#123491=CARTESIAN_POINT('Ctrl Pts',(-21.0373135712912,14.4748192512671,
131.28083347839)) ;
#123492=CARTESIAN_POINT('Ctrl Pts',(-20.9542091849475,14.5109473635331,
131.005069073046)) ;
#123493=CARTESIAN_POINT('Ctrl Pts',(-20.8711615353629,14.4698938664046,
130.729403038778)) ;
#123494=CARTESIAN_POINT('Ctrl Pts',(-20.7947773885022,14.3536144682459,
130.473115915764)) ;
#123495=CARTESIAN_POINT('Ctrl Pts',(-20.7314926566507,14.1706211200802,
130.255100908174)) ;
#123496=CARTESIAN_POINT('Ctrl Pts',(-20.6865866876849,13.9337365390504,
130.090746076654)) ;
#123497=CARTESIAN_POINT('Ctrl Pts',(-20.6640317813757,13.6617103922721,
129.991857066117)) ;
#123498=CARTESIAN_POINT('Ctrl Pts',(-20.6660448486166,13.3701431433412,
129.964445738418)) ;
#123499=CARTESIAN_POINT('Ctrl Pts',(-20.6933950437576,13.0839500606497,
130.011232944482)) ;
#123500=CARTESIAN_POINT('Ctrl Pts',(-20.7444685293644,12.8226368169183,
130.127408051906)) ;
#123501=CARTESIAN_POINT('Ctrl Pts',(-20.8166965559811,12.603615233857,130.305292057328)) ;
#123502=CARTESIAN_POINT('Ctrl Pts',(-20.9053725966928,12.443223881209,130.531268705482)) ;
#123503=CARTESIAN_POINT('Ctrl Pts',(-21.0058923229845,12.3525997217998,
130.791559536771)) ;
#123504=CARTESIAN_POINT('Ctrl Pts',(-21.109651199822,12.339390379435,131.061737133445)) ;
#123505=CARTESIAN_POINT('Ctrl Pts',(-21.2119649378887,12.4034681613504,
131.327439559372)) ;
#123506=CARTESIAN_POINT('Ctrl Pts',(-21.3052562726005,12.5405073209883,
131.56686992949)) ;
#123507=CARTESIAN_POINT('Ctrl Pts',(-21.3841471163856,12.742000710491,131.764047288441)) ;
#123508=CARTESIAN_POINT('Ctrl Pts',(-21.4427047415853,12.9900803066021,
131.902157135438)) ;
#123509=CARTESIAN_POINT('Ctrl Pts',(-21.4785501947781,13.2708160842573,
131.973683053502)) ;
#123510=CARTESIAN_POINT('Ctrl Pts',(-21.4892592807922,13.5613606280666,
131.971916172654)) ;
#123511=CARTESIAN_POINT('Ctrl Pts',(-21.4750643268527,13.8428562082264,
131.897307591027)) ;
#123512=CARTESIAN_POINT('Ctrl Pts',(-21.4372222388411,14.0951248182504,
131.753467391875)) ;
#123513=CARTESIAN_POINT('Ctrl Pts',(-21.3801699783513,14.2968155376203,
131.553906783451)) ;
#123514=CARTESIAN_POINT('Ctrl Pts',(-21.3073404665403,14.4382063534547,
131.307842622038)) ;
#123515=CARTESIAN_POINT('Ctrl Pts',(-21.2257750525136,14.5055714123115,
131.036462132016)) ;
#123516=CARTESIAN_POINT('Ctrl Pts',(-21.1419504646032,14.4957941615493,
130.758568660941)) ;
#123517=CARTESIAN_POINT('Ctrl Pts',(-21.062130144461,14.4095661599452,130.492310196492)) ;
#123518=CARTESIAN_POINT('Ctrl Pts',(-20.9925528707413,14.2515334104405,
130.255766002423)) ;
#123519=CARTESIAN_POINT('Ctrl Pts',(-20.9397828713012,14.0347235705321,
130.068496746948)) ;
#123520=CARTESIAN_POINT('Ctrl Pts',(-20.9078955950986,13.7751698912538,
129.94233748602)) ;
#123521=CARTESIAN_POINT('Ctrl Pts',(-20.8997160785567,13.489554992756,129.885321758747)) ;
#123522=CARTESIAN_POINT('Ctrl Pts',(-20.9167899789178,13.1989623651925,
129.902052359333)) ;
#123523=CARTESIAN_POINT('Ctrl Pts',(-20.9585152633915,12.9245155111551,
129.990817188961)) ;
#123524=CARTESIAN_POINT('Ctrl Pts',(-21.0230710384516,12.6850931696754,
130.1461348862)) ;
#123525=CARTESIAN_POINT('Ctrl Pts',(-21.1051698936851,12.5007200280461,
130.353109490092)) ;
#123526=CARTESIAN_POINT('Ctrl Pts',(-21.2017300839304,12.3802347954754,
130.601895637296)) ;
#123527=CARTESIAN_POINT('Ctrl Pts',(-21.3047713404402,12.3354177836866,
130.86988001272)) ;
#123528=CARTESIAN_POINT('Ctrl Pts',(-21.4088230503547,12.3682931667049,
131.140651524699)) ;
#123529=CARTESIAN_POINT('Ctrl Pts',(-21.5062542759513,12.4764500212594,
131.392235920731)) ;
#123530=CARTESIAN_POINT('Ctrl Pts',(-21.5916025918959,12.6527561710341,
131.608397293271)) ;
#123531=CARTESIAN_POINT('Ctrl Pts',(-21.6590311393467,12.8841372623909,
131.77224964389)) ;
#123532=CARTESIAN_POINT('Ctrl Pts',(-21.7046072134825,13.1550291138396,
131.87215932753)) ;
#123533=CARTESIAN_POINT('Ctrl Pts',(-21.7255333174223,13.4437302446049,
131.900234737756)) ;
#123534=CARTESIAN_POINT('Ctrl Pts',(-21.7212604449213,13.7319393210826,
131.854574354767)) ;
#123535=CARTESIAN_POINT('Ctrl Pts',(-21.6929317986939,13.996548190544,131.738831324701)) ;
#123536=CARTESIAN_POINT('Ctrl Pts',(-21.6430685171198,14.2215298509627,
131.56000823255)) ;
#123537=CARTESIAN_POINT('Ctrl Pts',(-21.5759281474204,14.38914835891,131.330697063604)) ;
#123538=CARTESIAN_POINT('Ctrl Pts',(-21.4974078326725,14.4871687209254,
131.068241553781)) ;
#123539=CARTESIAN_POINT('Ctrl Pts',(-21.4134771466602,14.5093408038881,
130.789919219591)) ;
#123540=CARTESIAN_POINT('Ctrl Pts',(-21.3307764849043,14.4530254210031,
130.515076303721)) ;
#123541=CARTESIAN_POINT('Ctrl Pts',(-21.2568613332395,14.3240304850431,
130.266200944563)) ;
#123542=CARTESIAN_POINT('Ctrl Pts',(-21.1965031358292,14.1290978573837,
130.056618503273)) ;
#123543=CARTESIAN_POINT('Ctrl Pts',(-21.1557411885856,13.8855602682148,
129.904586032072)) ;
#123544=CARTESIAN_POINT('Ctrl Pts',(-21.1375373161458,13.605841493294,129.818053721067)) ;
#123545=CARTESIAN_POINT('Ctrl Pts',(-21.1444136266794,13.3160019490386,
129.805155623741)) ;
#123546=CARTESIAN_POINT('Ctrl Pts',(-21.1762636439198,13.0326884812318,
129.865076095617)) ;
#123547=CARTESIAN_POINT('Ctrl Pts',(-21.2319115326232,12.7766370515925,
129.994424641396)) ;
#123548=CARTESIAN_POINT('Ctrl Pts',(-21.3078505230511,12.5676696843858,
130.183109710706)) ;
#123549=CARTESIAN_POINT('Ctrl Pts',(-21.3987133740418,12.4206516952527,
130.415612728524)) ;
#123550=CARTESIAN_POINT('Ctrl Pts',(-21.5001018874593,12.34431502245,130.678595897684)) ;
#123551=CARTESIAN_POINT('Ctrl Pts',(-21.604355434881,12.345456773331,130.950092534873)) ;
#123552=CARTESIAN_POINT('Ctrl Pts',(-21.7056774142942,12.4241540990105,
131.212838185246)) ;
#123553=CARTESIAN_POINT('Ctrl Pts',(-21.7963153488062,12.5736455946733,
131.444615300507)) ;
#123554=CARTESIAN_POINT('Ctrl Pts',(-21.8716294111361,12.7844245874558,
131.631479009685)) ;
#123555=CARTESIAN_POINT('Ctrl Pts',(-21.926464113242,13.0412646550238,131.758504009558)) ;
#123556=CARTESIAN_POINT('Ctrl Pts',(-21.9575791398446,13.3250315602578,
131.816289040301)) ;
#123557=CARTESIAN_POINT('Ctrl Pts',(-21.9635975249706,13.615649410723,131.800779000358)) ;
#123558=CARTESIAN_POINT('Ctrl Pts',(-21.9447887810927,13.8929004143671,
131.712695653985)) ;
#123559=CARTESIAN_POINT('Ctrl Pts',(-21.9031267111208,14.1366367418866,
131.557822791133)) ;
#123560=CARTESIAN_POINT('Ctrl Pts',(-21.8425040812558,14.3287834464846,
131.347629205609)) ;
#123561=CARTESIAN_POINT('Ctrl Pts',(-21.7678540280259,14.4563288635319,
131.096426004095)) ;
#123562=CARTESIAN_POINT('Ctrl Pts',(-21.6851288303161,14.5097636487804,
130.821575692504)) ;
#123563=CARTESIAN_POINT('Ctrl Pts',(-21.6014964088301,14.4852491667338,
130.544211499597)) ;
#123564=CARTESIAN_POINT('Ctrl Pts',(-21.523248358388,14.3852131560936,130.282568889525)) ;
#123565=CARTESIAN_POINT('Ctrl Pts',(-21.4563633176233,14.2148994142931,
130.053885615142)) ;
#123566=CARTESIAN_POINT('Ctrl Pts',(-21.4073363060667,13.9895604970269,
129.877675130071)) ;
#123567=CARTESIAN_POINT('Ctrl Pts',(-21.3795391128537,13.722649621575,129.763310479199)) ;
#123568=CARTESIAN_POINT('Ctrl Pts',(-21.3761385230511,13.4342098870415,
129.720221810057)) ;
#123569=CARTESIAN_POINT('Ctrl Pts',(-21.3978578853594,13.145818281647,129.750615209782)) ;
#123570=CARTESIAN_POINT('Ctrl Pts',(-21.4442331193328,12.8759127187507,
129.852856124059)) ;
#123571=CARTESIAN_POINT('Ctrl Pts',(-21.512001278979,12.646886857505,130.017831473784)) ;
#123572=CARTESIAN_POINT('Ctrl Pts',(-21.5978716016616,12.4721832267463,
130.23548160431)) ;
#123573=CARTESIAN_POINT('Ctrl Pts',(-21.6955599071442,12.3661739230268,
130.487824821297)) ;
#123574=CARTESIAN_POINT('Ctrl Pts',(-21.8000520177911,12.3355863381279,
130.759770244015)) ;
#123575=CARTESIAN_POINT('Ctrl Pts',(-21.9029799864568,12.383119877217,131.027414224694)) ;
#123576=CARTESIAN_POINT('Ctrl Pts',(-21.9989039448222,12.5053833335783,
131.274450432666)) ;
#123577=CARTESIAN_POINT('Ctrl Pts',(-22.0808309670336,12.6923271245218,
131.480792497128)) ;
#123578=CARTESIAN_POINT('Ctrl Pts',(-22.1446987970862,12.933586655108,131.634070485524)) ;
#123579=CARTESIAN_POINT('Ctrl Pts',(-22.1855556015519,13.2085815637178,
131.720337818846)) ;
#123580=CARTESIAN_POINT('Ctrl Pts',(-22.2017695623135,13.499055887524,131.734588727789)) ;
#123581=CARTESIAN_POINT('Ctrl Pts',(-22.1928346734152,13.7836908824952,
131.67542411847)) ;
#123582=CARTESIAN_POINT('Ctrl Pts',(-22.1601714423331,14.0427282723312,
131.546925391615)) ;
#123583=CARTESIAN_POINT('Ctrl Pts',(-22.1067337756389,14.2577310864089,
131.357698532383)) ;
#123584=CARTESIAN_POINT('Ctrl Pts',(-22.0370124630534,14.4131665395365,
131.120862803271)) ;
#123585=CARTESIAN_POINT('Ctrl Pts',(-21.9566962255491,14.4973756020118,
130.853040421815)) ;
#123586=CARTESIAN_POINT('Ctrl Pts',(-21.8729279876658,14.5046723914937,
130.575350665997)) ;
#123587=CARTESIAN_POINT('Ctrl Pts',(-21.7912035400918,14.4343110972272,
130.303348729222)) ;
#123588=CARTESIAN_POINT('Ctrl Pts',(-21.7191872942723,14.2913902739099,
130.059848443852)) ;
#123589=CARTESIAN_POINT('Ctrl Pts',(-21.6625256909842,14.0872938687907,
129.861320234201)) ;
#123590=CARTESIAN_POINT('Ctrl Pts',(-21.6255724955298,13.8349905737135,
129.720243192355)) ;
#123591=CARTESIAN_POINT('Ctrl Pts',(-21.6120328126858,13.5522016078203,
129.647460332955)) ;
#123592=CARTESIAN_POINT('Ctrl Pts',(-21.623622872742,13.261176925901,129.64821085162)) ;
#123593=CARTESIAN_POINT('Ctrl Pts',(-21.6602148810404,12.9814105366867,
129.721952022886)) ;
#123594=CARTESIAN_POINT('Ctrl Pts',(-21.7196534333109,12.7341368123324,
129.862553970206)) ;
#123595=CARTESIAN_POINT('Ctrl Pts',(-21.7988553081735,12.5351661127334,
130.060752426259)) ;
#123596=CARTESIAN_POINT('Ctrl Pts',(-21.8928056856465,12.4000170335594,
130.30200784534)) ;
#123597=CARTESIAN_POINT('Ctrl Pts',(-21.9950158650803,12.3385940998212,
130.567504847325)) ;
#123598=CARTESIAN_POINT('Ctrl Pts',(-22.0991055754472,12.3545286959988,
130.838523437866)) ;
#123599=CARTESIAN_POINT('Ctrl Pts',(-22.198792064463,12.4469846985816,131.096579489399)) ;
#123600=CARTESIAN_POINT('Ctrl Pts',(-22.2874703472673,12.6102580102747,
131.322388272232)) ;
#123601=CARTESIAN_POINT('Ctrl Pts',(-22.3586713429203,12.8296978065605,
131.4974644856)) ;
#123602=CARTESIAN_POINT('Ctrl Pts',(-22.4092935566175,13.0929764235486,
131.612190617179)) ;
#123603=CARTESIAN_POINT('Ctrl Pts',(-22.4357877911489,13.3798715648176,
131.656456165167)) ;
#123604=CARTESIAN_POINT('Ctrl Pts',(-22.4369919562027,13.6705227890218,
131.626757747734)) ;
#123605=CARTESIAN_POINT('Ctrl Pts',(-22.4136887889266,13.9421700624616,
131.525632072754)) ;
#123606=CARTESIAN_POINT('Ctrl Pts',(-22.3679163610009,14.1780191075409,
131.358654623663)) ;
#123607=CARTESIAN_POINT('Ctrl Pts',(-22.3045084630622,14.3579768131381,
131.140480788667)) ;
#123608=CARTESIAN_POINT('Ctrl Pts',(-22.2275826101986,14.4725057536027,
130.882499856807)) ;
#123609=CARTESIAN_POINT('Ctrl Pts',(-22.1444232291687,14.5110248787741,
130.60651491726)) ;
#123610=CARTESIAN_POINT('Ctrl Pts',(-22.0612174095962,14.4721191985818,
130.33036485736)) ;
#123611=CARTESIAN_POINT('Ctrl Pts',(-21.984532639996,14.3577454334386,130.073186159009)) ;
#123612=CARTESIAN_POINT('Ctrl Pts',(-21.9209902476645,14.1770688600788,
129.854519186806)) ;
#123613=CARTESIAN_POINT('Ctrl Pts',(-21.8754073396789,13.9416997135302,
129.688189111058)) ;
#123614=CARTESIAN_POINT('Ctrl Pts',(-21.8521280328219,13.6694103999149,
129.587060443625)) ;
#123615=CARTESIAN_POINT('Ctrl Pts',(-21.8533886977509,13.3798585419127,
129.557657884149)) ;
#123616=CARTESIAN_POINT('Ctrl Pts',(-21.8798930282876,13.0927639720694,
129.601925595743)) ;
#123617=CARTESIAN_POINT('Ctrl Pts',(-21.9305070655624,12.8294541996799,
129.716631316769)) ;
#123618=CARTESIAN_POINT('Ctrl Pts',(-22.0021915119571,12.6090079342562,
129.892932878091)) ;
#123619=CARTESIAN_POINT('Ctrl Pts',(-22.0906529644775,12.4466659033485,
130.118224388233)) ;
#123620=CARTESIAN_POINT('Ctrl Pts',(-22.1903372657479,12.3544265083851,
130.376275283153)) ;
#123621=CARTESIAN_POINT('Ctrl Pts',(-22.2942873445746,12.338485561048,130.646936791498)) ;
#123622=CARTESIAN_POINT('Ctrl Pts',(-22.3973135054693,12.4009576642386,
130.914537921283)) ;
#123623=CARTESIAN_POINT('Ctrl Pts',(-22.4904420137874,12.5356623711056,
131.153649825202)) ;
#123624=CARTESIAN_POINT('Ctrl Pts',(-22.5695739948327,12.7342794409358,
131.351681157617)) ;
#123625=CARTESIAN_POINT('Ctrl Pts',(-22.6291160828329,12.9822472239535,
131.492506830932)) ;
#123626=CARTESIAN_POINT('Ctrl Pts',(-22.6656693979879,13.2626106306711,
131.566076960599)) ;
#123627=CARTESIAN_POINT('Ctrl Pts',(-22.6770955873921,13.5537332478673,
131.566337188206)) ;
#123628=CARTESIAN_POINT('Ctrl Pts',(-22.6635414721597,13.835078244523,131.493672842858)) ;
#123629=CARTESIAN_POINT('Ctrl Pts',(-22.6266625017424,14.0872564093589,
131.352837031821)) ;
#123630=CARTESIAN_POINT('Ctrl Pts',(-22.5697278634071,14.2922554026262,
131.153365374301)) ;
#123631=CARTESIAN_POINT('Ctrl Pts',(-22.4973810272917,14.4349646687422,
130.908797184374)) ;
#123632=CARTESIAN_POINT('Ctrl Pts',(-22.4163391881196,14.50455407939,130.639073907025)) ;
#123633=CARTESIAN_POINT('Ctrl Pts',(-22.3321658591823,14.4973581073499,
130.360039361529)) ;
#123634=CARTESIAN_POINT('Ctrl Pts',(-22.2518685737339,14.4126016063702,
130.092261416254)) ;
#123635=CARTESIAN_POINT('Ctrl Pts',(-22.1824698979615,14.2578369760295,
129.856517613998)) ;
#123636=CARTESIAN_POINT('Ctrl Pts',(-22.128910794309,14.0423605049128,129.666858615955)) ;
#123637=CARTESIAN_POINT('Ctrl Pts',(-22.0962688121286,13.7833429469769,
129.538433890932)) ;
#123638=CARTESIAN_POINT('Ctrl Pts',(-22.087408581468,13.4972453189194,129.479321882593)) ;
#123639=CARTESIAN_POINT('Ctrl Pts',(-22.1036837457702,13.2077136867894,
129.493862670111)) ;
#123640=CARTESIAN_POINT('Ctrl Pts',(-22.1448226422972,12.9318530296234,
129.580826868233)) ;
#123641=CARTESIAN_POINT('Ctrl Pts',(-22.2083889117373,12.6922551548189,
129.733430569201)) ;
#123642=CARTESIAN_POINT('Ctrl Pts',(-22.2905762804596,12.5046664561304,
129.940421973245)) ;
#123643=CARTESIAN_POINT('Ctrl Pts',(-22.3868645087998,12.3825157092279,
130.188426397229)) ;
#123644=CARTESIAN_POINT('Ctrl Pts',(-22.4895735286878,12.3357140446238,
130.455506685267)) ;
#123645=CARTESIAN_POINT('Ctrl Pts',(-22.593480759488,12.36606795923,130.725932566438)) ;
#123646=CARTESIAN_POINT('Ctrl Pts',(-22.6916956961957,12.4727573842292,
130.979628387978)) ;
#123647=CARTESIAN_POINT('Ctrl Pts',(-22.7772373371253,12.6471452972706,
131.196428921888)) ;
#123648=CARTESIAN_POINT('Ctrl Pts',(-22.8450776069585,12.8766362128536,
131.361554408823)) ;
#123649=CARTESIAN_POINT('Ctrl Pts',(-22.8913157755796,13.1457609498557,
131.463497390875)) ;
#123650=CARTESIAN_POINT('Ctrl Pts',(-22.9131064687665,13.4362085163513,
131.493864737926)) ;
#123651=CARTESIAN_POINT('Ctrl Pts',(-22.9095252366571,13.7232902090159,
131.4503951076)) ;
#123652=CARTESIAN_POINT('Ctrl Pts',(-22.8818492535102,13.9896012437994,
131.336467064761)) ;
#123653=CARTESIAN_POINT('Ctrl Pts',(-22.8324906093414,14.215929645434,131.15911392552)) ;
#123654=CARTESIAN_POINT('Ctrl Pts',(-22.7659015545217,14.3851342373848,
130.931470999385)) ;
#123655=CARTESIAN_POINT('Ctrl Pts',(-22.6875045184051,14.4854517125692,
130.669322994244)) ;
#123656=CARTESIAN_POINT('Ctrl Pts',(-22.603799348601,14.5096986582257,130.391723047381)) ;
#123657=CARTESIAN_POINT('Ctrl Pts',(-22.5211552560533,14.4561737442075,
130.117138838309)) ;
#123658=CARTESIAN_POINT('Ctrl Pts',(-22.4464425125738,14.3282784828902,
129.865710255824)) ;
#123659=CARTESIAN_POINT('Ctrl Pts',(-22.3859620483162,14.1363002885468,
129.655987705534)) ;
#123660=CARTESIAN_POINT('Ctrl Pts',(-22.3443239578635,13.8924838529507,
129.501179650082)) ;
#123661=CARTESIAN_POINT('Ctrl Pts',(-22.3255548355993,13.6154600840217,
129.413243078531)) ;
#123662=CARTESIAN_POINT('Ctrl Pts',(-22.3316054927386,13.3244464776438,
129.397782302623)) ;
#123663=CARTESIAN_POINT('Ctrl Pts',(-22.362789865854,13.0407280398606,129.455770685946)) ;
#123664=CARTESIAN_POINT('Ctrl Pts',(-22.4175554506853,12.7843964023836,
129.582650808215)) ;
#123665=CARTESIAN_POINT('Ctrl Pts',(-22.4928772666945,12.5734337589229,
129.769524564463)) ;
#123666=CARTESIAN_POINT('Ctrl Pts',(-22.5839516709931,12.4236458719393,
130.002437978547)) ;
#123667=CARTESIAN_POINT('Ctrl Pts',(-22.6846738463837,12.3455712337427,
130.263634905139)) ;
#123668=CARTESIAN_POINT('Ctrl Pts',(-22.789260868032,12.3443023954149,130.535996594304)) ;
#123669=CARTESIAN_POINT('Ctrl Pts',(-22.89070007856,12.4209332624995,130.799108040952)) ;
#123670=CARTESIAN_POINT('Ctrl Pts',(-22.9817398361439,12.5684898191716,
131.032050055215)) ;
#123671=CARTESIAN_POINT('Ctrl Pts',(-23.0577480467898,12.7783873972307,
131.220853670815)) ;
#123672=CARTESIAN_POINT('Ctrl Pts',(-23.1130745475148,13.0341437387016,
131.349338722741)) ;
#123673=CARTESIAN_POINT('Ctrl Pts',(-23.1447720687108,13.3161554584295,
131.408969086763)) ;
#123674=CARTESIAN_POINT('Ctrl Pts',(-23.1515934109415,13.6077103928711,
131.395709155052)) ;
#123675=CARTESIAN_POINT('Ctrl Pts',(-23.1333286351704,13.8863968339185,
131.309116820984)) ;
#123676=CARTESIAN_POINT('Ctrl Pts',(-23.092261773277,14.1306964208414,131.156045144409)) ;
#123677=CARTESIAN_POINT('Ctrl Pts',(-23.0323203050515,14.3238933798465,
130.947948945004)) ;
#123678=CARTESIAN_POINT('Ctrl Pts',(-22.9580389719213,14.4535138148578,
130.697833001555)) ;
#123679=CARTESIAN_POINT('Ctrl Pts',(-22.8754326033728,14.5094099207336,
130.423321601385)) ;
#123680=CARTESIAN_POINT('Ctrl Pts',(-22.7912683304849,14.4867701490887,
130.144213707131)) ;
#123681=CARTESIAN_POINT('Ctrl Pts',(-22.7132364319315,14.3890643501402,
129.883381354507)) ;
#123682=CARTESIAN_POINT('Ctrl Pts',(-22.6459538319007,14.2211868758739,
129.65358774104)) ;
#123683=CARTESIAN_POINT('Ctrl Pts',(-22.5961304153725,13.9958857732727,
129.474863269661)) ;
#123684=CARTESIAN_POINT('Ctrl Pts',(-22.5678649144097,13.731479333369,129.359334414953)) ;
#123685=CARTESIAN_POINT('Ctrl Pts',(-22.5636217990249,13.44236393195,129.313663179006)) ;
#123686=CARTESIAN_POINT('Ctrl Pts',(-22.5848238291133,13.1530743208287,
129.342464490565)) ;
#123687=CARTESIAN_POINT('Ctrl Pts',(-22.6301149482752,12.884256615766,129.441790820135)) ;
#123688=CARTESIAN_POINT('Ctrl Pts',(-22.6978320294382,12.6519995409111,
129.606348451409)) ;
#123689=CARTESIAN_POINT('Ctrl Pts',(-22.7828059113389,12.4766942451725,
129.821579606252)) ;
#123690=CARTESIAN_POINT('Ctrl Pts',(-22.8804228762943,12.3681120664589,
130.073631874159)) ;
#123691=CARTESIAN_POINT('Ctrl Pts',(-22.9849198201405,12.3353450088633,
130.345571088682)) ;
#123692=CARTESIAN_POINT('Ctrl Pts',(-23.0880396701076,12.380878936013,130.613744761632)) ;
#123693=CARTESIAN_POINT('Ctrl Pts',(-23.1839462416439,12.5006496945069,
130.860845156785)) ;
#123694=CARTESIAN_POINT('Ctrl Pts',(-23.266521775703,12.6862349323656,131.06900841109)) ;
#123695=CARTESIAN_POINT('Ctrl Pts',(-23.3307747879631,12.9253055935091,
131.223534372518)) ;
#123696=CARTESIAN_POINT('Ctrl Pts',(-23.3724397745999,13.1996775352275,
131.31213337044)) ;
#123697=CARTESIAN_POINT('Ctrl Pts',(-23.3894540507773,13.4900584277301,
131.32871644911)) ;
#123698=CARTESIAN_POINT('Ctrl Pts',(-23.3812045124378,13.7765695978382,
131.27139174498)) ;
#123699=CARTESIAN_POINT('Ctrl Pts',(-23.3489874615433,14.036835781509,131.144138279515)) ;
#123700=CARTESIAN_POINT('Ctrl Pts',(-23.2963232747133,14.2522895995138,
130.957329544454)) ;
#123701=CARTESIAN_POINT('Ctrl Pts',(-23.226675069615,14.410142724822,130.720563800581)) ;
#123702=CARTESIAN_POINT('Ctrl Pts',(-23.1469566767061,14.4959011671627,
130.45465902455)) ;
#123703=CARTESIAN_POINT('Ctrl Pts',(-23.0630393438504,14.5055615409164,
130.176461828221)) ;
#123704=CARTESIAN_POINT('Ctrl Pts',(-22.9812984775672,14.4373878436055,
129.904473138408)) ;
#123705=CARTESIAN_POINT('Ctrl Pts',(-22.9089719408676,14.2968054840673,
129.660103398097)) ;
#123706=CARTESIAN_POINT('Ctrl Pts',(-22.8515548229148,14.0934338457394,
129.459228202194)) ;
#123707=CARTESIAN_POINT('Ctrl Pts',(-22.8141130964861,13.8423636115969,
129.316759095522)) ;
#123708=CARTESIAN_POINT('Ctrl Pts',(-22.7998637079465,13.5615575056706,
129.242062802515)) ;
#123709=CARTESIAN_POINT('Ctrl Pts',(-22.8107205774882,13.2694346825445,
129.240546215534)) ;
#123710=CARTESIAN_POINT('Ctrl Pts',(-22.8464960658209,12.9897645897098,
129.311993364082)) ;
#123711=CARTESIAN_POINT('Ctrl Pts',(-22.9054877650127,12.7403850896867,
129.451171580521)) ;
#123712=CARTESIAN_POINT('Ctrl Pts',(-22.9841235537869,12.5401777346667,
129.647762655678)) ;
#123713=CARTESIAN_POINT('Ctrl Pts',(-23.0774322582716,12.403253810304,129.887237341054)) ;
#123714=CARTESIAN_POINT('Ctrl Pts',(-23.1796029037189,12.3392654629647,
130.152574531222)) ;
#123715=CARTESIAN_POINT('Ctrl Pts',(-23.2840127627671,12.3529796001613,
130.424441355207)) ;
#123716=CARTESIAN_POINT('Ctrl Pts',(-23.3838205000932,12.4434150313968,
130.682876822953)) ;
#123717=CARTESIAN_POINT('Ctrl Pts',(-23.4725822238479,12.6038143238447,
130.909076120196)) ;
#123718=CARTESIAN_POINT('Ctrl Pts',(-23.5448588483883,12.8232747601352,
131.087059295261)) ;
#123719=CARTESIAN_POINT('Ctrl Pts',(-23.5959036411586,13.0848674968843,
131.203128049166)) ;
#123720=CARTESIAN_POINT('Ctrl Pts',(-23.6231518851354,13.3712341167296,
131.2496031028)) ;
#123721=CARTESIAN_POINT('Ctrl Pts',(-23.6251153546057,13.662067069188,131.222130850832)) ;
#123722=CARTESIAN_POINT('Ctrl Pts',(-23.602443415498,13.9347879566426,131.122806374667)) ;
#123723=CARTESIAN_POINT('Ctrl Pts',(-23.5575106719909,14.1711547211457,
130.958420904302)) ;
#123724=CARTESIAN_POINT('Ctrl Pts',(-23.4942303983001,14.3538986016763,
130.740436482537)) ;
#123725=CARTESIAN_POINT('Ctrl Pts',(-23.4179436544872,14.4699515412555,
130.484481417006)) ;
#123726=CARTESIAN_POINT('Ctrl Pts',(-23.3347210664795,14.5110117292323,
130.208235504847)) ;
#123727=CARTESIAN_POINT('Ctrl Pts',(-23.2514904333782,14.4745400439387,
129.932050841537)) ;
#123728=CARTESIAN_POINT('Ctrl Pts',(-23.1740871767367,14.3614975022745,
129.672577858496)) ;
#123729=CARTESIAN_POINT('Ctrl Pts',(-23.1103820389956,14.1829580281289,
129.453553214764)) ;
#123730=CARTESIAN_POINT('Ctrl Pts',(-23.0642199301642,13.94924048582,129.285561754027)) ;
#123731=CARTESIAN_POINT('Ctrl Pts',(-23.0402642951649,13.6775800783231,
129.182436219737)) ;
#123732=CARTESIAN_POINT('Ctrl Pts',(-23.0407276337131,13.3886494305686,
129.150753202406)) ;
#123733=CARTESIAN_POINT('Ctrl Pts',(-23.0667742903849,13.0993477502972,
129.193462997382)) ;
#123734=CARTESIAN_POINT('Ctrl Pts',(-23.1164380145016,12.8369457747394,
129.305623227605)) ;
#123735=CARTESIAN_POINT('Ctrl Pts',(-23.1878595146298,12.6140529182667,
129.481009963298)) ;
#123736=CARTESIAN_POINT('Ctrl Pts',(-23.2755753916716,12.4507322880218,
129.704266224405)) ;
#123737=CARTESIAN_POINT('Ctrl Pts',(-23.3750284522621,12.3558899058093,
129.961628164076)) ;
#123738=CARTESIAN_POINT('Ctrl Pts',(-23.479686446813,12.3380969168945,130.23411873229)) ;
#123739=CARTESIAN_POINT('Ctrl Pts',(-23.5815749533041,12.3976017184894,
130.498816720526)) ;
#123740=CARTESIAN_POINT('Ctrl Pts',(-23.6757182527375,12.5305839180843,
130.740682440716)) ;
#123741=CARTESIAN_POINT('Ctrl Pts',(-23.7554851540154,12.7283491883042,
130.94048328736)) ;
#123742=CARTESIAN_POINT('Ctrl Pts',(-23.8154207293665,12.97427729496,131.082573958484)) ;
#123743=CARTESIAN_POINT('Ctrl Pts',(-23.8527220355737,13.2539378203869,
131.158329529293)) ;
#123744=CARTESIAN_POINT('Ctrl Pts',(-23.8649208036644,13.5450905398915,
131.160841634587)) ;
#123745=CARTESIAN_POINT('Ctrl Pts',(-23.8520257273945,13.8275789493197,
131.090028727836)) ;
#123746=CARTESIAN_POINT('Ctrl Pts',(-23.8158317196429,14.0806196920483,
130.951236564935)) ;
#123747=CARTESIAN_POINT('Ctrl Pts',(-23.7591250103948,14.2877393448121,
130.75229965692)) ;
#123748=CARTESIAN_POINT('Ctrl Pts',(-23.6878258800452,14.4312139219373,
130.511104094141)) ;
#123749=CARTESIAN_POINT('Ctrl Pts',(-23.6063043055212,14.5038738405656,
130.239697508234)) ;
#123750=CARTESIAN_POINT('Ctrl Pts',(-23.5222933412203,14.4984557258389,
129.961208367374)) ;
#123751=CARTESIAN_POINT('Ctrl Pts',(-23.4420014140057,14.4164646007505,
129.693550319471)) ;
#123752=CARTESIAN_POINT('Ctrl Pts',(-23.3717344521323,14.262213927018,129.455014247246)) ;
#123753=CARTESIAN_POINT('Ctrl Pts',(-23.3180679682701,14.0497488038025,
129.265295151587)) ;
#123754=CARTESIAN_POINT('Ctrl Pts',(-23.28462466296,13.7905256830516,129.134359382709)) ;
#123755=CARTESIAN_POINT('Ctrl Pts',(-23.2750637821878,13.5064863468517,
129.073396466717)) ;
#123756=CARTESIAN_POINT('Ctrl Pts',(-23.2908264747081,13.2142514411646,
129.08613493592)) ;
#123757=CARTESIAN_POINT('Ctrl Pts',(-23.3308877115697,12.9406231812218,
129.170310866248)) ;
#123758=CARTESIAN_POINT('Ctrl Pts',(-23.3941166605255,12.6982138034392,
129.321733729284)) ;
#123759=CARTESIAN_POINT('Ctrl Pts',(-23.4755974532675,12.5096111619529,
129.5267733723)) ;
#123760=CARTESIAN_POINT('Ctrl Pts',(-23.5716249889959,12.3850648455084,
129.773982751165)) ;
#123761=CARTESIAN_POINT('Ctrl Pts',(-23.6743192939801,12.3359713262841,
130.040989207269)) ;
#123762=CARTESIAN_POINT('Ctrl Pts',(-23.7783222708398,12.3641515786215,
130.311684259488)) ;
#123763=CARTESIAN_POINT('Ctrl Pts',(-23.8766296215748,12.4683944870956,
130.565716794751)) ;
#123764=CARTESIAN_POINT('Ctrl Pts',(-23.9628554188596,12.6414744959111,
130.784415332904)) ;
#123765=CARTESIAN_POINT('Ctrl Pts',(-24.0312224543575,12.8692739699043,
130.951123740549)) ;
#123766=CARTESIAN_POINT('Ctrl Pts',(-24.0782810666364,13.1394382776975,
131.05524281683)) ;
#123767=CARTESIAN_POINT('Ctrl Pts',(-24.1005117267227,13.4257125359272,
131.08734716251)) ;
#123768=CARTESIAN_POINT('Ctrl Pts',(-24.0978093052541,13.7153678906251,
131.046186164397)) ;
#123769=CARTESIAN_POINT('Ctrl Pts',(-24.0707432978629,13.9823826139753,
130.934062209111)) ;
#123770=CARTESIAN_POINT('Ctrl Pts',(-24.0219040196936,14.2103512804348,
130.758187634576)) ;
#123771=CARTESIAN_POINT('Ctrl Pts',(-23.955849643307,14.3810373660196,130.532168758405)) ;
#123772=CARTESIAN_POINT('Ctrl Pts',(-23.8777434923671,14.4835203984391,
130.270877518445)) ;
#123773=CARTESIAN_POINT('Ctrl Pts',(-23.7940757142471,14.5102051461734,
129.993379912309)) ;
#123774=CARTESIAN_POINT('Ctrl Pts',(-23.710961553393,14.4584272237243,129.717276640743)) ;
#123775=CARTESIAN_POINT('Ctrl Pts',(-23.6363573990903,14.3332271033523,
129.466355935255)) ;
#123776=CARTESIAN_POINT('Ctrl Pts',(-23.5751477681758,14.1422678192608,
129.25437061071)) ;
#123777=CARTESIAN_POINT('Ctrl Pts',(-23.5330528209132,13.9003525396715,
129.09833046808)) ;
#123778=CARTESIAN_POINT('Ctrl Pts',(-23.5135309290713,13.6237174619485,
129.008149760957)) ;
#123779=CARTESIAN_POINT('Ctrl Pts',(-23.5188554697474,13.3329586763548,
128.990586666945)) ;
#123780=CARTESIAN_POINT('Ctrl Pts',(-23.5493589827656,13.0482789829305,
129.04653418521)) ;
#123781=CARTESIAN_POINT('Ctrl Pts',(-23.6036561801052,12.7905982685052,
129.171990054986)) ;
#123782=CARTESIAN_POINT('Ctrl Pts',(-23.6780760446673,12.5792073074467,
129.356398168754)) ;
#123783=CARTESIAN_POINT('Ctrl Pts',(-23.7687620320097,12.4271419499118,
129.588159424932)) ;
#123784=CARTESIAN_POINT('Ctrl Pts',(-23.8695614818099,12.3466854310429,
129.849494389191)) ;
#123785=CARTESIAN_POINT('Ctrl Pts',(-23.9740330662146,12.3433384713207,
130.121551280678)) ;
#123786=CARTESIAN_POINT('Ctrl Pts',(-24.0753253630592,12.4172569566232,
130.384352183791)) ;
#123787=CARTESIAN_POINT('Ctrl Pts',(-24.1671079597041,12.5633305895845,
130.619334311793)) ;
#123788=CARTESIAN_POINT('Ctrl Pts',(-24.2433540945366,12.7708595617965,
130.808958800106)) ;
#123789=CARTESIAN_POINT('Ctrl Pts',(-24.2994637691932,13.025326544213,130.939726803943)) ;
#123790=CARTESIAN_POINT('Ctrl Pts',(-24.3320328505517,13.3082180027096,
131.001740671946)) ;
#123791=CARTESIAN_POINT('Ctrl Pts',(-24.3395000117594,13.5990346851552,
130.990457636508)) ;
#123792=CARTESIAN_POINT('Ctrl Pts',(-24.3221220233207,13.8774217687766,
130.906582943428)) ;
#123793=CARTESIAN_POINT('Ctrl Pts',(-24.2816282044918,14.1239850259666,
130.755070979699)) ;
#123794=CARTESIAN_POINT('Ctrl Pts',(-24.2220244331506,14.3192777030772,
130.547886906491)) ;
#123795=CARTESIAN_POINT('Ctrl Pts',(-24.1480694747946,14.450773280104,130.298730541153)) ;
#123796=CARTESIAN_POINT('Ctrl Pts',(-24.0658520531097,14.5087792742394,
130.025451200729)) ;
#123797=CARTESIAN_POINT('Ctrl Pts',(-23.9816472191313,14.4887238114624,
129.746232190085)) ;
#123798=CARTESIAN_POINT('Ctrl Pts',(-23.9030406933561,14.3928284673273,
129.483590372223)) ;
#123799=CARTESIAN_POINT('Ctrl Pts',(-23.8353522715895,14.2263681576049,
129.252580503077)) ;
#123800=CARTESIAN_POINT('Ctrl Pts',(-23.7851963074406,14.0038696004935,
129.073071183983)) ;
#123801=CARTESIAN_POINT('Ctrl Pts',(-23.7560978597235,13.7389371650263,
128.954921255289)) ;
#123802=CARTESIAN_POINT('Ctrl Pts',(-23.7511852521391,13.4518073481161,
128.907486201909)) ;
#123803=CARTESIAN_POINT('Ctrl Pts',(-23.7715448720785,13.1616327343089,
128.933759632755)) ;
#123804=CARTESIAN_POINT('Ctrl Pts',(-23.8164865399758,12.8906304369754,
129.031889334722)) ;
#123805=CARTESIAN_POINT('Ctrl Pts',(-23.8832622051985,12.6585325356575,
129.193895242853)) ;
#123806=CARTESIAN_POINT('Ctrl Pts',(-23.9677809880381,12.4808578781887,
129.407766266249)) ;
#123807=CARTESIAN_POINT('Ctrl Pts',(-24.0659555708553,12.3697949694261,
129.661183417758)) ;
#123808=CARTESIAN_POINT('Ctrl Pts',(-24.1692259037943,12.3353140236409,
129.929908779407)) ;
#123809=CARTESIAN_POINT('Ctrl Pts',(-24.2728675346327,12.3783402030792,
130.199476077674)) ;
#123810=CARTESIAN_POINT('Ctrl Pts',(-24.3690489704881,12.4961138022352,
130.447389063353)) ;
#123811=CARTESIAN_POINT('Ctrl Pts',(-24.4521938819029,12.680095634731,130.657178424642)) ;
#123812=CARTESIAN_POINT('Ctrl Pts',(-24.5170522529408,12.9180877630852,
130.813452787442)) ;
#123813=CARTESIAN_POINT('Ctrl Pts',(-24.5593190809153,13.1911275854678,
130.903877630391)) ;
#123814=CARTESIAN_POINT('Ctrl Pts',(-24.5771155225395,13.4815073291889,
130.92272617817)) ;
#123815=CARTESIAN_POINT('Ctrl Pts',(-24.5695556225141,13.7684315330807,
130.867412489067)) ;
#123816=CARTESIAN_POINT('Ctrl Pts',(-24.538185743673,14.0290764110969,130.742738622054)) ;
#123817=CARTESIAN_POINT('Ctrl Pts',(-24.4856997530283,14.247309485019,130.556233652384)) ;
#123818=CARTESIAN_POINT('Ctrl Pts',(-24.4171085411696,14.4057092189414,
130.322868851461)) ;
#123819=CARTESIAN_POINT('Ctrl Pts',(-24.3371267720653,14.4946179014392,
130.055968417117)) ;
#123820=CARTESIAN_POINT('Ctrl Pts',(-24.2532493451519,14.5063975048984,
129.777903719166)) ;
#123821=CARTESIAN_POINT('Ctrl Pts',(-24.1711402608767,14.4401277902918,
129.504748463371)) ;
#123822=CARTESIAN_POINT('Ctrl Pts',(-24.0987765462439,14.3020000140496,
129.26040859703)) ;
#123823=CARTESIAN_POINT('Ctrl Pts',(-24.0408047371062,14.1003807123236,
129.057906743614)) ;
#123824=CARTESIAN_POINT('Ctrl Pts',(-24.0026765942932,13.8504600276244,
128.91342573659)) ;
#123825=CARTESIAN_POINT('Ctrl Pts',(-23.9876880401048,13.5690358349625,
128.836430226861)) ;
#123826=CARTESIAN_POINT('Ctrl Pts',(-23.9979033292696,13.2773475296497,
128.833089888645)) ;
#123827=CARTESIAN_POINT('Ctrl Pts',(-24.0328593108588,12.9978263790817,
128.902233054104)) ;
#123828=CARTESIAN_POINT('Ctrl Pts',(-24.0912618908182,12.7470236955785,
129.039657768494)) ;
#123829=CARTESIAN_POINT('Ctrl Pts',(-24.1692879855488,12.545343046617,129.234506974647)) ;
#123830=CARTESIAN_POINT('Ctrl Pts',(-24.2623972637648,12.4062332571894,
129.473344009218)) ;
#123831=CARTESIAN_POINT('Ctrl Pts',(-24.3641009492219,12.3400677783264,
129.737415771207)) ;
#123832=CARTESIAN_POINT('Ctrl Pts',(-24.469019024179,12.3515723275397,130.010611884495)) ;
#123833=CARTESIAN_POINT('Ctrl Pts',(-24.5686909269355,12.4396026158797,
130.268772857004)) ;
#123834=CARTESIAN_POINT('Ctrl Pts',(-24.658038837005,12.5983880408564,130.496613023796)) ;
#123835=CARTESIAN_POINT('Ctrl Pts',(-24.7306514855706,12.8155082856179,
130.675695316862)) ;
#123836=CARTESIAN_POINT('Ctrl Pts',(-24.7827238953065,13.0777481932152,
130.79455185343)) ;
#123837=CARTESIAN_POINT('Ctrl Pts',(-24.810519400862,13.364000804506,130.842603809486)) ;
#123838=CARTESIAN_POINT('Ctrl Pts',(-24.8132060187631,13.6530970935561,
130.817462981774)) ;
#123839=CARTESIAN_POINT('Ctrl Pts',(-24.7912152875116,13.9274411059631,
130.720031019279)) ;
#123840=CARTESIAN_POINT('Ctrl Pts',(-24.7468930831162,14.1649405749744,
130.557453547458)) ;
#123841=CARTESIAN_POINT('Ctrl Pts',(-24.6839050837765,14.3499177041157,
130.340235768366)) ;
#123842=CARTESIAN_POINT('Ctrl Pts',(-24.6078837456822,14.4676736772021,
130.085060886655)) ;
#123843=CARTESIAN_POINT('Ctrl Pts',(-24.5251215807483,14.5109849191037,
129.810302884381)) ;
#123844=CARTESIAN_POINT('Ctrl Pts',(-24.4413268590606,14.4763368013962,
129.532269637636)) ;
#123845=CARTESIAN_POINT('Ctrl Pts',(-24.364295503168,14.3664425306899,129.274177702535)) ;
#123846=CARTESIAN_POINT('Ctrl Pts',(-24.2995399933717,14.188260258707,129.051786368571)) ;
#123847=CARTESIAN_POINT('Ctrl Pts',(-24.253049988188,13.9563928722856,128.882950063364)) ;
#123848=CARTESIAN_POINT('Ctrl Pts',(-24.2283801196271,13.6856074997971,
128.77773581213)) ;
#123849=CARTESIAN_POINT('Ctrl Pts',(-24.2281882394076,13.3967977975017,
128.744126623715)) ;
#123850=CARTESIAN_POINT('Ctrl Pts',(-24.2533268914288,13.1083771825577,
128.784333743028)) ;
#123851=CARTESIAN_POINT('Ctrl Pts',(-24.3025480715288,12.8436200801875,
128.895028676077)) ;
#123852=CARTESIAN_POINT('Ctrl Pts',(-24.373340176417,12.6197329194616,129.068631449711)) ;
#123853=CARTESIAN_POINT('Ctrl Pts',(-24.4608094763246,12.4541609796659,
129.291101417274)) ;
#123854=CARTESIAN_POINT('Ctrl Pts',(-24.5602240039795,12.357518085621,129.548297185279)) ;
#123855=CARTESIAN_POINT('Ctrl Pts',(-24.6639285825146,12.3374075405641,
129.818292847781)) ;
#123856=CARTESIAN_POINT('Ctrl Pts',(-24.7667954318842,12.3950240901617,
130.085577579692)) ;
#123857=CARTESIAN_POINT('Ctrl Pts',(-24.8608236287849,12.5255975503683,
130.327260647649)) ;
#123858=CARTESIAN_POINT('Ctrl Pts',(-24.9413203502761,12.7221237769604,
130.529099363759)) ;
#123859=CARTESIAN_POINT('Ctrl Pts',(-25.0018011512601,12.9666439794892,
130.672820785154)) ;
#123860=CARTESIAN_POINT('Ctrl Pts',(-25.0398820518506,13.2467844847395,
130.750722329137)) ;
#123861=CARTESIAN_POINT('Ctrl Pts',(-25.0526700185416,13.5364086840901,
130.75512517665)) ;
#123862=CARTESIAN_POINT('Ctrl Pts',(-25.0405775899547,13.8193015445878,
130.686678315808)) ;
#123863=CARTESIAN_POINT('Ctrl Pts',(-25.0049851130658,14.0737432295645,
130.549605084074)) ;
#123864=CARTESIAN_POINT('Ctrl Pts',(-24.9488992260672,14.28233845815,130.352522488622)) ;
#123865=CARTESIAN_POINT('Ctrl Pts',(-24.8777495315051,14.428082061538,130.111665614575)) ;
#123866=CARTESIAN_POINT('Ctrl Pts',(-24.7968113224133,14.5027907453993,
129.842125577233)) ;
#123867=CARTESIAN_POINT('Ctrl Pts',(-24.712133705096,14.4996008871204,129.561426321041)) ;
#123868=CARTESIAN_POINT('Ctrl Pts',(-24.6321001925199,14.419843429899,129.29470250768)) ;
#123869=CARTESIAN_POINT('Ctrl Pts',(-24.561546919159,14.2682254316152,129.055404210481)) ;
#123870=CARTESIAN_POINT('Ctrl Pts',(-24.5071324236837,14.0566690769085,
128.863388893838)) ;
#123871=CARTESIAN_POINT('Ctrl Pts',(-24.4730352300617,13.7984045254372,
128.730536223149)) ;
#123872=CARTESIAN_POINT('Ctrl Pts',(-24.462811119128,13.5146253545805,128.667609596018)) ;
#123873=CARTESIAN_POINT('Ctrl Pts',(-24.4776804248282,13.223790028339,128.677916277619)) ;
#123874=CARTESIAN_POINT('Ctrl Pts',(-24.5172399081723,12.9476428894619,
128.760415328231)) ;
#123875=CARTESIAN_POINT('Ctrl Pts',(-24.5799331508047,12.7041857857084,
128.9102832082)) ;
#123876=CARTESIAN_POINT('Ctrl Pts',(-24.6608098075135,12.5142907834555,
129.113613331222)) ;
#123877=CARTESIAN_POINT('Ctrl Pts',(-24.7563003807409,12.3877724095918,
129.359323075658)) ;
#123878=CARTESIAN_POINT('Ctrl Pts',(-24.8593314709221,12.336191203021,129.627164443025)) ;
#123879=CARTESIAN_POINT('Ctrl Pts',(-24.9633392047127,12.3624798343251,
129.897889938277)) ;
#123880=CARTESIAN_POINT('Ctrl Pts',(-25.0615038639838,12.4640688198504,
130.151643847771)) ;
#123881=CARTESIAN_POINT('Ctrl Pts',(-25.1484909257269,12.6358046378966,
130.372452643299)) ;
#123882=CARTESIAN_POINT('Ctrl Pts',(-25.2172355488953,12.8620488663086,
130.54031108306)) ;
#123883=CARTESIAN_POINT('Ctrl Pts',(-25.264871833393,13.1294243702491,130.646328078678)) ;
#123884=CARTESIAN_POINT('Ctrl Pts',(-25.2880788707182,13.4191275485285,
130.68085061096)) ;
#123885=CARTESIAN_POINT('Ctrl Pts',(-25.2860495181123,13.7060585191979,
130.642009964889)) ;
#123886=CARTESIAN_POINT('Ctrl Pts',(-25.259565164561,13.9758635048128,130.531352932413)) ;
#123887=CARTESIAN_POINT('Ctrl Pts',(-25.2113485262632,14.2044690848735,
130.357391673997)) ;
#123888=CARTESIAN_POINT('Ctrl Pts',(-25.145657524814,14.3772046545246,130.132389371412)) ;
#123889=CARTESIAN_POINT('Ctrl Pts',(-25.0678187426741,14.4817041714967,
129.871892743955)) ;
#123890=CARTESIAN_POINT('Ctrl Pts',(-24.9841332217802,14.5103977603672,
129.594305292428)) ;
#123891=CARTESIAN_POINT('Ctrl Pts',(-24.9014475126332,14.4613877005576,
129.319684050441)) ;
#123892=CARTESIAN_POINT('Ctrl Pts',(-24.8261139461188,14.3378670133984,
129.066461861856)) ;
#123893=CARTESIAN_POINT('Ctrl Pts',(-24.7645055171052,14.1487648805611,
128.853351786338)) ;
#123894=CARTESIAN_POINT('Ctrl Pts',(-24.7217158233187,13.9077123498208,
128.695220753593)) ;
#123895=CARTESIAN_POINT('Ctrl Pts',(-24.70153541607,13.6318347847728,128.603127426418)) ;
#123896=CARTESIAN_POINT('Ctrl Pts',(-24.7061472404895,13.3411960486728,
128.583480186491)) ;
#123897=CARTESIAN_POINT('Ctrl Pts',(-24.7359035401613,13.0563345512955,
128.637281218857)) ;
#123898=CARTESIAN_POINT('Ctrl Pts',(-24.7895403296563,12.7976620834808,
128.760811148666)) ;
#123899=CARTESIAN_POINT('Ctrl Pts',(-24.8633359396006,12.5846251876044,
128.94341366769)) ;
#123900=CARTESIAN_POINT('Ctrl Pts',(-24.9543879402352,12.429833205716,129.17599010507)) ;
#123901=CARTESIAN_POINT('Ctrl Pts',(-25.0540797760828,12.3481748441672,
129.434397942324)) ;
#123902=CARTESIAN_POINT('Ctrl Pts',(-25.1589469114049,12.3422836443017,
129.707474708614)) ;
#123903=CARTESIAN_POINT('Ctrl Pts',(-25.2603506516879,12.4141623973689,
129.970624791442)) ;
#123904=CARTESIAN_POINT('Ctrl Pts',(-25.3525979224572,12.5584918127645,
130.206923087342)) ;
#123905=CARTESIAN_POINT('Ctrl Pts',(-25.4292776741146,12.7644626666543,
130.39783234548)) ;
#123906=CARTESIAN_POINT('Ctrl Pts',(-25.4859302720378,13.0174117066364,
130.530239879527)) ;
#123907=CARTESIAN_POINT('Ctrl Pts',(-25.5192334320429,13.2998966428893,
130.594380331104)) ;
#123908=CARTESIAN_POINT('Ctrl Pts',(-25.52743704701,13.5908801629709,130.585237694254)) ;
#123909=CARTESIAN_POINT('Ctrl Pts',(-25.5106586822041,13.8706961833489,
130.503017637028)) ;
#123910=CARTESIAN_POINT('Ctrl Pts',(-25.4707228131626,14.1180204039502,
130.353167605114)) ;
#123911=CARTESIAN_POINT('Ctrl Pts',(-25.4117996734716,14.3143766861394,
130.14807480119)) ;
#123912=CARTESIAN_POINT('Ctrl Pts',(-25.33799703275,14.4481661316014,129.899283579083)) ;
#123913=CARTESIAN_POINT('Ctrl Pts',(-25.256130538496,14.508083869743,129.627114688912)) ;
#123914=CARTESIAN_POINT('Ctrl Pts',(-25.171950397789,14.490551827571,129.347998386774)) ;
#123915=CARTESIAN_POINT('Ctrl Pts',(-25.0928509136473,14.3964091806781,
129.083806315848)) ;
#123916=CARTESIAN_POINT('Ctrl Pts',(-25.0249827301023,14.2323049271919,
128.852381341929)) ;
#123917=CARTESIAN_POINT('Ctrl Pts',(-24.9741907545614,14.0113006230555,
128.67099775518)) ;
#123918=CARTESIAN_POINT('Ctrl Pts',(-24.9443961472462,13.7469852751569,
128.550772683403)) ;
#123919=CARTESIAN_POINT('Ctrl Pts',(-24.9387279867118,13.4601450927403,
128.5011244625)) ;
#123920=CARTESIAN_POINT('Ctrl Pts',(-24.9585569147683,13.1687002988962,
128.525718513046)) ;
#123921=CARTESIAN_POINT('Ctrl Pts',(-25.0024370229123,12.8989650808956,
128.621013115827)) ;
#123922=CARTESIAN_POINT('Ctrl Pts',(-25.0691511475481,12.6635916502146,
128.782564629959)) ;
#123923=CARTESIAN_POINT('Ctrl Pts',(-25.1528982004687,12.4852398029377,
128.994341478292)) ;
#123924=CARTESIAN_POINT('Ctrl Pts',(-25.2508294675198,12.371925952002,129.247023302253)) ;
#123925=CARTESIAN_POINT('Ctrl Pts',(-25.3538720853292,12.3351771027553,
129.515132724498)) ;
#123926=CARTESIAN_POINT('Ctrl Pts',(-25.4579330532035,12.3762351051066,
129.785816630675)) ;
#123927=CARTESIAN_POINT('Ctrl Pts',(-25.5539034139904,12.4911992471527,
130.033297211774)) ;
#123928=CARTESIAN_POINT('Ctrl Pts',(-25.6380661056327,12.6745749417996,
130.245838468086)) ;
#123929=CARTESIAN_POINT('Ctrl Pts',(-25.7032387958614,12.9105841492293,
130.403148858585)) ;
#123930=CARTESIAN_POINT('Ctrl Pts',(-25.7462934438778,13.1834575977754,
130.495797184592)) ;
#123931=CARTESIAN_POINT('Ctrl Pts',(-25.7646883536981,13.472817267858,130.516488970866)) ;
#123932=CARTESIAN_POINT('Ctrl Pts',(-25.7580233507089,13.7593252919433,
130.463899550352)) ;
#123933=CARTESIAN_POINT('Ctrl Pts',(-25.7270360041595,14.0229112267302,
130.34008351448)) ;
#123934=CARTESIAN_POINT('Ctrl Pts',(-25.675498907428,14.2409569319606,130.156613033591)) ;
#123935=CARTESIAN_POINT('Ctrl Pts',(-25.6068834624728,14.4024703207306,
129.922947324608)) ;
#123936=CARTESIAN_POINT('Ctrl Pts',(-25.5273592175764,14.4930253207348,
129.657498279644)) ;
#123937=CARTESIAN_POINT('Ctrl Pts',(-25.4434689272461,14.5071137946879,
129.379370355167)) ;
#123938=CARTESIAN_POINT('Ctrl Pts',(-25.3615278491778,14.4434721690138,
129.106846352464)) ;
#123939=CARTESIAN_POINT('Ctrl Pts',(-25.2885360407668,14.3072990407348,
128.86057381183)) ;
#123940=CARTESIAN_POINT('Ctrl Pts',(-25.2298270357142,14.1061280190249,
128.655755058378)) ;
#123941=CARTESIAN_POINT('Ctrl Pts',(-25.1913201297001,13.8584456467317,
128.510325342625)) ;
#123942=CARTESIAN_POINT('Ctrl Pts',(-25.1755647513378,13.5782525507237,
128.431150931071)) ;
#123943=CARTESIAN_POINT('Ctrl Pts',(-25.1849885107696,13.2862403685174,
128.425460714649)) ;
#123944=CARTESIAN_POINT('Ctrl Pts',(-25.2192755405819,13.0054671404376,
128.492579206751)) ;
#123945=CARTESIAN_POINT('Ctrl Pts',(-25.2773394240981,12.7527976757228,
128.628896842881)) ;
#123946=CARTESIAN_POINT('Ctrl Pts',(-25.3544373750974,12.5507720823643,
128.821226560556)) ;
#123947=CARTESIAN_POINT('Ctrl Pts',(-25.4472393440595,12.4092692851511,
129.059132005569)) ;
#123948=CARTESIAN_POINT('Ctrl Pts',(-25.5489779403507,12.3409405879061,
129.323242391553)) ;
#123949=CARTESIAN_POINT('Ctrl Pts',(-25.6535733607532,12.3499819514293,
129.595610275213)) ;
#123950=CARTESIAN_POINT('Ctrl Pts',(-25.7539733542539,12.4363532900494,
129.855724418261)) ;
#123951=CARTESIAN_POINT('Ctrl Pts',(-25.8432653409665,12.592566468637,130.083565255521)) ;
#123952=CARTESIAN_POINT('Ctrl Pts',(-25.9166293802248,12.808517161013,130.264767590827)) ;
#123953=CARTESIAN_POINT('Ctrl Pts',(-25.9692694104626,13.0694867381501,
130.385320946943)) ;
#123954=CARTESIAN_POINT('Ctrl Pts',(-25.9978655735776,13.3550372325075,
130.435738703826)) ;
#123955=CARTESIAN_POINT('Ctrl Pts',(-26.0012228110646,13.6462143914832,
130.41233473643)) ;
#123956=CARTESIAN_POINT('Ctrl Pts',(-25.9799786820042,13.9195288326514,
130.317292866585)) ;
#123957=CARTESIAN_POINT('Ctrl Pts',(-25.9362831066957,14.1586151342569,
130.156518689827)) ;
#123958=CARTESIAN_POINT('Ctrl Pts',(-25.873895400124,14.3449690064031,129.941121871803)) ;
#123959=CARTESIAN_POINT('Ctrl Pts',(-25.798230728825,14.4652397459023,129.686991964219)) ;
#123960=CARTESIAN_POINT('Ctrl Pts',(-25.7149306992069,14.5107689860091,
129.410403584569)) ;
#123961=CARTESIAN_POINT('Ctrl Pts',(-25.6318516915594,14.4787461953136,
129.134788811335)) ;
#123962=CARTESIAN_POINT('Ctrl Pts',(-25.5538394007471,14.3700644333909,
128.873522851825)) ;
#123963=CARTESIAN_POINT('Ctrl Pts',(-25.4891252246343,14.1946408209154,
128.651483185167)) ;
#123964=CARTESIAN_POINT('Ctrl Pts',(-25.4419035532708,13.9639077381356,
128.480442817708)) ;
#123965=CARTESIAN_POINT('Ctrl Pts',(-25.416526533386,13.6940409342519,128.373177036019)) ;
#123966=CARTESIAN_POINT('Ctrl Pts',(-25.4156877261185,13.4043243870117,
128.337540729079)) ;
#123967=CARTESIAN_POINT('Ctrl Pts',(-25.4398971208575,13.1175424203496,
128.375270653993)) ;
#123968=CARTESIAN_POINT('Ctrl Pts',(-25.4887349254359,12.8501253800453,
128.484627505498)) ;
#123969=CARTESIAN_POINT('Ctrl Pts',(-25.5586262014652,12.6260375072132,
128.655777801442)) ;
#123970=CARTESIAN_POINT('Ctrl Pts',(-25.6457761900823,12.4581544955602,
128.877254650212)) ;
#123971=CARTESIAN_POINT('Ctrl Pts',(-25.7447128579694,12.3594525317711,
129.13313074971)) ;
#123972=CARTESIAN_POINT('Ctrl Pts',(-25.8487073343646,12.3367944106136,
129.403860832314)) ;
#123973=CARTESIAN_POINT('Ctrl Pts',(-25.9519835342391,12.3925085766977,
129.672255974499)) ;
#123974=CARTESIAN_POINT('Ctrl Pts',(-26.0462967491219,12.5213899475148,
129.914765311702)) ;
#123975=CARTESIAN_POINT('Ctrl Pts',(-26.1270148304609,12.715572513745,130.117365292637)) ;
#123976=CARTESIAN_POINT('Ctrl Pts',(-26.1882034971608,12.9595222132268,
130.263073734265)) ;
#123977=CARTESIAN_POINT('Ctrl Pts',(-26.2267435953605,13.2367790657483,
130.342576650586)) ;
#123978=CARTESIAN_POINT('Ctrl Pts',(-26.2404887282104,13.5277645483974,
130.34960696324)) ;
#123979=CARTESIAN_POINT('Ctrl Pts',(-26.2290166843068,13.8120455612361,
130.282873037212)) ;
#123980=CARTESIAN_POINT('Ctrl Pts',(-26.1939550681954,14.0676656402339,
130.147320284264)) ;
#123981=CARTESIAN_POINT('Ctrl Pts',(-26.1385064231525,14.2771421243593,
129.952187707759)) ;
#123982=CARTESIAN_POINT('Ctrl Pts',(-26.0677264199933,14.4250319650245,
129.712403604366)) ;
#123983=CARTESIAN_POINT('Ctrl Pts',(-25.9866105764485,14.5017260343279,
129.442204203795)) ;
#123984=CARTESIAN_POINT('Ctrl Pts',(-25.9029004553032,14.5010098763796,
129.164720483973)) ;
#123985=CARTESIAN_POINT('Ctrl Pts',(-25.8219478737643,14.4231232861786,
128.895020725302)) ;
#123986=CARTESIAN_POINT('Ctrl Pts',(-25.7512036699718,14.2735699420865,
128.655246017135)) ;
#123987=CARTESIAN_POINT('Ctrl Pts',(-25.6961574433566,14.0631259217895,
128.461311286501)) ;
#123988=CARTESIAN_POINT('Ctrl Pts',(-25.6615347817568,13.8068511447586,
128.327046916864)) ;
#123989=CARTESIAN_POINT('Ctrl Pts',(-25.6505331648762,13.5229066982492,
128.261764796241)) ;
#123990=CARTESIAN_POINT('Ctrl Pts',(-25.6646712038547,13.2323183656793,
128.269978142886)) ;
#123991=CARTESIAN_POINT('Ctrl Pts',(-25.7035121417102,12.9554622848227,
128.35037611329)) ;
#123992=CARTESIAN_POINT('Ctrl Pts',(-25.7655162081559,12.7108336294588,
128.498254383038)) ;
#123993=CARTESIAN_POINT('Ctrl Pts',(-25.846073101608,12.5189036240624,128.700584553235)) ;
#123994=CARTESIAN_POINT('Ctrl Pts',(-25.9409316376887,12.390658589764,128.944555230365)) ;
#123995=CARTESIAN_POINT('Ctrl Pts',(-26.0439737290693,12.3366531307129,
129.212373718036)) ;
#123996=CARTESIAN_POINT('Ctrl Pts',(-26.1478846663642,12.3602977893096,
129.482879326308)) ;
#123997=CARTESIAN_POINT('Ctrl Pts',(-26.2471522651563,12.4609988755096,
129.739549452939)) ;
#123998=CARTESIAN_POINT('Ctrl Pts',(-26.3336049302479,12.6291274896935,
129.959164506964)) ;
#123999=CARTESIAN_POINT('Ctrl Pts',(-26.403541070526,12.8555169939373,130.130239113931)) ;
#124000=CARTESIAN_POINT('Ctrl Pts',(-26.4515909872396,13.1215885619852,
130.237543390251)) ;
#124001=CARTESIAN_POINT('Ctrl Pts',(-26.4755139644934,13.4096083947618,
130.274304939758)) ;
#124002=CARTESIAN_POINT('Ctrl Pts',(-26.4742683561914,13.6982129377788,
130.237599168761)) ;
#124003=CARTESIAN_POINT('Ctrl Pts',(-26.4483350169052,13.969145223664,130.128507626156)) ;
#124004=CARTESIAN_POINT('Ctrl Pts',(-26.4008409219027,14.1982918384811,
129.956770249216)) ;
#124005=CARTESIAN_POINT('Ctrl Pts',(-26.3357094157164,14.3728095638234,
129.733441982711)) ;
#124006=CARTESIAN_POINT('Ctrl Pts',(-26.2580598390402,14.4796622896265,
129.47345820633)) ;
#124007=CARTESIAN_POINT('Ctrl Pts',(-26.1743828769687,14.5107460885462,
129.195872130029)) ;
#124008=CARTESIAN_POINT('Ctrl Pts',(-26.091350817327,14.4636147877097,128.920140958459)) ;
#124009=CARTESIAN_POINT('Ctrl Pts',(-26.0160489320887,14.3427084446703,
128.667164147215)) ;
#124010=CARTESIAN_POINT('Ctrl Pts',(-25.9536601172443,14.1545213571348,
128.451617980833)) ;
#124011=CARTESIAN_POINT('Ctrl Pts',(-25.9103939029223,13.9146657038493,
128.292116078991)) ;
#124012=CARTESIAN_POINT('Ctrl Pts',(-25.8895873786261,13.6405171669677,
128.198310769231)) ;
#124013=CARTESIAN_POINT('Ctrl Pts',(-25.8934300722509,13.3501101589506,
128.176423228012)) ;
#124014=CARTESIAN_POINT('Ctrl Pts',(-25.9223270326843,13.0651841999784,
128.227769457602)) ;
#124015=CARTESIAN_POINT('Ctrl Pts',(-25.9756051647074,12.8038875928186,
128.350055164985)) ;
#124016=CARTESIAN_POINT('Ctrl Pts',(-26.0488715170654,12.5899464176031,
128.531156076502)) ;
#124017=CARTESIAN_POINT('Ctrl Pts',(-26.1388470008162,12.4339562439877,
128.760815215957)) ;
#124018=CARTESIAN_POINT('Ctrl Pts',(-26.2391546987785,12.3491846670138,
129.020742228805)) ;
#124019=CARTESIAN_POINT('Ctrl Pts',(-26.3440686577084,12.3415474496416,
129.293939952554)) ;
#124020=CARTESIAN_POINT('Ctrl Pts',(-26.4452555059315,12.4110292965116,
129.556580973751)) ;
#124021=CARTESIAN_POINT('Ctrl Pts',(-26.5378931940764,12.5533606733183,
129.794011949483)) ;
#124022=CARTESIAN_POINT('Ctrl Pts',(-26.615000146917,12.7574393223527,129.986210703798)) ;
#124023=CARTESIAN_POINT('Ctrl Pts',(-26.6724404028421,13.009581913367,130.120867414048)) ;
#124024=CARTESIAN_POINT('Ctrl Pts',(-26.7064847425196,13.2928228925075,
130.187026380122)) ;
#124025=CARTESIAN_POINT('Ctrl Pts',(-26.7153278695728,13.582012204951,130.179963532695)) ;
#124026=CARTESIAN_POINT('Ctrl Pts',(-26.699241537175,13.8633231100431,130.099661124816)) ;
#124027=CARTESIAN_POINT('Ctrl Pts',(-26.6600020906481,14.1112604273849,
129.951925919837)) ;
#124028=CARTESIAN_POINT('Ctrl Pts',(-26.60148356948,14.3095522815314,129.747958126555)) ;
#124029=CARTESIAN_POINT('Ctrl Pts',(-26.5282846692839,14.44510578155,129.501042571553)) ;
#124030=CARTESIAN_POINT('Ctrl Pts',(-26.4458923835004,14.5076745879146,
129.227062356217)) ;
#124031=CARTESIAN_POINT('Ctrl Pts',(-26.3618964181972,14.4918702238892,
128.94857384037)) ;
#124032=CARTESIAN_POINT('Ctrl Pts',(-26.2828570043338,14.4001695332023,
128.68467078182)) ;
#124033=CARTESIAN_POINT('Ctrl Pts',(-26.2146127566021,14.2383391968108,
128.452190174529)) ;
#124034=CARTESIAN_POINT('Ctrl Pts',(-26.1630788147266,14.0178456765348,
128.268499220438)) ;
#124035=CARTESIAN_POINT('Ctrl Pts',(-26.132665228877,13.7549023993413,128.146527433501)) ;
#124036=CARTESIAN_POINT('Ctrl Pts',(-26.1264250234098,13.4669383110673,
128.095031448519)) ;
#124037=CARTESIAN_POINT('Ctrl Pts',(-26.1451597576439,13.179287796842,128.116902786845)) ;
#124038=CARTESIAN_POINT('Ctrl Pts',(-26.1887921440493,12.9054935054356,
128.21107289621)) ;
#124039=CARTESIAN_POINT('Ctrl Pts',(-26.2543181709187,12.6708451736549,
128.369465417359)) ;
#124040=CARTESIAN_POINT('Ctrl Pts',(-26.3383737496348,12.489010935019,128.581822970063)) ;
#124041=CARTESIAN_POINT('Ctrl Pts',(-26.4349845939226,12.3747427452421,
128.831010816488)) ;
#124042=CARTESIAN_POINT('Ctrl Pts',(-26.5386809419236,12.3351181280502,
129.100771617171)) ;
#124043=CARTESIAN_POINT('Ctrl Pts',(-26.6423270739193,12.3735357239234,
129.370425059392)) ;
#124044=CARTESIAN_POINT('Ctrl Pts',(-26.739590487989,12.4876827047378,129.621327059493)) ;
#124045=CARTESIAN_POINT('Ctrl Pts',(-26.8234966069003,12.6681438766094,
129.833383660537)) ;
#124046=CARTESIAN_POINT('Ctrl Pts',(-26.8894910230064,12.9033828008646,
129.992992511596)) ;
#124047=CARTESIAN_POINT('Ctrl Pts',(-26.9330590975584,13.1743601977476,
130.087278715581)) ;
#124048=CARTESIAN_POINT('Ctrl Pts',(-26.95234321523,13.4644840524054,130.110453366062)) ;
#124049=CARTESIAN_POINT('Ctrl Pts',(-26.9462750235192,13.7518156372007,
130.059550094245)) ;
#124050=CARTESIAN_POINT('Ctrl Pts',(-26.9162087617747,14.0147481121993,
129.938641619233)) ;
#124051=CARTESIAN_POINT('Ctrl Pts',(-26.8649460510337,14.2359323146828,
129.755751034222)) ;
#124052=CARTESIAN_POINT('Ctrl Pts',(-26.7965801586489,14.3990328961567,
129.52278375049)) ;
#124053=CARTESIAN_POINT('Ctrl Pts',(-26.7177443738962,14.4913721477539,
129.259533927694)) ;
#124054=CARTESIAN_POINT('Ctrl Pts',(-26.6334108075472,14.5077030506771,
128.979913126939)) ;
#124055=CARTESIAN_POINT('Ctrl Pts',(-26.5517638677785,14.4466726392651,
128.70844483765)) ;
#124056=CARTESIAN_POINT('Ctrl Pts',(-26.4778064684304,14.3110619945875,
128.459041808409)) ;
#124057=CARTESIAN_POINT('Ctrl Pts',(-26.4192231879076,14.1132679223134,
128.25491902626)) ;
#124058=CARTESIAN_POINT('Ctrl Pts',(-26.3797981720978,13.8656263142686,
128.106626377481)) ;
#124059=CARTESIAN_POINT('Ctrl Pts',(-26.3634473247229,13.5853315264496,
128.025647675686)) ;
#124060=CARTESIAN_POINT('Ctrl Pts',(-26.3722199816823,13.2939510978671,
128.018122216624)) ;
#124061=CARTESIAN_POINT('Ctrl Pts',(-26.405714171083,13.0136079092844,128.083036282935)) ;
#124062=CARTESIAN_POINT('Ctrl Pts',(-26.4628659654867,12.7604082845335,
128.216792359251)) ;
#124063=CARTESIAN_POINT('Ctrl Pts',(-26.5397813309025,12.5556139237626,
128.408426975407)) ;
#124064=CARTESIAN_POINT('Ctrl Pts',(-26.6324107937376,12.4121627059908,
128.645779498262)) ;
#124065=CARTESIAN_POINT('Ctrl Pts',(-26.7336873599695,12.3419224610127,
128.908634855302)) ;
#124066=CARTESIAN_POINT('Ctrl Pts',(-26.8381886857235,12.3485705952627,
129.180762238741)) ;
#124067=CARTESIAN_POINT('Ctrl Pts',(-26.9387702278677,12.4325162963297,
129.441425792212)) ;
#124068=CARTESIAN_POINT('Ctrl Pts',(-27.0287520463112,12.5872707160174,
129.671176207014)) ;
#124069=CARTESIAN_POINT('Ctrl Pts',(-27.1025641524698,12.8016743120911,
129.853709459553)) ;
#124070=CARTESIAN_POINT('Ctrl Pts',(-27.1557706951775,13.0608928169866,
129.97600170914)) ;
#124071=CARTESIAN_POINT('Ctrl Pts',(-27.1851489147898,13.3463628711479,
130.02865621953)) ;
#124072=CARTESIAN_POINT('Ctrl Pts',(-27.189300141959,13.6367414871714,130.007684109365)) ;
#124073=CARTESIAN_POINT('Ctrl Pts',(-27.1687387851865,13.9121235287477,
129.914488218401)) ;
#124074=CARTESIAN_POINT('Ctrl Pts',(-27.1254953280649,14.1528033818472,
129.754974456862)) ;
#124075=CARTESIAN_POINT('Ctrl Pts',(-27.0637389687625,14.3402810469184,
129.541515996158)) ;
#124076=CARTESIAN_POINT('Ctrl Pts',(-26.9884856177373,14.4626257228514,
129.288621690848)) ;
#124077=CARTESIAN_POINT('Ctrl Pts',(-26.9051827015451,14.5106364095724,
129.011977483569)) ;
#124078=CARTESIAN_POINT('Ctrl Pts',(-26.8218668490788,14.4805445911802,
128.735600274415)) ;
#124079=CARTESIAN_POINT('Ctrl Pts',(-26.7440463514374,14.3748126734896,
128.475104392524)) ;
#124080=CARTESIAN_POINT('Ctrl Pts',(-26.6785355196267,14.2005693780012,
128.250575368186)) ;
#124081=CARTESIAN_POINT('Ctrl Pts',(-26.630780882824,13.9714225005758,128.078016941159)) ;
#124082=CARTESIAN_POINT('Ctrl Pts',(-26.6047039211808,13.7016038518799,
127.968605933267)) ;
#124083=CARTESIAN_POINT('Ctrl Pts',(-26.6030915854038,13.4137877751622,
127.930902605108)) ;
#124084=CARTESIAN_POINT('Ctrl Pts',(-26.6267380627707,13.1249621012608,
127.966780515293)) ;
#124085=CARTESIAN_POINT('Ctrl Pts',(-26.6744609448017,12.8587597894488,
128.07316158682)) ;
#124086=CARTESIAN_POINT('Ctrl Pts',(-26.7442975058962,12.6311848852698,
128.243869033046)) ;
#124087=CARTESIAN_POINT('Ctrl Pts',(-26.830903329108,12.462061420416,128.463831733263)) ;
#124088=CARTESIAN_POINT('Ctrl Pts',(-26.9296939602677,12.3611529098997,
128.719242246554)) ;
#124089=CARTESIAN_POINT('Ctrl Pts',(-27.0333937390888,12.3364027391132,
128.989188260464)) ;
#124090=CARTESIAN_POINT('Ctrl Pts',(-27.1368020606483,12.3896955050154,
129.2579744258)) ;
#124091=CARTESIAN_POINT('Ctrl Pts',(-27.2316571620167,12.5169546340526,
129.501984988792)) ;
#124092=CARTESIAN_POINT('Ctrl Pts',(-27.3126444315144,12.709001546384,129.705455771372)) ;
#124093=CARTESIAN_POINT('Ctrl Pts',(-27.3745146596021,12.9518210421532,
129.853131534273)) ;
#124094=CARTESIAN_POINT('Ctrl Pts',(-27.4137510170451,13.2283912816006,
129.934670418908)) ;
#124095=CARTESIAN_POINT('Ctrl Pts',(-27.4282191216373,13.5192446194064,
129.943814180425)) ;
#124096=CARTESIAN_POINT('Ctrl Pts',(-27.4175340945595,13.8035931145738,
129.879438970957)) ;
#124097=CARTESIAN_POINT('Ctrl Pts',(-27.383044952722,14.0607676757129,129.745489590902)) ;
#124098=CARTESIAN_POINT('Ctrl Pts',(-27.3284746860088,14.2709777793726,
129.553094789489)) ;
#124099=CARTESIAN_POINT('Ctrl Pts',(-27.2575815807168,14.4220258992613,
129.312734052738)) ;
#124100=CARTESIAN_POINT('Ctrl Pts',(-27.1769127132677,14.5004900232679,
129.043957183488)) ;
#124101=CARTESIAN_POINT('Ctrl Pts',(-27.0930692805598,14.5020985489184,
128.766023699838)) ;
#124102=CARTESIAN_POINT('Ctrl Pts',(-27.0121212643559,14.4266675394507,
128.49642621361)) ;
#124103=CARTESIAN_POINT('Ctrl Pts',(-26.9407458153866,14.2786156866751,
128.254689867483)) ;
#124104=CARTESIAN_POINT('Ctrl Pts',(-26.8852334771517,14.0697688504795,
128.059416629246)) ;
#124105=CARTESIAN_POINT('Ctrl Pts',(-26.849975543147,13.8142974441725,127.923265218697)) ;
#124106=CARTESIAN_POINT('Ctrl Pts',(-26.8382987967745,13.5318060155786,
127.856120671583)) ;
#124107=CARTESIAN_POINT('Ctrl Pts',(-26.8516696284158,13.2403760089107,
127.862009333327)) ;
#124108=CARTESIAN_POINT('Ctrl Pts',(-26.890089361851,12.9618560085294,127.941045133668)) ;
#124109=CARTESIAN_POINT('Ctrl Pts',(-26.9512286696893,12.7173262571543,
128.086563315903)) ;
#124110=CARTESIAN_POINT('Ctrl Pts',(-27.0314174703486,12.5233446116289,
128.28776106198)) ;
#124111=CARTESIAN_POINT('Ctrl Pts',(-27.1260354307218,12.3931311939353,
128.531010608056)) ;
#124112=CARTESIAN_POINT('Ctrl Pts',(-27.2291064958659,12.3370752417009,
128.79886449417)) ;
#124113=CARTESIAN_POINT('Ctrl Pts',(-27.3326646670925,12.35867646463,129.068464529043)) ;
#124114=CARTESIAN_POINT('Ctrl Pts',(-27.4317434817778,12.4563696655718,
129.324745138766)) ;
#124115=CARTESIAN_POINT('Ctrl Pts',(-27.5191780495442,12.6234424548744,
129.547033430675)) ;
#124116=CARTESIAN_POINT('Ctrl Pts',(-27.5896064413482,12.8484690633149,
129.719557189226)) ;
#124117=CARTESIAN_POINT('Ctrl Pts',(-27.6383447085001,13.1134860837276,
129.828883494931)) ;
#124118=CARTESIAN_POINT('Ctrl Pts',(-27.6630194526296,13.4024250602232,
129.867700766758)) ;
#124119=CARTESIAN_POINT('Ctrl Pts',(-27.6623953842175,13.6901681965896,
129.832935013288)) ;
#124120=CARTESIAN_POINT('Ctrl Pts',(-27.6372548988728,13.9614083334907,
129.726232762252)) ;
#124121=CARTESIAN_POINT('Ctrl Pts',(-27.5902751351061,14.1924050626967,
129.55593800189)) ;
#124122=CARTESIAN_POINT('Ctrl Pts',(-27.5255259120584,14.3688010138631,
129.333704515503)) ;
#124123=CARTESIAN_POINT('Ctrl Pts',(-27.4481016761685,14.4776662108143,
129.074365641602)) ;
#124124=CARTESIAN_POINT('Ctrl Pts',(-27.3647643666235,14.5108828487548,
128.797872509103)) ;
#124125=CARTESIAN_POINT('Ctrl Pts',(-27.28160086979,14.4662997659133,128.521759647642)) ;
#124126=CARTESIAN_POINT('Ctrl Pts',(-27.2057377958646,14.3468724175,128.26701996428)) ;
#124127=CARTESIAN_POINT('Ctrl Pts',(-27.1432603861286,14.1616148952727,
128.051421722211)) ;
#124128=CARTESIAN_POINT('Ctrl Pts',(-27.0991941479983,13.9230022148217,
127.889534238923)) ;
#124129=CARTESIAN_POINT('Ctrl Pts',(-27.0776168898842,13.6485313215457,
127.793350195976)) ;
#124130=CARTESIAN_POINT('Ctrl Pts',(-27.0807484826604,13.3583010704495,
127.76939083884)) ;
#124131=CARTESIAN_POINT('Ctrl Pts',(-27.1090520806657,13.0725041550786,
127.818945431234)) ;
#124132=CARTESIAN_POINT('Ctrl Pts',(-27.1613516583747,12.8117565584391,
127.938573083935)) ;
#124133=CARTESIAN_POINT('Ctrl Pts',(-27.234133998536,12.5955170585835,128.118185428868)) ;
#124134=CARTESIAN_POINT('Ctrl Pts',(-27.3242615124707,12.4369579838143,
128.348106217854)) ;
#124135=CARTESIAN_POINT('Ctrl Pts',(-27.4239051442321,12.3507869319176,
128.606250511175)) ;
#124136=CARTESIAN_POINT('Ctrl Pts',(-27.5283170847605,12.3404899824772,
128.878131255211)) ;
#124137=CARTESIAN_POINT('Ctrl Pts',(-27.6301884886677,12.4078495192289,
129.142611995147)) ;
#124138=CARTESIAN_POINT('Ctrl Pts',(-27.7232432838034,12.548387321603,129.381237810726)) ;
#124139=CARTESIAN_POINT('Ctrl Pts',(-27.8009955997897,12.7513534766359,
129.575254101371)) ;
#124140=CARTESIAN_POINT('Ctrl Pts',(-27.8588477984997,13.0019415175825,
129.711186382699)) ;
#124141=CARTESIAN_POINT('Ctrl Pts',(-27.8935349743183,13.2828870424453,
129.779414110512)) ;
#124142=CARTESIAN_POINT('Ctrl Pts',(-27.9032420933332,13.5743280761341,
129.774620556531)) ;
#124143=CARTESIAN_POINT('Ctrl Pts',(-27.8877912603147,13.8554589732171,
129.696260558318)) ;
#124144=CARTESIAN_POINT('Ctrl Pts',(-27.8494200240865,14.1037392604584,
129.551189336801)) ;
#124145=CARTESIAN_POINT('Ctrl Pts',(-27.7912574236898,14.3046991320609,
129.348138971575)) ;
#124146=CARTESIAN_POINT('Ctrl Pts',(-27.7180698943492,14.4424189349425,
129.101130494134)) ;
#124147=CARTESIAN_POINT('Ctrl Pts',(-27.6365275795886,14.5067209378496,
128.829911927971)) ;
#124148=CARTESIAN_POINT('Ctrl Pts',(-27.5522869891486,14.4936392386325,
128.550624236163)) ;
#124149=CARTESIAN_POINT('Ctrl Pts',(-27.472842461916,14.4040066761143,128.285476965489)) ;
#124150=CARTESIAN_POINT('Ctrl Pts',(-27.4040161809218,14.2433941808528,
128.051188349872)) ;
#124151=CARTESIAN_POINT('Ctrl Pts',(-27.3521479099506,14.0252992108477,
127.866664237617)) ;
#124152=CARTESIAN_POINT('Ctrl Pts',(-27.321003828356,13.7626962224851,127.742470842385)) ;
#124153=CARTESIAN_POINT('Ctrl Pts',(-27.3140081793116,13.4766512855246,
127.688944617931)) ;
#124154=CARTESIAN_POINT('Ctrl Pts',(-27.3320904586992,13.186696570853,127.708668192988)) ;
#124155=CARTESIAN_POINT('Ctrl Pts',(-27.3751478872209,12.9123106604455,
127.801171448176)) ;
#124156=CARTESIAN_POINT('Ctrl Pts',(-27.4399784096183,12.676940859845,127.957598680988)) ;
#124157=CARTESIAN_POINT('Ctrl Pts',(-27.5233472974592,12.4935889461196,
128.168026659701)) ;
#124158=CARTESIAN_POINT('Ctrl Pts',(-27.6201918302586,12.3766908564608,
128.417719170936)) ;
#124159=CARTESIAN_POINT('Ctrl Pts',(-27.7235786308746,12.3352383867213,
128.686650110514)) ;
#124160=CARTESIAN_POINT('Ctrl Pts',(-27.8270763638829,12.3713735993149,
128.955940427189)) ;
#124161=CARTESIAN_POINT('Ctrl Pts',(-27.9243939471655,12.482759025907,129.207099816065)) ;
#124162=CARTESIAN_POINT('Ctrl Pts',(-28.0093322756141,12.6627224299211,
129.421938016894)) ;
#124163=CARTESIAN_POINT('Ctrl Pts',(-28.0755419239468,12.8955397907263,
129.582345907045)) ;
#124164=CARTESIAN_POINT('Ctrl Pts',(-28.119969509644,13.1663559129077,129.679051355865)) ;
#124165=CARTESIAN_POINT('Ctrl Pts',(-28.139919232561,13.4563321375684,129.70416618866)) ;
#124166=CARTESIAN_POINT('Ctrl Pts',(-28.1345989094075,13.7435418421396,
129.655505344651)) ;
#124167=CARTESIAN_POINT('Ctrl Pts',(-28.1051508122028,14.0078637990346,
129.536350066241)) ;
#124168=CARTESIAN_POINT('Ctrl Pts',(-28.0545171617177,14.2299792933114,
129.355360726874)) ;
#124169=CARTESIAN_POINT('Ctrl Pts',(-27.9868221963933,14.3948659933446,
129.124446850834)) ;
#124170=CARTESIAN_POINT('Ctrl Pts',(-27.9076947051592,14.489874104301,128.860121628846)) ;
#124171=CARTESIAN_POINT('Ctrl Pts',(-27.8239321297246,14.5084149170405,
128.582385907377)) ;
#124172=CARTESIAN_POINT('Ctrl Pts',(-27.7416214849835,14.4492458860129,
128.308762621808)) ;
#124173=CARTESIAN_POINT('Ctrl Pts',(-27.6678598600451,14.3166093969371,
128.060178483998)) ;
#124174=CARTESIAN_POINT('Ctrl Pts',(-27.6084375739192,14.1198899210566,
127.853454017954)) ;
#124175=CARTESIAN_POINT('Ctrl Pts',(-27.5684481950325,13.8734077643859,
127.703525149204)) ;
#124176=CARTESIAN_POINT('Ctrl Pts',(-27.551399761937,13.5947692208086,127.62061763421)) ;
#124177=CARTESIAN_POINT('Ctrl Pts',(-27.5592798183032,13.3033323132003,
127.610476269779)) ;
#124178=CARTESIAN_POINT('Ctrl Pts',(-27.5923075525496,13.0207082772212,
127.673820091286)) ;
#124179=CARTESIAN_POINT('Ctrl Pts',(-27.6485757964368,12.7676285186634,
127.805155390212)) ;
#124180=CARTESIAN_POINT('Ctrl Pts',(-27.7251843515254,12.5604750217273,
127.995784618736)) ;
#124181=CARTESIAN_POINT('Ctrl Pts',(-27.8174211146232,12.4152915919243,
128.232013295708)) ;
#124182=CARTESIAN_POINT('Ctrl Pts',(-27.9185391559007,12.3428120384338,
128.494396627763)) ;
#124183=CARTESIAN_POINT('Ctrl Pts',(-28.023337038121,12.3473797731266,128.767302447243)) ;
#124184=CARTESIAN_POINT('Ctrl Pts',(-28.1240157714969,12.4294696184163,
129.028273300787)) ;
#124185=CARTESIAN_POINT('Ctrl Pts',(-28.2139942287922,12.5816149593444,
129.258157610135)) ;
#124186=CARTESIAN_POINT('Ctrl Pts',(-28.2885971304493,12.7949908749712,
129.442905443656)) ;
#124187=CARTESIAN_POINT('Ctrl Pts',(-28.3425258290396,13.0541013315914,
129.567209238913)) ;
#124188=CARTESIAN_POINT('Ctrl Pts',(-28.3724481699799,13.3386275615382,
129.621515697744)) ;
#124189=CARTESIAN_POINT('Ctrl Pts',(-28.3773117940733,13.6281886067776,
129.602732220181)) ;
#124190=CARTESIAN_POINT('Ctrl Pts',(-28.3574855498393,13.9042250282851,
129.511693915976)) ;
#124191=CARTESIAN_POINT('Ctrl Pts',(-28.3148907454231,14.1463904196779,
129.354066819802)) ;
#124192=CARTESIAN_POINT('Ctrl Pts',(-28.253205086578,14.3364820143999,129.140624870235)) ;
#124193=CARTESIAN_POINT('Ctrl Pts',(-28.1786223292026,14.4598817897301,
128.889868366299)) ;
#124194=CARTESIAN_POINT('Ctrl Pts',(-28.095592031095,14.5104486172097,128.61407158427)) ;
#124195=CARTESIAN_POINT('Ctrl Pts',(-28.0117388077113,14.4822486282368,
128.33593709542)) ;
#124196=CARTESIAN_POINT('Ctrl Pts',(-27.9341428136596,14.3791732925603,
128.076300893861)) ;
#124197=CARTESIAN_POINT('Ctrl Pts',(-27.867892600365,14.2063740239316,127.849490613762)) ;
#124198=CARTESIAN_POINT('Ctrl Pts',(-27.8195738401177,13.977776586442,127.675203409093)) ;
#124199=CARTESIAN_POINT('Ctrl Pts',(-27.7929572214305,13.7109259547803,
127.564468320854)) ;
#124200=CARTESIAN_POINT('Ctrl Pts',(-27.7905925854493,13.4211174219504,
127.524298821139)) ;
#124201=CARTESIAN_POINT('Ctrl Pts',(-27.8134496811496,13.1336909374666,
127.558070503479)) ;
#124202=CARTESIAN_POINT('Ctrl Pts',(-27.8605400703067,12.8658812614538,
127.662521352308)) ;
#124203=CARTESIAN_POINT('Ctrl Pts',(-27.9298825210266,12.6367690077997,
127.831765044912)) ;
#124204=CARTESIAN_POINT('Ctrl Pts',(-28.0161685887183,12.4658337758404,
128.050762811657)) ;
#124205=CARTESIAN_POINT('Ctrl Pts',(-28.1143654830391,12.363124510772,128.30455384214)) ;
#124206=CARTESIAN_POINT('Ctrl Pts',(-28.2182189316931,12.3360466249849,
128.574875482197)) ;
#124207=CARTESIAN_POINT('Ctrl Pts',(-28.3213869556432,12.3868688211213,
128.843082429485)) ;
#124208=CARTESIAN_POINT('Ctrl Pts',(-28.4166731561539,12.5119418808478,
129.088323098358)) ;
#124209=CARTESIAN_POINT('Ctrl Pts',(-28.4982051798402,12.7021784508198,
129.293379489094)) ;
#124210=CARTESIAN_POINT('Ctrl Pts',(-28.5610042308682,12.9449354906641,
129.443606404056)) ;
#124211=CARTESIAN_POINT('Ctrl Pts',(-28.6008426985914,13.2214385193801,
129.526846062899)) ;
#124212=CARTESIAN_POINT('Ctrl Pts',(-28.6159465633725,13.5108149265418,
129.538005633189)) ;
#124213=CARTESIAN_POINT('Ctrl Pts',(-28.6058800353516,13.7968085806489,
129.475293641202)) ;
#124214=CARTESIAN_POINT('Ctrl Pts',(-28.5721530465612,14.0536577586376,
129.343741854781)) ;
#124215=CARTESIAN_POINT('Ctrl Pts',(-28.5180253984698,14.2659121796834,
129.152568163917)) ;
#124216=CARTESIAN_POINT('Ctrl Pts',(-28.4476164033553,14.4185013343906,
128.913682850671)) ;
#124217=CARTESIAN_POINT('Ctrl Pts',(-28.3672606870272,14.4992712533562,
128.645857764565)) ;
#124218=CARTESIAN_POINT('Ctrl Pts',(-28.2830619034491,14.5031359858994,
128.366746278371)) ;
#124219=CARTESIAN_POINT('Ctrl Pts',(-28.2020479697154,14.42962012524,128.096991292358)) ;
#124220=CARTESIAN_POINT('Ctrl Pts',(-28.1306108659269,14.2844129921914,
127.855234639704)) ;
#124221=CARTESIAN_POINT('Ctrl Pts',(-28.0743399793536,14.07647539704,127.657620218949)) ;
#124222=CARTESIAN_POINT('Ctrl Pts',(-28.038518814024,13.8227945386488,127.519914708429)) ;
#124223=CARTESIAN_POINT('Ctrl Pts',(-28.0260544093946,13.5398700971536,
127.450350848859)) ;
#124224=CARTESIAN_POINT('Ctrl Pts',(-28.0387376470672,13.2487715870731,
127.454277173227)) ;
#124225=CARTESIAN_POINT('Ctrl Pts',(-28.0762887916964,12.9703360488667,
127.530869359068)) ;
#124226=CARTESIAN_POINT('Ctrl Pts',(-28.1368163621099,12.724109148074,127.674556172722)) ;
#124227=CARTESIAN_POINT('Ctrl Pts',(-28.2167305097807,12.5279170556122,
127.874864580102)) ;
#124228=CARTESIAN_POINT('Ctrl Pts',(-28.3109689538554,12.3959938215062,
128.117030677241)) ;
#124229=CARTESIAN_POINT('Ctrl Pts',(-28.4134273221919,12.3376260911869,
128.383241476252)) ;
#124230=CARTESIAN_POINT('Ctrl Pts',(-28.5177715853634,12.3570498023057,
128.65490265925)) ;
#124231=CARTESIAN_POINT('Ctrl Pts',(-28.616753088127,12.4525560159372,128.911007152944)) ;
#124232=CARTESIAN_POINT('Ctrl Pts',(-28.7045988631486,12.6176036615847,
129.134503535126)) ;
#124233=CARTESIAN_POINT('Ctrl Pts',(-28.7756048272567,12.841094749517,129.308722571836)) ;
#124234=CARTESIAN_POINT('Ctrl Pts',(-28.8250390574099,13.1055203905307,
129.420039183832)) ;
#124235=CARTESIAN_POINT('Ctrl Pts',(-28.8504133952678,13.3928980582864,
129.461039192628)) ;
#124236=CARTESIAN_POINT('Ctrl Pts',(-28.8505343656059,13.682454377304,129.428266482564)) ;
#124237=CARTESIAN_POINT('Ctrl Pts',(-28.826180486495,13.953269278216,129.324020975927)) ;
#124238=CARTESIAN_POINT('Ctrl Pts',(-28.779745106423,14.1862511207232,129.155240175136)) ;
#124239=CARTESIAN_POINT('Ctrl Pts',(-28.7155326099511,14.3643962047435,
128.934612491699)) ;
#124240=CARTESIAN_POINT('Ctrl Pts',(-28.6379231259812,14.4759024798905,
128.674537064384)) ;
#124241=CARTESIAN_POINT('Ctrl Pts',(-28.5549498566636,14.5109062470025,
128.399225139776)) ;
#124242=CARTESIAN_POINT('Ctrl Pts',(-28.4717526539607,14.4687351613561,
128.123044427645)) ;
#124243=CARTESIAN_POINT('Ctrl Pts',(-28.395557559578,14.3512437869113,127.867313690745)) ;
#124244=CARTESIAN_POINT('Ctrl Pts',(-28.3326545693278,14.1681343320696,
127.650520958287)) ;
#124245=CARTESIAN_POINT('Ctrl Pts',(-28.2877790237795,13.9291093087556,
127.486048344275)) ;
#124246=CARTESIAN_POINT('Ctrl Pts',(-28.265717377919,13.6572014758575,127.388679901215)) ;
#124247=CARTESIAN_POINT('Ctrl Pts',(-28.2681157526834,13.3659145810937,
127.362431930975)) ;
#124248=CARTESIAN_POINT('Ctrl Pts',(-28.2956553555426,13.0809590498869,
127.40989746564)) ;
#124249=CARTESIAN_POINT('Ctrl Pts',(-28.3471963188551,12.8188858312814,
127.527295565738)) ;
#124250=CARTESIAN_POINT('Ctrl Pts',(-28.4200761323168,12.5999509531083,
127.706953707642)) ;
#124251=CARTESIAN_POINT('Ctrl Pts',(-28.5086819650502,12.441498416931,127.932849511783)) ;
#124252=CARTESIAN_POINT('Ctrl Pts',(-28.6086670984304,12.3520342804443,
128.191780765644)) ;
#124253=CARTESIAN_POINT('Ctrl Pts',(-28.7133402836128,12.339805477818,128.464339419248)) ;
#124254=CARTESIAN_POINT('Ctrl Pts',(-28.8150120925492,12.404786593097,128.72835260752)) ;
#124255=CARTESIAN_POINT('Ctrl Pts',(-28.9084344751011,12.543193504082,128.968052605152)) ;
#124256=CARTESIAN_POINT('Ctrl Pts',(-28.9867401792367,12.7444967223723,
129.163680460267)) ;
#124257=CARTESIAN_POINT('Ctrl Pts',(-29.0453267744929,12.9945027181083,
129.301684319518)) ;
#124258=CARTESIAN_POINT('Ctrl Pts',(-29.0806918598349,13.2745331235142,
129.371935091382)) ;
#124259=CARTESIAN_POINT('Ctrl Pts',(-29.0910577293678,13.5670628518901,
129.368934829634)) ;
#124260=CARTESIAN_POINT('Ctrl Pts',(-29.076494701345,13.8462372757585,129.293480346358)) ;
#124261=CARTESIAN_POINT('Ctrl Pts',(-29.0385132292895,14.0979242906841,
129.14926585312)) ;
#124262=CARTESIAN_POINT('Ctrl Pts',(-28.9808663325831,14.299738463193,128.947793088852)) ;
#124263=CARTESIAN_POINT('Ctrl Pts',(-28.9083068168729,14.4393312892027,
128.702723448988)) ;
#124264=CARTESIAN_POINT('Ctrl Pts',(-28.8262915558581,14.5060643737482,
128.429867504545)) ;
#124265=CARTESIAN_POINT('Ctrl Pts',(-28.7426422363419,14.4951758470579,
128.152560658863)) ;
#124266=CARTESIAN_POINT('Ctrl Pts',(-28.6625995451793,14.4072622582047,
127.885495825799)) ;
#124267=CARTESIAN_POINT('Ctrl Pts',(-28.5937320513035,14.2495038720977,
127.651282692144)) ;
#124268=CARTESIAN_POINT('Ctrl Pts',(-28.5409096402226,14.0308220187667,
127.463666032205)) ;
#124269=CARTESIAN_POINT('Ctrl Pts',(-28.5094830415525,13.7719099555025,
127.339007189851)) ;
#124270=CARTESIAN_POINT('Ctrl Pts',(-28.5016223810496,13.4847455489294,
127.282758603318)) ;
#124271=CARTESIAN_POINT('Ctrl Pts',(-28.5189628663482,13.1955424238471,
127.300427535986)) ;
#124272=CARTESIAN_POINT('Ctrl Pts',(-28.5612901890702,12.9200552439899,
127.390764466653)) ;
#124273=CARTESIAN_POINT('Ctrl Pts',(-28.6255879815174,12.6831184051196,
127.545604609315)) ;
#124274=CARTESIAN_POINT('Ctrl Pts',(-28.7085274648009,12.4980281051702,
127.754767655982)) ;
#124275=CARTESIAN_POINT('Ctrl Pts',(-28.8048707795907,12.3791543391629,
128.003062725603)) ;
#124276=CARTESIAN_POINT('Ctrl Pts',(-28.9084505011422,12.3353503724763,
128.272456641543)) ;
#124277=CARTESIAN_POINT('Ctrl Pts',(-29.0119290399947,12.3691099624238,
128.541734986675)) ;
#124278=CARTESIAN_POINT('Ctrl Pts',(-29.1100844988828,12.4795856754925,
128.795121393085)) ;
#124279=CARTESIAN_POINT('Ctrl Pts',(-29.1943370244015,12.655336096254,129.008407922735)) ;
#124280=CARTESIAN_POINT('Ctrl Pts',(-29.2617806972532,12.8882259195335,
129.172162118277)) ;
#124281=CARTESIAN_POINT('Ctrl Pts',(-29.3067986316922,13.1581921439883,
129.27061431898)) ;
#124282=CARTESIAN_POINT('Ctrl Pts',(-29.3274947127435,13.4482190553547,
129.297870820219)) ;
#124283=CARTESIAN_POINT('Ctrl Pts',(-29.3228861406397,13.7352663481711,
129.251351301865)) ;
#124284=CARTESIAN_POINT('Ctrl Pts',(-29.2941391682194,14.0004787801146,
129.134251206445)) ;
#124285=CARTESIAN_POINT('Ctrl Pts',(-29.2440911045041,14.224240187898,128.954965629854)) ;
#124286=CARTESIAN_POINT('Ctrl Pts',(-29.1764772767869,14.391486040761,128.724142908791)) ;
#124287=CARTESIAN_POINT('Ctrl Pts',(-29.0980269041192,14.4880342043903,
128.4619863877)) ;
#124288=CARTESIAN_POINT('Ctrl Pts',(-29.0139943422698,14.508976716731,128.183329278251)) ;
#124289=CARTESIAN_POINT('Ctrl Pts',(-28.9317871778469,14.4520806960152,
127.910110797654)) ;
#124290=CARTESIAN_POINT('Ctrl Pts',(-28.8575866214198,14.3213934161067,
127.660199327887)) ;
#124291=CARTESIAN_POINT('Ctrl Pts',(-28.7977078233166,14.1264275067293,
127.452160129362)) ;
#124292=CARTESIAN_POINT('Ctrl Pts',(-28.7570216525618,13.8807879238241,
127.300143854661)) ;
#124293=CARTESIAN_POINT('Ctrl Pts',(-28.7393381079918,13.6022564662603,
127.215325042563)) ;
#124294=CARTESIAN_POINT('Ctrl Pts',(-28.7464673511228,13.3123737627951,
127.203159550126)) ;
#124295=CARTESIAN_POINT('Ctrl Pts',(-28.7787003276841,13.0290002093282,
127.264164185569)) ;
#124296=CARTESIAN_POINT('Ctrl Pts',(-28.8344853392707,12.7741269018416,
127.394000134619)) ;
#124297=CARTESIAN_POINT('Ctrl Pts',(-28.9105332614011,12.5657350925596,
127.583024031671)) ;
#124298=CARTESIAN_POINT('Ctrl Pts',(-29.0020340800631,12.4188761283997,
127.817221451334)) ;
#124299=CARTESIAN_POINT('Ctrl Pts',(-29.1033490521045,12.3438128182006,
128.08005015539)) ;
#124300=CARTESIAN_POINT('Ctrl Pts',(-29.2077611012054,12.346102551177,128.351954688411)) ;
#124301=CARTESIAN_POINT('Ctrl Pts',(-29.3086983900599,12.4255736713201,
128.613675945362)) ;
#124302=CARTESIAN_POINT('Ctrl Pts',(-29.3995090119233,12.5765458005785,
128.845828673796)) ;
#124303=CARTESIAN_POINT('Ctrl Pts',(-29.4743911046107,12.7879288159169,
129.031482386916)) ;
#124304=CARTESIAN_POINT('Ctrl Pts',(-29.528866555057,13.0448055751977,129.157510490086)) ;
#124305=CARTESIAN_POINT('Ctrl Pts',(-29.5597228216667,13.3297564879043,
129.214430894783)) ;
#124306=CARTESIAN_POINT('Ctrl Pts',(-29.5653119671571,13.6201108686768,
129.197692480837)) ;
#124307=CARTESIAN_POINT('Ctrl Pts',(-29.5461454694217,13.8967555620889,
129.108587621245)) ;
#124308=CARTESIAN_POINT('Ctrl Pts',(-29.5043003614803,14.1394984275279,
128.953246429327)) ;
#124309=CARTESIAN_POINT('Ctrl Pts',(-29.4431774798725,14.3315002121409,
128.741455873336)) ;
#124310=CARTESIAN_POINT('Ctrl Pts',(-29.368615149488,14.4575223198637,128.490628214048)) ;
#124311=CARTESIAN_POINT('Ctrl Pts',(-29.2856254843638,14.5099977953481,
128.214919388015)) ;
#124312=CARTESIAN_POINT('Ctrl Pts',(-29.2021625668279,14.4843800737971,
127.938111696582)) ;
#124313=CARTESIAN_POINT('Ctrl Pts',(-29.1238742274253,14.3828781274989,
127.676265154723)) ;
#124314=CARTESIAN_POINT('Ctrl Pts',(-29.0575885175731,14.2128161512202,
127.449543125235)) ;
#124315=CARTESIAN_POINT('Ctrl Pts',(-29.0084776120694,13.9854781588929,
127.272874876826)) ;
#124316=CARTESIAN_POINT('Ctrl Pts',(-28.9811292783656,13.7179644901035,
127.159826468009)) ;
#124317=CARTESIAN_POINT('Ctrl Pts',(-28.9781179163729,13.4301920421151,
127.117966111952)) ;
#124318=CARTESIAN_POINT('Ctrl Pts',(-29.0001132553344,13.1421055702502,
127.149189708795)) ;
#124319=CARTESIAN_POINT('Ctrl Pts',(-29.047053104884,12.871501287512,127.252936726976)) ;
#124320=CARTESIAN_POINT('Ctrl Pts',(-29.1151027479743,12.6436097972574,
127.418773188666)) ;
#124321=CARTESIAN_POINT('Ctrl Pts',(-29.2011947687253,12.469849836909,127.637073459389)) ;
#124322=CARTESIAN_POINT('Ctrl Pts',(-29.2991274824965,12.3651221790713,
127.890102388539)) ;
#124323=CARTESIAN_POINT('Ctrl Pts',(-29.4030193284557,12.3356922244687,
128.160499003177)) ;
#124324=CARTESIAN_POINT('Ctrl Pts',(-29.5063698934818,12.3844432220599,
128.429219190107)) ;
#124325=CARTESIAN_POINT('Ctrl Pts',(-29.6017701668784,12.5072148267233,
128.674860804049)) ;
#124326=CARTESIAN_POINT('Ctrl Pts',(-29.6838564893298,12.695755079112,128.881517005376)) ;
#124327=CARTESIAN_POINT('Ctrl Pts',(-29.7472379158472,12.9373000432248,
129.033441592439)) ;
#124328=CARTESIAN_POINT('Ctrl Pts',(-29.7877524940672,13.2121500744088,
129.118761133929)) ;
#124329=CARTESIAN_POINT('Ctrl Pts',(-29.8036385546026,13.503246650252,129.131988911234)) ;
#124330=CARTESIAN_POINT('Ctrl Pts',(-29.7944161810133,13.7871081777778,
129.072056104051)) ;
#124331=CARTESIAN_POINT('Ctrl Pts',(-29.7612451453642,14.04691061429,128.941902135837)) ;
#124332=CARTESIAN_POINT('Ctrl Pts',(-29.7076298212576,14.260565028937,128.752241000725)) ;
#124333=CARTESIAN_POINT('Ctrl Pts',(-29.6374049797901,14.4153650292754,
128.513802744357)) ;
#124334=CARTESIAN_POINT('Ctrl Pts',(-29.5575729299202,14.4978583100618,
128.247645906219)) ;
#124335=CARTESIAN_POINT('Ctrl Pts',(-29.4733841555509,14.5041773759635,
127.968557400909)) ;
#124336=CARTESIAN_POINT('Ctrl Pts',(-29.3921490619895,14.4329778405108,
127.698149651333)) ;
#124337=CARTESIAN_POINT('Ctrl Pts',(-29.3200604919066,14.2890421003468,
127.454349974841)) ;
#124338=CARTESIAN_POINT('Ctrl Pts',(-29.2634311723797,14.0827792612075,
127.255738950957)) ;
#124339=CARTESIAN_POINT('Ctrl Pts',(-29.2270568377556,13.830933510425,127.116507499098)) ;
#124340=CARTESIAN_POINT('Ctrl Pts',(-29.2138529064416,13.5483118095736,
127.044750757746)) ;
#124341=CARTESIAN_POINT('Ctrl Pts',(-29.2257641491017,13.2574775512287,
127.046461089286)) ;
#124342=CARTESIAN_POINT('Ctrl Pts',(-29.2626784751596,12.9779695749568,
127.121137886348)) ;
#124343=CARTESIAN_POINT('Ctrl Pts',(-29.3223683269202,12.7311578821155,
127.262476188241)) ;
#124344=CARTESIAN_POINT('Ctrl Pts',(-29.4021493735836,12.5323979618,127.46224042951)) ;
#124345=CARTESIAN_POINT('Ctrl Pts',(-29.4957297661686,12.3989896763175,
127.702606498418)) ;
#124346=CARTESIAN_POINT('Ctrl Pts',(-29.5982391003597,12.3382487508946,
127.96889464722)) ;
#124347=CARTESIAN_POINT('Ctrl Pts',(-29.7022741235999,12.3552058345121,
128.239769962473)) ;
#124348=CARTESIAN_POINT('Ctrl Pts',(-29.8021494393376,12.449068120654,128.498271362135)) ;
#124349=CARTESIAN_POINT('Ctrl Pts',(-29.890357842438,12.6128543666523,128.722805283861)) ;
#124350=CARTESIAN_POINT('Ctrl Pts',(-29.9614573415197,12.8333918946772,
128.897516477767)) ;
#124351=CARTESIAN_POINT('Ctrl Pts',(-30.0117536796374,13.0975419716129,
129.01125406221)) ;
#124352=CARTESIAN_POINT('Ctrl Pts',(-30.0378168368427,13.38437019925,129.054290739338)) ;
#124353=CARTESIAN_POINT('Ctrl Pts',(-30.0386639542191,13.6749248877936,
129.023552155716)) ;
#124354=CARTESIAN_POINT('Ctrl Pts',(-30.0148871543085,13.9463602698171,
128.920997210423)) ;
#124355=CARTESIAN_POINT('Ctrl Pts',(-29.969281069923,14.179832441143,128.754782276744)) ;
#124356=CARTESIAN_POINT('Ctrl Pts',(-29.9051021306394,14.3606302747574,
128.534050459932)) ;
#124357=CARTESIAN_POINT('Ctrl Pts',(-29.8284637932964,14.4733618846649,
128.277111973948)) ;
#124358=CARTESIAN_POINT('Ctrl Pts',(-29.744806599407,14.5110756603655,127.999483924866)) ;
#124359=CARTESIAN_POINT('Ctrl Pts',(-29.6619786972772,14.4709889018576,
127.724569420284)) ;
#124360=CARTESIAN_POINT('Ctrl Pts',(-29.5853193662016,14.3556941953622,
127.467426228982)) ;
#124361=CARTESIAN_POINT('Ctrl Pts',(-29.5217947117476,14.1731666349653,
127.24867559156)) ;
#124362=CARTESIAN_POINT('Ctrl Pts',(-29.4767596890819,13.9378583888153,
127.084070689769)) ;
#124363=CARTESIAN_POINT('Ctrl Pts',(-29.4537789685261,13.665635486159,126.983860518829)) ;
#124364=CARTESIAN_POINT('Ctrl Pts',(-29.4554655103503,13.3744562424158,
126.955530110006)) ;
#124365=CARTESIAN_POINT('Ctrl Pts',(-29.482352001784,13.0885611024712,127.001023851845)) ;
#124366=CARTESIAN_POINT('Ctrl Pts',(-29.5331352905586,12.8263305673749,
127.116301798459)) ;
#124367=CARTESIAN_POINT('Ctrl Pts',(-29.6050937436806,12.6063806997543,
127.293387240896)) ;
#124368=CARTESIAN_POINT('Ctrl Pts',(-29.6939157301013,12.4447492337382,
127.519673899328)) ;
#124369=CARTESIAN_POINT('Ctrl Pts',(-29.793684780295,12.353502559508,127.777985701848)) ;
#124370=CARTESIAN_POINT('Ctrl Pts',(-29.8981426431129,12.3391045182876,
128.049969682744)) ;
#124371=CARTESIAN_POINT('Ctrl Pts',(-29.999995923788,12.4018104838522,128.314511218612)) ;
#124372=CARTESIAN_POINT('Ctrl Pts',(-30.0940583651971,12.5389587593729,
128.555960228962)) ;
#124373=CARTESIAN_POINT('Ctrl Pts',(-30.1724238258053,12.7377765995817,
128.751929330358)) ;
#124374=CARTESIAN_POINT('Ctrl Pts',(-30.231666115958,12.9863021610025,128.891870713091)) ;
#124375=CARTESIAN_POINT('Ctrl Pts',(-30.2677813975979,13.26603407284,128.9642745019)) ;
#124376=CARTESIAN_POINT('Ctrl Pts',(-30.278920299464,13.5582234410802,128.963573253356)) ;
#124377=CARTESIAN_POINT('Ctrl Pts',(-30.26499159685,13.8387406073518,128.889873934224)) ;
#124378=CARTESIAN_POINT('Ctrl Pts',(-30.2278772365566,14.0904926888755,
128.748354891165)) ;
#124379=CARTESIAN_POINT('Ctrl Pts',(-30.1702932972715,14.2955137272415,
128.546803394523)) ;
#124380=CARTESIAN_POINT('Ctrl Pts',(-30.0984120784379,14.4360007562524,
128.303894575953)) ;
#124381=CARTESIAN_POINT('Ctrl Pts',(-30.0167909849871,14.5051703131075,
128.032264264772)) ;
#124382=CARTESIAN_POINT('Ctrl Pts',(-29.9328311834785,14.4966323444729,
127.753939337243)) ;
#124383=CARTESIAN_POINT('Ctrl Pts',(-29.8525465680788,14.4108290646986,
127.48616105779)) ;
#124384=CARTESIAN_POINT('Ctrl Pts',(-29.7832722853812,14.2547208432748,
127.250733345617)) ;
#124385=CARTESIAN_POINT('Ctrl Pts',(-29.7301231215459,14.0388604849956,
127.062340185207)) ;
#124386=CARTESIAN_POINT('Ctrl Pts',(-29.6977837486614,13.7794054501878,
126.934803763672)) ;
#124387=CARTESIAN_POINT('Ctrl Pts',(-29.6893035192315,13.4926640432345,
126.876755208931)) ;
#124388=CARTESIAN_POINT('Ctrl Pts',(-29.7059159424158,13.2038301120676,
126.892352602474)) ;
#124389=CARTESIAN_POINT('Ctrl Pts',(-29.7474057347377,12.9280759212708,
126.980311855023)) ;
#124390=CARTESIAN_POINT('Ctrl Pts',(-29.8113849358203,12.6887447030163,
127.134072403226)) ;
#124391=CARTESIAN_POINT('Ctrl Pts',(-29.8938930194494,12.5022966098147,
127.341991684149)) ;
#124392=CARTESIAN_POINT('Ctrl Pts',(-29.9895145374687,12.3817639702232,
127.588316710086)) ;
#124393=CARTESIAN_POINT('Ctrl Pts',(-30.0933362893935,12.3354318122153,
127.858302940627)) ;
#124394=CARTESIAN_POINT('Ctrl Pts',(-30.1967145851462,12.3672035542546,
128.127339641179)) ;
#124395=CARTESIAN_POINT('Ctrl Pts',(-30.2946449394812,12.4744264817991,
128.380263197516)) ;
#124396=CARTESIAN_POINT('Ctrl Pts',(-30.3803208267645,12.6503068789,128.59733206961)) ;
#124397=CARTESIAN_POINT('Ctrl Pts',(-30.447925069988,12.88124813694,128.761691535732)) ;
#124398=CARTESIAN_POINT('Ctrl Pts',(-30.4935671315089,13.1494231043328,
128.862066641)) ;
#124399=CARTESIAN_POINT('Ctrl Pts',(-30.5150767542471,13.4405328336443,
128.891547059133)) ;
#124400=CARTESIAN_POINT('Ctrl Pts',(-30.5111288053941,13.7272524235385,
128.847033061191)) ;
#124401=CARTESIAN_POINT('Ctrl Pts',(-30.4830702446878,13.9933198018618,
128.731951447052)) ;
#124402=CARTESIAN_POINT('Ctrl Pts',(-30.4336230875361,14.2183989347204,
128.554443162596)) ;
#124403=CARTESIAN_POINT('Ctrl Pts',(-30.3663826934686,14.3876287809154,
128.32468557259)) ;
#124404=CARTESIAN_POINT('Ctrl Pts',(-30.2882857864212,14.4861871139801,
128.063606645417)) ;
#124405=CARTESIAN_POINT('Ctrl Pts',(-30.2042479014223,14.5095212263095,
127.784908710589)) ;
#124406=CARTESIAN_POINT('Ctrl Pts',(-30.121812915052,14.4547286941079,127.510988806245)) ;
#124407=CARTESIAN_POINT('Ctrl Pts',(-30.047335214886,14.3261104850367,127.260287876867)) ;
#124408=CARTESIAN_POINT('Ctrl Pts',(-29.9869536457719,14.1327423956962,
127.05076735835)) ;
#124409=CARTESIAN_POINT('Ctrl Pts',(-29.9456867841733,13.8885304573601,
126.897084193712)) ;
#124410=CARTESIAN_POINT('Ctrl Pts',(-29.9273110105387,13.6107522710193,
126.810248321643)) ;
#124411=CARTESIAN_POINT('Ctrl Pts',(-29.933619766616,13.3210540758006,126.795703495367)) ;
#124412=CARTESIAN_POINT('Ctrl Pts',(-29.9655096904855,13.0351249391052,
126.855452075723)) ;
#124413=CARTESIAN_POINT('Ctrl Pts',(-30.0202087483359,12.7816148571452,
126.982424137597)) ;
#124414=CARTESIAN_POINT('Ctrl Pts',(-30.0959655060956,12.5706516748794,
127.170461842928)) ;
#124415=CARTESIAN_POINT('Ctrl Pts',(-30.187075628918,12.4220918167394,127.403541558847)) ;
#124416=CARTESIAN_POINT('Ctrl Pts',(-30.2883231009899,12.3448083545055,
127.666131810962)) ;
#124417=CARTESIAN_POINT('Ctrl Pts',(-30.3926830064791,12.3450375900235,
127.93790207961)) ;
#124418=CARTESIAN_POINT('Ctrl Pts',(-30.4936514271429,12.4222141215766,
128.199767789345)) ;
#124419=CARTESIAN_POINT('Ctrl Pts',(-30.5848893407942,12.5713074000372,
128.433150896225)) ;
#124420=CARTESIAN_POINT('Ctrl Pts',(-30.6603311521981,12.7812070105723,
128.620428718384)) ;
#124421=CARTESIAN_POINT('Ctrl Pts',(-30.7155665117066,13.0378488607775,
128.748579693311)) ;
#124422=CARTESIAN_POINT('Ctrl Pts',(-30.7469885961688,13.3220974223082,
128.807185014511)) ;
#124423=CARTESIAN_POINT('Ctrl Pts',(-30.7532932333332,13.611647883706,128.792639705149)) ;
#124424=CARTESIAN_POINT('Ctrl Pts',(-30.7347671239028,13.8896345343945,
128.705325771604)) ;
#124425=CARTESIAN_POINT('Ctrl Pts',(-30.693600390576,14.1329049356831,128.552051589304)) ;
#124426=CARTESIAN_POINT('Ctrl Pts',(-30.633070371467,14.3266158098986,128.342023513571)) ;
#124427=CARTESIAN_POINT('Ctrl Pts',(-30.5585711021984,14.4550272244897,
128.091269880465)) ;
#124428=CARTESIAN_POINT('Ctrl Pts',(-30.4759843115532,14.5094869188899,
127.816847983147)) ;
#124429=CARTESIAN_POINT('Ctrl Pts',(-30.3924156986506,14.4863254941317,
127.539715217734)) ;
#124430=CARTESIAN_POINT('Ctrl Pts',(-30.3137804479421,14.3868080621077,
127.276813774952)) ;
#124431=CARTESIAN_POINT('Ctrl Pts',(-30.2470276101846,14.2186053489218,
127.04872115819)) ;
#124432=CARTESIAN_POINT('Ctrl Pts',(-30.1972622816575,13.9916146636668,
126.870012022956)) ;
#124433=CARTESIAN_POINT('Ctrl Pts',(-30.1694297843685,13.7271394613145,
126.755815447488)) ;
#124434=CARTESIAN_POINT('Ctrl Pts',(-30.1656502016795,13.4373621630931,
126.711435528483)) ;
#124435=CARTESIAN_POINT('Ctrl Pts',(-30.1869265241885,13.1504054567353,
126.740721815544)) ;
#124436=CARTESIAN_POINT('Ctrl Pts',(-30.2331958971664,12.8786465082132,
126.842474926041)) ;
#124437=CARTESIAN_POINT('Ctrl Pts',(-30.3005045160255,12.6500332847712,
127.006235986259)) ;
#124438=CARTESIAN_POINT('Ctrl Pts',(-30.3859680592901,12.4743183889617,
127.222741912272)) ;
#124439=CARTESIAN_POINT('Ctrl Pts',(-30.484292867573,12.3668547885935,127.476696341652)) ;
#124440=CARTESIAN_POINT('Ctrl Pts',(-30.587616388384,12.3355629410877,127.745593654544)) ;
#124441=CARTESIAN_POINT('Ctrl Pts',(-30.6910287858327,12.3817108160481,
128.014514918498)) ;
#124442=CARTESIAN_POINT('Ctrl Pts',(-30.7871323371635,12.5028398511796,
128.262083898072)) ;
#124443=CARTESIAN_POINT('Ctrl Pts',(-30.8697321583824,12.6903514923922,
128.470177876443)) ;
#124444=CARTESIAN_POINT('Ctrl Pts',(-30.9332422444198,12.9285060131068,
128.622757398001)) ;
#124445=CARTESIAN_POINT('Ctrl Pts',(-30.9748295562401,13.2046732930674,
128.710950155907)) ;
#124446=CARTESIAN_POINT('Ctrl Pts',(-30.9913101196902,13.4951334329262,
128.725980834387)) ;
#124447=CARTESIAN_POINT('Ctrl Pts',(-30.9827689117977,13.7795013395347,
128.668022330097)) ;
#124448=CARTESIAN_POINT('Ctrl Pts',(-30.9503979576926,14.0394109591315,
128.540333225843)) ;
#124449=CARTESIAN_POINT('Ctrl Pts',(-30.8971895152289,14.2552142278511,
128.351765160571)) ;
#124450=CARTESIAN_POINT('Ctrl Pts',(-30.827703837052,14.4112842986504,128.115645384182)) ;
#124451=CARTESIAN_POINT('Ctrl Pts',(-30.7478762186822,14.4966304081093,
127.849398626646)) ;
#124452=CARTESIAN_POINT('Ctrl Pts',(-30.6632860167029,14.5049768575903,
127.568975433367)) ;
#124453=CARTESIAN_POINT('Ctrl Pts',(-30.5822812878458,14.4360834976797,
127.299398037642)) ;
#124454=CARTESIAN_POINT('Ctrl Pts',(-30.5099274709679,14.2946512650185,
127.054884795324)) ;
#124455=CARTESIAN_POINT('Ctrl Pts',(-30.4526678489903,14.0899138392311,
126.854394854671)) ;
#124456=CARTESIAN_POINT('Ctrl Pts',(-30.4155401891835,13.8386915040984,
126.712892259472)) ;
#124457=CARTESIAN_POINT('Ctrl Pts',(-30.4016797337328,13.5555689993548,
126.639099979704)) ;
#124458=CARTESIAN_POINT('Ctrl Pts',(-30.4128387173659,13.2663899085958,
126.638804628752)) ;
#124459=CARTESIAN_POINT('Ctrl Pts',(-30.4489906096477,12.9858845454111,
126.711220297671)) ;
#124460=CARTESIAN_POINT('Ctrl Pts',(-30.5082151997129,12.737510093137,126.851136088065)) ;
#124461=CARTESIAN_POINT('Ctrl Pts',(-30.5871935739308,12.5376375211986,
127.048669841167)) ;
#124462=CARTESIAN_POINT('Ctrl Pts',(-30.6809240837796,12.4015826391132,
127.289300668043)) ;
#124463=CARTESIAN_POINT('Ctrl Pts',(-30.7827898108076,12.3390360778661,
127.553872708322)) ;
#124464=CARTESIAN_POINT('Ctrl Pts',(-30.8870946705224,12.3535754317009,
127.825461319271)) ;
#124465=CARTESIAN_POINT('Ctrl Pts',(-30.9870766402844,12.4452741320202,
128.084312934138)) ;
#124466=CARTESIAN_POINT('Ctrl Pts',(-31.0756876477193,12.6067972439988,
128.310049838523)) ;
#124467=CARTESIAN_POINT('Ctrl Pts',(-31.1477578491021,12.8274893323333,
128.487374513247)) ;
#124468=CARTESIAN_POINT('Ctrl Pts',(-31.1983271909888,13.0891409681253,
128.602118684947)) ;
#124469=CARTESIAN_POINT('Ctrl Pts',(-31.2251992522325,13.3757401842095,
128.647491129551)) ;
#124470=CARTESIAN_POINT('Ctrl Pts',(-31.2267800238666,13.6659116467556,
128.618963093478)) ;
#124471=CARTESIAN_POINT('Ctrl Pts',(-31.2038312103077,13.9383430933064,
128.518829961431)) ;
#124472=CARTESIAN_POINT('Ctrl Pts',(-31.1583764244852,14.1747318891546,
128.352797912173)) ;
#124473=CARTESIAN_POINT('Ctrl Pts',(-31.0952754500218,14.3556000253484,
128.135542669314)) ;
#124474=CARTESIAN_POINT('Ctrl Pts',(-31.0182491364109,14.4715471838241,
127.877162829971)) ;
#124475=CARTESIAN_POINT('Ctrl Pts',(-30.9352331910558,14.5109306883494,
127.601637155271)) ;
#124476=CARTESIAN_POINT('Ctrl Pts',(-30.8521513235924,14.4734197529204,
127.325920803467)) ;
#124477=CARTESIAN_POINT('Ctrl Pts',(-30.7749550777624,14.3595613324345,
127.067091655152)) ;
#124478=CARTESIAN_POINT('Ctrl Pts',(-30.7112774432419,14.1794661673076,
126.848033266043)) ;
#124479=CARTESIAN_POINT('Ctrl Pts',(-30.6655292058414,13.945518104717,126.681323661303)) ;
#124480=CARTESIAN_POINT('Ctrl Pts',(-30.6418404807834,13.6723045433651,
126.578842288596)) ;
#124481=CARTESIAN_POINT('Ctrl Pts',(-30.6428557130489,13.3834915419228,
126.548801546779)) ;
#124482=CARTESIAN_POINT('Ctrl Pts',(-30.6689836005855,13.096613347718,126.59201192854)) ;
#124483=CARTESIAN_POINT('Ctrl Pts',(-30.7192056164411,12.8330520382444,
126.705604956252)) ;
#124484=CARTESIAN_POINT('Ctrl Pts',(-30.790834532404,12.611232367513,126.881647244547)) ;
#124485=CARTESIAN_POINT('Ctrl Pts',(-30.8791960095022,12.4482428501487,
127.1066335396)) ;
#124486=CARTESIAN_POINT('Ctrl Pts',(-30.9782658750989,12.3553252132509,
127.363054948833)) ;
#124487=CARTESIAN_POINT('Ctrl Pts',(-31.0825679140159,12.3382107203878,
127.634621858498)) ;
#124488=CARTESIAN_POINT('Ctrl Pts',(-31.1851705795097,12.3992481995866,
127.901152590329)) ;
#124489=CARTESIAN_POINT('Ctrl Pts',(-31.2787737046393,12.533120575299,128.141551668428)) ;
#124490=CARTESIAN_POINT('Ctrl Pts',(-31.3581694597885,12.7309389352082,
128.340353310314)) ;
#124491=CARTESIAN_POINT('Ctrl Pts',(-31.4181700324155,12.9791526214122,
128.482412755056)) ;
#124492=CARTESIAN_POINT('Ctrl Pts',(-31.4549351457382,13.2585792633392,
128.556683953962)) ;
#124493=CARTESIAN_POINT('Ctrl Pts',(-31.4667178812962,13.5499400001449,
128.557952145081)) ;
#124494=CARTESIAN_POINT('Ctrl Pts',(-31.4535429896863,13.831171440361,128.486447666919)) ;
#124495=CARTESIAN_POINT('Ctrl Pts',(-31.4167705477339,14.0848087373092,
128.345787022824)) ;
#124496=CARTESIAN_POINT('Ctrl Pts',(-31.3604022147667,14.2892042753313,
128.148175854391)) ;
#124497=CARTESIAN_POINT('Ctrl Pts',(-31.2883262191337,14.4332159857665,
127.904406939294)) ;
#124498=CARTESIAN_POINT('Ctrl Pts',(-31.2070359185829,14.5042074008981,
127.63382430801)) ;
#124499=CARTESIAN_POINT('Ctrl Pts',(-31.1228911241346,14.4978850234615,
127.35488500635)) ;
#124500=CARTESIAN_POINT('Ctrl Pts',(-31.0426799297735,14.4145533230364,
127.087444540291)) ;
#124501=CARTESIAN_POINT('Ctrl Pts',(-30.9728258224195,14.2600829811303,
126.850238813674)) ;
#124502=CARTESIAN_POINT('Ctrl Pts',(-30.9192125542816,14.0459658246631,
126.660532770035)) ;
#124503=CARTESIAN_POINT('Ctrl Pts',(-30.8862030827133,13.7875806302573,
126.53103679406)) ;
#124504=CARTESIAN_POINT('Ctrl Pts',(-30.8769652131714,13.5015007624486,
126.470798628312)) ;
#124505=CARTESIAN_POINT('Ctrl Pts',(-30.8928913009424,13.2119710918027,
126.484325214026)) ;
#124506=CARTESIAN_POINT('Ctrl Pts',(-30.9335291322578,12.9363052863804,
126.569902948706)) ;
#124507=CARTESIAN_POINT('Ctrl Pts',(-30.9969656458465,12.6952735982691,
126.722023128662)) ;
#124508=CARTESIAN_POINT('Ctrl Pts',(-31.0787937782132,12.5071256429724,
126.928019042158)) ;
#124509=CARTESIAN_POINT('Ctrl Pts',(-31.1750192801707,12.383762838378,127.175802450844)) ;
#124510=CARTESIAN_POINT('Ctrl Pts',(-31.2776023117639,12.3357954087545,
127.442538372625)) ;
#124511=CARTESIAN_POINT('Ctrl Pts',(-31.3818855655355,12.3652711313032,
127.713950589831)) ;
#124512=CARTESIAN_POINT('Ctrl Pts',(-31.4797808939481,12.4705156862028,
127.966863975208)) ;
#124513=CARTESIAN_POINT('Ctrl Pts',(-31.5656441790736,12.6439184984734,
128.184578603)) ;
#124514=CARTESIAN_POINT('Ctrl Pts',(-31.6338998959943,12.8730354014428,
128.350870354409)) ;
#124515=CARTESIAN_POINT('Ctrl Pts',(-31.6804874469165,13.1424159380097,
128.453758787972)) ;
#124516=CARTESIAN_POINT('Ctrl Pts',(-31.7025235008913,13.4306391713404,
128.485081697739)) ;
#124517=CARTESIAN_POINT('Ctrl Pts',(-31.6994134419099,13.7191539467883,
128.442846383316)) ;
#124518=CARTESIAN_POINT('Ctrl Pts',(-31.6719894670492,13.9861294006722,
128.329622243672)) ;
#124519=CARTESIAN_POINT('Ctrl Pts',(-31.6230063053965,14.2128684177951,
128.153415320966)) ;
#124520=CARTESIAN_POINT('Ctrl Pts',(-31.5564974117218,14.3833348165239,
127.925939532501)) ;
#124521=CARTESIAN_POINT('Ctrl Pts',(-31.4782582440777,14.4845639234701,
127.664272210316)) ;
#124522=CARTESIAN_POINT('Ctrl Pts',(-31.3945103482704,14.5099092452808,
127.386518238402)) ;
#124523=CARTESIAN_POINT('Ctrl Pts',(-31.3118033167592,14.4573340950599,
127.111748041755)) ;
#124524=CARTESIAN_POINT('Ctrl Pts',(-31.2370170461689,14.3305257687139,
126.860139050925)) ;
#124525=CARTESIAN_POINT('Ctrl Pts',(-31.1763161492696,14.1393929887669,
126.649775812031)) ;
#124526=CARTESIAN_POINT('Ctrl Pts',(-31.1343568830856,13.8963011605845,
126.494040620924)) ;
#124527=CARTESIAN_POINT('Ctrl Pts',(-31.1152511809763,13.6185277978384,
126.404996071388)) ;
#124528=CARTESIAN_POINT('Ctrl Pts',(-31.1209459798989,13.3290636880528,
126.388670020425)) ;
#124529=CARTESIAN_POINT('Ctrl Pts',(-31.1517877758926,13.0445547365035,
126.44559285922)) ;
#124530=CARTESIAN_POINT('Ctrl Pts',(-31.2062319103761,12.7876682378207,
126.571537992278)) ;
#124531=CARTESIAN_POINT('Ctrl Pts',(-31.2816236951061,12.5753841966509,
126.758494307984)) ;
#124532=CARTESIAN_POINT('Ctrl Pts',(-31.3720200163798,12.4255193729721,
126.989613193023)) ;
#124533=CARTESIAN_POINT('Ctrl Pts',(-31.4730863859192,12.3459765323798,
127.251666609436)) ;
#124534=CARTESIAN_POINT('Ctrl Pts',(-31.5773109497355,12.3439073605975,
127.523083026688)) ;
#124535=CARTESIAN_POINT('Ctrl Pts',(-31.6786559521164,12.4188280799993,
127.785997053854)) ;
#124536=CARTESIAN_POINT('Ctrl Pts',(-31.7706041117922,12.5669348779127,
128.021308309052)) ;
#124537=CARTESIAN_POINT('Ctrl Pts',(-31.8460678201719,12.7740278443755,
128.208861704662)) ;
#124538=CARTESIAN_POINT('Ctrl Pts',(-31.9021441339329,13.0302841857639,
128.339365368756)) ;
#124539=CARTESIAN_POINT('Ctrl Pts',(-31.9341916798789,13.313391034623,128.39987822107)) ;
#124540=CARTESIAN_POINT('Ctrl Pts',(-31.9412308825654,13.603463825877,128.387421784324)) ;
#124541=CARTESIAN_POINT('Ctrl Pts',(-31.9235255942991,13.881303539034,128.302617667535)) ;
#124542=CARTESIAN_POINT('Ctrl Pts',(-31.8826193869947,14.1277804532013,
128.149829200477)) ;
#124543=CARTESIAN_POINT('Ctrl Pts',(-31.8226073128335,14.3222500271651,
127.941403939693)) ;
#124544=CARTESIAN_POINT('Ctrl Pts',(-31.7486997913269,14.4521801534422,
127.692492488672)) ;
#124545=CARTESIAN_POINT('Ctrl Pts',(-31.6663643399628,14.5090397064551,
127.418847768858)) ;
#124546=CARTESIAN_POINT('Ctrl Pts',(-31.5824009229194,14.4879536180509,
127.140421787047)) ;
#124547=CARTESIAN_POINT('Ctrl Pts',(-31.5036370266105,14.3907168838663,
126.877206024863)) ;
#124548=CARTESIAN_POINT('Ctrl Pts',(-31.436238274105,14.2230874548014,126.647049834908)) ;
#124549=CARTESIAN_POINT('Ctrl Pts',(-31.386526275312,14.0008520915057,126.468970265157)) ;
#124550=CARTESIAN_POINT('Ctrl Pts',(-31.3576250453209,13.7343152411408,
126.351250585093)) ;
#124551=CARTESIAN_POINT('Ctrl Pts',(-31.3531426090254,13.4474451384185,
126.305130028153)) ;
#124552=CARTESIAN_POINT('Ctrl Pts',(-31.3738726128369,13.1575373566889,
126.332496699286)) ;
#124553=CARTESIAN_POINT('Ctrl Pts',(-31.4189399340047,12.8878586213282,
126.431113174391)) ;
#124554=CARTESIAN_POINT('Ctrl Pts',(-31.486140272065,12.6555337208909,126.594256475355)) ;
#124555=CARTESIAN_POINT('Ctrl Pts',(-31.5711382567036,12.4784852889698,
126.809445172476)) ;
#124556=CARTESIAN_POINT('Ctrl Pts',(-31.6691499143102,12.3688435118071,
127.062490447939)) ;
#124557=CARTESIAN_POINT('Ctrl Pts',(-31.7726188430086,12.3353790498827,
127.331744180192)) ;
#124558=CARTESIAN_POINT('Ctrl Pts',(-31.8759336246217,12.3794309096132,
127.600441979446)) ;
#124559=CARTESIAN_POINT('Ctrl Pts',(-31.9720889415792,12.4979553163596,
127.848259175371)) ;
#124560=CARTESIAN_POINT('Ctrl Pts',(-32.0554688914873,12.6843641883006,
128.05850963336)) ;
#124561=CARTESIAN_POINT('Ctrl Pts',(-32.1194424670517,12.9208195747622,
128.212508863396)) ;
#124562=CARTESIAN_POINT('Ctrl Pts',(-32.161757747067,13.1965599985602,128.302784788776)) ;
#124563=CARTESIAN_POINT('Ctrl Pts',(-32.1789423174569,13.4854151022566,
128.320037673356)) ;
#124564=CARTESIAN_POINT('Ctrl Pts',(-32.1711933637879,13.7715246215189,
128.264248994403)) ;
#124565=CARTESIAN_POINT('Ctrl Pts',(-32.1393291975497,14.0329604460064,
128.137965297033)) ;
#124566=CARTESIAN_POINT('Ctrl Pts',(-32.0867940958276,14.2495175049027,
127.951460801025)) ;
#124567=CARTESIAN_POINT('Ctrl Pts',(-32.0177979789177,14.4077222066367,
127.716792376886)) ;
#124568=CARTESIAN_POINT('Ctrl Pts',(-31.9375247117624,14.4954975109272,
127.44898097478)) ;
#124569=CARTESIAN_POINT('Ctrl Pts',(-31.8537460867362,14.5058124049383,
127.171244726261)) ;
#124570=CARTESIAN_POINT('Ctrl Pts',(-31.772123804296,14.4390539454557,126.899685772576)) ;
#124571=CARTESIAN_POINT('Ctrl Pts',(-31.6993301037076,14.2988993787837,
126.653821842272)) ;
#124572=CARTESIAN_POINT('Ctrl Pts',(-31.6417494548733,14.0959845150152,
126.452461138729)) ;
#124573=CARTESIAN_POINT('Ctrl Pts',(-31.6041498202792,13.8467236092075,
126.309691385775)) ;
#124574=CARTESIAN_POINT('Ctrl Pts',(-31.5895140395483,13.5651497445093,
126.233737086702)) ;
#124575=CARTESIAN_POINT('Ctrl Pts',(-31.5999241287719,13.2745208567972,
126.231092292525)) ;
#124576=CARTESIAN_POINT('Ctrl Pts',(-31.6355120865293,12.9930479903862,
126.301811575219)) ;
#124577=CARTESIAN_POINT('Ctrl Pts',(-31.6939636509035,12.744268366307,126.439563836285)) ;
#124578=CARTESIAN_POINT('Ctrl Pts',(-31.7723241051701,12.5428868462353,
126.635326857753)) ;
#124579=CARTESIAN_POINT('Ctrl Pts',(-31.8656254635545,12.4047082626809,
126.874723079366)) ;
#124580=CARTESIAN_POINT('Ctrl Pts',(-31.9676540092607,12.3396945376806,
127.139665153436)) ;
#124581=CARTESIAN_POINT('Ctrl Pts',(-32.0719191102728,12.3521469878651,
127.411159614694)) ;
#124582=CARTESIAN_POINT('Ctrl Pts',(-32.1718927341903,12.4413144196275,
127.670070810723)) ;
#124583=CARTESIAN_POINT('Ctrl Pts',(-32.2610423474875,12.6011044167591,
127.8973332851)) ;
#124584=CARTESIAN_POINT('Ctrl Pts',(-32.3334806640345,12.8194225372239,
128.075845726197)) ;
#124585=CARTESIAN_POINT('Ctrl Pts',(-32.3850196376036,13.0811435285209,
128.193273866145)) ;
#124586=CARTESIAN_POINT('Ctrl Pts',(-32.4125817943959,13.3679218651448,
128.240601929342)) ;
#124587=CARTESIAN_POINT('Ctrl Pts',(-32.4148577451004,13.6574454628282,
128.214198686858)) ;
#124588=CARTESIAN_POINT('Ctrl Pts',(-32.3926720296224,13.9304219315962,
128.116328916553)) ;
#124589=CARTESIAN_POINT('Ctrl Pts',(-32.3477869876259,14.1686008809453,
127.951913381079)) ;
#124590=CARTESIAN_POINT('Ctrl Pts',(-32.284971158177,14.3514046906987,127.735422298426)) ;
#124591=CARTESIAN_POINT('Ctrl Pts',(-32.2087232804531,14.4688537021457,
127.479519830962)) ;
#124592=CARTESIAN_POINT('Ctrl Pts',(-32.1254819939557,14.5110084059665,
127.203197805899)) ;
#124593=CARTESIAN_POINT('Ctrl Pts',(-32.042186619966,14.4754271671864,126.926806872625)) ;
#124594=CARTESIAN_POINT('Ctrl Pts',(-31.9649675676906,14.3641624837098,
126.668028698741)) ;
#124595=CARTESIAN_POINT('Ctrl Pts',(-31.9005738315734,14.1852632714168,
126.446754200325)) ;
#124596=CARTESIAN_POINT('Ctrl Pts',(-31.8543504110818,13.9526451363771,
126.278680058295)) ;
#124597=CARTESIAN_POINT('Ctrl Pts',(-31.8300493968808,13.6818446977071,
126.174592372268)) ;
#124598=CARTESIAN_POINT('Ctrl Pts',(-31.8301771516343,13.3926206183681,
126.141881666587)) ;
#124599=CARTESIAN_POINT('Ctrl Pts',(-31.8557646547221,13.1038754492096,
126.183340661804)) ;
#124600=CARTESIAN_POINT('Ctrl Pts',(-31.9052187214914,12.840383579606,126.294805831761)) ;
#124601=CARTESIAN_POINT('Ctrl Pts',(-31.97602772857,12.6175434058043,126.468540816622)) ;
#124602=CARTESIAN_POINT('Ctrl Pts',(-32.0641273166764,12.452017834643,126.692686648714)) ;
#124603=CARTESIAN_POINT('Ctrl Pts',(-32.1634651082686,12.3567780373273,
126.949731371185)) ;
#124604=CARTESIAN_POINT('Ctrl Pts',(-32.2671759723703,12.3376561181457,
127.219747078339)) ;
#124605=CARTESIAN_POINT('Ctrl Pts',(-32.3700590194861,12.3963495269004,
127.487055840793)) ;
#124606=CARTESIAN_POINT('Ctrl Pts',(-32.4640016861435,12.5282530119487,
127.728446795974)) ;
#124607=CARTESIAN_POINT('Ctrl Pts',(-32.5438766891884,12.7243874356401,
127.928650447838)) ;
#124608=CARTESIAN_POINT('Ctrl Pts',(-32.6044439637128,12.9708925599776,
128.072424865895)) ;
#124609=CARTESIAN_POINT('Ctrl Pts',(-32.6419759471104,13.2502128136118,
128.148867357921)) ;
#124610=CARTESIAN_POINT('Ctrl Pts',(-32.6545321724612,13.5400585853171,
128.152566906686)) ;
#124611=CARTESIAN_POINT('Ctrl Pts',(-32.6420230728552,13.8239340251458,
128.082761152627)) ;
#124612=CARTESIAN_POINT('Ctrl Pts',(-32.6059615988536,14.0777678447128,
127.944294228757)) ;
#124613=CARTESIAN_POINT('Ctrl Pts',(-32.5500370870999,14.2841379825029,
127.74791925335)) ;
#124614=CARTESIAN_POINT('Ctrl Pts',(-32.4785189411542,14.4298157397374,
127.50586889978)) ;
#124615=CARTESIAN_POINT('Ctrl Pts',(-32.3971370747449,14.5033259419055,
127.234901175803)) ;
#124616=CARTESIAN_POINT('Ctrl Pts',(-32.3130267071577,14.499135083616,126.956085571107)) ;
#124617=CARTESIAN_POINT('Ctrl Pts',(-32.2325533904374,14.4177797503692,
126.687848133579)) ;
#124618=CARTESIAN_POINT('Ctrl Pts',(-32.1625451627168,14.2657375874764,
126.450301985178)) ;
#124619=CARTESIAN_POINT('Ctrl Pts',(-32.1082043097961,14.0527572687347,
126.258387004546)) ;
#124620=CARTESIAN_POINT('Ctrl Pts',(-32.0745277451477,13.7942042748117,
126.126810553039)) ;
#124621=CARTESIAN_POINT('Ctrl Pts',(-32.0646864224014,13.5099720674089,
126.064975641642)) ;
#124622=CARTESIAN_POINT('Ctrl Pts',(-32.0798874202907,13.2198346279653,
126.076326920652)) ;
#124623=CARTESIAN_POINT('Ctrl Pts',(-32.1199058770128,12.943315390008,126.160076953794)) ;
#124624=CARTESIAN_POINT('Ctrl Pts',(-32.1828974962533,12.7008041601945,
126.310848236002)) ;
#124625=CARTESIAN_POINT('Ctrl Pts',(-32.2639968728833,12.5118987867612,
126.514840222286)) ;
#124626=CARTESIAN_POINT('Ctrl Pts',(-32.3593853092676,12.3867144274878,
126.760340270936)) ;
#124627=CARTESIAN_POINT('Ctrl Pts',(-32.4624376893913,12.3359851179155,
127.028252288718)) ;
#124628=CARTESIAN_POINT('Ctrl Pts',(-32.5667565587772,12.3634203975105,
127.299779078233)) ;
#124629=CARTESIAN_POINT('Ctrl Pts',(-32.6648922781871,12.4663876776292,
127.553408260374)) ;
#124630=CARTESIAN_POINT('Ctrl Pts',(-32.7515226393346,12.638970046877,127.773214375674)) ;
#124631=CARTESIAN_POINT('Ctrl Pts',(-32.8199640950515,12.8657476347374,
127.940206666324)) ;
#124632=CARTESIAN_POINT('Ctrl Pts',(-32.8673394624009,13.1346340040003,
128.045343963703)) ;
#124633=CARTESIAN_POINT('Ctrl Pts',(-32.8824457910606,13.3266515427633,
128.067433585776)) ;
#124634=CARTESIAN_POINT('Ctrl Pts',(-32.8858452579044,13.4226803244344,
128.066343554261)) ;
#124635=CARTESIAN_POINT('Ctrl Pts',(-11.4002577710971,13.1368456608817,
133.107754941818)) ;
#124636=CARTESIAN_POINT('Ctrl Pts',(-11.4010320218078,13.130243425216,133.109285763722)) ;
#124637=CARTESIAN_POINT('Ctrl Pts',(-11.4136660872789,13.0249708380281,
133.134510598115)) ;
#124638=CARTESIAN_POINT('Ctrl Pts',(-11.4481829779826,12.8263019600079,
133.212368232307)) ;
#124639=CARTESIAN_POINT('Ctrl Pts',(-11.5209841688121,12.5833994930382,
133.392016397403)) ;
#124640=CARTESIAN_POINT('Ctrl Pts',(-11.6125279315863,12.399626766211,133.62633286024)) ;
#124641=CARTESIAN_POINT('Ctrl Pts',(-11.717528730411,12.2890731618772,133.899793229475)) ;
#124642=CARTESIAN_POINT('Ctrl Pts',(-11.827489308955,12.2602312948732,134.188086633698)) ;
#124643=CARTESIAN_POINT('Ctrl Pts',(-11.9373256353546,12.3144254522227,
134.475720243095)) ;
#124644=CARTESIAN_POINT('Ctrl Pts',(-12.0385056054605,12.4480642946114,
134.738200462315)) ;
#124645=CARTESIAN_POINT('Ctrl Pts',(-12.1250966539337,12.6516399899179,
134.958011136489)) ;
#124646=CARTESIAN_POINT('Ctrl Pts',(-12.1914055409655,12.9104453038702,
135.118592717814)) ;
#124647=CARTESIAN_POINT('Ctrl Pts',(-12.2334481989971,13.2058492691314,
135.208295779282)) ;
#124648=CARTESIAN_POINT('Ctrl Pts',(-12.2490421032075,13.5166185684314,
135.22075896859)) ;
#124649=CARTESIAN_POINT('Ctrl Pts',(-12.237555231611,13.8224101024019,135.153913230989)) ;
#124650=CARTESIAN_POINT('Ctrl Pts',(-12.2009286992494,14.0967865746008,
135.013956211633)) ;
#124651=CARTESIAN_POINT('Ctrl Pts',(-12.1422243505478,14.3244563595429,
134.80933681038)) ;
#124652=CARTESIAN_POINT('Ctrl Pts',(-12.0664283308639,14.4874742407207,
134.554802811274)) ;
#124653=CARTESIAN_POINT('Ctrl Pts',(-11.9794532032229,14.5744205093284,
134.267514255778)) ;
#124654=CARTESIAN_POINT('Ctrl Pts',(-11.8887376179606,14.5784621609188,
133.969391386105)) ;
#124655=CARTESIAN_POINT('Ctrl Pts',(-11.8014099454108,14.5000469368875,
133.68121510151)) ;
#124656=CARTESIAN_POINT('Ctrl Pts',(-11.7242121847904,14.344572658684,133.422597490784)) ;
#124657=CARTESIAN_POINT('Ctrl Pts',(-11.6633872837288,14.1228337492368,
133.211761354524)) ;
#124658=CARTESIAN_POINT('Ctrl Pts',(-11.6241753304534,13.8501516005036,
133.063988873109)) ;
#124659=CARTESIAN_POINT('Ctrl Pts',(-11.6102266012163,13.5490422759736,
132.990262219122)) ;
#124660=CARTESIAN_POINT('Ctrl Pts',(-11.6229330001199,13.2374716075454,
132.994238843195)) ;
#124661=CARTESIAN_POINT('Ctrl Pts',(-11.6625289722949,12.9386843836575,
133.076700641843)) ;
#124662=CARTESIAN_POINT('Ctrl Pts',(-11.7263131186438,12.6761376580761,
133.230018897246)) ;
#124663=CARTESIAN_POINT('Ctrl Pts',(-11.8111790631952,12.4657586342273,
133.444735878277)) ;
#124664=CARTESIAN_POINT('Ctrl Pts',(-11.911077725081,12.3246285440834,133.703497239924)) ;
#124665=CARTESIAN_POINT('Ctrl Pts',(-12.0203931142099,12.2619062203987,
133.989607303608)) ;
#124666=CARTESIAN_POINT('Ctrl Pts',(-12.1308137714884,12.282438847825,134.27917184153)) ;
#124667=CARTESIAN_POINT('Ctrl Pts',(-12.2365472028457,12.3848777791117,
134.554833667752)) ;
#124668=CARTESIAN_POINT('Ctrl Pts',(-12.3296655117059,12.5614992054213,
134.79376665016)) ;
#124669=CARTESIAN_POINT('Ctrl Pts',(-12.4047561054307,12.7995868451149,
134.980026506312)) ;
#124670=CARTESIAN_POINT('Ctrl Pts',(-12.4572212407894,13.0840300183346,
135.100012153463)) ;
#124671=CARTESIAN_POINT('Ctrl Pts',(-12.4834787916185,13.3899587420559,
135.143757569566)) ;
#124672=CARTESIAN_POINT('Ctrl Pts',(-12.4830515741286,13.6996411471026,
135.109395157013)) ;
#124673=CARTESIAN_POINT('Ctrl Pts',(-12.4562104047493,13.9903747367888,
134.997768916073)) ;
#124674=CARTESIAN_POINT('Ctrl Pts',(-12.4058859416825,14.2393240379775,
134.817669866416)) ;
#124675=CARTESIAN_POINT('Ctrl Pts',(-12.3364587321995,14.4298400275378,
134.581797033424)) ;
#124676=CARTESIAN_POINT('Ctrl Pts',(-12.2533791769935,14.5487685200995,
134.305983497596)) ;
#124677=CARTESIAN_POINT('Ctrl Pts',(-12.1631769591534,14.5869290465038,
134.009273625762)) ;
#124678=CARTESIAN_POINT('Ctrl Pts',(-12.0737300908341,14.5417666874379,
133.714933939927)) ;
#124679=CARTESIAN_POINT('Ctrl Pts',(-11.9913868019149,14.4163781165351,
133.441217765322)) ;
#124680=CARTESIAN_POINT('Ctrl Pts',(-11.9231930742505,14.2194053123055,
133.20883093906)) ;
#124681=CARTESIAN_POINT('Ctrl Pts',(-11.8749035853691,13.966643682879,133.034747880334)) ;
#124682=CARTESIAN_POINT('Ctrl Pts',(-11.8502504010927,13.6737230006816,
132.929549053018)) ;
#124683=CARTESIAN_POINT('Ctrl Pts',(-11.8520956128137,13.3629182756251,
132.901779915529)) ;
#124684=CARTESIAN_POINT('Ctrl Pts',(-11.8808821309348,13.0570540996615,
132.952775125275)) ;
#124685=CARTESIAN_POINT('Ctrl Pts',(-11.935206739513,12.7772473921445,133.078373319798)) ;
#124686=CARTESIAN_POINT('Ctrl Pts',(-12.0124542548402,12.5427680100154,
133.270768883532)) ;
#124687=CARTESIAN_POINT('Ctrl Pts',(-12.1065821193436,12.3730788139632,
133.512777848402)) ;
#124688=CARTESIAN_POINT('Ctrl Pts',(-12.2128884056889,12.2773830368376,
133.790156787178)) ;
#124689=CARTESIAN_POINT('Ctrl Pts',(-12.3238251084816,12.2641121803462,
134.081112530677)) ;
#124690=CARTESIAN_POINT('Ctrl Pts',(-12.4322664877904,12.3337583656513,
134.364784452925)) ;
#124691=CARTESIAN_POINT('Ctrl Pts',(-12.5311880770591,12.4813161327732,
134.620657084876)) ;
#124692=CARTESIAN_POINT('Ctrl Pts',(-12.6143995811317,12.6966780658121,
134.830578372292)) ;
#124693=CARTESIAN_POINT('Ctrl Pts',(-12.6763987510127,12.9640585789761,
134.978555464806)) ;
#124694=CARTESIAN_POINT('Ctrl Pts',(-12.7135158186447,13.263362217281,135.053945116895)) ;
#124695=CARTESIAN_POINT('Ctrl Pts',(-12.7240587194064,13.5752569117425,
135.051579196554)) ;
#124696=CARTESIAN_POINT('Ctrl Pts',(-12.7076312662777,13.8766503644376,
134.970371111819)) ;
#124697=CARTESIAN_POINT('Ctrl Pts',(-12.6665728722074,14.1438627014427,
134.817419676745)) ;
#124698=CARTESIAN_POINT('Ctrl Pts',(-12.6039948511626,14.3611558948339,
134.601376453978)) ;
#124699=CARTESIAN_POINT('Ctrl Pts',(-12.525511231779,14.5102071341288,134.338966946009)) ;
#124700=CARTESIAN_POINT('Ctrl Pts',(-12.437892956187,14.5813677967462,134.050044481287)) ;
#124701=CARTESIAN_POINT('Ctrl Pts',(-12.3470512850699,14.5701314848988,
133.751485197144)) ;
#124702=CARTESIAN_POINT('Ctrl Pts',(-12.2606985128047,14.4759918680502,
133.465989914691)) ;
#124703=CARTESIAN_POINT('Ctrl Pts',(-12.1862330004605,14.3066892261713,
133.21535199468)) ;
#124704=CARTESIAN_POINT('Ctrl Pts',(-12.1294493909379,14.0751878259722,
133.016480731285)) ;
#124705=CARTESIAN_POINT('Ctrl Pts',(-12.0947410023423,13.7962286301239,
132.881967768999)) ;
#124706=CARTESIAN_POINT('Ctrl Pts',(-12.0856036163849,13.489739255107,132.822078592483)) ;
#124707=CARTESIAN_POINT('Ctrl Pts',(-12.1036908448989,13.1781056591445,
132.841674234956)) ;
#124708=CARTESIAN_POINT('Ctrl Pts',(-12.1476711989599,12.8871394405402,
132.93727175541)) ;
#124709=CARTESIAN_POINT('Ctrl Pts',(-12.2160680563488,12.6313542948275,
133.103833575226)) ;
#124710=CARTESIAN_POINT('Ctrl Pts',(-12.304329738268,12.4333423799844,133.328491824527)) ;
#124711=CARTESIAN_POINT('Ctrl Pts',(-12.4060576918611,12.3067788244502,
133.592708701729)) ;
#124712=CARTESIAN_POINT('Ctrl Pts',(-12.5164365286364,12.2592790120272,
133.88187589207)) ;
#124713=CARTESIAN_POINT('Ctrl Pts',(-12.6267907100765,12.2958890745914,
134.171123224698)) ;
#124714=CARTESIAN_POINT('Ctrl Pts',(-12.7300880676908,12.412515961838,134.439866942717)) ;
#124715=CARTESIAN_POINT('Ctrl Pts',(-12.8204242204879,12.6017795181092,
134.670628068448)) ;
#124716=CARTESIAN_POINT('Ctrl Pts',(-12.8917076442904,12.8508820386888,
134.845636319413)) ;
#124717=CARTESIAN_POINT('Ctrl Pts',(-12.9391378423724,13.1389626270395,
134.951203029648)) ;
#124718=CARTESIAN_POINT('Ctrl Pts',(-12.9606749539296,13.4502019217322,
134.980813679307)) ;
#124719=CARTESIAN_POINT('Ctrl Pts',(-12.9549597016316,13.7571545307035,
134.931066987763)) ;
#124720=CARTESIAN_POINT('Ctrl Pts',(-12.9237083445955,14.0399279839555,
134.806780374082)) ;
#124721=CARTESIAN_POINT('Ctrl Pts',(-12.8691654878234,14.2804627639154,
134.614188843193)) ;
#124722=CARTESIAN_POINT('Ctrl Pts',(-12.796779207288,14.4580430592262,134.369713555185)) ;
#124723=CARTESIAN_POINT('Ctrl Pts',(-12.7117359750767,14.5623041916472,
134.08810713179)) ;
#124724=CARTESIAN_POINT('Ctrl Pts',(-12.6214033477903,14.5848738279965,
133.791154683889)) ;
#124725=CARTESIAN_POINT('Ctrl Pts',(-12.5321103413004,14.5236285085623,
133.496991779123)) ;
#124726=CARTESIAN_POINT('Ctrl Pts',(-12.4524536540473,14.3842858340258,
133.231308118728)) ;
#124727=CARTESIAN_POINT('Ctrl Pts',(-12.3875985781014,14.1760036072079,
133.008727211519)) ;
#124728=CARTESIAN_POINT('Ctrl Pts',(-12.343257008202,13.9123644757914,132.845931511127)) ;
#124729=CARTESIAN_POINT('Ctrl Pts',(-12.3236960043334,13.6155078278093,
132.755750850139)) ;
#124730=CARTESIAN_POINT('Ctrl Pts',(-12.3305423757926,13.3048785674805,
132.742701375793)) ;
#124731=CARTESIAN_POINT('Ctrl Pts',(-12.364391139041,13.0013157661824,132.808379578404)) ;
#124732=CARTESIAN_POINT('Ctrl Pts',(-12.4232870796455,12.7290184016179,
132.947345432854)) ;
#124733=CARTESIAN_POINT('Ctrl Pts',(-12.5039453987805,12.5059452399051,
133.149824850825)) ;
#124734=CARTESIAN_POINT('Ctrl Pts',(-12.601100948694,12.3489356287849,133.400549810363)) ;
#124735=CARTESIAN_POINT('Ctrl Pts',(-12.7085376350216,12.2685725543234,
133.681330547702)) ;
#124736=CARTESIAN_POINT('Ctrl Pts',(-12.81992922974,12.2709800429639,133.973502340089)) ;
#124737=CARTESIAN_POINT('Ctrl Pts',(-12.9269390332323,12.3558597729099,
134.253043661359)) ;
#124738=CARTESIAN_POINT('Ctrl Pts',(-13.0234674587026,12.5173149603475,
134.501876529553)) ;
#124739=CARTESIAN_POINT('Ctrl Pts',(-13.1029392456179,12.7436533990505,
134.700909775251)) ;
#124740=CARTESIAN_POINT('Ctrl Pts',(-13.1604706398527,13.0184391558732,
134.835869526156)) ;
#124741=CARTESIAN_POINT('Ctrl Pts',(-13.1927351300675,13.3224259864685,
134.896992447974)) ;
#124742=CARTESIAN_POINT('Ctrl Pts',(-13.1980809728987,13.6337497242247,
134.879467221621)) ;
#124743=CARTESIAN_POINT('Ctrl Pts',(-13.1768448022821,13.9298382282655,
134.784301593456)) ;
#124744=CARTESIAN_POINT('Ctrl Pts',(-13.1313657290487,14.189430649662,134.618348210303)) ;
#124745=CARTESIAN_POINT('Ctrl Pts',(-13.0654522975526,14.394475769408,134.392641880832)) ;
#124746=CARTESIAN_POINT('Ctrl Pts',(-12.9849210113024,14.5294751555696,
134.124342295431)) ;
#124747=CARTESIAN_POINT('Ctrl Pts',(-12.8958448031638,14.5857784692471,
133.831003029331)) ;
#124748=CARTESIAN_POINT('Ctrl Pts',(-12.8052622704107,14.5584757915825,
133.533179544693)) ;
#124749=CARTESIAN_POINT('Ctrl Pts',(-12.7209347423681,14.4499269428434,
133.253742933785)) ;
#124750=CARTESIAN_POINT('Ctrl Pts',(-12.6492262981972,14.2678362353556,
133.011138377953)) ;
#124751=CARTESIAN_POINT('Ctrl Pts',(-12.5961058796925,14.025181457992,132.822834388908)) ;
#124752=CARTESIAN_POINT('Ctrl Pts',(-12.566099157907,13.7395989373351,132.70207237033)) ;
#124753=CARTESIAN_POINT('Ctrl Pts',(-12.5620613966533,13.4312396323536,
132.657157630282)) ;
#124754=CARTESIAN_POINT('Ctrl Pts',(-12.5849599127162,13.1225497358479,
132.690961347731)) ;
#124755=CARTESIAN_POINT('Ctrl Pts',(-12.6341066221525,12.8344723691042,
132.801333767966)) ;
#124756=CARTESIAN_POINT('Ctrl Pts',(-12.7064275143261,12.5894057797878,
132.97950088557)) ;
#124757=CARTESIAN_POINT('Ctrl Pts',(-12.7976132379566,12.403866954954,133.212753563123)) ;
#124758=CARTESIAN_POINT('Ctrl Pts',(-12.9017755510911,12.2913271395126,
133.483934150059)) ;
#124759=CARTESIAN_POINT('Ctrl Pts',(-13.0125233870004,12.2598830910024,
133.774265375283)) ;
#124760=CARTESIAN_POINT('Ctrl Pts',(-13.1219338101741,12.3117248800856,
134.060824044522)) ;
#124761=CARTESIAN_POINT('Ctrl Pts',(-13.2236212395332,12.4432581969561,
134.3247309762)) ;
#124762=CARTESIAN_POINT('Ctrl Pts',(-13.3105761021659,12.6447768479475,
134.545654875861)) ;
#124763=CARTESIAN_POINT('Ctrl Pts',(-13.3775463734392,12.9020427023331,
134.708180411592)) ;
#124764=CARTESIAN_POINT('Ctrl Pts',(-13.4203792864058,13.1969220955149,
134.800163305388)) ;
#124765=CARTESIAN_POINT('Ctrl Pts',(-13.4367503191474,13.5073634201221,
134.814917250719)) ;
#124766=CARTESIAN_POINT('Ctrl Pts',(-13.4260632417067,13.8135028677167,
134.750425039199)) ;
#124767=CARTESIAN_POINT('Ctrl Pts',(-13.3902019475775,14.0890635163078,
134.612711315212)) ;
#124768=CARTESIAN_POINT('Ctrl Pts',(-13.3317903671586,14.3192685446141,
134.408803368418)) ;
#124769=CARTESIAN_POINT('Ctrl Pts',(-13.2566727359362,14.4835637983032,
134.156382324995)) ;
#124770=CARTESIAN_POINT('Ctrl Pts',(-13.169938469823,14.5730188285823,133.869793548611)) ;
#124771=CARTESIAN_POINT('Ctrl Pts',(-13.0792140349077,14.5795967764284,
133.571640925124)) ;
#124772=CARTESIAN_POINT('Ctrl Pts',(-12.9915123363953,14.5032853646564,
133.282297922924)) ;
#124773=CARTESIAN_POINT('Ctrl Pts',(-12.9140022949989,14.3501151249434,
133.022810830752)) ;
#124774=CARTESIAN_POINT('Ctrl Pts',(-12.8524828347806,14.1289951799062,
132.809814591485)) ;
#124775=CARTESIAN_POINT('Ctrl Pts',(-12.812909471201,13.8600883343583,132.661298344278)) ;
#124776=CARTESIAN_POINT('Ctrl Pts',(-12.7979838300487,13.5571075891159,
132.584435996641)) ;
#124777=CARTESIAN_POINT('Ctrl Pts',(-12.8100524681606,13.246144038551,132.586620648894)) ;
#124778=CARTESIAN_POINT('Ctrl Pts',(-12.8486585081772,12.9474784018938,
132.666294839717)) ;
#124779=CARTESIAN_POINT('Ctrl Pts',(-12.9123435540383,12.6818049804595,
132.819067818709)) ;
#124780=CARTESIAN_POINT('Ctrl Pts',(-12.9960885885724,12.4713261551404,
133.030763914884)) ;
#124781=CARTESIAN_POINT('Ctrl Pts',(-13.0961110849497,12.3273775060339,
133.28971686147)) ;
#124782=CARTESIAN_POINT('Ctrl Pts',(-13.2046537208031,12.2625380401702,
133.573765385136)) ;
#124783=CARTESIAN_POINT('Ctrl Pts',(-13.3161047474788,12.2810707697993,
133.866034649765)) ;
#124784=CARTESIAN_POINT('Ctrl Pts',(-13.4209550321827,12.3803129449242,
134.139476431641)) ;
#124785=CARTESIAN_POINT('Ctrl Pts',(-13.5151074581699,12.5556239471542,
134.381234906763)) ;
#124786=CARTESIAN_POINT('Ctrl Pts',(-13.5905152917745,12.7914917481058,
134.56853383512)) ;
#124787=CARTESIAN_POINT('Ctrl Pts',(-13.6438208480912,13.0750410185669,
134.690941087749)) ;
#124788=CARTESIAN_POINT('Ctrl Pts',(-13.6708818850032,13.3808908825506,
134.737002821677)) ;
#124789=CARTESIAN_POINT('Ctrl Pts',(-13.6712113749413,13.6908805105498,
134.704840536306)) ;
#124790=CARTESIAN_POINT('Ctrl Pts',(-13.6451962539586,13.9819858860809,
134.595693722298)) ;
#124791=CARTESIAN_POINT('Ctrl Pts',(-13.5953602405429,14.2331023170552,
134.416922555225)) ;
#124792=CARTESIAN_POINT('Ctrl Pts',(-13.5264879005436,14.425373738482,134.18270881116)) ;
#124793=CARTESIAN_POINT('Ctrl Pts',(-13.4431809018768,14.5469025467051,
133.906032348469)) ;
#124794=CARTESIAN_POINT('Ctrl Pts',(-13.3536808661597,14.5868798002751,
133.611604960804)) ;
#124795=CARTESIAN_POINT('Ctrl Pts',(-13.2640066674077,14.544243012127,133.316555537026)) ;
#124796=CARTESIAN_POINT('Ctrl Pts',(-13.1814521156651,14.4211466682183,
133.042262184532)) ;
#124797=CARTESIAN_POINT('Ctrl Pts',(-13.1127573154354,14.2262607668007,
132.808422365474)) ;
#124798=CARTESIAN_POINT('Ctrl Pts',(-13.0637294316636,13.9744157440355,
132.632118382732)) ;
#124799=CARTESIAN_POINT('Ctrl Pts',(-13.0384131550304,13.6824769956245,
132.525002593695)) ;
#124800=CARTESIAN_POINT('Ctrl Pts',(-13.0393827410548,13.3726811075526,
132.494761352875)) ;
#124801=CARTESIAN_POINT('Ctrl Pts',(-13.0676131106458,13.0644552653701,
132.54392030028)) ;
#124802=CARTESIAN_POINT('Ctrl Pts',(-13.121061409599,12.7851437456734,132.667125642549)) ;
#124803=CARTESIAN_POINT('Ctrl Pts',(-13.1974519715877,12.5493640024945,
132.85708998106)) ;
#124804=CARTESIAN_POINT('Ctrl Pts',(-13.2913743910714,12.376970726474,133.098407984603)) ;
#124805=CARTESIAN_POINT('Ctrl Pts',(-13.3977315690652,12.2789142943649,
133.375849754409)) ;
#124806=CARTESIAN_POINT('Ctrl Pts',(-13.5083089279773,12.2633331335236,
133.665852727719)) ;
#124807=CARTESIAN_POINT('Ctrl Pts',(-13.6171709080123,12.3306602868788,
133.950680512518)) ;
#124808=CARTESIAN_POINT('Ctrl Pts',(-13.716558237696,12.4766203405944,134.20786333325)) ;
#124809=CARTESIAN_POINT('Ctrl Pts',(-13.7998719371381,12.6891737116268,
134.418250852531)) ;
#124810=CARTESIAN_POINT('Ctrl Pts',(-13.8626642883641,12.9552556025245,
134.568527949207)) ;
#124811=CARTESIAN_POINT('Ctrl Pts',(-13.9006336626054,13.2547271279824,
134.646319603981)) ;
#124812=CARTESIAN_POINT('Ctrl Pts',(-13.9118864628166,13.5662747472623,
134.646059940436)) ;
#124813=CARTESIAN_POINT('Ctrl Pts',(-13.8963623296496,13.8673047437589,
134.567609313136)) ;
#124814=CARTESIAN_POINT('Ctrl Pts',(-13.8558569907757,14.1368397654386,
134.416143585266)) ;
#124815=CARTESIAN_POINT('Ctrl Pts',(-13.7940607472378,14.3550474854522,
134.202509973235)) ;
#124816=CARTESIAN_POINT('Ctrl Pts',(-13.7160248113303,14.5066809969925,
133.941403361426)) ;
#124817=CARTESIAN_POINT('Ctrl Pts',(-13.6281511120074,14.5805550021418,
133.651572184232)) ;
#124818=CARTESIAN_POINT('Ctrl Pts',(-13.5375371319342,14.5715434154247,
133.353768334661)) ;
#124819=CARTESIAN_POINT('Ctrl Pts',(-13.45124859715,14.4804614253832,133.068587808668)) ;
#124820=CARTESIAN_POINT('Ctrl Pts',(-13.37603363823,14.3129344322758,132.815646261363)) ;
#124821=CARTESIAN_POINT('Ctrl Pts',(-13.3185466362034,14.0824719348205,
132.61464582826)) ;
#124822=CARTESIAN_POINT('Ctrl Pts',(-13.2831865687033,13.8045959520742,
132.478235291779)) ;
#124823=CARTESIAN_POINT('Ctrl Pts',(-13.2732886080672,13.4994871825109,
132.416220120997)) ;
#124824=CARTESIAN_POINT('Ctrl Pts',(-13.2904782460621,13.1877258357311,
132.4332010356)) ;
#124825=CARTESIAN_POINT('Ctrl Pts',(-13.3338717484347,12.8947281462995,
132.526953391422)) ;
#124826=CARTESIAN_POINT('Ctrl Pts',(-13.4017873141061,12.6375710279023,
132.692078445121)) ;
#124827=CARTESIAN_POINT('Ctrl Pts',(-13.4890204567564,12.4386468610117,
132.91391883166)) ;
#124828=CARTESIAN_POINT('Ctrl Pts',(-13.5909900935397,12.3091460957756,
133.178653315814)) ;
#124829=CARTESIAN_POINT('Ctrl Pts',(-13.7006170362624,12.2596124823544,
133.465818195012)) ;
#124830=CARTESIAN_POINT('Ctrl Pts',(-13.8113185228843,12.2934287608505,
133.756004819139)) ;
#124831=CARTESIAN_POINT('Ctrl Pts',(-13.915353328685,12.4085128327331,134.026758002108)) ;
#124832=CARTESIAN_POINT('Ctrl Pts',(-14.0058487547682,12.5956557289105,
134.25806721356)) ;
#124833=CARTESIAN_POINT('Ctrl Pts',(-14.0775354249195,12.8419007225992,
134.434408810845)) ;
#124834=CARTESIAN_POINT('Ctrl Pts',(-14.1259869919832,13.1310174961036,
134.542734109053)) ;
#124835=CARTESIAN_POINT('Ctrl Pts',(-14.1481532280157,13.4394174357417,
134.574460881878)) ;
#124836=CARTESIAN_POINT('Ctrl Pts',(-14.1433213153389,13.7489280911395,
134.52706348914)) ;
#124837=CARTESIAN_POINT('Ctrl Pts',(-14.1126273341243,14.0326636377924,
134.4043884176)) ;
#124838=CARTESIAN_POINT('Ctrl Pts',(-14.0589544553989,14.2739040852335,
134.214471649233)) ;
#124839=CARTESIAN_POINT('Ctrl Pts',(-13.9866513654702,14.4542739196418,
133.970073178127)) ;
#124840=CARTESIAN_POINT('Ctrl Pts',(-13.9022431575821,14.5602989728585,
133.69047622448)) ;
#124841=CARTESIAN_POINT('Ctrl Pts',(-13.8116472296482,14.5853165149043,
133.392628115289)) ;
#124842=CARTESIAN_POINT('Ctrl Pts',(-13.7227715761924,14.5269566975762,
133.099903849994)) ;
#124843=CARTESIAN_POINT('Ctrl Pts',(-13.6421710441629,14.3891797557674,
132.831239376946)) ;
#124844=CARTESIAN_POINT('Ctrl Pts',(-13.5768120757702,14.1817902541555,
132.607121636432)) ;
#124845=CARTESIAN_POINT('Ctrl Pts',(-13.5321752968255,13.9219441435514,
132.443766715308)) ;
#124846=CARTESIAN_POINT('Ctrl Pts',(-13.5116468125809,13.6244332360091,
132.350588803698)) ;
#124847=CARTESIAN_POINT('Ctrl Pts',(-13.5177395880814,13.3138307533241,
132.335338987358)) ;
#124848=CARTESIAN_POINT('Ctrl Pts',(-13.550960796519,13.0089906490168,132.399097001905)) ;
#124849=CARTESIAN_POINT('Ctrl Pts',(-13.6089629814311,12.7367004546504,
132.535589377863)) ;
#124850=CARTESIAN_POINT('Ctrl Pts',(-13.6890168410449,12.5117902226442,
132.736297036857)) ;
#124851=CARTESIAN_POINT('Ctrl Pts',(-13.7857765994093,12.3525055718321,
132.985859011256)) ;
#124852=CARTESIAN_POINT('Ctrl Pts',(-13.8934707756066,12.2695603422194,
133.26725204525)) ;
#124853=CARTESIAN_POINT('Ctrl Pts',(-14.0046967664786,12.2698997587057,
133.55899053355)) ;
#124854=CARTESIAN_POINT('Ctrl Pts',(-14.1116278789902,12.3521640390818,
133.838391990892)) ;
#124855=CARTESIAN_POINT('Ctrl Pts',(-14.2086596235602,12.5116415634716,
134.088662656359)) ;
#124856=CARTESIAN_POINT('Ctrl Pts',(-14.2886301094502,12.7360069700772,
134.289191940705)) ;
#124857=CARTESIAN_POINT('Ctrl Pts',(-14.3469357043129,13.0100796293743,
134.426358261043)) ;
#124858=CARTESIAN_POINT('Ctrl Pts',(-14.3799244113915,13.3126253374921,
134.489695495591)) ;
#124859=CARTESIAN_POINT('Ctrl Pts',(-14.3860830172785,13.6254715524663,
134.474389220875)) ;
#124860=CARTESIAN_POINT('Ctrl Pts',(-14.3656426582198,13.9212365418522,
134.381670680832)) ;
#124861=CARTESIAN_POINT('Ctrl Pts',(-14.3207442896342,14.1826934673073,
134.217342153918)) ;
#124862=CARTESIAN_POINT('Ctrl Pts',(-14.2556054285751,14.3889686584202,
133.994016051553)) ;
#124863=CARTESIAN_POINT('Ctrl Pts',(-14.1749150301037,14.5271450156122,
133.725037501823)) ;
#124864=CARTESIAN_POINT('Ctrl Pts',(-14.0858847391717,14.5852339348323,
133.431810575258)) ;
#124865=CARTESIAN_POINT('Ctrl Pts',(-13.995836417164,14.5605427661762,133.135766593463)) ;
#124866=CARTESIAN_POINT('Ctrl Pts',(-13.9109761751291,14.4541441537073,
132.854676254093)) ;
#124867=CARTESIAN_POINT('Ctrl Pts',(-13.8388670781715,14.2740963281162,
132.610925952439)) ;
#124868=CARTESIAN_POINT('Ctrl Pts',(-13.7850008698074,14.0323112919108,
132.420355351968)) ;
#124869=CARTESIAN_POINT('Ctrl Pts',(-13.75439702107,13.747634010638,132.297856801284)) ;
#124870=CARTESIAN_POINT('Ctrl Pts',(-13.7495551212371,13.4408490944308,
132.250724773907)) ;
#124871=CARTESIAN_POINT('Ctrl Pts',(-13.7718087995071,13.1304291630284,
132.282485369413)) ;
#124872=CARTESIAN_POINT('Ctrl Pts',(-13.8200527246112,12.8426172833002,
132.390360822731)) ;
#124873=CARTESIAN_POINT('Ctrl Pts',(-13.8920711083226,12.5951022439345,
132.567502086748)) ;
#124874=CARTESIAN_POINT('Ctrl Pts',(-13.9823448757499,12.4086451367459,
132.798263093832)) ;
#124875=CARTESIAN_POINT('Ctrl Pts',(-14.0864872492279,12.2933533526165,
133.069289241896)) ;
#124876=CARTESIAN_POINT('Ctrl Pts',(-14.1971250254784,12.2596356642452,
133.359312878413)) ;
#124877=CARTESIAN_POINT('Ctrl Pts',(-14.3066070487481,12.3091205579985,
133.646092913872)) ;
#124878=CARTESIAN_POINT('Ctrl Pts',(-14.4084397056733,12.4379929419073,
133.910495450968)) ;
#124879=CARTESIAN_POINT('Ctrl Pts',(-14.4963291891085,12.6386445208212,
134.133986510367)) ;
#124880=CARTESIAN_POINT('Ctrl Pts',(-14.5637307355296,12.8942395319149,
134.297835385292)) ;
#124881=CARTESIAN_POINT('Ctrl Pts',(-14.6072585432434,13.1876524015431,
134.391918163003)) ;
#124882=CARTESIAN_POINT('Ctrl Pts',(-14.6244317780042,13.4984175352415,
134.408961571031)) ;
#124883=CARTESIAN_POINT('Ctrl Pts',(-14.6145964259596,13.804322978022,134.347044191526)) ;
#124884=CARTESIAN_POINT('Ctrl Pts',(-14.5792218548473,14.0825044690989,
134.210565926119)) ;
#124885=CARTESIAN_POINT('Ctrl Pts',(-14.5215034218389,14.3134151939565,
134.008790285794)) ;
#124886=CARTESIAN_POINT('Ctrl Pts',(-14.4467983753446,14.4799820430956,
133.757558503687)) ;
#124887=CARTESIAN_POINT('Ctrl Pts',(-14.3599545208039,14.5717629111611,
133.470532635478)) ;
#124888=CARTESIAN_POINT('Ctrl Pts',(-14.2697026757989,14.5804902345133,
133.173926231809)) ;
#124889=CARTESIAN_POINT('Ctrl Pts',(-14.1818550312755,14.5068426017295,
132.884179222822)) ;
#124890=CARTESIAN_POINT('Ctrl Pts',(-14.1038707278137,14.3556215142155,
132.62326810925)) ;
#124891=CARTESIAN_POINT('Ctrl Pts',(-14.0418273324944,14.1365915328991,
132.408782119764)) ;
#124892=CARTESIAN_POINT('Ctrl Pts',(-14.0014978593324,13.8680779330351,
132.25795920505)) ;
#124893=CARTESIAN_POINT('Ctrl Pts',(-13.9858123788647,13.567186800724,132.1790395569)) ;
#124894=CARTESIAN_POINT('Ctrl Pts',(-13.9971900795798,13.2537545062593,
132.178943151311)) ;
#124895=CARTESIAN_POINT('Ctrl Pts',(-14.0349672123987,12.9561224404112,
132.256375223925)) ;
#124896=CARTESIAN_POINT('Ctrl Pts',(-14.0977176900152,12.6895769772328,
132.406492249292)) ;
#124897=CARTESIAN_POINT('Ctrl Pts',(-14.1811824094918,12.4765148457442,
132.617258389176)) ;
#124898=CARTESIAN_POINT('Ctrl Pts',(-14.2808752566479,12.3303992852147,
132.875241621594)) ;
#124899=CARTESIAN_POINT('Ctrl Pts',(-14.3893361764667,12.2633426599666,
133.159025189874)) ;
#124900=CARTESIAN_POINT('Ctrl Pts',(-14.5002482335499,12.279103982185,133.44989801271)) ;
#124901=CARTESIAN_POINT('Ctrl Pts',(-14.606036142801,12.3764767576561,133.725867717232)) ;
#124902=CARTESIAN_POINT('Ctrl Pts',(-14.7005487610914,12.5500289101503,
133.968688363446)) ;
#124903=CARTESIAN_POINT('Ctrl Pts',(-14.7763877253057,12.7839578561676,
134.157302063182)) ;
#124904=CARTESIAN_POINT('Ctrl Pts',(-14.8303556214475,13.0658041228342,
134.281713139573)) ;
#124905=CARTESIAN_POINT('Ctrl Pts',(-14.8583242280902,13.3726170647806,
134.330277268878)) ;
#124906=CARTESIAN_POINT('Ctrl Pts',(-14.8593033695257,13.6826397531364,
134.300029063359)) ;
#124907=CARTESIAN_POINT('Ctrl Pts',(-14.8341682762792,13.9734160289762,
134.193592262512)) ;
#124908=CARTESIAN_POINT('Ctrl Pts',(-14.7848225301107,14.2269288377743,
134.01613594009)) ;
#124909=CARTESIAN_POINT('Ctrl Pts',(-14.7165117945592,14.4205112274409,
133.783623816956)) ;
#124910=CARTESIAN_POINT('Ctrl Pts',(-14.6339676590262,14.5441065971854,
133.509333914104)) ;
#124911=CARTESIAN_POINT('Ctrl Pts',(-14.543930379516,14.5870792664814,133.213098404156)) ;
#124912=CARTESIAN_POINT('Ctrl Pts',(-14.4540579265701,14.5462510463569,
132.917427016041)) ;
#124913=CARTESIAN_POINT('Ctrl Pts',(-14.371611013546,14.426108976537,132.643620532443)) ;
#124914=CARTESIAN_POINT('Ctrl Pts',(-14.3020392766499,14.2320089292168,
132.40702833977)) ;
#124915=CARTESIAN_POINT('Ctrl Pts',(-14.2526185482894,13.9821034896837,
132.229676391051)) ;
#124916=CARTESIAN_POINT('Ctrl Pts',(-14.2265818489062,13.6914860951574,
132.120501165582)) ;
#124917=CARTESIAN_POINT('Ctrl Pts',(-14.2267429244149,13.3820426901867,
132.087911578203)) ;
#124918=CARTESIAN_POINT('Ctrl Pts',(-14.254191395465,13.0731824495073,132.134765071221)) ;
#124919=CARTESIAN_POINT('Ctrl Pts',(-14.3069443025686,12.7927891220342,
132.255932871511)) ;
#124920=CARTESIAN_POINT('Ctrl Pts',(-14.3827474169739,12.5553086793863,
132.444172542437)) ;
#124921=CARTESIAN_POINT('Ctrl Pts',(-14.4764049521844,12.3807971317929,
132.684665215156)) ;
#124922=CARTESIAN_POINT('Ctrl Pts',(-14.5821181703053,12.2807361314401,
132.960349357715)) ;
#124923=CARTESIAN_POINT('Ctrl Pts',(-14.6930022007284,12.2625961547027,
133.25114070724)) ;
#124924=CARTESIAN_POINT('Ctrl Pts',(-14.8018555982343,12.3275534841213,
133.535998308902)) ;
#124925=CARTESIAN_POINT('Ctrl Pts',(-14.9016022738294,12.4713200428819,
133.794229183378)) ;
#124926=CARTESIAN_POINT('Ctrl Pts',(-14.9854766671218,12.6818354528321,
134.006273987192)) ;
#124927=CARTESIAN_POINT('Ctrl Pts',(-15.0492924045249,12.9488696704077,
134.159286266937)) ;
#124928=CARTESIAN_POINT('Ctrl Pts',(-15.0875838966062,13.2449965342222,
134.238327513091)) ;
#124929=CARTESIAN_POINT('Ctrl Pts',(-15.0997594597476,13.5577147943103,
134.240627823641)) ;
#124930=CARTESIAN_POINT('Ctrl Pts',(-15.084934557853,13.85913805832,134.164243465792)) ;
#124931=CARTESIAN_POINT('Ctrl Pts',(-15.045045788871,14.1301670031634,134.014537631445)) ;
#124932=CARTESIAN_POINT('Ctrl Pts',(-14.9837834759939,14.3498259886228,
133.802481832815)) ;
#124933=CARTESIAN_POINT('Ctrl Pts',(-14.9062566288333,14.5033075932482,
133.542915911526)) ;
#124934=CARTESIAN_POINT('Ctrl Pts',(-14.8185287898435,14.5795881010438,
133.253492977493)) ;
#124935=CARTESIAN_POINT('Ctrl Pts',(-14.7278599526965,14.5729975043218,
132.95551789938)) ;
#124936=CARTESIAN_POINT('Ctrl Pts',(-14.6411058259546,14.4837968036715,
132.668880234287)) ;
#124937=CARTESIAN_POINT('Ctrl Pts',(-14.5656171298555,14.3181445279312,
132.415171042367)) ;
#124938=CARTESIAN_POINT('Ctrl Pts',(-14.5077297104301,14.0900336140832,
132.213103849881)) ;
#124939=CARTESIAN_POINT('Ctrl Pts',(-14.4715993847153,13.812578673719,132.074363369864)) ;
#124940=CARTESIAN_POINT('Ctrl Pts',(-14.4610127677944,13.5087142835403,
132.010421751901)) ;
#124941=CARTESIAN_POINT('Ctrl Pts',(-14.4773187825163,13.1970641651478,
132.024851943105)) ;
#124942=CARTESIAN_POINT('Ctrl Pts',(-14.5201391181318,12.9023258221912,
132.116819737304)) ;
#124943=CARTESIAN_POINT('Ctrl Pts',(-14.5872047154943,12.644685125118,132.279571832042)) ;
#124944=CARTESIAN_POINT('Ctrl Pts',(-14.6739254344846,12.4436426605292,
132.499899000355)) ;
#124945=CARTESIAN_POINT('Ctrl Pts',(-14.7756943865195,12.3118006025232,
132.76400568983)) ;
#124946=CARTESIAN_POINT('Ctrl Pts',(-14.8852228559566,12.2597626712743,
133.050877142863)) ;
#124947=CARTESIAN_POINT('Ctrl Pts',(-14.996405412822,12.291703918078,133.342339118856)) ;
#124948=CARTESIAN_POINT('Ctrl Pts',(-15.0999158484911,12.4035190278675,
133.611829800801)) ;
#124949=CARTESIAN_POINT('Ctrl Pts',(-15.1916464629765,12.5902948833878,
133.846460292102)) ;
#124950=CARTESIAN_POINT('Ctrl Pts',(-15.263459595405,12.8337324563932,134.023377894843)) ;
#124951=CARTESIAN_POINT('Ctrl Pts',(-15.3129209886316,13.1235886445067,
134.134455736189)) ;
#124952=CARTESIAN_POINT('Ctrl Pts',(-15.3355967699743,13.4302519414742,
134.167832537199)) ;
#124953=CARTESIAN_POINT('Ctrl Pts',(-15.3317353809439,13.7390104772614,
134.123396838734)) ;
#124954=CARTESIAN_POINT('Ctrl Pts',(-15.3014976225916,14.0260062302898,
134.001786192092)) ;
#124955=CARTESIAN_POINT('Ctrl Pts',(-15.2486500083372,14.267226902407,133.814466538076)) ;
#124956=CARTESIAN_POINT('Ctrl Pts',(-15.1769102109966,14.4498458952908,
133.571722166596)) ;
#124957=CARTESIAN_POINT('Ctrl Pts',(-15.092355680759,14.5586319352592,133.291541367095)) ;
#124958=CARTESIAN_POINT('Ctrl Pts',(-15.0017957168739,14.5856242088894,
132.993790062797)) ;
#124959=CARTESIAN_POINT('Ctrl Pts',(-14.913162148146,14.5299078181027,132.701917946807)) ;
#124960=CARTESIAN_POINT('Ctrl Pts',(-14.8320122022859,14.3940107606991,
132.431562888425)) ;
#124961=CARTESIAN_POINT('Ctrl Pts',(-14.766278636578,14.1888420463645,132.206424468802)) ;
#124962=CARTESIAN_POINT('Ctrl Pts',(-14.7209263709597,13.9299824320437,
132.040931181505)) ;
#124963=CARTESIAN_POINT('Ctrl Pts',(-14.6996678155027,13.6339608398866,
131.94570431671)) ;
#124964=CARTESIAN_POINT('Ctrl Pts',(-14.7049859859979,13.3227158538243,
131.928107883363)) ;
#124965=CARTESIAN_POINT('Ctrl Pts',(-14.737248964863,13.018724359071,131.989222699374)) ;
#124966=CARTESIAN_POINT('Ctrl Pts',(-14.794605691487,12.7442183705068,132.123727500233)) ;
#124967=CARTESIAN_POINT('Ctrl Pts',(-14.8745544931001,12.5167188464288,
132.323966018835)) ;
#124968=CARTESIAN_POINT('Ctrl Pts',(-14.9704908580808,12.3563385813199,
132.571280103058)) ;
#124969=CARTESIAN_POINT('Ctrl Pts',(-15.0777402856303,12.2709228201269,
132.851435182846)) ;
#124970=CARTESIAN_POINT('Ctrl Pts',(-15.1890905041819,12.2686101214329,
133.143498939687)) ;
#124971=CARTESIAN_POINT('Ctrl Pts',(-15.296477362581,12.3485946759632,133.42416126715)) ;
#124972=CARTESIAN_POINT('Ctrl Pts',(-15.3941920414611,12.5068357117029,
133.676309304964)) ;
#124973=CARTESIAN_POINT('Ctrl Pts',(-15.4742237583938,12.7283302241023,
133.877209325191)) ;
#124974=CARTESIAN_POINT('Ctrl Pts',(-15.5333688655842,13.0013551128606,
134.016794223351)) ;
#124975=CARTESIAN_POINT('Ctrl Pts',(-15.5671263312359,13.3039532563625,
134.082313844199)) ;
#124976=CARTESIAN_POINT('Ctrl Pts',(-15.5741033716375,13.6158509275634,
134.069512761149)) ;
#124977=CARTESIAN_POINT('Ctrl Pts',(-15.554290548579,13.9138456123568,133.978453644798)) ;
#124978=CARTESIAN_POINT('Ctrl Pts',(-15.510233046302,14.1752853033959,133.816745546828)) ;
#124979=CARTESIAN_POINT('Ctrl Pts',(-15.4455219248175,14.3839669210711,
133.594594016653)) ;
#124980=CARTESIAN_POINT('Ctrl Pts',(-15.3652594931835,14.5240578631267,
133.326904321361)) ;
#124981=CARTESIAN_POINT('Ctrl Pts',(-15.2764638116133,14.584818935146,133.034389619939)) ;
#124982=CARTESIAN_POINT('Ctrl Pts',(-15.1857623337452,14.5621167265827,
132.736215402154)) ;
#124983=CARTESIAN_POINT('Ctrl Pts',(-15.1011943241471,14.4583966229727,
132.456187822001)) ;
#124984=CARTESIAN_POINT('Ctrl Pts',(-15.0285434791858,14.2803903749363,
132.210827677929)) ;
#124985=CARTESIAN_POINT('Ctrl Pts',(-14.9741792799019,14.0406559377366,
132.018869665459)) ;
#124986=CARTESIAN_POINT('Ctrl Pts',(-14.9427029763615,13.7571590105316,
131.893825492125)) ;
#124987=CARTESIAN_POINT('Ctrl Pts',(-14.9371721138493,13.4483332581187,
131.844421725102)) ;
#124988=CARTESIAN_POINT('Ctrl Pts',(-14.9584157245602,13.140610392606,131.873559202715)) ;
#124989=CARTESIAN_POINT('Ctrl Pts',(-15.006332152192,12.8492377200964,131.980169977206)) ;
#124990=CARTESIAN_POINT('Ctrl Pts',(-15.0773325730432,12.6021186062381,
132.154566622699)) ;
#124991=CARTESIAN_POINT('Ctrl Pts',(-15.1672005368303,12.4130744443633,
132.384082222969)) ;
#124992=CARTESIAN_POINT('Ctrl Pts',(-15.2714613998002,12.2953575363629,
132.655337022259)) ;
#124993=CARTESIAN_POINT('Ctrl Pts',(-15.3815448297722,12.259540004683,132.943880410845)) ;
#124994=CARTESIAN_POINT('Ctrl Pts',(-15.4912456386987,12.3063152851138,
133.231278361687)) ;
#124995=CARTESIAN_POINT('Ctrl Pts',(-15.5939663384943,12.4341408318063,
133.498072171221)) ;
#124996=CARTESIAN_POINT('Ctrl Pts',(-15.6816501279818,12.6316134862806,
133.721213083362)) ;
#124997=CARTESIAN_POINT('Ctrl Pts',(-15.7499030351048,12.8861350461837,
133.887481728305)) ;
#124998=CARTESIAN_POINT('Ctrl Pts',(-15.7942059688853,13.179213941093,133.98378356009)) ;
#124999=CARTESIAN_POINT('Ctrl Pts',(-15.8121296747286,13.4905687882747,
134.002938802132)) ;
#125000=CARTESIAN_POINT('Ctrl Pts',(-15.8029511716908,13.7964604527636,
133.942985156857)) ;
#125001=CARTESIAN_POINT('Ctrl Pts',(-15.7684329938962,14.0743848720617,
133.809160750471)) ;
#125002=CARTESIAN_POINT('Ctrl Pts',(-15.7114766984834,14.3070163090694,
133.609649645911)) ;
#125003=CARTESIAN_POINT('Ctrl Pts',(-15.6367201521411,14.4764518819419,
133.358067464935)) ;
#125004=CARTESIAN_POINT('Ctrl Pts',(-15.550868483393,14.5698501931718,133.074231883872)) ;
#125005=CARTESIAN_POINT('Ctrl Pts',(-15.4601765122184,14.5816111155488,
132.776162534956)) ;
#125006=CARTESIAN_POINT('Ctrl Pts',(-15.3718833098534,14.5098991366122,
132.48501685371)) ;
#125007=CARTESIAN_POINT('Ctrl Pts',(-15.2934983361019,14.3604029768198,
132.222904357616)) ;
#125008=CARTESIAN_POINT('Ctrl Pts',(-15.2311225152342,14.1435656071336,
132.007535897725)) ;
#125009=CARTESIAN_POINT('Ctrl Pts',(-15.1900514509045,13.8762645151226,
131.854539360844)) ;
#125010=CARTESIAN_POINT('Ctrl Pts',(-15.173721426937,13.5746433207973,131.77359639711)) ;
#125011=CARTESIAN_POINT('Ctrl Pts',(-15.1841222852425,13.2647985797715,
131.771035600231)) ;
#125012=CARTESIAN_POINT('Ctrl Pts',(-15.2213411645311,12.9638355607027,
131.846545765161)) ;
#125013=CARTESIAN_POINT('Ctrl Pts',(-15.2833515972968,12.6967406329269,
131.994582271641)) ;
#125014=CARTESIAN_POINT('Ctrl Pts',(-15.3664540430693,12.4815166817384,
132.204216153634)) ;
#125015=CARTESIAN_POINT('Ctrl Pts',(-15.465420080429,12.3337893264045,132.460199514638)) ;
#125016=CARTESIAN_POINT('Ctrl Pts',(-15.5739645042299,12.2640797848313,
132.744142825912)) ;
#125017=CARTESIAN_POINT('Ctrl Pts',(-15.6847782481481,12.2774691635847,
133.034771337634)) ;
#125018=CARTESIAN_POINT('Ctrl Pts',(-15.7908127641154,12.3724670755757,
133.311459425319)) ;
#125019=CARTESIAN_POINT('Ctrl Pts',(-15.8857243578106,12.5437674769879,
133.555469238688)) ;
#125020=CARTESIAN_POINT('Ctrl Pts',(-15.9622886843345,12.7765747381498,
133.746136071001)) ;
#125021=CARTESIAN_POINT('Ctrl Pts',(-16.0168222647185,13.056442748956,133.872306944188)) ;
#125022=CARTESIAN_POINT('Ctrl Pts',(-16.0456475901748,13.3632374806636,
133.923318739201)) ;
#125023=CARTESIAN_POINT('Ctrl Pts',(-16.0475237873609,13.6730055446753,
133.895754018573)) ;
#125024=CARTESIAN_POINT('Ctrl Pts',(-16.0227887843929,13.9671153512335,
133.790179973524)) ;
#125025=CARTESIAN_POINT('Ctrl Pts',(-15.9745831485738,14.2192391234479,
133.616422532478)) ;
#125026=CARTESIAN_POINT('Ctrl Pts',(-15.9062934997798,14.4164802375927,
133.3837039056)) ;
#125027=CARTESIAN_POINT('Ctrl Pts',(-15.8242106414318,14.5415580398573,
133.110853663732)) ;
#125028=CARTESIAN_POINT('Ctrl Pts',(-15.7345851181313,14.5869148378636,
132.815919319322)) ;
#125029=CARTESIAN_POINT('Ctrl Pts',(-15.6446503042506,14.549009953407,132.520094917807)) ;
#125030=CARTESIAN_POINT('Ctrl Pts',(-15.5613259222977,14.4299835709606,
132.243476421726)) ;
#125031=CARTESIAN_POINT('Ctrl Pts',(-15.4918978635437,14.2395160277486,
132.007608598271)) ;
#125032=CARTESIAN_POINT('Ctrl Pts',(-15.441493990576,13.9900850952094,131.827215612351)) ;
#125033=CARTESIAN_POINT('Ctrl Pts',(-15.4147523737952,13.7002631098511,
131.715984820068)) ;
#125034=CARTESIAN_POINT('Ctrl Pts',(-15.4141848692343,13.3906063370585,
131.681212767504)) ;
#125035=CARTESIAN_POINT('Ctrl Pts',(-15.4406987166013,13.0826197342829,
131.725480875401)) ;
#125036=CARTESIAN_POINT('Ctrl Pts',(-15.4929987863392,12.7997480934514,
131.845153004214)) ;
#125037=CARTESIAN_POINT('Ctrl Pts',(-15.5680380099016,12.5614902723847,
132.031257977271)) ;
#125038=CARTESIAN_POINT('Ctrl Pts',(-15.6613888907222,12.3846250062646,
132.270799254956)) ;
#125039=CARTESIAN_POINT('Ctrl Pts',(-15.7668964947916,12.2824687795427,
132.545876098705)) ;
#125040=CARTESIAN_POINT('Ctrl Pts',(-15.8774268513273,12.2619556367439,
132.835724393864)) ;
#125041=CARTESIAN_POINT('Ctrl Pts',(-15.9865462840208,12.3244285368361,
133.121329823739)) ;
#125042=CARTESIAN_POINT('Ctrl Pts',(-16.0868856191326,12.4664340564494,
133.381215648153)) ;
#125043=CARTESIAN_POINT('Ctrl Pts',(-16.1711609881106,12.6753487848156,
133.594444113081)) ;
#125044=CARTESIAN_POINT('Ctrl Pts',(-16.2352956880658,12.9390315175275,
133.748624282027)) ;
#125045=CARTESIAN_POINT('Ctrl Pts',(-16.274758335238,13.2369183961831,133.830804549625)) ;
#125046=CARTESIAN_POINT('Ctrl Pts',(-16.2875416134419,13.5497744886041,
133.834864948315)) ;
#125047=CARTESIAN_POINT('Ctrl Pts',(-16.27350948019,13.8506095454533,133.76092084741)) ;
#125048=CARTESIAN_POINT('Ctrl Pts',(-16.2343148511589,14.1229210683533,
133.613234990865)) ;
#125049=CARTESIAN_POINT('Ctrl Pts',(-16.1736950386534,14.3440341407498,
133.403097622042)) ;
#125050=CARTESIAN_POINT('Ctrl Pts',(-16.0964629275866,14.5000650906738,
133.144340925564)) ;
#125051=CARTESIAN_POINT('Ctrl Pts',(-16.0085177153032,14.5786444747034,
132.854136319792)) ;
#125052=CARTESIAN_POINT('Ctrl Pts',(-15.9184051398423,14.5743811476286,
132.557997834982)) ;
#125053=CARTESIAN_POINT('Ctrl Pts',(-15.8311646501359,14.4873598311618,
132.269835416294)) ;
#125054=CARTESIAN_POINT('Ctrl Pts',(-15.7554385199139,14.3240886154077,
132.015513010405)) ;
#125055=CARTESIAN_POINT('Ctrl Pts',(-15.6968978333521,14.0972552260208,
131.811480466257)) ;
#125056=CARTESIAN_POINT('Ctrl Pts',(-15.660121717312,13.8219066558181,131.670965445006)) ;
#125057=CARTESIAN_POINT('Ctrl Pts',(-15.6487014566343,13.516025574875,131.604313184565)) ;
#125058=CARTESIAN_POINT('Ctrl Pts',(-15.6643812999087,13.2050736952722,
131.617003925741)) ;
#125059=CARTESIAN_POINT('Ctrl Pts',(-15.7063207684821,12.9106473531297,
131.706512006777)) ;
#125060=CARTESIAN_POINT('Ctrl Pts',(-15.7725855680298,12.6518068036689,
131.866967709783)) ;
#125061=CARTESIAN_POINT('Ctrl Pts',(-15.8591726098178,12.4481718276841,
132.086764482203)) ;
#125062=CARTESIAN_POINT('Ctrl Pts',(-15.9604476025779,12.3143466020562,
132.349489674931)) ;
#125063=CARTESIAN_POINT('Ctrl Pts',(-16.0704199585515,12.2602411283263,
132.637481151036)) ;
#125064=CARTESIAN_POINT('Ctrl Pts',(-16.180142994227,12.289044221804,132.925153256942)) ;
#125065=CARTESIAN_POINT('Ctrl Pts',(-16.2851832841205,12.3996399121577,
133.19871199035)) ;
#125066=CARTESIAN_POINT('Ctrl Pts',(-16.3765661818685,12.5827969137066,
133.432639291923)) ;
#125067=CARTESIAN_POINT('Ctrl Pts',(-16.4496897001009,12.8269629913892,
133.613061201054)) ;
#125068=CARTESIAN_POINT('Ctrl Pts',(-16.4993504127323,13.1127056194501,
133.725096180988)) ;
#125069=CARTESIAN_POINT('Ctrl Pts',(-16.5231792047334,13.4217118754633,
133.761539786929)) ;
#125070=CARTESIAN_POINT('Ctrl Pts',(-16.5199738631592,13.7304251092952,
133.719063366019)) ;
#125071=CARTESIAN_POINT('Ctrl Pts',(-16.490503384238,14.0183443121755,133.599699786057)) ;
#125072=CARTESIAN_POINT('Ctrl Pts',(-16.4381141934094,14.2615012050008,
133.413650952144)) ;
#125073=CARTESIAN_POINT('Ctrl Pts',(-16.3669280545773,14.4455241702922,
133.172585659673)) ;
#125074=CARTESIAN_POINT('Ctrl Pts',(-16.2829194787264,14.5564730573808,
132.894096731923)) ;
#125075=CARTESIAN_POINT('Ctrl Pts',(-16.1921044498383,14.5860332568258,
132.59547783415)) ;
#125076=CARTESIAN_POINT('Ctrl Pts',(-16.103500275386,14.5327319791753,132.303757320234)) ;
#125077=CARTESIAN_POINT('Ctrl Pts',(-16.0219268181338,14.3988254927601,
132.032121654547)) ;
#125078=CARTESIAN_POINT('Ctrl Pts',(-15.9559637229476,14.1966329256883,
131.806478335606)) ;
#125079=CARTESIAN_POINT('Ctrl Pts',(-15.9096631410881,13.9381994026002,
131.638070209423)) ;
#125080=CARTESIAN_POINT('Ctrl Pts',(-15.8876877659076,13.6421506980583,
131.540674271844)) ;
#125081=CARTESIAN_POINT('Ctrl Pts',(-15.892259652353,13.3319747136995,131.520994310315)) ;
#125082=CARTESIAN_POINT('Ctrl Pts',(-15.9236182041974,13.0275240722509,
131.579488272079)) ;
#125083=CARTESIAN_POINT('Ctrl Pts',(-15.9808594345229,12.7499512402199,
131.71339289058)) ;
#125084=CARTESIAN_POINT('Ctrl Pts',(-16.0595419330876,12.5230805349149,
131.910248319882)) ;
#125085=CARTESIAN_POINT('Ctrl Pts',(-16.1555190707494,12.3595163071095,
132.1575039903)) ;
#125086=CARTESIAN_POINT('Ctrl Pts',(-16.2628242846162,12.2720600916224,
132.437756364617)) ;
#125087=CARTESIAN_POINT('Ctrl Pts',(-16.3739355148782,12.2676665525214,
132.729189014784)) ;
#125088=CARTESIAN_POINT('Ctrl Pts',(-16.4811396900132,12.3451448696153,
133.009429281113)) ;
#125089=CARTESIAN_POINT('Ctrl Pts',(-16.5790070302067,12.5004783202174,
133.26212619254)) ;
#125090=CARTESIAN_POINT('Ctrl Pts',(-16.6600475484308,12.7212078449696,
133.465811461035)) ;
#125091=CARTESIAN_POINT('Ctrl Pts',(-16.7198827149784,12.9936146304865,
133.607363218945)) ;
#125092=CARTESIAN_POINT('Ctrl Pts',(-16.754273605641,13.2947838231295,133.67482792291)) ;
#125093=CARTESIAN_POINT('Ctrl Pts',(-16.7620692032191,13.6064069014527,
133.664452435759)) ;
#125094=CARTESIAN_POINT('Ctrl Pts',(-16.7430907146308,13.9050218268895,
133.575849688899)) ;
#125095=CARTESIAN_POINT('Ctrl Pts',(-16.6995705306357,14.1686337353897,
133.415605636576)) ;
#125096=CARTESIAN_POINT('Ctrl Pts',(-16.6353883774132,14.3788183161701,
133.195021357759)) ;
#125097=CARTESIAN_POINT('Ctrl Pts',(-16.5557065457281,14.520866298431,132.929111709198)) ;
#125098=CARTESIAN_POINT('Ctrl Pts',(-16.4669529903276,14.5841620003351,
132.636672229951)) ;
#125099=CARTESIAN_POINT('Ctrl Pts',(-16.3764933029576,14.5641966090762,
132.339316751059)) ;
#125100=CARTESIAN_POINT('Ctrl Pts',(-16.2912541780602,14.4625801801971,
132.057180085173)) ;
#125101=CARTESIAN_POINT('Ctrl Pts',(-16.2180694744256,14.2860054922745,
131.810200069221)) ;
#125102=CARTESIAN_POINT('Ctrl Pts',(-16.1632868666625,14.0484511491475,
131.617113761597)) ;
#125103=CARTESIAN_POINT('Ctrl Pts',(-16.1310808580205,13.7663469405247,
131.48997210374)) ;
#125104=CARTESIAN_POINT('Ctrl Pts',(-16.1247064234406,13.4574607709576,
131.438056091553)) ;
#125105=CARTESIAN_POINT('Ctrl Pts',(-16.1452962590473,13.1488899250601,
131.465215238141)) ;
#125106=CARTESIAN_POINT('Ctrl Pts',(-16.1921499049796,12.8583365008137,
131.568923429512)) ;
#125107=CARTESIAN_POINT('Ctrl Pts',(-16.2627019723822,12.6085157648157,
131.741877002118)) ;
#125108=CARTESIAN_POINT('Ctrl Pts',(-16.3523422100756,12.4173946912655,
131.970658735821)) ;
#125109=CARTESIAN_POINT('Ctrl Pts',(-16.4557143149458,12.2980452527152,
132.239501066131)) ;
#125110=CARTESIAN_POINT('Ctrl Pts',(-16.5657958992365,12.2592457777712,
132.528006891345)) ;
#125111=CARTESIAN_POINT('Ctrl Pts',(-16.6761302057644,12.3040208605449,
132.817096151529)) ;
#125112=CARTESIAN_POINT('Ctrl Pts',(-16.7784620002637,12.4286939369855,
133.082985219044)) ;
#125113=CARTESIAN_POINT('Ctrl Pts',(-16.8670042340399,12.6243590090332,
133.308543332453)) ;
#125114=CARTESIAN_POINT('Ctrl Pts',(-16.9362046600572,12.8789083522399,
133.477410666535)) ;
#125115=CARTESIAN_POINT('Ctrl Pts',(-16.981013129791,13.1702261318585,133.575303882571)) ;
#125116=CARTESIAN_POINT('Ctrl Pts',(-16.9997593267908,13.4805037318096,
133.596949956385)) ;
#125117=CARTESIAN_POINT('Ctrl Pts',(-16.9914405859225,13.7876511812746,
133.539432418538)) ;
#125118=CARTESIAN_POINT('Ctrl Pts',(-16.9573735315458,14.0678452982214,
133.406766511356)) ;
#125119=CARTESIAN_POINT('Ctrl Pts',(-16.9012614485024,14.3007432991358,
133.209897343)) ;
#125120=CARTESIAN_POINT('Ctrl Pts',(-16.8268882457025,14.472578666663,132.959393972783)) ;
#125121=CARTESIAN_POINT('Ctrl Pts',(-16.7412612448846,14.5682598997855,
132.676214692444)) ;
#125122=CARTESIAN_POINT('Ctrl Pts',(-16.6506173444698,14.5824152858443,
132.378287771747)) ;
#125123=CARTESIAN_POINT('Ctrl Pts',(-16.5622810767315,14.5133614382036,
132.087075773177)) ;
#125124=CARTESIAN_POINT('Ctrl Pts',(-16.4833786073322,14.3656854854221,
131.823382600048)) ;
#125125=CARTESIAN_POINT('Ctrl Pts',(-16.4206953534256,14.1519222579812,
131.60728783786)) ;
#125126=CARTESIAN_POINT('Ctrl Pts',(-16.378605818651,13.8839964820202,131.451069851381)) ;
#125127=CARTESIAN_POINT('Ctrl Pts',(-16.3616265485276,13.5839684953717,
131.368347064637)) ;
#125128=CARTESIAN_POINT('Ctrl Pts',(-16.3712407110028,13.2736209953703,
131.363427796788)) ;
#125129=CARTESIAN_POINT('Ctrl Pts',(-16.4075816986682,12.9727615411734,
131.436462345173)) ;
#125130=CARTESIAN_POINT('Ctrl Pts',(-16.4691084518117,12.7034620049653,
131.582968291489)) ;
#125131=CARTESIAN_POINT('Ctrl Pts',(-16.5516508067842,12.4867211493109,
131.790989127946)) ;
#125132=CARTESIAN_POINT('Ctrl Pts',(-16.6503484981561,12.3368636809282,
132.046157336608)) ;
#125133=CARTESIAN_POINT('Ctrl Pts',(-16.7583562953978,12.2650346838616,
132.328642824857)) ;
#125134=CARTESIAN_POINT('Ctrl Pts',(-16.8694876280613,12.2758062745913,
132.620115626391)) ;
#125135=CARTESIAN_POINT('Ctrl Pts',(-16.9761391690963,12.3692807546481,
132.898474485446)) ;
#125136=CARTESIAN_POINT('Ctrl Pts',(-17.0709660600708,12.5378929706017,
133.142402959768)) ;
#125137=CARTESIAN_POINT('Ctrl Pts',(-17.1482588531112,12.7694277831183,
133.335140705917)) ;
#125138=CARTESIAN_POINT('Ctrl Pts',(-17.203480116346,13.0484836383152,133.463302136376)) ;
#125139=CARTESIAN_POINT('Ctrl Pts',(-17.2330309055993,13.3553252345684,
133.516383957086)) ;
#125140=CARTESIAN_POINT('Ctrl Pts',(-17.2355770259433,13.6640556396721,
133.490901219807)) ;
#125141=CARTESIAN_POINT('Ctrl Pts',(-17.2118345762843,13.9577070644724,
133.38838860845)) ;
#125142=CARTESIAN_POINT('Ctrl Pts',(-17.1640544883737,14.2128779960594,
133.215679321086)) ;
#125143=CARTESIAN_POINT('Ctrl Pts',(-17.0962318726985,14.4117544272494,
132.984335525429)) ;
#125144=CARTESIAN_POINT('Ctrl Pts',(-17.0145165993263,14.5391283033453,
132.712572701399)) ;
#125145=CARTESIAN_POINT('Ctrl Pts',(-16.9245932202189,14.5867879380275,
132.416618791262)) ;
#125146=CARTESIAN_POINT('Ctrl Pts',(-16.8350007935137,14.5512051546367,
132.121952756565)) ;
#125147=CARTESIAN_POINT('Ctrl Pts',(-16.7512399326396,14.4343419889086,
131.844006100408)) ;
#125148=CARTESIAN_POINT('Ctrl Pts',(-16.6813663736858,14.2455278937518,
131.606828317341)) ;
#125149=CARTESIAN_POINT('Ctrl Pts',(-16.6304533077385,13.9981929158514,
131.425029652249)) ;
#125150=CARTESIAN_POINT('Ctrl Pts',(-16.6029110965595,13.7085066698523,
131.311373710203)) ;
#125151=CARTESIAN_POINT('Ctrl Pts',(-16.6016472246784,13.3995793870564,
131.274618331211)) ;
#125152=CARTESIAN_POINT('Ctrl Pts',(-16.6272259405872,13.0919774585784,
131.316244261262)) ;
#125153=CARTESIAN_POINT('Ctrl Pts',(-16.6790956075483,12.8067303604848,
131.434491745221)) ;
#125154=CARTESIAN_POINT('Ctrl Pts',(-16.7531642097008,12.5682008646981,
131.617936014673)) ;
#125155=CARTESIAN_POINT('Ctrl Pts',(-16.846195785703,12.3888212047449,131.85647832136)) ;
#125156=CARTESIAN_POINT('Ctrl Pts',(-16.9512994964481,12.2844119375082,
132.130420874405)) ;
#125157=CARTESIAN_POINT('Ctrl Pts',(-17.0621203595401,12.2613333969067,
132.421013195999)) ;
#125158=CARTESIAN_POINT('Ctrl Pts',(-17.1712584780037,12.3215794743214,
132.706710232666)) ;
#125159=CARTESIAN_POINT('Ctrl Pts',(-17.2716303151699,12.4606919481936,
132.966808168993)) ;
#125160=CARTESIAN_POINT('Ctrl Pts',(-17.3568271309369,12.6684214506416,
133.182599772503)) ;
#125161=CARTESIAN_POINT('Ctrl Pts',(-17.4217613046076,12.9319196123432,
133.339000010842)) ;
#125162=CARTESIAN_POINT('Ctrl Pts',(-17.4617001910976,13.2279083302756,
133.42271072074)) ;
#125163=CARTESIAN_POINT('Ctrl Pts',(-17.4753487897358,13.5392234184095,
133.429453311327)) ;
#125164=CARTESIAN_POINT('Ctrl Pts',(-17.462103295986,13.8421684111979,133.357645852584)) ;
#125165=CARTESIAN_POINT('Ctrl Pts',(-17.4235361943751,14.1158321070144,
133.211769875002)) ;
#125166=CARTESIAN_POINT('Ctrl Pts',(-17.363322316069,14.339009376798,133.002750514916)) ;
#125167=CARTESIAN_POINT('Ctrl Pts',(-17.2866062600397,14.4964746049257,
132.745573553595)) ;
#125168=CARTESIAN_POINT('Ctrl Pts',(-17.199397296313,14.5773715889881,132.457710585118)) ;
#125169=CARTESIAN_POINT('Ctrl Pts',(-17.1085822658646,14.5757025147149,
132.159265391924)) ;
#125170=CARTESIAN_POINT('Ctrl Pts',(-17.0213774045602,14.490867072331,131.871293001474)) ;
#125171=CARTESIAN_POINT('Ctrl Pts',(-16.9454927949128,14.330592253299,131.616635348384)) ;
#125172=CARTESIAN_POINT('Ctrl Pts',(-16.8860651829023,14.1048089901007,
131.409889551505)) ;
#125173=CARTESIAN_POINT('Ctrl Pts',(-16.84857731132,13.8293690778141,131.267169165395)) ;
#125174=CARTESIAN_POINT('Ctrl Pts',(-16.8364706813943,13.526576284789,131.198790499997)) ;
#125175=CARTESIAN_POINT('Ctrl Pts',(-16.8512333940757,13.2147294294983,
131.208717499866)) ;
#125176=CARTESIAN_POINT('Ctrl Pts',(-16.8924752507082,12.9189024654219,
131.296126903513)) ;
#125177=CARTESIAN_POINT('Ctrl Pts',(-16.9583514927503,12.6580299108607,
131.455339791763)) ;
#125178=CARTESIAN_POINT('Ctrl Pts',(-17.044063698862,12.4534345481142,131.672724444165)) ;
#125179=CARTESIAN_POINT('Ctrl Pts',(-17.1452480350567,12.3171076600088,
131.935097166867)) ;
#125180=CARTESIAN_POINT('Ctrl Pts',(-17.2545016602799,12.2606844017973,
132.221165652428)) ;
#125181=CARTESIAN_POINT('Ctrl Pts',(-17.3650975011876,12.2870889602567,
132.511145676812)) ;
#125182=CARTESIAN_POINT('Ctrl Pts',(-17.4703391463682,12.3957983185939,
132.785305386783)) ;
#125183=CARTESIAN_POINT('Ctrl Pts',(-17.5619519450176,12.576725714127,133.019970693794)) ;
#125184=CARTESIAN_POINT('Ctrl Pts',(-17.6355785374756,12.8186993235838,
133.201938865071)) ;
#125185=CARTESIAN_POINT('Ctrl Pts',(-17.686204034739,13.1050418168408,133.316613415552)) ;
#125186=CARTESIAN_POINT('Ctrl Pts',(-17.7106472500127,13.4130762749516,
133.354929376056)) ;
#125187=CARTESIAN_POINT('Ctrl Pts',(-17.708198005418,13.7214651862128,133.314720701507)) ;
#125188=CARTESIAN_POINT('Ctrl Pts',(-17.6797043677166,14.0093161749257,
133.198352418862)) ;
#125189=CARTESIAN_POINT('Ctrl Pts',(-17.6275067830574,14.2560736746896,
133.012580543426)) ;
#125190=CARTESIAN_POINT('Ctrl Pts',(-17.5569227810102,14.4412184365536,
132.773378196759)) ;
#125191=CARTESIAN_POINT('Ctrl Pts',(-17.47320903247,14.5543182537731,132.495749100207)) ;
#125192=CARTESIAN_POINT('Ctrl Pts',(-17.3828982361184,14.5864671229327,
132.198763951724)) ;
#125193=CARTESIAN_POINT('Ctrl Pts',(-17.2935482114435,14.5351930359694,
131.904630245163)) ;
#125194=CARTESIAN_POINT('Ctrl Pts',(-17.212146566953,14.4042256510203,131.633704988442)) ;
#125195=CARTESIAN_POINT('Ctrl Pts',(-17.1453646293854,14.2033619799806,
131.405542254505)) ;
#125196=CARTESIAN_POINT('Ctrl Pts',(-17.0984468920315,13.9460942692561,
131.235324126716)) ;
#125197=CARTESIAN_POINT('Ctrl Pts',(-17.0757509849467,13.6510939576202,
131.135850406364)) ;
#125198=CARTESIAN_POINT('Ctrl Pts',(-17.0795112397246,13.3409631929891,
131.113791894958)) ;
#125199=CARTESIAN_POINT('Ctrl Pts',(-17.1102336251651,13.0355468372364,
131.170367824082)) ;
#125200=CARTESIAN_POINT('Ctrl Pts',(-17.1663842613516,12.7584809477333,
131.301291574706)) ;
#125201=CARTESIAN_POINT('Ctrl Pts',(-17.2447371033767,12.5287898024968,
131.497044500039)) ;
#125202=CARTESIAN_POINT('Ctrl Pts',(-17.3403102773083,12.3633456659364,
131.743129508113)) ;
#125203=CARTESIAN_POINT('Ctrl Pts',(-17.4470084964624,12.2737023197767,
132.021718516189)) ;
#125204=CARTESIAN_POINT('Ctrl Pts',(-17.5581425262806,12.2663504667095,
132.31320916941)) ;
#125205=CARTESIAN_POINT('Ctrl Pts',(-17.6662007298593,12.34208017502,132.595736728779)) ;
#125206=CARTESIAN_POINT('Ctrl Pts',(-17.7639779601898,12.4946576903152,
132.848330696143)) ;
#125207=CARTESIAN_POINT('Ctrl Pts',(-17.845869332575,12.7142650578431,133.054392423635)) ;
#125208=CARTESIAN_POINT('Ctrl Pts',(-17.9062976280735,12.9853995961956,
133.197700199445)) ;
#125209=CARTESIAN_POINT('Ctrl Pts',(-17.9414670577148,13.2860375673385,
133.267430288951)) ;
#125210=CARTESIAN_POINT('Ctrl Pts',(-17.9500100804759,13.5985523264733,
133.259150343869)) ;
#125211=CARTESIAN_POINT('Ctrl Pts',(-17.9316672579666,13.8975129640997,
133.17242792376)) ;
#125212=CARTESIAN_POINT('Ctrl Pts',(-17.8890068524942,14.1612607305214,
133.014839223972)) ;
#125213=CARTESIAN_POINT('Ctrl Pts',(-17.8252095466582,14.3739608986485,
132.795283644914)) ;
#125214=CARTESIAN_POINT('Ctrl Pts',(-17.745594810308,14.5182947311408,132.529471937836)) ;
#125215=CARTESIAN_POINT('Ctrl Pts',(-17.6571488015363,14.5834512891337,
132.23799331013)) ;
#125216=CARTESIAN_POINT('Ctrl Pts',(-17.5669390064096,14.5659482056826,
131.94147536579)) ;
#125217=CARTESIAN_POINT('Ctrl Pts',(-17.4814696878511,14.4667697468738,
131.65867637402)) ;
#125218=CARTESIAN_POINT('Ctrl Pts',(-17.4077725179851,14.2923285358451,
131.410191086964)) ;
#125219=CARTESIAN_POINT('Ctrl Pts',(-17.3521425033157,14.0548140143778,
131.21443926717)) ;
#125220=CARTESIAN_POINT('Ctrl Pts',(-17.3195158312481,13.7751053966171,
131.086247525205)) ;
#125221=CARTESIAN_POINT('Ctrl Pts',(-17.312239483779,13.4671706685235,131.031747960473)) ;
#125222=CARTESIAN_POINT('Ctrl Pts',(-17.3322332196275,13.1566326629542,
131.056977756949)) ;
#125223=CARTESIAN_POINT('Ctrl Pts',(-17.3780975395808,12.8670308580196,
131.158001609314)) ;
#125224=CARTESIAN_POINT('Ctrl Pts',(-17.4482094790245,12.614625742012,131.329541047974)) ;
#125225=CARTESIAN_POINT('Ctrl Pts',(-17.5375995577901,12.4216271710516,
131.557537586871)) ;
#125226=CARTESIAN_POINT('Ctrl Pts',(-17.6401822990097,12.3004936351809,
131.824227815252)) ;
#125227=CARTESIAN_POINT('Ctrl Pts',(-17.7507907280733,12.2591976942699,
132.114082356459)) ;
#125228=CARTESIAN_POINT('Ctrl Pts',(-17.8604775826945,12.3014766458867,
132.401506605415)) ;
#125229=CARTESIAN_POINT('Ctrl Pts',(-17.9633872935851,12.4236752425343,
132.669020376417)) ;
#125230=CARTESIAN_POINT('Ctrl Pts',(-18.0529404696377,12.6191375618547,
132.897304914097)) ;
#125231=CARTESIAN_POINT('Ctrl Pts',(-18.1222475619153,12.8707902517674,
133.066702627176)) ;
#125232=CARTESIAN_POINT('Ctrl Pts',(-18.1679096652003,13.1617413465553,
133.167025713482)) ;
#125233=CARTESIAN_POINT('Ctrl Pts',(-18.1873626654556,13.4713353015044,
133.190791441837)) ;
#125234=CARTESIAN_POINT('Ctrl Pts',(-18.1798609889004,13.7785022490456,
133.135703081782)) ;
#125235=CARTESIAN_POINT('Ctrl Pts',(-18.1466211271099,14.0596469751513,
133.005485313342)) ;
#125236=CARTESIAN_POINT('Ctrl Pts',(-18.0908146756498,14.2953142931135,
132.80933989071)) ;
#125237=CARTESIAN_POINT('Ctrl Pts',(-18.0168560810249,14.468964761841,132.560061748028)) ;
#125238=CARTESIAN_POINT('Ctrl Pts',(-17.9311937335186,14.566840747798,132.276680512061)) ;
#125239=CARTESIAN_POINT('Ctrl Pts',(-17.8410327874371,14.5831863557758,
131.980333879477)) ;
#125240=CARTESIAN_POINT('Ctrl Pts',(-17.7521647268769,14.5160478882273,
131.687421881803)) ;
#125241=CARTESIAN_POINT('Ctrl Pts',(-17.6733234585166,14.3710572999732,
131.424079417212)) ;
#125242=CARTESIAN_POINT('Ctrl Pts',(-17.6099533809622,14.1586831437498,
131.205906158547)) ;
#125243=CARTESIAN_POINT('Ctrl Pts',(-17.567311041449,13.8924167167611,131.04813455033)) ;
#125244=CARTESIAN_POINT('Ctrl Pts',(-17.5495214646108,13.5934589593166,
130.963081615833)) ;
#125245=CARTESIAN_POINT('Ctrl Pts',(-17.5583972008256,13.2817948443867,
130.95586528545)) ;
#125246=CARTESIAN_POINT('Ctrl Pts',(-17.5940640660166,12.9807519837477,
131.02696560632)) ;
#125247=CARTESIAN_POINT('Ctrl Pts',(-17.6545564421108,12.7114087835464,
131.170609668857)) ;
#125248=CARTESIAN_POINT('Ctrl Pts',(-17.7368226999729,12.4920355070178,
131.377698689643)) ;
#125249=CARTESIAN_POINT('Ctrl Pts',(-17.8348724901337,12.340409192469,131.631065455317)) ;
#125250=CARTESIAN_POINT('Ctrl Pts',(-17.9430670356921,12.2658594126602,
131.913978129015)) ;
#125251=CARTESIAN_POINT('Ctrl Pts',(-18.054069728851,12.2744067953506,132.205121446175)) ;
#125252=CARTESIAN_POINT('Ctrl Pts',(-18.1606637543709,12.3651074088565,
132.483406049134)) ;
#125253=CARTESIAN_POINT('Ctrl Pts',(-18.2560924961007,12.5316553295761,
132.729048365178)) ;
#125254=CARTESIAN_POINT('Ctrl Pts',(-18.3341778607555,12.7621962066438,
132.924014416432)) ;
#125255=CARTESIAN_POINT('Ctrl Pts',(-18.3899839397294,13.0400249877383,
133.0539094655)) ;
#125256=CARTESIAN_POINT('Ctrl Pts',(-18.4202910006776,13.3449925663018,
133.109347316149)) ;
#125257=CARTESIAN_POINT('Ctrl Pts',(-18.4236631714754,13.6560824874518,
133.086042456464)) ;
#125258=CARTESIAN_POINT('Ctrl Pts',(-18.4006453620218,13.949523069505,132.98575486702)) ;
#125259=CARTESIAN_POINT('Ctrl Pts',(-18.3535646409171,14.2060602321428,
132.815095461345)) ;
#125260=CARTESIAN_POINT('Ctrl Pts',(-18.2862713344444,14.4068533843326,
132.585305948808)) ;
#125261=CARTESIAN_POINT('Ctrl Pts',(-18.2047737795013,14.5364834537221,
132.314136374667)) ;
#125262=CARTESIAN_POINT('Ctrl Pts',(-18.115348409199,14.5865952294226,132.019776237642)) ;
#125263=CARTESIAN_POINT('Ctrl Pts',(-18.0251839000944,14.5532896916384,
131.723255892366)) ;
#125264=CARTESIAN_POINT('Ctrl Pts',(-17.9415200376328,14.4391769961996,
131.445750322776)) ;
#125265=CARTESIAN_POINT('Ctrl Pts',(-17.8709865879843,14.2521193934998,
131.206572721742)) ;
#125266=CARTESIAN_POINT('Ctrl Pts',(-17.8194372166682,14.0064610043906,
131.02293735799)) ;
#125267=CARTESIAN_POINT('Ctrl Pts',(-17.7910798255988,13.7162751862111,
130.906740249931)) ;
#125268=CARTESIAN_POINT('Ctrl Pts',(-17.789099001038,13.4088590372399,130.868028561726)) ;
#125269=CARTESIAN_POINT('Ctrl Pts',(-17.8139225822361,13.10053389726,130.907404974492)) ;
#125270=CARTESIAN_POINT('Ctrl Pts',(-17.8648392613618,12.8153801351655,
131.023001165044)) ;
#125271=CARTESIAN_POINT('Ctrl Pts',(-17.9384487251623,12.5742829301141,
131.20499722078)) ;
#125272=CARTESIAN_POINT('Ctrl Pts',(-18.031524743861,12.3924207645517,131.443517414331)) ;
#125273=CARTESIAN_POINT('Ctrl Pts',(-18.1358382897965,12.2864008460228,
131.715324149777)) ;
#125274=CARTESIAN_POINT('Ctrl Pts',(-18.2469528531772,12.2608494094795,
132.006664764433)) ;
#125275=CARTESIAN_POINT('Ctrl Pts',(-18.3557753142692,12.318610673207,132.291578909571)) ;
#125276=CARTESIAN_POINT('Ctrl Pts',(-18.4567104546273,12.4554523498405,
132.553270393945)) ;
#125277=CARTESIAN_POINT('Ctrl Pts',(-18.5427096959362,12.6626735869421,
132.771253835525)) ;
#125278=CARTESIAN_POINT('Ctrl Pts',(-18.6076529154857,12.9221026671482,
132.928024921922)) ;
#125279=CARTESIAN_POINT('Ctrl Pts',(-18.648750425879,13.2188659560216,133.014929938329)) ;
#125280=CARTESIAN_POINT('Ctrl Pts',(-18.6631067095924,13.5309970504502,
133.023649164472)) ;
#125281=CARTESIAN_POINT('Ctrl Pts',(-18.6506464875791,13.833391117926,132.954252667471)) ;
#125282=CARTESIAN_POINT('Ctrl Pts',(-18.612818085529,14.1082733327472,132.810534597262)) ;
#125283=CARTESIAN_POINT('Ctrl Pts',(-18.5531811994103,14.333273457915,132.603195859953)) ;
#125284=CARTESIAN_POINT('Ctrl Pts',(-18.4766889860136,14.493089968581,132.346598986185)) ;
#125285=CARTESIAN_POINT('Ctrl Pts',(-18.3897834881845,14.5762694878071,
132.059665220926)) ;
#125286=CARTESIAN_POINT('Ctrl Pts',(-18.2986311211206,14.5766426332955,
131.760103485388)) ;
#125287=CARTESIAN_POINT('Ctrl Pts',(-18.212007783448,14.4950561386841,131.474141881949)) ;
#125288=CARTESIAN_POINT('Ctrl Pts',(-18.1350292671629,14.3357812086937,
131.216006764261)) ;
#125289=CARTESIAN_POINT('Ctrl Pts',(-18.075283615151,14.1117725486506,131.008402983714)) ;
#125290=CARTESIAN_POINT('Ctrl Pts',(-18.0371145753747,13.8385111509001,
130.863796970643)) ;
#125291=CARTESIAN_POINT('Ctrl Pts',(-18.0242445077644,13.5338961508562,
130.792932325099)) ;
#125292=CARTESIAN_POINT('Ctrl Pts',(-18.038169338582,13.224257482388,130.800665239807)) ;
#125293=CARTESIAN_POINT('Ctrl Pts',(-18.0788682297641,12.9262818286679,
130.886318330355)) ;
#125294=CARTESIAN_POINT('Ctrl Pts',(-18.1436956382508,12.6654697880194,
131.042663175476)) ;
#125295=CARTESIAN_POINT('Ctrl Pts',(-18.2297053008849,12.4574145749278,
131.260611523241)) ;
#125296=CARTESIAN_POINT('Ctrl Pts',(-18.3295006899858,12.3205165370977,
131.519286625616)) ;
#125297=CARTESIAN_POINT('Ctrl Pts',(-18.4392025215922,12.2610390449612,
131.806469003895)) ;
#125298=CARTESIAN_POINT('Ctrl Pts',(-18.5495038928619,12.2851065235111,
132.095701138264)) ;
#125299=CARTESIAN_POINT('Ctrl Pts',(-18.6551377015888,12.3913707658575,
132.370972967707)) ;
#125300=CARTESIAN_POINT('Ctrl Pts',(-18.7473031876051,12.5705078939367,
132.607221974091)) ;
#125301=CARTESIAN_POINT('Ctrl Pts',(-18.8215355648859,12.8110531024917,
132.79094927383)) ;
#125302=CARTESIAN_POINT('Ctrl Pts',(-18.8728254696963,13.0958081066442,
132.907631481588)) ;
#125303=CARTESIAN_POINT('Ctrl Pts',(-18.8981142773173,13.4043791396556,
132.948317043376)) ;
#125304=CARTESIAN_POINT('Ctrl Pts',(-18.8964748240015,13.7127503611852,
132.91051808184)) ;
#125305=CARTESIAN_POINT('Ctrl Pts',(-18.8683636782998,14.0031465384866,
132.795046521471)) ;
#125306=CARTESIAN_POINT('Ctrl Pts',(-18.8174880240775,14.2480984869967,
132.613588092215)) ;
#125307=CARTESIAN_POINT('Ctrl Pts',(-18.7469572957245,14.4370589144751,
132.37428276721)) ;
#125308=CARTESIAN_POINT('Ctrl Pts',(-18.6635307918454,14.5521322480481,
132.097514975815)) ;
#125309=CARTESIAN_POINT('Ctrl Pts',(-18.5732136816833,14.5867077636068,
131.800472743053)) ;
#125310=CARTESIAN_POINT('Ctrl Pts',(-18.4839003383178,14.5378478925882,
131.506508305884)) ;
#125311=CARTESIAN_POINT('Ctrl Pts',(-18.402187454381,14.409203021957,131.234680849945)) ;
#125312=CARTESIAN_POINT('Ctrl Pts',(-18.334836902335,14.2102655044933,131.004850153329)) ;
#125313=CARTESIAN_POINT('Ctrl Pts',(-18.2871464008144,13.9531164546974,
130.83222870879)) ;
#125314=CARTESIAN_POINT('Ctrl Pts',(-18.2638580254884,13.6605444903127,
130.731214892336)) ;
#125315=CARTESIAN_POINT('Ctrl Pts',(-18.2668270499817,13.3493859295917,
130.706712302463)) ;
#125316=CARTESIAN_POINT('Ctrl Pts',(-18.2967304908482,13.0444134847032,
130.760998390813)) ;
#125317=CARTESIAN_POINT('Ctrl Pts',(-18.3522199844922,12.7658508385772,
130.889945672519)) ;
#125318=CARTESIAN_POINT('Ctrl Pts',(-18.4299598853039,12.5346698137633,
131.083926894411)) ;
#125319=CARTESIAN_POINT('Ctrl Pts',(-18.5252575613863,12.3668712653983,
131.32915520716)) ;
#125320=CARTESIAN_POINT('Ctrl Pts',(-18.6319362740028,12.2750736353354,
131.607631262067)) ;
#125321=CARTESIAN_POINT('Ctrl Pts',(-18.7424805338833,12.2654123935104,
131.897568237114)) ;
#125322=CARTESIAN_POINT('Ctrl Pts',(-18.8508042611965,12.3385001490515,
132.180853971329)) ;
#125323=CARTESIAN_POINT('Ctrl Pts',(-18.9492299885013,12.4893941605664,
132.435254667707)) ;
#125324=CARTESIAN_POINT('Ctrl Pts',(-19.0315407300344,12.7071836242874,
132.642573907651)) ;
#125325=CARTESIAN_POINT('Ctrl Pts',(-19.0925135202913,12.976008781698,132.787590925835)) ;
#125326=CARTESIAN_POINT('Ctrl Pts',(-19.1286176776364,13.2771672423765,
132.859921686262)) ;
#125327=CARTESIAN_POINT('Ctrl Pts',(-19.1379114672632,13.5885364783272,
132.853960762233)) ;
#125328=CARTESIAN_POINT('Ctrl Pts',(-19.1204771380458,13.8883475892356,
132.769887384823)) ;
#125329=CARTESIAN_POINT('Ctrl Pts',(-19.0782724812617,14.1546798103871,
132.613467494316)) ;
#125330=CARTESIAN_POINT('Ctrl Pts',(-19.0151377103599,14.3683945721778,
132.395937643212)) ;
#125331=CARTESIAN_POINT('Ctrl Pts',(-18.9362575078144,14.5146640723976,
132.132398804477)) ;
#125332=CARTESIAN_POINT('Ctrl Pts',(-18.8476989080688,14.5827891637854,
131.840476972232)) ;
#125333=CARTESIAN_POINT('Ctrl Pts',(-18.7572366847191,14.5676065821518,
131.543147243417)) ;
#125334=CARTESIAN_POINT('Ctrl Pts',(-18.6715544040139,14.4706130851543,
131.259732284729)) ;
#125335=CARTESIAN_POINT('Ctrl Pts',(-18.5976273893705,14.2987448591994,
131.010671404235)) ;
#125336=CARTESIAN_POINT('Ctrl Pts',(-18.5413330377305,14.063095759129,130.812986254615)) ;
#125337=CARTESIAN_POINT('Ctrl Pts',(-18.5078379421256,13.7833207941159,
130.682126791118)) ;
#125338=CARTESIAN_POINT('Ctrl Pts',(-18.4999097117007,13.4754882889809,
130.625692161167)) ;
#125339=CARTESIAN_POINT('Ctrl Pts',(-18.5189512412166,13.1664272505894,
130.648326923808)) ;
#125340=CARTESIAN_POINT('Ctrl Pts',(-18.5643283555043,12.8743475054809,
130.747739702902)) ;
#125341=CARTESIAN_POINT('Ctrl Pts',(-18.6334328686697,12.6220180592587,
130.916528129785)) ;
#125342=CARTESIAN_POINT('Ctrl Pts',(-18.7224073978982,12.4263341461984,
131.143243760147)) ;
#125343=CARTESIAN_POINT('Ctrl Pts',(-18.8252741733722,12.3026056592769,
131.410587938808)) ;
#125344=CARTESIAN_POINT('Ctrl Pts',(-18.9351163454627,12.2593725249827,
131.698402442325)) ;
#125345=CARTESIAN_POINT('Ctrl Pts',(-19.0450419186209,12.2987734012192,
131.986493383599)) ;
#125346=CARTESIAN_POINT('Ctrl Pts',(-19.1490013516762,12.4202091762236,
132.256809604344)) ;
#125347=CARTESIAN_POINT('Ctrl Pts',(-19.2380191086713,12.611773656706,132.483899442427)) ;
#125348=CARTESIAN_POINT('Ctrl Pts',(-19.3083453259853,12.8626551620978,
132.656143653974)) ;
#125349=CARTESIAN_POINT('Ctrl Pts',(-19.3547040728807,13.1527448434828,
132.758511459085)) ;
#125350=CARTESIAN_POINT('Ctrl Pts',(-19.3749834629373,13.4624298007765,
132.784654095395)) ;
#125351=CARTESIAN_POINT('Ctrl Pts',(-19.36820543525,13.7701811084813,132.731659693189)) ;
#125352=CARTESIAN_POINT('Ctrl Pts',(-19.3357421024822,14.0517728674994,
132.603778078472)) ;
#125353=CARTESIAN_POINT('Ctrl Pts',(-19.2805289193557,14.2892527094167,
132.40934630679)) ;
#125354=CARTESIAN_POINT('Ctrl Pts',(-19.2069909200465,14.4648240462418,
132.161293233759)) ;
#125355=CARTESIAN_POINT('Ctrl Pts',(-19.1218686179884,14.5650403206084,
131.879594398651)) ;
#125356=CARTESIAN_POINT('Ctrl Pts',(-19.031177665857,14.583748953291,131.581482686387)) ;
#125357=CARTESIAN_POINT('Ctrl Pts',(-18.9429516230396,14.5197167656378,
131.290759379113)) ;
#125358=CARTESIAN_POINT('Ctrl Pts',(-18.8631562519392,14.3763314306489,
131.024403462222)) ;
#125359=CARTESIAN_POINT('Ctrl Pts',(-18.7992959670841,14.1656644644825,
130.804814101691)) ;
#125360=CARTESIAN_POINT('Ctrl Pts',(-18.7559154993296,13.8999127599495,
130.644795322315)) ;
#125361=CARTESIAN_POINT('Ctrl Pts',(-18.7374861463171,13.6028234452547,
130.558011913804)) ;
#125362=CARTESIAN_POINT('Ctrl Pts',(-18.7455135996191,13.291184455058,130.548311267216)) ;
#125363=CARTESIAN_POINT('Ctrl Pts',(-18.78038027663,12.9894029525186,130.617067330366)) ;
#125364=CARTESIAN_POINT('Ctrl Pts',(-18.8404755456934,12.717765879006,130.759411419359)) ;
#125365=CARTESIAN_POINT('Ctrl Pts',(-18.9221464088355,12.4972589130398,
130.964811609339)) ;
#125366=CARTESIAN_POINT('Ctrl Pts',(-19.0195332489729,12.3438957008414,
131.216331735262)) ;
#125367=CARTESIAN_POINT('Ctrl Pts',(-19.1276333368959,12.2668705096983,
131.498935943536)) ;
#125368=CARTESIAN_POINT('Ctrl Pts',(-19.2385329213481,12.2729078297229,
131.789817260693)) ;
#125369=CARTESIAN_POINT('Ctrl Pts',(-19.3455156987851,12.3614501849398,
132.069182436036)) ;
#125370=CARTESIAN_POINT('Ctrl Pts',(-19.4411172478051,12.5253315667214,
132.315428252389)) ;
#125371=CARTESIAN_POINT('Ctrl Pts',(-19.5201398347916,12.7552771114224,
132.512976833561)) ;
#125372=CARTESIAN_POINT('Ctrl Pts',(-19.5764232616451,13.0310570491295,
132.644388654594)) ;
#125373=CARTESIAN_POINT('Ctrl Pts',(-19.6075743657055,13.3361218325012,
132.702220642329)) ;
#125374=CARTESIAN_POINT('Ctrl Pts',(-19.6117652558764,13.6463105662156,
132.681424980702)) ;
#125375=CARTESIAN_POINT('Ctrl Pts',(-19.5893821264966,13.9424874348681,
132.582777301933)) ;
#125376=CARTESIAN_POINT('Ctrl Pts',(-19.5427449303092,14.2002009461362,
132.413391756609)) ;
#125377=CARTESIAN_POINT('Ctrl Pts',(-19.4764078517587,14.4015262761072,
132.186614554798)) ;
#125378=CARTESIAN_POINT('Ctrl Pts',(-19.3950352335705,14.5339055048123,
131.915712480138)) ;
#125379=CARTESIAN_POINT('Ctrl Pts',(-19.3057924258839,14.5863178640293,
131.621910109743)) ;
#125380=CARTESIAN_POINT('Ctrl Pts',(-19.2153083863566,14.55532217226,131.324369164492)) ;
#125381=CARTESIAN_POINT('Ctrl Pts',(-19.1314276970006,14.4431215003341,
131.046235050427)) ;
#125382=CARTESIAN_POINT('Ctrl Pts',(-19.0606803517198,14.2589451908106,
130.806575496976)) ;
#125383=CARTESIAN_POINT('Ctrl Pts',(-19.0082723613581,14.0132050933504,
130.620231148887)) ;
#125384=CARTESIAN_POINT('Ctrl Pts',(-18.9794027695462,13.7264814781089,
130.502832395796)) ;
#125385=CARTESIAN_POINT('Ctrl Pts',(-18.976561908527,13.4166671262314,130.461310037739)) ;
#125386=CARTESIAN_POINT('Ctrl Pts',(-19.0006755833375,13.1090562119369,
130.498725654268)) ;
#125387=CARTESIAN_POINT('Ctrl Pts',(-19.0508377132365,12.8228936687179,
130.612115355244)) ;
#125388=CARTESIAN_POINT('Ctrl Pts',(-19.123922843109,12.5803482500096,130.792567588959)) ;
#125389=CARTESIAN_POINT('Ctrl Pts',(-19.2160850433945,12.3971382780487,
131.028568123365)) ;
#125390=CARTESIAN_POINT('Ctrl Pts',(-19.3206538990753,12.2881794710329,
131.300948176029)) ;
#125391=CARTESIAN_POINT('Ctrl Pts',(-19.431532048178,12.260444774343,131.591652829408)) ;
#125392=CARTESIAN_POINT('Ctrl Pts',(-19.5407246258012,12.3158800590199,
131.877582205411)) ;
#125393=CARTESIAN_POINT('Ctrl Pts',(-19.6420758380499,12.4512316435153,
132.140435538389)) ;
#125394=CARTESIAN_POINT('Ctrl Pts',(-19.7279001857045,12.6546809911043,
132.358198342916)) ;
#125395=CARTESIAN_POINT('Ctrl Pts',(-19.7940662440651,12.9147731891358,
132.518270409866)) ;
#125396=CARTESIAN_POINT('Ctrl Pts',(-19.8356553710753,13.2095560207855,
132.606765160291)) ;
#125397=CARTESIAN_POINT('Ctrl Pts',(-19.8508741819814,13.5223875094378,
132.617909927863)) ;
#125398=CARTESIAN_POINT('Ctrl Pts',(-19.8391683542652,13.8250175828272,
132.550755217814)) ;
#125399=CARTESIAN_POINT('Ctrl Pts',(-19.8018217312818,14.1019896446971,
132.408313123862)) ;
#125400=CARTESIAN_POINT('Ctrl Pts',(-19.7429921890077,14.3273313285593,
132.203502388414)) ;
#125401=CARTESIAN_POINT('Ctrl Pts',(-19.6670062696929,14.4893435909273,
131.948405833705)) ;
#125402=CARTESIAN_POINT('Ctrl Pts',(-19.5802153190921,14.5749600250314,
131.661768392291)) ;
#125403=CARTESIAN_POINT('Ctrl Pts',(-19.4891679081042,14.5779281119493,
131.362553988494)) ;
#125404=CARTESIAN_POINT('Ctrl Pts',(-19.4021090416363,14.4983364866609,
131.075222238346)) ;
#125405=CARTESIAN_POINT('Ctrl Pts',(-19.3250576696382,14.3420895520869,
130.817036674605)) ;
#125406=CARTESIAN_POINT('Ctrl Pts',(-19.2642816474385,14.1180210697834,
130.60616026518)) ;
#125407=CARTESIAN_POINT('Ctrl Pts',(-19.2257474518653,13.8471807636704,
130.460666873348)) ;
#125408=CARTESIAN_POINT('Ctrl Pts',(-19.2120103918454,13.5439412036153,
130.387343681072)) ;
#125409=CARTESIAN_POINT('Ctrl Pts',(-19.225155205879,13.2331633714353,130.39268687927)) ;
#125410=CARTESIAN_POINT('Ctrl Pts',(-19.2651252384059,12.9343807646982,
130.476204059893)) ;
#125411=CARTESIAN_POINT('Ctrl Pts',(-19.3293892623455,12.6721977503837,
130.630876869171)) ;
#125412=CARTESIAN_POINT('Ctrl Pts',(-19.414367024647,12.4632419123552,130.845988794884)) ;
#125413=CARTESIAN_POINT('Ctrl Pts',(-19.5144157619604,12.3231158449139,
131.105192868357)) ;
#125414=CARTESIAN_POINT('Ctrl Pts',(-19.6239682958549,12.2616017868531,
131.391949064764)) ;
#125415=CARTESIAN_POINT('Ctrl Pts',(-19.7341251748847,12.2833201930426,
131.680814419557)) ;
#125416=CARTESIAN_POINT('Ctrl Pts',(-19.8398307670297,12.3868877539332,
131.956364921524)) ;
#125417=CARTESIAN_POINT('Ctrl Pts',(-19.9328715849158,12.5648231593225,
132.195022075704)) ;
#125418=CARTESIAN_POINT('Ctrl Pts',(-20.0075697806433,12.8039602386114,
132.380126700454)) ;
#125419=CARTESIAN_POINT('Ctrl Pts',(-20.0593917089716,13.0864729218444,
132.498501302387)) ;
#125420=CARTESIAN_POINT('Ctrl Pts',(-20.0855942601537,13.3957238551008,
132.541742553164)) ;
#125421=CARTESIAN_POINT('Ctrl Pts',(-20.0846180974026,13.7038340489926,
132.505928237067)) ;
#125422=CARTESIAN_POINT('Ctrl Pts',(-20.0576118412634,13.9936201437027,
132.39389473662)) ;
#125423=CARTESIAN_POINT('Ctrl Pts',(-20.0066670074455,14.2431366533872,
132.211800147466)) ;
#125424=CARTESIAN_POINT('Ctrl Pts',(-19.9372867453542,14.4318623911142,
131.976209777932)) ;
#125425=CARTESIAN_POINT('Ctrl Pts',(-19.8536336247197,14.5502397440411,
131.698547738352)) ;
#125426=CARTESIAN_POINT('Ctrl Pts',(-19.763624304503,14.5868194748713,131.402499062289)) ;
#125427=CARTESIAN_POINT('Ctrl Pts',(-19.6740868384927,14.5403267777303,
131.107834963745)) ;
#125428=CARTESIAN_POINT('Ctrl Pts',(-19.5920809579075,14.4138414860088,
130.835165145447)) ;
#125429=CARTESIAN_POINT('Ctrl Pts',(-19.5242274982525,14.2163546818928,
130.60382730934)) ;
#125430=CARTESIAN_POINT('Ctrl Pts',(-19.4761656045147,13.9624647587777,
130.430351339929)) ;
#125431=CARTESIAN_POINT('Ctrl Pts',(-19.4519267245949,13.6693367218364,
130.326390171342)) ;
#125432=CARTESIAN_POINT('Ctrl Pts',(-19.4541360813185,13.3586797958361,
130.299708635269)) ;
#125433=CARTESIAN_POINT('Ctrl Pts',(-19.4833072792466,13.0526929008547,
130.351794296597)) ;
#125434=CARTESIAN_POINT('Ctrl Pts',(-19.5381123459215,12.7731727546938,
130.478753263755)) ;
#125435=CARTESIAN_POINT('Ctrl Pts',(-19.6152840129382,12.5404161552581,
130.671072410998)) ;
#125436=CARTESIAN_POINT('Ctrl Pts',(-19.7100584664821,12.370760764573,130.914808573912)) ;
#125437=CARTESIAN_POINT('Ctrl Pts',(-19.8164805054715,12.2766729448487,
131.192538102687)) ;
#125438=CARTESIAN_POINT('Ctrl Pts',(-19.9269545882548,12.2643218542415,
131.482288089165)) ;
#125439=CARTESIAN_POINT('Ctrl Pts',(-20.0362420787139,12.336020687125,131.768135189097)) ;
#125440=CARTESIAN_POINT('Ctrl Pts',(-20.1341015859013,12.4836397645111,
132.021190312288)) ;
#125441=CARTESIAN_POINT('Ctrl Pts',(-20.2173448724865,12.7003320009064,
132.231098128125)) ;
#125442=CARTESIAN_POINT('Ctrl Pts',(-20.2788998542731,12.9678918714247,
132.377839505011)) ;
#125443=CARTESIAN_POINT('Ctrl Pts',(-20.3157857749859,13.2687870375049,
132.452412734401)) ;
#125444=CARTESIAN_POINT('Ctrl Pts',(-20.3257878201776,13.5800036106842,
132.44853887218)) ;
#125445=CARTESIAN_POINT('Ctrl Pts',(-20.3091319227027,13.8799730706512,
132.366793007165)) ;
#125446=CARTESIAN_POINT('Ctrl Pts',(-20.2675833294922,14.1476994881547,
132.212271797659)) ;
#125447=CARTESIAN_POINT('Ctrl Pts',(-20.2049654614363,14.3632525192321,
131.996240979151)) ;
#125448=CARTESIAN_POINT('Ctrl Pts',(-20.1261959413298,14.5119336191473,
131.732928450416)) ;
#125449=CARTESIAN_POINT('Ctrl Pts',(-20.0378705228692,14.5819602234039,
131.44171981574)) ;
#125450=CARTESIAN_POINT('Ctrl Pts',(-19.9476548293995,14.5692454166129,
131.145213230718)) ;
#125451=CARTESIAN_POINT('Ctrl Pts',(-19.8615317882014,14.4742854326631,
130.860430878038)) ;
#125452=CARTESIAN_POINT('Ctrl Pts',(-19.7873954923186,14.3047438743695,
130.610843930884)) ;
#125453=CARTESIAN_POINT('Ctrl Pts',(-19.7304993539858,14.0710830609088,
130.411431376984)) ;
#125454=CARTESIAN_POINT('Ctrl Pts',(-19.6962102503808,13.7914035953126,
130.278142215268)) ;
#125455=CARTESIAN_POINT('Ctrl Pts',(-19.6875605883208,13.48501227345,130.219710120386)) ;
#125456=CARTESIAN_POINT('Ctrl Pts',(-19.7057561296348,13.1755843630713,
130.239857217883)) ;
#125457=CARTESIAN_POINT('Ctrl Pts',(-19.7504585123233,12.8823157457974,
130.337257450733)) ;
#125458=CARTESIAN_POINT('Ctrl Pts',(-19.8189208985259,12.6284362839445,
130.504164057257)) ;
#125459=CARTESIAN_POINT('Ctrl Pts',(-19.9078147749595,12.4304595143626,
130.730514989918)) ;
#125460=CARTESIAN_POINT('Ctrl Pts',(-20.0095479920409,12.3053999518157,
130.994813742423)) ;
#125461=CARTESIAN_POINT('Ctrl Pts',(-20.1201667027676,12.2593484399968,
131.284622101872)) ;
#125462=CARTESIAN_POINT('Ctrl Pts',(-20.2296622699611,12.2965483921961,
131.571617133664)) ;
#125463=CARTESIAN_POINT('Ctrl Pts',(-20.3339911299089,12.4156949295869,
131.842988009414)) ;
#125464=CARTESIAN_POINT('Ctrl Pts',(-20.4233888978307,12.6050470782002,
132.071237235801)) ;
#125465=CARTESIAN_POINT('Ctrl Pts',(-20.4945228765996,12.85534209768,132.245732745191)) ;
#125466=CARTESIAN_POINT('Ctrl Pts',(-20.5413967325497,13.1429454569684,
132.349789520615)) ;
#125467=CARTESIAN_POINT('Ctrl Pts',(-20.562611118273,13.4543917047447,132.378442216463)) ;
#125468=CARTESIAN_POINT('Ctrl Pts',(-20.5565479376348,13.7614620059086,
132.327653889222)) ;
#125469=CARTESIAN_POINT('Ctrl Pts',(-20.5247270670738,14.0447128346805,
132.201571129089)) ;
#125470=CARTESIAN_POINT('Ctrl Pts',(-20.4702093585612,14.2828873109444,
132.009265977188)) ;
#125471=CARTESIAN_POINT('Ctrl Pts',(-20.3974418851067,14.4603132478387,
131.763573851832)) ;
#125472=CARTESIAN_POINT('Ctrl Pts',(-20.3119076274948,14.5634617520393,
131.480411939824)) ;
#125473=CARTESIAN_POINT('Ctrl Pts',(-20.221960576711,14.5844329879889,131.184735879175)) ;
#125474=CARTESIAN_POINT('Ctrl Pts',(-20.1329704818831,14.5225343310152,
130.891550458131)) ;
#125475=CARTESIAN_POINT('Ctrl Pts',(-20.0531091686615,14.381544806336,130.625116747778)) ;
#125476=CARTESIAN_POINT('Ctrl Pts',(-19.9886753908938,14.1725754677665,
130.403826414472)) ;
#125477=CARTESIAN_POINT('Ctrl Pts',(-19.9447676258649,13.9093040451571,
130.242407723814)) ;
#125478=CARTESIAN_POINT('Ctrl Pts',(-19.9253917310527,13.6121558294026,
130.152761370539)) ;
#125479=CARTESIAN_POINT('Ctrl Pts',(-19.9327640731267,13.2990170967779,
130.140983614842)) ;
#125480=CARTESIAN_POINT('Ctrl Pts',(-19.966784211622,12.9981565078101,130.207424474512)) ;
#125481=CARTESIAN_POINT('Ctrl Pts',(-20.0259934420432,12.7257032392755,
130.347241404834)) ;
#125482=CARTESIAN_POINT('Ctrl Pts',(-20.1071478867376,12.50307580565,130.551095389013)) ;
#125483=CARTESIAN_POINT('Ctrl Pts',(-20.2043408359347,12.3471529691752,
130.801978619226)) ;
#125484=CARTESIAN_POINT('Ctrl Pts',(-20.3126508795515,12.2678408556735,
131.085078506438)) ;
#125485=CARTESIAN_POINT('Ctrl Pts',(-20.4229187326262,12.2715869300384,
131.374306233546)) ;
#125486=CARTESIAN_POINT('Ctrl Pts',(-20.5302578375964,12.3575776259723,
131.654678476933)) ;
#125487=CARTESIAN_POINT('Ctrl Pts',(-20.6264204325903,12.5198592417277,
131.902499896415)) ;
#125488=CARTESIAN_POINT('Ctrl Pts',(-20.7057938697997,12.7472701152985,
132.101187732545)) ;
#125489=CARTESIAN_POINT('Ctrl Pts',(-20.7630472962772,13.0233715005783,
132.235259403599)) ;
#125490=CARTESIAN_POINT('Ctrl Pts',(-20.7947740167793,13.3264775703159,
132.294936955644)) ;
#125491=CARTESIAN_POINT('Ctrl Pts',(-20.7998253098923,13.6374829528976,
132.276579789714)) ;
#125492=CARTESIAN_POINT('Ctrl Pts',(-20.7781798467671,13.9340523066843,
132.180125678852)) ;
#125493=CARTESIAN_POINT('Ctrl Pts',(-20.7323182863517,14.1931239778517,
132.013032839121)) ;
#125494=CARTESIAN_POINT('Ctrl Pts',(-20.6659952400125,14.3974304902421,
131.78607443323)) ;
#125495=CARTESIAN_POINT('Ctrl Pts',(-20.5854240712101,14.5309245532204,
131.517722674269)) ;
#125496=CARTESIAN_POINT('Ctrl Pts',(-20.4962685721323,14.5859814539265,
131.224148101963)) ;
#125497=CARTESIAN_POINT('Ctrl Pts',(-20.4058963569354,14.5574777806989,
130.927001172984)) ;
#125498=CARTESIAN_POINT('Ctrl Pts',(-20.3216691370053,14.4480150523887,
130.647857808576)) ;
#125499=CARTESIAN_POINT('Ctrl Pts',(-20.2499907856577,14.2640746902433,
130.405219408407)) ;
#125500=CARTESIAN_POINT('Ctrl Pts',(-20.1974565013379,14.0222278683344,
130.218833806972)) ;
#125501=CARTESIAN_POINT('Ctrl Pts',(-20.1675706919809,13.7339092296597,
130.098157959704)) ;
#125502=CARTESIAN_POINT('Ctrl Pts',(-20.1640677436926,13.4264443376891,
130.054932391349)) ;
#125503=CARTESIAN_POINT('Ctrl Pts',(-20.1873548159157,13.1179337351116,
130.089866611451)) ;
#125504=CARTESIAN_POINT('Ctrl Pts',(-20.2367558298266,12.8308236558004,
130.201047137032)) ;
#125505=CARTESIAN_POINT('Ctrl Pts',(-20.3095840954364,12.5859821192932,
130.380611728237)) ;
#125506=CARTESIAN_POINT('Ctrl Pts',(-20.4006241545898,12.4020104607834,
130.613571603836)) ;
#125507=CARTESIAN_POINT('Ctrl Pts',(-20.5055712162227,12.2899875616105,
130.886838354764)) ;
#125508=CARTESIAN_POINT('Ctrl Pts',(-20.6158038744858,12.260124778228,131.175836440016)) ;
#125509=CARTESIAN_POINT('Ctrl Pts',(-20.725325813667,12.3130229090721,131.46266764125)) ;
#125510=CARTESIAN_POINT('Ctrl Pts',(-20.8268144993231,12.445755568189,131.72599885581)) ;
#125511=CARTESIAN_POINT('Ctrl Pts',(-20.9134907572975,12.6478749143986,
131.94613786665)) ;
#125512=CARTESIAN_POINT('Ctrl Pts',(-20.9804389337324,12.9074235529971,
132.108409295979)) ;
#125513=CARTESIAN_POINT('Ctrl Pts',(-21.0226586722023,13.201587990353,132.198739885101)) ;
#125514=CARTESIAN_POINT('Ctrl Pts',(-21.0386105188704,13.5132462797945,
132.212140657446)) ;
#125515=CARTESIAN_POINT('Ctrl Pts',(-21.0275858269164,13.8170405083281,
132.14689488238)) ;
#125516=CARTESIAN_POINT('Ctrl Pts',(-20.9912734830522,14.0930904717493,
132.007734125149)) ;
#125517=CARTESIAN_POINT('Ctrl Pts',(-20.9328468771947,14.3215765569393,
131.803931803933)) ;
#125518=CARTESIAN_POINT('Ctrl Pts',(-20.8569974472105,14.4860164684736,
131.549134598391)) ;
#125519=CARTESIAN_POINT('Ctrl Pts',(-20.7703215178779,14.5737422146348,
131.262802859148)) ;
#125520=CARTESIAN_POINT('Ctrl Pts',(-20.6795334980067,14.5789283273619,
130.964434672584)) ;
#125521=CARTESIAN_POINT('Ctrl Pts',(-20.5922289646685,14.5018179973275,
130.676378069679)) ;
#125522=CARTESIAN_POINT('Ctrl Pts',(-20.5145673896872,14.3465570817491,
130.416269496224)) ;
#125523=CARTESIAN_POINT('Ctrl Pts',(-20.4538879568746,14.1268974135735,
130.206064475321)) ;
#125524=CARTESIAN_POINT('Ctrl Pts',(-20.4142221803974,13.8551171351805,
130.056974334884)) ;
#125525=CARTESIAN_POINT('Ctrl Pts',(-20.3998288749854,13.5530512913373,
129.981815424211)) ;
#125526=CARTESIAN_POINT('Ctrl Pts',(-20.4122289800202,13.2415863722887,
129.98490917036)) ;
#125527=CARTESIAN_POINT('Ctrl Pts',(-20.451304951926,12.9431696446184,130.06593789593)) ;
#125528=CARTESIAN_POINT('Ctrl Pts',(-20.5150277326967,12.6789855652346,
130.218945397434)) ;
#125529=CARTESIAN_POINT('Ctrl Pts',(-20.59938870539,12.4685393411929,130.432298405932)) ;
#125530=CARTESIAN_POINT('Ctrl Pts',(-20.6990677999997,12.3261974567536,
130.690420636)) ;
#125531=CARTESIAN_POINT('Ctrl Pts',(-20.8083842807917,12.2622045863294,
130.976510913894)) ;
#125532=CARTESIAN_POINT('Ctrl Pts',(-20.9188027504055,12.2815898353466,
131.266074603366)) ;
#125533=CARTESIAN_POINT('Ctrl Pts',(-21.0244452528796,12.3824517800912,
131.541548083244)) ;
#125534=CARTESIAN_POINT('Ctrl Pts',(-21.118092393428,12.5585397023802,131.781921448334)) ;
#125535=CARTESIAN_POINT('Ctrl Pts',(-21.1933604529092,12.7954955062998,
131.968753676057)) ;
#125536=CARTESIAN_POINT('Ctrl Pts',(-21.2462570078652,13.0796940190917,
132.089961785782)) ;
#125537=CARTESIAN_POINT('Ctrl Pts',(-21.2729118079994,13.3852304458179,
132.134891546362)) ;
#125538=CARTESIAN_POINT('Ctrl Pts',(-21.2728211559508,13.69604445911,132.101399472322)) ;
#125539=CARTESIAN_POINT('Ctrl Pts',(-21.2464415175453,13.985866733445,131.991275439313)) ;
#125540=CARTESIAN_POINT('Ctrl Pts',(-21.1964399533081,14.2358877356182,
131.812083957128)) ;
#125541=CARTESIAN_POINT('Ctrl Pts',(-21.1272541863527,14.4275999337175,
131.57690711089)) ;
#125542=CARTESIAN_POINT('Ctrl Pts',(-21.0437448885435,14.5480862858471,
131.299621047924)) ;
#125543=CARTESIAN_POINT('Ctrl Pts',(-20.9541410393014,14.5868446718797,
131.004870001721)) ;
#125544=CARTESIAN_POINT('Ctrl Pts',(-20.8645870046891,14.5430357670067,
130.71019710521)) ;
#125545=CARTESIAN_POINT('Ctrl Pts',(-20.7821504245794,14.41874401797,130.436229232474)) ;
#125546=CARTESIAN_POINT('Ctrl Pts',(-20.7137193836823,14.2230681528207,
130.203180502296)) ;
#125547=CARTESIAN_POINT('Ctrl Pts',(-20.6649423891261,13.9697197453762,
130.027517386602)) ;
#125548=CARTESIAN_POINT('Ctrl Pts',(-20.6400754360656,13.6787523324498,
129.921874279192)) ;
#125549=CARTESIAN_POINT('Ctrl Pts',(-20.6414819785661,13.3668522755562,
129.892691132996)) ;
#125550=CARTESIAN_POINT('Ctrl Pts',(-20.6699979410068,13.060672465625,129.942883851846)) ;
#125551=CARTESIAN_POINT('Ctrl Pts',(-20.7238971217684,12.7810810976344,
130.067313557987)) ;
#125552=CARTESIAN_POINT('Ctrl Pts',(-20.8004298736072,12.5467077229853,
130.257772798001)) ;
#125553=CARTESIAN_POINT('Ctrl Pts',(-20.8945661196432,12.375036029875,130.499700142091)) ;
#125554=CARTESIAN_POINT('Ctrl Pts',(-21.0013745401089,12.2779852364334,
130.778361903145)) ;
#125555=CARTESIAN_POINT('Ctrl Pts',(-21.1116666074204,12.263745955446,131.067624667673)) ;
#125556=CARTESIAN_POINT('Ctrl Pts',(-21.2204165815676,12.3321871906188,
131.352129032139)) ;
#125557=CARTESIAN_POINT('Ctrl Pts',(-21.3195254329621,12.4786900321498,
131.608553898707)) ;
#125558=CARTESIAN_POINT('Ctrl Pts',(-21.4032330604707,12.6941599570478,
131.81980234989)) ;
#125559=CARTESIAN_POINT('Ctrl Pts',(-21.4652019062618,12.9594898311094,
131.967877269519)) ;
#125560=CARTESIAN_POINT('Ctrl Pts',(-21.5028731218885,13.2597802878034,
132.044736719879)) ;
#125561=CARTESIAN_POINT('Ctrl Pts',(-21.5136586591111,13.5705933911082,
132.043193173102)) ;
#125562=CARTESIAN_POINT('Ctrl Pts',(-21.4977998320591,13.8717555022921,
131.963723980422)) ;
#125563=CARTESIAN_POINT('Ctrl Pts',(-21.4566374898941,14.1416796956212,
131.810184445512)) ;
#125564=CARTESIAN_POINT('Ctrl Pts',(-21.3949269775792,14.3575208853318,
131.597015858169)) ;
#125565=CARTESIAN_POINT('Ctrl Pts',(-21.3163223809269,14.5088742851846,
131.334081154852)) ;
#125566=CARTESIAN_POINT('Ctrl Pts',(-21.2283674664414,14.5810485932283,
131.044035253294)) ;
#125567=CARTESIAN_POINT('Ctrl Pts',(-21.1379878817008,14.5707018107426,
130.74699291225)) ;
#125568=CARTESIAN_POINT('Ctrl Pts',(-21.0518809543132,14.4785662345022,
130.46236961443)) ;
#125569=CARTESIAN_POINT('Ctrl Pts',(-20.976718142438,14.3096045878152,130.209508594268)) ;
#125570=CARTESIAN_POINT('Ctrl Pts',(-20.9195313547551,14.0777449679159,
130.009336738625)) ;
#125571=CARTESIAN_POINT('Ctrl Pts',(-20.8846809598118,13.8001341455209,
129.874521428525)) ;
#125572=CARTESIAN_POINT('Ctrl Pts',(-20.8751865502058,13.4946152703642,
129.813664552878)) ;
#125573=CARTESIAN_POINT('Ctrl Pts',(-20.8927061896601,13.1837406589244,
129.831697274769)) ;
#125574=CARTESIAN_POINT('Ctrl Pts',(-20.9365995694632,12.8901082273082,
129.926795681337)) ;
#125575=CARTESIAN_POINT('Ctrl Pts',(-21.0049177915536,12.6339160706406,
130.093104476252)) ;
#125576=CARTESIAN_POINT('Ctrl Pts',(-21.0920187661593,12.4365925645623,
130.314691586752)) ;
#125577=CARTESIAN_POINT('Ctrl Pts',(-21.1945890656971,12.3075969590058,
130.581034844336)) ;
#125578=CARTESIAN_POINT('Ctrl Pts',(-21.3041078767494,12.2595413699531,
130.867941860621)) ;
#125579=CARTESIAN_POINT('Ctrl Pts',(-21.414714087137,12.2945981250866,131.157860792763)) ;
#125580=CARTESIAN_POINT('Ctrl Pts',(-21.5182505698646,12.4101972577176,
131.42728025094)) ;
#125581=CARTESIAN_POINT('Ctrl Pts',(-21.6088669941318,12.598715944425,131.658831153717)) ;
#125582=CARTESIAN_POINT('Ctrl Pts',(-21.6803208590174,12.8461743706132,
131.834442515426)) ;
#125583=CARTESIAN_POINT('Ctrl Pts',(-21.7283998303603,13.1359262374288,
131.941663820147)) ;
#125584=CARTESIAN_POINT('Ctrl Pts',(-21.7501146102558,13.4447581529336,
131.97204316023)) ;
#125585=CARTESIAN_POINT('Ctrl Pts',(-21.7448694054129,13.7530929209566,
131.923542338584)) ;
#125586=CARTESIAN_POINT('Ctrl Pts',(-21.7138911823186,14.0362080508941,
131.800059197407)) ;
#125587=CARTESIAN_POINT('Ctrl Pts',(-21.6598673248284,14.2769560090218,
131.609081968409)) ;
#125588=CARTESIAN_POINT('Ctrl Pts',(-21.5873536841721,14.4563581984587,
131.364074061383)) ;
#125589=CARTESIAN_POINT('Ctrl Pts',(-21.5026599241299,14.5613193565883,
131.083584293766)) ;
#125590=CARTESIAN_POINT('Ctrl Pts',(-21.4121679015584,14.5851466740993,
130.786094569346)) ;
#125591=CARTESIAN_POINT('Ctrl Pts',(-21.3229798957179,14.5250094201889,
130.492300414709)) ;
#125592=CARTESIAN_POINT('Ctrl Pts',(-21.2431880284182,14.3871118872338,
130.226257623174)) ;
#125593=CARTESIAN_POINT('Ctrl Pts',(-21.1778843641689,14.1786613146333,
130.002228172161)) ;
#125594=CARTESIAN_POINT('Ctrl Pts',(-21.1335446386563,13.9181921404444,
129.839744069384)) ;
#125595=CARTESIAN_POINT('Ctrl Pts',(-21.1133238256431,13.6189922621126,
129.747319744249)) ;
#125596=CARTESIAN_POINT('Ctrl Pts',(-21.1199394173291,13.3089360963624,
129.733660018502)) ;
#125597=CARTESIAN_POINT('Ctrl Pts',(-21.15326877726,13.0058324971489,129.797902039434)) ;
#125598=CARTESIAN_POINT('Ctrl Pts',(-21.2120574557122,12.7318651916952,
129.936425658188)) ;
#125599=CARTESIAN_POINT('Ctrl Pts',(-21.2925597772729,12.5082426234418,
130.138441418088)) ;
#125600=CARTESIAN_POINT('Ctrl Pts',(-21.3890394795578,12.3508732167538,
130.387352736043)) ;
#125601=CARTESIAN_POINT('Ctrl Pts',(-21.496781967904,12.2691036353101,130.668897537391)) ;
#125602=CARTESIAN_POINT('Ctrl Pts',(-21.6076020846144,12.2702137418504,
130.959576850838)) ;
#125603=CARTESIAN_POINT('Ctrl Pts',(-21.7152916878763,12.3542930287051,
131.240924005532)) ;
#125604=CARTESIAN_POINT('Ctrl Pts',(-21.8115660696969,12.5141177100409,
131.489166666111)) ;
#125605=CARTESIAN_POINT('Ctrl Pts',(-21.8914520404614,12.7395234896818,
131.689386122552)) ;
#125606=CARTESIAN_POINT('Ctrl Pts',(-21.949435548747,13.0142280160873,131.825609613672)) ;
#125607=CARTESIAN_POINT('Ctrl Pts',(-21.9820492110329,13.3177663479764,
131.887772553571)) ;
#125608=CARTESIAN_POINT('Ctrl Pts',(-21.9878167428512,13.6286638171374,
131.871529705244)) ;
#125609=CARTESIAN_POINT('Ctrl Pts',(-21.9670224795337,13.925291931835,131.777646134426)) ;
#125610=CARTESIAN_POINT('Ctrl Pts',(-21.9217757158089,14.1860950196788,
131.61230143831)) ;
#125611=CARTESIAN_POINT('Ctrl Pts',(-21.8562405122822,14.3917324528471,
131.387756932998)) ;
#125612=CARTESIAN_POINT('Ctrl Pts',(-21.7756903472869,14.5282787585867,
131.119317953133)) ;
#125613=CARTESIAN_POINT('Ctrl Pts',(-21.6864909606961,14.585553871015,130.825554832936)) ;
#125614=CARTESIAN_POINT('Ctrl Pts',(-21.5963140146045,14.5594424124574,
130.529072362239)) ;
#125615=CARTESIAN_POINT('Ctrl Pts',(-21.5118873080126,14.452533822029,130.249380272377)) ;
#125616=CARTESIAN_POINT('Ctrl Pts',(-21.4396023594563,14.2704301815678,
130.004922447039)) ;
#125617=CARTESIAN_POINT('Ctrl Pts',(-21.3864210307148,14.0294404722423,
129.816576108765)) ;
#125618=CARTESIAN_POINT('Ctrl Pts',(-21.3559418238359,13.7439522492757,
129.694376590572)) ;
#125619=CARTESIAN_POINT('Ctrl Pts',(-21.3515590072131,13.4354033023599,
129.648418578587)) ;
#125620=CARTESIAN_POINT('Ctrl Pts',(-21.3740511377046,13.1268757917154,
129.681069437497)) ;
#125621=CARTESIAN_POINT('Ctrl Pts',(-21.4229183024262,12.8380942366352,
129.790589937005)) ;
#125622=CARTESIAN_POINT('Ctrl Pts',(-21.4946813071599,12.5930207366324,
129.967235280058)) ;
#125623=CARTESIAN_POINT('Ctrl Pts',(-21.5858119382305,12.406038861412,130.200252155053)) ;
#125624=CARTESIAN_POINT('Ctrl Pts',(-21.68959704384,12.292531234905,130.470405728911)) ;
#125625=CARTESIAN_POINT('Ctrl Pts',(-21.8006640611008,12.259700175239,130.761558183255)) ;
#125626=CARTESIAN_POINT('Ctrl Pts',(-21.9100727883452,12.3104428593725,
131.048134164405)) ;
#125627=CARTESIAN_POINT('Ctrl Pts',(-22.0119946874219,12.4411375655696,
131.312691934815)) ;
#125628=CARTESIAN_POINT('Ctrl Pts',(-22.0989549674782,12.6410412802729,
131.533737469327)) ;
#125629=CARTESIAN_POINT('Ctrl Pts',(-22.1665960353877,12.8990710258353,
131.698038077876)) ;
#125630=CARTESIAN_POINT('Ctrl Pts',(-22.2096292017843,13.1932159520557,
131.790663136746)) ;
#125631=CARTESIAN_POINT('Ctrl Pts',(-22.2263015712469,13.5039484440362,
131.80625317794)) ;
#125632=CARTESIAN_POINT('Ctrl Pts',(-22.2160709879322,13.8084630693567,
131.743303504259)) ;
#125633=CARTESIAN_POINT('Ctrl Pts',(-22.1804532453563,14.0856215831729,
131.606173872007)) ;
#125634=CARTESIAN_POINT('Ctrl Pts',(-22.1226056277055,14.3156974837171,
131.404064385855)) ;
#125635=CARTESIAN_POINT('Ctrl Pts',(-22.0473303523545,14.482069329469,131.1510040704)) ;
#125636=CARTESIAN_POINT('Ctrl Pts',(-21.9607116573561,14.5722583544091,
130.864770552622)) ;
#125637=CARTESIAN_POINT('Ctrl Pts',(-21.8703953183131,14.5801736799871,
130.567952070754)) ;
#125638=CARTESIAN_POINT('Ctrl Pts',(-21.7822499355248,14.5050113517495,
130.277192893103)) ;
#125639=CARTESIAN_POINT('Ctrl Pts',(-21.7044840301903,14.3522164750112,
130.01689633979)) ;
#125640=CARTESIAN_POINT('Ctrl Pts',(-21.6431388088135,14.1339602612738,
129.804686049646)) ;
#125641=CARTESIAN_POINT('Ctrl Pts',(-21.6028682983574,13.8641112712326,
129.65391825805)) ;
#125642=CARTESIAN_POINT('Ctrl Pts',(-21.5876385948603,13.5616225014003,
129.576198403786)) ;
#125643=CARTESIAN_POINT('Ctrl Pts',(-21.5992932161767,13.2502934236062,
129.577137522919)) ;
#125644=CARTESIAN_POINT('Ctrl Pts',(-21.6376942912837,12.9509782560257,
129.656163454282)) ;
#125645=CARTESIAN_POINT('Ctrl Pts',(-21.7005423302571,12.6863948819192,
129.806725409211)) ;
#125646=CARTESIAN_POINT('Ctrl Pts',(-21.7845354885147,12.4734606146631,
130.018920464526)) ;
#125647=CARTESIAN_POINT('Ctrl Pts',(-21.8843134729441,12.3287823734524,
130.277199856625)) ;
#125648=CARTESIAN_POINT('Ctrl Pts',(-21.9929392570174,12.262963408062,130.561438527531)) ;
#125649=CARTESIAN_POINT('Ctrl Pts',(-22.1035861834769,12.2798963364109,
130.851612471303)) ;
#125650=CARTESIAN_POINT('Ctrl Pts',(-22.2095302910128,12.3786944152069,
131.127948672773)) ;
#125651=CARTESIAN_POINT('Ctrl Pts',(-22.3037053420613,12.5532637477409,
131.369814961767)) ;
#125652=CARTESIAN_POINT('Ctrl Pts',(-22.3791978821218,12.7879392173085,
131.557427905372)) ;
#125653=CARTESIAN_POINT('Ctrl Pts',(-22.432676499044,13.0695371613245,131.68049834232)) ;
#125654=CARTESIAN_POINT('Ctrl Pts',(-22.460347286562,13.3764287313842,131.728200911231)) ;
#125655=CARTESIAN_POINT('Ctrl Pts',(-22.460962142873,13.6873693944069,131.696780968098)) ;
#125656=CARTESIAN_POINT('Ctrl Pts',(-22.4353608541561,13.9780097537181,
131.58894187598)) ;
#125657=CARTESIAN_POINT('Ctrl Pts',(-22.385713314181,14.2303816916052,131.410644205357)) ;
#125658=CARTESIAN_POINT('Ctrl Pts',(-22.3171996696004,14.4229832275646,
131.177555141404)) ;
#125659=CARTESIAN_POINT('Ctrl Pts',(-22.2342095372013,14.545607197334,130.901858853861)) ;
#125660=CARTESIAN_POINT('Ctrl Pts',(-22.1445457999827,14.5869244372964,
130.606872978911)) ;
#125661=CARTESIAN_POINT('Ctrl Pts',(-22.0548221478016,14.545413999477,130.311682615408)) ;
#125662=CARTESIAN_POINT('Ctrl Pts',(-21.9720637241757,14.4231615318539,
130.036761175897)) ;
#125663=CARTESIAN_POINT('Ctrl Pts',(-21.9033593370502,14.2299646003197,
129.803014658946)) ;
#125664=CARTESIAN_POINT('Ctrl Pts',(-21.8538582145753,13.9782380349311,
129.625238447864)) ;
#125665=CARTESIAN_POINT('Ctrl Pts',(-21.8282135190343,13.6869896701315,
129.517199857734)) ;
#125666=CARTESIAN_POINT('Ctrl Pts',(-21.8288197658371,13.3772462280803,
129.48588557063)) ;
#125667=CARTESIAN_POINT('Ctrl Pts',(-21.8564296864021,13.0701026348063,
129.533383001369)) ;
#125668=CARTESIAN_POINT('Ctrl Pts',(-21.9098344339023,12.7883757721948,
129.656241120906)) ;
#125669=CARTESIAN_POINT('Ctrl Pts',(-21.9857856890572,12.5524788061311,
129.84500715286)) ;
#125670=CARTESIAN_POINT('Ctrl Pts',(-22.0796909556344,12.3787205922408,
130.086201475717)) ;
#125671=CARTESIAN_POINT('Ctrl Pts',(-22.1856098910202,12.2799428361804,
130.362465376775)) ;
#125672=CARTESIAN_POINT('Ctrl Pts',(-22.2961046110537,12.26278144672,130.652245503551)) ;
#125673=CARTESIAN_POINT('Ctrl Pts',(-22.4056125857822,12.3295044441556,
130.938781716438)) ;
#125674=CARTESIAN_POINT('Ctrl Pts',(-22.5045503687808,12.4735104762095,
131.194864039758)) ;
#125675=CARTESIAN_POINT('Ctrl Pts',(-22.5885187900511,12.6859036202202,
131.407023886207)) ;
#125676=CARTESIAN_POINT('Ctrl Pts',(-22.6515372036972,12.9511128750471,
131.558004821108)) ;
#125677=CARTESIAN_POINT('Ctrl Pts',(-22.689964997057,13.2510042881428,131.637050794627)) ;
#125678=CARTESIAN_POINT('Ctrl Pts',(-22.7015161637052,13.5624349033162,
131.637676113596)) ;
#125679=CARTESIAN_POINT('Ctrl Pts',(-22.686344284073,13.8634351893562,131.560285852855)) ;
#125680=CARTESIAN_POINT('Ctrl Pts',(-22.6462161333374,14.1332614315187,
131.409958331396)) ;
#125681=CARTESIAN_POINT('Ctrl Pts',(-22.5846264147229,14.3526410215066,
131.196887959862)) ;
#125682=CARTESIAN_POINT('Ctrl Pts',(-22.506540094871,14.5054039917793,130.935553228196)) ;
#125683=CARTESIAN_POINT('Ctrl Pts',(-22.4191482201114,14.5799567731311,
130.647279826546)) ;
#125684=CARTESIAN_POINT('Ctrl Pts',(-22.3283933686161,14.572371407252,130.349018922444)) ;
#125685=CARTESIAN_POINT('Ctrl Pts',(-22.2417737954577,14.4818104179813,
130.062771911775)) ;
#125686=CARTESIAN_POINT('Ctrl Pts',(-22.1668084149478,14.3163442533983,
129.810766300736)) ;
#125687=CARTESIAN_POINT('Ctrl Pts',(-22.1087759662198,14.0859120132609,
129.608039485136)) ;
#125688=CARTESIAN_POINT('Ctrl Pts',(-22.0731170711164,13.8088757639041,
129.470801563983)) ;
#125689=CARTESIAN_POINT('Ctrl Pts',(-22.0628921530061,13.5028415696086,
129.407702944784)) ;
#125690=CARTESIAN_POINT('Ctrl Pts',(-22.0795605465254,13.1931030740132,
129.423392458417)) ;
#125691=CARTESIAN_POINT('Ctrl Pts',(-22.1228245546184,12.8979592088334,
129.516564666613)) ;
#125692=CARTESIAN_POINT('Ctrl Pts',(-22.1900878866385,12.6415806575113,
129.679968460052)) ;
#125693=CARTESIAN_POINT('Ctrl Pts',(-22.2772779130057,12.4408172036161,
129.901573943192)) ;
#125694=CARTESIAN_POINT('Ctrl Pts',(-22.379557207116,12.3100401552364,130.167079846431)) ;
#125695=CARTESIAN_POINT('Ctrl Pts',(-22.4887216341412,12.2598615756175,
130.453018076937)) ;
#125696=CARTESIAN_POINT('Ctrl Pts',(-22.5991744377342,12.2922205464447,
130.742565298188)) ;
#125697=CARTESIAN_POINT('Ctrl Pts',(-22.7035453793508,12.40624849515,131.014244429529)) ;
#125698=CARTESIAN_POINT('Ctrl Pts',(-22.7943699277688,12.5927140641391,
131.246477725961)) ;
#125699=CARTESIAN_POINT('Ctrl Pts',(-22.8662655898373,12.8381488954601,
131.423450080432)) ;
#125700=CARTESIAN_POINT('Ctrl Pts',(-22.9150550731725,13.1260095358548,
131.532846123897)) ;
#125701=CARTESIAN_POINT('Ctrl Pts',(-22.9376902134472,13.4367097241923,
131.565680322971)) ;
#125702=CARTESIAN_POINT('Ctrl Pts',(-22.9331885517525,13.7438376773702,
131.519521875637)) ;
#125703=CARTESIAN_POINT('Ctrl Pts',(-22.9029068463003,14.0287736558089,
131.397981832409)) ;
#125704=CARTESIAN_POINT('Ctrl Pts',(-22.8494229071779,14.2709621799374,
131.20857762131)) ;
#125705=CARTESIAN_POINT('Ctrl Pts',(-22.7775004359681,14.4520608011874,
130.965354382792)) ;
#125706=CARTESIAN_POINT('Ctrl Pts',(-22.6929376253596,14.5594794464979,
130.685194528285)) ;
#125707=CARTESIAN_POINT('Ctrl Pts',(-22.6026883853366,14.5855261750269,
130.38847763073)) ;
#125708=CARTESIAN_POINT('Ctrl Pts',(-22.5135631277621,14.5283738687936,
130.094960233559)) ;
#125709=CARTESIAN_POINT('Ctrl Pts',(-22.4329133576036,14.3916536122689,
129.826188034227)) ;
#125710=CARTESIAN_POINT('Ctrl Pts',(-22.367483851615,14.1863632945959,129.602008031043)) ;
#125711=CARTESIAN_POINT('Ctrl Pts',(-22.3222022530891,13.9255968041967,
129.43655632992)) ;
#125712=CARTESIAN_POINT('Ctrl Pts',(-22.3013824069524,13.6292800303555,
129.342629054356)) ;
#125713=CARTESIAN_POINT('Ctrl Pts',(-22.3071114891914,13.3179689166563,
129.326228873449)) ;
#125714=CARTESIAN_POINT('Ctrl Pts',(-22.3397290895377,13.0144328238462,
129.388404090424)) ;
#125715=CARTESIAN_POINT('Ctrl Pts',(-22.3975763598925,12.7401667038842,
129.524286626664)) ;
#125716=CARTESIAN_POINT('Ctrl Pts',(-22.4774181520926,12.5144106692782,
129.724364422283)) ;
#125717=CARTESIAN_POINT('Ctrl Pts',(-22.5741193712273,12.3540784251448,
129.973715242602)) ;
#125718=CARTESIAN_POINT('Ctrl Pts',(-22.6811523681517,12.2704506674806,
130.253347738944)) ;
#125719=CARTESIAN_POINT('Ctrl Pts',(-22.7923265389067,12.2689821034606,
130.544952223405)) ;
#125720=CARTESIAN_POINT('Ctrl Pts',(-22.9001417640839,12.350850990926,130.826689686085)) ;
#125721=CARTESIAN_POINT('Ctrl Pts',(-22.9968454884217,12.5086055972373,
131.076177637184)) ;
#125722=CARTESIAN_POINT('Ctrl Pts',(-23.0774719156549,12.7330677829212,
131.278472278326)) ;
#125723=CARTESIAN_POINT('Ctrl Pts',(-23.1359818046982,13.0066124889692,
131.416256845004)) ;
#125724=CARTESIAN_POINT('Ctrl Pts',(-23.1692213521271,13.308272601369,131.480391873357)) ;
#125725=CARTESIAN_POINT('Ctrl Pts',(-23.1758458307034,13.6201713325224,
131.466556851235)) ;
#125726=CARTESIAN_POINT('Ctrl Pts',(-23.1556315248226,13.9183341039009,
131.374269427024)) ;
#125727=CARTESIAN_POINT('Ctrl Pts',(-23.1110228710728,14.1797388278147,
131.210851244888)) ;
#125728=CARTESIAN_POINT('Ctrl Pts',(-23.0462187780778,14.3864987369051,
130.988550039522)) ;
#125729=CARTESIAN_POINT('Ctrl Pts',(-22.966063587632,14.5252641755352,130.721275013867)) ;
#125730=CARTESIAN_POINT('Ctrl Pts',(-22.8769915510678,14.5851721038055,
130.42787569678)) ;
#125731=CARTESIAN_POINT('Ctrl Pts',(-22.7862418920941,14.5610669162746,
130.129530157643)) ;
#125732=CARTESIAN_POINT('Ctrl Pts',(-22.7020506121271,14.4566509798001,
129.850704631775)) ;
#125733=CARTESIAN_POINT('Ctrl Pts',(-22.6293418474591,14.2771545198569,
129.605059764206)) ;
#125734=CARTESIAN_POINT('Ctrl Pts',(-22.5753044942391,14.0362065305465,
129.414025275407)) ;
#125735=CARTESIAN_POINT('Ctrl Pts',(-22.5443289524662,13.753398715095,129.290579678709)) ;
#125736=CARTESIAN_POINT('Ctrl Pts',(-22.5390419745757,13.4441283585126,
129.241859045919)) ;
#125737=CARTESIAN_POINT('Ctrl Pts',(-22.5609786844499,13.1346408966579,
129.272806550467)) ;
#125738=CARTESIAN_POINT('Ctrl Pts',(-22.6086912148905,12.8470251737848,
129.379206459385)) ;
#125739=CARTESIAN_POINT('Ctrl Pts',(-22.6803934288997,12.5984937869307,
129.555405712019)) ;
#125740=CARTESIAN_POINT('Ctrl Pts',(-22.7705691384996,12.4108688278635,
129.785832773901)) ;
#125741=CARTESIAN_POINT('Ctrl Pts',(-22.8742759459874,12.2946081096869,
130.055675073743)) ;
#125742=CARTESIAN_POINT('Ctrl Pts',(-22.9853475814919,12.2594450533974,
130.346820691978)) ;
#125743=CARTESIAN_POINT('Ctrl Pts',(-23.0949607973134,12.30804814686,130.633963194578)) ;
#125744=CARTESIAN_POINT('Ctrl Pts',(-23.1968663509126,12.4360760991486,
130.898588194265)) ;
#125745=CARTESIAN_POINT('Ctrl Pts',(-23.2845187744347,12.634525822386,131.12158237805)) ;
#125746=CARTESIAN_POINT('Ctrl Pts',(-23.352574330873,12.8902137015407,131.287216571131)) ;
#125747=CARTESIAN_POINT('Ctrl Pts',(-23.3964713954108,13.1836915440523,
131.382336055602)) ;
#125748=CARTESIAN_POINT('Ctrl Pts',(-23.4139997612099,13.4943234250401,
131.400420925134)) ;
#125749=CARTESIAN_POINT('Ctrl Pts',(-23.4044990531187,13.8008444914087,
131.339441224861)) ;
#125750=CARTESIAN_POINT('Ctrl Pts',(-23.3693574684695,14.0793170573489,
131.203644426842)) ;
#125751=CARTESIAN_POINT('Ctrl Pts',(-23.3123406169852,14.3098745304063,
131.004120413233)) ;
#125752=CARTESIAN_POINT('Ctrl Pts',(-23.2371407307095,14.4788324739109,
130.751136748099)) ;
#125753=CARTESIAN_POINT('Ctrl Pts',(-23.1511653084581,14.5706780118123,
130.466953543331)) ;
#125754=CARTESIAN_POINT('Ctrl Pts',(-23.0606882221465,14.5811216563982,
130.169593581504)) ;
#125755=CARTESIAN_POINT('Ctrl Pts',(-22.9725268245407,14.5082991498853,
129.878848830671)) ;
#125756=CARTESIAN_POINT('Ctrl Pts',(-22.8944300957472,14.3580057871193,
129.61762284133)) ;
#125757=CARTESIAN_POINT('Ctrl Pts',(-22.8322738880316,14.1405256903455,
129.402903517555)) ;
#125758=CARTESIAN_POINT('Ctrl Pts',(-22.7914817526284,13.8719961113424,
129.250646984915)) ;
#125759=CARTESIAN_POINT('Ctrl Pts',(-22.7754966150293,13.5716289607196,
129.170880112309)) ;
#125760=CARTESIAN_POINT('Ctrl Pts',(-22.7863642218149,13.2591262832754,
129.169394891665)) ;
#125761=CARTESIAN_POINT('Ctrl Pts',(-22.8238939066087,12.9599151059205,
129.245966509562)) ;
#125762=CARTESIAN_POINT('Ctrl Pts',(-22.8862611929524,12.6930800437845,
129.395005704093)) ;
#125763=CARTESIAN_POINT('Ctrl Pts',(-22.9696496692536,12.4788237616548,
129.605480629806)) ;
#125764=CARTESIAN_POINT('Ctrl Pts',(-23.0687430408362,12.332247898292,129.861853849545)) ;
#125765=CARTESIAN_POINT('Ctrl Pts',(-23.1773252167152,12.2636849567094,
130.14592080679)) ;
#125766=CARTESIAN_POINT('Ctrl Pts',(-23.2883124035474,12.2782423804387,
130.437001735549)) ;
#125767=CARTESIAN_POINT('Ctrl Pts',(-23.3943864358888,12.3748788763276,
130.713742699543)) ;
#125768=CARTESIAN_POINT('Ctrl Pts',(-23.4886534469715,12.5463735135204,
130.956024389397)) ;
#125769=CARTESIAN_POINT('Ctrl Pts',(-23.5652915574259,12.7810696956234,
131.146748612279)) ;
#125770=CARTESIAN_POINT('Ctrl Pts',(-23.6192243080399,13.0608633683861,
131.271253850874)) ;
#125771=CARTESIAN_POINT('Ctrl Pts',(-23.6477017970955,13.3671883117348,
131.321319852897)) ;
#125772=CARTESIAN_POINT('Ctrl Pts',(-23.6491292020382,13.6783221132163,
131.292281615599)) ;
#125773=CARTESIAN_POINT('Ctrl Pts',(-23.6242025058468,13.9701100820096,
131.18637040101)) ;
#125774=CARTESIAN_POINT('Ctrl Pts',(-23.5754565039934,14.2230345342298,
131.010845400058)) ;
#125775=CARTESIAN_POINT('Ctrl Pts',(-23.5070759200868,14.4186168912711,
130.777961630613)) ;
#125776=CARTESIAN_POINT('Ctrl Pts',(-23.4247733783215,14.5428705870382,
130.504432836877)) ;
#125777=CARTESIAN_POINT('Ctrl Pts',(-23.335040863465,14.5869069845901,130.209169715997)) ;
#125778=CARTESIAN_POINT('Ctrl Pts',(-23.2452918150756,14.5480013185182,
129.913943046972)) ;
#125779=CARTESIAN_POINT('Ctrl Pts',(-23.1617603223781,14.4271740783889,
129.63656787434)) ;
#125780=CARTESIAN_POINT('Ctrl Pts',(-23.09288452206,14.2362638793065,129.402438365019)) ;
#125781=CARTESIAN_POINT('Ctrl Pts',(-23.0427644300731,13.9863048350813,
129.222884594247)) ;
#125782=CARTESIAN_POINT('Ctrl Pts',(-23.0163956850893,13.6957298115947,
129.112709730807)) ;
#125783=CARTESIAN_POINT('Ctrl Pts',(-23.0161499853956,13.3866515588876,
129.078955426148)) ;
#125784=CARTESIAN_POINT('Ctrl Pts',(-23.0432652761747,13.0771469470951,
129.124786982275)) ;
#125785=CARTESIAN_POINT('Ctrl Pts',(-23.0956584483429,12.7963920748989,
129.244920648132)) ;
#125786=CARTESIAN_POINT('Ctrl Pts',(-23.1713250322537,12.5578779077828,
129.432708390056)) ;
#125787=CARTESIAN_POINT('Ctrl Pts',(-23.2644357106903,12.3830735450268,
129.671724285025)) ;
#125788=CARTESIAN_POINT('Ctrl Pts',(-23.3701067648639,12.2815115080033,
129.947250619451)) ;
#125789=CARTESIAN_POINT('Ctrl Pts',(-23.4813534599636,12.262368243914,130.238988514974)) ;
#125790=CARTESIAN_POINT('Ctrl Pts',(-23.5896531894837,12.3259184462842,
130.522415372058)) ;
#125791=CARTESIAN_POINT('Ctrl Pts',(-23.6896717899316,12.4680809705656,
130.78144439189)) ;
#125792=CARTESIAN_POINT('Ctrl Pts',(-23.7743174451553,12.6795623808911,
130.995497362049)) ;
#125793=CARTESIAN_POINT('Ctrl Pts',(-23.8377589698062,12.9425895546652,
131.147829833242)) ;
#125794=CARTESIAN_POINT('Ctrl Pts',(-23.8769867469141,13.2417283918,131.229213132218)) ;
#125795=CARTESIAN_POINT('Ctrl Pts',(-23.8893641527961,13.5531903661268,
131.232247085425)) ;
#125796=CARTESIAN_POINT('Ctrl Pts',(-23.8748957358541,13.8554129193782,
131.156838036651)) ;
#125797=CARTESIAN_POINT('Ctrl Pts',(-23.8355012217854,14.1261609524352,
131.008696352866)) ;
#125798=CARTESIAN_POINT('Ctrl Pts',(-23.7741527595749,14.3478085326463,
130.796199663414)) ;
#125799=CARTESIAN_POINT('Ctrl Pts',(-23.6971938021371,14.5013887047212,
130.538470256886)) ;
#125800=CARTESIAN_POINT('Ctrl Pts',(-23.6092831974912,14.5792263128841,
130.248399633376)) ;
#125801=CARTESIAN_POINT('Ctrl Pts',(-23.5187037661353,14.5735423168914,
129.950722272445)) ;
#125802=CARTESIAN_POINT('Ctrl Pts',(-23.4320925272048,14.4859391814988,
129.664603852775)) ;
#125803=CARTESIAN_POINT('Ctrl Pts',(-23.3561930515529,14.3210239309704,
129.409613726262)) ;
#125804=CARTESIAN_POINT('Ctrl Pts',(-23.2980515559861,14.0938128758495,
129.206821944333)) ;
#125805=CARTESIAN_POINT('Ctrl Pts',(-23.2615318957367,13.8165579042321,
129.066899333572)) ;
#125806=CARTESIAN_POINT('Ctrl Pts',(-23.2505619538317,13.5127263915299,
129.001820179472)) ;
#125807=CARTESIAN_POINT('Ctrl Pts',(-23.2666753004263,13.2000971209204,
129.015583001645)) ;
#125808=CARTESIAN_POINT('Ctrl Pts',(-23.3087944429129,12.907342662141,129.105770615746)) ;
#125809=CARTESIAN_POINT('Ctrl Pts',(-23.3756923407858,12.6479572241649,
129.267911443883)) ;
#125810=CARTESIAN_POINT('Ctrl Pts',(-23.4621286873441,12.4461100173765,
129.487427563302)) ;
#125811=CARTESIAN_POINT('Ctrl Pts',(-23.564127946314,12.3127706189861,129.752081916825)) ;
#125812=CARTESIAN_POINT('Ctrl Pts',(-23.6732755910501,12.2601401087974,
130.037940276038)) ;
#125813=CARTESIAN_POINT('Ctrl Pts',(-23.7838302243714,12.2901733256143,
130.327774440353)) ;
#125814=CARTESIAN_POINT('Ctrl Pts',(-23.8883010360076,12.4015833067204,
130.599812066351)) ;
#125815=CARTESIAN_POINT('Ctrl Pts',(-23.9798552045445,12.5866483791686,
130.834076178681)) ;
#125816=CARTESIAN_POINT('Ctrl Pts',(-24.0523151917746,12.8302723289068,
131.012741175065)) ;
#125817=CARTESIAN_POINT('Ctrl Pts',(-24.1019779789025,13.1192440261277,
131.124467731164)) ;
#125818=CARTESIAN_POINT('Ctrl Pts',(-24.1250931579403,13.4254781915307,
131.159155989376)) ;
#125819=CARTESIAN_POINT('Ctrl Pts',(-24.1215266149602,13.7353596810941,
131.11547066498)) ;
#125820=CARTESIAN_POINT('Ctrl Pts',(-24.0918980981446,14.0210482002996,
130.995860945524)) ;
#125821=CARTESIAN_POINT('Ctrl Pts',(-24.0389691525216,14.2649914716046,
130.808039376452)) ;
#125822=CARTESIAN_POINT('Ctrl Pts',(-23.9676201622106,14.4476747030691,
130.566553540134)) ;
#125823=CARTESIAN_POINT('Ctrl Pts',(-23.8833688710434,14.5574100040251,
130.287310728939)) ;
#125824=CARTESIAN_POINT('Ctrl Pts',(-23.7931596806364,14.5860647514156,
129.990703936635)) ;
#125825=CARTESIAN_POINT('Ctrl Pts',(-23.7035285456496,14.5307819261163,
129.695562869129)) ;
#125826=CARTESIAN_POINT('Ctrl Pts',(-23.6229992772553,14.3969445095406,
129.42733334663)) ;
#125827=CARTESIAN_POINT('Ctrl Pts',(-23.5567869860424,14.1927448984532,
129.200733935221)) ;
#125828=CARTESIAN_POINT('Ctrl Pts',(-23.5110190745614,13.93401239778,129.033964097782)) ;
#125829=CARTESIAN_POINT('Ctrl Pts',(-23.4893930698321,13.6381121003486,
128.93763672327)) ;
#125830=CARTESIAN_POINT('Ctrl Pts',(-23.494345890272,13.3270742285028,128.918987736531)) ;
#125831=CARTESIAN_POINT('Ctrl Pts',(-23.5262340039663,13.0225106106699,
128.978980037465)) ;
#125832=CARTESIAN_POINT('Ctrl Pts',(-23.5835789347515,12.7468019660475,
129.113339138239)) ;
#125833=CARTESIAN_POINT('Ctrl Pts',(-23.6624595718155,12.5205887293237,
129.310778341826)) ;
#125834=CARTESIAN_POINT('Ctrl Pts',(-23.7587447135317,12.3578209293796,
129.558896200725)) ;
#125835=CARTESIAN_POINT('Ctrl Pts',(-23.8658582136432,12.2716454717833,
129.838676166816)) ;
#125836=CARTESIAN_POINT('Ctrl Pts',(-23.9769093594406,12.2679543097138,
130.129953687869)) ;
#125837=CARTESIAN_POINT('Ctrl Pts',(-24.0845696446032,12.3469222200597,
130.411357159961)) ;
#125838=CARTESIAN_POINT('Ctrl Pts',(-24.1820649364697,12.503089881748,130.663027573452)) ;
#125839=CARTESIAN_POINT('Ctrl Pts',(-24.2629482232578,12.7250182855012,
130.866198402469)) ;
#125840=CARTESIAN_POINT('Ctrl Pts',(-24.3222955108618,12.9971829063299,
131.006424325435)) ;
#125841=CARTESIAN_POINT('Ctrl Pts',(-24.3564639158183,13.2997829333183,
131.07311023844)) ;
#125842=CARTESIAN_POINT('Ctrl Pts',(-24.3637810053582,13.6108911186927,
131.061388804265)) ;
#125843=CARTESIAN_POINT('Ctrl Pts',(-24.3445179230017,13.9087324272285,
130.972007256068)) ;
#125844=CARTESIAN_POINT('Ctrl Pts',(-24.3005201013976,14.1725576742086,
130.810259178625)) ;
#125845=CARTESIAN_POINT('Ctrl Pts',(-24.2360759456044,14.3815588265502,
130.588935069275)) ;
#125846=CARTESIAN_POINT('Ctrl Pts',(-24.1562702964475,14.5223296073452,
130.322687297205)) ;
#125847=CARTESIAN_POINT('Ctrl Pts',(-24.0676167127849,14.5844939687617,
130.030606234737)) ;
#125848=CARTESIAN_POINT('Ctrl Pts',(-23.9768242528743,14.5631534202887,
129.732143036026)) ;
#125849=CARTESIAN_POINT('Ctrl Pts',(-23.892015745999,14.4606750911625,129.451383600056)) ;
#125850=CARTESIAN_POINT('Ctrl Pts',(-23.8188724297923,14.2826953933965,
129.204438549508)) ;
#125851=CARTESIAN_POINT('Ctrl Pts',(-23.7644837114012,14.0447463333177,
129.01256424196)) ;
#125852=CARTESIAN_POINT('Ctrl Pts',(-23.7326129631891,13.7613771036905,
128.886315694404)) ;
#125853=CARTESIAN_POINT('Ctrl Pts',(-23.7266140527177,13.4542323232824,
128.835707264658)) ;
#125854=CARTESIAN_POINT('Ctrl Pts',(-23.7476478247381,13.143799460901,128.86395007119)) ;
#125855=CARTESIAN_POINT('Ctrl Pts',(-23.7949823521457,12.8538469192422,
128.969069945321)) ;
#125856=CARTESIAN_POINT('Ctrl Pts',(-23.8656813263339,12.6054873495862,
129.142536871026)) ;
#125857=CARTESIAN_POINT('Ctrl Pts',(-23.9553690976935,12.4153273206803,
129.37150786963)) ;
#125858=CARTESIAN_POINT('Ctrl Pts',(-24.0596667735144,12.2964112458501,
129.642812186469)) ;
#125859=CARTESIAN_POINT('Ctrl Pts',(-24.169433739975,12.2594155900217,129.930515923544)) ;
#125860=CARTESIAN_POINT('Ctrl Pts',(-24.279602294317,12.3053349442499,130.2191500822)) ;
#125861=CARTESIAN_POINT('Ctrl Pts',(-24.3818019884218,12.4312259098382,
130.484643983243)) ;
#125862=CARTESIAN_POINT('Ctrl Pts',(-24.4700626756975,12.6279597260861,
130.709377871418)) ;
#125863=CARTESIAN_POINT('Ctrl Pts',(-24.5387653735917,12.8824933120028,
130.876882524073)) ;
#125864=CARTESIAN_POINT('Ctrl Pts',(-24.5833076087164,13.1745455822002,
130.973954429722)) ;
#125865=CARTESIAN_POINT('Ctrl Pts',(-24.6016723074617,13.485175620818,130.994463005875)) ;
#125866=CARTESIAN_POINT('Ctrl Pts',(-24.5929092913481,13.7921379938219,
130.935634698017)) ;
#125867=CARTESIAN_POINT('Ctrl Pts',(-24.5586761808863,14.0710148384314,
130.802596578121)) ;
#125868=CARTESIAN_POINT('Ctrl Pts',(-24.501845620011,14.3045452555015,130.603399975795)) ;
#125869=CARTESIAN_POINT('Ctrl Pts',(-24.4277830561673,14.4740866338348,
130.35405191635)) ;
#125870=CARTESIAN_POINT('Ctrl Pts',(-24.3415214169763,14.5693022561264,
130.068806329395)) ;
#125871=CARTESIAN_POINT('Ctrl Pts',(-24.2510875787444,14.582012624519,129.771588629195)) ;
#125872=CARTESIAN_POINT('Ctrl Pts',(-24.1625305892248,14.5112270801159,
129.47959734592)) ;
#125873=CARTESIAN_POINT('Ctrl Pts',(-24.0843973310296,14.3635590913307,
129.218403125075)) ;
#125874=CARTESIAN_POINT('Ctrl Pts',(-24.021647896778,14.1479538826623,129.001944571865)) ;
#125875=CARTESIAN_POINT('Ctrl Pts',(-23.9801215750542,13.8806546187411,
128.847536590297)) ;
#125876=CARTESIAN_POINT('Ctrl Pts',(-23.963342779706,13.5796272829373,128.765311315185)) ;
#125877=CARTESIAN_POINT('Ctrl Pts',(-23.9735252945803,13.2675901061276,
128.761875234646)) ;
#125878=CARTESIAN_POINT('Ctrl Pts',(-24.0101803838354,12.9685391977506,
128.835981940567)) ;
#125879=CARTESIAN_POINT('Ctrl Pts',(-24.0719166755097,12.7001826766663,
128.98314530386)) ;
#125880=CARTESIAN_POINT('Ctrl Pts',(-24.1546536581567,12.4843513272629,
129.191756252885)) ;
#125881=CARTESIAN_POINT('Ctrl Pts',(-24.2535322461022,12.3354377542164,
129.447446958892)) ;
#125882=CARTESIAN_POINT('Ctrl Pts',(-24.3616167437817,12.2645466478322,
129.730158751956)) ;
#125883=CARTESIAN_POINT('Ctrl Pts',(-24.4731438929875,12.276740062036,130.022661709796)) ;
#125884=CARTESIAN_POINT('Ctrl Pts',(-24.5790748900288,12.3708039289104,
130.299107143294)) ;
#125885=CARTESIAN_POINT('Ctrl Pts',(-24.6739671483137,12.5405714665883,
130.543143809825)) ;
#125886=CARTESIAN_POINT('Ctrl Pts',(-24.7509668752168,12.7727637010119,
130.735041912881)) ;
#125887=CARTESIAN_POINT('Ctrl Pts',(-24.8059943713008,13.0532482908803,
130.862531034195)) ;
#125888=CARTESIAN_POINT('Ctrl Pts',(-24.8350568114348,13.3594504233503,
130.914284039588)) ;
#125889=CARTESIAN_POINT('Ctrl Pts',(-24.8372623159899,13.6687251009062,
130.887737753365)) ;
#125890=CARTESIAN_POINT('Ctrl Pts',(-24.8130625569726,13.9622484425501,
130.78385263984)) ;
#125891=CARTESIAN_POINT('Ctrl Pts',(-24.7649704899683,14.2163837439272,
130.610262407807)) ;
#125892=CARTESIAN_POINT('Ctrl Pts',(-24.696901125032,14.4143549492585,130.378200623285)) ;
#125893=CARTESIAN_POINT('Ctrl Pts',(-24.6148829741244,14.5404303849103,
130.105507473975)) ;
#125894=CARTESIAN_POINT('Ctrl Pts',(-24.5256465957694,14.5868747911533,
129.811836591317)) ;
#125895=CARTESIAN_POINT('Ctrl Pts',(-24.4352900112969,14.5499212467829,
129.514634417336)) ;
#125896=CARTESIAN_POINT('Ctrl Pts',(-24.3521632833049,14.4324626312606,
129.238736296956)) ;
#125897=CARTESIAN_POINT('Ctrl Pts',(-24.282156962627,14.2419356966938,129.001005963156)) ;
#125898=CARTESIAN_POINT('Ctrl Pts',(-24.2316886119294,13.9939564791264,
128.820547864145)) ;
#125899=CARTESIAN_POINT('Ctrl Pts',(-24.2045556444576,13.7043181769273,
128.708138252988)) ;
#125900=CARTESIAN_POINT('Ctrl Pts',(-24.2036086367596,13.395369790062,128.672323138478)) ;
#125901=CARTESIAN_POINT('Ctrl Pts',(-24.2297557957195,13.086808383261,128.715476371712)) ;
#125902=CARTESIAN_POINT('Ctrl Pts',(-24.2816715668208,12.8035341555048,
128.834042913763)) ;
#125903=CARTESIAN_POINT('Ctrl Pts',(-24.3566659267985,12.5639567351557,
129.019921579767)) ;
#125904=CARTESIAN_POINT('Ctrl Pts',(-24.4495112025863,12.3867441251715,
129.258096186901)) ;
#125905=CARTESIAN_POINT('Ctrl Pts',(-24.555139738116,12.2832559633923,129.533444706346)) ;
#125906=CARTESIAN_POINT('Ctrl Pts',(-24.6653725410066,12.2616345665819,
129.822511029336)) ;
#125907=CARTESIAN_POINT('Ctrl Pts',(-24.7747128452521,12.3231638960011,
130.108706425634)) ;
#125908=CARTESIAN_POINT('Ctrl Pts',(-24.8746113532042,12.4627500215576,
130.367538216252)) ;
#125909=CARTESIAN_POINT('Ctrl Pts',(-24.9600355501279,12.6729053974916,
130.583771384125)) ;
#125910=CARTESIAN_POINT('Ctrl Pts',(-25.0240609203247,12.9344260822497,
130.737847424504)) ;
#125911=CARTESIAN_POINT('Ctrl Pts',(-25.0641198333657,13.234077565713,130.821527263044)) ;
#125912=CARTESIAN_POINT('Ctrl Pts',(-25.0771308739537,13.5439039553039,
130.826581768022)) ;
#125913=CARTESIAN_POINT('Ctrl Pts',(-25.0635214617943,13.8465582342306,
130.753703399045)) ;
#125914=CARTESIAN_POINT('Ctrl Pts',(-25.0247696848298,14.1188040415087,
130.607401020676)) ;
#125915=CARTESIAN_POINT('Ctrl Pts',(-24.9640862870837,14.3420291426398,
130.396887886905)) ;
#125916=CARTESIAN_POINT('Ctrl Pts',(-24.8872853575658,14.4980360771653,
130.13952226897)) ;
#125917=CARTESIAN_POINT('Ctrl Pts',(-24.8000024335385,14.5780642539032,
129.85144765031)) ;
#125918=CARTESIAN_POINT('Ctrl Pts',(-24.7087046539535,14.5747644514925,
129.551409158721)) ;
#125919=CARTESIAN_POINT('Ctrl Pts',(-24.6223739304756,14.489550077403,129.266289535855)) ;
#125920=CARTESIAN_POINT('Ctrl Pts',(-24.5461701581343,14.3274511232625,
129.010484644828)) ;
#125921=CARTESIAN_POINT('Ctrl Pts',(-24.4872263455305,14.10121310871,128.805238001483)) ;
#125922=CARTESIAN_POINT('Ctrl Pts',(-24.4500072639137,13.8249843797631,
128.663265474858)) ;
#125923=CARTESIAN_POINT('Ctrl Pts',(-24.438327381082,13.5214320860101,128.59608615518)) ;
#125924=CARTESIAN_POINT('Ctrl Pts',(-24.4534890626492,13.2103011439188,
128.607246943733)) ;
#125925=CARTESIAN_POINT('Ctrl Pts',(-24.495066640313,12.9148531024708,128.695641378851)) ;
#125926=CARTESIAN_POINT('Ctrl Pts',(-24.5613915132952,12.6543477240414,
128.856118206563)) ;
#125927=CARTESIAN_POINT('Ctrl Pts',(-24.6471825551665,12.4511188454898,
129.073804541509)) ;
#125928=CARTESIAN_POINT('Ctrl Pts',(-24.7486084980389,12.3156705346788,
129.336853062175)) ;
#125929=CARTESIAN_POINT('Ctrl Pts',(-24.8581128521185,12.2603783289395,
129.62360453636)) ;
#125930=CARTESIAN_POINT('Ctrl Pts',(-24.9686726023263,12.2883877322888,
129.913470195239)) ;
#125931=CARTESIAN_POINT('Ctrl Pts',(-25.0729932645916,12.396958266653,130.185207408956)) ;
#125932=CARTESIAN_POINT('Ctrl Pts',(-25.1653592270199,12.5805839766397,
130.421729388471)) ;
#125933=CARTESIAN_POINT('Ctrl Pts',(-25.2382239831384,12.8225431268309,
130.601623820474)) ;
#125934=CARTESIAN_POINT('Ctrl Pts',(-25.2885089962269,13.1085293602313,
130.715378449147)) ;
#125935=CARTESIAN_POINT('Ctrl Pts',(-25.3126600961537,13.4184312820959,
130.752658836677)) ;
#125936=CARTESIAN_POINT('Ctrl Pts',(-25.3098210842849,13.725396855158,130.711452962924)) ;
#125937=CARTESIAN_POINT('Ctrl Pts',(-25.2808102713298,14.0140710233184,
130.593415477902)) ;
#125938=CARTESIAN_POINT('Ctrl Pts',(-25.2285495788724,14.2586953082214,
130.407640473417)) ;
#125939=CARTESIAN_POINT('Ctrl Pts',(-25.1575885801058,14.4435712393275,
130.167243122289)) ;
#125940=CARTESIAN_POINT('Ctrl Pts',(-25.0736237827417,14.5554638081498,
129.888850792781)) ;
#125941=CARTESIAN_POINT('Ctrl Pts',(-24.9833949472367,14.5862678501096,
129.592148597905)) ;
#125942=CARTESIAN_POINT('Ctrl Pts',(-24.8942273387361,14.5339455279845,
129.298592022686)) ;
#125943=CARTESIAN_POINT('Ctrl Pts',(-24.8129142069753,14.4019055584218,
129.027901950915)) ;
#125944=CARTESIAN_POINT('Ctrl Pts',(-24.746276318339,14.1996929308369,128.800099500665)) ;
#125945=CARTESIAN_POINT('Ctrl Pts',(-24.699763961038,13.9418839763085,128.631093588378)) ;
#125946=CARTESIAN_POINT('Ctrl Pts',(-24.6774338462082,13.6467945517117,
128.532720399714)) ;
#125947=CARTESIAN_POINT('Ctrl Pts',(-24.6816242532169,13.3358857358536,
128.511842088529)) ;
#125948=CARTESIAN_POINT('Ctrl Pts',(-24.7127138700083,13.0311283359512,
128.569538090796)) ;
#125949=CARTESIAN_POINT('Ctrl Pts',(-24.7693523753043,12.7543595067604,
128.70183682194)) ;
#125950=CARTESIAN_POINT('Ctrl Pts',(-24.8475655059419,12.5263863833961,
128.897344080859)) ;
#125951=CARTESIAN_POINT('Ctrl Pts',(-24.9442364116292,12.3607017684255,
129.146334817841)) ;
#125952=CARTESIAN_POINT('Ctrl Pts',(-25.0501716622116,12.2732420029804,
129.422981311838)) ;
#125953=CARTESIAN_POINT('Ctrl Pts',(-25.161642701429,12.2668291294782,129.715349818511)) ;
#125954=CARTESIAN_POINT('Ctrl Pts',(-25.2694224447278,12.3436152480751,
129.997125883339)) ;
#125955=CARTESIAN_POINT('Ctrl Pts',(-25.3674136502751,12.4979168003383,
130.250203723664)) ;
#125956=CARTESIAN_POINT('Ctrl Pts',(-25.4487609142858,12.7181781437397,
130.454748013193)) ;
#125957=CARTESIAN_POINT('Ctrl Pts',(-25.5086898509027,12.9887185054322,
130.596726594436)) ;
#125958=CARTESIAN_POINT('Ctrl Pts',(-25.5436429825189,13.2908827967775,
130.665687047163)) ;
#125959=CARTESIAN_POINT('Ctrl Pts',(-25.5517475698564,13.6021684785122,
130.656255124618)) ;
#125960=CARTESIAN_POINT('Ctrl Pts',(-25.5331239691341,13.901537415506,130.568644647974)) ;
#125961=CARTESIAN_POINT('Ctrl Pts',(-25.48972374552,14.1661758295122,130.408674325154)) ;
#125962=CARTESIAN_POINT('Ctrl Pts',(-25.4260099872032,14.3763137224392,
130.189586864129)) ;
#125963=CARTESIAN_POINT('Ctrl Pts',(-25.3463659017589,14.5195379343594,
129.923731245516)) ;
#125964=CARTESIAN_POINT('Ctrl Pts',(-25.2580898168815,14.5837467777198,
129.632838255193)) ;
#125965=CARTESIAN_POINT('Ctrl Pts',(-25.1673248310042,14.5651055472896,
129.334485888311)) ;
#125966=CARTESIAN_POINT('Ctrl Pts',(-25.0819869198981,14.4645028537766,
129.052069731339)) ;
#125967=CARTESIAN_POINT('Ctrl Pts',(-25.0086540266316,14.2890439615902,
128.80468090298)) ;
#125968=CARTESIAN_POINT('Ctrl Pts',(-24.9535847938953,14.0526944517644,
128.610802322953)) ;
#125969=CARTESIAN_POINT('Ctrl Pts',(-24.9209684987911,13.7699865640071,
128.482334359054)) ;
#125970=CARTESIAN_POINT('Ctrl Pts',(-24.914161154007,13.4631529119525,128.429358281431)) ;
#125971=CARTESIAN_POINT('Ctrl Pts',(-24.9346241902268,13.1513620896954,
128.455804728885)) ;
#125972=CARTESIAN_POINT('Ctrl Pts',(-24.9808286764254,12.8627668245119,
128.557889451478)) ;
#125973=CARTESIAN_POINT('Ctrl Pts',(-25.0514554263938,12.6109028721184,
128.730870773543)) ;
#125974=CARTESIAN_POINT('Ctrl Pts',(-25.1403206144582,12.4200193080497,
128.957599041015)) ;
#125975=CARTESIAN_POINT('Ctrl Pts',(-25.2443570951015,12.298694725006,129.228115799905)) ;
#125976=CARTESIAN_POINT('Ctrl Pts',(-25.3538813352196,12.2592723921271,
129.515159745908)) ;
#125977=CARTESIAN_POINT('Ctrl Pts',(-25.4644961600716,12.3030853474822,
129.804989192264)) ;
#125978=CARTESIAN_POINT('Ctrl Pts',(-25.5664737135498,12.4259705793417,
130.070018363366)) ;
#125979=CARTESIAN_POINT('Ctrl Pts',(-25.6558186570055,12.6220550039555,
130.297698340302)) ;
#125980=CARTESIAN_POINT('Ctrl Pts',(-25.7248599756662,12.8744669424422,
130.466310011983)) ;
#125981=CARTESIAN_POINT('Ctrl Pts',(-25.7702434103864,13.1663406139675,
130.565761336406)) ;
#125982=CARTESIAN_POINT('Ctrl Pts',(-25.78925027389,13.475878892664,130.588240800229)) ;
#125983=CARTESIAN_POINT('Ctrl Pts',(-25.7814468787295,13.7823953075606,
130.532325836571)) ;
#125984=CARTESIAN_POINT('Ctrl Pts',(-25.7476177585212,14.064418215805,130.400208232113)) ;
#125985=CARTESIAN_POINT('Ctrl Pts',(-25.6918077811808,14.2977471414108,
130.204255542855)) ;
#125986=CARTESIAN_POINT('Ctrl Pts',(-25.6177147063912,14.4706194179794,
129.95458823605)) ;
#125987=CARTESIAN_POINT('Ctrl Pts',(-25.5319450619605,14.5675955159237,
129.670894736031)) ;
#125988=CARTESIAN_POINT('Ctrl Pts',(-25.4414971518042,14.5827755983601,
129.373610278919)) ;
#125989=CARTESIAN_POINT('Ctrl Pts',(-25.3531231344059,14.5148008413574,
129.082293968107)) ;
#125990=CARTESIAN_POINT('Ctrl Pts',(-25.2743161800529,14.3692242855325,
128.81903385639)) ;
#125991=CARTESIAN_POINT('Ctrl Pts',(-25.2107747912008,14.1540994204916,
128.600098438583)) ;
#125992=CARTESIAN_POINT('Ctrl Pts',(-25.168846979142,13.889194577701,128.444675356342)) ;
#125993=CARTESIAN_POINT('Ctrl Pts',(-25.1512494519835,13.5894848313417,
128.36011954352)) ;
#125994=CARTESIAN_POINT('Ctrl Pts',(-25.1605845207115,13.2771021698192,
128.354170238193)) ;
#125995=CARTESIAN_POINT('Ctrl Pts',(-25.1965224543068,12.9767128859996,
128.426111454514)) ;
#125996=CARTESIAN_POINT('Ctrl Pts',(-25.2578937374659,12.7063601582146,
128.572090875043)) ;
#125997=CARTESIAN_POINT('Ctrl Pts',(-25.3396420278382,12.4901609157503,
128.778005457338)) ;
#125998=CARTESIAN_POINT('Ctrl Pts',(-25.4381908746274,12.338688213011,129.032699044275)) ;
#125999=CARTESIAN_POINT('Ctrl Pts',(-25.5463110659534,12.2654833215425,
129.315451748126)) ;
#126000=CARTESIAN_POINT('Ctrl Pts',(-25.6574951807458,12.2750423939134,
129.607066941372)) ;
#126001=CARTESIAN_POINT('Ctrl Pts',(-25.7642010115431,12.3673309477628,
129.885602094051)) ;
#126002=CARTESIAN_POINT('Ctrl Pts',(-25.8590365897066,12.5343469793072,
130.129637220304)) ;
#126003=CARTESIAN_POINT('Ctrl Pts',(-25.9368382713176,12.7652871615339,
130.32380307639)) ;
#126004=CARTESIAN_POINT('Ctrl Pts',(-25.9924735837026,13.0444119641298,
130.453106439739)) ;
#126005=CARTESIAN_POINT('Ctrl Pts',(-26.0223929863957,13.3498617711502,
130.507389727664)) ;
#126006=CARTESIAN_POINT('Ctrl Pts',(-26.0253114098023,13.6613615410962,
130.482703869082)) ;
#126007=CARTESIAN_POINT('Ctrl Pts',(-26.0019147375177,13.9537822456917,
130.381373854376)) ;
#126008=CARTESIAN_POINT('Ctrl Pts',(-25.9544927342726,14.2096141723503,
130.209713801522)) ;
#126009=CARTESIAN_POINT('Ctrl Pts',(-25.8870673150101,14.4090573352496,
129.979600499692)) ;
#126010=CARTESIAN_POINT('Ctrl Pts',(-25.8054312777494,14.5378227777349,
129.70802666148)) ;
#126011=CARTESIAN_POINT('Ctrl Pts',(-25.7156142292361,14.5866410232384,
129.41240035545)) ;
#126012=CARTESIAN_POINT('Ctrl Pts',(-25.6260309545434,14.5524956968184,
129.117784907284)) ;
#126013=CARTESIAN_POINT('Ctrl Pts',(-25.5418482572694,14.4363359787846,
128.838493567448)) ;
#126014=CARTESIAN_POINT('Ctrl Pts',(-25.4718915415956,14.2487612531945,
128.601139063692)) ;
#126015=CARTESIAN_POINT('Ctrl Pts',(-25.42063882581,14.0019963672536,128.4183229551)) ;
#126016=CARTESIAN_POINT('Ctrl Pts',(-25.392749544608,13.7133413750086,128.303718197207)) ;
#126017=CARTESIAN_POINT('Ctrl Pts',(-25.391107247378,13.4034231078491,128.265734684646)) ;
#126018=CARTESIAN_POINT('Ctrl Pts',(-25.4162654592174,13.0966156009071,
128.306236353819)) ;
#126019=CARTESIAN_POINT('Ctrl Pts',(-25.4677661028884,12.8104956204696,
128.423372058635)) ;
#126020=CARTESIAN_POINT('Ctrl Pts',(-25.5418005766506,12.5707042349948,
128.606625724916)) ;
#126021=CARTESIAN_POINT('Ctrl Pts',(-25.6343027539285,12.3910193657153,
128.84373772453)) ;
#126022=CARTESIAN_POINT('Ctrl Pts',(-25.7394215596981,12.285328864528,129.117673474855)) ;
#126023=CARTESIAN_POINT('Ctrl Pts',(-25.8499618498709,12.2609818529467,
129.407525601254)) ;
#126024=CARTESIAN_POINT('Ctrl Pts',(-25.9597380713748,12.3204757590526,
129.694909016279)) ;
#126025=CARTESIAN_POINT('Ctrl Pts',(-26.0599411656007,12.4582515921679,
129.954624240264)) ;
#126026=CARTESIAN_POINT('Ctrl Pts',(-26.145604357151,12.6658998652864,130.171670188794)) ;
#126027=CARTESIAN_POINT('Ctrl Pts',(-26.2103851275808,12.9268096194457,
130.32787211021)) ;
#126028=CARTESIAN_POINT('Ctrl Pts',(-26.2509404211424,13.2233761882574,
130.413261942169)) ;
#126029=CARTESIAN_POINT('Ctrl Pts',(-26.2649718352972,13.5346577028184,
130.421128557714)) ;
#126030=CARTESIAN_POINT('Ctrl Pts',(-26.2520240327405,13.8387961550216,
130.350083552355)) ;
#126031=CARTESIAN_POINT('Ctrl Pts',(-26.2138395505756,14.1123018093557,
130.205408086112)) ;
#126032=CARTESIAN_POINT('Ctrl Pts',(-26.153839721311,14.3364687446635,129.996980303238)) ;
#126033=CARTESIAN_POINT('Ctrl Pts',(-26.0774343121864,14.494770833943,129.74076290921)) ;
#126034=CARTESIAN_POINT('Ctrl Pts',(-25.9899586435841,14.5769227995843,
129.45198478666)) ;
#126035=CARTESIAN_POINT('Ctrl Pts',(-25.8997042911877,14.5762675412157,
129.155383645879)) ;
#126036=CARTESIAN_POINT('Ctrl Pts',(-25.812384586297,14.4930554177443,128.867083845034)) ;
#126037=CARTESIAN_POINT('Ctrl Pts',(-25.73597860465,14.3331650364545,128.610769594454)) ;
#126038=CARTESIAN_POINT('Ctrl Pts',(-25.6763576726058,14.1081176093321,
128.403470945939)) ;
#126039=CARTESIAN_POINT('Ctrl Pts',(-25.6385794389391,13.8340178637995,
128.259988320297)) ;
#126040=CARTESIAN_POINT('Ctrl Pts',(-25.6260661068604,13.5302898798933,
128.190290082024)) ;
#126041=CARTESIAN_POINT('Ctrl Pts',(-25.6404465317525,13.2194241455141,
128.199211501796)) ;
#126042=CARTESIAN_POINT('Ctrl Pts',(-25.6812553568026,12.9232187981691,
128.285358188475)) ;
#126043=CARTESIAN_POINT('Ctrl Pts',(-25.7468433316738,12.6614612454166,
128.443705997656)) ;
#126044=CARTESIAN_POINT('Ctrl Pts',(-25.8322906105427,12.4560560128417,
128.660322270214)) ;
#126045=CARTESIAN_POINT('Ctrl Pts',(-25.9330424236509,12.3187614460116,
128.921508759944)) ;
#126046=CARTESIAN_POINT('Ctrl Pts',(-26.0425569662323,12.2608758912203,
129.208234980341)) ;
#126047=CARTESIAN_POINT('Ctrl Pts',(-26.1530140665807,12.2860567579314,
129.497863653022)) ;
#126048=CARTESIAN_POINT('Ctrl Pts',(-26.2585079710758,12.3936760882031,
129.772722456645)) ;
#126049=CARTESIAN_POINT('Ctrl Pts',(-26.3503095104322,12.5734427246259,
130.007962979543)) ;
#126050=CARTESIAN_POINT('Ctrl Pts',(-26.4244433834245,12.8155556850103,
130.191300268138)) ;
#126051=CARTESIAN_POINT('Ctrl Pts',(-26.4751724700827,13.1001458972495,
130.306431104727)) ;
#126052=CARTESIAN_POINT('Ctrl Pts',(-26.5000925783719,13.4082451879306,
130.346105536368)) ;
#126053=CARTESIAN_POINT('Ctrl Pts',(-26.4980891723479,13.7170001803432,
130.307186038938)) ;
#126054=CARTESIAN_POINT('Ctrl Pts',(-26.4696671842496,14.0068803402206,
130.190824498522)) ;
#126055=CARTESIAN_POINT('Ctrl Pts',(-26.4181820684679,14.2520830293328,
130.007428300008)) ;
#126056=CARTESIAN_POINT('Ctrl Pts',(-26.3478207017117,14.4388654830233,
129.768822234995)) ;
#126057=CARTESIAN_POINT('Ctrl Pts',(-26.2640576549974,14.5532758732377,
129.490979404376)) ;
#126058=CARTESIAN_POINT('Ctrl Pts',(-26.1738376378664,14.5866372920254,
129.194279342961)) ;
#126059=CARTESIAN_POINT('Ctrl Pts',(-26.0842975023075,14.5363254176441,
128.899536369528)) ;
#126060=CARTESIAN_POINT('Ctrl Pts',(-26.0030217669562,14.4070821621483,
128.629108370544)) ;
#126061=CARTESIAN_POINT('Ctrl Pts',(-25.9355456978039,14.2058492083664,
128.398700995927)) ;
#126062=CARTESIAN_POINT('Ctrl Pts',(-25.8885241340143,13.9493209948446,
128.22822873028)) ;
#126063=CARTESIAN_POINT('Ctrl Pts',(-25.8655269249234,13.6560816427411,
128.12802385383)) ;
#126064=CARTESIAN_POINT('Ctrl Pts',(-25.8688947460715,13.3454213686902,
128.104749085037)) ;
#126065=CARTESIAN_POINT('Ctrl Pts',(-25.8990663345431,13.0405957785926,
128.159818838281)) ;
#126066=CARTESIAN_POINT('Ctrl Pts',(-25.9553167132455,12.761020315257,128.290787259896)) ;
#126067=CARTESIAN_POINT('Ctrl Pts',(-26.0329645870705,12.5320804704421,
128.484687748095)) ;
#126068=CARTESIAN_POINT('Ctrl Pts',(-26.1284887813019,12.3651153247515,
128.730556130345)) ;
#126069=CARTESIAN_POINT('Ctrl Pts',(-26.2350764396969,12.2743249868604,
129.008828559484)) ;
#126070=CARTESIAN_POINT('Ctrl Pts',(-26.3465970340771,12.2660445265336,
129.301326003185)) ;
#126071=CARTESIAN_POINT('Ctrl Pts',(-26.4541471683152,12.3402671637665,
129.582555856666)) ;
#126072=CARTESIAN_POINT('Ctrl Pts',(-26.552555555769,12.492431210345,129.836844563032)) ;
#126073=CARTESIAN_POINT('Ctrl Pts',(-26.634360399724,12.7106681794057,130.042767093069)) ;
#126074=CARTESIAN_POINT('Ctrl Pts',(-26.6951305941108,12.9803450583886,
130.187151429511)) ;
#126075=CARTESIAN_POINT('Ctrl Pts',(-26.7308734422664,13.2833171432177,
130.258272185674)) ;
#126076=CARTESIAN_POINT('Ctrl Pts',(-26.7396663356869,13.5926828813481,
130.251062592622)) ;
#126077=CARTESIAN_POINT('Ctrl Pts',(-26.7217809067384,13.8936498651441,
130.165504550532)) ;
#126078=CARTESIAN_POINT('Ctrl Pts',(-26.6791273969298,14.1589431067745,
130.007795968708)) ;
#126079=CARTESIAN_POINT('Ctrl Pts',(-26.6158454773809,14.3711507970921,
129.789913035813)) ;
#126080=CARTESIAN_POINT('Ctrl Pts',(-26.5368498372877,14.5162610816314,
129.526063678826)) ;
#126081=CARTESIAN_POINT('Ctrl Pts',(-26.4480058430415,14.583306350133,129.233236326082)) ;
#126082=CARTESIAN_POINT('Ctrl Pts',(-26.3574400513536,14.5665129586633,
128.93555561929)) ;
#126083=CARTESIAN_POINT('Ctrl Pts',(-26.2721691927967,14.4685223967189,
128.653448871717)) ;
#126084=CARTESIAN_POINT('Ctrl Pts',(-26.1984352857841,14.2954966012034,
128.404931525748)) ;
#126085=CARTESIAN_POINT('Ctrl Pts',(-26.1425694482062,14.0596946296019,
128.208585964953)) ;
#126086=CARTESIAN_POINT('Ctrl Pts',(-26.1092924899254,13.7784555956093,
128.078249514083)) ;
#126087=CARTESIAN_POINT('Ctrl Pts',(-26.1018692508435,13.4704205391721,
128.02329757689)) ;
#126088=CARTESIAN_POINT('Ctrl Pts',(-26.1211722195802,13.1626906793203,
128.046828877772)) ;
#126089=CARTESIAN_POINT('Ctrl Pts',(-26.1671025371893,12.8697533216184,
128.147711848821)) ;
#126090=CARTESIAN_POINT('Ctrl Pts',(-26.2364647283035,12.6186668370347,
128.317310814944)) ;
#126091=CARTESIAN_POINT('Ctrl Pts',(-26.3256526534725,12.4240570551779,
128.544661301817)) ;
#126092=CARTESIAN_POINT('Ctrl Pts',(-26.4282836894432,12.301712902155,128.811435711836)) ;
#126093=CARTESIAN_POINT('Ctrl Pts',(-26.5385014971337,12.2592124433866,
129.100247411797)) ;
#126094=CARTESIAN_POINT('Ctrl Pts',(-26.648676203193,12.3002004237818,129.388972536211)) ;
#126095=CARTESIAN_POINT('Ctrl Pts',(-26.7520297398877,12.4222100081088,
129.657665386469)) ;
#126096=CARTESIAN_POINT('Ctrl Pts',(-26.8411055662838,12.6151763804986,
129.88482406291)) ;
#126097=CARTESIAN_POINT('Ctrl Pts',(-26.9110238859048,12.866763553233,130.055895668219)) ;
#126098=CARTESIAN_POINT('Ctrl Pts',(-26.9569593910413,13.1566083036236,
130.157097759597)) ;
#126099=CARTESIAN_POINT('Ctrl Pts',(-26.9769152324821,13.4669635155183,
130.182234691764)) ;
#126100=CARTESIAN_POINT('Ctrl Pts',(-26.9697491794495,13.7743605860558,
130.128124278071)) ;
#126101=CARTESIAN_POINT('Ctrl Pts',(-26.9369099290201,14.0556835712851,
129.999115173521)) ;
#126102=CARTESIAN_POINT('Ctrl Pts',(-26.8813890693662,14.2923698679386,
129.803785415256)) ;
#126103=CARTESIAN_POINT('Ctrl Pts',(-26.8075624299722,14.4669398360514,
129.554865852864)) ;
#126104=CARTESIAN_POINT('Ctrl Pts',(-26.7225333981472,14.5658237204842,
129.273523926098)) ;
#126105=CARTESIAN_POINT('Ctrl Pts',(-26.6316073168798,14.5834030750835,
128.974644654919)) ;
#126106=CARTESIAN_POINT('Ctrl Pts',(-26.5435523900135,14.5182209369221,
128.68445694957)) ;
#126107=CARTESIAN_POINT('Ctrl Pts',(-26.4637060287768,14.3732472228341,
128.41785071339)) ;
#126108=CARTESIAN_POINT('Ctrl Pts',(-26.4003065211889,14.161734042983,128.199658464977)) ;
#126109=CARTESIAN_POINT('Ctrl Pts',(-26.3573928265329,13.8968738672396,
128.041174467491)) ;
#126110=CARTESIAN_POINT('Ctrl Pts',(-26.3391569924333,13.5970560174392,
127.954689223546)) ;
#126111=CARTESIAN_POINT('Ctrl Pts',(-26.3477971534029,13.285349771455,127.946776708797)) ;
#126112=CARTESIAN_POINT('Ctrl Pts',(-26.3828895156986,12.9854213227035,
128.016359458515)) ;
#126113=CARTESIAN_POINT('Ctrl Pts',(-26.4432873742687,12.7145025865389,
128.159598142136)) ;
#126114=CARTESIAN_POINT('Ctrl Pts',(-26.5248365779504,12.4953422149561,
128.364769418823)) ;
#126115=CARTESIAN_POINT('Ctrl Pts',(-26.6231996145882,12.3417857538749,
128.618871219026)) ;
#126116=CARTESIAN_POINT('Ctrl Pts',(-26.7308273833783,12.2665368093941,
128.900280109487)) ;
#126117=CARTESIAN_POINT('Ctrl Pts',(-26.8419112559872,12.2735361740405,
129.191636843919)) ;
#126118=CARTESIAN_POINT('Ctrl Pts',(-26.9488113349784,12.3632299565235,
129.470758505725)) ;
#126119=CARTESIAN_POINT('Ctrl Pts',(-27.044382308045,12.5286847950401,129.716836311528)) ;
#126120=CARTESIAN_POINT('Ctrl Pts',(-27.122663508425,12.7579694730324,129.912424964013)) ;
#126121=CARTESIAN_POINT('Ctrl Pts',(-27.1789063470941,13.0352202971202,
130.043587032945)) ;
#126122=CARTESIAN_POINT('Ctrl Pts',(-27.2096612668745,13.3405829184085,
130.100263246823)) ;
#126123=CARTESIAN_POINT('Ctrl Pts',(-27.2134313544353,13.6512271972451,
130.078177727749)) ;
#126124=CARTESIAN_POINT('Ctrl Pts',(-27.1907621951,13.9458587168303,129.978824391193)) ;
#126125=CARTESIAN_POINT('Ctrl Pts',(-27.1438228231877,14.2033946727232,
129.808513890498)) ;
#126126=CARTESIAN_POINT('Ctrl Pts',(-27.0770750626635,14.4040391264647,
129.580474233963)) ;
#126127=CARTESIAN_POINT('Ctrl Pts',(-26.9958801704917,14.5350227428464,
129.310223124161)) ;
#126128=CARTESIAN_POINT('Ctrl Pts',(-26.906059475308,14.5864958766325,129.014538770092)) ;
#126129=CARTESIAN_POINT('Ctrl Pts',(-26.8162216028424,14.5544169233344,
128.719109024983)) ;
#126130=CARTESIAN_POINT('Ctrl Pts',(-26.732249151307,14.4414134366696,128.440641667586)) ;
#126131=CARTESIAN_POINT('Ctrl Pts',(-26.6614367576336,14.2551029691134,
128.200625386532)) ;
#126132=CARTESIAN_POINT('Ctrl Pts',(-26.6096148301924,14.0100365412081,
128.016185333679)) ;
#126133=CARTESIAN_POINT('Ctrl Pts',(-26.5809743060425,13.7214335751914,
127.899285485358)) ;
#126134=CARTESIAN_POINT('Ctrl Pts',(-26.5785086522485,13.4135493095884,
127.859089390774)) ;
#126135=CARTESIAN_POINT('Ctrl Pts',(-26.6030598393761,13.1045553543373,
127.897610196084)) ;
#126136=CARTESIAN_POINT('Ctrl Pts',(-26.6533738007603,12.819735905808,128.011560491911)) ;
#126137=CARTESIAN_POINT('Ctrl Pts',(-26.7273433263528,12.5762135123813,
128.194341414483)) ;
#126138=CARTESIAN_POINT('Ctrl Pts',(-26.8192648566206,12.3952019865551,
128.429832693203)) ;
#126139=CARTESIAN_POINT('Ctrl Pts',(-26.9242264204427,12.2871509096393,
128.703270123928)) ;
#126140=CARTESIAN_POINT('Ctrl Pts',(-27.0344529109704,12.2605661260812,
128.992282379476)) ;
#126141=CARTESIAN_POINT('Ctrl Pts',(-27.1443703931417,12.3174696156297,
129.280083515023)) ;
#126142=CARTESIAN_POINT('Ctrl Pts',(-27.2451512743396,12.4535095799729,
129.541404839542)) ;
#126143=CARTESIAN_POINT('Ctrl Pts',(-27.331104012236,12.6588731415835,129.759381061345)) ;
#126144=CARTESIAN_POINT('Ctrl Pts',(-27.3966132229069,12.9185733098552,
129.917687249482)) ;
#126145=CARTESIAN_POINT('Ctrl Pts',(-27.437913249649,13.2144047799764,130.005254654864)) ;
#126146=CARTESIAN_POINT('Ctrl Pts',(-27.4527179999152,13.5255442513147,
130.015381846826)) ;
#126147=CARTESIAN_POINT('Ctrl Pts',(-27.4406132753305,13.8297540824603,
129.946859327367)) ;
#126148=CARTESIAN_POINT('Ctrl Pts',(-27.4030398195296,14.1049218673864,
129.803899854786)) ;
#126149=CARTESIAN_POINT('Ctrl Pts',(-27.3439832338372,14.3298724417038,
129.59839933543)) ;
#126150=CARTESIAN_POINT('Ctrl Pts',(-27.2674519754825,14.4915528402348,
129.34156807038)) ;
#126151=CARTESIAN_POINT('Ctrl Pts',(-27.1804570845726,14.5755974614276,
129.054311222488)) ;
#126152=CARTESIAN_POINT('Ctrl Pts',(-27.0900591437139,14.5774288175943,
128.75723029633)) ;
#126153=CARTESIAN_POINT('Ctrl Pts',(-27.0027465267917,14.4968431022692,
128.469040137176)) ;
#126154=CARTESIAN_POINT('Ctrl Pts',(-26.9256630669634,14.3385595023236,
128.210629189847)) ;
#126155=CARTESIAN_POINT('Ctrl Pts',(-26.8655442910329,14.1152209980979,
128.00189933541)) ;
#126156=CARTESIAN_POINT('Ctrl Pts',(-26.8270860169213,13.8419813754815,
127.856398889617)) ;
#126157=CARTESIAN_POINT('Ctrl Pts',(-26.8138530884316,13.5398084238246,
127.784708325254)) ;
#126158=CARTESIAN_POINT('Ctrl Pts',(-26.8274109995624,13.2280435028726,
127.791143495503)) ;
#126159=CARTESIAN_POINT('Ctrl Pts',(-26.8677662548996,12.9300590292135,
127.875833464593)) ;
#126160=CARTESIAN_POINT('Ctrl Pts',(-26.9324327506608,12.6684083848218,
128.031655490712)) ;
#126161=CARTESIAN_POINT('Ctrl Pts',(-27.0174847633721,12.4608091208846,
128.247059958605)) ;
#126162=CARTESIAN_POINT('Ctrl Pts',(-27.1179785264983,12.3214093347923,
128.507474270325)) ;
#126163=CARTESIAN_POINT('Ctrl Pts',(-27.2275226737143,12.2613302981185,
128.794237732112)) ;
#126164=CARTESIAN_POINT('Ctrl Pts',(-27.3376047432448,12.2843255086961,
129.082895790181)) ;
#126165=CARTESIAN_POINT('Ctrl Pts',(-27.4428996493216,12.3887269891781,
129.357335238183)) ;
#126166=CARTESIAN_POINT('Ctrl Pts',(-27.5357472832916,12.567362762576,129.595436520551)) ;
#126167=CARTESIAN_POINT('Ctrl Pts',(-27.6104078073465,12.8080166965812,
129.780323450839)) ;
#126168=CARTESIAN_POINT('Ctrl Pts',(-27.6618734446833,13.0914774469774,
129.897617122415)) ;
#126169=CARTESIAN_POINT('Ctrl Pts',(-27.6875950196144,13.4005589719555,
129.939492462511)) ;
#126170=CARTESIAN_POINT('Ctrl Pts',(-27.6862592435431,13.7083911607305,
129.902647623818)) ;
#126171=CARTESIAN_POINT('Ctrl Pts',(-27.6586873787824,13.9985991355892,
129.788842673993)) ;
#126172=CARTESIAN_POINT('Ctrl Pts',(-27.6077515908902,14.2457812535683,
129.606991326531)) ;
#126173=CARTESIAN_POINT('Ctrl Pts',(-27.5377989327998,14.434573414283,129.369557237588)) ;
#126174=CARTESIAN_POINT('Ctrl Pts',(-27.4542768495757,14.5511370884747,
129.092404947508)) ;
#126175=CARTESIAN_POINT('Ctrl Pts',(-27.3644225518952,14.5867802191552,
128.796873978276)) ;
#126176=CARTESIAN_POINT('Ctrl Pts',(-27.2747420069069,14.5391948457713,
128.501723104712)) ;
#126177=CARTESIAN_POINT('Ctrl Pts',(-27.1928633072709,14.4115345320068,
128.229410196093)) ;
#126178=CARTESIAN_POINT('Ctrl Pts',(-27.125297150064,14.2134355726879,127.998946383917)) ;
#126179=CARTESIAN_POINT('Ctrl Pts',(-27.0774187575892,13.958237750451,127.825922594833)) ;
#126180=CARTESIAN_POINT('Ctrl Pts',(-27.0535942488343,13.6646542433851,
127.723173741456)) ;
#126181=CARTESIAN_POINT('Ctrl Pts',(-27.0562015090421,13.3541836423797,
127.697682670805)) ;
#126182=CARTESIAN_POINT('Ctrl Pts',(-27.0857370264101,13.0484268899304,
127.750836023562)) ;
#126183=CARTESIAN_POINT('Ctrl Pts',(-27.1409450439948,12.769439556936,127.87895999406)) ;
#126184=CARTESIAN_POINT('Ctrl Pts',(-27.2180733512631,12.538041732005,128.071268052011)) ;
#126185=CARTESIAN_POINT('Ctrl Pts',(-27.3137559998053,12.3683285737822,
128.317416850313)) ;
#126186=CARTESIAN_POINT('Ctrl Pts',(-27.4196365681885,12.2760420146323,
128.593780876063)) ;
#126187=CARTESIAN_POINT('Ctrl Pts',(-27.5306231079652,12.2649172046645,
128.884867753868)) ;
#126188=CARTESIAN_POINT('Ctrl Pts',(-27.6389017948996,12.3368690960139,
129.1680658529)) ;
#126189=CARTESIAN_POINT('Ctrl Pts',(-27.7377556093054,12.4871143046054,
129.423632129144)) ;
#126190=CARTESIAN_POINT('Ctrl Pts',(-27.8202491494068,12.7041606562746,
129.631498782579)) ;
#126191=CARTESIAN_POINT('Ctrl Pts',(-27.8814612994333,12.9721743226057,
129.777246365525)) ;
#126192=CARTESIAN_POINT('Ctrl Pts',(-27.9178954972168,13.2726903984431,
129.850577604052)) ;
#126193=CARTESIAN_POINT('Ctrl Pts',(-27.9276073498743,13.5844635777056,
129.845797878301)) ;
#126194=CARTESIAN_POINT('Ctrl Pts',(-27.9104034593952,13.8852371899129,
129.762316738143)) ;
#126195=CARTESIAN_POINT('Ctrl Pts',(-27.8686813644329,14.1508961258859,
129.607456776857)) ;
#126196=CARTESIAN_POINT('Ctrl Pts',(-27.805777890454,14.3659570919706,129.390557072871)) ;
#126197=CARTESIAN_POINT('Ctrl Pts',(-27.7267920219095,14.5133844766524,
129.126610121449)) ;
#126198=CARTESIAN_POINT('Ctrl Pts',(-27.6388634022396,14.5822824975676,
128.836735478804)) ;
#126199=CARTESIAN_POINT('Ctrl Pts',(-27.5480345518923,14.5684017551043,
128.538201746879)) ;
#126200=CARTESIAN_POINT('Ctrl Pts',(-27.4623293694807,14.4726240030268,
128.254765455669)) ;
#126201=CARTESIAN_POINT('Ctrl Pts',(-27.3879707689627,14.3009017831871,
128.004315479595)) ;
#126202=CARTESIAN_POINT('Ctrl Pts',(-27.3317507009227,14.0676661547484,
127.807078623479)) ;
#126203=CARTESIAN_POINT('Ctrl Pts',(-27.2976904983125,13.7867922981234,
127.67436647184)) ;
#126204=CARTESIAN_POINT('Ctrl Pts',(-27.2894631150385,13.4808115386222,
127.61724202784)) ;
#126205=CARTESIAN_POINT('Ctrl Pts',(-27.3080625977825,13.1706177086878,
127.638476490103)) ;
#126206=CARTESIAN_POINT('Ctrl Pts',(-27.3533779369102,12.877048394192,127.737575696294)) ;
#126207=CARTESIAN_POINT('Ctrl Pts',(-27.4219972748813,12.6251910446387,
127.905071056163)) ;
#126208=CARTESIAN_POINT('Ctrl Pts',(-27.5104518024654,12.4289584730978,
128.130355526478)) ;
#126209=CARTESIAN_POINT('Ctrl Pts',(-27.6133286223986,12.3038002385442,
128.397669935348)) ;
#126210=CARTESIAN_POINT('Ctrl Pts',(-27.7232164389536,12.2593442702032,
128.68559205266)) ;
#126211=CARTESIAN_POINT('Ctrl Pts',(-27.8332334336571,12.2978898762746,
128.973926847691)) ;
#126212=CARTESIAN_POINT('Ctrl Pts',(-27.9366469237781,12.4169444265874,
129.242893983991)) ;
#126213=CARTESIAN_POINT('Ctrl Pts',(-28.0268222922301,12.6093773192219,
129.473030956235)) ;
#126214=CARTESIAN_POINT('Ctrl Pts',(-28.0969743287122,12.8583734151229,
129.644955599161)) ;
#126215=CARTESIAN_POINT('Ctrl Pts',(-28.1438275325612,13.1480449796925,
129.748746916576)) ;
#126216=CARTESIAN_POINT('Ctrl Pts',(-28.1644954117435,13.4582418088587,
129.775959672609)) ;
#126217=CARTESIAN_POINT('Ctrl Pts',(-28.1581306779681,13.7655079341762,
129.724247830302)) ;
#126218=CARTESIAN_POINT('Ctrl Pts',(-28.1259517579114,14.048316994012,129.59711509984)) ;
#126219=CARTESIAN_POINT('Ctrl Pts',(-28.0711052803105,14.2859990299988,
129.403818984126)) ;
#126220=CARTESIAN_POINT('Ctrl Pts',(-27.9979984934453,14.4624790722787,
129.157095753605)) ;
#126221=CARTESIAN_POINT('Ctrl Pts',(-27.9126529086255,14.5642184031824,
128.874605844398)) ;
#126222=CARTESIAN_POINT('Ctrl Pts',(-27.82234244871,14.584160945988,128.577742029782)) ;
#126223=CARTESIAN_POINT('Ctrl Pts',(-27.7335731289501,14.5209707107522,
128.285251255355)) ;
#126224=CARTESIAN_POINT('Ctrl Pts',(-27.6539417613536,14.3791778899535,
128.019520055056)) ;
#126225=CARTESIAN_POINT('Ctrl Pts',(-27.5896417043547,14.1688150689694,
127.798546337055)) ;
#126226=CARTESIAN_POINT('Ctrl Pts',(-27.5461247472488,13.9051956236196,
127.638312484282)) ;
#126227=CARTESIAN_POINT('Ctrl Pts',(-27.5271452909361,13.6071499712881,
127.54976394242)) ;
#126228=CARTESIAN_POINT('Ctrl Pts',(-27.5348305475125,13.2953842790605,
127.539053516484)) ;
#126229=CARTESIAN_POINT('Ctrl Pts',(-27.5694192910359,12.9930168542047,
127.606957456664)) ;
#126230=CARTESIAN_POINT('Ctrl Pts',(-27.6288755570811,12.722227284065,127.747605806903)) ;
#126231=CARTESIAN_POINT('Ctrl Pts',(-27.7100939855666,12.5005440271994,
127.951701688244)) ;
#126232=CARTESIAN_POINT('Ctrl Pts',(-27.8080372736976,12.3451352919228,
128.204600625969)) ;
#126233=CARTESIAN_POINT('Ctrl Pts',(-27.9154950057297,12.2674914162103,
128.485503862418)) ;
#126234=CARTESIAN_POINT('Ctrl Pts',(-28.0268939179855,12.2722652816386,
128.777693027108)) ;
#126235=CARTESIAN_POINT('Ctrl Pts',(-28.1338981955741,12.3599738875374,
129.057142459325)) ;
#126236=CARTESIAN_POINT('Ctrl Pts',(-28.2294682857705,12.522637910065,129.303361399343)) ;
#126237=CARTESIAN_POINT('Ctrl Pts',(-28.3085931444286,12.7508223350777,
129.501319058887)) ;
#126238=CARTESIAN_POINT('Ctrl Pts',(-28.3656063081004,13.0279566235447,
129.634633388162)) ;
#126239=CARTESIAN_POINT('Ctrl Pts',(-28.3969444639279,13.3323088318152,
129.693075814844)) ;
#126240=CARTESIAN_POINT('Ctrl Pts',(-28.4014787981811,13.6420774787073,
129.673330395157)) ;
#126241=CARTESIAN_POINT('Ctrl Pts',(-28.3795963264581,13.9374078863426,
129.576285309709)) ;
#126242=CARTESIAN_POINT('Ctrl Pts',(-28.3333509219362,14.1965319765984,
129.407993850494)) ;
#126243=CARTESIAN_POINT('Ctrl Pts',(-28.266675124667,14.3999725992787,129.179974394099)) ;
#126244=CARTESIAN_POINT('Ctrl Pts',(-28.1862016672231,14.5320840225921,
128.912009605806)) ;
#126245=CARTESIAN_POINT('Ctrl Pts',(-28.0966741913854,14.5862914481746,
128.617232858697)) ;
#126246=CARTESIAN_POINT('Ctrl Pts',(-28.0062577051871,14.5562373139742,
128.319925352826)) ;
#126247=CARTESIAN_POINT('Ctrl Pts',(-27.9225302663962,14.446076002877,128.042377588389)) ;
#126248=CARTESIAN_POINT('Ctrl Pts',(-27.8509244482422,14.2613118658137,
127.799922177814)) ;
#126249=CARTESIAN_POINT('Ctrl Pts',(-27.798497284698,14.0168342944467,127.613633246462)) ;
#126250=CARTESIAN_POINT('Ctrl Pts',(-27.7692851272863,13.7314084945653,
127.495315906887)) ;
#126251=CARTESIAN_POINT('Ctrl Pts',(-27.7660083743788,13.4213927806631,
127.45248187371)) ;
#126252=CARTESIAN_POINT('Ctrl Pts',(-27.7897193573963,13.1138964829047,
127.488747985494)) ;
#126253=CARTESIAN_POINT('Ctrl Pts',(-27.8393546178715,12.8273574952535,
127.600633072825)) ;
#126254=CARTESIAN_POINT('Ctrl Pts',(-27.9127949354444,12.5821904217373,
127.781847712348)) ;
#126255=CARTESIAN_POINT('Ctrl Pts',(-28.0043735492926,12.3992406566731,
128.016306398527)) ;
#126256=CARTESIAN_POINT('Ctrl Pts',(-28.1087022331987,12.2892635320147,
128.288009999253)) ;
#126257=CARTESIAN_POINT('Ctrl Pts',(-28.2190913648179,12.2601882735182,
128.57742408835)) ;
#126258=CARTESIAN_POINT('Ctrl Pts',(-28.3287542082612,12.3144490437337,
128.864604111698)) ;
#126259=CARTESIAN_POINT('Ctrl Pts',(-28.4299954593875,12.4481500552587,
129.127241049758)) ;
#126260=CARTESIAN_POINT('Ctrl Pts',(-28.5165306603846,12.6515765738091,
129.346913037363)) ;
#126261=CARTESIAN_POINT('Ctrl Pts',(-28.5830300089725,12.911209097722,129.507949494699)) ;
#126262=CARTESIAN_POINT('Ctrl Pts',(-28.6249728675832,13.2069681338802,
129.597336632742)) ;
#126263=CARTESIAN_POINT('Ctrl Pts',(-28.6404608703377,13.5165271467016,
129.609618370989)) ;
#126264=CARTESIAN_POINT('Ctrl Pts',(-28.6290148464267,13.8224961920609,
129.542876508472)) ;
#126265=CARTESIAN_POINT('Ctrl Pts',(-28.5922601971028,14.0973150821475,
129.402480129101)) ;
#126266=CARTESIAN_POINT('Ctrl Pts',(-28.5336757378928,14.3244518569206,
129.198286920491)) ;
#126267=CARTESIAN_POINT('Ctrl Pts',(-28.4576637523532,14.4877799967397,
128.943033798244)) ;
#126268=CARTESIAN_POINT('Ctrl Pts',(-28.3710048581047,14.5742905029568,
128.656795471305)) ;
#126269=CARTESIAN_POINT('Ctrl Pts',(-28.2802241255344,14.5785355282753,
128.35845638066)) ;
#126270=CARTESIAN_POINT('Ctrl Pts',(-28.1928419853,14.4999982805016,128.070098188264)) ;
#126271=CARTESIAN_POINT('Ctrl Pts',(-28.1156963429542,14.344757358462,127.811665392834)) ;
#126272=CARTESIAN_POINT('Ctrl Pts',(-28.0547636884467,14.1223923332962,
127.600432721674)) ;
#126273=CARTESIAN_POINT('Ctrl Pts',(-28.0157051647959,13.8510685521418,
127.45327003594)) ;
#126274=CARTESIAN_POINT('Ctrl Pts',(-28.0016271877878,13.5484335086258,
127.378992507059)) ;
#126275=CARTESIAN_POINT('Ctrl Pts',(-28.014450669107,13.2370240609784,127.383328520091)) ;
#126276=CARTESIAN_POINT('Ctrl Pts',(-28.0538788566097,12.9391310692164,
127.465404042021)) ;
#126277=CARTESIAN_POINT('Ctrl Pts',(-28.1178898237982,12.6756659712694,
127.619266774088)) ;
#126278=CARTESIAN_POINT('Ctrl Pts',(-28.2026458744836,12.4657027471288,
127.833719653981)) ;
#126279=CARTESIAN_POINT('Ctrl Pts',(-28.3027339455981,12.3244745287068,
128.092974050606)) ;
#126280=CARTESIAN_POINT('Ctrl Pts',(-28.4116254389229,12.2619232724697,
128.377977700105)) ;
#126281=CARTESIAN_POINT('Ctrl Pts',(-28.5225430499368,12.2825882461712,
128.668841361449)) ;
#126282=CARTESIAN_POINT('Ctrl Pts',(-28.6277358208058,12.3846501373822,
128.943090603315)) ;
#126283=CARTESIAN_POINT('Ctrl Pts',(-28.7210231729538,12.5611187376007,
129.182483263865)) ;
#126284=CARTESIAN_POINT('Ctrl Pts',(-28.7963015152677,12.8001289118654,
129.369183041344)) ;
#126285=CARTESIAN_POINT('Ctrl Pts',(-28.848510718025,13.0829558583446,129.488606078419)) ;
#126286=CARTESIAN_POINT('Ctrl Pts',(-28.8749835754297,13.3903655570018,
129.532815151912)) ;
#126287=CARTESIAN_POINT('Ctrl Pts',(-28.8744412770404,13.7001366244489,
129.498104859533)) ;
#126288=CARTESIAN_POINT('Ctrl Pts',(-28.8477145078455,13.9898881879969,
129.386927516853)) ;
#126289=CARTESIAN_POINT('Ctrl Pts',(-28.7973599708568,14.2391934604651,
129.206697827823)) ;
#126290=CARTESIAN_POINT('Ctrl Pts',(-28.7279827552736,14.4298567276207,
128.970982641298)) ;
#126291=CARTESIAN_POINT('Ctrl Pts',(-28.644258384591,14.5492471456149,128.693044021335)) ;
#126292=CARTESIAN_POINT('Ctrl Pts',(-28.554796284374,14.5868020959289,128.39877651472)) ;
#126293=CARTESIAN_POINT('Ctrl Pts',(-28.4650804844611,14.5417975153692,
128.103553265323)) ;
#126294=CARTESIAN_POINT('Ctrl Pts',(-28.3828462169605,14.4162088209851,
127.830180515014)) ;
#126295=CARTESIAN_POINT('Ctrl Pts',(-28.3148259514202,14.2204083214859,
127.598438875209)) ;
#126296=CARTESIAN_POINT('Ctrl Pts',(-28.2660768691486,13.9647701024183,
127.422650641298)) ;
#126297=CARTESIAN_POINT('Ctrl Pts',(-28.2417393818523,13.6739288437871,
127.318633866623)) ;
#126298=CARTESIAN_POINT('Ctrl Pts',(-28.2435589798425,13.362328471029,127.290695136997)) ;
#126299=CARTESIAN_POINT('Ctrl Pts',(-28.272280384429,13.0574724209015,127.341613025253)) ;
#126300=CARTESIAN_POINT('Ctrl Pts',(-28.3266764891578,12.7770676806865,
127.467351744318)) ;
#126301=CARTESIAN_POINT('Ctrl Pts',(-28.4039036629146,12.5427864739332,
127.659709669059)) ;
#126302=CARTESIAN_POINT('Ctrl Pts',(-28.4979676565153,12.3731888111629,
127.901550196768)) ;
#126303=CARTESIAN_POINT('Ctrl Pts',(-28.6042086691124,12.2773794230824,
128.178756519312)) ;
#126304=CARTESIAN_POINT('Ctrl Pts',(-28.715472627962,12.2641879723106,128.47056855639)) ;
#126305=CARTESIAN_POINT('Ctrl Pts',(-28.8235400299554,12.3335960858358,
128.753264954274)) ;
#126306=CARTESIAN_POINT('Ctrl Pts',(-28.9227867930702,12.4815617101667,
129.009979499555)) ;
#126307=CARTESIAN_POINT('Ctrl Pts',(-29.0058719352323,12.6968288003286,
129.219569350323)) ;
#126308=CARTESIAN_POINT('Ctrl Pts',(-29.0678679462344,12.9642191171328,
129.367533009777)) ;
#126309=CARTESIAN_POINT('Ctrl Pts',(-29.1050280217852,13.2637556030546,
129.443027420191)) ;
#126310=CARTESIAN_POINT('Ctrl Pts',(-29.1154418002506,13.5766924952844,
129.440167113031)) ;
#126311=CARTESIAN_POINT('Ctrl Pts',(-29.0991939031422,13.8753723119149,
129.359790683957)) ;
#126312=CARTESIAN_POINT('Ctrl Pts',(-29.0578831159195,14.1446746282912,
129.205850385365)) ;
#126313=CARTESIAN_POINT('Ctrl Pts',(-28.9955328716822,14.3606486732163,
128.990637905782)) ;
#126314=CARTESIAN_POINT('Ctrl Pts',(-28.9172212199739,14.510078619128,128.72876476362)) ;
#126315=CARTESIAN_POINT('Ctrl Pts',(-28.8287816094018,14.5815775918547,
128.437141604284)) ;
#126316=CARTESIAN_POINT('Ctrl Pts',(-28.7385909291533,14.5700419701179,
128.140725723263)) ;
#126317=CARTESIAN_POINT('Ctrl Pts',(-28.6522425556229,14.4761037327312,
127.855240333411)) ;
#126318=CARTESIAN_POINT('Ctrl Pts',(-28.5778444620489,14.3074346005472,
127.604870863317)) ;
#126319=CARTESIAN_POINT('Ctrl Pts',(-28.5205972031991,14.073572566118,127.404328059254)) ;
#126320=CARTESIAN_POINT('Ctrl Pts',(-28.4862429573869,13.7966474057212,
127.271116789574)) ;
#126321=CARTESIAN_POINT('Ctrl Pts',(-28.4770859270264,13.4894704941488,
127.211081165859)) ;
#126322=CARTESIAN_POINT('Ctrl Pts',(-28.4948943292332,13.1800818047294,
127.230117007035)) ;
#126323=CARTESIAN_POINT('Ctrl Pts',(-28.5394276796164,12.8853355952022,
127.326898324992)) ;
#126324=CARTESIAN_POINT('Ctrl Pts',(-28.6074761504503,12.6318025855322,
127.492695185973)) ;
#126325=CARTESIAN_POINT('Ctrl Pts',(-28.695470726565,12.4337108442548,127.716625488695)) ;
#126326=CARTESIAN_POINT('Ctrl Pts',(-28.7978123159624,12.3064394695167,
127.982443096435)) ;
#126327=CARTESIAN_POINT('Ctrl Pts',(-28.9079039717027,12.259467253753,128.270860085229)) ;
#126328=CARTESIAN_POINT('Ctrl Pts',(-29.0179009527206,12.2954707770716,
128.559180514689)) ;
#126329=CARTESIAN_POINT('Ctrl Pts',(-29.1222060572925,12.4135506736779,
128.830531653871)) ;
#126330=CARTESIAN_POINT('Ctrl Pts',(-29.2116568789094,12.6014761688176,
129.059003773852)) ;
#126331=CARTESIAN_POINT('Ctrl Pts',(-29.2831239492051,12.8505488617132,
129.234511371657)) ;
#126332=CARTESIAN_POINT('Ctrl Pts',(-29.3306092364222,13.1393106642719,
129.340171358804)) ;
#126333=CARTESIAN_POINT('Ctrl Pts',(-29.3520748841438,13.4495612707078,
129.369675966618)) ;
#126334=CARTESIAN_POINT('Ctrl Pts',(-29.3464729517262,13.7566531065693,
129.320254581372)) ;
#126335=CARTESIAN_POINT('Ctrl Pts',(-29.3150443593479,14.0404143617275,
129.195320768512)) ;
#126336=CARTESIAN_POINT('Ctrl Pts',(-29.2608243465156,14.2798568103851,
129.003847830969)) ;
#126337=CARTESIAN_POINT('Ctrl Pts',(-29.1878014525805,14.4588607973601,
128.757223804424)) ;
#126338=CARTESIAN_POINT('Ctrl Pts',(-29.1031844107461,14.5622468207321,
128.477052820405)) ;
#126339=CARTESIAN_POINT('Ctrl Pts',(-29.0125825178535,14.5847589284177,
128.179204966729)) ;
#126340=CARTESIAN_POINT('Ctrl Pts',(-28.9239262939069,14.5239999294188,
127.887147086676)) ;
#126341=CARTESIAN_POINT('Ctrl Pts',(-28.8438246268334,14.3842925756614,
127.619996920254)) ;
#126342=CARTESIAN_POINT('Ctrl Pts',(-28.7790368369442,14.1758058754008,
127.397617265261)) ;
#126343=CARTESIAN_POINT('Ctrl Pts',(-28.7347735365329,13.9130883833925,
127.235151253729)) ;
#126344=CARTESIAN_POINT('Ctrl Pts',(-28.7151135618664,13.6151579335754,
127.144558769301)) ;
#126345=CARTESIAN_POINT('Ctrl Pts',(-28.7219995435927,13.3050553518441,
127.131682646232)) ;
#126346=CARTESIAN_POINT('Ctrl Pts',(-28.7557377597948,13.0018870987347,
127.197084482543)) ;
#126347=CARTESIAN_POINT('Ctrl Pts',(-28.814675083667,12.7291797299788,127.336129164948)) ;
#126348=CARTESIAN_POINT('Ctrl Pts',(-28.8952944144317,12.5061726224373,
127.538507349107)) ;
#126349=CARTESIAN_POINT('Ctrl Pts',(-28.992452875052,12.3489725905771,127.789232229175)) ;
#126350=CARTESIAN_POINT('Ctrl Pts',(-29.1001181450375,12.2685649990364,
128.070611823995)) ;
#126351=CARTESIAN_POINT('Ctrl Pts',(-29.2111067626934,12.2709027590492,
128.361728243776)) ;
#126352=CARTESIAN_POINT('Ctrl Pts',(-29.3183871335447,12.3558100715775,
128.641979311852)) ;
#126353=CARTESIAN_POINT('Ctrl Pts',(-29.4148436719289,12.5172182560686,
128.890625247685)) ;
#126354=CARTESIAN_POINT('Ctrl Pts',(-29.4942688116787,12.743270611073,129.089550396418)) ;
#126355=CARTESIAN_POINT('Ctrl Pts',(-29.551869204403,13.0180148278647,129.224707278106)) ;
#126356=CARTESIAN_POINT('Ctrl Pts',(-29.5842039318189,13.3228200342207,
129.285946655861)) ;
#126357=CARTESIAN_POINT('Ctrl Pts',(-29.5895128485569,13.6334362897112,
129.268389620136)) ;
#126358=CARTESIAN_POINT('Ctrl Pts',(-29.5683363278282,13.929416387864,129.173412954777)) ;
#126359=CARTESIAN_POINT('Ctrl Pts',(-29.5228950497417,14.1891570751448,
129.007566404027)) ;
#126360=CARTESIAN_POINT('Ctrl Pts',(-29.4568217632275,14.3946402332245,
128.78131441326)) ;
#126361=CARTESIAN_POINT('Ctrl Pts',(-29.3763677570869,14.5295569095383,
128.513275619402)) ;
#126362=CARTESIAN_POINT('Ctrl Pts',(-29.2868834281595,14.5858061320267,
128.218594172143)) ;
#126363=CARTESIAN_POINT('Ctrl Pts',(-29.1968889427481,14.5585141684262,
127.922706052922)) ;
#126364=CARTESIAN_POINT('Ctrl Pts',(-29.1124170400181,14.4500372102403,
127.642795696124)) ;
#126365=CARTESIAN_POINT('Ctrl Pts',(-29.0407778038687,14.268202012558,127.400434608182)) ;
#126366=CARTESIAN_POINT('Ctrl Pts',(-28.9875018774522,14.0250734119471,
127.211599238186)) ;
#126367=CARTESIAN_POINT('Ctrl Pts',(-28.9575029477622,13.7389393518604,
127.090807741331)) ;
#126368=CARTESIAN_POINT('Ctrl Pts',(-28.9535386701218,13.4311037036194,
127.046163668047)) ;
#126369=CARTESIAN_POINT('Ctrl Pts',(-28.9763267200494,13.1229020321195,
127.079702982171)) ;
#126370=CARTESIAN_POINT('Ctrl Pts',(-29.0257949317233,12.8333723855065,
127.190836011178)) ;
#126371=CARTESIAN_POINT('Ctrl Pts',(-29.0978600733987,12.5895126789185,
127.368402800474)) ;
#126372=CARTESIAN_POINT('Ctrl Pts',(-29.1892280354939,12.4035404975601,
127.602115483622)) ;
#126373=CARTESIAN_POINT('Ctrl Pts',(-29.2932741260525,12.2914040477839,
127.873003194407)) ;
#126374=CARTESIAN_POINT('Ctrl Pts',(-29.4037033629628,12.259812265838,128.162497247571)) ;
#126375=CARTESIAN_POINT('Ctrl Pts',(-29.5135609204899,12.3118570241587,
128.450226071125)) ;
#126376=CARTESIAN_POINT('Ctrl Pts',(-29.6149254569401,12.4430958843788,
128.713290866227)) ;
#126377=CARTESIAN_POINT('Ctrl Pts',(-29.7020530820368,12.6447072746916,
128.934674038552)) ;
#126378=CARTESIAN_POINT('Ctrl Pts',(-29.7691752470244,12.9030427397014,
129.097526306521)) ;
#126379=CARTESIAN_POINT('Ctrl Pts',(-29.8118434047462,13.1970329557463,
129.189137020104)) ;
#126380=CARTESIAN_POINT('Ctrl Pts',(-29.8281637012964,13.5084313502234,
129.203633314877)) ;
#126381=CARTESIAN_POINT('Ctrl Pts',(-29.8176270439828,13.8121188302543,
129.139861139091)) ;
#126382=CARTESIAN_POINT('Ctrl Pts',(-29.7814625744293,14.0900962513971,
129.000962562861)) ;
#126383=CARTESIAN_POINT('Ctrl Pts',(-29.7234265946476,14.31872996458,128.798387529551)) ;
#126384=CARTESIAN_POINT('Ctrl Pts',(-29.6476098832969,14.484422730659,128.543613950177)) ;
#126385=CARTESIAN_POINT('Ctrl Pts',(-29.5615142448024,14.5727758927101,
128.259159521948)) ;
#126386=CARTESIAN_POINT('Ctrl Pts',(-29.4707443641585,14.5796460422286,
127.960845873962)) ;
#126387=CARTESIAN_POINT('Ctrl Pts',(-29.3831258062148,14.5035865487986,
127.671790345692)) ;
#126388=CARTESIAN_POINT('Ctrl Pts',(-29.3052805384703,14.3497062950072,
127.411173840987)) ;
#126389=CARTESIAN_POINT('Ctrl Pts',(-29.2439657968061,14.1291329679128,
127.198875466525)) ;
#126390=CARTESIAN_POINT('Ctrl Pts',(-29.2043177636014,13.8597726326946,
127.05008067997)) ;
#126391=CARTESIAN_POINT('Ctrl Pts',(-29.1894481468779,13.557462341525,126.973458033413)) ;
#126392=CARTESIAN_POINT('Ctrl Pts',(-29.2014467723286,13.2463365194833,
126.975423633126)) ;
#126393=CARTESIAN_POINT('Ctrl Pts',(-29.240192496977,12.9472973154242,127.055450427306)) ;
#126394=CARTESIAN_POINT('Ctrl Pts',(-29.3033094304608,12.6832077780023,
127.2068001365)) ;
#126395=CARTESIAN_POINT('Ctrl Pts',(-29.3879194372612,12.4704982394892,
127.420671040737)) ;
#126396=CARTESIAN_POINT('Ctrl Pts',(-29.4873059937918,12.3276823235439,
127.677998441968)) ;
#126397=CARTESIAN_POINT('Ctrl Pts',(-29.5962501169316,12.2625925201889,
127.963084302124)) ;
#126398=CARTESIAN_POINT('Ctrl Pts',(-29.7068390569069,12.280619224966,128.25310533232)) ;
#126399=CARTESIAN_POINT('Ctrl Pts',(-29.8129831084837,12.3809214756921,
128.529919358557)) ;
#126400=CARTESIAN_POINT('Ctrl Pts',(-29.906657709987,12.556040128184,128.770421483879)) ;
#126401=CARTESIAN_POINT('Ctrl Pts',(-29.9820403676067,12.7918901581632,
128.957644910704)) ;
#126402=CARTESIAN_POINT('Ctrl Pts',(-30.0351697168892,13.0744209862709,
129.079658466158)) ;
#126403=CARTESIAN_POINT('Ctrl Pts',(-30.0623799674238,13.3812416833702,
129.126046104789)) ;
#126404=CARTESIAN_POINT('Ctrl Pts',(-30.0626128615332,13.6920797161949,
129.093513213577)) ;
#126405=CARTESIAN_POINT('Ctrl Pts',(-30.0365037669751,13.9824941766623,
128.984145022211)) ;
#126406=CARTESIAN_POINT('Ctrl Pts',(-29.987039803891,14.2323227471641,128.806660210106)) ;
#126407=CARTESIAN_POINT('Ctrl Pts',(-29.9176946082372,14.4258243482768,
128.570836399515)) ;
#126408=CARTESIAN_POINT('Ctrl Pts',(-29.8350161561935,14.5465247223938,
128.29625314965)) ;
#126409=CARTESIAN_POINT('Ctrl Pts',(-29.7448155074623,14.5869806833893,
127.999509947687)) ;
#126410=CARTESIAN_POINT('Ctrl Pts',(-29.6554990618739,14.5442058476213,
127.705640700795)) ;
#126411=CARTESIAN_POINT('Ctrl Pts',(-29.5727669786191,14.4209679586328,
127.430757402841)) ;
#126412=CARTESIAN_POINT('Ctrl Pts',(-29.5040785211676,14.2257906516459,
127.196921938398)) ;
#126413=CARTESIAN_POINT('Ctrl Pts',(-29.4551663445329,13.9741287595616,
127.020990849854)) ;
#126414=CARTESIAN_POINT('Ctrl Pts',(-29.4298421339555,13.6829512293512,
126.91393472797)) ;
#126415=CARTESIAN_POINT('Ctrl Pts',(-29.4309001415048,13.37146650651,126.88376820502)) ;
#126416=CARTESIAN_POINT('Ctrl Pts',(-29.4589213897168,13.0656058260286,
126.932576869768)) ;
#126417=CARTESIAN_POINT('Ctrl Pts',(-29.5125089739452,12.7850334229127,
127.056046900933)) ;
#126418=CARTESIAN_POINT('Ctrl Pts',(-29.5887530272508,12.5496672671412,
127.24565170869)) ;
#126419=CARTESIAN_POINT('Ctrl Pts',(-29.6830427688529,12.3766688304073,
127.487911118153)) ;
#126420=CARTESIAN_POINT('Ctrl Pts',(-29.7890527274797,12.2789529109886,
127.76445425575)) ;
#126421=CARTESIAN_POINT('Ctrl Pts',(-29.9000873163388,12.2634413575716,
128.055650583301)) ;
#126422=CARTESIAN_POINT('Ctrl Pts',(-30.0083485486883,12.3304157181155,
128.338911431539)) ;
#126423=CARTESIAN_POINT('Ctrl Pts',(-30.1082772334579,12.4770344340702,
128.597497281747)) ;
#126424=CARTESIAN_POINT('Ctrl Pts',(-30.1914295574665,12.6896430839443,
128.807450070267)) ;
#126425=CARTESIAN_POINT('Ctrl Pts',(-30.2541271970478,12.9554492280344,
128.957485437549)) ;
#126426=CARTESIAN_POINT('Ctrl Pts',(-30.2920888176688,13.2546656267019,
129.035282868155)) ;
#126427=CARTESIAN_POINT('Ctrl Pts',(-30.3033302444878,13.5672375771819,
129.034881121933)) ;
#126428=CARTESIAN_POINT('Ctrl Pts',(-30.2877588882589,13.8673528503954,
128.956383179478)) ;
#126429=CARTESIAN_POINT('Ctrl Pts',(-30.2473790223749,14.1367236573279,
128.805324735594)) ;
#126430=CARTESIAN_POINT('Ctrl Pts',(-30.1850909266063,14.3561277006207,
128.590031160462)) ;
#126431=CARTESIAN_POINT('Ctrl Pts',(-30.1075087264643,14.5065131900063,
128.33046827587)) ;
#126432=CARTESIAN_POINT('Ctrl Pts',(-30.0194926425284,14.5806176996537,
128.040156515334)) ;
#126433=CARTESIAN_POINT('Ctrl Pts',(-29.9289678243319,14.5715966835969,
127.742653447193)) ;
#126434=CARTESIAN_POINT('Ctrl Pts',(-29.8423608500082,14.4799160450286,
127.456405894327)) ;
#126435=CARTESIAN_POINT('Ctrl Pts',(-29.7675273190922,14.3130125765193,
127.204738155842)) ;
#126436=CARTESIAN_POINT('Ctrl Pts',(-29.7099347429233,14.0821691302311,
127.003364619287)) ;
#126437=CARTESIAN_POINT('Ctrl Pts',(-29.6745995577671,13.8046644835193,
126.86707664218)) ;
#126438=CARTESIAN_POINT('Ctrl Pts',(-29.6647800371637,13.4979410489725,
126.805115665796)) ;
#126439=CARTESIAN_POINT('Ctrl Pts',(-29.6818108175296,13.1889483563346,
126.821935190838)) ;
#126440=CARTESIAN_POINT('Ctrl Pts',(-29.725449588497,12.8939178220345,126.916172175486)) ;
#126441=CARTESIAN_POINT('Ctrl Pts',(-29.7931536798143,12.6378239154038,
127.080814108066)) ;
#126442=CARTESIAN_POINT('Ctrl Pts',(-29.8806868304317,12.4382802078468,
127.303412931666)) ;
#126443=CARTESIAN_POINT('Ctrl Pts',(-29.9822588186338,12.3092349638881,
127.567120846418)) ;
#126444=CARTESIAN_POINT('Ctrl Pts',(-30.0926065124654,12.2595575251469,
127.856171070087)) ;
#126445=CARTESIAN_POINT('Ctrl Pts',(-30.2024969870066,12.2934341319413,
128.14423155801)) ;
#126446=CARTESIAN_POINT('Ctrl Pts',(-30.3065648134954,12.4080333826879,
128.415084285074)) ;
#126447=CARTESIAN_POINT('Ctrl Pts',(-30.3975305959679,12.5960960403323,
128.647606332589)) ;
#126448=CARTESIAN_POINT('Ctrl Pts',(-30.4691722757746,12.843083593107,128.823760213034)) ;
#126449=CARTESIAN_POINT('Ctrl Pts',(-30.5173273876776,13.1299282656209,
128.931476599513)) ;
#126450=CARTESIAN_POINT('Ctrl Pts',(-30.5396604134547,13.4413370847319,
128.963362394438)) ;
#126451=CARTESIAN_POINT('Ctrl Pts',(-30.5347668850085,13.7480777848253,
128.916086109686)) ;
#126452=CARTESIAN_POINT('Ctrl Pts',(-30.5040750576494,14.0327532963684,
128.793312030853)) ;
#126453=CARTESIAN_POINT('Ctrl Pts',(-30.4504985045057,14.2736050959338,
128.603740694333)) ;
#126454=CARTESIAN_POINT('Ctrl Pts',(-30.3778747113513,14.4547314296563,
128.358256779292)) ;
#126455=CARTESIAN_POINT('Ctrl Pts',(-30.2936369428916,14.5602675742185,
128.079238780443)) ;
#126456=CARTESIAN_POINT('Ctrl Pts',(-30.2030290094892,14.5853381801731,
127.781348005785)) ;
#126457=CARTESIAN_POINT('Ctrl Pts',(-30.1141284940414,14.5268295873478,
127.488540590074)) ;
#126458=CARTESIAN_POINT('Ctrl Pts',(-30.0337309834468,14.3893357497607,
127.220546337056)) ;
#126459=CARTESIAN_POINT('Ctrl Pts',(-29.9684052682184,14.1825586684621,
126.996582667017)) ;
#126460=CARTESIAN_POINT('Ctrl Pts',(-29.9235216001179,13.9213687845982,
126.832333859035)) ;
#126461=CARTESIAN_POINT('Ctrl Pts',(-29.9031213775104,13.6242447212575,
126.739584038851)) ;
#126462=CARTESIAN_POINT('Ctrl Pts',(-29.9091301453683,13.3143403284212,
126.724162867979)) ;
#126463=CARTESIAN_POINT('Ctrl Pts',(-29.9424957055977,13.0084389968774,
126.788222170186)) ;
#126464=CARTESIAN_POINT('Ctrl Pts',(-30.0002782546044,12.7371908431784,
126.924201920801)) ;
#126465=CARTESIAN_POINT('Ctrl Pts',(-30.080582965063,12.5114337629303,127.125525392247)) ;
#126466=CARTESIAN_POINT('Ctrl Pts',(-30.1773238460316,12.3524149247727,
127.375054033863)) ;
#126467=CARTESIAN_POINT('Ctrl Pts',(-30.2849157680511,12.2696327934899,
127.656178093181)) ;
#126468=CARTESIAN_POINT('Ctrl Pts',(-30.3958487396615,12.2697667408868,
127.947150017038)) ;
#126469=CARTESIAN_POINT('Ctrl Pts',(-30.5031632538382,12.3522197325102,
128.227554335304)) ;
#126470=CARTESIAN_POINT('Ctrl Pts',(-30.6000761875062,12.5116177862274,
128.477515668528)) ;
#126471=CARTESIAN_POINT('Ctrl Pts',(-30.6800995647237,12.736082772034,128.678177449685)) ;
#126472=CARTESIAN_POINT('Ctrl Pts',(-30.738510649036,13.0105747690242,128.815605552237)) ;
#126473=CARTESIAN_POINT('Ctrl Pts',(-30.7714511773727,13.3146279151312,
128.878646647535)) ;
#126474=CARTESIAN_POINT('Ctrl Pts',(-30.7775275155768,13.6243832359542,
128.863434416948)) ;
#126475=CARTESIAN_POINT('Ctrl Pts',(-30.7570344764649,13.9217978697246,
128.770374564534)) ;
#126476=CARTESIAN_POINT('Ctrl Pts',(-30.7123207653944,14.1821018677862,
128.606738727323)) ;
#126477=CARTESIAN_POINT('Ctrl Pts',(-30.6468826077252,14.3894123612741,
128.382372687917)) ;
#126478=CARTESIAN_POINT('Ctrl Pts',(-30.5664940708433,14.5268848445949,
128.114414955078)) ;
#126479=CARTESIAN_POINT('Ctrl Pts',(-30.4774434259798,14.585256166508,127.821110439417)) ;
#126480=CARTESIAN_POINT('Ctrl Pts',(-30.387335916858,14.5605921317333,127.524875838204)) ;
#126481=CARTESIAN_POINT('Ctrl Pts',(-30.3024923367865,14.4542388415829,
127.243838232397)) ;
#126482=CARTESIAN_POINT('Ctrl Pts',(-30.230353520966,14.2743936202259,127.000011757054)) ;
#126483=CARTESIAN_POINT('Ctrl Pts',(-30.1763747618644,14.0316377152924,
126.808994082915)) ;
#126484=CARTESIAN_POINT('Ctrl Pts',(-30.1458639176194,13.7487556087195,
126.686973351521)) ;
#126485=CARTESIAN_POINT('Ctrl Pts',(-30.1410714925664,13.4387761357976,
126.639634653648)) ;
#126486=CARTESIAN_POINT('Ctrl Pts',(-30.1630937482503,13.131784657343,126.671100007775)) ;
#126487=CARTESIAN_POINT('Ctrl Pts',(-30.2118435570482,12.8410201909971,
126.78009912382)) ;
#126488=CARTESIAN_POINT('Ctrl Pts',(-30.2831176592298,12.5963886012332,
126.955444403938)) ;
#126489=CARTESIAN_POINT('Ctrl Pts',(-30.3738139118341,12.4083250161853,
127.187236450367)) ;
#126490=CARTESIAN_POINT('Ctrl Pts',(-30.4782746115266,12.2932606214,127.459115432517)) ;
#126491=CARTESIAN_POINT('Ctrl Pts',(-30.5880990881978,12.2596773190563,
127.747003747489)) ;
#126492=CARTESIAN_POINT('Ctrl Pts',(-30.6980230573031,12.3089369873083,
128.03494702501)) ;
#126493=CARTESIAN_POINT('Ctrl Pts',(-30.8001371723159,12.4384179192494,
128.300074442046)) ;
#126494=CARTESIAN_POINT('Ctrl Pts',(-30.887812752522,12.6389284665683,128.522996047447)) ;
#126495=CARTESIAN_POINT('Ctrl Pts',(-30.9550781560894,12.8936369055523,
128.686545839235)) ;
#126496=CARTESIAN_POINT('Ctrl Pts',(-30.9988884958278,13.1890353554826,
128.781232646274)) ;
#126497=CARTESIAN_POINT('Ctrl Pts',(-31.0158460752313,13.4997524264947,
128.797656813682)) ;
#126498=CARTESIAN_POINT('Ctrl Pts',(-31.0060377770145,13.8039809535807,
128.735996805114)) ;
#126499=CARTESIAN_POINT('Ctrl Pts',(-30.9707318332435,14.0820722250227,
128.599733823845)) ;
#126500=CARTESIAN_POINT('Ctrl Pts',(-30.9131292647479,14.3130041304952,
128.398329360413)) ;
#126501=CARTESIAN_POINT('Ctrl Pts',(-30.8381066903904,14.4800545558914,
128.146034853665)) ;
#126502=CARTESIAN_POINT('Ctrl Pts',(-30.7520139126598,14.5714592047604,
127.861485917471)) ;
#126503=CARTESIAN_POINT('Ctrl Pts',(-30.6608114307688,14.580498376248,127.561746515086)) ;
#126504=CARTESIAN_POINT('Ctrl Pts',(-30.5734428928017,14.5069052062207,
127.273578758881)) ;
#126505=CARTESIAN_POINT('Ctrl Pts',(-30.4953155212185,14.355702929433,127.012199444464)) ;
#126506=CARTESIAN_POINT('Ctrl Pts',(-30.4333260025628,14.1367618967332,
126.797892231372)) ;
#126507=CARTESIAN_POINT('Ctrl Pts',(-30.3928708035435,13.8680692745211,
126.646669018808)) ;
#126508=CARTESIAN_POINT('Ctrl Pts',(-30.3772964122241,13.5652241802336,
126.567869881532)) ;
#126509=CARTESIAN_POINT('Ctrl Pts',(-30.3884947265944,13.2558695648544,
126.567689426035)) ;
#126510=CARTESIAN_POINT('Ctrl Pts',(-30.4264241019016,12.9557645621013,
126.645297590501)) ;
#126511=CARTESIAN_POINT('Ctrl Pts',(-30.489041829683,12.6900041384903,126.795125628811)) ;
#126512=CARTESIAN_POINT('Ctrl Pts',(-30.5727955453991,12.4761054960812,
127.006609410694)) ;
#126513=CARTESIAN_POINT('Ctrl Pts',(-30.6723385952662,12.330458638013,127.264220196088)) ;
#126514=CARTESIAN_POINT('Ctrl Pts',(-30.7805975050551,12.2634381555471,
127.547468405064)) ;
#126515=CARTESIAN_POINT('Ctrl Pts',(-30.8914731168471,12.2788783725225,
127.838251911419)) ;
#126516=CARTESIAN_POINT('Ctrl Pts',(-30.997731735831,12.3768660101259,128.115439269918)) ;
#126517=CARTESIAN_POINT('Ctrl Pts',(-31.0918372330593,12.5495630530058,
128.357227024484)) ;
#126518=CARTESIAN_POINT('Ctrl Pts',(-31.1682535327665,12.7855771799242,
128.547247795842)) ;
#126519=CARTESIAN_POINT('Ctrl Pts',(-31.2216790671275,13.0654345443907,
128.67033565722)) ;
#126520=CARTESIAN_POINT('Ctrl Pts',(-31.249754075546,13.3720089515071,128.719222227115)) ;
#126521=CARTESIAN_POINT('Ctrl Pts',(-31.2507732919044,13.6824357040732,
128.689053740515)) ;
#126522=CARTESIAN_POINT('Ctrl Pts',(-31.2255503193694,13.9739144872618,
128.582277192005)) ;
#126523=CARTESIAN_POINT('Ctrl Pts',(-31.1762431065979,14.2268633761364,
128.404991190371)) ;
#126524=CARTESIAN_POINT('Ctrl Pts',(-31.1080584867575,14.4204385567601,
128.172885282172)) ;
#126525=CARTESIAN_POINT('Ctrl Pts',(-31.0249588173677,14.5445800980489,
127.896763573076)) ;
#126526=CARTESIAN_POINT('Ctrl Pts',(-30.9354496148306,14.5868220517618,
127.602269386102)) ;
#126527=CARTESIAN_POINT('Ctrl Pts',(-30.8458602695974,14.5468039115563,
127.307542979927)) ;
#126528=CARTESIAN_POINT('Ctrl Pts',(-30.762551181364,14.4251034056979,127.030856610899)) ;
#126529=CARTESIAN_POINT('Ctrl Pts',(-30.6937022254225,14.2325286559051,
126.796691431518)) ;
#126530=CARTESIAN_POINT('Ctrl Pts',(-30.6440265776777,13.9823226082249,
126.618508827956)) ;
#126531=CARTESIAN_POINT('Ctrl Pts',(-30.6179403580397,13.6900857614276,
126.509023742768)) ;
#126532=CARTESIAN_POINT('Ctrl Pts',(-30.6182858076127,13.3811329933267,
126.4770263894)) ;
#126533=CARTESIAN_POINT('Ctrl Pts',(-30.6454939352929,13.0742211924304,
126.523392436635)) ;
#126534=CARTESIAN_POINT('Ctrl Pts',(-30.6984799823791,12.7922255681548,
126.645059926506)) ;
#126535=CARTESIAN_POINT('Ctrl Pts',(-30.7743696130924,12.5548593941868,
126.833548883208)) ;
#126536=CARTESIAN_POINT('Ctrl Pts',(-30.8681675859231,12.3804086208566,
127.074416612223)) ;
#126537=CARTESIAN_POINT('Ctrl Pts',(-30.9734327320213,12.2809059673708,
127.348936065361)) ;
#126538=CARTESIAN_POINT('Ctrl Pts',(-31.0843011975214,12.2624888540407,
127.639685234248)) ;
#126539=CARTESIAN_POINT('Ctrl Pts',(-31.1933595883704,12.3276777325191,
127.925074837892)) ;
#126540=CARTESIAN_POINT('Ctrl Pts',(-31.2928028436846,12.4707929525642,
128.182534472415)) ;
#126541=CARTESIAN_POINT('Ctrl Pts',(-31.3770533192461,12.6823314867526,
128.395518029563)) ;
#126542=CARTESIAN_POINT('Ctrl Pts',(-31.4405599270799,12.9478032750239,
128.547819525315)) ;
#126543=CARTESIAN_POINT('Ctrl Pts',(-31.4792159130957,13.2466924677811,
128.627614460685)) ;
#126544=CARTESIAN_POINT('Ctrl Pts',(-31.4911477632263,13.5583773879723,
128.629318254641)) ;
#126545=CARTESIAN_POINT('Ctrl Pts',(-31.4763826013898,13.8592557726353,
128.553168178792)) ;
#126546=CARTESIAN_POINT('Ctrl Pts',(-31.4363656825528,14.1306426193177,
128.403029564233)) ;
#126547=CARTESIAN_POINT('Ctrl Pts',(-31.3753860029681,14.3493760513521,
128.191947439307)) ;
#126548=CARTESIAN_POINT('Ctrl Pts',(-31.2975897155965,14.5035317935641,
127.93146804733)) ;
#126549=CARTESIAN_POINT('Ctrl Pts',(-31.2099294270891,14.5795845166173,
127.642277005627)) ;
#126550=CARTESIAN_POINT('Ctrl Pts',(-31.119205465658,14.5729335427119,127.344118226607)) ;
#126551=CARTESIAN_POINT('Ctrl Pts',(-31.0326800003559,14.4838964505683,
127.058232114227)) ;
#126552=CARTESIAN_POINT('Ctrl Pts',(-30.9572247193135,14.3187457002778,
126.804663885965)) ;
#126553=CARTESIAN_POINT('Ctrl Pts',(-30.8991368803147,14.0897675242826,
126.601886443905)) ;
#126554=CARTESIAN_POINT('Ctrl Pts',(-30.8630850303705,13.8134082052382,
126.463502880507)) ;
#126555=CARTESIAN_POINT('Ctrl Pts',(-30.8524556689723,13.5073935686165,
126.399199801176)) ;
#126556=CARTESIAN_POINT('Ctrl Pts',(-30.8687507658311,13.1976576575877,
126.413804359631)) ;
#126557=CARTESIAN_POINT('Ctrl Pts',(-30.9114804240192,12.902722923634,126.505492871026)) ;
#126558=CARTESIAN_POINT('Ctrl Pts',(-30.9786025123769,12.6448108187769,
126.668379584555)) ;
#126559=CARTESIAN_POINT('Ctrl Pts',(-31.0654092817325,12.4434495534872,
126.888919406482)) ;
#126560=CARTESIAN_POINT('Ctrl Pts',(-31.1676204617471,12.3113759719957,
127.154188555509)) ;
#126561=CARTESIAN_POINT('Ctrl Pts',(-31.2766504169667,12.2599503304337,
127.439757637193)) ;
#126562=CARTESIAN_POINT('Ctrl Pts',(-31.3875029822561,12.291369325937,127.730360541563)) ;
#126563=CARTESIAN_POINT('Ctrl Pts',(-31.4915349615509,12.4038516063155,
128.00120069853)) ;
#126564=CARTESIAN_POINT('Ctrl Pts',(-31.5827029401584,12.5892626492753,
128.23441173148)) ;
#126565=CARTESIAN_POINT('Ctrl Pts',(-31.6550420442372,12.8342966688913,
128.412632130978)) ;
#126566=CARTESIAN_POINT('Ctrl Pts',(-31.7042037977048,13.122430564087,128.523040487345)) ;
#126567=CARTESIAN_POINT('Ctrl Pts',(-31.7271063430556,13.4307504301952,
128.55689464633)) ;
#126568=CARTESIAN_POINT('Ctrl Pts',(-31.7231059517512,13.7394115406098,
128.512058436927)) ;
#126569=CARTESIAN_POINT('Ctrl Pts',(-31.6930932489722,14.0250582572476,
128.391271941973)) ;
#126570=CARTESIAN_POINT('Ctrl Pts',(-31.6400121197202,14.2676857637035,
128.203093777817)) ;
#126571=CARTESIAN_POINT('Ctrl Pts',(-31.5681740871473,14.4501343866895,
127.960050172645)) ;
#126572=CARTESIAN_POINT('Ctrl Pts',(-31.4837806638188,14.5585281733049,
127.680404650567)) ;
#126573=CARTESIAN_POINT('Ctrl Pts',(-31.393485187641,14.5857500263022,127.383523473882)) ;
#126574=CARTESIAN_POINT('Ctrl Pts',(-31.3042926382178,14.5296138137444,
127.089807373214)) ;
#126575=CARTESIAN_POINT('Ctrl Pts',(-31.2235650511201,14.3940563365778,
126.820842233824)) ;
#126576=CARTESIAN_POINT('Ctrl Pts',(-31.157899893824,14.1896705870724,126.595977084309)) ;
#126577=CARTESIAN_POINT('Ctrl Pts',(-31.112275041275,13.929679500594,126.42953375103)) ;
#126578=CARTESIAN_POINT('Ctrl Pts',(-31.0910923977529,13.6325613008054,
126.334421909125)) ;
#126579=CARTESIAN_POINT('Ctrl Pts',(-31.0964447394053,13.3229079041448,
126.31709545029)) ;
#126580=CARTESIAN_POINT('Ctrl Pts',(-31.1286944233721,13.0185266052724,
126.378131100081)) ;
#126581=CARTESIAN_POINT('Ctrl Pts',(-31.1861978833459,12.7436673209471,
126.513013327565)) ;
#126582=CARTESIAN_POINT('Ctrl Pts',(-31.2661117501715,12.5164978313935,
126.713179834526)) ;
#126583=CARTESIAN_POINT('Ctrl Pts',(-31.3620916624292,12.3560839841268,
126.960609857562)) ;
#126584=CARTESIAN_POINT('Ctrl Pts',(-31.4694894479972,12.2708854639731,
127.241159005647)) ;
#126585=CARTESIAN_POINT('Ctrl Pts',(-31.5802782657031,12.2685612257957,
127.531751335238)) ;
#126586=CARTESIAN_POINT('Ctrl Pts',(-31.6879941774975,12.3486010166685,
127.813276464684)) ;
#126587=CARTESIAN_POINT('Ctrl Pts',(-31.7856635186791,12.5069431442139,
128.065300796062)) ;
#126588=CARTESIAN_POINT('Ctrl Pts',(-31.8657144711242,12.7284060361604,
128.266254738305)) ;
#126589=CARTESIAN_POINT('Ctrl Pts',(-31.9250227559616,13.0024846524795,
128.406199840165)) ;
#126590=CARTESIAN_POINT('Ctrl Pts',(-31.95863385165,13.3053157268251,128.471280232653)) ;
#126591=CARTESIAN_POINT('Ctrl Pts',(-31.9654947472056,13.6156287863426,
128.458302913958)) ;
#126592=CARTESIAN_POINT('Ctrl Pts',(-31.9458820818508,13.9128850712382,
128.367926847057)) ;
#126593=CARTESIAN_POINT('Ctrl Pts',(-31.9014415972457,14.1766185876755,
128.204813826453)) ;
#126594=CARTESIAN_POINT('Ctrl Pts',(-31.8365595302308,14.3847399014371,
127.982162035615)) ;
#126595=CARTESIAN_POINT('Ctrl Pts',(-31.7568066659652,14.5238361204557,
127.716174800887)) ;
#126596=CARTESIAN_POINT('Ctrl Pts',(-31.6680261972628,14.5847743037998,
127.423702490199)) ;
#126597=CARTESIAN_POINT('Ctrl Pts',(-31.5774936879742,14.562330930931,127.126086462082)) ;
#126598=CARTESIAN_POINT('Ctrl Pts',(-31.4925141748482,14.4584177990408,
126.844713248296)) ;
#126599=CARTESIAN_POINT('Ctrl Pts',(-31.4196806977938,14.2791868588028,
126.59868079849)) ;
#126600=CARTESIAN_POINT('Ctrl Pts',(-31.365769806941,14.0415186925473,126.408335160599)) ;
#126601=CARTESIAN_POINT('Ctrl Pts',(-31.3341067123459,13.7564325224017,
126.28254734767)) ;
#126602=CARTESIAN_POINT('Ctrl Pts',(-31.3285693219295,13.4495648486799,
126.233344992335)) ;
#126603=CARTESIAN_POINT('Ctrl Pts',(-31.3499996979768,13.1394167822153,
126.262757635103)) ;
#126604=CARTESIAN_POINT('Ctrl Pts',(-31.3974714496979,12.8508801279426,
126.368398084406)) ;
#126605=CARTESIAN_POINT('Ctrl Pts',(-31.4686226776466,12.6022770183791,
126.543082974062)) ;
#126606=CARTESIAN_POINT('Ctrl Pts',(-31.5588216270401,12.4127865792607,
126.773465057354)) ;
#126607=CARTESIAN_POINT('Ctrl Pts',(-31.662947243727,12.2953916608247,127.044370815528)) ;
#126608=CARTESIAN_POINT('Ctrl Pts',(-31.7729256743816,12.2594835078991,
127.332640515269)) ;
#126609=CARTESIAN_POINT('Ctrl Pts',(-31.8827463763512,12.3065006928956,
127.620343819185)) ;
#126610=CARTESIAN_POINT('Ctrl Pts',(-31.984917749441,12.4331949975966,127.8857354975)) ;
#126611=CARTESIAN_POINT('Ctrl Pts',(-32.0734252963866,12.6325251245457,
128.110965015092)) ;
#126612=CARTESIAN_POINT('Ctrl Pts',(-32.1411877862138,12.8854154202419,
128.276032660269)) ;
#126613=CARTESIAN_POINT('Ctrl Pts',(-32.185775956454,13.1803567120122,128.37294829569)) ;
#126614=CARTESIAN_POINT('Ctrl Pts',(-32.2034899901905,13.4893561619414,
128.391747881859)) ;
#126615=CARTESIAN_POINT('Ctrl Pts',(-32.1945262955173,13.7954471105094,
128.33241062473)) ;
#126616=CARTESIAN_POINT('Ctrl Pts',(-32.1597610137556,14.0751705649909,
128.197652005603)) ;
#126617=CARTESIAN_POINT('Ctrl Pts',(-32.102880816017,14.3069080842483,127.998454341013)) ;
#126618=CARTESIAN_POINT('Ctrl Pts',(-32.0283825626093,14.4762413340772,
127.747712728677)) ;
#126619=CARTESIAN_POINT('Ctrl Pts',(-31.9418077598481,14.5702449830263,
127.461492883282)) ;
#126620=CARTESIAN_POINT('Ctrl Pts',(-31.8514803012559,14.5813885604022,
127.16462576914)) ;
#126621=CARTESIAN_POINT('Ctrl Pts',(-31.7634476739157,14.5100796553899,
126.874340511653)) ;
#126622=CARTESIAN_POINT('Ctrl Pts',(-31.6848485468524,14.3602444697485,
126.611517403404)) ;
#126623=CARTESIAN_POINT('Ctrl Pts',(-31.6225173073783,14.1432531479422,
126.396278974897)) ;
#126624=CARTESIAN_POINT('Ctrl Pts',(-31.5815599114105,13.8766589305714,
126.243700317679)) ;
#126625=CARTESIAN_POINT('Ctrl Pts',(-31.5651586334022,13.575471110015,126.162588536627)) ;
#126626=CARTESIAN_POINT('Ctrl Pts',(-31.5755523169396,13.2645667872771,
126.159895817134)) ;
#126627=CARTESIAN_POINT('Ctrl Pts',(-31.6128773468518,12.9634276879521,
126.235689544571)) ;
#126628=CARTESIAN_POINT('Ctrl Pts',(-31.6746702091294,12.6972348288673,
126.383202615797)) ;
#126629=CARTESIAN_POINT('Ctrl Pts',(-31.7577635170574,12.4817230037899,
126.592791547872)) ;
#126630=CARTESIAN_POINT('Ctrl Pts',(-31.8568476398735,12.3338051645045,
126.849080745658)) ;
#126631=CARTESIAN_POINT('Ctrl Pts',(-31.9652781019356,12.2641455947444,
127.132724501552)) ;
#126632=CARTESIAN_POINT('Ctrl Pts',(-32.0761113464017,12.2773535863406,
127.423406237724)) ;
#126633=CARTESIAN_POINT('Ctrl Pts',(-32.1823624472709,12.3726335000392,
127.700655595375)) ;
#126634=CARTESIAN_POINT('Ctrl Pts',(-32.2770427894398,12.5434758841393,
127.944074783812)) ;
#126635=CARTESIAN_POINT('Ctrl Pts',(-32.3538549195629,12.7769498129424,
128.135364285058)) ;
#126636=CARTESIAN_POINT('Ctrl Pts',(-32.4083145195709,13.0568800238177,
128.261324343271)) ;
#126637=CARTESIAN_POINT('Ctrl Pts',(-32.4371265032857,13.3636449854545,
128.312303479849)) ;
#126638=CARTESIAN_POINT('Ctrl Pts',(-32.4388913807184,13.6733774781512,
128.28440725804)) ;
#126639=CARTESIAN_POINT('Ctrl Pts',(-32.4144856546222,13.9654381108949,
128.180052252876)) ;
#126640=CARTESIAN_POINT('Ctrl Pts',(-32.3657873055419,14.2203012801684,
128.004497044474)) ;
#126641=CARTESIAN_POINT('Ctrl Pts',(-32.2979066090449,14.4159470499748,
127.773210152946)) ;
#126642=CARTESIAN_POINT('Ctrl Pts',(-32.2156445726619,14.541694367896,127.499738746105)) ;
#126643=CARTESIAN_POINT('Ctrl Pts',(-32.1258917680055,14.5869018897487,
127.204394863701)) ;
#126644=CARTESIAN_POINT('Ctrl Pts',(-32.0360732595204,14.5489491309812,
126.908948138677)) ;
#126645=CARTESIAN_POINT('Ctrl Pts',(-31.9527424544331,14.4300240468882,
126.632315927122)) ;
#126646=CARTESIAN_POINT('Ctrl Pts',(-31.8831245966444,14.2387296194583,
126.395780395041)) ;
#126647=CARTESIAN_POINT('Ctrl Pts',(-31.8329411061117,13.9899468992174,
126.216137846651)) ;
#126648=CARTESIAN_POINT('Ctrl Pts',(-31.8062039119009,13.7002922296482,
126.10493343788)) ;
#126649=CARTESIAN_POINT('Ctrl Pts',(-31.8055981139312,13.3909003011237,
126.070079831623)) ;
#126650=CARTESIAN_POINT('Ctrl Pts',(-31.8322241901464,13.0819914193172,
126.114572771983)) ;
#126651=CARTESIAN_POINT('Ctrl Pts',(-31.8843911764362,12.8000707089261,
126.233963093376)) ;
#126652=CARTESIAN_POINT('Ctrl Pts',(-31.959405494078,12.561613461146,126.419982896461)) ;
#126653=CARTESIAN_POINT('Ctrl Pts',(-32.0529214736794,12.3844498728761,
126.659951432733)) ;
#126654=CARTESIAN_POINT('Ctrl Pts',(-32.1584695989366,12.2824628123426,
126.935138173326)) ;
#126655=CARTESIAN_POINT('Ctrl Pts',(-32.2687092503971,12.2618989630133,
127.224226185651)) ;
#126656=CARTESIAN_POINT('Ctrl Pts',(-32.3780664721287,12.3245801672036,
127.510447715042)) ;
#126657=CARTESIAN_POINT('Ctrl Pts',(-32.4778727214042,12.4655890286878,
127.768967737361)) ;
#126658=CARTESIAN_POINT('Ctrl Pts',(-32.562635692592,12.6753258983896,127.983450429838)) ;
#126659=CARTESIAN_POINT('Ctrl Pts',(-32.6267495393494,12.9389696147355,
128.137585318208)) ;
#126660=CARTESIAN_POINT('Ctrl Pts',(-32.6662243013269,13.2377442398154,
128.219703177418)) ;
#126661=CARTESIAN_POINT('Ctrl Pts',(-32.6789869482266,13.5478078732814,
128.224005737763)) ;
#126662=CARTESIAN_POINT('Ctrl Pts',(-32.6649289811142,13.8515136096922,
128.149675334215)) ;
#126663=CARTESIAN_POINT('Ctrl Pts',(-32.6256750103247,14.1231097969316,
128.001882287398)) ;
#126664=CARTESIAN_POINT('Ctrl Pts',(-32.5651689894839,14.3439547255393,
127.792123518752)) ;
#126665=CARTESIAN_POINT('Ctrl Pts',(-32.4879714740893,14.4998917409251,
127.533482233047)) ;
#126666=CARTESIAN_POINT('Ctrl Pts',(-32.400211067042,14.5786386561727,127.243881113999)) ;
#126667=CARTESIAN_POINT('Ctrl Pts',(-32.3095247060737,14.574267489829,126.945855302846)) ;
#126668=CARTESIAN_POINT('Ctrl Pts',(-32.2227184803242,14.4873446647109,
126.65911777222)) ;
#126669=CARTESIAN_POINT('Ctrl Pts',(-32.1471010239481,14.3247913257021,
126.405185591465)) ;
#126670=CARTESIAN_POINT('Ctrl Pts',(-32.0882333339096,14.0970301472897,
126.200046528919)) ;
#126671=CARTESIAN_POINT('Ctrl Pts',(-32.0514651201517,13.820492300365,126.059438557222)) ;
#126672=CARTESIAN_POINT('Ctrl Pts',(-32.0401940508131,13.5164548784845,
125.993426980055)) ;
#126673=CARTESIAN_POINT('Ctrl Pts',(-32.0557122282716,13.2060699162722,
126.00570482415)) ;
#126674=CARTESIAN_POINT('Ctrl Pts',(-32.0977788098025,12.9102232065258,
126.095437968778)) ;
#126675=CARTESIAN_POINT('Ctrl Pts',(-32.1644236899613,12.6507291243944,
126.25688138731)) ;
#126676=CARTESIAN_POINT('Ctrl Pts',(-32.2504533776306,12.4485585440169,
126.475276109183)) ;
#126677=CARTESIAN_POINT('Ctrl Pts',(-32.3517721832678,12.3145373722517,
126.738100326614)) ;
#126678=CARTESIAN_POINT('Ctrl Pts',(-32.4612996077681,12.2601564021124,
127.024927652369)) ;
#126679=CARTESIAN_POINT('Ctrl Pts',(-32.572190253351,12.2893926148143,127.315652329271)) ;
#126680=CARTESIAN_POINT('Ctrl Pts',(-32.6764790046662,12.3994366791386,
127.587256135716)) ;
#126681=CARTESIAN_POINT('Ctrl Pts',(-32.7684650814352,12.5839727255082,
127.822707706638)) ;
#126682=CARTESIAN_POINT('Ctrl Pts',(-32.841004593203,12.8264920327129,128.001671494392)) ;
#126683=CARTESIAN_POINT('Ctrl Pts',(-32.8910099340424,13.1141225858941,
128.11449164118)) ;
#126684=CARTESIAN_POINT('Ctrl Pts',(-32.9067217529341,13.3194871424456,
128.138350053268)) ;
#126685=CARTESIAN_POINT('Ctrl Pts',(-32.9101349058941,13.4222384841719,
128.137300004128)) ;
#126686=CARTESIAN_POINT('Ctrl Pts',(-11.3289906305328,13.1368456608817,
133.132150944256)) ;
#126687=CARTESIAN_POINT('Ctrl Pts',(-11.3297648820373,13.1302434176427,
133.133681768478)) ;
#126688=CARTESIAN_POINT('Ctrl Pts',(-11.3423989273914,13.0249710001428,
133.158906544104)) ;
#126689=CARTESIAN_POINT('Ctrl Pts',(-11.3769158459995,12.826301888656,133.236764259813)) ;
#126690=CARTESIAN_POINT('Ctrl Pts',(-11.4497170247885,12.5833995163819,
133.416412389735)) ;
#126691=CARTESIAN_POINT('Ctrl Pts',(-11.5412607886117,12.3996267668574,
133.650728855637)) ;
#126692=CARTESIAN_POINT('Ctrl Pts',(-11.646261583587,12.289073168245,133.924189213627)) ;
#126693=CARTESIAN_POINT('Ctrl Pts',(-11.756222160173,12.2602312941192,134.21248261213)) ;
#126694=CARTESIAN_POINT('Ctrl Pts',(-11.8660584839532,12.3144254424815,
134.500116213875)) ;
#126695=CARTESIAN_POINT('Ctrl Pts',(-11.9672384530468,12.4480642715863,
134.762596430137)) ;
#126696=CARTESIAN_POINT('Ctrl Pts',(-12.0538295019936,12.6516399513856,
134.982407105695)) ;
#126697=CARTESIAN_POINT('Ctrl Pts',(-12.1201383915298,12.9104452496318,
135.142988694336)) ;
#126698=CARTESIAN_POINT('Ctrl Pts',(-12.1621810540703,13.2058492015505,
135.232691768976)) ;
#126699=CARTESIAN_POINT('Ctrl Pts',(-12.1777749644098,13.5166184921212,
135.245154976188)) ;
#126700=CARTESIAN_POINT('Ctrl Pts',(-12.1662881003302,13.8224100223415,
135.178309260546)) ;
#126701=CARTESIAN_POINT('Ctrl Pts',(-12.1296615754862,14.0967865008827,
135.038352263151)) ;
#126702=CARTESIAN_POINT('Ctrl Pts',(-12.0709572339323,14.3244562986112,
134.833732882778)) ;
#126703=CARTESIAN_POINT('Ctrl Pts',(-11.9951612200146,14.4874741997871,
134.579198900516)) ;
#126704=CARTESIAN_POINT('Ctrl Pts',(-11.9081860961099,14.5744204937736,
134.291910355936)) ;
#126705=CARTESIAN_POINT('Ctrl Pts',(-11.8174705117483,14.5784621737365,
133.993787488894)) ;
#126706=CARTESIAN_POINT('Ctrl Pts',(-11.7301428372465,14.5000469778991,
133.705611198596)) ;
#126707=CARTESIAN_POINT('Ctrl Pts',(-11.6529450720055,14.3445727249932,
133.446993574372)) ;
#126708=CARTESIAN_POINT('Ctrl Pts',(-11.5921201640469,14.122833835347,133.236157417965)) ;
#126709=CARTESIAN_POINT('Ctrl Pts',(-11.5529082022929,13.8501516984393,
133.088384911782)) ;
#126710=CARTESIAN_POINT('Ctrl Pts',(-11.5389594641307,13.5490423779197,
133.014658231721)) ;
#126711=CARTESIAN_POINT('Ctrl Pts',(-11.5516658542996,13.2374717045801,
133.018634830279)) ;
#126712=CARTESIAN_POINT('Ctrl Pts',(-11.5912618190877,12.9386844676289,
133.101096607348)) ;
#126713=CARTESIAN_POINT('Ctrl Pts',(-11.6550459597695,12.6761377246457,
133.254414846195)) ;
#126714=CARTESIAN_POINT('Ctrl Pts',(-11.739911901217,12.4657586790897,133.469131818159)) ;
#126715=CARTESIAN_POINT('Ctrl Pts',(-11.8398105621753,12.3246285674056,
133.727893177096)) ;
#126716=CARTESIAN_POINT('Ctrl Pts',(-11.9491259530435,12.2619062239342,
134.014003245861)) ;
#126717=CARTESIAN_POINT('Ctrl Pts',(-12.0595466130642,12.282438835861,134.303567791795)) ;
#126718=CARTESIAN_POINT('Ctrl Pts',(-12.1652800488837,12.3848777571664,
134.579229631052)) ;
#126719=CARTESIAN_POINT('Ctrl Pts',(-12.2583983620761,12.5614991790326,
134.818162626115)) ;
#126720=CARTESIAN_POINT('Ctrl Pts',(-12.3334889598739,12.7995868191894,
135.004422494166)) ;
#126721=CARTESIAN_POINT('Ctrl Pts',(-12.3859540985011,13.084029998422,135.124408150865)) ;
#126722=CARTESIAN_POINT('Ctrl Pts',(-12.4122116510868,13.3899587273314,
135.168153572099)) ;
#126723=CARTESIAN_POINT('Ctrl Pts',(-12.4117844343827,13.6996411393276,
135.133791161841)) ;
#126724=CARTESIAN_POINT('Ctrl Pts',(-12.3849432646615,13.9903747350237,
135.022164919903)) ;
#126725=CARTESIAN_POINT('Ctrl Pts',(-12.3346188008902,14.2393240390192,
134.842065868188)) ;
#126726=CARTESIAN_POINT('Ctrl Pts',(-12.2651915907767,14.429840029191,134.606193033354)) ;
#126727=CARTESIAN_POINT('Ctrl Pts',(-12.1821120354275,14.5487685207819,
134.330379497108)) ;
#126728=CARTESIAN_POINT('Ctrl Pts',(-12.0919098184049,14.5869290462078,
134.033669627662)) ;
#126729=CARTESIAN_POINT('Ctrl Pts',(-12.0024629512785,14.5417666879112,
133.739329945311)) ;
#126730=CARTESIAN_POINT('Ctrl Pts',(-11.920119663901,14.4163781206347,133.46561377521)) ;
#126731=CARTESIAN_POINT('Ctrl Pts',(-11.8519259373826,14.2194053236093,
133.233226952296)) ;
#126732=CARTESIAN_POINT('Ctrl Pts',(-11.8036364484147,13.9666437025949,
133.059143893317)) ;
#126733=CARTESIAN_POINT('Ctrl Pts',(-11.7789832629656,13.6737230311142,
132.953945062575)) ;
#126734=CARTESIAN_POINT('Ctrl Pts',(-11.7808284718151,13.3629183159293,
132.926175916698)) ;
#126735=CARTESIAN_POINT('Ctrl Pts',(-11.8096149856141,13.0570541461369,
132.977171113818)) ;
#126736=CARTESIAN_POINT('Ctrl Pts',(-11.8639395888902,12.7772474401736,
133.102769292852)) ;
#126737=CARTESIAN_POINT('Ctrl Pts',(-11.9411870980062,12.542768054334,133.295164838442)) ;
#126738=CARTESIAN_POINT('Ctrl Pts',(-12.0353149573993,12.3730788461159,
133.537173788383)) ;
#126739=CARTESIAN_POINT('Ctrl Pts',(-12.1416212392354,12.2773830517675,
133.814552713987)) ;
#126740=CARTESIAN_POINT('Ctrl Pts',(-12.2525579395139,12.2641121727855,
134.105508450141)) ;
#126741=CARTESIAN_POINT('Ctrl Pts',(-12.3609993187246,12.3337583329821,
134.389180372102)) ;
#126742=CARTESIAN_POINT('Ctrl Pts',(-12.4599209105406,12.4813160749921,
134.645053011495)) ;
#126743=CARTESIAN_POINT('Ctrl Pts',(-12.5431324196802,12.6966779854676,
134.854974313712)) ;
#126744=CARTESIAN_POINT('Ctrl Pts',(-12.60513159688,12.964058481658,135.002951427607)) ;
#126745=CARTESIAN_POINT('Ctrl Pts',(-12.642248673285,13.2633621106785,135.078341105324)) ;
#126746=CARTESIAN_POINT('Ctrl Pts',(-12.6527915834591,13.5752568041736,
135.075975212479)) ;
#126747=CARTESIAN_POINT('Ctrl Pts',(-12.6363641393793,13.8766502651513,
134.994767154178)) ;
#126748=CARTESIAN_POINT('Ctrl Pts',(-12.5953057530699,14.1438626179913,
134.841815741776)) ;
#126749=CARTESIAN_POINT('Ctrl Pts',(-12.5327277376817,14.3611558339141,
134.625772535533)) ;
#126750=CARTESIAN_POINT('Ctrl Pts',(-12.454244121328,14.5102070990302,134.363363036415)) ;
#126751=CARTESIAN_POINT('Ctrl Pts',(-12.3666258464247,14.5813677878946,
134.074440573705)) ;
#126752=CARTESIAN_POINT('Ctrl Pts',(-12.2757841730223,14.5701315008181,
133.775881282886)) ;
#126753=CARTESIAN_POINT('Ctrl Pts',(-12.1894313961296,14.4759919036324,
133.490385986915)) ;
#126754=CARTESIAN_POINT('Ctrl Pts',(-12.114965878112,14.3066892752371,133.239748050331)) ;
#126755=CARTESIAN_POINT('Ctrl Pts',(-12.0581822625266,14.0751878826871,
133.040876769225)) ;
#126756=CARTESIAN_POINT('Ctrl Pts',(-12.0234738677265,13.7962286869884,
132.906363788813)) ;
#126757=CARTESIAN_POINT('Ctrl Pts',(-12.0143364764407,13.4897393053989,
132.846474596732)) ;
#126758=CARTESIAN_POINT('Ctrl Pts',(-12.0324237013593,13.1781056984616,
132.866070228703)) ;
#126759=CARTESIAN_POINT('Ctrl Pts',(-12.076404053086,12.8871394706553,132.961667742337)) ;
#126760=CARTESIAN_POINT('Ctrl Pts',(-12.144800910124,12.6313543123433,133.128229561128)) ;
#126761=CARTESIAN_POINT('Ctrl Pts',(-12.2330625930333,12.4333423882355,
133.352887813321)) ;
#126762=CARTESIAN_POINT('Ctrl Pts',(-12.3347905478153,12.3067788270204,
133.617104693997)) ;
#126763=CARTESIAN_POINT('Ctrl Pts',(-12.4451693867627,12.2592790115486,
133.906271890683)) ;
#126764=CARTESIAN_POINT('Ctrl Pts',(-12.555523569585,12.2958890743791,134.195519227349)) ;
#126765=CARTESIAN_POINT('Ctrl Pts',(-12.6588209278628,12.412515962942,134.464262947306)) ;
#126766=CARTESIAN_POINT('Ctrl Pts',(-12.7491570807097,12.6017795206287,
134.695024073182)) ;
#126767=CARTESIAN_POINT('Ctrl Pts',(-12.8204405039154,12.850882040149,134.870032322403)) ;
#126768=CARTESIAN_POINT('Ctrl Pts',(-12.8678707015775,13.1389626258658,
134.975599031413)) ;
#126769=CARTESIAN_POINT('Ctrl Pts',(-12.8894078132323,13.4502019142914,
135.005209681357)) ;
#126770=CARTESIAN_POINT('Ctrl Pts',(-12.8836925621681,13.7571545177325,
134.955462993416)) ;
#126771=CARTESIAN_POINT('Ctrl Pts',(-12.8524412071742,14.0399279671086,
134.831176385702)) ;
#126772=CARTESIAN_POINT('Ctrl Pts',(-12.7978983539385,14.2804627439869,
134.638584865143)) ;
#126773=CARTESIAN_POINT('Ctrl Pts',(-12.7255120770098,14.4580430421026,
134.394109587671)) ;
#126774=CARTESIAN_POINT('Ctrl Pts',(-12.6404688487952,14.5623041816762,
134.112503175951)) ;
#126775=CARTESIAN_POINT('Ctrl Pts',(-12.5501362245032,14.5848738304735,
133.815550736798)) ;
#126776=CARTESIAN_POINT('Ctrl Pts',(-12.4608432203707,14.5236285286568,
133.521387838919)) ;
#126777=CARTESIAN_POINT('Ctrl Pts',(-12.3811865324715,14.3842858734187,
133.255704176636)) ;
#126778=CARTESIAN_POINT('Ctrl Pts',(-12.316331454127,14.176003666528,133.03312326242)) ;
#126779=CARTESIAN_POINT('Ctrl Pts',(-12.2719898795752,13.9123645540699,
132.870327548437)) ;
#126780=CARTESIAN_POINT('Ctrl Pts',(-12.2524288688057,13.6155079184588,
132.780146867289)) ;
#126781=CARTESIAN_POINT('Ctrl Pts',(-12.25927523216,13.3048786639477,132.767097369268)) ;
#126782=CARTESIAN_POINT('Ctrl Pts',(-12.2931239866176,13.0013158611206,
132.832775546198)) ;
#126783=CARTESIAN_POINT('Ctrl Pts',(-12.3520199188583,12.7290184859203,
132.971741376215)) ;
#126784=CARTESIAN_POINT('Ctrl Pts',(-12.4326782308627,12.5059453059748,
133.174220773356)) ;
#126785=CARTESIAN_POINT('Ctrl Pts',(-12.5298337757618,12.3489356704195,
133.424945718245)) ;
#126786=CARTESIAN_POINT('Ctrl Pts',(-12.6372704596358,12.2685725679141,
133.705726448417)) ;
#126787=CARTESIAN_POINT('Ctrl Pts',(-12.7486620548609,12.2709800275436,
133.997898242284)) ;
#126788=CARTESIAN_POINT('Ctrl Pts',(-12.8556718615591,12.3558597307768,
134.27743957292)) ;
#126789=CARTESIAN_POINT('Ctrl Pts',(-12.9522002926599,12.5173148963124,
134.526272457561)) ;
#126790=CARTESIAN_POINT('Ctrl Pts',(-13.0316720868523,12.7436533200346,
134.725305724518)) ;
#126791=CARTESIAN_POINT('Ctrl Pts',(-13.0892034891378,13.018439069694,134.860265498941)) ;
#126792=CARTESIAN_POINT('Ctrl Pts',(-13.1214679873254,13.3224259013371,
134.92138844405)) ;
#126793=CARTESIAN_POINT('Ctrl Pts',(-13.1268138371495,13.6337496474671,
134.903863238124)) ;
#126794=CARTESIAN_POINT('Ctrl Pts',(-13.1055776718622,13.9298381651934,
134.808697625528)) ;
#126795=CARTESIAN_POINT('Ctrl Pts',(-13.0600986020032,14.1894306031692,
134.642744252233)) ;
#126796=CARTESIAN_POINT('Ctrl Pts',(-12.9941851716164,14.3944757405405,
134.417037926002)) ;
#126797=CARTESIAN_POINT('Ctrl Pts',(-12.913653884883,14.5294751420936,134.14873833919)) ;
#126798=CARTESIAN_POINT('Ctrl Pts',(-12.8245776745816,14.5857784683659,
133.855399066771)) ;
#126799=CARTESIAN_POINT('Ctrl Pts',(-12.7339951385361,14.5584757984426,
133.557575572516)) ;
#126800=CARTESIAN_POINT('Ctrl Pts',(-12.6496676074224,14.4499269528594,
133.278138952637)) ;
#126801=CARTESIAN_POINT('Ctrl Pts',(-12.5779591604913,14.2678362445854,
133.035534388741)) ;
#126802=CARTESIAN_POINT('Ctrl Pts',(-12.524838740077,14.0251814638135,132.847230394118)) ;
#126803=CARTESIAN_POINT('Ctrl Pts',(-12.4948320173684,13.7395989389894,
132.726468372843)) ;
#126804=CARTESIAN_POINT('Ctrl Pts',(-12.4907942560101,13.4312396305714,
132.681553632489)) ;
#126805=CARTESIAN_POINT('Ctrl Pts',(-12.5136927724239,13.122549732562,132.715357350964)) ;
#126806=CARTESIAN_POINT('Ctrl Pts',(-12.5628394820659,12.8344723669187,
132.825729771799)) ;
#126807=CARTESIAN_POINT('Ctrl Pts',(-12.6351603737995,12.5894057801397,
133.003896888117)) ;
#126808=CARTESIAN_POINT('Ctrl Pts',(-12.7263460961529,12.403866957567,133.23714956194)) ;
#126809=CARTESIAN_POINT('Ctrl Pts',(-12.8305084073274,12.2913271425025,
133.508330143151)) ;
#126810=CARTESIAN_POINT('Ctrl Pts',(-12.9412562406573,12.2598830910493,
133.79866136084)) ;
#126811=CARTESIAN_POINT('Ctrl Pts',(-13.0506666618133,12.3117248733074,
134.085220024184)) ;
#126812=CARTESIAN_POINT('Ctrl Pts',(-13.1523540896968,12.443258179484,134.349126951551)) ;
#126813=CARTESIAN_POINT('Ctrl Pts',(-13.2393089523663,12.6447768173015,
134.57005085132)) ;
#126814=CARTESIAN_POINT('Ctrl Pts',(-13.3062792253377,12.9020426575426,
134.732576392011)) ;
#126815=CARTESIAN_POINT('Ctrl Pts',(-13.3491121418991,13.1969220375029,
134.824559296309)) ;
#126816=CARTESIAN_POINT('Ctrl Pts',(-13.3654831799169,13.5073633530841,
134.839313257053)) ;
#126817=CARTESIAN_POINT('Ctrl Pts',(-13.3547961092594,13.8135027955519,
134.774821065349)) ;
#126818=CARTESIAN_POINT('Ctrl Pts',(-13.3189348221119,14.0890634485619,
134.637107361757)) ;
#126819=CARTESIAN_POINT('Ctrl Pts',(-13.2605232489219,14.3192684868255,
134.433199436081)) ;
#126820=CARTESIAN_POINT('Ctrl Pts',(-13.1854056232735,14.4835637589644,
134.18077840894)) ;
#126821=CARTESIAN_POINT('Ctrl Pts',(-13.0986713612669,14.5730188127273,
133.894189644553)) ;
#126822=CARTESIAN_POINT('Ctrl Pts',(-13.0079469277613,14.57959678794,133.596037025184)) ;
#126823=CARTESIAN_POINT('Ctrl Pts',(-12.9202452278553,14.5032854042053,
133.306694018913)) ;
#126824=CARTESIAN_POINT('Ctrl Pts',(-12.8427351822991,14.3501151902807,
133.047206914589)) ;
#126825=CARTESIAN_POINT('Ctrl Pts',(-12.7812157154848,14.1289952661381,
132.834210656053)) ;
#126826=CARTESIAN_POINT('Ctrl Pts',(-12.7416423436877,13.8600884343622,
132.685694384841)) ;
#126827=CARTESIAN_POINT('Ctrl Pts',(-12.7267166933267,13.5571076942101,
132.608832010303)) ;
#126828=CARTESIAN_POINT('Ctrl Pts',(-12.7387853224196,13.2461441401465,
132.611016636209)) ;
#126829=CARTESIAN_POINT('Ctrl Pts',(-12.7773913543468,12.9474784920459,
132.690690803401)) ;
#126830=CARTESIAN_POINT('Ctrl Pts',(-12.8410763941597,12.6818050518092,
132.843463764725)) ;
#126831=CARTESIAN_POINT('Ctrl Pts',(-12.9248214245163,12.4713262054323,
133.055159848696)) ;
#126832=CARTESIAN_POINT('Ctrl Pts',(-13.0248439197258,12.3273775325765,
133.314112791871)) ;
#126833=CARTESIAN_POINT('Ctrl Pts',(-13.1333865563481,12.2625380449618,
133.598161317782)) ;
#126834=CARTESIAN_POINT('Ctrl Pts',(-13.2448375865862,12.2810707567545,
133.890430592819)) ;
#126835=CARTESIAN_POINT('Ctrl Pts',(-13.349687874794,12.3803129183538,134.16387238493)) ;
#126836=CARTESIAN_POINT('Ctrl Pts',(-13.4438403061782,12.5556239144648,
134.405630875818)) ;
#126837=CARTESIAN_POINT('Ctrl Pts',(-13.5192481442775,12.7914917134663,
134.592929817305)) ;
#126838=CARTESIAN_POINT('Ctrl Pts',(-13.5725537048544,13.0750409894439,
134.715337082379)) ;
#126839=CARTESIAN_POINT('Ctrl Pts',(-13.5996147443617,13.3808908591526,
134.76139882389)) ;
#126840=CARTESIAN_POINT('Ctrl Pts',(-13.5999442357729,13.6908804953288,
134.729236542822)) ;
#126841=CARTESIAN_POINT('Ctrl Pts',(-13.5739291149334,13.9819858786258,
134.620089729232)) ;
#126842=CARTESIAN_POINT('Ctrl Pts',(-13.5240931007593,14.2331023151693,
134.441318559943)) ;
#126843=CARTESIAN_POINT('Ctrl Pts',(-13.4552207598495,14.4253737390559,
134.207104813219)) ;
#126844=CARTESIAN_POINT('Ctrl Pts',(-13.3719137602938,14.5469025476726,
133.930428347931)) ;
#126845=CARTESIAN_POINT('Ctrl Pts',(-13.2824137245965,14.5868798001592,
133.636000960324)) ;
#126846=CARTESIAN_POINT('Ctrl Pts',(-13.1927395264543,14.5442430115436,
133.340951538328)) ;
#126847=CARTESIAN_POINT('Ctrl Pts',(-13.1101849758616,14.4211466691175,
133.066658189192)) ;
#126848=CARTESIAN_POINT('Ctrl Pts',(-13.0414901767957,14.2262607722871,
132.832818373534)) ;
#126849=CARTESIAN_POINT('Ctrl Pts',(-12.9924622934676,13.9744157563079,
132.656514392088)) ;
#126850=CARTESIAN_POINT('Ctrl Pts',(-12.9671460162565,13.6824770169396,
132.549398601363)) ;
#126851=CARTESIAN_POINT('Ctrl Pts',(-12.9681156003432,13.3726811372132,
132.519157354883)) ;
#126852=CARTESIAN_POINT('Ctrl Pts',(-12.9963459663067,13.0644553037201,
132.568316291691)) ;
#126853=CARTESIAN_POINT('Ctrl Pts',(-13.0497942608992,12.7851437851833,
132.691521621221)) ;
#126854=CARTESIAN_POINT('Ctrl Pts',(-13.1261848175249,12.5493640401518,
132.881485944065)) ;
#126855=CARTESIAN_POINT('Ctrl Pts',(-13.2201072319773,12.3769707551736,
133.122803932911)) ;
#126856=CARTESIAN_POINT('Ctrl Pts',(-13.3264644051921,12.2789143084507,
133.400245688756)) ;
#126857=CARTESIAN_POINT('Ctrl Pts',(-13.4370417615997,12.2633331273902,
133.690248654749)) ;
#126858=CARTESIAN_POINT('Ctrl Pts',(-13.5459037408289,12.3306602572705,
133.975076437194)) ;
#126859=CARTESIAN_POINT('Ctrl Pts',(-13.6452910724307,12.476620286477,134.232259263529)) ;
#126860=CARTESIAN_POINT('Ctrl Pts',(-13.7286047765094,12.6891736358698,
134.442646796355)) ;
#126861=CARTESIAN_POINT('Ctrl Pts',(-13.791397134402,12.9552555089657,134.592923912506)) ;
#126862=CARTESIAN_POINT('Ctrl Pts',(-13.8293665170543,13.2547270236638,
134.670715591851)) ;
#126863=CARTESIAN_POINT('Ctrl Pts',(-13.840619326519,13.5662746405731,134.670455955337)) ;
#126864=CARTESIAN_POINT('Ctrl Pts',(-13.8250952024996,13.8673046435887,
134.592005354761)) ;
#126865=CARTESIAN_POINT('Ctrl Pts',(-13.7845898717327,14.1368396800883,
134.440539650573)) ;
#126866=CARTESIAN_POINT('Ctrl Pts',(-13.7227936344222,14.3550474216671,
134.226906056734)) ;
#126867=CARTESIAN_POINT('Ctrl Pts',(-13.6447577022458,14.5066809592571,
133.965799455824)) ;
#126868=CARTESIAN_POINT('Ctrl Pts',(-13.5568840038658,14.5805549920085,
133.675968281385)) ;
#126869=CARTESIAN_POINT('Ctrl Pts',(-13.466270022072,14.5715434315125,133.378164426788)) ;
#126870=CARTESIAN_POINT('Ctrl Pts',(-13.3799814831956,14.480461463905,133.09298388884)) ;
#126871=CARTESIAN_POINT('Ctrl Pts',(-13.3047665182075,14.3129344866538,
132.840042323809)) ;
#126872=CARTESIAN_POINT('Ctrl Pts',(-13.2472795095458,14.0824719984918,
132.639041871323)) ;
#126873=CARTESIAN_POINT('Ctrl Pts',(-13.2119194352514,13.8045960176135,
132.502631314994)) ;
#126874=CARTESIAN_POINT('Ctrl Pts',(-13.2020214685182,13.4994872434927,
132.440616126401)) ;
#126875=CARTESIAN_POINT('Ctrl Pts',(-13.2192111018863,13.1877258858405,
132.457597027487)) ;
#126876=CARTESIAN_POINT('Ctrl Pts',(-13.2626046011989,12.8947281848912,
132.551349374371)) ;
#126877=CARTESIAN_POINT('Ctrl Pts',(-13.3305201660103,12.6375710521211,
132.716474425557)) ;
#126878=CARTESIAN_POINT('Ctrl Pts',(-13.417753308808,12.4386468746083,132.938314812527)) ;
#126879=CARTESIAN_POINT('Ctrl Pts',(-13.5197229471736,12.3091461004709,
133.203049301303)) ;
#126880=CARTESIAN_POINT('Ctrl Pts',(-13.6293498918982,12.259612482053,133.490214186349)) ;
#126881=CARTESIAN_POINT('Ctrl Pts',(-13.7400513807603,12.2934287591009,
133.78040081702)) ;
#126882=CARTESIAN_POINT('Ctrl Pts',(-13.8440861880681,12.4085128322788,
134.051154004392)) ;
#126883=CARTESIAN_POINT('Ctrl Pts',(-13.9345816147693,12.5956557303843,
134.28246321765)) ;
#126884=CARTESIAN_POINT('Ctrl Pts',(-14.0062682849132,12.8419007256208,
134.458804814913)) ;
#126885=CARTESIAN_POINT('Ctrl Pts',(-14.0547198515339,13.1310174981793,
134.567130111826)) ;
#126886=CARTESIAN_POINT('Ctrl Pts',(-14.0768860873263,13.4394174350743,
134.598856883951)) ;
#126887=CARTESIAN_POINT('Ctrl Pts',(-14.0720541751936,13.7489280848763,
134.551459492802)) ;
#126888=CARTESIAN_POINT('Ctrl Pts',(-14.0413601954176,14.0326636274873,
134.428784425465)) ;
#126889=CARTESIAN_POINT('Ctrl Pts',(-13.9876873191308,14.2739040718616,
134.238867664221)) ;
#126890=CARTESIAN_POINT('Ctrl Pts',(-13.9153842326398,14.4542739063911,
133.994469203157)) ;
#126891=CARTESIAN_POINT('Ctrl Pts',(-13.8309760279277,14.5602989647872,
133.714872258789)) ;
#126892=CARTESIAN_POINT('Ctrl Pts',(-13.7403801033257,14.5853165165248,
133.417024159331)) ;
#126893=CARTESIAN_POINT('Ctrl Pts',(-13.65150445181,14.5269567135038,133.124299899704)) ;
#126894=CARTESIAN_POINT('Ctrl Pts',(-13.5709039203925,14.3891797896351,
132.855635428443)) ;
#126895=CARTESIAN_POINT('Ctrl Pts',(-13.5055449502742,14.1817903074031,
132.631517682888)) ;
#126896=CARTESIAN_POINT('Ctrl Pts',(-13.460908167106,13.9219442128278,132.468162749426)) ;
#126897=CARTESIAN_POINT('Ctrl Pts',(-13.4403796769414,13.6244333194243,
132.374984820522)) ;
#126898=CARTESIAN_POINT('Ctrl Pts',(-13.4464724449161,13.3138308436316,
132.359734982198)) ;
#126899=CARTESIAN_POINT('Ctrl Pts',(-13.4796936448716,13.0089907399567,
132.423492971966)) ;
#126900=CARTESIAN_POINT('Ctrl Pts',(-13.5376958216924,12.7367005360714,
132.559985324287)) ;
#126901=CARTESIAN_POINT('Ctrl Pts',(-13.6177496740489,12.5117902877451,
132.760692962081)) ;
#126902=CARTESIAN_POINT('Ctrl Pts',(-13.7145094270354,12.3525056138097,
133.010254920769)) ;
#126903=CARTESIAN_POINT('Ctrl Pts',(-13.8222036002752,12.2695603566645,
133.291647946124)) ;
#126904=CARTESIAN_POINT('Ctrl Pts',(-13.9334295911699,12.2698997440141,
133.58338643449)) ;
#126905=CARTESIAN_POINT('Ctrl Pts',(-14.0403607064271,12.352163996818,133.862787899853)) ;
#126906=CARTESIAN_POINT('Ctrl Pts',(-14.1373924563583,12.5116414977634,
134.113058580981)) ;
#126907=CARTESIAN_POINT('Ctrl Pts',(-14.2173629494588,12.7360068873482,
134.313587886391)) ;
#126908=CARTESIAN_POINT('Ctrl Pts',(-14.2756685526493,13.0100795378332,
134.450754231057)) ;
#126909=CARTESIAN_POINT('Ctrl Pts',(-14.3086572681643,13.3126252447019,
134.514091490249)) ;
#126910=CARTESIAN_POINT('Ctrl Pts',(-14.3148158817546,13.6254714681501,
134.498785238037)) ;
#126911=CARTESIAN_POINT('Ctrl Pts',(-14.2943755288969,13.921236470121,134.406066716109)) ;
#126912=CARTESIAN_POINT('Ctrl Pts',(-14.2494771644102,14.1826934134292,
134.241738201168)) ;
#126913=CARTESIAN_POINT('Ctrl Pts',(-14.1843383054734,14.3889686231296,
134.018412105004)) ;
#126914=CARTESIAN_POINT('Ctrl Pts',(-14.1036479063904,14.5271449992224,
133.749433553487)) ;
#126915=CARTESIAN_POINT('Ctrl Pts',(-14.0146176133587,14.5852339330884,
133.456206620789)) ;
#126916=CARTESIAN_POINT('Ctrl Pts',(-13.9245692886674,14.5605427750385,
133.160162631154)) ;
#126917=CARTESIAN_POINT('Ctrl Pts',(-13.8397090427971,14.4541441679249,
132.879072280579)) ;
#126918=CARTESIAN_POINT('Ctrl Pts',(-13.7675999424785,14.2740963431477,
132.635321969107)) ;
#126919=CARTESIAN_POINT('Ctrl Pts',(-13.7137337312793,14.0323113034301,
132.444751360353)) ;
#126920=CARTESIAN_POINT('Ctrl Pts',(-13.6831298810078,13.7476340175603,
132.322252805189)) ;
#126921=CARTESIAN_POINT('Ctrl Pts',(-13.6782879805551,13.4408490970619,
132.275120776001)) ;
#126922=CARTESIAN_POINT('Ctrl Pts',(-13.7005416589842,13.1304291613817,
132.306881371971)) ;
#126923=CARTESIAN_POINT('Ctrl Pts',(-13.7487855845768,12.8426172804035,
132.414756826716)) ;
#126924=CARTESIAN_POINT('Ctrl Pts',(-13.8208039684073,12.5951022421241,
132.591898091082)) ;
#126925=CARTESIAN_POINT('Ctrl Pts',(-13.9110777354065,12.4086451366849,
132.822659096915)) ;
#126926=CARTESIAN_POINT('Ctrl Pts',(-14.0152201075138,12.2933533540089,
133.093685240975)) ;
#126927=CARTESIAN_POINT('Ctrl Pts',(-14.1258578816827,12.259635664544,133.383708871411)) ;
#126928=CARTESIAN_POINT('Ctrl Pts',(-14.2353399031304,12.3091205538474,
133.670488901547)) ;
#126929=CARTESIAN_POINT('Ctrl Pts',(-14.3371725585979,12.4379929301553,
133.934891434385)) ;
#126930=CARTESIAN_POINT('Ctrl Pts',(-14.4250620411893,12.6386444970783,
134.158382491319)) ;
#126931=CARTESIAN_POINT('Ctrl Pts',(-14.4924635887895,12.8942394959608,
134.322231369689)) ;
#126932=CARTESIAN_POINT('Ctrl Pts',(-14.5359913992517,13.1876523538433,
134.416314155428)) ;
#126933=CARTESIAN_POINT('Ctrl Pts',(-14.5531646384012,13.4984174777635,
134.433357576276)) ;
#126934=CARTESIAN_POINT('Ctrl Pts',(-14.5433292922397,13.804322914882,134.371440213958)) ;
#126935=CARTESIAN_POINT('Ctrl Pts',(-14.5079547278182,14.0825044071424,
134.234961968097)) ;
#126936=CARTESIAN_POINT('Ctrl Pts',(-14.4502363015794,14.3134151405244,
134.033186347547)) ;
#126937=CARTESIAN_POINT('Ctrl Pts',(-14.3755312606289,14.4799820056889,
133.781954581635)) ;
#126938=CARTESIAN_POINT('Ctrl Pts',(-14.2886874107007,14.5717628953294,
133.4949287269)) ;
#126939=CARTESIAN_POINT('Ctrl Pts',(-14.1984355671894,14.5804902446719,
133.198322327595)) ;
#126940=CARTESIAN_POINT('Ctrl Pts',(-14.1105879218463,14.5068426391239,
132.908575316213)) ;
#126941=CARTESIAN_POINT('Ctrl Pts',(-14.0326036147844,14.3556215775595,
132.647664192124)) ;
#126942=CARTESIAN_POINT('Ctrl Pts',(-13.9705602133679,14.1365916181852,
132.433178184827)) ;
#126943=CARTESIAN_POINT('Ctrl Pts',(-13.9302307321672,13.8680780332019,
132.282355246629)) ;
#126944=CARTESIAN_POINT('Ctrl Pts',(-13.9145452425664,13.5671869080058,
132.2034355718)) ;
#126945=CARTESIAN_POINT('Ctrl Pts',(-13.9259229339394,13.2537546109161,
132.20333913892)) ;
#126946=CARTESIAN_POINT('Ctrl Pts',(-13.9637000582678,12.9561225351469,
132.280771186731)) ;
#126947=CARTESIAN_POINT('Ctrl Pts',(-14.0264505290295,12.6895770541959,
132.430888192073)) ;
#126948=CARTESIAN_POINT('Ctrl Pts',(-14.1099152437945,12.4765149005577,
132.641654318194)) ;
#126949=CARTESIAN_POINT('Ctrl Pts',(-14.2096080891455,12.3303993150384,
132.899637545338)) ;
#126950=CARTESIAN_POINT('Ctrl Pts',(-14.3180690093773,12.2633426661684,
133.183421114825)) ;
#126951=CARTESIAN_POINT('Ctrl Pts',(-14.4289810692293,12.2791039677748,
133.474293945749)) ;
#126952=CARTESIAN_POINT('Ctrl Pts',(-14.5347689827399,12.3764767274057,
133.750263662714)) ;
#126953=CARTESIAN_POINT('Ctrl Pts',(-14.6292816067322,12.5500288715812,
133.993084325586)) ;
#126954=CARTESIAN_POINT('Ctrl Pts',(-14.7051205759119,12.78395781333,134.181698039827)) ;
#126955=CARTESIAN_POINT('Ctrl Pts',(-14.7590884771075,13.0658040836913,
134.306109130981)) ;
#126956=CARTESIAN_POINT('Ctrl Pts',(-14.7870570873247,13.3726170327576,
134.354673270728)) ;
#126957=CARTESIAN_POINT('Ctrl Pts',(-14.7880362308985,13.6826397298667,
134.324425071455)) ;
#126958=CARTESIAN_POINT('Ctrl Pts',(-14.7629011385649,13.9734160140871,
134.217988273275)) ;
#126959=CARTESIAN_POINT('Ctrl Pts',(-14.7135553917032,14.2269288316592,
134.040531948829)) ;
#126960=CARTESIAN_POINT('Ctrl Pts',(-14.6452446553135,14.4205112254327,
133.808019823246)) ;
#126961=CARTESIAN_POINT('Ctrl Pts',(-14.5627005184461,14.5441065975964,
133.533729916496)) ;
#126962=CARTESIAN_POINT('Ctrl Pts',(-14.4726632379768,14.5870792666042,
133.237494403746)) ;
#126963=CARTESIAN_POINT('Ctrl Pts',(-14.3827907850209,14.5462510454972,
132.941823015601)) ;
#126964=CARTESIAN_POINT('Ctrl Pts',(-14.3003438724804,14.4261089753038,
132.668016533417)) ;
#126965=CARTESIAN_POINT('Ctrl Pts',(-14.2307721367749,14.2320089308133,
132.431424344221)) ;
#126966=CARTESIAN_POINT('Ctrl Pts',(-14.1813514089669,13.9821034957132,
132.254072397116)) ;
#126967=CARTESIAN_POINT('Ctrl Pts',(-14.155314709505,13.6914861079863,132.144897171417)) ;
#126968=CARTESIAN_POINT('Ctrl Pts',(-14.1554757838754,13.3820427102498,
132.112307580713)) ;
#126969=CARTESIAN_POINT('Ctrl Pts',(-14.1829242521949,13.0731824784138,
132.159161065755)) ;
#126970=CARTESIAN_POINT('Ctrl Pts',(-14.2356771557397,12.7927891532511,
132.280328855648)) ;
#126971=CARTESIAN_POINT('Ctrl Pts',(-14.3114802654347,12.555308710761,132.468568512814)) ;
#126972=CARTESIAN_POINT('Ctrl Pts',(-14.405137795849,12.3807971567645,132.709061171522)) ;
#126973=CARTESIAN_POINT('Ctrl Pts',(-14.5108510096583,12.2807361442519,
132.984745301486)) ;
#126974=CARTESIAN_POINT('Ctrl Pts',(-14.6217350370507,12.2625961499198,
133.275536642157)) ;
#126975=CARTESIAN_POINT('Ctrl Pts',(-14.7305884334379,12.3275534579407,
133.560394240551)) ;
#126976=CARTESIAN_POINT('Ctrl Pts',(-14.8303351103071,12.4713199935408,
133.818625118749)) ;
#126977=CARTESIAN_POINT('Ctrl Pts',(-14.9142095075345,12.6818353825156,
134.030669934059)) ;
#126978=CARTESIAN_POINT('Ctrl Pts',(-14.9780252508446,12.9488695805188,
134.183682231059)) ;
#126979=CARTESIAN_POINT('Ctrl Pts',(-15.0163167509657,13.2449964341876,
134.2627235007)) ;
#126980=CARTESIAN_POINT('Ctrl Pts',(-15.0284923230541,13.5577146897345,
134.265023837386)) ;
#126981=CARTESIAN_POINT('Ctrl Pts',(-15.0136674302917,13.8591379588549,
134.188639506214)) ;
#126982=CARTESIAN_POINT('Ctrl Pts',(-14.9737786696409,14.1301669170847,
134.038933696206)) ;
#126983=CARTESIAN_POINT('Ctrl Pts',(-14.9125163633659,14.3498259232659,
133.826877916861)) ;
#126984=CARTESIAN_POINT('Ctrl Pts',(-14.8349895204821,14.5033075535996,
133.567312008067)) ;
#126985=CARTESIAN_POINT('Ctrl Pts',(-14.7472616829707,14.5795880895815,
133.277889078353)) ;
#126986=CARTESIAN_POINT('Ctrl Pts',(-14.6565928445212,14.5729975204269,
132.979913996434)) ;
#126987=CARTESIAN_POINT('Ctrl Pts',(-14.5698387137469,14.4837968438998,
132.693276319562)) ;
#126988=CARTESIAN_POINT('Ctrl Pts',(-14.4943500116682,14.3181445860539,
132.439567110174)) ;
#126989=CARTESIAN_POINT('Ctrl Pts',(-14.4364625855008,14.0900336842333,
132.237499897993)) ;
#126990=CARTESIAN_POINT('Ctrl Pts',(-14.4003322523361,13.8125787469842,
132.098759396213)) ;
#126991=CARTESIAN_POINT('Ctrl Pts',(-14.3897456286772,13.5087143541534,
132.034817758566)) ;
#126992=CARTESIAN_POINT('Ctrl Pts',(-14.4060516377967,13.1970642256003,
132.049247933405)) ;
#126993=CARTESIAN_POINT('Ctrl Pts',(-14.4488719696154,12.9023258693894,
132.141215716512)) ;
#126994=CARTESIAN_POINT('Ctrl Pts',(-14.5159375651983,12.6446851573858,
132.303967806051)) ;
#126995=CARTESIAN_POINT('Ctrl Pts',(-14.6026582838117,12.4436426796563,
132.524294973263)) ;
#126996=CARTESIAN_POINT('Ctrl Pts',(-14.704427237355,12.3118006099846,132.788401667145)) ;
#126997=CARTESIAN_POINT('Ctrl Pts',(-14.8139557089677,12.259762671147,133.075273126533)) ;
#126998=CARTESIAN_POINT('Ctrl Pts',(-14.9251382688252,12.2917039149137,
133.366735111266)) ;
#126999=CARTESIAN_POINT('Ctrl Pts',(-15.0286487061425,12.4035190243102,
133.636225798027)) ;
#127000=CARTESIAN_POINT('Ctrl Pts',(-15.1203793223657,12.5902948826821,
133.870856294404)) ;
#127001=CARTESIAN_POINT('Ctrl Pts',(-15.1921924551787,12.8337324578526,
134.047773898269)) ;
#127002=CARTESIAN_POINT('Ctrl Pts',(-15.2416538483721,13.1235886478701,
134.158851739517)) ;
#127003=CARTESIAN_POINT('Ctrl Pts',(-15.2643296293558,13.4302519439914,
134.192228539478)) ;
#127004=CARTESIAN_POINT('Ctrl Pts',(-15.2604682402602,13.7390104771059,
134.147792840823)) ;
#127005=CARTESIAN_POINT('Ctrl Pts',(-15.2302304828528,14.0260062251914,
134.026182196942)) ;
#127006=CARTESIAN_POINT('Ctrl Pts',(-15.1773828700923,14.267226894927,133.83886254729)) ;
#127007=CARTESIAN_POINT('Ctrl Pts',(-15.1056430753497,14.4498458863908,
133.596118183399)) ;
#127008=CARTESIAN_POINT('Ctrl Pts',(-15.021088548327,14.5586319287784,133.315937393289)) ;
#127009=CARTESIAN_POINT('Ctrl Pts',(-14.9305285876603,14.5856242099091,
133.018186098394)) ;
#127010=CARTESIAN_POINT('Ctrl Pts',(-14.8418950205614,14.5299078303726,
132.726313987162)) ;
#127011=CARTESIAN_POINT('Ctrl Pts',(-14.7607450760407,14.3940107888909,
132.455958932693)) ;
#127012=CARTESIAN_POINT('Ctrl Pts',(-14.6950115091372,14.1888420918384,
132.230820509577)) ;
#127013=CARTESIAN_POINT('Ctrl Pts',(-14.6496592401671,13.9299824930108,
132.065327212489)) ;
#127014=CARTESIAN_POINT('Ctrl Pts',(-14.6284006795938,13.6339609144374,
131.970100332748)) ;
#127015=CARTESIAN_POINT('Ctrl Pts',(-14.6337188432872,13.3227159368467,
131.952503879531)) ;
#127016=CARTESIAN_POINT('Ctrl Pts',(-14.6659818143214,13.0187244434426,
132.013618672665)) ;
#127017=CARTESIAN_POINT('Ctrl Pts',(-14.7233385330698,12.7442184480219,
132.148123450518)) ;
#127018=CARTESIAN_POINT('Ctrl Pts',(-14.8032873271645,12.516718909921,132.348361947156)) ;
#127019=CARTESIAN_POINT('Ctrl Pts',(-14.8992236867721,12.3563386228632,
132.595676015683)) ;
#127020=CARTESIAN_POINT('Ctrl Pts',(-15.00647311092,12.2709228353889,132.875831085534)) ;
#127021=CARTESIAN_POINT('Ctrl Pts',(-15.1178233288828,12.2686101077704,
133.167894840655)) ;
#127022=CARTESIAN_POINT('Ctrl Pts',(-15.2252101895966,12.3485946341444,
133.44855717488)) ;
#127023=CARTESIAN_POINT('Ctrl Pts',(-15.3229248735586,12.5068356453483,
133.70070522754)) ;
#127024=CARTESIAN_POINT('Ctrl Pts',(-15.4029565974295,12.728330138996,133.901605268035)) ;
#127025=CARTESIAN_POINT('Ctrl Pts',(-15.4621017130809,13.0013550169445,
134.041190190912)) ;
#127026=CARTESIAN_POINT('Ctrl Pts',(-15.4958591875495,13.303953158046,134.106709837516)) ;
#127027=CARTESIAN_POINT('Ctrl Pts',(-15.5028362362812,13.6158508355622,
134.093908778801)) ;
#127028=CARTESIAN_POINT('Ctrl Pts',(-15.4830234200552,13.9138455338492,
134.002849682409)) ;
#127029=CARTESIAN_POINT('Ctrl Pts',(-15.4389659228457,14.1752852419692,
133.841141599243)) ;
#127030=CARTESIAN_POINT('Ctrl Pts',(-15.3742548041053,14.3839668801463,
133.618990077083)) ;
#127031=CARTESIAN_POINT('Ctrl Pts',(-15.2939923725203,14.5240578429112,
133.351300381935)) ;
#127032=CARTESIAN_POINT('Ctrl Pts',(-15.2051966892418,14.584818932524,133.058785675523)) ;
#127033=CARTESIAN_POINT('Ctrl Pts',(-15.1144952079084,14.5621167369362,
132.760611447614)) ;
#127034=CARTESIAN_POINT('Ctrl Pts',(-15.0299271948312,14.4583966415937,
132.480583857298)) ;
#127035=CARTESIAN_POINT('Ctrl Pts',(-14.9572763457915,14.2803903963779,
132.235223701312)) ;
#127036=CARTESIAN_POINT('Ctrl Pts',(-14.9029121430072,14.0406559571458,
132.043265678617)) ;
#127037=CARTESIAN_POINT('Ctrl Pts',(-14.8714358369862,13.7571590252373,
131.918221498036)) ;
#127038=CARTESIAN_POINT('Ctrl Pts',(-14.8659049731751,13.4483332658606,
131.868817727218)) ;
#127039=CARTESIAN_POINT('Ctrl Pts',(-14.8871485835861,13.1406103959238,
131.897955203955)) ;
#127040=CARTESIAN_POINT('Ctrl Pts',(-14.9350650117889,12.849237718573,132.004565980115)) ;
#127041=CARTESIAN_POINT('Ctrl Pts',(-15.0060654331534,12.6021186040621,
132.178962627107)) ;
#127042=CARTESIAN_POINT('Ctrl Pts',(-15.0959333972116,12.4130744428075,
132.408478228169)) ;
#127043=CARTESIAN_POINT('Ctrl Pts',(-15.2001942594425,12.295357536539,132.6797330253)) ;
#127044=CARTESIAN_POINT('Ctrl Pts',(-15.3102776881432,12.2595400049776,
132.968276410172)) ;
#127045=CARTESIAN_POINT('Ctrl Pts',(-15.4199784955262,12.3063152833776,
133.255674356506)) ;
#127046=CARTESIAN_POINT('Ctrl Pts',(-15.522699193365,12.4341408238282,133.522468160323)) ;
#127047=CARTESIAN_POINT('Ctrl Pts',(-15.6103829822627,12.6316134700122,
133.745609070741)) ;
#127048=CARTESIAN_POINT('Ctrl Pts',(-15.6786358897342,12.8861350192124,
133.911877716703)) ;
#127049=CARTESIAN_POINT('Ctrl Pts',(-15.7229388254079,13.1792139028364,
134.008179554018)) ;
#127050=CARTESIAN_POINT('Ctrl Pts',(-15.7408625348171,13.490568739432,134.027334806477)) ;
#127051=CARTESIAN_POINT('Ctrl Pts',(-15.7316840369272,13.7964603979055,
133.96738117624)) ;
#127052=CARTESIAN_POINT('Ctrl Pts',(-15.6971658649045,14.0743848180785,
133.833556786715)) ;
#127053=CARTESIAN_POINT('Ctrl Pts',(-15.640209575695,14.3070162611111,133.634045700277)) ;
#127054=CARTESIAN_POINT('Ctrl Pts',(-15.5654530352524,14.476451846962,133.382463536536)) ;
#127055=CARTESIAN_POINT('Ctrl Pts',(-15.4796013706087,14.569850177848,133.098627967463)) ;
#127056=CARTESIAN_POINT('Ctrl Pts',(-15.3889094017471,14.5816111241078,
132.800558625303)) ;
#127057=CARTESIAN_POINT('Ctrl Pts',(-15.300616199253,14.5098991717079,132.50941294368)) ;
#127058=CARTESIAN_POINT('Ctrl Pts',(-15.2222312224412,14.360403037698,132.247300438646)) ;
#127059=CARTESIAN_POINT('Ctrl Pts',(-15.1598553959439,14.143565690272,132.031931962309)) ;
#127060=CARTESIAN_POINT('Ctrl Pts',(-15.1187843239202,13.8762646142661,
131.878935402952)) ;
#127061=CARTESIAN_POINT('Ctrl Pts',(-15.1024542909266,13.5746434283165,
131.79799241285)) ;
#127062=CARTESIAN_POINT('Ctrl Pts',(-15.1128551398615,13.2647986868619,
131.795431588597)) ;
#127063=CARTESIAN_POINT('Ctrl Pts',(-15.1500740102669,12.9638356585252,
131.870941727578)) ;
#127064=CARTESIAN_POINT('Ctrl Pts',(-15.2120844356372,12.696740713892,132.018978212453)) ;
#127065=CARTESIAN_POINT('Ctrl Pts',(-15.2951868761685,12.4815167402667,
132.228612079136)) ;
#127066=CARTESIAN_POINT('Ctrl Pts',(-15.3941529108664,12.3337893595149,
132.484595432364)) ;
#127067=CARTESIAN_POINT('Ctrl Pts',(-15.5026973347409,12.2640797923872,
132.768538743853)) ;
#127068=CARTESIAN_POINT('Ctrl Pts',(-15.6135110810389,12.2774691483239,
133.059167262527)) ;
#127069=CARTESIAN_POINT('Ctrl Pts',(-15.7195456012451,12.3724670418659,
133.335855362595)) ;
#127070=CARTESIAN_POINT('Ctrl Pts',(-15.8144572008724,12.543767432119,133.579865193293)) ;
#127071=CARTESIAN_POINT('Ctrl Pts',(-15.8910215330709,12.7765746874498,
133.770532042184)) ;
#127072=CARTESIAN_POINT('Ctrl Pts',(-15.9455551191463,13.056442699504,133.896702931996)) ;
#127073=CARTESIAN_POINT('Ctrl Pts',(-15.9743804491519,13.3632374383365,
133.947714740299)) ;
#127074=CARTESIAN_POINT('Ctrl Pts',(-15.9762566494674,13.6730055112077,
133.920150028813)) ;
#127075=CARTESIAN_POINT('Ctrl Pts',(-15.9515216477166,13.9671153301203,
133.81457598732)) ;
#127076=CARTESIAN_POINT('Ctrl Pts',(-15.9033160121956,14.2192391105439,
133.640818547145)) ;
#127077=CARTESIAN_POINT('Ctrl Pts',(-15.835026362201,14.4164802327196,133.408099916759)) ;
#127078=CARTESIAN_POINT('Ctrl Pts',(-15.7529435024503,14.5415580388922,
133.135249670794)) ;
#127079=CARTESIAN_POINT('Ctrl Pts',(-15.6633179777156,14.5869148382087,
132.840315322194)) ;
#127080=CARTESIAN_POINT('Ctrl Pts',(-15.5733831628916,14.5490099529441,
132.544490917924)) ;
#127081=CARTESIAN_POINT('Ctrl Pts',(-15.490058780783,14.4299835692337,132.267872421387)) ;
#127082=CARTESIAN_POINT('Ctrl Pts',(-15.4206307225619,14.2395160261302,
132.032004599489)) ;
#127083=CARTESIAN_POINT('Ctrl Pts',(-15.3702268503173,13.9900850961344,
131.851611615681)) ;
#127084=CARTESIAN_POINT('Ctrl Pts',(-15.3434852338531,13.7002631156838,
131.740380824323)) ;
#127085=CARTESIAN_POINT('Ctrl Pts',(-15.34291772876,13.3906063492619,131.705608770205)) ;
#127086=CARTESIAN_POINT('Ctrl Pts',(-15.3694315743629,13.0826197535591,
131.749876872948)) ;
#127087=CARTESIAN_POINT('Ctrl Pts',(-15.4217316411397,12.7997481172877,
131.869548993111)) ;
#127088=CARTESIAN_POINT('Ctrl Pts',(-15.4967708608653,12.5614902971475,
132.05565395496)) ;
#127089=CARTESIAN_POINT('Ctrl Pts',(-15.5901217372407,12.3846250273346,
132.295195219659)) ;
#127090=CARTESIAN_POINT('Ctrl Pts',(-15.695629337142,12.2824687909252,132.570272051232)) ;
#127091=CARTESIAN_POINT('Ctrl Pts',(-15.8061596908325,12.2619556332192,
132.860120338079)) ;
#127092=CARTESIAN_POINT('Ctrl Pts',(-15.9152791218839,12.3244285143439,
133.145725763157)) ;
#127093=CARTESIAN_POINT('Ctrl Pts',(-16.0156184574548,12.4664340119557,
133.405611588913)) ;
#127094=CARTESIAN_POINT('Ctrl Pts',(-16.0998938298251,12.675348720281,133.618840063751)) ;
#127095=CARTESIAN_POINT('Ctrl Pts',(-16.1640285350581,12.9390314346698,
133.773020248114)) ;
#127096=CARTESIAN_POINT('Ctrl Pts',(-16.2034911895346,13.2369183007794,
133.85520053705)) ;
#127097=CARTESIAN_POINT('Ctrl Pts',(-16.2162744763826,13.549774387286,133.859260960991)) ;
#127098=CARTESIAN_POINT('Ctrl Pts',(-16.2022423520224,13.850609448165,133.785316886062)) ;
#127099=CARTESIAN_POINT('Ctrl Pts',(-16.1630477314313,14.1229209827014,
133.637631054172)) ;
#127100=CARTESIAN_POINT('Ctrl Pts',(-16.1024279258205,14.3440340746158,
133.42749370549)) ;
#127101=CARTESIAN_POINT('Ctrl Pts',(-16.0251958195372,14.5000650496519,
133.168737022986)) ;
#127102=CARTESIAN_POINT('Ctrl Pts',(-15.9372506091348,14.578644462167,132.878532422709)) ;
#127103=CARTESIAN_POINT('Ctrl Pts',(-15.8471380330024,14.5743811633841,
132.582393935937)) ;
#127104=CARTESIAN_POINT('Ctrl Pts',(-15.7598975395241,14.4873598726622,
132.29423150623)) ;
#127105=CARTESIAN_POINT('Ctrl Pts',(-15.6841714035355,14.3240886770746,
132.039909083496)) ;
#127106=CARTESIAN_POINT('Ctrl Pts',(-15.625630709951,14.0972553014586,131.835876518833)) ;
#127107=CARTESIAN_POINT('Ctrl Pts',(-15.5888545861176,13.8219067372358,
131.695361474815)) ;
#127108=CARTESIAN_POINT('Ctrl Pts',(-15.5774343178227,13.5160256526642,
131.628709192123)) ;
#127109=CARTESIAN_POINT('Ctrl Pts',(-15.5931141548672,13.2050737641674,
131.6413999151)) ;
#127110=CARTESIAN_POINT('Ctrl Pts',(-15.6350536186872,12.9106474096039,
131.73090798225)) ;
#127111=CARTESIAN_POINT('Ctrl Pts',(-15.7013184155062,12.6518068441283,
131.891363677284)) ;
#127112=CARTESIAN_POINT('Ctrl Pts',(-15.7879054566775,12.4481718520534,
132.111160447903)) ;
#127113=CARTESIAN_POINT('Ctrl Pts',(-15.8891804504899,12.3143466124611,
132.373885643705)) ;
#127114=CARTESIAN_POINT('Ctrl Pts',(-15.9991528091625,12.2602411287431,
132.661877127695)) ;
#127115=CARTESIAN_POINT('Ctrl Pts',(-16.1088758468445,12.289044216294,132.949549239462)) ;
#127116=CARTESIAN_POINT('Ctrl Pts',(-16.2139161399805,12.3996399053781,
133.223107982342)) ;
#127117=CARTESIAN_POINT('Ctrl Pts',(-16.3052990396997,12.5827969083002,
133.457035289673)) ;
#127118=CARTESIAN_POINT('Ctrl Pts',(-16.3784225593528,12.826962989628,133.637457202955)) ;
#127119=CARTESIAN_POINT('Ctrl Pts',(-16.4280832723587,13.1127056207623,
133.749492183983)) ;
#127120=CARTESIAN_POINT('Ctrl Pts',(-16.4519120641996,13.421711878802,133.785935789456)) ;
#127121=CARTESIAN_POINT('Ctrl Pts',(-16.4487067222851,13.7304251120726,
133.743459367552)) ;
#127122=CARTESIAN_POINT('Ctrl Pts',(-16.4192362436366,14.018344311728,133.624095788386)) ;
#127123=CARTESIAN_POINT('Ctrl Pts',(-16.3668470537399,14.2615012017521,
133.438046957195)) ;
#127124=CARTESIAN_POINT('Ctrl Pts',(-16.2956609167277,14.4455241651706,
133.196981670041)) ;
#127125=CARTESIAN_POINT('Ctrl Pts',(-16.2116523432265,14.5564730529287,
132.918492749156)) ;
#127126=CARTESIAN_POINT('Ctrl Pts',(-16.1208373176366,14.58603325722,132.619873861017)) ;
#127127=CARTESIAN_POINT('Ctrl Pts',(-16.0322331447019,14.5327319880778,
132.328153351535)) ;
#127128=CARTESIAN_POINT('Ctrl Pts',(-15.9506596892589,14.3988255152791,
132.056517691132)) ;
#127129=CARTESIAN_POINT('Ctrl Pts',(-15.8846965931716,14.1966329622431,
131.830874369559)) ;
#127130=CARTESIAN_POINT('Ctrl Pts',(-15.8383960091304,13.9381994545952,
131.662466237002)) ;
#127131=CARTESIAN_POINT('Ctrl Pts',(-15.8164206296693,13.6421507642692,
131.565070286919)) ;
#127132=CARTESIAN_POINT('Ctrl Pts',(-15.8209925100705,13.3319747880892,
131.545390307733)) ;
#127133=CARTESIAN_POINT('Ctrl Pts',(-15.8523510548153,13.0275241495644,
131.603884248757)) ;
#127134=CARTESIAN_POINT('Ctrl Pts',(-15.90959227723,12.7499513139427,131.737788844149)) ;
#127135=CARTESIAN_POINT('Ctrl Pts',(-15.9882747688464,12.5230805952481,
131.934644253153)) ;
#127136=CARTESIAN_POINT('Ctrl Pts',(-16.0842519007302,12.3595163479197,
132.181899906692)) ;
#127137=CARTESIAN_POINT('Ctrl Pts',(-16.1915571107785,12.2720601072795,
132.462152269854)) ;
#127138=CARTESIAN_POINT('Ctrl Pts',(-16.3026683400584,12.2676665398888,
132.753584917152)) ;
#127139=CARTESIAN_POINT('Ctrl Pts',(-16.4098725171092,12.3451448289758,
133.033825189078)) ;
#127140=CARTESIAN_POINT('Ctrl Pts',(-16.5077398618101,12.5004782540512,
133.286522113672)) ;
#127141=CARTESIAN_POINT('Ctrl Pts',(-16.5887803868399,12.7212077587515,
133.490207402048)) ;
#127142=CARTESIAN_POINT('Ctrl Pts',(-16.6486155618414,12.9936145319541,
133.631759184654)) ;
#127143=CARTESIAN_POINT('Ctrl Pts',(-16.6830064614964,13.2947837203187,
133.699223914889)) ;
#127144=CARTESIAN_POINT('Ctrl Pts',(-16.690802067885,13.6064068032795,133.688848453476)) ;
#127145=CARTESIAN_POINT('Ctrl Pts',(-16.6718235868781,13.9050217412781,
133.600245728763)) ;
#127146=CARTESIAN_POINT('Ctrl Pts',(-16.6283034085852,14.1686336677941,
133.440001693097)) ;
#127147=CARTESIAN_POINT('Ctrl Pts',(-16.5641212588145,14.3788182698461,
133.219417424364)) ;
#127148=CARTESIAN_POINT('Ctrl Pts',(-16.4844394280471,14.5208662743525,
132.953507778483)) ;
#127149=CARTESIAN_POINT('Ctrl Pts',(-16.3956858711808,14.5841619964858,
132.661068294954)) ;
#127150=CARTESIAN_POINT('Ctrl Pts',(-16.3052261807868,14.5641966212731,
132.363712807229)) ;
#127151=CARTESIAN_POINT('Ctrl Pts',(-16.219987051645,14.4625802031817,132.081576128943)) ;
#127152=CARTESIAN_POINT('Ctrl Pts',(-16.1468023432749,14.286005519678,131.834596099158)) ;
#127153=CARTESIAN_POINT('Ctrl Pts',(-16.092019731511,14.0484511766116,131.641509779847)) ;
#127154=CARTESIAN_POINT('Ctrl Pts',(-16.0598137195397,13.7663469641466,
131.514368112264)) ;
#127155=CARTESIAN_POINT('Ctrl Pts',(-16.0534392828027,13.4574607862846,
131.462452093776)) ;
#127156=CARTESIAN_POINT('Ctrl Pts',(-16.0740291175869,13.1488899343714,
131.489611237961)) ;
#127157=CARTESIAN_POINT('Ctrl Pts',(-16.1208827636923,12.8583365038161,
131.593319429838)) ;
#127158=CARTESIAN_POINT('Ctrl Pts',(-16.1914348318743,12.6085157642258,
131.76627300472)) ;
#127159=CARTESIAN_POINT('Ctrl Pts',(-16.2810750702995,12.417394689709,131.995054740562)) ;
#127160=CARTESIAN_POINT('Ctrl Pts',(-16.3844471754088,12.2980452519264,
132.26389707157)) ;
#127161=CARTESIAN_POINT('Ctrl Pts',(-16.4945287592018,12.2592457780577,
132.55240289533)) ;
#127162=CARTESIAN_POINT('Ctrl Pts',(-16.6048630643841,12.304020860261,132.841492151583)) ;
#127163=CARTESIAN_POINT('Ctrl Pts',(-16.7071948575937,12.4286939335528,
133.107381215331)) ;
#127164=CARTESIAN_POINT('Ctrl Pts',(-16.7957370903251,12.6243589997422,
133.332939325687)) ;
#127165=CARTESIAN_POINT('Ctrl Pts',(-16.8649375159105,12.878908332841,133.501806658507)) ;
#127166=CARTESIAN_POINT('Ctrl Pts',(-16.9097459869717,13.1702261034011,
133.599699878422)) ;
#127167=CARTESIAN_POINT('Ctrl Pts',(-16.9284921865684,13.4805036941569,
133.621345959822)) ;
#127168=CARTESIAN_POINT('Ctrl Pts',(-16.9201734499076,13.7876511360062,
133.563828434265)) ;
#127169=CARTESIAN_POINT('Ctrl Pts',(-16.8861064009168,14.0678452510403,
133.431162542818)) ;
#127170=CARTESIAN_POINT('Ctrl Pts',(-16.8299943231887,14.3007432572347,
133.234293389989)) ;
#127171=CARTESIAN_POINT('Ctrl Pts',(-16.7556211261533,14.4725786347777,
132.983790036611)) ;
#127172=CARTESIAN_POINT('Ctrl Pts',(-16.669994129504,14.5682598851549,132.70061076845)) ;
#127173=CARTESIAN_POINT('Ctrl Pts',(-16.5793502317154,14.5824152929646,
132.402683855424)) ;
#127174=CARTESIAN_POINT('Ctrl Pts',(-16.4910139643223,14.5133614701989,
132.111471857863)) ;
#127175=CARTESIAN_POINT('Ctrl Pts',(-16.412111492588,14.3656855427812,131.847778677913)) ;
#127176=CARTESIAN_POINT('Ctrl Pts',(-16.3494282335617,14.1519223371762,
131.631683900769)) ;
#127177=CARTESIAN_POINT('Ctrl Pts',(-16.3073386916834,13.8839965789022,
131.475465893538)) ;
#127178=CARTESIAN_POINT('Ctrl Pts',(-16.2903594127806,13.5839686018203,
131.392743081148)) ;
#127179=CARTESIAN_POINT('Ctrl Pts',(-16.2999735659199,13.2736211027787,
131.387823786026)) ;
#127180=CARTESIAN_POINT('Ctrl Pts',(-16.3363145444872,12.9727616409807,
131.460858307833)) ;
#127181=CARTESIAN_POINT('Ctrl Pts',(-16.3978412897984,12.7034620887289,
131.607364231269)) ;
#127182=CARTESIAN_POINT('Ctrl Pts',(-16.4803836389756,12.4867212109574,
131.815385050795)) ;
#127183=CARTESIAN_POINT('Ctrl Pts',(-16.5790813271514,12.3368637166341,
132.070553250121)) ;
#127184=CARTESIAN_POINT('Ctrl Pts',(-16.6870891237373,12.265034692949,132.353038736455)) ;
#127185=CARTESIAN_POINT('Ctrl Pts',(-16.7982204585899,12.2758062586622,
132.644511544384)) ;
#127186=CARTESIAN_POINT('Ctrl Pts',(-16.9048720041156,12.3692807185403,
132.922870416557)) ;
#127187=CARTESIAN_POINT('Ctrl Pts',(-16.9996989007579,12.5378929203228,
133.166798907436)) ;
#127188=CARTESIAN_POINT('Ctrl Pts',(-17.0769917000868,12.7694277251572,
133.359536671956)) ;
#127189=CARTESIAN_POINT('Ctrl Pts',(-17.1322129697081,13.0484835802669,
133.487698121072)) ;
#127190=CARTESIAN_POINT('Ctrl Pts',(-17.1617637643126,13.3553251834758,
133.540779957413)) ;
#127191=CARTESIAN_POINT('Ctrl Pts',(-17.1643098885835,13.664055596243,133.515297231606)) ;
#127192=CARTESIAN_POINT('Ctrl Pts',(-17.1405674412535,13.9577070332473,
133.412784627053)) ;
#127193=CARTESIAN_POINT('Ctrl Pts',(-17.0927873539426,14.2128779767414,
133.240075341441)) ;
#127194=CARTESIAN_POINT('Ctrl Pts',(-17.0249647373013,14.4117544181439,
133.008731542962)) ;
#127195=CARTESIAN_POINT('Ctrl Pts',(-16.9432494624858,14.539128300591,132.736968714715)) ;
#127196=CARTESIAN_POINT('Ctrl Pts',(-16.8533260812375,14.5867879384206,
132.441014798324)) ;
#127197=CARTESIAN_POINT('Ctrl Pts',(-16.7637336532915,14.5512051552351,
132.146348760003)) ;
#127198=CARTESIAN_POINT('Ctrl Pts',(-16.6799727913344,14.4343419878625,
131.868402100681)) ;
#127199=CARTESIAN_POINT('Ctrl Pts',(-16.6100992323604,14.2455278913779,
131.631224317555)) ;
#127200=CARTESIAN_POINT('Ctrl Pts',(-16.5591861668346,13.9981929136205,
131.449425653695)) ;
#127201=CARTESIAN_POINT('Ctrl Pts',(-16.5316439561812,13.7085066706188,
131.335769713184)) ;
#127202=CARTESIAN_POINT('Ctrl Pts',(-16.5303800842125,13.3995793923712,
131.299014333936)) ;
#127203=CARTESIAN_POINT('Ctrl Pts',(-16.5559587992191,13.0919774693214,
131.340640261352)) ;
#127204=CARTESIAN_POINT('Ctrl Pts',(-16.6078284638175,12.8067303773131,
131.458887738409)) ;
#127205=CARTESIAN_POINT('Ctrl Pts',(-16.6818970632097,12.5682008824759,
131.642331999797)) ;
#127206=CARTESIAN_POINT('Ctrl Pts',(-16.774928635233,12.3888212214355,131.88087429486)) ;
#127207=CARTESIAN_POINT('Ctrl Pts',(-16.8800323422373,12.2844119471438,
132.154816836978)) ;
#127208=CARTESIAN_POINT('Ctrl Pts',(-16.9908532021063,12.2613333945147,
132.445409149157)) ;
#127209=CARTESIAN_POINT('Ctrl Pts',(-17.0999913187427,12.3215794553672,
132.731106180485)) ;
#127210=CARTESIAN_POINT('Ctrl Pts',(-17.2003631560383,12.4606919099578,
132.991204117191)) ;
#127211=CARTESIAN_POINT('Ctrl Pts',(-17.2855599741373,12.6684213928488,
133.206995727513)) ;
#127212=CARTESIAN_POINT('Ctrl Pts',(-17.3504941522615,12.9319195354802,
133.363395978862)) ;
#127213=CARTESIAN_POINT('Ctrl Pts',(-17.3904330455179,13.2279082414743,
133.447106708526)) ;
#127214=CARTESIAN_POINT('Ctrl Pts',(-17.4040816521376,13.5392233230321,
133.453849322429)) ;
#127215=CARTESIAN_POINT('Ctrl Pts',(-17.390836167045,13.8421683173594,133.382041888976)) ;
#127216=CARTESIAN_POINT('Ctrl Pts',(-17.3522690738895,14.1158320229517,
133.236165936095)) ;
#127217=CARTESIAN_POINT('Ctrl Pts',(-17.2920552027206,14.3390093108208,
133.027146596858)) ;
#127218=CARTESIAN_POINT('Ctrl Pts',(-17.2153391517714,14.4964745631391,
132.769969650378)) ;
#127219=CARTESIAN_POINT('Ctrl Pts',(-17.128130190575,14.5773715751741,132.482106689292)) ;
#127220=CARTESIAN_POINT('Ctrl Pts',(-17.0373151597888,14.5757025299613,
132.183661495111)) ;
#127221=CARTESIAN_POINT('Ctrl Pts',(-16.9501102952013,14.4908671144554,
131.895689095071)) ;
#127222=CARTESIAN_POINT('Ctrl Pts',(-16.8742256801646,14.3305923177535,
131.641031426237)) ;
#127223=CARTESIAN_POINT('Ctrl Pts',(-16.8147980608555,14.1048090701634,
131.434285608037)) ;
#127224=CARTESIAN_POINT('Ctrl Pts',(-16.7773101810593,13.8293691647795,
131.291565197932)) ;
#127225=CARTESIAN_POINT('Ctrl Pts',(-16.7652035431411,13.5265763718341,
131.223186509187)) ;
#127226=CARTESIAN_POINT('Ctrl Pts',(-16.7799662486554,13.2147295079812,
131.233113488118)) ;
#127227=CARTESIAN_POINT('Ctrl Pts',(-16.8212080996971,12.9189025307067,
131.320522875433)) ;
#127228=CARTESIAN_POINT('Ctrl Pts',(-16.887084338435,12.6580299583616,131.47973575403)) ;
#127229=CARTESIAN_POINT('Ctrl Pts',(-16.9727965429337,12.4534345786707,
131.697120401721)) ;
#127230=CARTESIAN_POINT('Ctrl Pts',(-17.0739808799952,12.3171076737635,
131.959493126955)) ;
#127231=CARTESIAN_POINT('Ctrl Pts',(-17.1832345072622,12.2606844029487,
132.245561618487)) ;
#127232=CARTESIAN_POINT('Ctrl Pts',(-17.2938303511549,12.2870889528383,
132.53554165159)) ;
#127233=CARTESIAN_POINT('Ctrl Pts',(-17.399072000023,12.3957983082861,132.809701372333)) ;
#127234=CARTESIAN_POINT('Ctrl Pts',(-17.4906848011028,12.5767257036487,
133.044366686444)) ;
#127235=CARTESIAN_POINT('Ctrl Pts',(-17.5643113957083,12.818699316301,133.226334863995)) ;
#127236=CARTESIAN_POINT('Ctrl Pts',(-17.6149368941073,13.105041814552,133.341009417793)) ;
#127237=CARTESIAN_POINT('Ctrl Pts',(-17.6393801095251,13.4130762761878,
133.379325378718)) ;
#127238=CARTESIAN_POINT('Ctrl Pts',(-17.636930864629,13.7214651892491,133.339116703289)) ;
#127239=CARTESIAN_POINT('Ctrl Pts',(-17.6084372265889,14.0093161776234,
133.222748419654)) ;
#127240=CARTESIAN_POINT('Ctrl Pts',(-17.5562396423716,14.2560736746046,
133.036976545508)) ;
#127241=CARTESIAN_POINT('Ctrl Pts',(-17.4856556413898,14.4412184345139,
132.797774201954)) ;
#127242=CARTESIAN_POINT('Ctrl Pts',(-17.4019418945911,14.5543182512014,
132.52014511049)) ;
#127243=CARTESIAN_POINT('Ctrl Pts',(-17.3116311006331,14.5864671227743,
132.223159968999)) ;
#127244=CARTESIAN_POINT('Ctrl Pts',(-17.2222810781303,14.5351930421584,
131.929026268783)) ;
#127245=CARTESIAN_POINT('Ctrl Pts',(-17.1408794351008,14.4042256673591,
131.65810101633)) ;
#127246=CARTESIAN_POINT('Ctrl Pts',(-17.0740974975755,14.2033620088234,
131.429938282516)) ;
#127247=CARTESIAN_POINT('Ctrl Pts',(-17.0271797587778,13.9460943123355,
131.25972015051)) ;
#127248=CARTESIAN_POINT('Ctrl Pts',(-17.0044838482656,13.651094014162,131.160246420146)) ;
#127249=CARTESIAN_POINT('Ctrl Pts',(-17.0082440978773,13.340963258282,131.138187893648)) ;
#127250=CARTESIAN_POINT('Ctrl Pts',(-17.0389664768321,13.0355469071403,
131.194763803826)) ;
#127251=CARTESIAN_POINT('Ctrl Pts',(-17.0951171059167,12.7584810147084,
131.325687533703)) ;
#127252=CARTESIAN_POINT('Ctrl Pts',(-17.1734699410036,12.5287898592304,
131.521440438767)) ;
#127253=CARTESIAN_POINT('Ctrl Pts',(-17.2690431091153,12.3633457050948,
131.76752542984)) ;
#127254=CARTESIAN_POINT('Ctrl Pts',(-17.3757413243156,12.2737023356338,
132.046114426366)) ;
#127255=CARTESIAN_POINT('Ctrl Pts',(-17.4868753525456,12.2663504555484,
132.337605074947)) ;
#127256=CARTESIAN_POINT('Ctrl Pts',(-17.594933557408,12.3420801358765,132.620132638066)) ;
#127257=CARTESIAN_POINT('Ctrl Pts',(-17.6927107918119,12.4946576254463,
132.872726617329)) ;
#127258=CARTESIAN_POINT('Ctrl Pts',(-17.7746021706281,12.7142649717312,
133.078788363608)) ;
#127259=CARTESIAN_POINT('Ctrl Pts',(-17.8350304744198,12.9853994961716,
133.222096163646)) ;
#127260=CARTESIAN_POINT('Ctrl Pts',(-17.8701999131744,13.2860374615536,
133.291826279773)) ;
#127261=CARTESIAN_POINT('Ctrl Pts',(-17.8787429450958,13.5985522242575,
133.283546361451)) ;
#127262=CARTESIAN_POINT('Ctrl Pts',(-17.860400130644,13.8975128735152,133.19682396488)) ;
#127263=CARTESIAN_POINT('Ctrl Pts',(-17.817739731672,14.1612606569833,133.039235284081)) ;
#127264=CARTESIAN_POINT('Ctrl Pts',(-17.7539424298962,14.3739608476098,
132.819679716885)) ;
#127265=CARTESIAN_POINT('Ctrl Pts',(-17.6743276947805,14.518294704107,132.553868013413)) ;
#127266=CARTESIAN_POINT('Ctrl Pts',(-17.5858816850883,14.5834512840226,
132.262389383018)) ;
#127267=CARTESIAN_POINT('Ctrl Pts',(-17.495671887429,14.5659482192211,131.965871431279)) ;
#127268=CARTESIAN_POINT('Ctrl Pts',(-17.4102025645197,14.4667697740707,
131.683072426799)) ;
#127269=CARTESIAN_POINT('Ctrl Pts',(-17.3365053893818,14.2923285700355,
131.434587124343)) ;
#127270=CARTESIAN_POINT('Ctrl Pts',(-17.2808753696568,14.0548140486651,
131.23883528978)) ;
#127271=CARTESIAN_POINT('Ctrl Pts',(-17.2482486938309,13.7751054294997,
131.110643536837)) ;
#127272=CARTESIAN_POINT('Ctrl Pts',(-17.2409723432271,13.4671706932676,
131.056143962947)) ;
#127273=CARTESIAN_POINT('Ctrl Pts',(-17.2609660776528,13.1566326789877,
131.081373755266)) ;
#127274=CARTESIAN_POINT('Ctrl Pts',(-17.3068303971445,12.8670308674408,
131.182397606284)) ;
#127275=CARTESIAN_POINT('Ctrl Pts',(-17.3769423374258,12.6146257445343,
131.353937047391)) ;
#127276=CARTESIAN_POINT('Ctrl Pts',(-17.4663324172258,12.4216271707414,
131.581933589309)) ;
#127277=CARTESIAN_POINT('Ctrl Pts',(-17.5689151592292,12.3004936343569,
131.848623819979)) ;
#127278=CARTESIAN_POINT('Ctrl Pts',(-17.6795235886028,12.2591976943178,
132.138478362093)) ;
#127279=CARTESIAN_POINT('Ctrl Pts',(-17.7892104427003,12.3014766465694,
132.425902609519)) ;
#127280=CARTESIAN_POINT('Ctrl Pts',(-17.8921201526179,12.4236752423031,
132.693416377678)) ;
#127281=CARTESIAN_POINT('Ctrl Pts',(-17.9816733272528,12.6191375568078,
132.921700911216)) ;
#127282=CARTESIAN_POINT('Ctrl Pts',(-18.0509804191005,12.8707902400354,
133.091098623039)) ;
#127283=CARTESIAN_POINT('Ctrl Pts',(-18.0966425229612,13.1617413268143,
133.191421711028)) ;
#127284=CARTESIAN_POINT('Ctrl Pts',(-18.1160955250332,13.4713352737269,
133.215187444689)) ;
#127285=CARTESIAN_POINT('Ctrl Pts',(-18.1085938517289,13.7785022138413,
133.160099094131)) ;
#127286=CARTESIAN_POINT('Ctrl Pts',(-18.0753539943821,14.0596469368124,
133.029881338672)) ;
#127287=CARTESIAN_POINT('Ctrl Pts',(-18.0195475480246,14.2953142567661,
132.833735930946)) ;
#127288=CARTESIAN_POINT('Ctrl Pts',(-17.9455889588625,14.4689647332084,
132.584457804222)) ;
#127289=CARTESIAN_POINT('Ctrl Pts',(-17.8599266157843,14.5668407340065,
132.301076581191)) ;
#127290=CARTESIAN_POINT('Ctrl Pts',(-17.7697656720865,14.5831863615057,
132.004729955571)) ;
#127291=CARTESIAN_POINT('Ctrl Pts',(-17.6808976127122,14.5160479174659,
131.711817961361)) ;
#127292=CARTESIAN_POINT('Ctrl Pts',(-17.6020563422739,14.3710573530436,
131.448475490699)) ;
#127293=CARTESIAN_POINT('Ctrl Pts',(-17.5386862603335,14.1586832186318,
131.230302219222)) ;
#127294=CARTESIAN_POINT('Ctrl Pts',(-17.4960439142544,13.8924168097658,
131.072530591824)) ;
#127295=CARTESIAN_POINT('Ctrl Pts',(-17.4782543290687,13.5934590630732,
130.987477632941)) ;
#127296=CARTESIAN_POINT('Ctrl Pts',(-17.4871300560662,13.2817949508325,
130.980261275632)) ;
#127297=CARTESIAN_POINT('Ctrl Pts',(-17.5227969121146,12.9807520838768,
131.051361569795)) ;
#127298=CARTESIAN_POINT('Ctrl Pts',(-17.5832892800494,12.7114088692144,
131.195005608496)) ;
#127299=CARTESIAN_POINT('Ctrl Pts',(-17.6655555316227,12.4920355710748,
131.402094610911)) ;
#127300=CARTESIAN_POINT('Ctrl Pts',(-17.763605317929,12.3404092306431,131.655461365325)) ;
#127301=CARTESIAN_POINT('Ctrl Pts',(-17.8717998624488,12.2658594230555,
131.938374035989)) ;
#127302=CARTESIAN_POINT('Ctrl Pts',(-17.9828025573186,12.2744067792623,
132.229517358147)) ;
#127303=CARTESIAN_POINT('Ctrl Pts',(-18.0893965868874,12.3651073701196,
132.507801972934)) ;
#127304=CARTESIAN_POINT('Ctrl Pts',(-18.1848253344922,12.5316552741645,
132.75344430614)) ;
#127305=CARTESIAN_POINT('Ctrl Pts',(-18.262910706008,12.7621961418758,132.948410377436)) ;
#127306=CARTESIAN_POINT('Ctrl Pts',(-18.3187167918841,13.0400249210017,
133.078305446668)) ;
#127307=CARTESIAN_POINT('Ctrl Pts',(-18.3490238590159,13.3449925039121,
133.133743315381)) ;
#127308=CARTESIAN_POINT('Ctrl Pts',(-18.3523960346358,13.6560824350963,
133.110438469782)) ;
#127309=CARTESIAN_POINT('Ctrl Pts',(-18.3293782283672,13.9495230290834,
133.010150889642)) ;
#127310=CARTESIAN_POINT('Ctrl Pts',(-18.2822975086196,14.2060602053469,
132.839491487932)) ;
#127311=CARTESIAN_POINT('Ctrl Pts',(-18.2150042015936,14.4068533701998,
132.609701973779)) ;
#127312=CARTESIAN_POINT('Ctrl Pts',(-18.1335066452029,14.5364834485285,
132.338532395409)) ;
#127313=CARTESIAN_POINT('Ctrl Pts',(-18.0440812727696,14.5865952297017,
132.044172252159)) ;
#127314=CARTESIAN_POINT('Ctrl Pts',(-17.9539167615346,14.553289693682,131.747651900659)) ;
#127315=CARTESIAN_POINT('Ctrl Pts',(-17.8702528974652,14.4391769973074,
131.470146326373)) ;
#127316=CARTESIAN_POINT('Ctrl Pts',(-17.7997194469578,14.2521193924325,
131.230968722829)) ;
#127317=CARTESIAN_POINT('Ctrl Pts',(-17.7481700755364,14.0064610013992,
131.04733335877)) ;
#127318=CARTESIAN_POINT('Ctrl Pts',(-17.719812684897,13.7162751839027,130.931136251967)) ;
#127319=CARTESIAN_POINT('Ctrl Pts',(-17.7178318605647,13.4088590372776,
130.89242456443)) ;
#127320=CARTESIAN_POINT('Ctrl Pts',(-17.7426554414359,13.1005339015723,
130.93180097624)) ;
#127321=CARTESIAN_POINT('Ctrl Pts',(-17.7935721191777,12.8153801442626,
131.04739716275)) ;
#127322=CARTESIAN_POINT('Ctrl Pts',(-17.8671815808783,12.5742829419459,
131.229393212351)) ;
#127323=CARTESIAN_POINT('Ctrl Pts',(-17.9602575957707,12.3924207775489,
131.467913394784)) ;
#127324=CARTESIAN_POINT('Ctrl Pts',(-18.0645711388433,12.2864008537638,
131.739720121866)) ;
#127325=CARTESIAN_POINT('Ctrl Pts',(-18.1756856987231,12.2608494079679,
132.031060726295)) ;
#127326=CARTESIAN_POINT('Ctrl Pts',(-18.2845081582116,12.3186106579848,
132.315974866748)) ;
#127327=CARTESIAN_POINT('Ctrl Pts',(-18.385443297942,12.4554523175926,132.577666349289)) ;
#127328=CARTESIAN_POINT('Ctrl Pts',(-18.4714425406617,12.6626735352652,
132.79564979499)) ;
#127329=CARTESIAN_POINT('Ctrl Pts',(-18.5363857643237,12.9221025997255,
132.952420893401)) ;
#127330=CARTESIAN_POINT('Ctrl Pts',(-18.577483280411,13.2188658748081,133.039325926442)) ;
#127331=CARTESIAN_POINT('Ctrl Pts',(-18.5918395715828,13.5309969609299,
133.048045174373)) ;
#127332=CARTESIAN_POINT('Ctrl Pts',(-18.579379357718,13.8333910291505,132.978648701175)) ;
#127333=CARTESIAN_POINT('Ctrl Pts',(-18.5415509639557,14.1082732516314,
132.834930655177)) ;
#127334=CARTESIAN_POINT('Ctrl Pts',(-18.4819140851022,14.3332733930533,
132.627591939092)) ;
#127335=CARTESIAN_POINT('Ctrl Pts',(-18.4054218771447,14.4930899265818,
132.370995081213)) ;
#127336=CARTESIAN_POINT('Ctrl Pts',(-18.318516382284,14.5762694731203,132.084061324625)) ;
#127337=CARTESIAN_POINT('Ctrl Pts',(-18.2273640153455,14.5766426477847,
131.784499589454)) ;
#127338=CARTESIAN_POINT('Ctrl Pts',(-18.1407406750204,14.4950561808568,
131.498537978266)) ;
#127339=CARTESIAN_POINT('Ctrl Pts',(-18.0637621533931,14.3357812745788,
131.240402844972)) ;
#127340=CARTESIAN_POINT('Ctrl Pts',(-18.0040164942051,14.1117726317635,
131.032799043462)) ;
#127341=CARTESIAN_POINT('Ctrl Pts',(-17.9658474460896,13.8385112435954,
130.88819300603)) ;
#127342=CARTESIAN_POINT('Ctrl Pts',(-17.9529773698967,13.5338962434735,
130.817328335414)) ;
#127343=CARTESIAN_POINT('Ctrl Pts',(-17.966902192937,13.2242575692473,130.825061227403)) ;
#127344=CARTESIAN_POINT('Ctrl Pts',(-18.0076010778523,12.9262819012927,
130.910714299643)) ;
#127345=CARTESIAN_POINT('Ctrl Pts',(-18.0724284818989,12.6654698435916,
131.067059131794)) ;
#127346=CARTESIAN_POINT('Ctrl Pts',(-18.1584381429643,12.4574146101121,
131.285007474977)) ;
#127347=CARTESIAN_POINT('Ctrl Pts',(-18.2582335314427,12.3205165550688,
131.543682575533)) ;
#127348=CARTESIAN_POINT('Ctrl Pts',(-18.3679353654617,12.2610390468186,
131.83086496086)) ;
#127349=CARTESIAN_POINT('Ctrl Pts',(-18.4782367394613,12.2851065141721,
132.120097103203)) ;
#127350=CARTESIAN_POINT('Ctrl Pts',(-18.5838705524631,12.3913707511119,
132.395368945134)) ;
#127351=CARTESIAN_POINT('Ctrl Pts',(-18.6760360416254,12.5705078775683,
132.631617960708)) ;
#127352=CARTESIAN_POINT('Ctrl Pts',(-18.7502684218209,12.8110530886845,
132.815345268963)) ;
#127353=CARTESIAN_POINT('Ctrl Pts',(-18.8015583285115,13.0958080980136,
132.932027482214)) ;
#127354=CARTESIAN_POINT('Ctrl Pts',(-18.8268471368734,13.4043791366155,
132.972713046166)) ;
#127355=CARTESIAN_POINT('Ctrl Pts',(-18.8252076834743,13.7127503618814,
132.934914084386)) ;
#127356=CARTESIAN_POINT('Ctrl Pts',(-18.7970965372467,14.0031465413693,
132.819442522481)) ;
#127357=CARTESIAN_POINT('Ctrl Pts',(-18.7462208827452,14.2480984891944,
132.637984092409)) ;
#127358=CARTESIAN_POINT('Ctrl Pts',(-18.6756901548005,14.4370589148149,
132.398678768597)) ;
#127359=CARTESIAN_POINT('Ctrl Pts',(-18.5922636520362,14.5521322470153,
132.121910980458)) ;
#127360=CARTESIAN_POINT('Ctrl Pts',(-18.5019465438144,14.5867077632741,
131.824868753365)) ;
#127361=CARTESIAN_POINT('Ctrl Pts',(-18.412633202275,14.5378478961583,131.53090432153)) ;
#127362=CARTESIAN_POINT('Ctrl Pts',(-18.330920319899,14.4092030329905,131.25907687015)) ;
#127363=CARTESIAN_POINT('Ctrl Pts',(-18.263569768423,14.2102655256447,131.0292461752)) ;
#127364=CARTESIAN_POINT('Ctrl Pts',(-18.2158792663467,13.953116489833,130.856624729037)) ;
#127365=CARTESIAN_POINT('Ctrl Pts',(-18.1925908882483,13.6605445363077,
130.755610904485)) ;
#127366=CARTESIAN_POINT('Ctrl Pts',(-18.1955599085021,13.3493859858442,
130.731108302227)) ;
#127367=CARTESIAN_POINT('Ctrl Pts',(-18.225463343713,13.0444135456855,130.785394374056)) ;
#127368=CARTESIAN_POINT('Ctrl Pts',(-18.2809528308207,12.7658508988887,
130.914341636667)) ;
#127369=CARTESIAN_POINT('Ctrl Pts',(-18.3586927250528,12.5346698659633,
131.108322839338)) ;
#127370=CARTESIAN_POINT('Ctrl Pts',(-18.4539903952345,12.3668713025773,
131.35355113485)) ;
#127371=CARTESIAN_POINT('Ctrl Pts',(-18.5606691035786,12.2750736510529,
131.632027177276)) ;
#127372=CARTESIAN_POINT('Ctrl Pts',(-18.6712133617814,12.2654123837922,
131.921964147422)) ;
#127373=CARTESIAN_POINT('Ctrl Pts',(-18.7795370897269,12.3385001121927,
132.205249883484)) ;
#127374=CARTESIAN_POINT('Ctrl Pts',(-18.8779628205114,12.4893940977294,
132.459650590027)) ;
#127375=CARTESIAN_POINT('Ctrl Pts',(-18.9602735680414,12.7071835395625,
132.66696984749)) ;
#127376=CARTESIAN_POINT('Ctrl Pts',(-19.0212463662573,12.9760086815988,
132.811986888924)) ;
#127377=CARTESIAN_POINT('Ctrl Pts',(-19.0573505327277,13.2771671350434,
132.884317676009)) ;
#127378=CARTESIAN_POINT('Ctrl Pts',(-19.0666443316968,13.5885363726329,
132.878356779271)) ;
#127379=CARTESIAN_POINT('Ctrl Pts',(-19.0492100110848,13.8883474938027,
132.794283427)) ;
#127380=CARTESIAN_POINT('Ctrl Pts',(-19.0070053612913,14.1546797324028,
132.637863556914)) ;
#127381=CARTESIAN_POINT('Ctrl Pts',(-18.9438705951811,14.3683945164845,
132.420333719808)) ;
#127382=CARTESIAN_POINT('Ctrl Pts',(-18.8649903948833,14.5146640414989,
132.156794887638)) ;
#127383=CARTESIAN_POINT('Ctrl Pts',(-18.7764317944818,14.5827891573481,
131.864873053478)) ;
#127384=CARTESIAN_POINT('Ctrl Pts',(-18.6859695685718,14.5676065967762,
131.567543317184)) ;
#127385=CARTESIAN_POINT('Ctrl Pts',(-18.6002872834926,14.4706131159399,
131.284128345717)) ;
#127386=CARTESIAN_POINT('Ctrl Pts',(-18.5263602634957,14.2987449000821,
131.035067449585)) ;
#127387=CARTESIAN_POINT('Ctrl Pts',(-18.4700659060945,14.063095802434,130.837382283135)) ;
#127388=CARTESIAN_POINT('Ctrl Pts',(-18.4365708056881,13.7833208359645,
130.706522805611)) ;
#127389=CARTESIAN_POINT('Ctrl Pts',(-18.4286425713622,13.4754883225496,
130.650088164264)) ;
#127390=CARTESIAN_POINT('Ctrl Pts',(-18.4476840985486,13.1664272763286,
130.6727229201)) ;
#127391=CARTESIAN_POINT('Ctrl Pts',(-18.4930612119151,12.8743475214726,
130.772135696503)) ;
#127392=CARTESIAN_POINT('Ctrl Pts',(-18.5621657253508,12.6220180673462,
130.940924124175)) ;
#127393=CARTESIAN_POINT('Ctrl Pts',(-18.6511402558302,12.4263341483682,
131.167639758192)) ;
#127394=CARTESIAN_POINT('Ctrl Pts',(-18.7540070326684,12.302605659073,131.434983940839)) ;
#127395=CARTESIAN_POINT('Ctrl Pts',(-18.863849205629,12.2593725247806,131.722798446897)) ;
#127396=CARTESIAN_POINT('Ctrl Pts',(-18.973774779168,12.2987734021689,132.010889389283)) ;
#127397=CARTESIAN_POINT('Ctrl Pts',(-19.0777342115767,12.4202091773167,
132.281205608139)) ;
#127398=CARTESIAN_POINT('Ctrl Pts',(-19.1667519677935,12.6117736562181,
132.508295443949)) ;
#127399=CARTESIAN_POINT('Ctrl Pts',(-19.2370781843148,12.8626551569237,
132.68053965318)) ;
#127400=CARTESIAN_POINT('Ctrl Pts',(-19.2834369312527,13.1527448320073,
132.782907458416)) ;
#127401=CARTESIAN_POINT('Ctrl Pts',(-19.3037163223515,13.4624297819909,
132.809050097769)) ;
#127402=CARTESIAN_POINT('Ctrl Pts',(-19.2969382971085,13.7701810821573,
132.756055702704)) ;
#127403=CARTESIAN_POINT('Ctrl Pts',(-19.2644749678557,14.0517728376964,
132.628174098256)) ;
#127404=CARTESIAN_POINT('Ctrl Pts',(-19.2092617891683,14.2892526795151,
132.433742339541)) ;
#127405=CARTESIAN_POINT('Ctrl Pts',(-19.1357237949252,14.4648240216747,
132.18568928131)) ;
#127406=CARTESIAN_POINT('Ctrl Pts',(-19.0506014968616,14.5650403080843,
131.903990457871)) ;
#127407=CARTESIAN_POINT('Ctrl Pts',(-18.9599105479305,14.5837489578772,
131.605878754956)) ;
#127408=CARTESIAN_POINT('Ctrl Pts',(-18.8716845059285,14.519716790758,131.315155450063)) ;
#127409=CARTESIAN_POINT('Ctrl Pts',(-18.7918891339899,14.3763314788885,
131.048799530724)) ;
#127410=CARTESIAN_POINT('Ctrl Pts',(-18.7280288453663,14.1656645339802,
130.829210159184)) ;
#127411=CARTESIAN_POINT('Ctrl Pts',(-18.6846483717695,13.8999128484359,
130.669191362741)) ;
#127412=CARTESIAN_POINT('Ctrl Pts',(-18.6662190108552,13.6028235446839,
130.582407931147)) ;
#127413=CARTESIAN_POINT('Ctrl Pts',(-18.6742464552894,13.291184558806,130.572707258654)) ;
#127414=CARTESIAN_POINT('Ctrl Pts',(-18.7091131232011,12.9894030516706,
130.641463295222)) ;
#127415=CARTESIAN_POINT('Ctrl Pts',(-18.7692083838662,12.7177659651588,
130.783807359682)) ;
#127416=CARTESIAN_POINT('Ctrl Pts',(-18.8508792403486,12.49725897855,130.989207530208)) ;
#127417=CARTESIAN_POINT('Ctrl Pts',(-18.9482660761094,12.3438957408669,
131.240727643345)) ;
#127418=CARTESIAN_POINT('Ctrl Pts',(-19.05636616245,12.2668705214432,131.523331846997)) ;
#127419=CARTESIAN_POINT('Ctrl Pts',(-19.1672657480986,12.2729078136877,
131.814213167649)) ;
#127420=CARTESIAN_POINT('Ctrl Pts',(-19.2742485294026,12.3614501444855,
132.093578354288)) ;
#127421=CARTESIAN_POINT('Ctrl Pts',(-19.3698500840989,12.5253315069565,
132.339824187223)) ;
#127422=CARTESIAN_POINT('Ctrl Pts',(-19.4488726784715,12.75527704082,132.537372789972)) ;
#127423=CARTESIAN_POINT('Ctrl Pts',(-19.5051561125912,13.0310569738766,
132.668784632231)) ;
#127424=CARTESIAN_POINT('Ctrl Pts',(-19.5363072236389,13.336121760913,132.726616640379)) ;
#127425=CARTESIAN_POINT('Ctrl Pts',(-19.5404981195686,13.6463105031288,
132.705820995574)) ;
#127426=CARTESIAN_POINT('Ctrl Pts',(-19.518114994087,13.942487386476,132.607173328192)) ;
#127427=CARTESIAN_POINT('Ctrl Pts',(-19.4714777997713,14.2002009126819,
132.437787788337)) ;
#127428=CARTESIAN_POINT('Ctrl Pts',(-19.4051407217541,14.4015262560108,
132.211010588083)) ;
#127429=CARTESIAN_POINT('Ctrl Pts',(-19.3237681020821,14.5339054968789,
131.940108509089)) ;
#127430=CARTESIAN_POINT('Ctrl Pts',(-19.2345252922065,14.5863178640126,
131.646306132299)) ;
#127431=CARTESIAN_POINT('Ctrl Pts',(-19.1440412498707,14.5553221759541,
131.348765178843)) ;
#127432=CARTESIAN_POINT('Ctrl Pts',(-19.0601605583772,14.4431215041297,
131.070631058535)) ;
#127433=CARTESIAN_POINT('Ctrl Pts',(-18.9894132116751,14.2589451929284,
130.830971500932)) ;
#127434=CARTESIAN_POINT('Ctrl Pts',(-18.937005220446,14.0132050920919,130.644627150308)) ;
#127435=CARTESIAN_POINT('Ctrl Pts',(-18.9081356286921,13.7264814749198,
130.527228397387)) ;
#127436=CARTESIAN_POINT('Ctrl Pts',(-18.9052947680092,13.4166671234753,
130.485706040313)) ;
#127437=CARTESIAN_POINT('Ctrl Pts',(-18.929408442906,13.1090562116308,130.523121657094)) ;
#127438=CARTESIAN_POINT('Ctrl Pts',(-18.9795705721345,12.82289367226,130.636511356112)) ;
#127439=CARTESIAN_POINT('Ctrl Pts',(-19.0526557005628,12.5803482566307,
130.816963585608)) ;
#127440=CARTESIAN_POINT('Ctrl Pts',(-19.1448178981947,12.3971382864686,
131.052964112262)) ;
#127441=CARTESIAN_POINT('Ctrl Pts',(-19.2493867509754,12.2881794770673,
131.325344156453)) ;
#127442=CARTESIAN_POINT('Ctrl Pts',(-19.3602648969248,12.2604447735571,
131.616048800621)) ;
#127443=CARTESIAN_POINT('Ctrl Pts',(-19.4694574725562,12.3158800471475,
131.901978170805)) ;
#127444=CARTESIAN_POINT('Ctrl Pts',(-19.5708086836812,12.4512316162553,
132.164831500501)) ;
#127445=CARTESIAN_POINT('Ctrl Pts',(-19.6566330326797,12.6546809483565,
132.382594308953)) ;
#127446=CARTESIAN_POINT('Ctrl Pts',(-19.7227990938615,12.9147731293523,
132.542666384145)) ;
#127447=CARTESIAN_POINT('Ctrl Pts',(-19.7643882259244,13.2095559485039,
132.63116114933)) ;
#127448=CARTESIAN_POINT('Ctrl Pts',(-19.7796070435146,13.5223874270332,
132.642305936428)) ;
#127449=CARTESIAN_POINT('Ctrl Pts',(-19.7679012234026,13.825017500004,132.575151248593)) ;
#127450=CARTESIAN_POINT('Ctrl Pts',(-19.7305546086185,14.1019895669497,
132.432709178594)) ;
#127451=CARTESIAN_POINT('Ctrl Pts',(-19.6717250733561,14.3273312659445,
132.227898463628)) ;
#127452=CARTESIAN_POINT('Ctrl Pts',(-19.5957391597017,14.4893435493457,
131.972801925455)) ;
#127453=CARTESIAN_POINT('Ctrl Pts',(-19.5089482125021,14.5749600096558,
131.686164493976)) ;
#127454=CARTESIAN_POINT('Ctrl Pts',(-19.417900802232,14.5779281254001,131.386950092277)) ;
#127455=CARTESIAN_POINT('Ctrl Pts',(-19.3308419334919,14.4983365281884,
131.099618335491)) ;
#127456=CARTESIAN_POINT('Ctrl Pts',(-19.2537905566691,14.3420896185929,
130.841432757655)) ;
#127457=CARTESIAN_POINT('Ctrl Pts',(-19.1930145272651,14.1180211548404,
130.630556327185)) ;
#127458=CARTESIAN_POINT('Ctrl Pts',(-19.154480323418,13.8471808602615,130.485062911182)) ;
#127459=CARTESIAN_POINT('Ctrl Pts',(-19.1407432544812,13.5439413026185,
130.411739692858)) ;
#127460=CARTESIAN_POINT('Ctrl Pts',(-19.15388806011,13.2331634650753,130.417082866503)) ;
#127461=CARTESIAN_POINT('Ctrl Pts',(-19.1938580856356,12.9343808446189,
130.500600026674)) ;
#127462=CARTESIAN_POINT('Ctrl Pts',(-19.2581221044548,12.672197812707,130.655272820994)) ;
#127463=CARTESIAN_POINT('Ctrl Pts',(-19.3430998639908,12.4632419540624,
130.870384738628)) ;
#127464=CARTESIAN_POINT('Ctrl Pts',(-19.4431486006855,12.3231158661213,
131.129588810294)) ;
#127465=CARTESIAN_POINT('Ctrl Pts',(-19.5527011367039,12.2616017897263,
131.416345012905)) ;
#127466=CARTESIAN_POINT('Ctrl Pts',(-19.6628580182651,12.2833201820527,
131.705210375093)) ;
#127467=CARTESIAN_POINT('Ctrl Pts',(-19.7685636148286,12.3868877345153,
131.980760889968)) ;
#127468=CARTESIAN_POINT('Ctrl Pts',(-19.8616044368723,12.5648231371291,
132.219418056293)) ;
#127469=CARTESIAN_POINT('Ctrl Pts',(-19.9363026361166,12.8039602179339,
132.404522691316)) ;
#127470=CARTESIAN_POINT('Ctrl Pts',(-19.9881245670103,13.0864729050957,
132.522897300744)) ;
#127471=CARTESIAN_POINT('Ctrl Pts',(-20.0143271197124,13.3957238460679,
132.566138555961)) ;
#127472=CARTESIAN_POINT('Ctrl Pts',(-20.0133509573114,13.7038340446914,
132.530324240887)) ;
#127473=CARTESIAN_POINT('Ctrl Pts',(-19.9863447007775,13.9936201440332,
132.418290739287)) ;
#127474=CARTESIAN_POINT('Ctrl Pts',(-19.9353998662376,14.2431366555827,
132.236196148023)) ;
#127475=CARTESIAN_POINT('Ctrl Pts',(-19.8660196038327,14.4318623927357,
132.000605777573)) ;
#127476=CARTESIAN_POINT('Ctrl Pts',(-19.7823664836586,14.5502397441639,
131.722943739338)) ;
#127477=CARTESIAN_POINT('Ctrl Pts',(-19.6923571646773,14.5868194745111,
131.426895066885)) ;
#127478=CARTESIAN_POINT('Ctrl Pts',(-19.6028197002359,14.5403267792944,
131.132230972924)) ;
#127479=CARTESIAN_POINT('Ctrl Pts',(-19.5208138211862,14.4138414926087,
130.859561159112)) ;
#127480=CARTESIAN_POINT('Ctrl Pts',(-19.4529603624471,14.2163546967306,
130.62822332568)) ;
#127481=CARTESIAN_POINT('Ctrl Pts',(-19.404898468416,13.962464783628,130.454747355412)) ;
#127482=CARTESIAN_POINT('Ctrl Pts',(-19.3806595868205,13.6693367580008,
130.35078618193)) ;
#127483=CARTESIAN_POINT('Ctrl Pts',(-19.3828689401698,13.3586798418074,
130.324104636)) ;
#127484=CARTESIAN_POINT('Ctrl Pts',(-19.4120401332624,13.0526929530247,
130.376190283202)) ;
#127485=CARTESIAN_POINT('Ctrl Pts',(-19.4668451940639,12.7731728077457,
130.503149233202)) ;
#127486=CARTESIAN_POINT('Ctrl Pts',(-19.5440168549277,12.5404162023862,
130.695468362471)) ;
#127487=CARTESIAN_POINT('Ctrl Pts',(-19.6387913027967,12.3707607989948,
130.939204508807)) ;
#127488=CARTESIAN_POINT('Ctrl Pts',(-19.7452133373752,12.2766729601255,
131.216934024696)) ;
#127489=CARTESIAN_POINT('Ctrl Pts',(-19.8556874181351,12.2643218460961,
131.506684005263)) ;
#127490=CARTESIAN_POINT('Ctrl Pts',(-19.9649749082845,12.3360206522436,
131.792531104291)) ;
#127491=CARTESIAN_POINT('Ctrl Pts',(-20.0628344188298,12.4836397048973,
132.045586237291)) ;
#127492=CARTESIAN_POINT('Ctrl Pts',(-20.1460777106979,12.7003319185399,
132.255494068561)) ;
#127493=CARTESIAN_POINT('Ctrl Pts',(-20.2076327001099,12.9678917727225,
132.402235467722)) ;
#127494=CARTESIAN_POINT('Ctrl Pts',(-20.2445186297781,13.2687869300656,
132.476808723273)) ;
#127495=CARTESIAN_POINT('Ctrl Pts',(-20.2545206843836,13.5800035034693,
132.472934888553)) ;
#127496=CARTESIAN_POINT('Ctrl Pts',(-20.2378647958217,13.8799729722643,
132.391189049575)) ;
#127497=CARTESIAN_POINT('Ctrl Pts',(-20.196316210114,14.14769940646,132.236667861987)) ;
#127498=CARTESIAN_POINT('Ctrl Pts',(-20.1336983474538,14.3632524598664,
132.020637059241)) ;
#127499=CARTESIAN_POINT('Ctrl Pts',(-20.0549288300243,14.511933585639,131.757324538327)) ;
#127500=CARTESIAN_POINT('Ctrl Pts',(-19.9666034114372,14.5819602156047,
131.46611590328)) ;
#127501=CARTESIAN_POINT('Ctrl Pts',(-19.8763877159582,14.5692454320411,
131.169609312389)) ;
#127502=CARTESIAN_POINT('Ctrl Pts',(-19.7902646702084,14.4742854665662,
130.884826946412)) ;
#127503=CARTESIAN_POINT('Ctrl Pts',(-19.7161283689557,14.3047439211162,
130.635239983571)) ;
#127504=CARTESIAN_POINT('Ctrl Pts',(-19.6592322243353,14.0710831127117,
130.435827411304)) ;
#127505=CARTESIAN_POINT('Ctrl Pts',(-19.62494311501,13.7914036460412,130.302538232877)) ;
#127506=CARTESIAN_POINT('Ctrl Pts',(-19.6162934482715,13.4850123175133,
130.244106124328)) ;
#127507=CARTESIAN_POINT('Ctrl Pts',(-19.6344889863082,13.1755843986706,
130.264253212252)) ;
#127508=CARTESIAN_POINT('Ctrl Pts',(-19.6791913673902,12.8823157698566,
130.361653440408)) ;
#127509=CARTESIAN_POINT('Ctrl Pts',(-19.7476537533918,12.628436297888,130.528560046345)) ;
#127510=CARTESIAN_POINT('Ctrl Pts',(-19.8365476312442,12.4304595196238,
130.754910983151)) ;
#127511=CARTESIAN_POINT('Ctrl Pts',(-19.9382808494003,12.3053999531995,
131.019209738796)) ;
#127512=CARTESIAN_POINT('Ctrl Pts',(-20.048899562009,12.2593484395974,131.309018103742)) ;
#127513=CARTESIAN_POINT('Ctrl Pts',(-20.1583951299693,12.2965483924972,
131.596013137775)) ;
#127514=CARTESIAN_POINT('Ctrl Pts',(-20.2627239903333,12.4156949312687,
131.86738401474)) ;
#127515=CARTESIAN_POINT('Ctrl Pts',(-20.3521217577948,12.6050470802083,
132.095633239782)) ;
#127516=CARTESIAN_POINT('Ctrl Pts',(-20.4232557357957,12.8553420969347,
132.270128746928)) ;
#127517=CARTESIAN_POINT('Ctrl Pts',(-20.4701295915053,13.14294545291,132.374185521651)) ;
#127518=CARTESIAN_POINT('Ctrl Pts',(-20.4913439775976,13.4543916932758,
132.402838218576)) ;
#127519=CARTESIAN_POINT('Ctrl Pts',(-20.4852807985954,13.7614619882681,
132.352049896115)) ;
#127520=CARTESIAN_POINT('Ctrl Pts',(-20.4534599308289,14.0447128123048,
132.225967144145)) ;
#127521=CARTESIAN_POINT('Ctrl Pts',(-20.3989422258876,14.2828872878416,
132.033662002677)) ;
#127522=CARTESIAN_POINT('Ctrl Pts',(-20.3261747565817,14.4603132279032,
131.78796988944)) ;
#127523=CARTESIAN_POINT('Ctrl Pts',(-20.2406405035968,14.5634617408265,
131.504807990948)) ;
#127524=CARTESIAN_POINT('Ctrl Pts',(-20.1506934552704,14.5844329912441,
131.209131937478)) ;
#127525=CARTESIAN_POINT('Ctrl Pts',(-20.0617033623463,14.5225343527704,
130.915946521996)) ;
#127526=CARTESIAN_POINT('Ctrl Pts',(-19.9818420485813,14.3815448492318,
130.649512810055)) ;
#127527=CARTESIAN_POINT('Ctrl Pts',(-19.917408267804,14.172575531033,130.428222467957)) ;
#127528=CARTESIAN_POINT('Ctrl Pts',(-19.8735004975879,13.9093041266096,
130.266803762146)) ;
#127529=CARTESIAN_POINT('Ctrl Pts',(-19.8541245956283,13.6121559231782,
130.177157387992)) ;
#127530=CARTESIAN_POINT('Ctrl Pts',(-19.8614969291783,13.2990171970743,
130.165379607394)) ;
#127531=CARTESIAN_POINT('Ctrl Pts',(-19.8955170588464,12.998156604328,130.231820441278)) ;
#127532=CARTESIAN_POINT('Ctrl Pts',(-19.9547262808423,12.7257033246492,
130.371637346986)) ;
#127533=CARTESIAN_POINT('Ctrl Pts',(-20.0358807184934,12.5030758718665,
130.57549131059)) ;
#127534=CARTESIAN_POINT('Ctrl Pts',(-20.1330736628754,12.3471530104355,
130.826374526737)) ;
#127535=CARTESIAN_POINT('Ctrl Pts',(-20.2413837044624,12.2678408684918,
131.109474408019)) ;
#127536=CARTESIAN_POINT('Ctrl Pts',(-20.3516515581445,12.2715869144481,
131.398702136902)) ;
#127537=CARTESIAN_POINT('Ctrl Pts',(-20.458990666618,12.3575775842601,131.679074390523)) ;
#127538=CARTESIAN_POINT('Ctrl Pts',(-20.5551532672935,12.5198591790598,
131.926895826603)) ;
#127539=CARTESIAN_POINT('Ctrl Pts',(-20.6345267118374,12.7472700388984,
132.125583684159)) ;
#127540=CARTESIAN_POINT('Ctrl Pts',(-20.6917801462354,13.0233714187906,
132.259655378351)) ;
#127541=CARTESIAN_POINT('Ctrl Pts',(-20.7235068742326,13.3264774895314,
132.319332952291)) ;
#127542=CARTESIAN_POINT('Ctrl Pts',(-20.7285581739825,13.6374828806093,
132.300975805749)) ;
#127543=CARTESIAN_POINT('Ctrl Pts',(-20.7069127156367,13.9340522489258,
132.204521708848)) ;
#127544=CARTESIAN_POINT('Ctrl Pts',(-20.6610511580448,14.1931239362593,
132.037428877366)) ;
#127545=CARTESIAN_POINT('Ctrl Pts',(-20.5947281122293,14.3974304653898,
131.810470473005)) ;
#127546=CARTESIAN_POINT('Ctrl Pts',(-20.5141569428622,14.5309245418109,
131.542118712394)) ;
#127547=CARTESIAN_POINT('Ctrl Pts',(-20.4250014415483,14.5859814534191,
131.248544133556)) ;
#127548=CARTESIAN_POINT('Ctrl Pts',(-20.3346292234116,14.5574777864012,
130.951397195989)) ;
#127549=CARTESIAN_POINT('Ctrl Pts',(-20.2504020006507,14.448015060185,130.672253823311)) ;
#127550=CARTESIAN_POINT('Ctrl Pts',(-20.1787236467894,14.2640746959558,
130.429615415799)) ;
#127551=CARTESIAN_POINT('Ctrl Pts',(-20.1261893612446,14.0222278715719,
130.243229810785)) ;
#127552=CARTESIAN_POINT('Ctrl Pts',(-20.0963035511799,13.733909228241,130.12255396145)) ;
#127553=CARTESIAN_POINT('Ctrl Pts',(-20.0928006031125,13.4264443346404,
130.079328393741)) ;
#127554=CARTESIAN_POINT('Ctrl Pts',(-20.1160876756408,13.1179337320863,
130.114262614734)) ;
#127555=CARTESIAN_POINT('Ctrl Pts',(-20.1654886895204,12.8308236550973,
130.225443140224)) ;
#127556=CARTESIAN_POINT('Ctrl Pts',(-20.2383169541712,12.5859821218942,
130.405007728628)) ;
#127557=CARTESIAN_POINT('Ctrl Pts',(-20.3293570118732,12.4020104650746,
130.637967599986)) ;
#127558=CARTESIAN_POINT('Ctrl Pts',(-20.4343040706677,12.289987565929,130.911234342623)) ;
#127559=CARTESIAN_POINT('Ctrl Pts',(-20.5445367265671,12.2601247779834,
131.20023242097)) ;
#127560=CARTESIAN_POINT('Ctrl Pts',(-20.6540586635509,12.3130229005744,
131.487063615784)) ;
#127561=CARTESIAN_POINT('Ctrl Pts',(-20.7555473479129,12.4457555473525,
131.750394826563)) ;
#127562=CARTESIAN_POINT('Ctrl Pts',(-20.8422236062708,12.6478748794645,
131.970533838524)) ;
#127563=CARTESIAN_POINT('Ctrl Pts',(-20.9091717846165,12.9074235012635,
132.132805273435)) ;
#127564=CARTESIAN_POINT('Ctrl Pts',(-20.9513915274105,13.2015879263547,
132.223135875189)) ;
#127565=CARTESIAN_POINT('Ctrl Pts',(-20.9673433799513,13.5132462059268,
132.23653666469)) ;
#127566=CARTESIAN_POINT('Ctrl Pts',(-20.9563186950524,13.8170404321959,
132.171290910233)) ;
#127567=CARTESIAN_POINT('Ctrl Pts',(-20.9200063586161,14.0930904001558,
132.032130174702)) ;
#127568=CARTESIAN_POINT('Ctrl Pts',(-20.8615797598591,14.3215764972773,
131.828327874227)) ;
#127569=CARTESIAN_POINT('Ctrl Pts',(-20.7857303358652,14.4860164278212,
131.573530686186)) ;
#127570=CARTESIAN_POINT('Ctrl Pts',(-20.6990544102765,14.573742198897,131.287198957879)) ;
#127571=CARTESIAN_POINT('Ctrl Pts',(-20.6082663915268,14.5789283396522,
130.988830774591)) ;
#127572=CARTESIAN_POINT('Ctrl Pts',(-20.5209618564176,14.5018180377366,
130.700774166513)) ;
#127573=CARTESIAN_POINT('Ctrl Pts',(-20.4433002769759,14.346557147794,130.440665580027)) ;
#127574=CARTESIAN_POINT('Ctrl Pts',(-20.3826208374421,14.1268974997841,
130.23046053949)) ;
#127575=CARTESIAN_POINT('Ctrl Pts',(-20.3429550525631,13.8551172342444,
130.081370374509)) ;
#127576=CARTESIAN_POINT('Ctrl Pts',(-20.3285617380619,13.5530513946411,
130.006211437284)) ;
#127577=CARTESIAN_POINT('Ctrl Pts',(-20.3409618342516,13.2415864711832,
130.009305157595)) ;
#127578=CARTESIAN_POINT('Ctrl Pts',(-20.3800377984526,12.9431697313624,
130.090333860656)) ;
#127579=CARTESIAN_POINT('Ctrl Pts',(-20.4437605734203,12.6789856337564,
130.243341345209)) ;
#127580=CARTESIAN_POINT('Ctrl Pts',(-20.5281215425679,12.4685393883903,
130.456694343348)) ;
#127581=CARTESIAN_POINT('Ctrl Pts',(-20.6278006359466,12.3261974816525,
130.714816569821)) ;
#127582=CARTESIAN_POINT('Ctrl Pts',(-20.7371171183746,12.2622045903834,
131.000906852494)) ;
#127583=CARTESIAN_POINT('Ctrl Pts',(-20.8475355906631,12.2815898228841,
131.29047054978)) ;
#127584=CARTESIAN_POINT('Ctrl Pts',(-20.9531780974456,12.3824517560788,
131.565944042244)) ;
#127585=CARTESIAN_POINT('Ctrl Pts',(-21.0468252428417,12.5585396734663,
131.806317421495)) ;
#127586=CARTESIAN_POINT('Ctrl Pts',(-21.1220933065646,12.7954954768117,
131.993149661609)) ;
#127587=CARTESIAN_POINT('Ctrl Pts',(-21.1749898652116,13.0796939956766,
132.114357782116)) ;
#127588=CARTESIAN_POINT('Ctrl Pts',(-21.2016446674372,13.3852304275537,
132.159287548806)) ;
#127589=CARTESIAN_POINT('Ctrl Pts',(-21.2015540163802,13.6960444491442,
132.125795477662)) ;
#127590=CARTESIAN_POINT('Ctrl Pts',(-21.1751743778786,13.9858667293059,
132.015671444373)) ;
#127591=CARTESIAN_POINT('Ctrl Pts',(-21.1251728129277,14.2358877355362,
131.836479960103)) ;
#127592=CARTESIAN_POINT('Ctrl Pts',(-21.0559870451211,14.4275999351318,
131.601303111379)) ;
#127593=CARTESIAN_POINT('Ctrl Pts',(-20.9724777469102,14.5480862866817,
131.324017047238)) ;
#127594=CARTESIAN_POINT('Ctrl Pts',(-20.8828738981426,14.5868446716621,
131.029266002422)) ;
#127595=CARTESIAN_POINT('Ctrl Pts',(-20.793319864488,14.5430357669594,130.734593108709)) ;
#127596=CARTESIAN_POINT('Ctrl Pts',(-20.7108832857753,14.4187440206734,
130.460625240054)) ;
#127597=CARTESIAN_POINT('Ctrl Pts',(-20.6424522460287,14.2230681613756,
130.227576513237)) ;
#127598=CARTESIAN_POINT('Ctrl Pts',(-20.5936752517832,13.9697197628044,
130.05191339845)) ;
#127599=CARTESIAN_POINT('Ctrl Pts',(-20.5688082976389,13.6787523584359,
129.946270287874)) ;
#127600=CARTESIAN_POINT('Ctrl Pts',(-20.5702148377031,13.3668523124778,
129.917087134561)) ;
#127601=CARTESIAN_POINT('Ctrl Pts',(-20.5987307960509,13.0606725090592,
129.967279841455)) ;
#127602=CARTESIAN_POINT('Ctrl Pts',(-20.6526299718924,12.7810811423454,
130.091709533223)) ;
#127603=CARTESIAN_POINT('Ctrl Pts',(-20.7291627181641,12.5467077639777,
130.282168756974)) ;
#127604=CARTESIAN_POINT('Ctrl Pts',(-20.8232989589554,12.3750360607571,
130.524096085743)) ;
#127605=CARTESIAN_POINT('Ctrl Pts',(-20.9301073743537,12.2779852511976,
130.802757831994)) ;
#127606=CARTESIAN_POINT('Ctrl Pts',(-21.0403994395651,12.2637459485192,
131.092020590387)) ;
#127607=CARTESIAN_POINT('Ctrl Pts',(-21.1491494132192,12.3321871592446,
131.376524953412)) ;
#127608=CARTESIAN_POINT('Ctrl Pts',(-21.2482582669085,12.4786899759448,
131.632949826684)) ;
#127609=CARTESIAN_POINT('Ctrl Pts',(-21.3319658991696,12.6941598777831,
131.84419829175)) ;
#127610=CARTESIAN_POINT('Ctrl Pts',(-21.393934752169,12.9594897352697,131.992273232436)) ;
#127611=CARTESIAN_POINT('Ctrl Pts',(-21.4316059764268,13.2597801817525,
132.06913270801)) ;
#127612=CARTESIAN_POINT('Ctrl Pts',(-21.4423915229943,13.5705932837916,
132.067589188532)) ;
#127613=CARTESIAN_POINT('Ctrl Pts',(-21.4265327050768,13.8717554022753,
131.988120022536)) ;
#127614=CARTESIAN_POINT('Ctrl Pts',(-21.3853703707677,14.1416796116284,
131.834580510575)) ;
#127615=CARTESIAN_POINT('Ctrl Pts',(-21.3236598644603,14.3575208228019,
131.621411940782)) ;
#127616=CARTESIAN_POINT('Ctrl Pts',(-21.2450552710407,14.5088742490897,
131.358477246909)) ;
#127617=CARTESIAN_POINT('Ctrl Pts',(-21.1571003571,14.5810485839828,131.068431346942)) ;
#127618=CARTESIAN_POINT('Ctrl Pts',(-21.0667207705511,14.57070182657,130.771389000615)) ;
#127619=CARTESIAN_POINT('Ctrl Pts',(-20.9806138390254,14.4785662715794,
130.486765690707)) ;
#127620=CARTESIAN_POINT('Ctrl Pts',(-20.9054510209352,14.3096046389662,
130.233904652389)) ;
#127621=CARTESIAN_POINT('Ctrl Pts',(-20.8482642268115,14.0777450263891,
130.033732777931)) ;
#127622=CARTESIAN_POINT('Ctrl Pts',(-20.8134138256627,13.8001342055984,
129.898917449703)) ;
#127623=CARTESIAN_POINT('Ctrl Pts',(-20.8039194104589,13.4946153250832,
129.838060557703)) ;
#127624=CARTESIAN_POINT('Ctrl Pts',(-20.8214390457908,13.1837407036183,
129.856093267552)) ;
#127625=CARTESIAN_POINT('Ctrl Pts',(-20.8653324231382,12.8901082598339,
129.951191666946)) ;
#127626=CARTESIAN_POINT('Ctrl Pts',(-20.9336506448477,12.6339160902113,
130.117500460749)) ;
#127627=CARTESIAN_POINT('Ctrl Pts',(-21.0207516195137,12.4365925755612,
130.339087571425)) ;
#127628=CARTESIAN_POINT('Ctrl Pts',(-21.1233219210523,12.3075969620248,
130.605430834854)) ;
#127629=CARTESIAN_POINT('Ctrl Pts',(-21.2328407338124,12.2595413696365,
130.892337856127)) ;
#127630=CARTESIAN_POINT('Ctrl Pts',(-21.3434469460394,12.294598124244,131.182256793643)) ;
#127631=CARTESIAN_POINT('Ctrl Pts',(-21.4469834297355,12.4101972582257,
131.451676254649)) ;
#127632=CARTESIAN_POINT('Ctrl Pts',(-21.537599854355,12.5987159467278,131.683227158455)) ;
#127633=CARTESIAN_POINT('Ctrl Pts',(-21.6090537188666,12.8461743732165,
131.858838519072)) ;
#127634=CARTESIAN_POINT('Ctrl Pts',(-21.6571326896814,13.1359262373299,
131.96605982225)) ;
#127635=CARTESIAN_POINT('Ctrl Pts',(-21.6788474695644,13.4447581486374,
131.996439162296)) ;
#127636=CARTESIAN_POINT('Ctrl Pts',(-21.673602265646,13.7530929107791,131.947938343351)) ;
#127637=CARTESIAN_POINT('Ctrl Pts',(-21.6426240443624,14.0362080368137,
131.824455207463)) ;
#127638=CARTESIAN_POINT('Ctrl Pts',(-21.5886001898267,14.2769559920641,
131.633477987096)) ;
#127639=CARTESIAN_POINT('Ctrl Pts',(-21.5160865529743,14.4563581826417,
131.388470091183)) ;
#127640=CARTESIAN_POINT('Ctrl Pts',(-21.431392796522,14.5613193473425,131.107980334053)) ;
#127641=CARTESIAN_POINT('Ctrl Pts',(-21.3409007771702,14.5851466761501,
130.810490619039)) ;
#127642=CARTESIAN_POINT('Ctrl Pts',(-21.2517127735891,14.5250094388502,
130.516696471002)) ;
#127643=CARTESIAN_POINT('Ctrl Pts',(-21.1719209058277,14.3871119239881,
130.250653678118)) ;
#127644=CARTESIAN_POINT('Ctrl Pts',(-21.1066172396742,14.1786613718342,
130.026624221542)) ;
#127645=CARTESIAN_POINT('Ctrl Pts',(-21.0622775095093,13.9181922141156,
129.864140105175)) ;
#127646=CARTESIAN_POINT('Ctrl Pts',(-21.0420566901638,13.6189923508217,
129.771715761541)) ;
#127647=CARTESIAN_POINT('Ctrl Pts',(-21.0486722738493,13.3089361907061,
129.758056012422)) ;
#127648=CARTESIAN_POINT('Ctrl Pts',(-21.0820016252292,13.0058325903369,
129.822298008375)) ;
#127649=CARTESIAN_POINT('Ctrl Pts',(-21.1407902952181,12.7318652754408,
129.960821602405)) ;
#127650=CARTESIAN_POINT('Ctrl Pts',(-21.2212926096035,12.5082426893396,
130.162837341344)) ;
#127651=CARTESIAN_POINT('Ctrl Pts',(-21.3177723068254,12.3508732586718,
130.411748644509)) ;
#127652=CARTESIAN_POINT('Ctrl Pts',(-21.4255147925088,12.269103649341,130.693293438078)) ;
#127653=CARTESIAN_POINT('Ctrl Pts',(-21.5363349094351,12.2702137268432,
130.983972752155)) ;
#127654=CARTESIAN_POINT('Ctrl Pts',(-21.6440245158506,12.3542929865281,
131.265319916063)) ;
#127655=CARTESIAN_POINT('Ctrl Pts',(-21.7402989030464,12.5141176451976,
131.513562592344)) ;
#127656=CARTESIAN_POINT('Ctrl Pts',(-21.8201848811006,12.739523408871,131.71378207008)) ;
#127657=CARTESIAN_POINT('Ctrl Pts',(-21.8781683976227,13.0142279275944,
131.850005585261)) ;
#127658=CARTESIAN_POINT('Ctrl Pts',(-21.9107820680664,13.3177662597612,
131.912168548991)) ;
#127659=CARTESIAN_POINT('Ctrl Pts',(-21.9165496071981,13.6286637364164,
131.895925722029)) ;
#127660=CARTESIAN_POINT('Ctrl Pts',(-21.895755349626,13.925291864832,131.802042167994)) ;
#127661=CARTESIAN_POINT('Ctrl Pts',(-21.8505085895,14.1860949701751,131.636697482391)) ;
#127662=CARTESIAN_POINT('Ctrl Pts',(-21.7849733875124,14.39173242129,131.412152981576)) ;
#127663=CARTESIAN_POINT('Ctrl Pts',(-21.704423221989,14.5282787439252,131.143714000168)) ;
#127664=CARTESIAN_POINT('Ctrl Pts',(-21.6152238330637,14.5855538698207,
130.849950873151)) ;
#127665=CARTESIAN_POINT('Ctrl Pts',(-21.5250468841582,14.5594424200451,
130.553468394234)) ;
#127666=CARTESIAN_POINT('Ctrl Pts',(-21.4406201743331,14.4525338341733,
130.273776294927)) ;
#127667=CARTESIAN_POINT('Ctrl Pts',(-21.3683352223517,14.2704301925612,
130.029318459583)) ;
#127668=CARTESIAN_POINT('Ctrl Pts',(-21.3151538916505,14.029440480781,129.840972115584)) ;
#127669=CARTESIAN_POINT('Ctrl Pts',(-21.2846746834487,13.743952252976,129.718772593527)) ;
#127670=CARTESIAN_POINT('Ctrl Pts',(-21.2802918665529,13.4354033018238,
129.672814580744)) ;
#127671=CARTESIAN_POINT('Ctrl Pts',(-21.3027839973428,13.1268757888795,
129.705465440526)) ;
#127672=CARTESIAN_POINT('Ctrl Pts',(-21.3516511623997,12.8380942338867,
129.814985941014)) ;
#127673=CARTESIAN_POINT('Ctrl Pts',(-21.4234141670206,12.5930207357232,
129.991631283737)) ;
#127674=CARTESIAN_POINT('Ctrl Pts',(-21.5145447970548,12.406038862873,130.224648155705)) ;
#127675=CARTESIAN_POINT('Ctrl Pts',(-21.6183299011303,12.2925312371157,
130.494801725081)) ;
#127676=CARTESIAN_POINT('Ctrl Pts',(-21.729396915745,12.2597001754449,130.785954171696)) ;
#127677=CARTESIAN_POINT('Ctrl Pts',(-21.8388056410497,12.3104428537015,
131.072530147179)) ;
#127678=CARTESIAN_POINT('Ctrl Pts',(-21.9407275385059,12.4411375499462,
131.337087912855)) ;
#127679=CARTESIAN_POINT('Ctrl Pts',(-22.0276878186148,12.6410412531594,
131.558133447522)) ;
#127680=CARTESIAN_POINT('Ctrl Pts',(-22.0953288876102,12.8990709835383,
131.722434059242)) ;
#127681=CARTESIAN_POINT('Ctrl Pts',(-22.1383620574179,13.1932158971754,
131.815059128077)) ;
#127682=CARTESIAN_POINT('Ctrl Pts',(-22.155034431918,13.5039483796779,131.830649183986)) ;
#127683=CARTESIAN_POINT('Ctrl Pts',(-22.1448038549081,13.8084630012421,
131.767699528723)) ;
#127684=CARTESIAN_POINT('Ctrl Pts',(-22.109186119241,14.0856215177356,131.630569916654)) ;
#127685=CARTESIAN_POINT('Ctrl Pts',(-22.0513385084274,14.3156974280267,
131.428460450475)) ;
#127686=CARTESIAN_POINT('Ctrl Pts',(-21.9760632390203,14.4820692905758,
131.175400152384)) ;
#127687=CARTESIAN_POINT('Ctrl Pts',(-21.8894445481827,14.5722583385509,
130.88916664676)) ;
#127688=CARTESIAN_POINT('Ctrl Pts',(-21.7991282105243,14.5801736907429,
130.592348168938)) ;
#127689=CARTESIAN_POINT('Ctrl Pts',(-21.7109828267676,14.5050113905237,
130.301588988458)) ;
#127690=CARTESIAN_POINT('Ctrl Pts',(-21.6332169174199,14.3522165397239,
130.04129242342)) ;
#127691=CARTESIAN_POINT('Ctrl Pts',(-21.5718716896646,14.1339603470577,
129.829082114643)) ;
#127692=CARTESIAN_POINT('Ctrl Pts',(-21.5316011710367,13.8641113715177,
129.678314299176)) ;
#127693=CARTESIAN_POINT('Ctrl Pts',(-21.516371458328,13.5616226074544,129.600594418002)) ;
#127694=CARTESIAN_POINT('Ctrl Pts',(-21.528026070481,13.2502935266874,129.601533510366)) ;
#127695=CARTESIAN_POINT('Ctrl Pts',(-21.5664271373857,12.9509783477542,
129.680559417768)) ;
#127696=CARTESIAN_POINT('Ctrl Pts',(-21.6292751697968,12.686394956267,129.831121353527)) ;
#127697=CARTESIAN_POINT('Ctrl Pts',(-21.71326832387,12.4734606665479,130.043316396619)) ;
#127698=CARTESIAN_POINT('Ctrl Pts',(-21.81304630685,12.3287824012662,130.301595784484)) ;
#127699=CARTESIAN_POINT('Ctrl Pts',(-21.9216720916824,12.2629634134795,
130.585834457607)) ;
#127700=CARTESIAN_POINT('Ctrl Pts',(-22.0323190208263,12.2798963226628,
130.87600840922)) ;
#127701=CARTESIAN_POINT('Ctrl Pts',(-22.1382631328561,12.3786943874465,
131.152344623819)) ;
#127702=CARTESIAN_POINT('Ctrl Pts',(-22.2324381892803,12.5532637132079,
131.394210928517)) ;
#127703=CARTESIAN_POINT('Ctrl Pts',(-22.307930733872,12.7879391796142,131.581823885359)) ;
#127704=CARTESIAN_POINT('Ctrl Pts',(-22.3614093552365,13.0695371271683,
131.704894335283)) ;
#127705=CARTESIAN_POINT('Ctrl Pts',(-22.3890801459065,13.3764287043337,
131.752596913402)) ;
#127706=CARTESIAN_POINT('Ctrl Pts',(-22.3896950038745,13.6873693766845,
131.72117697511)) ;
#127707=CARTESIAN_POINT('Ctrl Pts',(-22.3640937155925,13.9780097436375,
131.613337884262)) ;
#127708=CARTESIAN_POINT('Ctrl Pts',(-22.3144461748257,14.2303816884254,
131.435040211327)) ;
#127709=CARTESIAN_POINT('Ctrl Pts',(-22.2459325294148,14.4229832272402,
131.201951144948)) ;
#127710=CARTESIAN_POINT('Ctrl Pts',(-22.1629423958746,14.5456071982134,
130.926254854072)) ;
#127711=CARTESIAN_POINT('Ctrl Pts',(-22.0732786583332,14.5869244372791,
130.631268978178)) ;
#127712=CARTESIAN_POINT('Ctrl Pts',(-21.9835550064987,14.5454139986495,
130.336078615688)) ;
#127713=CARTESIAN_POINT('Ctrl Pts',(-21.9007965838892,14.423161531977,130.061157179146)) ;
#127714=CARTESIAN_POINT('Ctrl Pts',(-21.8320921977162,14.2299646036066,
129.827410664978)) ;
#127715=CARTESIAN_POINT('Ctrl Pts',(-21.7825910759239,13.9782380445369,
129.64963445589)) ;
#127716=CARTESIAN_POINT('Ctrl Pts',(-21.7569463800142,13.6869896878631,
129.541595864683)) ;
#127717=CARTESIAN_POINT('Ctrl Pts',(-21.7575526251693,13.3772462538757,
129.510281572766)) ;
#127718=CARTESIAN_POINT('Ctrl Pts',(-21.7851625426909,13.0701026679002,
129.557778994613)) ;
#127719=CARTESIAN_POINT('Ctrl Pts',(-21.838567285868,12.7883758090077,129.680637101522)) ;
#127720=CARTESIAN_POINT('Ctrl Pts',(-21.9145185360536,12.5524788411572,
129.869403118959)) ;
#127721=CARTESIAN_POINT('Ctrl Pts',(-22.008423797552,12.3787206196838,130.11059742698)) ;
#127722=CARTESIAN_POINT('Ctrl Pts',(-22.1143427284911,12.2799428497071,
130.386861315047)) ;
#127723=CARTESIAN_POINT('Ctrl Pts',(-22.2248374459482,12.262781441409,130.676641434297)) ;
#127724=CARTESIAN_POINT('Ctrl Pts',(-22.3343454192335,12.3295044155471,
130.963177642968)) ;
#127725=CARTESIAN_POINT('Ctrl Pts',(-22.4332832043384,12.4735104244077,
131.219259972441)) ;
#127726=CARTESIAN_POINT('Ctrl Pts',(-22.5172516297272,12.6859035463297,
131.431419830921)) ;
#127727=CARTESIAN_POINT('Ctrl Pts',(-22.5802700498489,12.9511127833356,
131.58240078474)) ;
#127728=CARTESIAN_POINT('Ctrl Pts',(-22.6186978514235,13.2510041848706,
131.661446782256)) ;
#127729=CARTESIAN_POINT('Ctrl Pts',(-22.6302490272601,13.5624347972365,
131.662072128067)) ;
#127730=CARTESIAN_POINT('Ctrl Pts',(-22.6150771567607,13.8634350892771,
131.584681894005)) ;
#127731=CARTESIAN_POINT('Ctrl Pts',(-22.5749490142225,14.1332613456827,
131.434354396493)) ;
#127732=CARTESIAN_POINT('Ctrl Pts',(-22.5133593020274,14.352640956948,131.221284043712)) ;
#127733=CARTESIAN_POINT('Ctrl Pts',(-22.4352729860133,14.5054039533886,
130.959949323257)) ;
#127734=CARTESIAN_POINT('Ctrl Pts',(-22.3478811125609,14.5799567622948,
130.671675925426)) ;
#127735=CARTESIAN_POINT('Ctrl Pts',(-22.2571262594832,14.5723714233898,
130.373415016701)) ;
#127736=CARTESIAN_POINT('Ctrl Pts',(-22.1705066821009,14.4818104569399,
130.087167993693)) ;
#127737=CARTESIAN_POINT('Ctrl Pts',(-22.0955412959604,14.3163443098713,
129.835162366206)) ;
#127738=CARTESIAN_POINT('Ctrl Pts',(-22.0375088402051,14.085912079338,129.632435530077)) ;
#127739=CARTESIAN_POINT('Ctrl Pts',(-22.0018499381263,13.8088758328653,
129.495197588548)) ;
#127740=CARTESIAN_POINT('Ctrl Pts',(-21.9916250136062,13.502841633218,129.432098950623)) ;
#127741=CARTESIAN_POINT('Ctrl Pts',(-22.0082934021031,13.1931031291703,
129.447788449584)) ;
#127742=CARTESIAN_POINT('Ctrl Pts',(-22.0515574069593,12.8979592502217,
129.540960648325)) ;
#127743=CARTESIAN_POINT('Ctrl Pts',(-22.1188207375362,12.6415806855276,
129.704364437549)) ;
#127744=CARTESIAN_POINT('Ctrl Pts',(-22.2060107640497,12.4408172190554,
129.925969921115)) ;
#127745=CARTESIAN_POINT('Ctrl Pts',(-22.3082900601043,12.3100401605785,
130.191475830034)) ;
#127746=CARTESIAN_POINT('Ctrl Pts',(-22.4174544888081,12.2598615755304,
130.477414065444)) ;
#127747=CARTESIAN_POINT('Ctrl Pts',(-22.527907294651,12.2922205439251,130.766961293267)) ;
#127748=CARTESIAN_POINT('Ctrl Pts',(-22.6322782382144,12.4062484936796,
131.038640430295)) ;
#127749=CARTESIAN_POINT('Ctrl Pts',(-22.7231027875419,12.5927140648452,
131.270873729385)) ;
#127750=CARTESIAN_POINT('Ctrl Pts',(-22.7949984498098,12.8381488980971,
131.447846084438)) ;
#127751=CARTESIAN_POINT('Ctrl Pts',(-22.843787932828,13.1260095389923,131.557242126977)) ;
#127752=CARTESIAN_POINT('Ctrl Pts',(-22.8664230727776,13.4367097243977,
131.590076325101)) ;
#127753=CARTESIAN_POINT('Ctrl Pts',(-22.861921411388,13.7438376738668,131.543917878659)) ;
#127754=CARTESIAN_POINT('Ctrl Pts',(-22.8316397070447,14.0287736481255,
131.42237783867)) ;
#127755=CARTESIAN_POINT('Ctrl Pts',(-22.778155770167,14.2709621687312,131.232973634128)) ;
#127756=CARTESIAN_POINT('Ctrl Pts',(-22.7062333019467,14.4520607897228,
130.989750404344)) ;
#127757=CARTESIAN_POINT('Ctrl Pts',(-22.6216704946962,14.5594794390157,
130.709590559647)) ;
#127758=CARTESIAN_POINT('Ctrl Pts',(-22.5314212575681,14.5855261762896,
130.412873670548)) ;
#127759=CARTESIAN_POINT('Ctrl Pts',(-22.4422960022349,14.5283738832722,
130.119356279925)) ;
#127760=CARTESIAN_POINT('Ctrl Pts',(-22.3616462327386,14.391653643749,129.850584082527)) ;
#127761=CARTESIAN_POINT('Ctrl Pts',(-22.2962167251037,14.1863633435458,
129.626404074533)) ;
#127762=CARTESIAN_POINT('Ctrl Pts',(-22.2509351230502,13.9255968705726,
129.460952363105)) ;
#127763=CARTESIAN_POINT('Ctrl Pts',(-22.230115271223,13.6292801101744,129.367025070917)) ;
#127764=CARTESIAN_POINT('Ctrl Pts',(-22.2358443462118,13.3179690043923,
129.350624868831)) ;
#127765=CARTESIAN_POINT('Ctrl Pts',(-22.268461938418,13.0144329118731,129.412800062026)) ;
#127766=CARTESIAN_POINT('Ctrl Pts',(-22.3263092006397,12.7401667840787,
129.548682574508)) ;
#127767=CARTESIAN_POINT('Ctrl Pts',(-22.4061509855269,12.5144107338462,
129.748760348764)) ;
#127768=CARTESIAN_POINT('Ctrl Pts',(-22.5028521991577,12.3540784671315,
129.998111153004)) ;
#127769=CARTESIAN_POINT('Ctrl Pts',(-22.6098851930669,12.2704506823876,
130.277743640538)) ;
#127770=CARTESIAN_POINT('Ctrl Pts',(-22.7210593635,12.2689820893059,130.569348124059)) ;
#127771=CARTESIAN_POINT('Ctrl Pts',(-22.8288745913513,12.3508509488233,
130.85108559455)) ;
#127772=CARTESIAN_POINT('Ctrl Pts',(-22.9255783208102,12.5086055311564,
131.100573560609)) ;
#127773=CARTESIAN_POINT('Ctrl Pts',(-23.0062047553353,12.7330676993537,
131.302868223054)) ;
#127774=CARTESIAN_POINT('Ctrl Pts',(-23.0647146527384,13.0066123960221,
131.440652814153)) ;
#127775=CARTESIAN_POINT('Ctrl Pts',(-23.0979542086672,13.3082725062707,
131.504787867336)) ;
#127776=CARTESIAN_POINT('Ctrl Pts',(-23.1045786952682,13.6201712444572,
131.490952868656)) ;
#127777=CARTESIAN_POINT('Ctrl Pts',(-23.0843643957598,13.9183340301052,
131.39866546306)) ;
#127778=CARTESIAN_POINT('Ctrl Pts',(-23.0397557463822,14.1797387715242,
131.235247293697)) ;
#127779=CARTESIAN_POINT('Ctrl Pts',(-22.9749516558702,14.3864986993276,
131.012946095585)) ;
#127780=CARTESIAN_POINT('Ctrl Pts',(-22.8947964654787,14.5252641571149,
130.745671070089)) ;
#127781=CARTESIAN_POINT('Ctrl Pts',(-22.8057244267908,14.5851721018435,
130.452271746797)) ;
#127782=CARTESIAN_POINT('Ctrl Pts',(-22.7149747642661,14.5610669254243,
130.153926197287)) ;
#127783=CARTESIAN_POINT('Ctrl Pts',(-22.6307834813211,14.4566509961662,
129.875100662719)) ;
#127784=CARTESIAN_POINT('Ctrl Pts',(-22.5580747125729,14.2771545373181,
129.629455783231)) ;
#127785=CARTESIAN_POINT('Ctrl Pts',(-22.5040373563515,14.0362065449594,
129.438421285664)) ;
#127786=CARTESIAN_POINT('Ctrl Pts',(-22.4730618127373,13.7533987258428,
129.314975683587)) ;
#127787=CARTESIAN_POINT('Ctrl Pts',(-22.4677748338582,13.4441283625548,
129.266255047909)) ;
#127788=CARTESIAN_POINT('Ctrl Pts',(-22.4897115438146,13.1346408964387,
129.297202552698)) ;
#127789=CARTESIAN_POINT('Ctrl Pts',(-22.5374240746914,12.8470251714903,
129.403602462889)) ;
#127790=CARTESIAN_POINT('Ctrl Pts',(-22.6091262891195,12.5984937845751,
129.579801716748)) ;
#127791=CARTESIAN_POINT('Ctrl Pts',(-22.6993019984946,12.4108688271007,
129.810228777973)) ;
#127792=CARTESIAN_POINT('Ctrl Pts',(-22.8030088050855,12.2946081104034,
130.080071075194)) ;
#127793=CARTESIAN_POINT('Ctrl Pts',(-22.9140804384845,12.2594450538074,
130.371216687278)) ;
#127794=CARTESIAN_POINT('Ctrl Pts',(-23.0236936524705,12.308048143484,130.658359184517)) ;
#127795=CARTESIAN_POINT('Ctrl Pts',(-23.1255992046416,12.4360760888544,
130.922984180032)) ;
#127796=CARTESIAN_POINT('Ctrl Pts',(-23.2132516276065,12.6345258024436,
131.145978362189)) ;
#127797=CARTESIAN_POINT('Ctrl Pts',(-23.2813071846408,12.8902136692482,
131.311612557012)) ;
#127798=CARTESIAN_POINT('Ctrl Pts',(-23.325204251601,13.1836914998379,131.406732048559)) ;
#127799=CARTESIAN_POINT('Ctrl Pts',(-23.3427326214628,13.4943233710872,
131.424816929959)) ;
#127800=CARTESIAN_POINT('Ctrl Pts',(-23.3332319190002,13.8008444309758,
131.363837246129)) ;
#127801=CARTESIAN_POINT('Ctrl Pts',(-23.2980903408811,14.0793169977329,
131.228040467186)) ;
#127802=CARTESIAN_POINT('Ctrl Pts',(-23.2410734955542,14.3098744793808,
131.028516471564)) ;
#127803=CARTESIAN_POINT('Ctrl Pts',(-23.1658736155029,14.4788324369104,
130.775532824613)) ;
#127804=CARTESIAN_POINT('Ctrl Pts',(-23.079898197243,14.5706779961945,130.491349631505)) ;
#127805=CARTESIAN_POINT('Ctrl Pts',(-22.989421112829,14.5811216657767,130.193989675222)) ;
#127806=CARTESIAN_POINT('Ctrl Pts',(-22.9012597147346,14.508299186415,129.903244922961)) ;
#127807=CARTESIAN_POINT('Ctrl Pts',(-22.8231629825048,14.3580058494818,
129.642018923582)) ;
#127808=CARTESIAN_POINT('Ctrl Pts',(-22.7610067688908,14.1405257747425,
129.427299582576)) ;
#127809=CARTESIAN_POINT('Ctrl Pts',(-22.7202146255786,13.8719962112454,
129.275043026832)) ;
#127810=CARTESIAN_POINT('Ctrl Pts',(-22.7042294788993,13.571629068225,129.1952761277)) ;
#127811=CARTESIAN_POINT('Ctrl Pts',(-22.7150970762887,13.2591263892434,
129.193790879608)) ;
#127812=CARTESIAN_POINT('Ctrl Pts',(-22.7526267524281,12.9599152020145,
129.270362472223)) ;
#127813=CARTESIAN_POINT('Ctrl Pts',(-22.8149940316731,12.693080122514,129.419401646017)) ;
#127814=CARTESIAN_POINT('Ctrl Pts',(-22.8983825031158,12.478823817929,129.629876557537)) ;
#127815=CARTESIAN_POINT('Ctrl Pts',(-22.9974758723708,12.3322479297148,
129.886249770476)) ;
#127816=CARTESIAN_POINT('Ctrl Pts',(-23.1060580485817,12.2636849635138,
130.170316728691)) ;
#127817=CARTESIAN_POINT('Ctrl Pts',(-23.2170452381193,12.2782423656434,
130.461397665353)) ;
#127818=CARTESIAN_POINT('Ctrl Pts',(-23.323119274888,12.3748788450642,130.738138642281)) ;
#127819=CARTESIAN_POINT('Ctrl Pts',(-23.4173862913371,12.5463734718221,
130.980420347811)) ;
#127820=CARTESIAN_POINT('Ctrl Pts',(-23.4940244074986,12.7810696504838,
131.171144587366)) ;
#127821=CARTESIAN_POINT('Ctrl Pts',(-23.5479571630979,13.0608633247241,
131.295649840523)) ;
#127822=CARTESIAN_POINT('Ctrl Pts',(-23.5764346562346,13.3671882747387,
131.345715854469)) ;
#127823=CARTESIAN_POINT('Ctrl Pts',(-23.5778620636875,13.6783220863787,
131.316677624504)) ;
#127824=CARTESIAN_POINT('Ctrl Pts',(-23.5529353685211,13.970110064652,131.210766412908)) ;
#127825=CARTESIAN_POINT('Ctrl Pts',(-23.5041893664155,14.223034525395,131.03524141122)) ;
#127826=CARTESIAN_POINT('Ctrl Pts',(-23.4358087814074,14.4186168883369,
130.802357638557)) ;
#127827=CARTESIAN_POINT('Ctrl Pts',(-23.3535062382914,14.5428705869547,
130.528828840875)) ;
#127828=CARTESIAN_POINT('Ctrl Pts',(-23.2637737223295,14.5869069848455,
130.233565716766)) ;
#127829=CARTESIAN_POINT('Ctrl Pts',(-23.1740246734248,14.5480013176435,
129.938339046236)) ;
#127830=CARTESIAN_POINT('Ctrl Pts',(-23.0904931811877,14.4271740770577,
129.660963874949)) ;
#127831=CARTESIAN_POINT('Ctrl Pts',(-23.0216173815687,14.2362638791343,
129.42683436767)) ;
#127832=CARTESIAN_POINT('Ctrl Pts',(-22.97149729033,13.9863048386446,129.247280599084)) ;
#127833=CARTESIAN_POINT('Ctrl Pts',(-22.9451285454645,13.6957298215624,
129.13710573599)) ;
#127834=CARTESIAN_POINT('Ctrl Pts',(-22.9448828449131,13.3866515753752,
129.103351428825)) ;
#127835=CARTESIAN_POINT('Ctrl Pts',(-22.9719981332692,13.0771469727204,
129.149182977873)) ;
#127836=CARTESIAN_POINT('Ctrl Pts',(-23.0243913022096,12.796392103063,129.269316634301)) ;
#127837=CARTESIAN_POINT('Ctrl Pts',(-23.1000578815261,12.5578779370545,
129.457104362804)) ;
#127838=CARTESIAN_POINT('Ctrl Pts',(-23.193168555688,12.383073568111,129.696120245286)) ;
#127839=CARTESIAN_POINT('Ctrl Pts',(-23.2988396055172,12.2815115204251,
129.97164656702)) ;
#127840=CARTESIAN_POINT('Ctrl Pts',(-23.4100862971625,12.2623682395224,
130.263384452453)) ;
#127841=CARTESIAN_POINT('Ctrl Pts',(-23.5183860259816,12.3259184217804,
130.546811307489)) ;
#127842=CARTESIAN_POINT('Ctrl Pts',(-23.6184046272942,12.4680809238775,
130.805840329846)) ;
#127843=CARTESIAN_POINT('Ctrl Pts',(-23.7030502858861,12.6795623120404,
131.019893309845)) ;
#127844=CARTESIAN_POINT('Ctrl Pts',(-23.7664918164668,12.9425894685416,
131.17222579836)) ;
#127845=CARTESIAN_POINT('Ctrl Pts',(-23.8057196011872,13.2417282929866,
131.253609119574)) ;
#127846=CARTESIAN_POINT('Ctrl Pts',(-23.8180970159282,13.5531902629317,
131.25664309866)) ;
#127847=CARTESIAN_POINT('Ctrl Pts',(-23.8036286080686,13.8554128204607,
131.181234076418)) ;
#127848=CARTESIAN_POINT('Ctrl Pts',(-23.7642341023557,14.1261608663375,
131.033092417043)) ;
#127849=CARTESIAN_POINT('Ctrl Pts',(-23.7028856469184,14.3478084668955,
130.820595747378)) ;
#127850=CARTESIAN_POINT('Ctrl Pts',(-23.6259266939486,14.5013886643306,
130.562866353902)) ;
#127851=CARTESIAN_POINT('Ctrl Pts',(-23.5380160909599,14.5792263009218,
130.272795735233)) ;
#127852=CARTESIAN_POINT('Ctrl Pts',(-23.4474366584794,14.5735423327803,
129.975118371017)) ;
#127853=CARTESIAN_POINT('Ctrl Pts',(-23.3608254158504,14.4859392223761,
129.688999940543)) ;
#127854=CARTESIAN_POINT('Ctrl Pts',(-23.2849259341146,14.32102399054,129.434009796257)) ;
#127855=CARTESIAN_POINT('Ctrl Pts',(-23.2267844317318,14.0938129483377,
129.231217994417)) ;
#127856=CARTESIAN_POINT('Ctrl Pts',(-23.1902647637919,13.8165579803482,
129.091295361189)) ;
#127857=CARTESIAN_POINT('Ctrl Pts',(-23.1792948148417,13.5127264652926,
129.026216186509)) ;
#127858=CARTESIAN_POINT('Ctrl Pts',(-23.1954081556563,13.2000971837,129.039978991797)) ;
#127859=CARTESIAN_POINT('Ctrl Pts',(-23.2375272937591,12.9073427141145,
129.130166593091)) ;
#127860=CARTESIAN_POINT('Ctrl Pts',(-23.3044251896452,12.6479572594797,
129.292307415425)) ;
#127861=CARTESIAN_POINT('Ctrl Pts',(-23.3908615355677,12.4461100388149,
129.511823532986)) ;
#127862=CARTESIAN_POINT('Ctrl Pts',(-23.4928607963202,12.3127706272653,
129.776477891717)) ;
#127863=CARTESIAN_POINT('Ctrl Pts',(-23.602008442908,12.2601401090579,130.06233625634)) ;
#127864=CARTESIAN_POINT('Ctrl Pts',(-23.7125630788762,12.2901733213181,
130.352170428386)) ;
#127865=CARTESIAN_POINT('Ctrl Pts',(-23.8170338930274,12.4015833019759,
130.624208061731)) ;
#127866=CARTESIAN_POINT('Ctrl Pts',(-23.9085880633688,12.586648376757,130.858472179333)) ;
#127867=CARTESIAN_POINT('Ctrl Pts',(-23.9810480513961,12.8302723293176,
131.037137178046)) ;
#127868=CARTESIAN_POINT('Ctrl Pts',(-24.0307108386532,13.1192440292328,
131.148863734522)) ;
#127869=CARTESIAN_POINT('Ctrl Pts',(-24.0538260173367,13.4254781947616,
131.183551991699)) ;
#127870=CARTESIAN_POINT('Ctrl Pts',(-24.0502594742195,13.73535968212,131.139866666903)) ;
#127871=CARTESIAN_POINT('Ctrl Pts',(-24.0206309578773,14.0210481979202,
131.020256948829)) ;
#127872=CARTESIAN_POINT('Ctrl Pts',(-23.9677020137862,14.2649914654817,
130.832435384233)) ;
#127873=CARTESIAN_POINT('Ctrl Pts',(-23.8963530256599,14.4476746957159,
130.590949554297)) ;
#127874=CARTESIAN_POINT('Ctrl Pts',(-23.8121017373058,14.5574099985375,
130.311706751319)) ;
#127875=CARTESIAN_POINT('Ctrl Pts',(-23.7218925496199,14.5860647518339,
130.015099966965)) ;
#127876=CARTESIAN_POINT('Ctrl Pts',(-23.6322614174443,14.5307819376324,
129.719958907671)) ;
#127877=CARTESIAN_POINT('Ctrl Pts',(-23.5517321495787,14.3969445347875,
129.451729386716)) ;
#127878=CARTESIAN_POINT('Ctrl Pts',(-23.4855198577195,14.1927449402103,
129.225129973419)) ;
#127879=CARTESIAN_POINT('Ctrl Pts',(-23.439751943325,13.9340124552338,129.058360127469)) ;
#127880=CARTESIAN_POINT('Ctrl Pts',(-23.4181259338223,13.638112171606,128.962032739013)) ;
#127881=CARTESIAN_POINT('Ctrl Pts',(-23.4230787477534,13.3270743083993,
128.94338373326)) ;
#127882=CARTESIAN_POINT('Ctrl Pts',(-23.4549668538357,13.0225106928389,
129.003376011957)) ;
#127883=CARTESIAN_POINT('Ctrl Pts',(-23.5123117766841,12.7468020423806,
129.137735089545)) ;
#127884=CARTESIAN_POINT('Ctrl Pts',(-23.5911924067347,12.520588791344,129.335174272644)) ;
#127885=CARTESIAN_POINT('Ctrl Pts',(-23.6874775426794,12.3578209708367,
129.583292114684)) ;
#127886=CARTESIAN_POINT('Ctrl Pts',(-23.7945910392982,12.2716454872787,
129.863072070572)) ;
#127887=CARTESIAN_POINT('Ctrl Pts',(-23.9056421843192,12.26795429664,130.154349589356)) ;
#127888=CARTESIAN_POINT('Ctrl Pts',(-24.0133024715846,12.3469221787347,
130.435753067591)) ;
#127889=CARTESIAN_POINT('Ctrl Pts',(-24.1107977682431,12.5030898153774,
130.687423495081)) ;
#127890=CARTESIAN_POINT('Ctrl Pts',(-24.1916810620096,12.725018199882,130.890594344483)) ;
#127891=CARTESIAN_POINT('Ctrl Pts',(-24.2510283580468,12.997182809166,131.030820292085)) ;
#127892=CARTESIAN_POINT('Ctrl Pts',(-24.2851967719419,13.2997828332168,
131.097506231202)) ;
#127893=CARTESIAN_POINT('Ctrl Pts',(-24.2925138699755,13.6108910238796,
131.085784821839)) ;
#127894=CARTESIAN_POINT('Ctrl Pts',(-24.2732507948885,13.9087323450299,
130.996403294879)) ;
#127895=CARTESIAN_POINT('Ctrl Pts',(-24.2292529784254,14.1725576107312,
130.834655232453)) ;
#127896=CARTESIAN_POINT('Ctrl Pts',(-24.1648088256482,14.3815587835512,
130.613331131915)) ;
#127897=CARTESIAN_POINT('Ctrl Pts',(-24.0850031771026,14.522329585323,130.34708336163)) ;
#127898=CARTESIAN_POINT('Ctrl Pts',(-23.9963495919697,14.5844939655697,
130.055002294867)) ;
#127899=CARTESIAN_POINT('Ctrl Pts',(-23.9055571285422,14.5631534313931,
129.756539085882)) ;
#127900=CARTESIAN_POINT('Ctrl Pts',(-23.8207486179396,14.4606751117259,
129.475779639024)) ;
#127901=CARTESIAN_POINT('Ctrl Pts',(-23.7476052970787,14.2826954166288,
129.22883457488)) ;
#127902=CARTESIAN_POINT('Ctrl Pts',(-23.6932165752473,14.0447463561046,
129.036960257282)) ;
#127903=CARTESIAN_POINT('Ctrl Pts',(-23.6613458241508,13.7613771216005,
128.9107117013)) ;
#127904=CARTESIAN_POINT('Ctrl Pts',(-23.6553469120595,13.4542323350155,
128.860103266821)) ;
#127905=CARTESIAN_POINT('Ctrl Pts',(-23.6763806836081,13.1437994657192,
128.888346071975)) ;
#127906=CARTESIAN_POINT('Ctrl Pts',(-23.7237152114361,12.8538469194028,
128.993465947334)) ;
#127907=CARTESIAN_POINT('Ctrl Pts',(-23.7944141862397,12.6054873478473,
129.166932874837)) ;
#127908=CARTESIAN_POINT('Ctrl Pts',(-23.8841019581323,12.4153273189239,
129.395903874998)) ;
#127909=CARTESIAN_POINT('Ctrl Pts',(-23.988399633529,12.2964112456076,129.667208190599)) ;
#127910=CARTESIAN_POINT('Ctrl Pts',(-24.0981665990773,12.2594155903617,
129.954911925008)) ;
#127911=CARTESIAN_POINT('Ctrl Pts',(-24.2083351517853,12.3053349430094,
130.24354607889)) ;
#127912=CARTESIAN_POINT('Ctrl Pts',(-24.3105348444765,12.431225904051,130.509039975804)) ;
#127913=CARTESIAN_POINT('Ctrl Pts',(-24.3987955308139,12.6279597128561,
130.733773861238)) ;
#127914=CARTESIAN_POINT('Ctrl Pts',(-24.4674982287085,12.8824932881055,
130.901278513894)) ;
#127915=CARTESIAN_POINT('Ctrl Pts',(-24.5120404655204,13.1745455481659,
130.998350424472)) ;
#127916=CARTESIAN_POINT('Ctrl Pts',(-24.5304051673806,13.4851755770177,
131.018859009724)) ;
#127917=CARTESIAN_POINT('Ctrl Pts',(-24.5216421560698,13.7921379427258,
130.960030715897)) ;
#127918=CARTESIAN_POINT('Ctrl Pts',(-24.4874090511905,14.0710147871215,
130.826992612308)) ;
#127919=CARTESIAN_POINT('Ctrl Pts',(-24.4305784964973,14.3045452092941,
130.627796028043)) ;
#127920=CARTESIAN_POINT('Ctrl Pts',(-24.3565159379346,14.4740866003594,
130.378447984024)) ;
#127921=CARTESIAN_POINT('Ctrl Pts',(-24.2702543034482,14.5693022408221,
130.093202410812)) ;
#127922=CARTESIAN_POINT('Ctrl Pts',(-24.1798204674234,14.5820126324711,
129.79598471706)) ;
#127923=CARTESIAN_POINT('Ctrl Pts',(-24.0912634781252,14.5112271142504,
129.503993434432)) ;
#127924=CARTESIAN_POINT('Ctrl Pts',(-24.0131302168525,14.3635591504594,
129.242799204596)) ;
#127925=CARTESIAN_POINT('Ctrl Pts',(-23.9503807773228,14.147953964214,129.026340635967)) ;
#127926=CARTESIAN_POINT('Ctrl Pts',(-23.9088544481149,13.88065471692,128.871932632537)) ;
#127927=CARTESIAN_POINT('Ctrl Pts',(-23.8920756438526,13.5796273902736,
128.789707331385)) ;
#127928=CARTESIAN_POINT('Ctrl Pts',(-23.9022581492905,13.2675902134212,
128.786271223279)) ;
#127929=CARTESIAN_POINT('Ctrl Pts',(-23.9389132296133,12.9685392965924,
128.860377903106)) ;
#127930=CARTESIAN_POINT('Ctrl Pts',(-24.0006495136898,12.7001827589766,
129.007541244204)) ;
#127931=CARTESIAN_POINT('Ctrl Pts',(-24.0833864908175,12.4843513873254,
129.216152177106)) ;
#127932=CARTESIAN_POINT('Ctrl Pts',(-24.1822650759013,12.3354377885734,
129.471842874753)) ;
#127933=CARTESIAN_POINT('Ctrl Pts',(-24.2903495731683,12.2645466561417,
129.754554666612)) ;
#127934=CARTESIAN_POINT('Ctrl Pts',(-24.4018767251112,12.2767400465521,
130.047057632449)) ;
#127935=CARTESIAN_POINT('Ctrl Pts',(-24.5078077262226,12.3708038942679,
130.323503077836)) ;
#127936=CARTESIAN_POINT('Ctrl Pts',(-24.6026999902857,12.540571419273,130.567539761247)) ;
#127937=CARTESIAN_POINT('Ctrl Pts',(-24.6796997232066,12.7727636471261,
130.759437881883)) ;
#127938=CARTESIAN_POINT('Ctrl Pts',(-24.7347272254126,13.0532482388654,
130.88692702108)) ;
#127939=CARTESIAN_POINT('Ctrl Pts',(-24.7637896702919,13.3594503778047,
130.938680040336)) ;
#127940=CARTESIAN_POINT('Ctrl Pts',(-24.7659951782845,13.6687250636368,
130.912133764155)) ;
#127941=CARTESIAN_POINT('Ctrl Pts',(-24.7417954210052,13.9622484171183,
130.808248655707)) ;
#127942=CARTESIAN_POINT('Ctrl Pts',(-24.6937033542677,14.2163837288721,
130.634658424453)) ;
#127943=CARTESIAN_POINT('Ctrl Pts',(-24.6256339881966,14.4143549429609,
130.402596636616)) ;
#127944=CARTESIAN_POINT('Ctrl Pts',(-24.5436158358015,14.5404303833534,
130.12990348296)) ;
#127945=CARTESIAN_POINT('Ctrl Pts',(-24.4543794560575,14.5868747915152,
129.836232596245)) ;
#127946=CARTESIAN_POINT('Ctrl Pts',(-24.3640228701984,14.5499212466532,
129.539030418213)) ;
#127947=CARTESIAN_POINT('Ctrl Pts',(-24.280896141805,14.4324626296397,129.263132296661)) ;
#127948=CARTESIAN_POINT('Ctrl Pts',(-24.2108898214641,14.2419356946445,
129.025401963845)) ;
#127949=CARTESIAN_POINT('Ctrl Pts',(-24.1604214713888,13.9939564786199,
128.844943866652)) ;
#127950=CARTESIAN_POINT('Ctrl Pts',(-24.1332885043249,13.7043181806052,
128.732534256686)) ;
#127951=CARTESIAN_POINT('Ctrl Pts',(-24.1323414963115,13.3953697990708,
128.696719141255)) ;
#127952=CARTESIAN_POINT('Ctrl Pts',(-24.158488653808,13.0868083993376,128.739872370214)) ;
#127953=CARTESIAN_POINT('Ctrl Pts',(-24.2104044223131,12.8035341762303,
128.858438904681)) ;
#127954=CARTESIAN_POINT('Ctrl Pts',(-24.2853987784994,12.5639567579486,
129.044317559609)) ;
#127955=CARTESIAN_POINT('Ctrl Pts',(-24.3782440503395,12.3867441444795,
129.282492155211)) ;
#127956=CARTESIAN_POINT('Ctrl Pts',(-24.4838725815493,12.2832559742793,
129.557840662036)) ;
#127957=CARTESIAN_POINT('Ctrl Pts',(-24.5941053818413,12.2616345635869,
129.846906977435)) ;
#127958=CARTESIAN_POINT('Ctrl Pts',(-24.7034456841776,12.3231638748032,
130.133102368156)) ;
#127959=CARTESIAN_POINT('Ctrl Pts',(-24.8033441928373,12.4627499804897,
130.391934160841)) ;
#127960=CARTESIAN_POINT('Ctrl Pts',(-24.8887683921659,12.6729053346686,
130.608167335739)) ;
#127961=CARTESIAN_POINT('Ctrl Pts',(-24.9527937676412,12.9344260025205,
130.762243391538)) ;
#127962=CARTESIAN_POINT('Ctrl Pts',(-24.9928526876402,13.2340774716611,
130.845923250404)) ;
#127963=CARTESIAN_POINT('Ctrl Pts',(-25.005863736651,13.5439038566318,130.850977779988)) ;
#127964=CARTESIAN_POINT('Ctrl Pts',(-24.9922543333113,13.8465581380597,
130.778099436776)) ;
#127965=CARTESIAN_POINT('Ctrl Pts',(-24.9535025647549,14.1188039564303,
130.631797082968)) ;
#127966=CARTESIAN_POINT('Ctrl Pts',(-24.8928191741207,14.3420290763671,
130.421283969974)) ;
#127967=CARTESIAN_POINT('Ctrl Pts',(-24.8160182494298,14.4980360356998,
130.163918366139)) ;
#127968=CARTESIAN_POINT('Ctrl Pts',(-24.7287353277153,14.5780642406309,
129.875843754235)) ;
#127969=CARTESIAN_POINT('Ctrl Pts',(-24.637437547289,14.574764467068,129.575805260189)) ;
#127970=CARTESIAN_POINT('Ctrl Pts',(-24.5511068206059,14.4895501192037,
129.29068562796)) ;
#127971=CARTESIAN_POINT('Ctrl Pts',(-24.4749030425151,14.3274511862454,
129.034880720137)) ;
#127972=CARTESIAN_POINT('Ctrl Pts',(-24.4159592227421,14.1012131862614,
128.829634055848)) ;
#127973=CARTESIAN_POINT('Ctrl Pts',(-24.3787401330336,13.8249844629114,
128.687661505586)) ;
#127974=CARTESIAN_POINT('Ctrl Pts',(-24.3670602425512,13.5214321679055,
128.620482163558)) ;
#127975=CARTESIAN_POINT('Ctrl Pts',(-24.3822219174402,13.2103012172843,
128.631642932602)) ;
#127976=CARTESIAN_POINT('Ctrl Pts',(-24.4237994899699,12.914853162699,128.720037352722)) ;
#127977=CARTESIAN_POINT('Ctrl Pts',(-24.4901243602526,12.6543477666719,
128.880514172549)) ;
#127978=CARTESIAN_POINT('Ctrl Pts',(-24.5759154007368,12.4511188727926,
129.098200503442)) ;
#127979=CARTESIAN_POINT('Ctrl Pts',(-24.677341344801,12.3156705463735,129.36124902759)) ;
#127980=CARTESIAN_POINT('Ctrl Pts',(-24.7868457011832,12.2603783295909,
129.648000508501)) ;
#127981=CARTESIAN_POINT('Ctrl Pts',(-24.897405454224,12.2883877263298,129.937866175656)) ;
#127982=CARTESIAN_POINT('Ctrl Pts',(-25.0017261192026,12.396958257867,130.2096033973)) ;
#127983=CARTESIAN_POINT('Ctrl Pts',(-25.0940920844729,12.5805839699868,
130.446125385117)) ;
#127984=CARTESIAN_POINT('Ctrl Pts',(-25.166956841923,12.8225431227576,130.62601982101)) ;
#127985=CARTESIAN_POINT('Ctrl Pts',(-25.2172418557937,13.1085293602937,
130.739774451968)) ;
#127986=CARTESIAN_POINT('Ctrl Pts',(-25.2413929556375,13.4184312850536,
130.777054839255)) ;
#127987=CARTESIAN_POINT('Ctrl Pts',(-25.2385539434156,13.725396858395,130.73584896447)) ;
#127988=CARTESIAN_POINT('Ctrl Pts',(-25.2095431304425,14.0140710244904,
130.617811479396)) ;
#127989=CARTESIAN_POINT('Ctrl Pts',(-25.1572824387476,14.2586953063536,
130.432036477139)) ;
#127990=CARTESIAN_POINT('Ctrl Pts',(-25.0863214415307,14.4435712353924,
130.191639130538)) ;
#127991=CARTESIAN_POINT('Ctrl Pts',(-25.0023566464057,14.5554638044199,
129.913246807571)) ;
#127992=CARTESIAN_POINT('Ctrl Pts',(-24.9121278134356,14.5862678502014,
129.616544620099)) ;
#127993=CARTESIAN_POINT('Ctrl Pts',(-24.8229602070216,14.5339455357937,
129.322988050977)) ;
#127994=CARTESIAN_POINT('Ctrl Pts',(-24.7416470766687,14.4019055778879,
129.052297983318)) ;
#127995=CARTESIAN_POINT('Ctrl Pts',(-24.6750091878945,14.1996929646046,
128.824495532666)) ;
#127996=CARTESIAN_POINT('Ctrl Pts',(-24.6284968285961,13.9418840250199,
128.655489614543)) ;
#127997=CARTESIAN_POINT('Ctrl Pts',(-24.6061667098172,13.6467946138759,
128.557116414343)) ;
#127998=CARTESIAN_POINT('Ctrl Pts',(-24.6103571111199,13.3358858072713,
128.536238086489)) ;
#127999=CARTESIAN_POINT('Ctrl Pts',(-24.6414467209892,13.0311284107843,
128.593934068535)) ;
#128000=CARTESIAN_POINT('Ctrl Pts',(-24.6980852187812,12.7543595776973,
128.726232777758)) ;
#128001=CARTESIAN_POINT('Ctrl Pts',(-24.7762983426224,12.5263864421984,
128.921740016822)) ;
#128002=CARTESIAN_POINT('Ctrl Pts',(-24.8729692419651,12.360701809008,129.170730735271)) ;
#128003=CARTESIAN_POINT('Ctrl Pts',(-24.9789044892542,12.2732420187478,
129.447377219646)) ;
#128004=CARTESIAN_POINT('Ctrl Pts',(-25.0903755269925,12.2668291176247,
129.739745721998)) ;
#128005=CARTESIAN_POINT('Ctrl Pts',(-25.1981552719378,12.3436152080196,
130.021521791637)) ;
#128006=CARTESIAN_POINT('Ctrl Pts',(-25.2961464818128,12.4979167345461,
130.274599644604)) ;
#128007=CARTESIAN_POINT('Ctrl Pts',(-25.3774937525285,12.7181780575431,
130.47914395372)) ;
#128008=CARTESIAN_POINT('Ctrl Pts',(-25.4374226974674,12.9887184060059,
130.621122559274)) ;
#128009=CARTESIAN_POINT('Ctrl Pts',(-25.4723758382109,13.2908826927602,
130.690083038664)) ;
#128010=CARTESIAN_POINT('Ctrl Pts',(-25.4804804344778,13.6021683784905,
130.680651142204)) ;
#128011=CARTESIAN_POINT('Ctrl Pts',(-25.4618568415719,13.9015373279121,
130.593040688394)) ;
#128012=CARTESIAN_POINT('Ctrl Pts',(-25.4184566237588,14.1661757603649,
130.433070382521)) ;
#128013=CARTESIAN_POINT('Ctrl Pts',(-25.3547428693436,14.3763136740977,
130.213982932893)) ;
#128014=CARTESIAN_POINT('Ctrl Pts',(-25.2750987849152,14.519537909018,129.948127317248)) ;
#128015=CARTESIAN_POINT('Ctrl Pts',(-25.1868226991851,14.5837467731856,
129.657234324434)) ;
#128016=CARTESIAN_POINT('Ctrl Pts',(-25.0960577100225,14.5651055600629,
129.358881947955)) ;
#128017=CARTESIAN_POINT('Ctrl Pts',(-25.0107197946272,14.4645028782859,
129.076465778453)) ;
#128018=CARTESIAN_POINT('Ctrl Pts',(-24.937386896527,14.2890439916082,128.829076935974)) ;
#128019=CARTESIAN_POINT('Ctrl Pts',(-24.8823176595351,14.0526944829589,
128.635198343514)) ;
#128020=CARTESIAN_POINT('Ctrl Pts',(-24.8497013606514,13.7699865905546,
128.506730368574)) ;
#128021=CARTESIAN_POINT('Ctrl Pts',(-24.8428940134075,13.4631529317897,
128.453754283766)) ;
#128022=CARTESIAN_POINT('Ctrl Pts',(-24.8633570486409,13.1513621002968,
128.480200728338)) ;
#128023=CARTESIAN_POINT('Ctrl Pts',(-24.9095615347108,12.8627668300252,
128.582285450555)) ;
#128024=CARTESIAN_POINT('Ctrl Pts',(-24.9801882856006,12.6109028722605,
128.755266775312)) ;
#128025=CARTESIAN_POINT('Ctrl Pts',(-25.0690534743675,12.4200193070119,
128.981995044836)) ;
#128026=CARTESIAN_POINT('Ctrl Pts',(-25.1730899556213,12.2986947240349,
129.25251180551)) ;
#128027=CARTESIAN_POINT('Ctrl Pts',(-25.2826141954889,12.2592723923921,
129.539555750781)) ;
#128028=CARTESIAN_POINT('Ctrl Pts',(-25.3932290191672,12.3030853474788,
129.829385193708)) ;
#128029=CARTESIAN_POINT('Ctrl Pts',(-25.4952065717163,12.4259705775221,
130.094414362096)) ;
#128030=CARTESIAN_POINT('Ctrl Pts',(-25.584551513735,12.6220549960923,130.322094334834)) ;
#128031=CARTESIAN_POINT('Ctrl Pts',(-25.653592832138,12.8744669266435,130.490706005762)) ;
#128032=CARTESIAN_POINT('Ctrl Pts',(-25.6989762677483,13.1663405887179,
130.590157332786)) ;
#128033=CARTESIAN_POINT('Ctrl Pts',(-25.7179831336094,13.4758788590996,
130.612636803496)) ;
#128034=CARTESIAN_POINT('Ctrl Pts',(-25.7101797421068,13.7823952671727,
130.556721850523)) ;
#128035=CARTESIAN_POINT('Ctrl Pts',(-25.6763506271671,14.0644181714752,
130.424604261457)) ;
#128036=CARTESIAN_POINT('Ctrl Pts',(-25.6205406548785,14.2977471019388,
130.228651586956)) ;
#128037=CARTESIAN_POINT('Ctrl Pts',(-25.5464475856731,14.4706193874242,
129.978984296464)) ;
#128038=CARTESIAN_POINT('Ctrl Pts',(-25.460677945702,14.5675955014972,129.695290809472)) ;
#128039=CARTESIAN_POINT('Ctrl Pts',(-25.3702300380859,14.5827756049051,
129.398006359781)) ;
#128040=CARTESIAN_POINT('Ctrl Pts',(-25.2818560211881,14.5148008720864,
129.106690050431)) ;
#128041=CARTESIAN_POINT('Ctrl Pts',(-25.2030490646069,14.3692243405837,
128.843429932205)) ;
#128042=CARTESIAN_POINT('Ctrl Pts',(-25.1395076712243,14.1540994987709,
128.624494501162)) ;
#128043=CARTESIAN_POINT('Ctrl Pts',(-25.0975798520609,13.8891946725912,
128.469071398168)) ;
#128044=CARTESIAN_POINT('Ctrl Pts',(-25.0799823163942,13.5894849367596,
128.384515560491)) ;
#128045=CARTESIAN_POINT('Ctrl Pts',(-25.089317375755,13.2771022770821,128.3785662278)) ;
#128046=CARTESIAN_POINT('Ctrl Pts',(-25.1252553002292,12.9767129861419,
128.450507417475)) ;
#128047=CARTESIAN_POINT('Ctrl Pts',(-25.1866265754372,12.7063602426885,
128.596486814777)) ;
#128048=CARTESIAN_POINT('Ctrl Pts',(-25.2683748597299,12.490160978819,128.802401379313)) ;
#128049=CARTESIAN_POINT('Ctrl Pts',(-25.3669237030102,12.3386882499648,
129.057094955999)) ;
#128050=CARTESIAN_POINT('Ctrl Pts',(-25.4750438935506,12.2654833312748,
129.339847657555)) ;
#128051=CARTESIAN_POINT('Ctrl Pts',(-25.5862280103804,12.2750423779192,
129.631462856753)) ;
#128052=CARTESIAN_POINT('Ctrl Pts',(-25.6929338455416,12.3673309106593,
129.90999802218)) ;
#128053=CARTESIAN_POINT('Ctrl Pts',(-25.7877694292322,12.534346926541,130.154033164579)) ;
#128054=CARTESIAN_POINT('Ctrl Pts',(-25.8655711174805,12.7652871002756,
130.348199040054)) ;
#128055=CARTESIAN_POINT('Ctrl Pts',(-25.9212064365725,13.0444119027006,
130.477502422996)) ;
#128056=CARTESIAN_POINT('Ctrl Pts',(-25.9511258449652,13.3498617149792,
130.531785727571)) ;
#128057=CARTESIAN_POINT('Ctrl Pts',(-25.9540442725774,13.6613614956128,
130.507099881275)) ;
#128058=CARTESIAN_POINT('Ctrl Pts',(-25.9306476029736,13.9537822109427,
130.4057698744)) ;
#128059=CARTESIAN_POINT('Ctrl Pts',(-25.8832256006458,14.2096141501914,
130.234109824226)) ;
#128060=CARTESIAN_POINT('Ctrl Pts',(-25.8158001807284,14.409057323901,130.003996520483)) ;
#128061=CARTESIAN_POINT('Ctrl Pts',(-25.7341641419467,14.5378227740497,
129.732422677828)) ;
#128062=CARTESIAN_POINT('Ctrl Pts',(-25.6443470911794,14.5866410235712,
129.436796365213)) ;
#128063=CARTESIAN_POINT('Ctrl Pts',(-25.5547638150537,14.5524956980778,
129.142180912862)) ;
#128064=CARTESIAN_POINT('Ctrl Pts',(-25.4705811162127,14.436335978299,128.862889568447)) ;
#128065=CARTESIAN_POINT('Ctrl Pts',(-25.4006244003216,14.2487612510743,
128.625535064057)) ;
#128066=CARTESIAN_POINT('Ctrl Pts',(-25.3493716847571,14.0019963644833,
128.442718956111)) ;
#128067=CARTESIAN_POINT('Ctrl Pts',(-25.321482404065,13.7133413739479,128.328114199707)) ;
#128068=CARTESIAN_POINT('Ctrl Pts',(-25.3198401069144,13.4034231112183,
128.290130687378)) ;
#128069=CARTESIAN_POINT('Ctrl Pts',(-25.3449983181151,13.0966156086416,
128.330632354685)) ;
#128070=CARTESIAN_POINT('Ctrl Pts',(-25.3964989597862,12.8104956344232,
128.447768053659)) ;
#128071=CARTESIAN_POINT('Ctrl Pts',(-25.4705334308323,12.5707042508866,
128.631021712006)) ;
#128072=CARTESIAN_POINT('Ctrl Pts',(-25.5630356046663,12.3910193805736,
128.868133701558)) ;
#128073=CARTESIAN_POINT('Ctrl Pts',(-25.6681544066941,12.2853288734926,
129.142069440953)) ;
#128074=CARTESIAN_POINT('Ctrl Pts',(-25.778694693908,12.2609818511097,129.431921558708)) ;
#128075=CARTESIAN_POINT('Ctrl Pts',(-25.8884709129135,12.3204757411683,
129.719304966435)) ;
#128076=CARTESIAN_POINT('Ctrl Pts',(-25.9886740073855,12.4582515561699,
129.979020191138)) ;
#128077=CARTESIAN_POINT('Ctrl Pts',(-26.0743372008251,12.665899809485,130.196066145188)) ;
#128078=CARTESIAN_POINT('Ctrl Pts',(-26.1391179757226,12.926809546633,130.352268079656)) ;
#128079=CARTESIAN_POINT('Ctrl Pts',(-26.1796732755739,13.2233761024273,
130.437657929989)) ;
#128080=CARTESIAN_POINT('Ctrl Pts',(-26.1937046974809,13.5346576099115,
130.445524568179)) ;
#128081=CARTESIAN_POINT('Ctrl Pts',(-26.1807569035134,13.8387960624651,
130.374479587911)) ;
#128082=CARTESIAN_POINT('Ctrl Pts',(-26.1425724297029,14.1123017262305,
130.229804146074)) ;
#128083=CARTESIAN_POINT('Ctrl Pts',(-26.0825726076526,14.3364686788982,
130.021376384275)) ;
#128084=CARTESIAN_POINT('Ctrl Pts',(-26.0061672037188,14.4947707919197,
129.76515900541)) ;
#128085=CARTESIAN_POINT('Ctrl Pts',(-25.9186915378375,14.5769227854228,
129.476380890809)) ;
#128086=CARTESIAN_POINT('Ctrl Pts',(-25.828437185311,14.5762675559882,129.179779749649)) ;
#128087=CARTESIAN_POINT('Ctrl Pts',(-25.7411174774271,14.4930554599536,
128.891479940059)) ;
#128088=CARTESIAN_POINT('Ctrl Pts',(-25.6647114903275,14.3331651015145,
128.63516567355)) ;
#128089=CARTESIAN_POINT('Ctrl Pts',(-25.6050905510217,14.1081176905962,
128.427867003823)) ;
#128090=CARTESIAN_POINT('Ctrl Pts',(-25.5673123091255,13.8340179533061,
128.28438435414)) ;
#128091=CARTESIAN_POINT('Ctrl Pts',(-25.5547989687703,13.5302899691965,
128.21468609169)) ;
#128092=CARTESIAN_POINT('Ctrl Pts',(-25.5691793862707,13.2194242274908,
128.223607489868)) ;
#128093=CARTESIAN_POINT('Ctrl Pts',(-25.6099882053418,12.9232188670747,
128.309754159081)) ;
#128094=CARTESIAN_POINT('Ctrl Pts',(-25.6755761765933,12.661461296016,128.468101957688)) ;
#128095=CARTESIAN_POINT('Ctrl Pts',(-25.7610234535684,12.4560560459253,
128.684718224714)) ;
#128096=CARTESIAN_POINT('Ctrl Pts',(-25.8617752670754,12.3187614615208,
128.945904715609)) ;
#128097=CARTESIAN_POINT('Ctrl Pts',(-25.9712898119601,12.2608758926762,
129.232630942734)) ;
#128098=CARTESIAN_POINT('Ctrl Pts',(-26.0817469151749,12.2860567497161,
129.522259623789)) ;
#128099=CARTESIAN_POINT('Ctrl Pts',(-26.1872408236699,12.3936760762178,
129.797118439097)) ;
#128100=CARTESIAN_POINT('Ctrl Pts',(-26.2790423656848,12.5734427117125,
130.032358969761)) ;
#128101=CARTESIAN_POINT('Ctrl Pts',(-26.3531762412792,12.8155556757963,
130.215696265957)) ;
#128102=CARTESIAN_POINT('Ctrl Pts',(-26.4039053292045,13.1001458923633,
130.330827106248)) ;
#128103=CARTESIAN_POINT('Ctrl Pts',(-26.4288254379187,13.4082451874709,
130.370501539131)) ;
#128104=CARTESIAN_POINT('Ctrl Pts',(-26.426822031636,13.7170001828003,130.331582040945)) ;
#128105=CARTESIAN_POINT('Ctrl Pts',(-26.3984000431209,14.0068803431456,
130.215220499312)) ;
#128106=CARTESIAN_POINT('Ctrl Pts',(-26.3469149274336,14.2520830304775,
130.031824301073)) ;
#128107=CARTESIAN_POINT('Ctrl Pts',(-26.2765535613933,14.4388654821964,
129.793218238151)) ;
#128108=CARTESIAN_POINT('Ctrl Pts',(-26.1927905162966,14.5532758713035,
129.515375412257)) ;
#128109=CARTESIAN_POINT('Ctrl Pts',(-26.1025705013195,14.5866372917137,
129.218675357135)) ;
#128110=CARTESIAN_POINT('Ctrl Pts',(-26.013030368013,14.5363254229255,128.923932390282)) ;
#128111=CARTESIAN_POINT('Ctrl Pts',(-25.9317546338566,14.4070821758454,
128.653504394788)) ;
#128112=CARTESIAN_POINT('Ctrl Pts',(-25.8642785654878,14.2058492351143,
128.42309702246)) ;
#128113=CARTESIAN_POINT('Ctrl Pts',(-25.8172570002977,13.9493210351354,
128.252624752721)) ;
#128114=CARTESIAN_POINT('Ctrl Pts',(-25.7942597880218,13.6560816946818,
128.152419866967)) ;
#128115=CARTESIAN_POINT('Ctrl Pts',(-25.7976276043833,13.345421430163,128.129145084191)) ;
#128116=CARTESIAN_POINT('Ctrl Pts',(-25.8277991868315,13.040595844376,128.18421481984)) ;
#128117=CARTESIAN_POINT('Ctrl Pts',(-25.8840495582596,12.7610203807177,
128.315183220205)) ;
#128118=CARTESIAN_POINT('Ctrl Pts',(-25.9616974256306,12.5320805251594,
128.509083689549)) ;
#128119=CARTESIAN_POINT('Ctrl Pts',(-26.0572216139122,12.3651153632671,
128.754952054418)) ;
#128120=CARTESIAN_POINT('Ctrl Pts',(-26.16380926824,12.2743250028136,129.033224471676)) ;
#128121=CARTESIAN_POINT('Ctrl Pts',(-26.2753298606958,12.2660445158075,
129.325721909756)) ;
#128122=CARTESIAN_POINT('Ctrl Pts',(-26.3828799962309,12.3402671255805,
129.606951767026)) ;
#128123=CARTESIAN_POINT('Ctrl Pts',(-26.4812883874454,12.4924311460887,
129.861240484378)) ;
#128124=CARTESIAN_POINT('Ctrl Pts',(-26.5630932377152,12.7106680938423,
130.067163032861)) ;
#128125=CARTESIAN_POINT('Ctrl Pts',(-26.6238634402305,12.9803449580317,
130.211547393049)) ;
#128126=CARTESIAN_POINT('Ctrl Pts',(-26.6596062976098,13.2833170370261,
130.282668176157)) ;
#128127=CARTESIAN_POINT('Ctrl Pts',(-26.6683992001938,13.5926827772034,
130.275458609873)) ;
#128128=CARTESIAN_POINT('Ctrl Pts',(-26.6505137795868,13.8936497726217,
130.189900592151)) ;
#128129=CARTESIAN_POINT('Ctrl Pts',(-26.6078602763148,14.1589430320387,
130.032192029423)) ;
#128130=CARTESIAN_POINT('Ctrl Pts',(-26.5445783612324,14.3711507440271,
129.814309109576)) ;
#128131=CARTESIAN_POINT('Ctrl Pts',(-26.4655827230832,14.5162610526243,
129.550459758268)) ;
#128132=CARTESIAN_POINT('Ctrl Pts',(-26.376738727669,14.5833063446483,129.257632402111)) ;
#128133=CARTESIAN_POINT('Ctrl Pts',(-26.2861729331064,14.566512972423,128.959951686922)) ;
#128134=CARTESIAN_POINT('Ctrl Pts',(-26.2009020705313,14.4685224251672,
128.67784492761)) ;
#128135=CARTESIAN_POINT('Ctrl Pts',(-26.1271681583346,14.295496638092,128.429327566497)) ;
#128136=CARTESIAN_POINT('Ctrl Pts',(-26.0713023155461,14.0596946684097,
128.232981990481)) ;
#128137=CARTESIAN_POINT('Ctrl Pts',(-26.0380253527417,13.7784556311811,
128.102645526396)) ;
#128138=CARTESIAN_POINT('Ctrl Pts',(-26.0306021104224,13.4704205664196,
128.047693579746)) ;
#128139=CARTESIAN_POINT('Ctrl Pts',(-26.0499050772378,13.1626907003778,
128.071224875015)) ;
#128140=CARTESIAN_POINT('Ctrl Pts',(-26.0958353944327,12.8697533326654,
128.172107844854)) ;
#128141=CARTESIAN_POINT('Ctrl Pts',(-26.1651975859897,12.6186668419938,
128.341706812271)) ;
#128142=CARTESIAN_POINT('Ctrl Pts',(-26.2543855123382,12.4240570557475,
128.56905730259)) ;
#128143=CARTESIAN_POINT('Ctrl Pts',(-26.3570165493029,12.3017129015635,
128.835831715512)) ;
#128144=CARTESIAN_POINT('Ctrl Pts',(-26.4672343576536,12.259212443294,129.124643417402)) ;
#128145=CARTESIAN_POINT('Ctrl Pts',(-26.5774090635175,12.3002004247184,
129.413368541245)) ;
#128146=CARTESIAN_POINT('Ctrl Pts',(-26.6807625992197,12.4222100082891,
129.682061388604)) ;
#128147=CARTESIAN_POINT('Ctrl Pts',(-26.7698384246454,12.6151763777399,
129.90922006221)) ;
#128148=CARTESIAN_POINT('Ctrl Pts',(-26.8397567435722,12.8667635442981,
130.080291665491)) ;
#128149=CARTESIAN_POINT('Ctrl Pts',(-26.8856922490943,13.156608287975,130.181493757996)) ;
#128150=CARTESIAN_POINT('Ctrl Pts',(-26.905648091964,13.4669634913823,130.206630694337)) ;
#128151=CARTESIAN_POINT('Ctrl Pts',(-26.8984820418813,13.7743605544172,
130.152520289261)) ;
#128152=CARTESIAN_POINT('Ctrl Pts',(-26.8656427954947,14.0556835364492,
130.023511196521)) ;
#128153=CARTESIAN_POINT('Ctrl Pts',(-26.8101219407047,14.2923698340539,
129.828181452464)) ;
#128154=CARTESIAN_POINT('Ctrl Pts',(-26.7362953067133,14.4669398089711,
129.579261905855)) ;
#128155=CARTESIAN_POINT('Ctrl Pts',(-26.6512662787074,14.5658237072004,
129.297919990246)) ;
#128156=CARTESIAN_POINT('Ctrl Pts',(-26.5603402007787,14.5834030804103,
128.99904072882)) ;
#128157=CARTESIAN_POINT('Ctrl Pts',(-26.4722852743979,14.5182209640518,
128.70885302489)) ;
#128158=CARTESIAN_POINT('Ctrl Pts',(-26.3924389121312,14.3732472744243,
128.4422467857)) ;
#128159=CARTESIAN_POINT('Ctrl Pts',(-26.3290394001796,14.1617341160313,
128.22405452454)) ;
#128160=CARTESIAN_POINT('Ctrl Pts',(-26.2861256992153,13.8968739581495,
128.065570508626)) ;
#128161=CARTESIAN_POINT('Ctrl Pts',(-26.2678898569706,13.5970561201623,
127.979085240886)) ;
#128162=CARTESIAN_POINT('Ctrl Pts',(-26.2765300087796,13.2853498772371,
127.971172699377)) ;
#128163=CARTESIAN_POINT('Ctrl Pts',(-26.3116223620029,12.9854214225964,
128.040755422592)) ;
#128164=CARTESIAN_POINT('Ctrl Pts',(-26.3720202123015,12.7145026725385,
128.18399408205)) ;
#128165=CARTESIAN_POINT('Ctrl Pts',(-26.4535694094826,12.4953422799607,
128.389165339747)) ;
#128166=CARTESIAN_POINT('Ctrl Pts',(-26.5519324421244,12.341785792788,128.643267128277)) ;
#128167=CARTESIAN_POINT('Ctrl Pts',(-26.6595602095204,12.2665368205457,
128.924676014665)) ;
#128168=CARTESIAN_POINT('Ctrl Pts',(-26.7706440836229,12.2735361579836,
129.216032753461)) ;
#128169=CARTESIAN_POINT('Ctrl Pts',(-26.8775441666754,12.3632299170458,
129.49515442713)) ;
#128170=CARTESIAN_POINT('Ctrl Pts',(-26.9731151455713,12.5286847379392,
129.741232249963)) ;
#128171=CARTESIAN_POINT('Ctrl Pts',(-27.0513963528373,12.7579694052531,
129.936820922564)) ;
#128172=CARTESIAN_POINT('Ctrl Pts',(-27.1076391987102,13.0352202264865,
130.067983012539)) ;
#128173=CARTESIAN_POINT('Ctrl Pts',(-27.1383941250434,13.3405828522819,
130.124659245561)) ;
#128174=CARTESIAN_POINT('Ctrl Pts',(-27.142164217804,13.6512271404406,130.102573741676)) ;
#128175=CARTESIAN_POINT('Ctrl Pts',(-27.1194950619664,13.945858673121,130.003220415338)) ;
#128176=CARTESIAN_POINT('Ctrl Pts',(-27.0725556914897,14.2033946436315,
129.832909918837)) ;
#128177=CARTESIAN_POINT('Ctrl Pts',(-27.0058079309889,14.4040391097263,
129.60487026237)) ;
#128178=CARTESIAN_POINT('Ctrl Pts',(-26.9246130375758,14.5350227363909,
129.334619148942)) ;
#128179=CARTESIAN_POINT('Ctrl Pts',(-26.8347923397077,14.5864958768454,
129.038934787031)) ;
#128180=CARTESIAN_POINT('Ctrl Pts',(-26.7449544652946,14.554416926093,128.743505036233)) ;
#128181=CARTESIAN_POINT('Ctrl Pts',(-26.6609820117157,14.4414134388981,
128.465037672866)) ;
#128182=CARTESIAN_POINT('Ctrl Pts',(-26.5901696168786,14.2551029689439,
128.225021388413)) ;
#128183=CARTESIAN_POINT('Ctrl Pts',(-26.5383476891214,14.0100365387615,
128.040581334637)) ;
#128184=CARTESIAN_POINT('Ctrl Pts',(-26.5097071652286,13.7214335720741,
127.923681487066)) ;
#128185=CARTESIAN_POINT('Ctrl Pts',(-26.5072415117763,13.4135493080175,
127.883485393481)) ;
#128186=CARTESIAN_POINT('Ctrl Pts',(-26.5317926987144,13.1045553567054,
127.922006198238)) ;
#128187=CARTESIAN_POINT('Ctrl Pts',(-26.5821066591862,12.8197359120567,
128.035956491399)) ;
#128188=CARTESIAN_POINT('Ctrl Pts',(-26.6560761824492,12.576213522993,128.218737407166)) ;
#128189=CARTESIAN_POINT('Ctrl Pts',(-26.7479977099995,12.3952019972504,
128.454228677948)) ;
#128190=CARTESIAN_POINT('Ctrl Pts',(-26.852959270396,12.2871509168402,128.727666098665)) ;
#128191=CARTESIAN_POINT('Ctrl Pts',(-26.9631857583284,12.2605661250461,
129.016678346631)) ;
#128192=CARTESIAN_POINT('Ctrl Pts',(-27.0731032377883,12.3174696014915,
129.304479474258)) ;
#128193=CARTESIAN_POINT('Ctrl Pts',(-27.1738841185141,12.45350954949,129.565800797398)) ;
#128194=CARTESIAN_POINT('Ctrl Pts',(-27.2598368577993,12.6588730933983,
129.783777023258)) ;
#128195=CARTESIAN_POINT('Ctrl Pts',(-27.3253460720657,12.9185732452431,
129.942083221898)) ;
#128196=CARTESIAN_POINT('Ctrl Pts',(-27.3666461043042,13.2144047021654,
130.029650643336)) ;
#128197=CARTESIAN_POINT('Ctrl Pts',(-27.3814508616359,13.5255441654578,
130.039777855938)) ;
#128198=CARTESIAN_POINT('Ctrl Pts',(-27.3693461451008,13.8297539954917,
129.971255359995)) ;
#128199=CARTESIAN_POINT('Ctrl Pts',(-27.3317726975183,14.1049217876101,
129.828295911421)) ;
#128200=CARTESIAN_POINT('Ctrl Pts',(-27.2727161189021,14.329872377713,129.622795412737)) ;
#128201=CARTESIAN_POINT('Ctrl Pts',(-27.1961848662824,14.491552798162,129.365964164441)) ;
#128202=CARTESIAN_POINT('Ctrl Pts',(-27.1091899784791,14.5755974464537,
129.078707325624)) ;
#128203=CARTESIAN_POINT('Ctrl Pts',(-27.01879203794,14.5774288314458,128.781626400399)) ;
#128204=CARTESIAN_POINT('Ctrl Pts',(-26.9314794185646,14.4968431442199,
128.493436234079)) ;
#128205=CARTESIAN_POINT('Ctrl Pts',(-26.8543959535475,14.3385595684728,
128.235025271593)) ;
#128206=CARTESIAN_POINT('Ctrl Pts',(-26.7942771704595,14.1152210821619,
128.026295396246)) ;
#128207=CARTESIAN_POINT('Ctrl Pts',(-26.7558188879496,13.8419814694385,
127.880794925919)) ;
#128208=CARTESIAN_POINT('Ctrl Pts',(-26.7425859508397,13.5398085198315,
127.809104336374)) ;
#128209=CARTESIAN_POINT('Ctrl Pts',(-26.7561438538663,13.2280435921434,
127.81553948295)) ;
#128210=CARTESIAN_POINT('Ctrl Pts',(-26.7964991026641,12.9300591046375,
127.900229432936)) ;
#128211=CARTESIAN_POINT('Ctrl Pts',(-26.8611655938303,12.6684084427586,
128.056051445632)) ;
#128212=CARTESIAN_POINT('Ctrl Pts',(-26.9462176040478,12.4608091594121,
128.27145590624)) ;
#128213=CARTESIAN_POINT('Ctrl Pts',(-27.0467113671397,12.3214093535999,
128.53187021786)) ;
#128214=CARTESIAN_POINT('Ctrl Pts',(-27.1562555166034,12.261330300397,128.818633686213)) ;
#128215=CARTESIAN_POINT('Ctrl Pts',(-27.2663375886122,12.2843254988424,
129.107291751522)) ;
#128216=CARTESIAN_POINT('Ctrl Pts',(-27.3716324986393,12.3887269721217,
129.381731211064)) ;
#128217=CARTESIAN_POINT('Ctrl Pts',(-27.4644801364651,12.5673627436567,
129.619832504695)) ;
#128218=CARTESIAN_POINT('Ctrl Pts',(-27.5391406638283,12.8080166806353,
129.804719444648)) ;
#128219=CARTESIAN_POINT('Ctrl Pts',(-27.5906063032235,13.0914774354823,
129.922013122237)) ;
#128220=CARTESIAN_POINT('Ctrl Pts',(-27.616327879176,13.4005589670674,129.963888465317)) ;
#128221=CARTESIAN_POINT('Ctrl Pts',(-27.6149921031721,13.7083911596742,
129.927043626821)) ;
#128222=CARTESIAN_POINT('Ctrl Pts',(-27.5874202378808,13.9985991378762,
129.813238675445)) ;
#128223=CARTESIAN_POINT('Ctrl Pts',(-27.536484449555,14.2457812559265,129.631387326717)) ;
#128224=CARTESIAN_POINT('Ctrl Pts',(-27.4665317915239,14.4345734153115,
129.393953237947)) ;
#128225=CARTESIAN_POINT('Ctrl Pts',(-27.383009709236,14.5511370879547,129.116800950602)) ;
#128226=CARTESIAN_POINT('Ctrl Pts',(-27.2931554129536,14.5867802187907,
128.821269985454)) ;
#128227=CARTESIAN_POINT('Ctrl Pts',(-27.2034748698954,14.5391948483821,
128.526119117529)) ;
#128228=CARTESIAN_POINT('Ctrl Pts',(-27.1215961718606,14.411534541166,128.253806213587)) ;
#128229=CARTESIAN_POINT('Ctrl Pts',(-27.0540300153367,14.2134355911455,
128.023342403406)) ;
#128230=CARTESIAN_POINT('Ctrl Pts',(-27.0061516223831,13.9582377807151,
127.850318612923)) ;
#128231=CARTESIAN_POINT('Ctrl Pts',(-26.9823271114248,13.6646542857207,
127.747569753109)) ;
#128232=CARTESIAN_POINT('Ctrl Pts',(-26.9849343677111,13.354183694307,127.722078671003)) ;
#128233=CARTESIAN_POINT('Ctrl Pts',(-27.0144698797521,13.0484269475921,
127.775232008199)) ;
#128234=CARTESIAN_POINT('Ctrl Pts',(-27.0696778910055,12.7694396144753,
127.903355960201)) ;
#128235=CARTESIAN_POINT('Ctrl Pts',(-27.1468061921369,12.5380417818578,
128.095664000225)) ;
#128236=CARTESIAN_POINT('Ctrl Pts',(-27.2424888343211,12.3683286103215,
128.341812779954)) ;
#128237=CARTESIAN_POINT('Ctrl Pts',(-27.3483693988791,12.2760420301782,
128.618176794529)) ;
#128238=CARTESIAN_POINT('Ctrl Pts',(-27.4593559365058,12.2649171956023,
128.909263666053)) ;
#128239=CARTESIAN_POINT('Ctrl Pts',(-27.567634623934,12.3368690602114,129.192461766527)) ;
#128240=CARTESIAN_POINT('Ctrl Pts',(-27.666488441497,12.4871142426883,129.448028051994)) ;
#128241=CARTESIAN_POINT('Ctrl Pts',(-27.7489819874493,12.7041605723025,
129.655894722522)) ;
#128242=CARTESIAN_POINT('Ctrl Pts',(-27.8101941453054,12.9721742229255,
129.80164232834)) ;
#128243=CARTESIAN_POINT('Ctrl Pts',(-27.846628352146,13.2726902909237,129.874973593325)) ;
#128244=CARTESIAN_POINT('Ctrl Pts',(-27.8563402142155,13.5844634712024,
129.870193895069)) ;
#128245=CARTESIAN_POINT('Ctrl Pts',(-27.8391363324445,13.8852370935213,
129.786712780349)) ;
#128246=CARTESIAN_POINT('Ctrl Pts',(-27.7974142447192,14.1508960461137,
129.631852840205)) ;
#128247=CARTESIAN_POINT('Ctrl Pts',(-27.734510775802,14.3659570347197,129.414953151005)) ;
#128248=CARTESIAN_POINT('Ctrl Pts',(-27.6555249095009,14.513384444757,129.151006206137)) ;
#128249=CARTESIAN_POINT('Ctrl Pts',(-27.5675962898643,14.58228249035,128.861131563589)) ;
#128250=CARTESIAN_POINT('Ctrl Pts',(-27.4767674367506,14.5684017700248,
128.562597823583)) ;
#128251=CARTESIAN_POINT('Ctrl Pts',(-27.3910622500698,14.4726240352221,
128.279161519902)) ;
#128252=CARTESIAN_POINT('Ctrl Pts',(-27.3167036437953,14.3009018256013,
128.028711527011)) ;
#128253=CARTESIAN_POINT('Ctrl Pts',(-27.2604835702691,14.0676662021592,
127.831474654868)) ;
#128254=CARTESIAN_POINT('Ctrl Pts',(-27.2264233622165,13.7867923428731,
127.698762487331)) ;
#128255=CARTESIAN_POINT('Ctrl Pts',(-27.2181959748588,13.4808115770732,
127.641638031402)) ;
#128256=CARTESIAN_POINT('Ctrl Pts',(-27.2367954548246,13.1706177379304,
127.662872485548)) ;
#128257=CARTESIAN_POINT('Ctrl Pts',(-27.2821107930129,12.8770484120512,
127.761971688995)) ;
#128258=CARTESIAN_POINT('Ctrl Pts',(-27.3507301309266,12.6251910549939,
127.929467048696)) ;
#128259=CARTESIAN_POINT('Ctrl Pts',(-27.4391846595436,12.4289584768191,
128.154751522028)) ;
#128260=CARTESIAN_POINT('Ctrl Pts',(-27.5420614810931,12.3038002387545,
128.42206593562)) ;
#128261=CARTESIAN_POINT('Ctrl Pts',(-27.6519492987896,12.2593442699651,
128.709988056267)) ;
#128262=CARTESIAN_POINT('Ctrl Pts',(-27.7619662940764,12.2978898769658,
128.998322853002)) ;
#128263=CARTESIAN_POINT('Ctrl Pts',(-27.865379784088,12.4169444283248,129.267289988982)) ;
#128264=CARTESIAN_POINT('Ctrl Pts',(-27.9555551516384,12.6093773195972,
129.497426958593)) ;
#128265=CARTESIAN_POINT('Ctrl Pts',(-28.0257071874864,12.8583734122104,
129.669351599666)) ;
#128266=CARTESIAN_POINT('Ctrl Pts',(-28.0725603911615,13.1480449714035,
129.773142916573)) ;
#128267=CARTESIAN_POINT('Ctrl Pts',(-28.0932282711231,13.4582417931766,
129.800355674883)) ;
#128268=CARTESIAN_POINT('Ctrl Pts',(-28.0868635394014,13.7655079117814,
129.748643838575)) ;
#128269=CARTESIAN_POINT('Ctrl Pts',(-28.0546846226306,14.0483169670967,
129.621511117713)) ;
#128270=CARTESIAN_POINT('Ctrl Pts',(-27.9998381490793,14.285999002941,129.428215013828)) ;
#128271=CARTESIAN_POINT('Ctrl Pts',(-27.9267313668262,14.4624790496655,
129.18149179678)) ;
#128272=CARTESIAN_POINT('Ctrl Pts',(-27.8413857863696,14.5642183911393,
128.899001900319)) ;
#128273=CARTESIAN_POINT('Ctrl Pts',(-27.7510753292932,14.5841609498882,
128.602138093997)) ;
#128274=CARTESIAN_POINT('Ctrl Pts',(-27.6623060110327,14.520970734674,128.309647323951)) ;
#128275=CARTESIAN_POINT('Ctrl Pts',(-27.5826746424944,14.3791779358065,
128.0439161209)) ;
#128276=CARTESIAN_POINT('Ctrl Pts',(-27.518374582185,14.1688151362551,127.822942393228)) ;
#128277=CARTESIAN_POINT('Ctrl Pts',(-27.4748576193926,13.9051957088918,
127.662708523844)) ;
#128278=CARTESIAN_POINT('Ctrl Pts',(-27.455878155537,13.60715006879,127.574159959947)) ;
#128279=CARTESIAN_POINT('Ctrl Pts',(-27.4635634033647,13.2953843814918,
127.563449508453)) ;
#128280=CARTESIAN_POINT('Ctrl Pts',(-27.4981521378243,12.9930169526984,
127.631353422156)) ;
#128281=CARTESIAN_POINT('Ctrl Pts',(-27.557608395534,12.7222273700058,127.772001748044)) ;
#128282=CARTESIAN_POINT('Ctrl Pts',(-27.6388268171335,12.500544093303,127.97609760927)) ;
#128283=CARTESIAN_POINT('Ctrl Pts',(-27.7367701007511,12.3451353324325,
128.228996533809)) ;
#128284=CARTESIAN_POINT('Ctrl Pts',(-27.8442278309089,12.2674914285865,
128.509899764783)) ;
#128285=CARTESIAN_POINT('Ctrl Pts',(-27.9556267443121,12.2722652657277,
128.802088932825)) ;
#128286=CARTESIAN_POINT('Ctrl Pts',(-28.0626310256601,12.3599738467364,
129.081538376024)) ;
#128287=CARTESIAN_POINT('Ctrl Pts',(-28.1582011213712,12.5226378491769,
129.327757332152)) ;
#128288=CARTESIAN_POINT('Ctrl Pts',(-28.2373259873122,12.7508222616319,
129.525715012972)) ;
#128289=CARTESIAN_POINT('Ctrl Pts',(-28.2943391587573,13.0279565462644,
129.659029364955)) ;
#128290=CARTESIAN_POINT('Ctrl Pts',(-28.3256773216857,13.3323087573567,
129.71747181238)) ;
#128291=CARTESIAN_POINT('Ctrl Pts',(-28.3302116619813,13.6420774120511,
129.697726410344)) ;
#128292=CARTESIAN_POINT('Ctrl Pts',(-28.3083291946858,13.9374078331077,
129.600681337831)) ;
#128293=CARTESIAN_POINT('Ctrl Pts',(-28.2620837924338,14.1965319396346,
129.432389885247)) ;
#128294=CARTESIAN_POINT('Ctrl Pts',(-28.1954079952008,14.3999725779251,
129.204370428957)) ;
#128295=CARTESIAN_POINT('Ctrl Pts',(-28.1149345373054,14.5320840128439,
128.936405639346)) ;
#128296=CARTESIAN_POINT('Ctrl Pts',(-28.0254070588349,14.5862914481129,
128.641628884545)) ;
#128297=CARTESIAN_POINT('Ctrl Pts',(-27.9349905698168,14.5562373183141,
128.344321370437)) ;
#128298=CARTESIAN_POINT('Ctrl Pts',(-27.8512631288849,14.4460760086482,
128.066773599745)) ;
#128299=CARTESIAN_POINT('Ctrl Pts',(-27.7796573084958,14.2613118690052,
127.824318182641)) ;
#128300=CARTESIAN_POINT('Ctrl Pts',(-27.7272301440332,14.0168342944471,
127.638029248606)) ;
#128301=CARTESIAN_POINT('Ctrl Pts',(-27.6980179864544,13.7314084921459,
127.519711908543)) ;
#128302=CARTESIAN_POINT('Ctrl Pts',(-27.694741233829,13.4213927772855,127.476877876191)) ;
#128303=CARTESIAN_POINT('Ctrl Pts',(-27.7184522170526,13.1138964811438,
127.513143988576)) ;
#128304=CARTESIAN_POINT('Ctrl Pts',(-27.7680874772327,12.8273574964974,
127.625029075045)) ;
#128305=CARTESIAN_POINT('Ctrl Pts',(-27.8415277932473,12.5821904273637,
127.806243710016)) ;
#128306=CARTESIAN_POINT('Ctrl Pts',(-27.9331064049308,12.3992406636329,
128.040702389871)) ;
#128307=CARTESIAN_POINT('Ctrl Pts',(-28.0374350862425,12.2892635372044,
128.312405983018)) ;
#128308=CARTESIAN_POINT('Ctrl Pts',(-28.1478242152573,12.2601882731061,
128.601820064507)) ;
#128309=CARTESIAN_POINT('Ctrl Pts',(-28.2574870562922,12.3144490332909,
128.889000080819)) ;
#128310=CARTESIAN_POINT('Ctrl Pts',(-28.3587283063992,12.4481500310982,
129.151637015902)) ;
#128311=CARTESIAN_POINT('Ctrl Pts',(-28.4452635080364,12.6515765338915,
129.371309005377)) ;
#128312=CARTESIAN_POINT('Ctrl Pts',(-28.5117628591178,12.9112090409297,
129.532345469997)) ;
#128313=CARTESIAN_POINT('Ctrl Pts',(-28.5537057225309,13.2069680634014,
129.621732622069)) ;
#128314=CARTESIAN_POINT('Ctrl Pts',(-28.5691937316055,13.5165270688446,
129.634014378779)) ;
#128315=CARTESIAN_POINT('Ctrl Pts',(-28.5577477153071,13.8224961105202,
129.5672725385)) ;
#128316=CARTESIAN_POINT('Ctrl Pts',(-28.5209930737035,14.0973150070006,
129.426876181682)) ;
#128317=CARTESIAN_POINT('Ctrl Pts',(-28.4624086215617,14.3244517952957,
129.222682993721)) ;
#128318=CARTESIAN_POINT('Ctrl Pts',(-28.3863966418976,14.4877799553715,
128.967429888637)) ;
#128319=CARTESIAN_POINT('Ctrl Pts',(-28.2997377511392,14.5742904873528,
128.681191571893)) ;
#128320=CARTESIAN_POINT('Ctrl Pts',(-28.2089570194485,14.5785355411289,
128.382852483818)) ;
#128321=CARTESIAN_POINT('Ctrl Pts',(-28.1215748771768,14.4999983215905,
128.09449428547)) ;
#128322=CARTESIAN_POINT('Ctrl Pts',(-28.0444292301552,14.3447574247582,
127.836061476381)) ;
#128323=CARTESIAN_POINT('Ctrl Pts',(-27.9834965686545,14.1223924190304,
127.624828784792)) ;
#128324=CARTESIAN_POINT('Ctrl Pts',(-27.9444380366247,13.8510686498015,
127.477666074581)) ;
#128325=CARTESIAN_POINT('Ctrl Pts',(-27.930360050621,13.5484336095185,127.403388519421)) ;
#128326=CARTESIAN_POINT('Ctrl Pts',(-27.9431835233612,13.2370241566132,
127.407724507392)) ;
#128327=CARTESIAN_POINT('Ctrl Pts',(-27.9826117035251,12.9391311523709,
127.489800007884)) ;
#128328=CARTESIAN_POINT('Ctrl Pts',(-28.0466226653077,12.6756660362993,
127.643662724159)) ;
#128329=CARTESIAN_POINT('Ctrl Pts',(-28.1313787129563,12.4657027909829,
127.858115595181)) ;
#128330=CARTESIAN_POINT('Ctrl Pts',(-28.2314667834269,12.324474551251,128.117369989925)) ;
#128331=CARTESIAN_POINT('Ctrl Pts',(-28.3403582781537,12.2619232759168,
128.402373643518)) ;
#128332=CARTESIAN_POINT('Ctrl Pts',(-28.4512758924128,12.2825882347195,
128.693237314343)) ;
#128333=CARTESIAN_POINT('Ctrl Pts',(-28.5564686671438,12.3846501160854,
128.967486567491)) ;
#128334=CARTESIAN_POINT('Ctrl Pts',(-28.6497560237034,12.5611187121008,
129.206879240928)) ;
#128335=CARTESIAN_POINT('Ctrl Pts',(-28.7250343701191,12.800128888062,129.39357903039)) ;
#128336=CARTESIAN_POINT('Ctrl Pts',(-28.7772435757727,13.0829558390025,
129.513002075926)) ;
#128337=CARTESIAN_POINT('Ctrl Pts',(-28.803716434952,13.3903655442342,129.557211154603)) ;
#128338=CARTESIAN_POINT('Ctrl Pts',(-28.803174137136,13.7001366182577,129.522500863899)) ;
#128339=CARTESIAN_POINT('Ctrl Pts',(-28.7764473676396,13.9898881867711,
129.411323520338)) ;
#128340=CARTESIAN_POINT('Ctrl Pts',(-28.7260928299473,14.2391934618933,
129.231093829253)) ;
#128341=CARTESIAN_POINT('Ctrl Pts',(-28.656715613741,14.4298567293758,128.995378640907)) ;
#128342=CARTESIAN_POINT('Ctrl Pts',(-28.5729912432793,14.5492471460414,
128.717440021589)) ;
#128343=CARTESIAN_POINT('Ctrl Pts',(-28.4835291438219,14.5868020956478,
128.423172517193)) ;
#128344=CARTESIAN_POINT('Ctrl Pts',(-28.3938133452937,14.5417975160937,
128.127949271842)) ;
#128345=CARTESIAN_POINT('Ctrl Pts',(-28.3115790793439,14.416208825978,127.854576526063)) ;
#128346=CARTESIAN_POINT('Ctrl Pts',(-28.2435588146913,14.22040833296,127.622834888852)) ;
#128347=CARTESIAN_POINT('Ctrl Pts',(-28.1948097328007,13.9647701256438,
127.447046656053)) ;
#128348=CARTESIAN_POINT('Ctrl Pts',(-28.1704722438048,13.6739288758575,
127.343029876413)) ;
#128349=CARTESIAN_POINT('Ctrl Pts',(-28.1722918388017,13.3623285139176,
127.315091138043)) ;
#128350=CARTESIAN_POINT('Ctrl Pts',(-28.2010132389493,13.0574724687543,
127.366009013332)) ;
#128351=CARTESIAN_POINT('Ctrl Pts',(-28.2554093381646,12.7770677304932,
127.49174771629)) ;
#128352=CARTESIAN_POINT('Ctrl Pts',(-28.3326365056277,12.5427865194022,
127.684105622645)) ;
#128353=CARTESIAN_POINT('Ctrl Pts',(-28.426700494125,12.3731888439483,127.925946135446)) ;
#128354=CARTESIAN_POINT('Ctrl Pts',(-28.5329415022504,12.2773794382998,
128.203152444927)) ;
#128355=CARTESIAN_POINT('Ctrl Pts',(-28.6442054584027,12.2641879645069,
128.494964474125)) ;
#128356=CARTESIAN_POINT('Ctrl Pts',(-28.7522728606296,12.3335960528712,
128.777660872691)) ;
#128357=CARTESIAN_POINT('Ctrl Pts',(-28.8515196262173,12.4815616516049,
129.034375425197)) ;
#128358=CARTESIAN_POINT('Ctrl Pts',(-28.9346047736369,12.6968287193189,
129.243965291323)) ;
#128359=CARTESIAN_POINT('Ctrl Pts',(-28.9966007920383,12.9642190193072,
129.391928972392)) ;
#128360=CARTESIAN_POINT('Ctrl Pts',(-29.033760876432,13.2637554960381,129.467423408639)) ;
#128361=CARTESIAN_POINT('Ctrl Pts',(-29.0441746643463,13.5766923878532,
129.464563129082)) ;
#128362=CARTESIAN_POINT('Ctrl Pts',(-29.0279267762062,13.875372212648,129.384186726206)) ;
#128363=CARTESIAN_POINT('Ctrl Pts',(-28.9866159966681,14.1446745454968,
129.230246450064)) ;
#128364=CARTESIAN_POINT('Ctrl Pts',(-28.9242657580172,14.3606486125631,
129.015033986799)) ;
#128365=CARTESIAN_POINT('Ctrl Pts',(-28.8459541094201,14.5100785842148,
128.753160853726)) ;
#128366=CARTESIAN_POINT('Ctrl Pts',(-28.7575144988308,14.581577583442,128.46153769434)) ;
#128367=CARTESIAN_POINT('Ctrl Pts',(-28.6673238167247,14.5700419857243,
128.165121807893)) ;
#128368=CARTESIAN_POINT('Ctrl Pts',(-28.58097543859,14.4761037677004,127.879636404591)) ;
#128369=CARTESIAN_POINT('Ctrl Pts',(-28.5065773394975,14.3074346492421,
127.629266918375)) ;
#128370=CARTESIAN_POINT('Ctrl Pts',(-28.4493300740461,14.0735726196759,
127.428724095027)) ;
#128371=CARTESIAN_POINT('Ctrl Pts',(-28.4149758226597,13.7966474612173,
127.295512809063)) ;
#128372=CARTESIAN_POINT('Ctrl Pts',(-28.4058187870782,13.4894705422107,
127.235477170096)) ;
#128373=CARTESIAN_POINT('Ctrl Pts',(-28.4236271856564,13.1800818443726,
127.254513000672)) ;
#128374=CARTESIAN_POINT('Ctrl Pts',(-28.4681605342844,12.8853356216509,
127.351294313502)) ;
#128375=CARTESIAN_POINT('Ctrl Pts',(-28.5362090045899,12.6318026022688,
127.517091172939)) ;
#128376=CARTESIAN_POINT('Ctrl Pts',(-28.6242035815314,12.4337108519891,
127.741021478077)) ;
#128377=CARTESIAN_POINT('Ctrl Pts',(-28.7265451726035,12.3064394714406,
128.006839090709)) ;
#128378=CARTESIAN_POINT('Ctrl Pts',(-28.8366368301537,12.2594672533841,
128.29525608479)) ;
#128379=CARTESIAN_POINT('Ctrl Pts',(-28.9466338123818,12.2954707769561,
128.583576517785)) ;
#128380=CARTESIAN_POINT('Ctrl Pts',(-29.0509389176622,12.4135506751844,
128.854927659037)) ;
#128381=CARTESIAN_POINT('Ctrl Pts',(-29.1403897390576,12.6014761711869,
129.083399778371)) ;
#128382=CARTESIAN_POINT('Ctrl Pts',(-29.2118568087512,12.8505488628237,
129.258907374417)) ;
#128383=CARTESIAN_POINT('Ctrl Pts',(-29.2593420955227,13.1393106619413,
129.364567360262)) ;
#128384=CARTESIAN_POINT('Ctrl Pts',(-29.2808077434692,13.4495612623856,
129.394071968734)) ;
#128385=CARTESIAN_POINT('Ctrl Pts',(-29.2752058123139,13.756653092605,129.344650587175)) ;
#128386=CARTESIAN_POINT('Ctrl Pts',(-29.2437772223513,14.0404143429371,
129.219716781372)) ;
#128387=CARTESIAN_POINT('Ctrl Pts',(-29.1895572127953,14.279856789825,129.0282438534)) ;
#128388=CARTESIAN_POINT('Ctrl Pts',(-29.1165343233898,14.458860778503,128.781619840087)) ;
#128389=CARTESIAN_POINT('Ctrl Pts',(-29.031917285075,14.5622468104248,128.501448866349)) ;
#128390=CARTESIAN_POINT('Ctrl Pts',(-28.9413153955084,14.5847589311911,
128.20360102239)) ;
#128391=CARTESIAN_POINT('Ctrl Pts',(-28.852659173099,14.5239999496504,127.911543146827)) ;
#128392=CARTESIAN_POINT('Ctrl Pts',(-28.7725575058144,14.3842926160759,
127.644392979789)) ;
#128393=CARTESIAN_POINT('Ctrl Pts',(-28.7077697133043,14.1758059361387,
127.42201331714)) ;
#128394=CARTESIAN_POINT('Ctrl Pts',(-28.6635064080337,13.9130884623637,
127.259547291412)) ;
#128395=CARTESIAN_POINT('Ctrl Pts',(-28.6438464264205,13.6151580257587,
127.168954786691)) ;
#128396=CARTESIAN_POINT('Ctrl Pts',(-28.6507323999107,13.3050554492312,
127.156078639561)) ;
#128397=CARTESIAN_POINT('Ctrl Pts',(-28.6844706073222,13.0018871941951,
127.221480450194)) ;
#128398=CARTESIAN_POINT('Ctrl Pts',(-28.7434079227776,12.7291798147193,
127.360525108011)) ;
#128399=CARTESIAN_POINT('Ctrl Pts',(-28.8240272464479,12.5061726886818,
127.562903271445)) ;
#128400=CARTESIAN_POINT('Ctrl Pts',(-28.9211857020816,12.3489726322612,
127.813628136945)) ;
#128401=CARTESIAN_POINT('Ctrl Pts',(-29.0288509697157,12.2685650125514,
128.095007724897)) ;
#128402=CARTESIAN_POINT('Ctrl Pts',(-29.1398395878935,12.2709027437165,
128.386124146203)) ;
#128403=CARTESIAN_POINT('Ctrl Pts',(-29.2471199620601,12.3558100296643,
128.666375223964)) ;
#128404=CARTESIAN_POINT('Ctrl Pts',(-29.3435765060887,12.5172181925544,
128.915021176286)) ;
#128405=CARTESIAN_POINT('Ctrl Pts',(-29.4230016530534,12.7432705327431,
129.113946346094)) ;
#128406=CARTESIAN_POINT('Ctrl Pts',(-29.4806020538058,13.0180147425716,
129.249103251234)) ;
#128407=CARTESIAN_POINT('Ctrl Pts',(-29.5129367891446,13.3228199509295,
129.310342652135)) ;
#128408=CARTESIAN_POINT('Ctrl Pts',(-29.5182457127061,13.6334362143055,
129.292785636343)) ;
#128409=CARTESIAN_POINT('Ctrl Pts',(-29.4970691972156,13.9294163259488,
129.197808986286)) ;
#128410=CARTESIAN_POINT('Ctrl Pts',(-29.4516279224043,14.18915702975,129.031962445103)) ;
#128411=CARTESIAN_POINT('Ctrl Pts',(-29.38555463668,14.3946402056162,128.805710456645)) ;
#128412=CARTESIAN_POINT('Ctrl Pts',(-29.3051006300722,14.5295568967571,
128.537671661422)) ;
#128413=CARTESIAN_POINT('Ctrl Pts',(-29.2156162984668,14.5858061312981,
128.24299020634)) ;
#128414=CARTESIAN_POINT('Ctrl Pts',(-29.1256218105219,14.5585141748975,
127.947102079717)) ;
#128415=CARTESIAN_POINT('Ctrl Pts',(-29.0411499046358,14.4500372195652,
127.6671917137)) ;
#128416=CARTESIAN_POINT('Ctrl Pts',(-28.9695106659263,14.268202021056,127.424830618279)) ;
#128417=CARTESIAN_POINT('Ctrl Pts',(-28.916234737592,14.0250734165881,127.23599524268)) ;
#128418=CARTESIAN_POINT('Ctrl Pts',(-28.886235807132,13.7389393522913,127.115203743576)) ;
#128419=CARTESIAN_POINT('Ctrl Pts',(-28.8822715294914,13.4311037013635,
127.070559670291)) ;
#128420=CARTESIAN_POINT('Ctrl Pts',(-28.9050595797916,13.1229020286871,
127.104098985504)) ;
#128421=CARTESIAN_POINT('Ctrl Pts',(-28.9545277915126,12.8333723840705,
127.215232014648)) ;
#128422=CARTESIAN_POINT('Ctrl Pts',(-29.0265929326767,12.5895126798869,
127.392798802451)) ;
#128423=CARTESIAN_POINT('Ctrl Pts',(-29.1179608932549,12.4035405009807,
127.626511481168)) ;
#128424=CARTESIAN_POINT('Ctrl Pts',(-29.2220069817726,12.2914040510789,
127.897399185991)) ;
#128425=CARTESIAN_POINT('Ctrl Pts',(-29.3324362163145,12.2598122659222,
128.186893232235)) ;
#128426=CARTESIAN_POINT('Ctrl Pts',(-29.4422937713978,12.3118570167027,
128.474622048651)) ;
#128427=CARTESIAN_POINT('Ctrl Pts',(-29.543658306718,12.4430958660728,128.737686840452)) ;
#128428=CARTESIAN_POINT('Ctrl Pts',(-29.6307859317786,12.6447072426792,
128.959070012672)) ;
#128429=CARTESIAN_POINT('Ctrl Pts',(-29.6979080984891,12.9030426920416,
129.121922285674)) ;
#128430=CARTESIAN_POINT('Ctrl Pts',(-29.7405762601076,13.1970328957413,
129.21353301064)) ;
#128431=CARTESIAN_POINT('Ctrl Pts',(-29.7568965621962,13.5084312803207,
129.228029321592)) ;
#128432=CARTESIAN_POINT('Ctrl Pts',(-29.7463599115322,13.8121187578149,
129.164257165231)) ;
#128433=CARTESIAN_POINT('Ctrl Pts',(-29.7101954494671,14.0900961815241,
129.025358610877)) ;
#128434=CARTESIAN_POINT('Ctrl Pts',(-29.6521594765737,14.318729906323,128.822783597689)) ;
#128435=CARTESIAN_POINT('Ctrl Pts',(-29.5763427713784,14.4844226904234,
128.568010036296)) ;
#128436=CARTESIAN_POINT('Ctrl Pts',(-29.4902471364353,14.5727758768623,
128.283555618442)) ;
#128437=CARTESIAN_POINT('Ctrl Pts',(-29.3994772571984,14.5796460537581,
127.985241974566)) ;
#128438=CARTESIAN_POINT('Ctrl Pts',(-29.3118586977747,14.5035865884274,
127.696186441973)) ;
#128439=CARTESIAN_POINT('Ctrl Pts',(-29.2340134258281,14.3497063605797,
127.435569924992)) ;
#128440=CARTESIAN_POINT('Ctrl Pts',(-29.1726986774846,14.1291330540675,
127.223271531018)) ;
#128441=CARTESIAN_POINT('Ctrl Pts',(-29.1330506360304,13.8597727323871,
127.074476720364)) ;
#128442=CARTESIAN_POINT('Ctrl Pts',(-29.1181810101493,13.5574624461298,
126.997854047056)) ;
#128443=CARTESIAN_POINT('Ctrl Pts',(-29.1301796266018,13.2463366204199,
126.999819620482)) ;
#128444=CARTESIAN_POINT('Ctrl Pts',(-29.168925343338,12.9472974044437,127.079846391549)) ;
#128445=CARTESIAN_POINT('Ctrl Pts',(-29.2320422705623,12.6832078495132,
127.231196082457)) ;
#128446=CARTESIAN_POINT('Ctrl Pts',(-29.3166522738459,12.4704982882043,
127.44506697642)) ;
#128447=CARTESIAN_POINT('Ctrl Pts',(-29.4160388288635,12.3276823498278,
127.702394373232)) ;
#128448=CARTESIAN_POINT('Ctrl Pts',(-29.5249829531837,12.2625925248945,
127.987480236836)) ;
#128449=CARTESIAN_POINT('Ctrl Pts',(-29.6355718959069,12.2806192118825,
128.277501275059)) ;
#128450=CARTESIAN_POINT('Ctrl Pts',(-29.7417159522391,12.3809214505585,
128.554315315188)) ;
#128451=CARTESIAN_POINT('Ctrl Pts',(-29.8353905585785,12.5560400972574,
128.794817454638)) ;
#128452=CARTESIAN_POINT('Ctrl Pts',(-29.9107732205239,12.7918901255773,
128.9820408941)) ;
#128453=CARTESIAN_POINT('Ctrl Pts',(-29.963902573747,13.0744209582552,129.104054461065)) ;
#128454=CARTESIAN_POINT('Ctrl Pts',(-29.9911128268477,13.3812416621058,
129.150442107192)) ;
#128455=CARTESIAN_POINT('Ctrl Pts',(-29.9913457221614,13.6920797035989,
129.117909219499)) ;
#128456=CARTESIAN_POINT('Ctrl Pts',(-29.9652366276384,13.9824941706661,
129.008541028235)) ;
#128457=CARTESIAN_POINT('Ctrl Pts',(-29.9157726640117,14.2323227455577,
128.831056214545)) ;
#128458=CARTESIAN_POINT('Ctrl Pts',(-29.846427467267,14.4258243493526,128.595232400767)) ;
#128459=CARTESIAN_POINT('Ctrl Pts',(-29.7637490145916,14.5465247232896,
128.320649149057)) ;
#128460=CARTESIAN_POINT('Ctrl Pts',(-29.6735483660244,14.5869806832562,
128.023905947573)) ;
#128461=CARTESIAN_POINT('Ctrl Pts',(-29.5842319211393,14.5442058471831,
127.730036702735)) ;
#128462=CARTESIAN_POINT('Ctrl Pts',(-29.5014998391875,14.4209679601538,
127.455153408588)) ;
#128463=CARTESIAN_POINT('Ctrl Pts',(-29.4328113829598,14.2257906584797,
127.221317947719)) ;
#128464=CARTESIAN_POINT('Ctrl Pts',(-29.3838992065976,13.9741287735189,
127.045386859972)) ;
#128465=CARTESIAN_POINT('Ctrl Pts',(-29.3585749953142,13.6829512518686,
126.938330736026)) ;
#128466=CARTESIAN_POINT('Ctrl Pts',(-29.3596330007189,13.3714665393579,
126.90816420681)) ;
#128467=CARTESIAN_POINT('Ctrl Pts',(-29.3876542453033,13.0656058649526,
126.956972860961)) ;
#128468=CARTESIAN_POINT('Ctrl Pts',(-29.4412418248995,12.7850334641615,
127.080442878594)) ;
#128469=CARTESIAN_POINT('Ctrl Pts',(-29.5174858728615,12.5496673057456,
127.270047670741)) ;
#128470=CARTESIAN_POINT('Ctrl Pts',(-29.6117756090028,12.3766688601944,
127.512307064252)) ;
#128471=CARTESIAN_POINT('Ctrl Pts',(-29.7177855631625,12.2789529253499,
127.788850188799)) ;
#128472=CARTESIAN_POINT('Ctrl Pts',(-29.8288201491775,12.2634413511376,
128.080046508042)) ;
#128473=CARTESIAN_POINT('Ctrl Pts',(-29.9370813812663,12.330415688247,128.363307355518)) ;
#128474=CARTESIAN_POINT('Ctrl Pts',(-30.0370100677037,12.4770343788681,
128.621893210598)) ;
#128475=CARTESIAN_POINT('Ctrl Pts',(-30.1201623965983,12.6896430070817,
128.831846013391)) ;
#128476=CARTESIAN_POINT('Ctrl Pts',(-30.1828600429885,12.9554491336733,
128.981881400564)) ;
#128477=CARTESIAN_POINT('Ctrl Pts',(-30.220821672093,13.2546655218149,129.059678855952)) ;
#128478=CARTESIAN_POINT('Ctrl Pts',(-30.2320631082474,13.5672374700513,
129.059277137002)) ;
#128479=CARTESIAN_POINT('Ctrl Pts',(-30.2164917611136,13.8673527502542,
128.980779221117)) ;
#128480=CARTESIAN_POINT('Ctrl Pts',(-30.1761119033239,14.1367235720608,
128.829720800878)) ;
#128481=CARTESIAN_POINT('Ctrl Pts',(-30.1138238135701,14.3561276375805,
128.614427243316)) ;
#128482=CARTESIAN_POINT('Ctrl Pts',(-30.0362416171714,14.5065131525026,
128.354864369659)) ;
#128483=CARTESIAN_POINT('Ctrl Pts',(-29.9482255340251,14.58061768968,128.06455261143)) ;
#128484=CARTESIAN_POINT('Ctrl Pts',(-29.8577007140995,14.5715966995796,
127.767049538238)) ;
#128485=CARTESIAN_POINT('Ctrl Pts',(-29.7710937353391,14.4799160826423,
127.480801972411)) ;
#128486=CARTESIAN_POINT('Ctrl Pts',(-29.6962601987287,14.3130126299592,
127.229134217292)) ;
#128487=CARTESIAN_POINT('Ctrl Pts',(-29.6386676158855,14.0821691922297,
127.027760661239)) ;
#128488=CARTESIAN_POINT('Ctrl Pts',(-29.6033324240906,13.8046645474474,
126.891472664739)) ;
#128489=CARTESIAN_POINT('Ctrl Pts',(-29.5935128975474,13.4979411063597,
126.829511671003)) ;
#128490=CARTESIAN_POINT('Ctrl Pts',(-29.6105436734211,13.1889484059184,
126.846331182922)) ;
#128491=CARTESIAN_POINT('Ctrl Pts',(-29.6541824416548,12.8939178579835,
126.940568159584)) ;
#128492=CARTESIAN_POINT('Ctrl Pts',(-29.7218865320693,12.637823938518,127.105210089528)) ;
#128493=CARTESIAN_POINT('Ctrl Pts',(-29.8094196831743,12.4382802201008,
127.327808914552)) ;
#128494=CARTESIAN_POINT('Ctrl Pts',(-29.9109916726465,12.3092349682175,
127.591516833014)) ;
#128495=CARTESIAN_POINT('Ctrl Pts',(-30.0213393689754,12.2595575247746,
127.880567063978)) ;
#128496=CARTESIAN_POINT('Ctrl Pts',(-30.1312298450494,12.2934341304884,
128.168627556378)) ;
#128497=CARTESIAN_POINT('Ctrl Pts',(-30.2352976730363,12.4080333824313,
128.439480287819)) ;
#128498=CARTESIAN_POINT('Ctrl Pts',(-30.326263456122,12.5960960423707,128.672002337126)) ;
#128499=CARTESIAN_POINT('Ctrl Pts',(-30.3979051357112,12.8430835958632,
128.848156216935)) ;
#128500=CARTESIAN_POINT('Ctrl Pts',(-30.4460602471863,13.1299282675871,
128.955872602164)) ;
#128501=CARTESIAN_POINT('Ctrl Pts',(-30.4683932727674,13.4413370820985,
128.987758396516)) ;
#128502=CARTESIAN_POINT('Ctrl Pts',(-30.4634997449438,13.7480777778484,
128.940482113583)) ;
#128503=CARTESIAN_POINT('Ctrl Pts',(-30.4328079191952,14.0327532847483,
128.817708039455)) ;
#128504=CARTESIAN_POINT('Ctrl Pts',(-30.379231368512,14.2736050816731,128.628136710123)) ;
#128505=CARTESIAN_POINT('Ctrl Pts',(-30.3066075793135,14.454731415087,128.382652806639)) ;
#128506=CARTESIAN_POINT('Ctrl Pts',(-30.2223698139022,14.5602675657722,
128.103634816694)) ;
#128507=CARTESIAN_POINT('Ctrl Pts',(-30.1317618838712,14.5853381818847,
127.805744051885)) ;
#128508=CARTESIAN_POINT('Ctrl Pts',(-30.0428613703553,14.5268296040502,
127.512936641818)) ;
#128509=CARTESIAN_POINT('Ctrl Pts',(-29.962463860033,14.3893357844739,127.244942389594)) ;
#128510=CARTESIAN_POINT('Ctrl Pts',(-29.8971381429269,14.1825587222419,
127.020978714071)) ;
#128511=CARTESIAN_POINT('Ctrl Pts',(-29.8522544707252,13.9213688559687,
126.856729894108)) ;
#128512=CARTESIAN_POINT('Ctrl Pts',(-29.8318542419191,13.6242448062503,
126.763980055816)) ;
#128513=CARTESIAN_POINT('Ctrl Pts',(-29.8378630021939,13.3143404196874,
126.748558862791)) ;
#128514=CARTESIAN_POINT('Ctrl Pts',(-29.8712285537645,13.0084390891239,
126.812618139704)) ;
#128515=CARTESIAN_POINT('Ctrl Pts',(-29.929011094758,12.7371909250803,126.948597866911)) ;
#128516=CARTESIAN_POINT('Ctrl Pts',(-30.0093157978428,12.5114338285413,
127.149921316815)) ;
#128517=CARTESIAN_POINT('Ctrl Pts',(-30.1060566735137,12.3524149668545,
127.399449942956)) ;
#128518=CARTESIAN_POINT('Ctrl Pts',(-30.2136485926951,12.2696328079286,
127.680573993983)) ;
#128519=CARTESIAN_POINT('Ctrl Pts',(-30.3245815643694,12.2697667262583,
127.971545918026)) ;
#128520=CARTESIAN_POINT('Ctrl Pts',(-30.4318960813969,12.352219690353,128.251950244621)) ;
#128521=CARTESIAN_POINT('Ctrl Pts',(-30.5288090204638,12.5116177208884,
128.501911593616)) ;
#128522=CARTESIAN_POINT('Ctrl Pts',(-30.6088324049079,12.7360826900141,
128.702573395884)) ;
#128523=CARTESIAN_POINT('Ctrl Pts',(-30.6672434975921,13.0105746787141,
128.840001522892)) ;
#128524=CARTESIAN_POINT('Ctrl Pts',(-30.7001840342553,13.3146278251872,
128.903042642514)) ;
#128525=CARTESIAN_POINT('Ctrl Pts',(-30.7062603799839,13.6243831521928,
128.887830433908)) ;
#128526=CARTESIAN_POINT('Ctrl Pts',(-30.6857673468596,13.9217978,128.794770598986)) ;
#128527=CARTESIAN_POINT('Ctrl Pts',(-30.6410536399538,14.1821018146301,
128.631134773941)) ;
#128528=CARTESIAN_POINT('Ctrl Pts',(-30.5756154839279,14.389412327527,128.406768739336)) ;
#128529=CARTESIAN_POINT('Ctrl Pts',(-30.4952269467035,14.5268848285114,
128.138811005496)) ;
#128530=CARTESIAN_POINT('Ctrl Pts',(-30.4061762996858,14.5852561648766,
127.845506483541)) ;
#128531=CARTESIAN_POINT('Ctrl Pts',(-30.3160687878258,14.5605921402289,
127.54927187433)) ;
#128532=CARTESIAN_POINT('Ctrl Pts',(-30.2312252040183,14.4542388550499,
127.268234257609)) ;
#128533=CARTESIAN_POINT('Ctrl Pts',(-30.1590863849219,14.2743936343232,
127.024407772696)) ;
#128534=CARTESIAN_POINT('Ctrl Pts',(-30.105107623007,14.0316377250169,126.833390090339)) ;
#128535=CARTESIAN_POINT('Ctrl Pts',(-30.074596777505,13.7487556151288,126.711369355274)) ;
#128536=CARTESIAN_POINT('Ctrl Pts',(-30.0698043518736,13.4387761363986,
126.664030655711)) ;
#128537=CARTESIAN_POINT('Ctrl Pts',(-30.0918266077804,13.1317846555727,
126.695496010489)) ;
#128538=CARTESIAN_POINT('Ctrl Pts',(-30.1405764170373,12.8410201879509,
126.804495127875)) ;
#128539=CARTESIAN_POINT('Ctrl Pts',(-30.2118505192796,12.5963885995688,
126.97984040817)) ;
#128540=CARTESIAN_POINT('Ctrl Pts',(-30.3025467713188,12.4083250165559,
127.211632452948)) ;
#128541=CARTESIAN_POINT('Ctrl Pts',(-30.4070074692118,12.2932606232103,
127.483511429842)) ;
#128542=CARTESIAN_POINT('Ctrl Pts',(-30.5168319442806,12.2596773192959,
127.771399740132)) ;
#128543=CARTESIAN_POINT('Ctrl Pts',(-30.6267559112214,12.3089369828892,
128.05934301133)) ;
#128544=CARTESIAN_POINT('Ctrl Pts',(-30.7288700245111,12.4384179061081,
128.324470423332)) ;
#128545=CARTESIAN_POINT('Ctrl Pts',(-30.8165456041534,12.6389284410988,
128.547392027086)) ;
#128546=CARTESIAN_POINT('Ctrl Pts',(-30.8838110091402,12.893636868565,128.710941823021)) ;
#128547=CARTESIAN_POINT('Ctrl Pts',(-30.9276213515713,13.1890353043008,
128.805628637926)) ;
#128548=CARTESIAN_POINT('Ctrl Pts',(-30.9445789357736,13.4997523656822,
128.822052819352)) ;
#128549=CARTESIAN_POINT('Ctrl Pts',(-30.9347706434733,13.8039808891053,
128.760392828068)) ;
#128550=CARTESIAN_POINT('Ctrl Pts',(-30.8994647064315,14.0820721620834,
128.624129866457)) ;
#128551=CARTESIAN_POINT('Ctrl Pts',(-30.8418621446897,14.3130040763869,
128.422725422754)) ;
#128552=CARTESIAN_POINT('Ctrl Pts',(-30.7668395761858,14.4800545179009,
128.170430933106)) ;
#128553=CARTESIAN_POINT('Ctrl Pts',(-30.680746802464,14.5714591887958,127.885882008623)) ;
#128554=CARTESIAN_POINT('Ctrl Pts',(-30.5895443226898,14.5804983866051,
127.586142612422)) ;
#128555=CARTESIAN_POINT('Ctrl Pts',(-30.5021757835081,14.5069052438345,
127.297974852668)) ;
#128556=CARTESIAN_POINT('Ctrl Pts',(-30.4240484083233,14.3557029930728,
127.036595527731)) ;
#128557=CARTESIAN_POINT('Ctrl Pts',(-30.3620588834699,14.1367619821381,
126.822288296533)) ;
#128558=CARTESIAN_POINT('Ctrl Pts',(-30.3216036763726,13.868069374817,126.671065060371)) ;
#128559=CARTESIAN_POINT('Ctrl Pts',(-30.3060292758437,13.5652242868234,
126.592265896191)) ;
#128560=CARTESIAN_POINT('Ctrl Pts',(-30.3172275810128,13.2558696695954,
126.592085413816)) ;
#128561=CARTESIAN_POINT('Ctrl Pts',(-30.3551569478567,12.9557646560496,
126.669693553558)) ;
#128562=CARTESIAN_POINT('Ctrl Pts',(-30.4177746688459,12.6900042149153,
126.819521572026)) ;
#128563=CARTESIAN_POINT('Ctrl Pts',(-30.5015283801077,12.4761055498728,
127.031005340898)) ;
#128564=CARTESIAN_POINT('Ctrl Pts',(-30.6010714282225,12.3304586673531,
127.288616121173)) ;
#128565=CARTESIAN_POINT('Ctrl Pts',(-30.7093303383292,12.2634381617438,
127.571864331077)) ;
#128566=CARTESIAN_POINT('Ctrl Pts',(-30.8202059528667,12.278878358219,127.862647845452)) ;
#128567=CARTESIAN_POINT('Ctrl Pts',(-30.9264645765518,12.3768659810513,
128.139835217685)) ;
#128568=CARTESIAN_POINT('Ctrl Pts',(-31.020570079013,12.5495630151977,128.381622987538)) ;
#128569=CARTESIAN_POINT('Ctrl Pts',(-31.0969863841414,12.7855771404834,
128.571643774732)) ;
#128570=CARTESIAN_POINT('Ctrl Pts',(-31.1504119228565,13.0654345066809,
128.694731648829)) ;
#128571=CARTESIAN_POINT('Ctrl Pts',(-31.178486934808,13.3720089206918,128.743618229046)) ;
#128572=CARTESIAN_POINT('Ctrl Pts',(-31.1795061531803,13.682435682329,128.713449748328)) ;
#128573=CARTESIAN_POINT('Ctrl Pts',(-31.1542831813261,13.9739144742565,
128.606673201807)) ;
#128574=CARTESIAN_POINT('Ctrl Pts',(-31.1049759678819,14.2268633708939,
128.429387198208)) ;
#128575=CARTESIAN_POINT('Ctrl Pts',(-31.0367913472421,14.4204385553042,
128.197281287674)) ;
#128576=CARTESIAN_POINT('Ctrl Pts',(-30.9536916763409,14.5445800987763,
127.921159574163)) ;
#128577=CARTESIAN_POINT('Ctrl Pts',(-30.864182473291,14.5868220518321,127.626665385691)) ;
#128578=CARTESIAN_POINT('Ctrl Pts',(-30.7745931280078,14.5468039105965,
127.331938979369)) ;
#128579=CARTESIAN_POINT('Ctrl Pts',(-30.6912840406938,14.4251034051228,
127.055252613028)) ;
#128580=CARTESIAN_POINT('Ctrl Pts',(-30.6224350856795,14.2325286580178,
126.821087436355)) ;
#128581=CARTESIAN_POINT('Ctrl Pts',(-30.5727594385633,13.9823226151408,
126.642904834629)) ;
#128582=CARTESIAN_POINT('Ctrl Pts',(-30.5466732188835,13.6900857770298,
126.533419749319)) ;
#128583=CARTESIAN_POINT('Ctrl Pts',(-30.5470186669781,13.3811330160851,
126.501422391633)) ;
#128584=CARTESIAN_POINT('Ctrl Pts',(-30.5742267919639,13.0742212220075,
126.547788430997)) ;
#128585=CARTESIAN_POINT('Ctrl Pts',(-30.6272128351288,12.7922256015956,
126.669455909412)) ;
#128586=CARTESIAN_POINT('Ctrl Pts',(-30.7031024608963,12.5548594273492,
126.857944851666)) ;
#128587=CARTESIAN_POINT('Ctrl Pts',(-30.796900428706,12.3804086470547,127.098812566014)) ;
#128588=CARTESIAN_POINT('Ctrl Pts',(-30.9021655709172,12.2809059803651,
127.373332007797)) ;
#128589=CARTESIAN_POINT('Ctrl Pts',(-31.0130340334026,12.2624888492441,
127.664081167876)) ;
#128590=CARTESIAN_POINT('Ctrl Pts',(-31.122092423042,12.3276777056696,127.949470767987)) ;
#128591=CARTESIAN_POINT('Ctrl Pts',(-31.2215356799451,12.4707929028479,
128.206930407151)) ;
#128592=CARTESIAN_POINT('Ctrl Pts',(-31.3057861593304,12.6823314150819,
128.41991397547)) ;
#128593=CARTESIAN_POINT('Ctrl Pts',(-31.3692927733241,12.9478031848441,
128.572215489217)) ;
#128594=CARTESIAN_POINT('Ctrl Pts',(-31.4079487674031,13.2466923660168,
128.652010448141)) ;
#128595=CARTESIAN_POINT('Ctrl Pts',(-31.4198806266106,13.5583772827196,
128.653714268614)) ;
#128596=CARTESIAN_POINT('Ctrl Pts',(-31.4051154738825,13.8592556728242,
128.577564219372)) ;
#128597=CARTESIAN_POINT('Ctrl Pts',(-31.3650985633522,14.1306425332548,
128.42742562908)) ;
#128598=CARTESIAN_POINT('Ctrl Pts',(-31.3041188903048,14.3493759860233,
128.216343523251)) ;
#128599=CARTESIAN_POINT('Ctrl Pts',(-31.2263226071039,14.5035317541652,
127.955864143457)) ;
#128600=CARTESIAN_POINT('Ctrl Pts',(-31.1386623199781,14.5795845052791,
127.666673105791)) ;
#128601=CARTESIAN_POINT('Ctrl Pts',(-31.0479383571274,14.5729335586883,
127.368514322624)) ;
#128602=CARTESIAN_POINT('Ctrl Pts',(-30.9614128878974,14.4838964903463,
127.082628198769)) ;
#128603=CARTESIAN_POINT('Ctrl Pts',(-30.8859576009587,14.3187457579905,
126.829059953283)) ;
#128604=CARTESIAN_POINT('Ctrl Pts',(-30.827869755057,14.0897675929633,126.626282491058)) ;
#128605=CARTESIAN_POINT('Ctrl Pts',(-30.7918178978922,13.8134082777409,
126.487898906566)) ;
#128606=CARTESIAN_POINT('Ctrl Pts',(-30.7811885297415,13.5073936360873,
126.423595807509)) ;
#128607=CARTESIAN_POINT('Ctrl Pts',(-30.7974836212486,13.1976577168155,
126.438200350331)) ;
#128608=CARTESIAN_POINT('Ctrl Pts',(-30.8402132756921,12.9027229695694,
126.529888850786)) ;
#128609=CARTESIAN_POINT('Ctrl Pts',(-30.9073353624577,12.6448108497487,
126.692775559665)) ;
#128610=CARTESIAN_POINT('Ctrl Pts',(-30.9941421316234,12.4434495713625,
126.913315381037)) ;
#128611=CARTESIAN_POINT('Ctrl Pts',(-31.0963533136014,12.311375978469,127.1785845358)) ;
#128612=CARTESIAN_POINT('Ctrl Pts',(-31.2053832704872,12.2599503304442,
127.464153622351)) ;
#128613=CARTESIAN_POINT('Ctrl Pts',(-31.3162358384633,12.2913693228783,
127.754756534569)) ;
#128614=CARTESIAN_POINT('Ctrl Pts',(-31.4202678196451,12.4038516035479,
128.025596697049)) ;
#128615=CARTESIAN_POINT('Ctrl Pts',(-31.5114357995679,12.5892626487071,
128.258807733841)) ;
#128616=CARTESIAN_POINT('Ctrl Pts',(-31.5837749041298,12.8342966709516,
128.43702813475)) ;
#128617=CARTESIAN_POINT('Ctrl Pts',(-31.6329366574186,13.122430567382,128.547436490595)) ;
#128618=CARTESIAN_POINT('Ctrl Pts',(-31.6558392024168,13.4307504322514,
128.58129064855)) ;
#128619=CARTESIAN_POINT('Ctrl Pts',(-31.651838811182,13.7394115392885,128.53645443935)) ;
#128620=CARTESIAN_POINT('Ctrl Pts',(-31.6218261093011,14.0250582517609,
128.415667947021)) ;
#128621=CARTESIAN_POINT('Ctrl Pts',(-31.568744981883,14.2676857548662,128.227489788221)) ;
#128622=CARTESIAN_POINT('Ctrl Pts',(-31.4969069521766,14.4501343766899,
127.984446191423)) ;
#128623=CARTESIAN_POINT('Ctrl Pts',(-31.4125135319878,14.5585281665325,
127.704800678518)) ;
#128624=CARTESIAN_POINT('Ctrl Pts',(-31.3222180587387,14.5857500272389,
127.407919510387)) ;
#128625=CARTESIAN_POINT('Ctrl Pts',(-31.2330255116186,14.5296138269876,
127.114203416447)) ;
#128626=CARTESIAN_POINT('Ctrl Pts',(-31.152297925257,14.3940563657681,126.845238279208)) ;
#128627=CARTESIAN_POINT('Ctrl Pts',(-31.0866327665665,14.1896706330216,
126.620373125619)) ;
#128628=CARTESIAN_POINT('Ctrl Pts',(-31.0410079108427,13.9296795635546,
126.453929783066)) ;
#128629=CARTESIAN_POINT('Ctrl Pts',(-31.0198252619641,13.6325613783442,
126.358817925513)) ;
#128630=CARTESIAN_POINT('Ctrl Pts',(-31.0251775966313,13.3229079884786,
126.341491446272)) ;
#128631=CARTESIAN_POINT('Ctrl Pts',(-31.0574272726707,13.018526691074,126.402527072906)) ;
#128632=CARTESIAN_POINT('Ctrl Pts',(-31.1149307246031,12.7436673997071,
126.537409276898)) ;
#128633=CARTESIAN_POINT('Ctrl Pts',(-31.1948445839553,12.5164978954953,
126.737575762028)) ;
#128634=CARTESIAN_POINT('Ctrl Pts',(-31.2908244908384,12.3560840259889,
126.985005769363)) ;
#128635=CARTESIAN_POINT('Ctrl Pts',(-31.3982222730911,12.2708854791944,
127.265554907763)) ;
#128636=CARTESIAN_POINT('Ctrl Pts',(-31.5090110903784,12.2685612121641,
127.556147236131)) ;
#128637=CARTESIAN_POINT('Ctrl Pts',(-31.6167270045284,12.3486009748257,
127.837672372458)) ;
#128638=CARTESIAN_POINT('Ctrl Pts',(-31.7143963508923,12.5069430780995,
128.089696718975)) ;
#128639=CARTESIAN_POINT('Ctrl Pts',(-31.7944473102828,12.7284059514765,
128.290650681508)) ;
#128640=CARTESIAN_POINT('Ctrl Pts',(-31.8537556036786,13.0024845577893,
128.430595808369)) ;
#128641=CARTESIAN_POINT('Ctrl Pts',(-31.8873667080622,13.3053156304276,
128.495676226259)) ;
#128642=CARTESIAN_POINT('Ctrl Pts',(-31.8942276117398,13.6156286955051,
128.482698931289)) ;
#128643=CARTESIAN_POINT('Ctrl Pts',(-31.874614953271,13.9128849931579,128.392322884504)) ;
#128644=CARTESIAN_POINT('Ctrl Pts',(-31.8301744732298,14.1766185287715,
128.229209877233)) ;
#128645=CARTESIAN_POINT('Ctrl Pts',(-31.7652924085922,14.3847398624139,
128.00655809334)) ;
#128646=CARTESIAN_POINT('Ctrl Pts',(-31.6855395448521,14.5238361005913,
127.740570860147)) ;
#128647=CARTESIAN_POINT('Ctrl Pts',(-31.5967590744194,14.5847743012247,
127.448098544404)) ;
#128648=CARTESIAN_POINT('Ctrl Pts',(-31.506226561888,14.5623309410939,127.150482506814)) ;
#128649=CARTESIAN_POINT('Ctrl Pts',(-31.4212470448233,14.4584178167976,
126.869109281522)) ;
#128650=CARTESIAN_POINT('Ctrl Pts',(-31.3484135635736,14.2791868777477,
126.623076819461)) ;
#128651=CARTESIAN_POINT('Ctrl Pts',(-31.2945026699446,14.0415187113142,
126.43273117346)) ;
#128652=CARTESIAN_POINT('Ctrl Pts',(-31.2628395727632,13.7564325349983,
126.306943352975)) ;
#128653=CARTESIAN_POINT('Ctrl Pts',(-31.2573021812649,13.4495648560064,
126.25774099448)) ;
#128654=CARTESIAN_POINT('Ctrl Pts',(-31.2787325571399,13.1394167838631,
126.287153636745)) ;
#128655=CARTESIAN_POINT('Ctrl Pts',(-31.3262043092987,12.8508801265976,
126.392794087326)) ;
#128656=CARTESIAN_POINT('Ctrl Pts',(-31.3973555378242,12.6022770159485,
126.567478978667)) ;
#128657=CARTESIAN_POINT('Ctrl Pts',(-31.4875544873303,12.4127865779696,
126.797861062289)) ;
#128658=CARTESIAN_POINT('Ctrl Pts',(-31.5916801030867,12.2953916612225,
127.068766817743)) ;
#128659=CARTESIAN_POINT('Ctrl Pts',(-31.7016585324409,12.2594835082488,
127.357036513685)) ;
#128660=CARTESIAN_POINT('Ctrl Pts',(-31.8114792326934,12.3065006906036,
127.644739812586)) ;
#128661=CARTESIAN_POINT('Ctrl Pts',(-31.9136506042724,12.4331949897075,
127.910131486488)) ;
#128662=CARTESIAN_POINT('Ctrl Pts',(-32.0021581499909,12.6325251060339,
128.135361000495)) ;
#128663=CARTESIAN_POINT('Ctrl Pts',(-32.0699206406892,12.8854153923965,
128.300428648216)) ;
#128664=CARTESIAN_POINT('Ctrl Pts',(-32.1145088127622,13.1803566705807,
128.397344288992)) ;
#128665=CARTESIAN_POINT('Ctrl Pts',(-32.1322228503466,13.4893561125358,
128.416143886401)) ;
#128666=CARTESIAN_POINT('Ctrl Pts',(-32.1232591607492,13.7954470549273,
128.3568066441)) ;
#128667=CARTESIAN_POINT('Ctrl Pts',(-32.0884938852697,14.0751705086754,
128.222048043325)) ;
#128668=CARTESIAN_POINT('Ctrl Pts',(-32.0316136936814,14.3069080353192,
128.022850396701)) ;
#128669=CARTESIAN_POINT('Ctrl Pts',(-31.9571154459696,14.4762412985565,
127.772108801005)) ;
#128670=CARTESIAN_POINT('Ctrl Pts',(-31.8705406479889,14.5702449672957,
127.485888969575)) ;
#128671=CARTESIAN_POINT('Ctrl Pts',(-31.7802131912547,14.5813885693018,
127.18902186086)) ;
#128672=CARTESIAN_POINT('Ctrl Pts',(-31.6921805635413,14.5100796907114,
126.898736602283)) ;
#128673=CARTESIAN_POINT('Ctrl Pts',(-31.6135814334297,14.3602445312062,
126.635913485129)) ;
#128674=CARTESIAN_POINT('Ctrl Pts',(-31.5512501881816,14.143253231573,126.420675039755)) ;
#128675=CARTESIAN_POINT('Ctrl Pts',(-31.5102927844524,13.8766590298569,
126.268096359863)) ;
#128676=CARTESIAN_POINT('Ctrl Pts',(-31.4938914974148,13.575471217549,126.186984552435)) ;
#128677=CARTESIAN_POINT('Ctrl Pts',(-31.5042851715475,13.2645668941717,
126.184291805469)) ;
#128678=CARTESIAN_POINT('Ctrl Pts',(-31.5416101926573,12.9634277851347,
126.260085507192)) ;
#128679=CARTESIAN_POINT('Ctrl Pts',(-31.603403047589,12.6972349094739,126.407598556958)) ;
#128680=CARTESIAN_POINT('Ctrl Pts',(-31.6864963503388,12.4817230619034,
126.617187473906)) ;
#128681=CARTESIAN_POINT('Ctrl Pts',(-31.7855804706592,12.3338051971936,
126.873476664401)) ;
#128682=CARTESIAN_POINT('Ctrl Pts',(-31.8940109328035,12.2641456022445,
127.157120420535)) ;
#128683=CARTESIAN_POINT('Ctrl Pts',(-32.0048441796899,12.2773535712523,
127.447802163778)) ;
#128684=CARTESIAN_POINT('Ctrl Pts',(-32.1110952849965,12.3726334671979,
127.725051534391)) ;
#128685=CARTESIAN_POINT('Ctrl Pts',(-32.2057756328295,12.5434758401697,
127.968470739376)) ;
#128686=CARTESIAN_POINT('Ctrl Pts',(-32.2825877687635,12.7769497642035,
128.159760257596)) ;
#128687=CARTESIAN_POINT('Ctrl Pts',(-32.3370473742439,13.0568799766939,
128.285720331795)) ;
#128688=CARTESIAN_POINT('Ctrl Pts',(-32.3658593623225,13.3636449455261,
128.336699481122)) ;
#128689=CARTESIAN_POINT('Ctrl Pts',(-32.367624242602,13.6733774469028,128.308803267629)) ;
#128690=CARTESIAN_POINT('Ctrl Pts',(-32.3432185179846,13.9654380896254,
128.204448266785)) ;
#128691=CARTESIAN_POINT('Ctrl Pts',(-32.2945201685348,14.220301269476,128.028893057304)) ;
#128692=CARTESIAN_POINT('Ctrl Pts',(-32.2266394712445,14.415947045335,127.797606163458)) ;
#128693=CARTESIAN_POINT('Ctrl Pts',(-32.1443774332964,14.5416943673476,
127.524134752044)) ;
#128694=CARTESIAN_POINT('Ctrl Pts',(-32.0546246272659,14.586901890039,127.228790865626)) ;
#128695=CARTESIAN_POINT('Ctrl Pts',(-31.9648061180443,14.5489491303822,
126.933344138451)) ;
#128696=CARTESIAN_POINT('Ctrl Pts',(-31.8814753129527,14.4300240451422,
126.656711926884)) ;
#128697=CARTESIAN_POINT('Ctrl Pts',(-31.8118574558951,14.2387296185005,
126.420176396939)) ;
#128698=CARTESIAN_POINT('Ctrl Pts',(-31.761673966027,13.9899469010905,126.24053385049)) ;
#128699=CARTESIAN_POINT('Ctrl Pts',(-31.7349367720515,13.7002922366985,
126.129329442407)) ;
#128700=CARTESIAN_POINT('Ctrl Pts',(-31.7343309734707,13.3909003145637,
126.094475834364)) ;
#128701=CARTESIAN_POINT('Ctrl Pts',(-31.7609570476832,13.0819914408663,
126.138968768874)) ;
#128702=CARTESIAN_POINT('Ctrl Pts',(-31.8131240309607,12.8000707339927,
126.258359081467)) ;
#128703=CARTESIAN_POINT('Ctrl Pts',(-31.888138344661,12.5616134870626,126.444378873037)) ;
#128704=CARTESIAN_POINT('Ctrl Pts',(-31.9816543195415,12.384449895012,126.684347395518)) ;
#128705=CARTESIAN_POINT('Ctrl Pts',(-32.0872024405474,12.2824628240901,
126.959534123693)) ;
#128706=CARTESIAN_POINT('Ctrl Pts',(-32.1974420894517,12.2618989594336,
127.24862212855)) ;
#128707=CARTESIAN_POINT('Ctrl Pts',(-32.3067993093919,12.3245801439636,
127.534843652708)) ;
#128708=CARTESIAN_POINT('Ctrl Pts',(-32.4066055596616,12.4655889841413,
127.793363677931)) ;
#128709=CARTESIAN_POINT('Ctrl Pts',(-32.4913685339639,12.6753258327154,
128.007846379507)) ;
#128710=CARTESIAN_POINT('Ctrl Pts',(-32.5554823861655,12.9389695306945,
128.16198128378)) ;
#128711=CARTESIAN_POINT('Ctrl Pts',(-32.5949571555968,13.2377441429055,
128.244099164765)) ;
#128712=CARTESIAN_POINT('Ctrl Pts',(-32.6077198111152,13.5478077720715,
128.248401750288)) ;
#128713=CARTESIAN_POINT('Ctrl Pts',(-32.5936618530778,13.8515135114459,
128.17407137325)) ;
#128714=CARTESIAN_POINT('Ctrl Pts',(-32.5544078906928,14.1231097110526,
128.026278350984)) ;
#128715=CARTESIAN_POINT('Ctrl Pts',(-32.4939018766822,14.3439546593352,
127.816519602292)) ;
#128716=CARTESIAN_POINT('Ctrl Pts',(-32.4167043659917,14.4998916999394,
127.557878330328)) ;
#128717=CARTESIAN_POINT('Ctrl Pts',(-32.3289439608214,14.5786386436238,
127.268277216763)) ;
#128718=CARTESIAN_POINT('Ctrl Pts',(-32.2382575988989,14.5742675055765,
126.970251402823)) ;
#128719=CARTESIAN_POINT('Ctrl Pts',(-32.1514513694804,14.4873447057953,
126.683513861479)) ;
#128720=CARTESIAN_POINT('Ctrl Pts',(-32.0758339074813,14.324791387065,126.429581664298)) ;
#128721=CARTESIAN_POINT('Ctrl Pts',(-32.0169662101716,14.0970302215938,
126.22444258051)) ;
#128722=CARTESIAN_POINT('Ctrl Pts',(-31.9801979886195,13.8204923791666,
126.083834586045)) ;
#128723=CARTESIAN_POINT('Ctrl Pts',(-31.9689269120259,13.5164549549645,
126.017822987684)) ;
#128724=CARTESIAN_POINT('Ctrl Pts',(-31.9844450832782,13.2060699844781,
126.030100813649)) ;
#128725=CARTESIAN_POINT('Ctrl Pts',(-32.0265116602543,12.9102232608784,
126.119833944972)) ;
#128726=CARTESIAN_POINT('Ctrl Pts',(-32.0931565382583,12.6507291621381,
126.281277357209)) ;
#128727=CARTESIAN_POINT('Ctrl Pts',(-32.1791862247539,12.4485585677655,
126.499672075653)) ;
#128728=CARTESIAN_POINT('Ctrl Pts',(-32.2805050319855,12.3145373825205,
126.762496297742)) ;
#128729=CARTESIAN_POINT('Ctrl Pts',(-32.3900324574915,12.2601564012495,
127.049323626435)) ;
#128730=CARTESIAN_POINT('Ctrl Pts',(-32.5009231094152,12.2893926145907,
127.34004832186)) ;
#128731=CARTESIAN_POINT('Ctrl Pts',(-32.6052118557404,12.3994366582283,
127.611652113728)) ;
#128732=CARTESIAN_POINT('Ctrl Pts',(-32.6971979489033,12.5839727611718,
127.847103732541)) ;
#128733=CARTESIAN_POINT('Ctrl Pts',(-32.7697374400747,12.8264919442356,
128.026067460127)) ;
#128734=CARTESIAN_POINT('Ctrl Pts',(-32.8197428070764,13.1141227557289,
128.138887683343)) ;
#128735=CARTESIAN_POINT('Ctrl Pts',(-32.8354546045722,13.3194869799383,
128.162746032927)) ;
#128736=CARTESIAN_POINT('Ctrl Pts',(-32.8388677653298,13.4222384087837,
128.161696006566)) ;
#128737=CARTESIAN_POINT('Ctrl Pts',(-11.2577234899685,13.1368456608817,
133.156546946693)) ;
#128738=CARTESIAN_POINT('Ctrl Pts',(-11.2584977422668,13.1302434100695,
133.158077773235)) ;
#128739=CARTESIAN_POINT('Ctrl Pts',(-11.2711317675039,13.0249711622575,
133.183302490093)) ;
#128740=CARTESIAN_POINT('Ctrl Pts',(-11.3056487140165,12.8263018173041,
133.261160287319)) ;
#128741=CARTESIAN_POINT('Ctrl Pts',(-11.378449880765,12.5833995397257,133.440808382067)) ;
#128742=CARTESIAN_POINT('Ctrl Pts',(-11.4699936456372,12.3996267675037,
133.675124851034)) ;
#128743=CARTESIAN_POINT('Ctrl Pts',(-11.5749944367631,12.2890731746127,
133.948585197779)) ;
#128744=CARTESIAN_POINT('Ctrl Pts',(-11.6849550113911,12.2602312933653,
134.236878590562)) ;
#128745=CARTESIAN_POINT('Ctrl Pts',(-11.7947913325518,12.3144254327404,
134.524512184654)) ;
#128746=CARTESIAN_POINT('Ctrl Pts',(-11.8959713006331,12.4480642485612,
134.78699239796)) ;
#128747=CARTESIAN_POINT('Ctrl Pts',(-11.9825623500535,12.6516399128533,
135.006803074901)) ;
#128748=CARTESIAN_POINT('Ctrl Pts',(-12.048871242094,12.9104451953934,135.167384670857)) ;
#128749=CARTESIAN_POINT('Ctrl Pts',(-12.0909139091436,13.2058491339696,
135.25708775867)) ;
#128750=CARTESIAN_POINT('Ctrl Pts',(-12.1065078256121,13.5166184158111,
135.269550983787)) ;
#128751=CARTESIAN_POINT('Ctrl Pts',(-12.0950209690494,13.822409942281,135.202705290103)) ;
#128752=CARTESIAN_POINT('Ctrl Pts',(-12.0583944517229,14.0967864271645,
135.062748314668)) ;
#128753=CARTESIAN_POINT('Ctrl Pts',(-11.9996901173169,14.3244562376795,
134.858128955177)) ;
#128754=CARTESIAN_POINT('Ctrl Pts',(-11.9238941091653,14.4874741588536,
134.603594989759)) ;
#128755=CARTESIAN_POINT('Ctrl Pts',(-11.8369189889969,14.5744204782189,
134.316306456094)) ;
#128756=CARTESIAN_POINT('Ctrl Pts',(-11.746203405536,14.5784621865543,134.018183591682)) ;
#128757=CARTESIAN_POINT('Ctrl Pts',(-11.6588757290822,14.5000470189108,
133.730007295683)) ;
#128758=CARTESIAN_POINT('Ctrl Pts',(-11.5816779592207,14.3445727913024,
133.471389657961)) ;
#128759=CARTESIAN_POINT('Ctrl Pts',(-11.5208530443649,14.1228339214572,
133.260553481405)) ;
#128760=CARTESIAN_POINT('Ctrl Pts',(-11.4816410741325,13.850151796375,133.112780950454)) ;
#128761=CARTESIAN_POINT('Ctrl Pts',(-11.467692327045,13.5490424798657,133.039054244321)) ;
#128762=CARTESIAN_POINT('Ctrl Pts',(-11.4803987084794,13.2374718016147,
133.043030817363)) ;
#128763=CARTESIAN_POINT('Ctrl Pts',(-11.5199946658805,12.9386845516003,
133.125492572852)) ;
#128764=CARTESIAN_POINT('Ctrl Pts',(-11.5837788008953,12.6761377912153,
133.278810795145)) ;
#128765=CARTESIAN_POINT('Ctrl Pts',(-11.6686447392389,12.4657587239521,
133.493527758041)) ;
#128766=CARTESIAN_POINT('Ctrl Pts',(-11.7685433992697,12.3246285907277,
133.752289114269)) ;
#128767=CARTESIAN_POINT('Ctrl Pts',(-11.8778587918771,12.2619062274696,
134.038399188115)) ;
#128768=CARTESIAN_POINT('Ctrl Pts',(-11.98827945464,12.2824388238971,134.327963742059)) ;
#128769=CARTESIAN_POINT('Ctrl Pts',(-12.0940128949218,12.3848777352211,
134.603625594352)) ;
#128770=CARTESIAN_POINT('Ctrl Pts',(-12.1871312124463,12.5614991526439,
134.84255860207)) ;
#128771=CARTESIAN_POINT('Ctrl Pts',(-12.2622218143172,12.7995867932639,
135.02881848202)) ;
#128772=CARTESIAN_POINT('Ctrl Pts',(-12.3146869562127,13.0840299785093,
135.148804148266)) ;
#128773=CARTESIAN_POINT('Ctrl Pts',(-12.3409445105552,13.3899587126068,
135.192549574632)) ;
#128774=CARTESIAN_POINT('Ctrl Pts',(-12.3405172946369,13.6996411315525,
135.15818716667)) ;
#128775=CARTESIAN_POINT('Ctrl Pts',(-12.3136761245736,13.9903747332587,
135.046560923732)) ;
#128776=CARTESIAN_POINT('Ctrl Pts',(-12.263351660098,14.2393240400609,134.86646186996)) ;
#128777=CARTESIAN_POINT('Ctrl Pts',(-12.193924449354,14.4298400308443,134.630589033284)) ;
#128778=CARTESIAN_POINT('Ctrl Pts',(-12.1108448938615,14.5487685214643,
134.354775496619)) ;
#128779=CARTESIAN_POINT('Ctrl Pts',(-12.0206426776565,14.5869290459119,
134.058065629562)) ;
#128780=CARTESIAN_POINT('Ctrl Pts',(-11.9311958117229,14.5417666883846,
133.763725950696)) ;
#128781=CARTESIAN_POINT('Ctrl Pts',(-11.848852525887,14.4163781247343,133.490009785098)) ;
#128782=CARTESIAN_POINT('Ctrl Pts',(-11.7806588005147,14.2194053349132,
133.257622965532)) ;
#128783=CARTESIAN_POINT('Ctrl Pts',(-11.7323693114602,13.9666437223108,
133.0835399063)) ;
#128784=CARTESIAN_POINT('Ctrl Pts',(-11.7077161248384,13.6737230615468,
132.978341072132)) ;
#128785=CARTESIAN_POINT('Ctrl Pts',(-11.7095613308164,13.3629183562335,
132.950571917867)) ;
#128786=CARTESIAN_POINT('Ctrl Pts',(-11.7383478402933,13.0570541926124,
133.001567102361)) ;
#128787=CARTESIAN_POINT('Ctrl Pts',(-11.7926724382674,12.7772474882028,
133.127165265906)) ;
#128788=CARTESIAN_POINT('Ctrl Pts',(-11.8699199411722,12.5427680986525,
133.319560793352)) ;
#128789=CARTESIAN_POINT('Ctrl Pts',(-11.9640477954549,12.3730788782687,
133.561569728364)) ;
#128790=CARTESIAN_POINT('Ctrl Pts',(-12.0703540727819,12.2773830666973,
133.838948640795)) ;
#128791=CARTESIAN_POINT('Ctrl Pts',(-12.1812907705461,12.2641121652248,
134.129904369605)) ;
#128792=CARTESIAN_POINT('Ctrl Pts',(-12.2897321496588,12.3337583003129,
134.413576291279)) ;
#128793=CARTESIAN_POINT('Ctrl Pts',(-12.3886537440222,12.481316017211,134.669448938114)) ;
#128794=CARTESIAN_POINT('Ctrl Pts',(-12.4718652582287,12.6966779051232,
134.879370255133)) ;
#128795=CARTESIAN_POINT('Ctrl Pts',(-12.5338644427472,12.96405838434,135.027347390407)) ;
#128796=CARTESIAN_POINT('Ctrl Pts',(-12.5709815279252,13.2633620040759,
135.102737093753)) ;
#128797=CARTESIAN_POINT('Ctrl Pts',(-12.5815244475118,13.5752566966047,
135.100371228404)) ;
#128798=CARTESIAN_POINT('Ctrl Pts',(-12.5650970124809,13.8766501658651,
135.019163196537)) ;
#128799=CARTESIAN_POINT('Ctrl Pts',(-12.5240386339325,14.1438625345399,
134.866211806807)) ;
#128800=CARTESIAN_POINT('Ctrl Pts',(-12.4614606242008,14.3611557729943,
134.650168617088)) ;
#128801=CARTESIAN_POINT('Ctrl Pts',(-12.382977010877,14.5102070639316,134.387759126822)) ;
#128802=CARTESIAN_POINT('Ctrl Pts',(-12.2953587366625,14.5813677790431,
134.098836666124)) ;
#128803=CARTESIAN_POINT('Ctrl Pts',(-12.2045170609747,14.5701315167375,
133.800277368628)) ;
#128804=CARTESIAN_POINT('Ctrl Pts',(-12.1181642794546,14.4759919392145,
133.51478205914)) ;
#128805=CARTESIAN_POINT('Ctrl Pts',(-12.0436987557635,14.3066893243029,
133.264144105982)) ;
#128806=CARTESIAN_POINT('Ctrl Pts',(-11.9869151341152,14.075187939402,133.065272807165)) ;
#128807=CARTESIAN_POINT('Ctrl Pts',(-11.9522067331107,13.7962287438528,
132.930759808628)) ;
#128808=CARTESIAN_POINT('Ctrl Pts',(-11.9430693364966,13.4897393556908,
132.870870600982)) ;
#128809=CARTESIAN_POINT('Ctrl Pts',(-11.9611565578198,13.1781057377786,
132.890466222449)) ;
#128810=CARTESIAN_POINT('Ctrl Pts',(-12.0051369072121,12.8871395007703,
132.986063729264)) ;
#128811=CARTESIAN_POINT('Ctrl Pts',(-12.0735337638993,12.6313543298591,
133.152625547031)) ;
#128812=CARTESIAN_POINT('Ctrl Pts',(-12.1617954477986,12.4333423964865,
133.377283802115)) ;
#128813=CARTESIAN_POINT('Ctrl Pts',(-12.2635234037695,12.3067788295905,
133.641500686264)) ;
#128814=CARTESIAN_POINT('Ctrl Pts',(-12.373902244889,12.2592790110699,133.930667889296)) ;
#128815=CARTESIAN_POINT('Ctrl Pts',(-12.4842564290935,12.2958890741667,
134.219915229999)) ;
#128816=CARTESIAN_POINT('Ctrl Pts',(-12.5875537880349,12.412515964046,134.488658951895)) ;
#128817=CARTESIAN_POINT('Ctrl Pts',(-12.6778899409315,12.6017795231482,
134.719420077916)) ;
#128818=CARTESIAN_POINT('Ctrl Pts',(-12.7491733635404,12.8508820416093,
134.894428325394)) ;
#128819=CARTESIAN_POINT('Ctrl Pts',(-12.7966035607827,13.1389626246921,
134.999995033177)) ;
#128820=CARTESIAN_POINT('Ctrl Pts',(-12.818140672535,13.4502019068506,135.029605683406)) ;
#128821=CARTESIAN_POINT('Ctrl Pts',(-12.8124254227046,13.7571545047615,
134.97985899907)) ;
#128822=CARTESIAN_POINT('Ctrl Pts',(-12.7811740697528,14.0399279502617,
134.855572397321)) ;
#128823=CARTESIAN_POINT('Ctrl Pts',(-12.7266312200537,14.2804627240583,
134.662980887093)) ;
#128824=CARTESIAN_POINT('Ctrl Pts',(-12.6542449467316,14.4580430249791,
134.418505620157)) ;
#128825=CARTESIAN_POINT('Ctrl Pts',(-12.5692017225138,14.5623041717052,
134.136899220113)) ;
#128826=CARTESIAN_POINT('Ctrl Pts',(-12.4788691012162,14.5848738329504,
133.839946789707)) ;
#128827=CARTESIAN_POINT('Ctrl Pts',(-12.3895760994411,14.5236285487513,
133.545783898715)) ;
#128828=CARTESIAN_POINT('Ctrl Pts',(-12.3099194108957,14.3842859128116,
133.280100234544)) ;
#128829=CARTESIAN_POINT('Ctrl Pts',(-12.2450643301526,14.1760037258481,
133.057519313321)) ;
#128830=CARTESIAN_POINT('Ctrl Pts',(-12.2007227509484,13.9123646323485,
132.894723585747)) ;
#128831=CARTESIAN_POINT('Ctrl Pts',(-12.1811617332779,13.6155080091082,
132.80454288444)) ;
#128832=CARTESIAN_POINT('Ctrl Pts',(-12.1880080885275,13.3048787604148,
132.791493362742)) ;
#128833=CARTESIAN_POINT('Ctrl Pts',(-12.2218568341941,13.0013159560589,
132.857171513992)) ;
#128834=CARTESIAN_POINT('Ctrl Pts',(-12.2807527580712,12.7290185702227,
132.996137319577)) ;
#128835=CARTESIAN_POINT('Ctrl Pts',(-12.361411062945,12.5059453720444,133.198616695887)) ;
#128836=CARTESIAN_POINT('Ctrl Pts',(-12.4585666028295,12.348935712054,133.449341626127)) ;
#128837=CARTESIAN_POINT('Ctrl Pts',(-12.5660032842499,12.2685725815048,
133.730122349131)) ;
#128838=CARTESIAN_POINT('Ctrl Pts',(-12.6773948799817,12.2709800121234,
134.022294144479)) ;
#128839=CARTESIAN_POINT('Ctrl Pts',(-12.7844046898859,12.3558596886437,
134.30183548448)) ;
#128840=CARTESIAN_POINT('Ctrl Pts',(-12.8809331266172,12.5173148322773,
134.55066838557)) ;
#128841=CARTESIAN_POINT('Ctrl Pts',(-12.9604049280866,12.7436532410187,
134.749701673785)) ;
#128842=CARTESIAN_POINT('Ctrl Pts',(-13.0179363384229,13.0184389835147,
134.884661471726)) ;
#128843=CARTESIAN_POINT('Ctrl Pts',(-13.0502008445833,13.3224258162056,
134.945784440126)) ;
#128844=CARTESIAN_POINT('Ctrl Pts',(-13.0555467014002,13.6337495707095,
134.928259254628)) ;
#128845=CARTESIAN_POINT('Ctrl Pts',(-13.0343105414423,13.9298381021214,
134.8330936576)) ;
#128846=CARTESIAN_POINT('Ctrl Pts',(-12.9888314749578,14.1894305566765,
134.667140294163)) ;
#128847=CARTESIAN_POINT('Ctrl Pts',(-12.9229180456801,14.394475711673,134.441433971172)) ;
#128848=CARTESIAN_POINT('Ctrl Pts',(-12.8423867584635,14.5294751286176,
134.173134382948)) ;
#128849=CARTESIAN_POINT('Ctrl Pts',(-12.7533105459994,14.5857784674847,
133.879795104212)) ;
#128850=CARTESIAN_POINT('Ctrl Pts',(-12.6627280066615,14.5584758053027,
133.581971600338)) ;
#128851=CARTESIAN_POINT('Ctrl Pts',(-12.5784004724766,14.4499269628754,
133.302534971488)) ;
#128852=CARTESIAN_POINT('Ctrl Pts',(-12.5066920227855,14.2678362538152,
133.059930399529)) ;
#128853=CARTESIAN_POINT('Ctrl Pts',(-12.4535716004615,14.025181469635,132.871626399327)) ;
#128854=CARTESIAN_POINT('Ctrl Pts',(-12.4235648768297,13.7395989406437,
132.750864375356)) ;
#128855=CARTESIAN_POINT('Ctrl Pts',(-12.4195271153669,13.4312396287892,
132.705949634697)) ;
#128856=CARTESIAN_POINT('Ctrl Pts',(-12.4424256321316,13.1225497292761,
132.739753354196)) ;
#128857=CARTESIAN_POINT('Ctrl Pts',(-12.4915723419793,12.8344723647331,
132.850125775633)) ;
#128858=CARTESIAN_POINT('Ctrl Pts',(-12.5638932332728,12.5894057804916,
133.028292890665)) ;
#128859=CARTESIAN_POINT('Ctrl Pts',(-12.6550789543492,12.40386696018,133.261545560757)) ;
#128860=CARTESIAN_POINT('Ctrl Pts',(-12.7592412635636,12.2913271454925,
133.532726136242)) ;
#128861=CARTESIAN_POINT('Ctrl Pts',(-12.8699890943141,12.2598830910962,
133.823057346396)) ;
#128862=CARTESIAN_POINT('Ctrl Pts',(-12.9793995134526,12.3117248665292,
134.109616003847)) ;
#128863=CARTESIAN_POINT('Ctrl Pts',(-13.0810869398604,12.4432581620118,
134.373522926903)) ;
#128864=CARTESIAN_POINT('Ctrl Pts',(-13.1680418025667,12.6447767866554,
134.594446826779)) ;
#128865=CARTESIAN_POINT('Ctrl Pts',(-13.2350120772362,12.9020426127521,
134.756972372431)) ;
#128866=CARTESIAN_POINT('Ctrl Pts',(-13.2778449973924,13.1969219794908,
134.84895528723)) ;
#128867=CARTESIAN_POINT('Ctrl Pts',(-13.2942160406864,13.5073632860462,
134.863709263387)) ;
#128868=CARTESIAN_POINT('Ctrl Pts',(-13.2835289768122,13.813502723387,134.799217091499)) ;
#128869=CARTESIAN_POINT('Ctrl Pts',(-13.2476676966464,14.089063380816,134.661503408302)) ;
#128870=CARTESIAN_POINT('Ctrl Pts',(-13.1892561306851,14.319268429037,134.457595503743)) ;
#128871=CARTESIAN_POINT('Ctrl Pts',(-13.1141385106108,14.4835637196257,
134.205174492886)) ;
#128872=CARTESIAN_POINT('Ctrl Pts',(-13.0274042527108,14.5730187968723,
133.918585740495)) ;
#128873=CARTESIAN_POINT('Ctrl Pts',(-12.9366798206149,14.5795967994517,
133.620433125244)) ;
#128874=CARTESIAN_POINT('Ctrl Pts',(-12.8489781193153,14.5032854437543,
133.331090114902)) ;
#128875=CARTESIAN_POINT('Ctrl Pts',(-12.7714680695992,14.350115255618,133.071602998426)) ;
#128876=CARTESIAN_POINT('Ctrl Pts',(-12.7099485961889,14.1289953523701,
132.858606720622)) ;
#128877=CARTESIAN_POINT('Ctrl Pts',(-12.6703752161743,13.8600885343661,
132.710090425404)) ;
#128878=CARTESIAN_POINT('Ctrl Pts',(-12.6554495566048,13.5571077993043,
132.633228023965)) ;
#128879=CARTESIAN_POINT('Ctrl Pts',(-12.6675181766786,13.2461442417419,
132.635412623524)) ;
#128880=CARTESIAN_POINT('Ctrl Pts',(-12.7061242005164,12.9474785821981,
132.715086767085)) ;
#128881=CARTESIAN_POINT('Ctrl Pts',(-12.7698092342811,12.6818051231589,
132.86785971074)) ;
#128882=CARTESIAN_POINT('Ctrl Pts',(-12.8535542604601,12.4713262557242,
133.079555782508)) ;
#128883=CARTESIAN_POINT('Ctrl Pts',(-12.9535767545019,12.3273775591191,
133.338508722271)) ;
#128884=CARTESIAN_POINT('Ctrl Pts',(-13.062119391893,12.2625380497534,133.622557250429)) ;
#128885=CARTESIAN_POINT('Ctrl Pts',(-13.1735704256936,12.2810707437097,
133.914826535872)) ;
#128886=CARTESIAN_POINT('Ctrl Pts',(-13.2784207174052,12.3803128917833,
134.188268338219)) ;
#128887=CARTESIAN_POINT('Ctrl Pts',(-13.3725731541865,12.5556238817755,
134.430026844874)) ;
#128888=CARTESIAN_POINT('Ctrl Pts',(-13.4479809967805,12.7914916788268,
134.617325799491)) ;
#128889=CARTESIAN_POINT('Ctrl Pts',(-13.5012865616176,13.075040960321,134.73973307701)) ;
#128890=CARTESIAN_POINT('Ctrl Pts',(-13.5283476037201,13.3808908357546,
134.785794826102)) ;
#128891=CARTESIAN_POINT('Ctrl Pts',(-13.5286770966046,13.6908804801079,
134.753632549337)) ;
#128892=CARTESIAN_POINT('Ctrl Pts',(-13.5026619759082,13.9819858711707,
134.644485736166)) ;
#128893=CARTESIAN_POINT('Ctrl Pts',(-13.4528259609757,14.2331023132834,
134.465714564662)) ;
#128894=CARTESIAN_POINT('Ctrl Pts',(-13.3839536191554,14.4253737396298,
134.231500815278)) ;
#128895=CARTESIAN_POINT('Ctrl Pts',(-13.3006466187109,14.54690254864,133.954824347393)) ;
#128896=CARTESIAN_POINT('Ctrl Pts',(-13.2111465830334,14.5868798000434,
133.660396959844)) ;
#128897=CARTESIAN_POINT('Ctrl Pts',(-13.121472385501,14.5442430109602,133.365347539629)) ;
#128898=CARTESIAN_POINT('Ctrl Pts',(-13.038917836058,14.4211466700167,133.091054193852)) ;
#128899=CARTESIAN_POINT('Ctrl Pts',(-12.970223038156,14.2262607777735,132.857214381594)) ;
#128900=CARTESIAN_POINT('Ctrl Pts',(-12.9211951552716,13.9744157685803,
132.680910401444)) ;
#128901=CARTESIAN_POINT('Ctrl Pts',(-12.8958788774826,13.6824770382547,
132.573794609031)) ;
#128902=CARTESIAN_POINT('Ctrl Pts',(-12.8968484596315,13.3726811668738,
132.54355335689)) ;
#128903=CARTESIAN_POINT('Ctrl Pts',(-12.9250788219677,13.06445534207,132.592712283102)) ;
#128904=CARTESIAN_POINT('Ctrl Pts',(-12.9785271121994,12.7851438246932,
132.715917599892)) ;
#128905=CARTESIAN_POINT('Ctrl Pts',(-13.0549176634622,12.5493640778092,
132.905881907071)) ;
#128906=CARTESIAN_POINT('Ctrl Pts',(-13.1488400728833,12.3769707838731,
133.147199881218)) ;
#128907=CARTESIAN_POINT('Ctrl Pts',(-13.255197241319,12.2789143225366,133.424641623102)) ;
#128908=CARTESIAN_POINT('Ctrl Pts',(-13.3657745952221,12.2633331212568,
133.71464458178)) ;
#128909=CARTESIAN_POINT('Ctrl Pts',(-13.4746365736454,12.3306602276622,
133.99947236187)) ;
#128910=CARTESIAN_POINT('Ctrl Pts',(-13.5740239071654,12.4766202323596,
134.256655193809)) ;
#128911=CARTESIAN_POINT('Ctrl Pts',(-13.6573376158806,12.6891735601127,
134.467042740179)) ;
#128912=CARTESIAN_POINT('Ctrl Pts',(-13.7201299804399,12.9552554154068,
134.617319875805)) ;
#128913=CARTESIAN_POINT('Ctrl Pts',(-13.7580993715032,13.2547269193452,
134.69511157972)) ;
#128914=CARTESIAN_POINT('Ctrl Pts',(-13.7693521902213,13.5662745338838,
134.694851970239)) ;
#128915=CARTESIAN_POINT('Ctrl Pts',(-13.7538280753497,13.8673045434185,
134.616401396385)) ;
#128916=CARTESIAN_POINT('Ctrl Pts',(-13.7133227526897,14.1368395947381,
134.46493571588)) ;
#128917=CARTESIAN_POINT('Ctrl Pts',(-13.6515265216066,14.355047357882,134.251302140233)) ;
#128918=CARTESIAN_POINT('Ctrl Pts',(-13.5734905931613,14.5066809215218,
133.990195550223)) ;
#128919=CARTESIAN_POINT('Ctrl Pts',(-13.4856168957243,14.5805549818753,
133.700364378538)) ;
#128920=CARTESIAN_POINT('Ctrl Pts',(-13.3950029122098,14.5715434476004,
133.402560518914)) ;
#128921=CARTESIAN_POINT('Ctrl Pts',(-13.3087143692411,14.4804615024267,
133.117379969011)) ;
#128922=CARTESIAN_POINT('Ctrl Pts',(-13.233499398185,14.3129345410317,132.864438386254)) ;
#128923=CARTESIAN_POINT('Ctrl Pts',(-13.1760123828882,14.0824720621631,
132.663437914386)) ;
#128924=CARTESIAN_POINT('Ctrl Pts',(-13.1406523017996,13.8045960831527,
132.527027338209)) ;
#128925=CARTESIAN_POINT('Ctrl Pts',(-13.1307543289692,13.4994873044745,
132.465012131804)) ;
#128926=CARTESIAN_POINT('Ctrl Pts',(-13.1479439577104,13.1877259359498,
132.481993019375)) ;
#128927=CARTESIAN_POINT('Ctrl Pts',(-13.1913374539631,12.8947282234829,
132.575745357319)) ;
#128928=CARTESIAN_POINT('Ctrl Pts',(-13.2592530179144,12.6375710763399,
132.740870405993)) ;
#128929=CARTESIAN_POINT('Ctrl Pts',(-13.3464861608597,12.438646888205,132.962710793394)) ;
#128930=CARTESIAN_POINT('Ctrl Pts',(-13.4484558008074,12.3091461051662,
133.227445286792)) ;
#128931=CARTESIAN_POINT('Ctrl Pts',(-13.5580827475339,12.2596124817515,
133.514610177686)) ;
#128932=CARTESIAN_POINT('Ctrl Pts',(-13.6687842386363,12.2934287573512,
133.804796814901)) ;
#128933=CARTESIAN_POINT('Ctrl Pts',(-13.7728190474512,12.4085128318244,
134.075550006677)) ;
#128934=CARTESIAN_POINT('Ctrl Pts',(-13.8633144747704,12.5956557318582,
134.306859221739)) ;
#128935=CARTESIAN_POINT('Ctrl Pts',(-13.9350011449069,12.8419007286425,
134.483200818981)) ;
#128936=CARTESIAN_POINT('Ctrl Pts',(-13.9834527110846,13.131017500255,134.5915261146)) ;
#128937=CARTESIAN_POINT('Ctrl Pts',(-14.005618946637,13.4394174344068,134.623252886023)) ;
#128938=CARTESIAN_POINT('Ctrl Pts',(-14.0007870350482,13.7489280786131,
134.575855496463)) ;
#128939=CARTESIAN_POINT('Ctrl Pts',(-13.9700930567108,14.0326636171821,
134.453180433329)) ;
#128940=CARTESIAN_POINT('Ctrl Pts',(-13.9164201828627,14.2739040584896,
134.26326367921)) ;
#128941=CARTESIAN_POINT('Ctrl Pts',(-13.8441170998093,14.4542738931404,
134.018865228188)) ;
#128942=CARTESIAN_POINT('Ctrl Pts',(-13.7597088982733,14.5602989567159,
133.739268293097)) ;
#128943=CARTESIAN_POINT('Ctrl Pts',(-13.6691129770032,14.5853165181453,
133.441420203372)) ;
#128944=CARTESIAN_POINT('Ctrl Pts',(-13.5802373274275,14.5269567294315,
133.148695949413)) ;
#128945=CARTESIAN_POINT('Ctrl Pts',(-13.4996367966222,14.3891798235028,
132.880031479941)) ;
#128946=CARTESIAN_POINT('Ctrl Pts',(-13.4342778247782,14.1817903606507,
132.655913729344)) ;
#128947=CARTESIAN_POINT('Ctrl Pts',(-13.3896410373865,13.9219442821041,
132.492558783544)) ;
#128948=CARTESIAN_POINT('Ctrl Pts',(-13.3691125413019,13.6244334028394,
132.399380837347)) ;
#128949=CARTESIAN_POINT('Ctrl Pts',(-13.3752053017507,13.313830933939,132.384130977037)) ;
#128950=CARTESIAN_POINT('Ctrl Pts',(-13.4084264932242,13.0089908308966,
132.447888942027)) ;
#128951=CARTESIAN_POINT('Ctrl Pts',(-13.4664286619536,12.7367006174924,
132.584381270711)) ;
#128952=CARTESIAN_POINT('Ctrl Pts',(-13.5464825070529,12.511790352846,132.785088887304)) ;
#128953=CARTESIAN_POINT('Ctrl Pts',(-13.6432422546615,12.3525056557872,
133.034650830282)) ;
#128954=CARTESIAN_POINT('Ctrl Pts',(-13.7509364249438,12.2695603711095,
133.316043846998)) ;
#128955=CARTESIAN_POINT('Ctrl Pts',(-13.8621624158612,12.2698997293224,
133.60778233543)) ;
#128956=CARTESIAN_POINT('Ctrl Pts',(-13.9690935338641,12.3521639545542,
133.887183808814)) ;
#128957=CARTESIAN_POINT('Ctrl Pts',(-14.0661252891564,12.5116414320552,
134.137454505603)) ;
#128958=CARTESIAN_POINT('Ctrl Pts',(-14.1460957894673,12.7360068046191,
134.337983832077)) ;
#128959=CARTESIAN_POINT('Ctrl Pts',(-14.2044014009858,13.0100794462922,
134.475150201071)) ;
#128960=CARTESIAN_POINT('Ctrl Pts',(-14.237390124937,13.3126251519116,134.538487484907)) ;
#128961=CARTESIAN_POINT('Ctrl Pts',(-14.2435487462307,13.6254713838339,
134.523181255199)) ;
#128962=CARTESIAN_POINT('Ctrl Pts',(-14.2231083995741,13.9212363983898,
134.430462751386)) ;
#128963=CARTESIAN_POINT('Ctrl Pts',(-14.1782100391862,14.182693359551,134.266134248419)) ;
#128964=CARTESIAN_POINT('Ctrl Pts',(-14.1130711823717,14.388968587839,134.042808158454)) ;
#128965=CARTESIAN_POINT('Ctrl Pts',(-14.0323807826771,14.5271449828327,
133.773829605151)) ;
#128966=CARTESIAN_POINT('Ctrl Pts',(-13.9433504875457,14.5852339313446,
133.480602666319)) ;
#128967=CARTESIAN_POINT('Ctrl Pts',(-13.8533021601708,14.5605427839008,
133.184558668845)) ;
#128968=CARTESIAN_POINT('Ctrl Pts',(-13.768441910465,14.4541441821425,132.903468307066)) ;
#128969=CARTESIAN_POINT('Ctrl Pts',(-13.6963328067855,14.2740963581792,
132.659717985775)) ;
#128970=CARTESIAN_POINT('Ctrl Pts',(-13.6424665927511,14.0323113149494,
132.469147368739)) ;
#128971=CARTESIAN_POINT('Ctrl Pts',(-13.6118627409455,13.7476340244825,
132.346648809093)) ;
#128972=CARTESIAN_POINT('Ctrl Pts',(-13.6070208398731,13.4408490996929,
132.299516778095)) ;
#128973=CARTESIAN_POINT('Ctrl Pts',(-13.6292745184613,13.1304291597349,
132.33127737453)) ;
#128974=CARTESIAN_POINT('Ctrl Pts',(-13.6775184445424,12.8426172775068,
132.439152830702)) ;
#128975=CARTESIAN_POINT('Ctrl Pts',(-13.7495368284921,12.5951022403137,
132.616294095416)) ;
#128976=CARTESIAN_POINT('Ctrl Pts',(-13.839810595063,12.4086451366238,132.847055099998)) ;
#128977=CARTESIAN_POINT('Ctrl Pts',(-13.9439529657996,12.2933533554013,
133.118081240053)) ;
#128978=CARTESIAN_POINT('Ctrl Pts',(-14.0545907378869,12.2596356648428,
133.408104864409)) ;
#128979=CARTESIAN_POINT('Ctrl Pts',(-14.1640727575126,12.3091205496962,
133.694884889222)) ;
#128980=CARTESIAN_POINT('Ctrl Pts',(-14.2659054115225,12.4379929184033,
133.959287417802)) ;
#128981=CARTESIAN_POINT('Ctrl Pts',(-14.3537948932701,12.6386444733354,
134.182778472271)) ;
#128982=CARTESIAN_POINT('Ctrl Pts',(-14.4211964420494,12.8942394600066,
134.346627354086)) ;
#128983=CARTESIAN_POINT('Ctrl Pts',(-14.4647242552601,13.1876523061434,
134.440710147854)) ;
#128984=CARTESIAN_POINT('Ctrl Pts',(-14.4818974987982,13.4984174202856,
134.457753581522)) ;
#128985=CARTESIAN_POINT('Ctrl Pts',(-14.4720621585198,13.804322851742,134.39583623639)) ;
#128986=CARTESIAN_POINT('Ctrl Pts',(-14.4366876007892,14.0825043451859,
134.259358010074)) ;
#128987=CARTESIAN_POINT('Ctrl Pts',(-14.3789691813199,14.3134150870924,
134.057582409301)) ;
#128988=CARTESIAN_POINT('Ctrl Pts',(-14.3042641459132,14.4799819682822,
133.806350659583)) ;
#128989=CARTESIAN_POINT('Ctrl Pts',(-14.2174203005974,14.5717628794977,
133.519324818323)) ;
#128990=CARTESIAN_POINT('Ctrl Pts',(-14.1271684585799,14.5804902548306,
133.222718423381)) ;
#128991=CARTESIAN_POINT('Ctrl Pts',(-14.039320812417,14.5068426765183,132.932971409604)) ;
#128992=CARTESIAN_POINT('Ctrl Pts',(-13.9613365017552,14.3556216409034,
132.672060274999)) ;
#128993=CARTESIAN_POINT('Ctrl Pts',(-13.8992930942413,14.1365917034713,
132.45757424989)) ;
#128994=CARTESIAN_POINT('Ctrl Pts',(-13.8589636050019,13.8680781333687,
132.306751288209)) ;
#128995=CARTESIAN_POINT('Ctrl Pts',(-13.843278106268,13.5671870152877,132.227831586699)) ;
#128996=CARTESIAN_POINT('Ctrl Pts',(-13.854655788299,13.253754715573,132.227735126529)) ;
#128997=CARTESIAN_POINT('Ctrl Pts',(-13.8924329041369,12.9561226298826,
132.305167149537)) ;
#128998=CARTESIAN_POINT('Ctrl Pts',(-13.9551833680437,12.689577131159,132.455284134854)) ;
#128999=CARTESIAN_POINT('Ctrl Pts',(-14.0386480780972,12.4765149553713,
132.666050247211)) ;
#129000=CARTESIAN_POINT('Ctrl Pts',(-14.1383409216431,12.330399344862,132.924033469083)) ;
#129001=CARTESIAN_POINT('Ctrl Pts',(-14.2468018422879,12.2633426723701,
133.207817039776)) ;
#129002=CARTESIAN_POINT('Ctrl Pts',(-14.3577139049087,12.2791039533646,
133.498689878789)) ;
#129003=CARTESIAN_POINT('Ctrl Pts',(-14.4635018226789,12.3764766971553,
133.774659608197)) ;
#129004=CARTESIAN_POINT('Ctrl Pts',(-14.558014452373,12.5500288330121,134.017480287725)) ;
#129005=CARTESIAN_POINT('Ctrl Pts',(-14.6338534265181,12.7839577704924,
134.206094016471)) ;
#129006=CARTESIAN_POINT('Ctrl Pts',(-14.6878213327676,13.0658040445484,
134.330505122389)) ;
#129007=CARTESIAN_POINT('Ctrl Pts',(-14.7157899465591,13.3726170007347,
134.379069272578)) ;
#129008=CARTESIAN_POINT('Ctrl Pts',(-14.7167690922712,13.6826397065971,
134.348821079552)) ;
#129009=CARTESIAN_POINT('Ctrl Pts',(-14.6916340008505,13.973415999198,134.242384284039)) ;
#129010=CARTESIAN_POINT('Ctrl Pts',(-14.6422882532958,14.2269288255441,
134.064927957567)) ;
#129011=CARTESIAN_POINT('Ctrl Pts',(-14.5739775160678,14.4205112234245,
133.832415829536)) ;
#129012=CARTESIAN_POINT('Ctrl Pts',(-14.491433377866,14.5441065980074,133.558125918887)) ;
#129013=CARTESIAN_POINT('Ctrl Pts',(-14.4013960964376,14.5870792667271,
133.261890403336)) ;
#129014=CARTESIAN_POINT('Ctrl Pts',(-14.3115236434716,14.5462510446376,
132.966219015162)) ;
#129015=CARTESIAN_POINT('Ctrl Pts',(-14.2290767314148,14.4261089740706,
132.69241253439)) ;
#129016=CARTESIAN_POINT('Ctrl Pts',(-14.1595049968999,14.2320089324099,
132.455820348673)) ;
#129017=CARTESIAN_POINT('Ctrl Pts',(-14.1100842696443,13.9821035017428,
132.278468403181)) ;
#129018=CARTESIAN_POINT('Ctrl Pts',(-14.0840475701039,13.6914861208152,
132.169293177253)) ;
#129019=CARTESIAN_POINT('Ctrl Pts',(-14.0842086433358,13.3820427303129,
132.136703583224)) ;
#129020=CARTESIAN_POINT('Ctrl Pts',(-14.1116571089248,13.0731825073203,
132.183557060288)) ;
#129021=CARTESIAN_POINT('Ctrl Pts',(-14.1644100089108,12.792789184468,132.304724839785)) ;
#129022=CARTESIAN_POINT('Ctrl Pts',(-14.2402131138955,12.5553087421356,
132.492964483192)) ;
#129023=CARTESIAN_POINT('Ctrl Pts',(-14.3338706395137,12.3807971817362,
132.733457127888)) ;
#129024=CARTESIAN_POINT('Ctrl Pts',(-14.4395838490114,12.2807361570638,
133.009141245256)) ;
#129025=CARTESIAN_POINT('Ctrl Pts',(-14.5504678733731,12.2625961451368,
133.299932577075)) ;
#129026=CARTESIAN_POINT('Ctrl Pts',(-14.6593212686416,12.32755343176,133.584790172201)) ;
#129027=CARTESIAN_POINT('Ctrl Pts',(-14.7590679467847,12.4713199441997,
133.843021054121)) ;
#129028=CARTESIAN_POINT('Ctrl Pts',(-14.8429423479471,12.6818353121991,
134.055065880925)) ;
#129029=CARTESIAN_POINT('Ctrl Pts',(-14.9067580971644,12.9488694906299,
134.208078195182)) ;
#129030=CARTESIAN_POINT('Ctrl Pts',(-14.9450496053253,13.2449963341531,
134.287119488308)) ;
#129031=CARTESIAN_POINT('Ctrl Pts',(-14.9572251863606,13.5577145851588,
134.289419851131)) ;
#129032=CARTESIAN_POINT('Ctrl Pts',(-14.9424003027303,13.8591378593898,
134.213035546637)) ;
#129033=CARTESIAN_POINT('Ctrl Pts',(-14.9025115504108,14.130166831006,134.063329760966)) ;
#129034=CARTESIAN_POINT('Ctrl Pts',(-14.8412492507378,14.349825857909,133.851274000908)) ;
#129035=CARTESIAN_POINT('Ctrl Pts',(-14.7637224121309,14.5033075139511,
133.591708104607)) ;
#129036=CARTESIAN_POINT('Ctrl Pts',(-14.6759945760978,14.5795880781192,
133.302285179212)) ;
#129037=CARTESIAN_POINT('Ctrl Pts',(-14.5853257363459,14.5729975365321,
133.004310093488)) ;
#129038=CARTESIAN_POINT('Ctrl Pts',(-14.4985716015393,14.4837968841282,
132.717672404837)) ;
#129039=CARTESIAN_POINT('Ctrl Pts',(-14.4230828934808,14.3181446441766,
132.463963177981)) ;
#129040=CARTESIAN_POINT('Ctrl Pts',(-14.3651954605715,14.0900337543834,
132.261895946104)) ;
#129041=CARTESIAN_POINT('Ctrl Pts',(-14.3290651199569,13.8125788202494,
132.123155422561)) ;
#129042=CARTESIAN_POINT('Ctrl Pts',(-14.3184784895599,13.5087144247666,
132.059213765231)) ;
#129043=CARTESIAN_POINT('Ctrl Pts',(-14.3347844930772,13.1970642860529,
132.073643923704)) ;
#129044=CARTESIAN_POINT('Ctrl Pts',(-14.3776048210991,12.9023259165876,
132.165611695719)) ;
#129045=CARTESIAN_POINT('Ctrl Pts',(-14.4446704149023,12.6446851896536,
132.32836378006)) ;
#129046=CARTESIAN_POINT('Ctrl Pts',(-14.5313911331387,12.4436426987833,
132.54869094617)) ;
#129047=CARTESIAN_POINT('Ctrl Pts',(-14.6331600881906,12.311800617446,132.812797644459)) ;
#129048=CARTESIAN_POINT('Ctrl Pts',(-14.7426885619788,12.2597626710197,
133.099669110203)) ;
#129049=CARTESIAN_POINT('Ctrl Pts',(-14.8538711248284,12.2917039117493,
133.391131103677)) ;
#129050=CARTESIAN_POINT('Ctrl Pts',(-14.9573815637939,12.4035190207528,
133.660621795252)) ;
#129051=CARTESIAN_POINT('Ctrl Pts',(-15.049112181755,12.5902948819765,133.895252296706)) ;
#129052=CARTESIAN_POINT('Ctrl Pts',(-15.1209253149525,12.8337324593119,
134.072169901694)) ;
#129053=CARTESIAN_POINT('Ctrl Pts',(-15.1703867081126,13.1235886512336,
134.183247742845)) ;
#129054=CARTESIAN_POINT('Ctrl Pts',(-15.1930624887373,13.4302519465087,
134.216624541758)) ;
#129055=CARTESIAN_POINT('Ctrl Pts',(-15.1892010995764,13.7390104769504,
134.172188842912)) ;
#129056=CARTESIAN_POINT('Ctrl Pts',(-15.1589633431141,14.026006220093,134.050578201791)) ;
#129057=CARTESIAN_POINT('Ctrl Pts',(-15.1061157318474,14.267226887447,133.863258556503)) ;
#129058=CARTESIAN_POINT('Ctrl Pts',(-15.0343759397028,14.4498458774909,
133.620514200202)) ;
#129059=CARTESIAN_POINT('Ctrl Pts',(-14.9498214158949,14.5586319222976,
133.340333419483)) ;
#129060=CARTESIAN_POINT('Ctrl Pts',(-14.8592614584468,14.5856242109288,
133.04258213399)) ;
#129061=CARTESIAN_POINT('Ctrl Pts',(-14.7706278929769,14.5299078426425,
132.750710027517)) ;
#129062=CARTESIAN_POINT('Ctrl Pts',(-14.6894779497955,14.3940108170827,
132.480354976961)) ;
#129063=CARTESIAN_POINT('Ctrl Pts',(-14.6237443816963,14.1888421373124,
132.255216550352)) ;
#129064=CARTESIAN_POINT('Ctrl Pts',(-14.5783921093744,13.9299825539778,
132.089723243472)) ;
#129065=CARTESIAN_POINT('Ctrl Pts',(-14.5571335436849,13.6339609889882,
131.994496348785)) ;
#129066=CARTESIAN_POINT('Ctrl Pts',(-14.5624517005765,13.322716019869,131.976899875698)) ;
#129067=CARTESIAN_POINT('Ctrl Pts',(-14.5947146637798,13.0187245278142,
132.038014645956)) ;
#129068=CARTESIAN_POINT('Ctrl Pts',(-14.6520713746526,12.7442185255371,
132.172519400802)) ;
#129069=CARTESIAN_POINT('Ctrl Pts',(-14.7320201612289,12.5167189734132,
132.372757875477)) ;
#129070=CARTESIAN_POINT('Ctrl Pts',(-14.8279565154633,12.3563386644065,
132.620071928308)) ;
#129071=CARTESIAN_POINT('Ctrl Pts',(-14.9352059362097,12.2709228506509,
132.900226988222)) ;
#129072=CARTESIAN_POINT('Ctrl Pts',(-15.0465561535837,12.268610094108,133.192290741623)) ;
#129073=CARTESIAN_POINT('Ctrl Pts',(-15.1539430166123,12.3485945923255,
133.47295308261)) ;
#129074=CARTESIAN_POINT('Ctrl Pts',(-15.2516577056561,12.5068355789937,
133.725101150116)) ;
#129075=CARTESIAN_POINT('Ctrl Pts',(-15.3316894364652,12.7283300538896,
133.926001210879)) ;
#129076=CARTESIAN_POINT('Ctrl Pts',(-15.3908345605777,13.0013549210284,
134.065586158473)) ;
#129077=CARTESIAN_POINT('Ctrl Pts',(-15.4245920438632,13.3039530597295,
134.131105830834)) ;
#129078=CARTESIAN_POINT('Ctrl Pts',(-15.4315691009249,13.615850743561,134.118304796452)) ;
#129079=CARTESIAN_POINT('Ctrl Pts',(-15.4117562915314,13.9138454553417,
134.02724572002)) ;
#129080=CARTESIAN_POINT('Ctrl Pts',(-15.3676987993894,14.1752851805425,
133.865537651657)) ;
#129081=CARTESIAN_POINT('Ctrl Pts',(-15.302987683393,14.3839668392215,133.643386137514)) ;
#129082=CARTESIAN_POINT('Ctrl Pts',(-15.2227252518571,14.5240578226957,
133.375696442509)) ;
#129083=CARTESIAN_POINT('Ctrl Pts',(-15.1339295668703,14.584818929902,133.083181731107)) ;
#129084=CARTESIAN_POINT('Ctrl Pts',(-15.0432280820715,14.5621167472896,
132.785007493075)) ;
#129085=CARTESIAN_POINT('Ctrl Pts',(-14.9586600655153,14.4583966602146,
132.504979892596)) ;
#129086=CARTESIAN_POINT('Ctrl Pts',(-14.8860092123973,14.2803904178195,
132.259619724696)) ;
#129087=CARTESIAN_POINT('Ctrl Pts',(-14.8316450061125,14.0406559765549,
132.067661691774)) ;
#129088=CARTESIAN_POINT('Ctrl Pts',(-14.8001686976109,13.7571590399429,
131.942617503947)) ;
#129089=CARTESIAN_POINT('Ctrl Pts',(-14.7946378325009,13.4483332736025,
131.893213729335)) ;
#129090=CARTESIAN_POINT('Ctrl Pts',(-14.8158814426119,13.1406103992417,
131.922351205196)) ;
#129091=CARTESIAN_POINT('Ctrl Pts',(-14.8637978713857,12.8492377170497,
132.028961983023)) ;
#129092=CARTESIAN_POINT('Ctrl Pts',(-14.9347982932636,12.6021186018862,
132.203358631515)) ;
#129093=CARTESIAN_POINT('Ctrl Pts',(-15.0246662575928,12.4130744412516,
132.432874233369)) ;
#129094=CARTESIAN_POINT('Ctrl Pts',(-15.1289271190847,12.2953575367152,
132.704129028341)) ;
#129095=CARTESIAN_POINT('Ctrl Pts',(-15.2390105465142,12.2595400052722,
132.9926724095)) ;
#129096=CARTESIAN_POINT('Ctrl Pts',(-15.3487113523538,12.3063152816415,
133.280070351324)) ;
#129097=CARTESIAN_POINT('Ctrl Pts',(-15.4514320482357,12.4341408158502,
133.546864149425)) ;
#129098=CARTESIAN_POINT('Ctrl Pts',(-15.5391158365436,12.6316134537437,
133.770005058121)) ;
#129099=CARTESIAN_POINT('Ctrl Pts',(-15.6073687443637,12.8861349922411,
133.9362737051)) ;
#129100=CARTESIAN_POINT('Ctrl Pts',(-15.6516716819306,13.1792138645797,
134.032575547946)) ;
#129101=CARTESIAN_POINT('Ctrl Pts',(-15.6695953949056,13.4905686905893,
134.051730810821)) ;
#129102=CARTESIAN_POINT('Ctrl Pts',(-15.6604169021637,13.7964603430473,
133.991777195623)) ;
#129103=CARTESIAN_POINT('Ctrl Pts',(-15.6258987359129,14.0743847640953,
133.857952822959)) ;
#129104=CARTESIAN_POINT('Ctrl Pts',(-15.5689424529067,14.3070162131528,
133.658441754643)) ;
#129105=CARTESIAN_POINT('Ctrl Pts',(-15.4941859183638,14.4764518119822,
133.406859608136)) ;
#129106=CARTESIAN_POINT('Ctrl Pts',(-15.4083342578243,14.5698501625241,
133.123024051053)) ;
#129107=CARTESIAN_POINT('Ctrl Pts',(-15.3176422912758,14.5816111326668,
132.82495471565)) ;
#129108=CARTESIAN_POINT('Ctrl Pts',(-15.2293490886526,14.5098992068035,
132.53380903365)) ;
#129109=CARTESIAN_POINT('Ctrl Pts',(-15.1509641087805,14.3604030985763,
132.271696519676)) ;
#129110=CARTESIAN_POINT('Ctrl Pts',(-15.0885882766536,14.1435657734104,
132.056328026894)) ;
#129111=CARTESIAN_POINT('Ctrl Pts',(-15.0475171969358,13.8762647134096,
131.90333144506)) ;
#129112=CARTESIAN_POINT('Ctrl Pts',(-15.0311871549161,13.5746435358358,
131.822388428591)) ;
#129113=CARTESIAN_POINT('Ctrl Pts',(-15.0415879944804,13.2647987939523,
131.819827576964)) ;
#129114=CARTESIAN_POINT('Ctrl Pts',(-15.0788068560028,12.9638357563477,
131.895337689995)) ;
#129115=CARTESIAN_POINT('Ctrl Pts',(-15.1408172739775,12.6967407948571,
132.043374153266)) ;
#129116=CARTESIAN_POINT('Ctrl Pts',(-15.2239197092677,12.481516798795,132.253008004637)) ;
#129117=CARTESIAN_POINT('Ctrl Pts',(-15.3228857413039,12.3337893926253,
132.50899135009)) ;
#129118=CARTESIAN_POINT('Ctrl Pts',(-15.431430165252,12.264079799943,132.792934661794)) ;
#129119=CARTESIAN_POINT('Ctrl Pts',(-15.5422439139297,12.2774691330631,
133.08356318742)) ;
#129120=CARTESIAN_POINT('Ctrl Pts',(-15.6482784383748,12.3724670081561,
133.360251299871)) ;
#129121=CARTESIAN_POINT('Ctrl Pts',(-15.7431900439343,12.5437673872502,
133.604261147898)) ;
#129122=CARTESIAN_POINT('Ctrl Pts',(-15.8197543818073,12.7765746367498,
133.794928013366)) ;
#129123=CARTESIAN_POINT('Ctrl Pts',(-15.8742879735741,13.056442650052,133.921098919805)) ;
#129124=CARTESIAN_POINT('Ctrl Pts',(-15.9031133081289,13.3632373960093,
133.972110741397)) ;
#129125=CARTESIAN_POINT('Ctrl Pts',(-15.9049895115739,13.6730054777402,
133.944546039053)) ;
#129126=CARTESIAN_POINT('Ctrl Pts',(-15.8802545110404,13.9671153090071,
133.838972001116)) ;
#129127=CARTESIAN_POINT('Ctrl Pts',(-15.8320488758174,14.2192390976399,
133.665214561811)) ;
#129128=CARTESIAN_POINT('Ctrl Pts',(-15.7637592246223,14.4164802278466,
133.432495927919)) ;
#129129=CARTESIAN_POINT('Ctrl Pts',(-15.6816763634688,14.5415580379271,
133.159645677855)) ;
#129130=CARTESIAN_POINT('Ctrl Pts',(-15.5920508372998,14.5869148385537,
132.864711325066)) ;
#129131=CARTESIAN_POINT('Ctrl Pts',(-15.5021160215326,14.5490099524811,
132.56888691804)) ;
#129132=CARTESIAN_POINT('Ctrl Pts',(-15.4187916392682,14.4299835675068,
132.292268421048)) ;
#129133=CARTESIAN_POINT('Ctrl Pts',(-15.3493635815801,14.2395160245118,
132.056400600707)) ;
#129134=CARTESIAN_POINT('Ctrl Pts',(-15.2989597100586,13.9900850970595,
131.876007619012)) ;
#129135=CARTESIAN_POINT('Ctrl Pts',(-15.272218093911,13.7002631215164,131.764776828578)) ;
#129136=CARTESIAN_POINT('Ctrl Pts',(-15.2716505882856,13.3906063614652,
131.730004772905)) ;
#129137=CARTESIAN_POINT('Ctrl Pts',(-15.2981644321246,13.0826197728353,
131.774272870496)) ;
#129138=CARTESIAN_POINT('Ctrl Pts',(-15.3504644959401,12.799748141124,131.893944982008)) ;
#129139=CARTESIAN_POINT('Ctrl Pts',(-15.4255037118289,12.5614903219102,
132.080049932649)) ;
#129140=CARTESIAN_POINT('Ctrl Pts',(-15.5188545837591,12.3846250484045,
132.319591184362)) ;
#129141=CARTESIAN_POINT('Ctrl Pts',(-15.6243621794924,12.2824688023076,
132.594668003759)) ;
#129142=CARTESIAN_POINT('Ctrl Pts',(-15.7348925303378,12.2619556296945,
132.884516282295)) ;
#129143=CARTESIAN_POINT('Ctrl Pts',(-15.8440119597469,12.3244284918516,
133.170121702575)) ;
#129144=CARTESIAN_POINT('Ctrl Pts',(-15.9443512957769,12.4664339674621,
133.430007529672)) ;
#129145=CARTESIAN_POINT('Ctrl Pts',(-16.0286266715396,12.6753486557463,
133.64323601442)) ;
#129146=CARTESIAN_POINT('Ctrl Pts',(-16.0927613820503,12.9390313518122,
133.797416214201)) ;
#129147=CARTESIAN_POINT('Ctrl Pts',(-16.1322240438312,13.2369182053758,
133.879596524475)) ;
#129148=CARTESIAN_POINT('Ctrl Pts',(-16.1450073393233,13.5497742859679,
133.883656973668)) ;
#129149=CARTESIAN_POINT('Ctrl Pts',(-16.1309752238549,13.8506093508767,
133.809712924713)) ;
#129150=CARTESIAN_POINT('Ctrl Pts',(-16.0917806117036,14.1229208970494,
133.662027117479)) ;
#129151=CARTESIAN_POINT('Ctrl Pts',(-16.0311608129876,14.3440340084818,
133.451889788938)) ;
#129152=CARTESIAN_POINT('Ctrl Pts',(-15.9539287114878,14.5000650086301,
133.193133120408)) ;
#129153=CARTESIAN_POINT('Ctrl Pts',(-15.8659835029665,14.5786444496306,
132.902928525626)) ;
#129154=CARTESIAN_POINT('Ctrl Pts',(-15.7758709261625,14.5743811791395,
132.606790036893)) ;
#129155=CARTESIAN_POINT('Ctrl Pts',(-15.6886304289123,14.4873599141627,
132.318627596167)) ;
#129156=CARTESIAN_POINT('Ctrl Pts',(-15.6129042871571,14.3240887387416,
132.064305156587)) ;
#129157=CARTESIAN_POINT('Ctrl Pts',(-15.5543635865499,14.0972553768965,
131.860272571408)) ;
#129158=CARTESIAN_POINT('Ctrl Pts',(-15.517587454923,13.8219068186535,131.719757504624)) ;
#129159=CARTESIAN_POINT('Ctrl Pts',(-15.5061671790112,13.5160257304535,
131.653105199681)) ;
#129160=CARTESIAN_POINT('Ctrl Pts',(-15.5218470098257,13.2050738330625,
131.665795904458)) ;
#129161=CARTESIAN_POINT('Ctrl Pts',(-15.5637864688922,12.9106474660782,
131.755303957723)) ;
#129162=CARTESIAN_POINT('Ctrl Pts',(-15.6300512629826,12.6518068845878,
131.915759644786)) ;
#129163=CARTESIAN_POINT('Ctrl Pts',(-15.7166383035372,12.4481718764226,
132.135556413603)) ;
#129164=CARTESIAN_POINT('Ctrl Pts',(-15.8179132984019,12.314346622866,132.398281612479)) ;
#129165=CARTESIAN_POINT('Ctrl Pts',(-15.9278856597735,12.2602411291599,
132.686273104354)) ;
#129166=CARTESIAN_POINT('Ctrl Pts',(-16.0376086994621,12.289044210784,132.973945221982)) ;
#129167=CARTESIAN_POINT('Ctrl Pts',(-16.1426489958405,12.3996398985986,
133.247503974334)) ;
#129168=CARTESIAN_POINT('Ctrl Pts',(-16.2340318975309,12.5827969028938,
133.481431287424)) ;
#129169=CARTESIAN_POINT('Ctrl Pts',(-16.3071554186046,12.8269629878668,
133.661853204856)) ;
#129170=CARTESIAN_POINT('Ctrl Pts',(-16.3568161319852,13.1127056220744,
133.773888186978)) ;
#129171=CARTESIAN_POINT('Ctrl Pts',(-16.3806449236658,13.4217118821407,
133.810331791983)) ;
#129172=CARTESIAN_POINT('Ctrl Pts',(-16.377439581411,13.73042511485,133.767855369085)) ;
#129173=CARTESIAN_POINT('Ctrl Pts',(-16.3479691030351,14.0183443112805,
133.648491790716)) ;
#129174=CARTESIAN_POINT('Ctrl Pts',(-16.2955799140703,14.2615011985034,
133.462442962247)) ;
#129175=CARTESIAN_POINT('Ctrl Pts',(-16.2243937788781,14.4455241600489,
133.221377680409)) ;
#129176=CARTESIAN_POINT('Ctrl Pts',(-16.1403852077266,14.5564730484766,
132.942888766388)) ;
#129177=CARTESIAN_POINT('Ctrl Pts',(-16.049570185435,14.5860332576142,132.644269887885)) ;
#129178=CARTESIAN_POINT('Ctrl Pts',(-15.9609660140179,14.5327319969804,
132.352549382835)) ;
#129179=CARTESIAN_POINT('Ctrl Pts',(-15.879392560384,14.3988255377981,132.080913727718)) ;
#129180=CARTESIAN_POINT('Ctrl Pts',(-15.8134294633956,14.1966329987979,
131.855270403513)) ;
#129181=CARTESIAN_POINT('Ctrl Pts',(-15.7671288771727,13.9381995065902,
131.686862264582)) ;
#129182=CARTESIAN_POINT('Ctrl Pts',(-15.7451534934309,13.64215083048,131.589466301994)) ;
#129183=CARTESIAN_POINT('Ctrl Pts',(-15.7497253677879,13.3319748624789,
131.569786305151)) ;
#129184=CARTESIAN_POINT('Ctrl Pts',(-15.7810839054332,13.0275242268779,
131.628280225436)) ;
#129185=CARTESIAN_POINT('Ctrl Pts',(-15.8383251199372,12.7499513876655,
131.762184797718)) ;
#129186=CARTESIAN_POINT('Ctrl Pts',(-15.9170076046053,12.5230806555812,
131.959040186424)) ;
#129187=CARTESIAN_POINT('Ctrl Pts',(-16.0129847307109,12.3595163887299,
132.206295823084)) ;
#129188=CARTESIAN_POINT('Ctrl Pts',(-16.1202899369408,12.2720601229367,
132.486548175091)) ;
#129189=CARTESIAN_POINT('Ctrl Pts',(-16.2314011652386,12.2676665272562,
132.77798081952)) ;
#129190=CARTESIAN_POINT('Ctrl Pts',(-16.3386053442053,12.3451447883363,
133.058221097043)) ;
#129191=CARTESIAN_POINT('Ctrl Pts',(-16.4364726934134,12.5004781878849,
133.310918034804)) ;
#129192=CARTESIAN_POINT('Ctrl Pts',(-16.5175132252489,12.7212076725333,
133.514603343061)) ;
#129193=CARTESIAN_POINT('Ctrl Pts',(-16.5773484087044,12.9936144334216,
133.656155150364)) ;
#129194=CARTESIAN_POINT('Ctrl Pts',(-16.6117393173517,13.2947836175078,
133.723619906867)) ;
#129195=CARTESIAN_POINT('Ctrl Pts',(-16.6195349325509,13.6064067051063,
133.713244471192)) ;
#129196=CARTESIAN_POINT('Ctrl Pts',(-16.6005564591254,13.9050216556666,
133.624641768626)) ;
#129197=CARTESIAN_POINT('Ctrl Pts',(-16.5570362865346,14.1686336001984,
133.464397749618)) ;
#129198=CARTESIAN_POINT('Ctrl Pts',(-16.4928541402158,14.378818223522,133.243813490969)) ;
#129199=CARTESIAN_POINT('Ctrl Pts',(-16.4131723103661,14.520866250274,132.977903847769)) ;
#129200=CARTESIAN_POINT('Ctrl Pts',(-16.324418752034,14.5841619926364,132.685464359958)) ;
#129201=CARTESIAN_POINT('Ctrl Pts',(-16.2339590586159,14.5641966334699,
132.388108863399)) ;
#129202=CARTESIAN_POINT('Ctrl Pts',(-16.1487199252297,14.4625802261662,
132.105972172714)) ;
#129203=CARTESIAN_POINT('Ctrl Pts',(-16.0755352121241,14.2860055470816,
131.858992129095)) ;
#129204=CARTESIAN_POINT('Ctrl Pts',(-16.0207525963594,14.0484512040757,
131.665905798097)) ;
#129205=CARTESIAN_POINT('Ctrl Pts',(-15.988546581059,13.7663469877686,131.538764120789)) ;
#129206=CARTESIAN_POINT('Ctrl Pts',(-15.9821721421647,13.4574608016115,
131.486848095998)) ;
#129207=CARTESIAN_POINT('Ctrl Pts',(-16.0027619761264,13.1488899436826,
131.514007237781)) ;
#129208=CARTESIAN_POINT('Ctrl Pts',(-16.049615622405,12.8583365068185,131.617715430164)) ;
#129209=CARTESIAN_POINT('Ctrl Pts',(-16.1201676913662,12.6085157636358,
131.790669007322)) ;
#129210=CARTESIAN_POINT('Ctrl Pts',(-16.2098079305234,12.4173946881525,
132.019450745302)) ;
#129211=CARTESIAN_POINT('Ctrl Pts',(-16.3131800358718,12.2980452511377,
132.288293077009)) ;
#129212=CARTESIAN_POINT('Ctrl Pts',(-16.423261619167,12.2592457783441,132.576798899315)) ;
#129213=CARTESIAN_POINT('Ctrl Pts',(-16.5335959230037,12.3040208599772,
132.865888151637)) ;
#129214=CARTESIAN_POINT('Ctrl Pts',(-16.6359277149238,12.42869393012,133.131777211617)) ;
#129215=CARTESIAN_POINT('Ctrl Pts',(-16.7244699466103,12.6243589904513,
133.357335318922)) ;
#129216=CARTESIAN_POINT('Ctrl Pts',(-16.7936703717637,12.8789083134422,
133.52620265048)) ;
#129217=CARTESIAN_POINT('Ctrl Pts',(-16.8384788441524,13.1702260749438,
133.624095874272)) ;
#129218=CARTESIAN_POINT('Ctrl Pts',(-16.857225046346,13.4805036565043,133.645741963258)) ;
#129219=CARTESIAN_POINT('Ctrl Pts',(-16.8489063138927,13.7876510907378,
133.588224449993)) ;
#129220=CARTESIAN_POINT('Ctrl Pts',(-16.8148392702879,14.0678452038592,
133.455558574279)) ;
#129221=CARTESIAN_POINT('Ctrl Pts',(-16.7587271978749,14.3007432153336,
133.258689436977)) ;
#129222=CARTESIAN_POINT('Ctrl Pts',(-16.684354006604,14.4725786028925,133.00818610044)) ;
#129223=CARTESIAN_POINT('Ctrl Pts',(-16.5987270141233,14.5682598705244,
132.725006844455)) ;
#129224=CARTESIAN_POINT('Ctrl Pts',(-16.508083118961,14.582415300085,132.427079939102)) ;
#129225=CARTESIAN_POINT('Ctrl Pts',(-16.4197468519132,14.5133615021942,
132.13586794255)) ;
#129226=CARTESIAN_POINT('Ctrl Pts',(-16.3408443778437,14.3656856001402,
131.872174755778)) ;
#129227=CARTESIAN_POINT('Ctrl Pts',(-16.2781611136979,14.1519224163712,
131.656079963678)) ;
#129228=CARTESIAN_POINT('Ctrl Pts',(-16.2360715647158,13.8839966757843,
131.499861935695)) ;
#129229=CARTESIAN_POINT('Ctrl Pts',(-16.2190922770335,13.5839687082689,
131.417139097658)) ;
#129230=CARTESIAN_POINT('Ctrl Pts',(-16.228706420837,13.2736212101871,131.412219775263)) ;
#129231=CARTESIAN_POINT('Ctrl Pts',(-16.2650473903063,12.972761740788,131.485254270493)) ;
#129232=CARTESIAN_POINT('Ctrl Pts',(-16.3265741277852,12.7034621724925,
131.631760171048)) ;
#129233=CARTESIAN_POINT('Ctrl Pts',(-16.4091164711671,12.4867212726039,
131.839780973645)) ;
#129234=CARTESIAN_POINT('Ctrl Pts',(-16.5078141561467,12.33686375234,132.094949163634)) ;
#129235=CARTESIAN_POINT('Ctrl Pts',(-16.6158219520768,12.2650347020363,
132.377434648052)) ;
#129236=CARTESIAN_POINT('Ctrl Pts',(-16.7269532891186,12.2758062427332,
132.668907462376)) ;
#129237=CARTESIAN_POINT('Ctrl Pts',(-16.8336048391349,12.3692806824326,
132.947266347668)) ;
#129238=CARTESIAN_POINT('Ctrl Pts',(-16.9284317414451,12.5378928700438,
133.191194855104)) ;
#129239=CARTESIAN_POINT('Ctrl Pts',(-17.0057245470623,12.7694276671961,
133.383932637994)) ;
#129240=CARTESIAN_POINT('Ctrl Pts',(-17.0609458230703,13.0484835222186,
133.512094105767)) ;
#129241=CARTESIAN_POINT('Ctrl Pts',(-17.0904966230258,13.3553251323831,
133.565175957741)) ;
#129242=CARTESIAN_POINT('Ctrl Pts',(-17.0930427512237,13.6640555528138,
133.539693243404)) ;
#129243=CARTESIAN_POINT('Ctrl Pts',(-17.0693003062227,13.9577070020221,
133.437180645655)) ;
#129244=CARTESIAN_POINT('Ctrl Pts',(-17.0215202195115,14.2128779574234,
133.264471361795)) ;
#129245=CARTESIAN_POINT('Ctrl Pts',(-16.9536976019041,14.4117544090383,
133.033127560494)) ;
#129246=CARTESIAN_POINT('Ctrl Pts',(-16.8719823256452,14.5391282978367,
132.761364728031)) ;
#129247=CARTESIAN_POINT('Ctrl Pts',(-16.7820589422562,14.5867879388137,
132.465410805386)) ;
#129248=CARTESIAN_POINT('Ctrl Pts',(-16.6924665130693,14.5512051558335,
132.17074476344)) ;
#129249=CARTESIAN_POINT('Ctrl Pts',(-16.6087056500292,14.4343419868163,
131.892798100955)) ;
#129250=CARTESIAN_POINT('Ctrl Pts',(-16.538832091035,14.2455278890041,131.65562031777)) ;
#129251=CARTESIAN_POINT('Ctrl Pts',(-16.4879190259306,13.9981929113896,
131.47382165514)) ;
#129252=CARTESIAN_POINT('Ctrl Pts',(-16.4603768158028,13.7085066713852,
131.360165716165)) ;
#129253=CARTESIAN_POINT('Ctrl Pts',(-16.4591129437466,13.399579397686,131.323410336661)) ;
#129254=CARTESIAN_POINT('Ctrl Pts',(-16.484691657851,13.0919774800644,131.365036261441)) ;
#129255=CARTESIAN_POINT('Ctrl Pts',(-16.5365613200866,12.8067303941414,
131.483283731596)) ;
#129256=CARTESIAN_POINT('Ctrl Pts',(-16.6106299167186,12.5682009002538,
131.666727984921)) ;
#129257=CARTESIAN_POINT('Ctrl Pts',(-16.703661484763,12.3888212381261,131.905270268361)) ;
#129258=CARTESIAN_POINT('Ctrl Pts',(-16.8087651880266,12.2844119567793,
132.179212799551)) ;
#129259=CARTESIAN_POINT('Ctrl Pts',(-16.9195860446724,12.2613333921228,
132.469805102314)) ;
#129260=CARTESIAN_POINT('Ctrl Pts',(-17.0287241594816,12.3215794364131,
132.755502128305)) ;
#129261=CARTESIAN_POINT('Ctrl Pts',(-17.1290959969068,12.460691871722,133.015600065389)) ;
#129262=CARTESIAN_POINT('Ctrl Pts',(-17.2142928173378,12.6684213350559,
133.231391682523)) ;
#129263=CARTESIAN_POINT('Ctrl Pts',(-17.2792269999154,12.9319194586172,
133.387791946882)) ;
#129264=CARTESIAN_POINT('Ctrl Pts',(-17.3191658999381,13.227908152673,133.471502696313)) ;
#129265=CARTESIAN_POINT('Ctrl Pts',(-17.3328145145393,13.5392232276546,
133.478245333532)) ;
#129266=CARTESIAN_POINT('Ctrl Pts',(-17.319569038104,13.842168223521,133.406437925368)) ;
#129267=CARTESIAN_POINT('Ctrl Pts',(-17.2810019534039,14.115831938889,133.260561997188)) ;
#129268=CARTESIAN_POINT('Ctrl Pts',(-17.2207880893722,14.3390092448437,
133.0515426788)) ;
#129269=CARTESIAN_POINT('Ctrl Pts',(-17.1440720435031,14.4964745213525,
132.794365747161)) ;
#129270=CARTESIAN_POINT('Ctrl Pts',(-17.0568630848371,14.5773715613601,
132.506502793467)) ;
#129271=CARTESIAN_POINT('Ctrl Pts',(-16.9660480537129,14.5757025452078,
132.208057598299)) ;
#129272=CARTESIAN_POINT('Ctrl Pts',(-16.8788431858424,14.4908671565799,
131.920085188668)) ;
#129273=CARTESIAN_POINT('Ctrl Pts',(-16.8029585654165,14.3305923822081,
131.665427504091)) ;
#129274=CARTESIAN_POINT('Ctrl Pts',(-16.7435309388087,14.104809150226,131.458681664569)) ;
#129275=CARTESIAN_POINT('Ctrl Pts',(-16.7060430507986,13.8293692517449,
131.315961230469)) ;
#129276=CARTESIAN_POINT('Ctrl Pts',(-16.693936404888,13.5265764588792,131.247582518376)) ;
#129277=CARTESIAN_POINT('Ctrl Pts',(-16.708699103235,13.2147295864641,131.25750947637)) ;
#129278=CARTESIAN_POINT('Ctrl Pts',(-16.749940948686,12.9189025959915,131.344918847352)) ;
#129279=CARTESIAN_POINT('Ctrl Pts',(-16.8158171841197,12.6580300058624,
131.504131716298)) ;
#129280=CARTESIAN_POINT('Ctrl Pts',(-16.9015293870053,12.4534346092271,
131.721516359276)) ;
#129281=CARTESIAN_POINT('Ctrl Pts',(-17.0027137249338,12.3171076875182,
131.983889087043)) ;
#129282=CARTESIAN_POINT('Ctrl Pts',(-17.1119673542446,12.2606844041001,
132.269957584545)) ;
#129283=CARTESIAN_POINT('Ctrl Pts',(-17.2225632011221,12.28708894542,132.559937626368)) ;
#129284=CARTESIAN_POINT('Ctrl Pts',(-17.3278048536779,12.3957982979784,
132.834097357884)) ;
#129285=CARTESIAN_POINT('Ctrl Pts',(-17.4194176571879,12.5767256931705,
133.068762679094)) ;
#129286=CARTESIAN_POINT('Ctrl Pts',(-17.493044253941,12.8186993090181,133.250730862918)) ;
#129287=CARTESIAN_POINT('Ctrl Pts',(-17.5436697534756,13.1050418122632,
133.365405420034)) ;
#129288=CARTESIAN_POINT('Ctrl Pts',(-17.5681129690375,13.4130762774239,
133.40372138138)) ;
#129289=CARTESIAN_POINT('Ctrl Pts',(-17.5656637238399,13.7214651922854,
133.36351270507)) ;
#129290=CARTESIAN_POINT('Ctrl Pts',(-17.5371700854611,14.0093161803211,
133.247144420446)) ;
#129291=CARTESIAN_POINT('Ctrl Pts',(-17.4849725016858,14.2560736745197,
133.061372547591)) ;
#129292=CARTESIAN_POINT('Ctrl Pts',(-17.4143885017694,14.4412184324741,
132.822170207149)) ;
#129293=CARTESIAN_POINT('Ctrl Pts',(-17.3306747567121,14.5543182486296,
132.544541120772)) ;
#129294=CARTESIAN_POINT('Ctrl Pts',(-17.2403639651478,14.5864671226158,
132.247555986274)) ;
#129295=CARTESIAN_POINT('Ctrl Pts',(-17.1510139448171,14.5351930483474,
131.953422292404)) ;
#129296=CARTESIAN_POINT('Ctrl Pts',(-17.0696123032485,14.4042256836979,
131.682497044218)) ;
#129297=CARTESIAN_POINT('Ctrl Pts',(-17.0028303657657,14.2033620376663,
131.454334310528)) ;
#129298=CARTESIAN_POINT('Ctrl Pts',(-16.9559126255241,13.9460943554148,
131.284116174304)) ;
#129299=CARTESIAN_POINT('Ctrl Pts',(-16.9332167115845,13.6510940707038,
131.184642433927)) ;
#129300=CARTESIAN_POINT('Ctrl Pts',(-16.9369769560301,13.340963323575,131.162583892338)) ;
#129301=CARTESIAN_POINT('Ctrl Pts',(-16.9676993284991,13.0355469770442,
131.219159783569)) ;
#129302=CARTESIAN_POINT('Ctrl Pts',(-17.0238499504818,12.7584810816834,
131.3500834927)) ;
#129303=CARTESIAN_POINT('Ctrl Pts',(-17.1022027786305,12.5287899159639,
131.545836377495)) ;
#129304=CARTESIAN_POINT('Ctrl Pts',(-17.1977759409222,12.3633457442531,
131.791921351567)) ;
#129305=CARTESIAN_POINT('Ctrl Pts',(-17.3044741521689,12.2737023514909,
132.070510336543)) ;
#129306=CARTESIAN_POINT('Ctrl Pts',(-17.4156081788106,12.2663504443872,
132.362000980484)) ;
#129307=CARTESIAN_POINT('Ctrl Pts',(-17.5236663849567,12.3420800967331,
132.644528547353)) ;
#129308=CARTESIAN_POINT('Ctrl Pts',(-17.6214436234339,12.4946575605773,
132.897122538516)) ;
#129309=CARTESIAN_POINT('Ctrl Pts',(-17.7033350086812,12.7142648856192,
133.103184303582)) ;
#129310=CARTESIAN_POINT('Ctrl Pts',(-17.7637633207662,12.9853993961476,
133.246492127846)) ;
#129311=CARTESIAN_POINT('Ctrl Pts',(-17.7989327686341,13.2860373557687,
133.316222270595)) ;
#129312=CARTESIAN_POINT('Ctrl Pts',(-17.8074758097156,13.5985521220417,
133.307942379033)) ;
#129313=CARTESIAN_POINT('Ctrl Pts',(-17.7891330033214,13.8975127829307,
133.221220006)) ;
#129314=CARTESIAN_POINT('Ctrl Pts',(-17.7464726108498,14.1612605834451,
133.063631344191)) ;
#129315=CARTESIAN_POINT('Ctrl Pts',(-17.6826753131341,14.3739607965711,
132.844075788855)) ;
#129316=CARTESIAN_POINT('Ctrl Pts',(-17.603060579253,14.5182946770733,132.578264088989)) ;
#129317=CARTESIAN_POINT('Ctrl Pts',(-17.5146145686403,14.5834512789115,
132.286785455906)) ;
#129318=CARTESIAN_POINT('Ctrl Pts',(-17.4244047684484,14.5659482327596,
131.990267496769)) ;
#129319=CARTESIAN_POINT('Ctrl Pts',(-17.3389354411882,14.4667698012676,
131.707468479579)) ;
#129320=CARTESIAN_POINT('Ctrl Pts',(-17.2652382607785,14.2923286042259,
131.458983161722)) ;
#129321=CARTESIAN_POINT('Ctrl Pts',(-17.2096082359978,14.0548140829524,
131.26323131239)) ;
#129322=CARTESIAN_POINT('Ctrl Pts',(-17.1769815564138,13.7751054623822,
131.135039548468)) ;
#129323=CARTESIAN_POINT('Ctrl Pts',(-17.1697052026753,13.4671707180117,
131.080539965422)) ;
#129324=CARTESIAN_POINT('Ctrl Pts',(-17.1896989356781,13.1566326950211,
131.105769753584)) ;
#129325=CARTESIAN_POINT('Ctrl Pts',(-17.2355632547082,12.867030876862,131.206793603253)) ;
#129326=CARTESIAN_POINT('Ctrl Pts',(-17.3056751958271,12.6146257470566,
131.378333046807)) ;
#129327=CARTESIAN_POINT('Ctrl Pts',(-17.3950652766615,12.4216271704312,
131.606329591747)) ;
#129328=CARTESIAN_POINT('Ctrl Pts',(-17.4976480194487,12.300493633533,131.873019824707)) ;
#129329=CARTESIAN_POINT('Ctrl Pts',(-17.6082564491324,12.2591976943658,
132.162874367726)) ;
#129330=CARTESIAN_POINT('Ctrl Pts',(-17.7179433027061,12.3014766472521,
132.450298613622)) ;
#129331=CARTESIAN_POINT('Ctrl Pts',(-17.8208530116508,12.4236752420719,
132.717812378939)) ;
#129332=CARTESIAN_POINT('Ctrl Pts',(-17.9104061848678,12.619137551761,132.946096908335)) ;
#129333=CARTESIAN_POINT('Ctrl Pts',(-17.9797132762857,12.8707902283033,
133.115494618903)) ;
#129334=CARTESIAN_POINT('Ctrl Pts',(-18.0253753807221,13.1617413070734,
133.215817708573)) ;
#129335=CARTESIAN_POINT('Ctrl Pts',(-18.0448283846108,13.4713352459494,
133.239583447541)) ;
#129336=CARTESIAN_POINT('Ctrl Pts',(-18.0373267145574,13.778502178637,133.18449510648)) ;
#129337=CARTESIAN_POINT('Ctrl Pts',(-18.0040868616542,14.0596468984735,
133.054277364002)) ;
#129338=CARTESIAN_POINT('Ctrl Pts',(-17.9482804203993,14.2953142204187,
132.858131971183)) ;
#129339=CARTESIAN_POINT('Ctrl Pts',(-17.8743218367002,14.4689647045759,
132.608853860417)) ;
#129340=CARTESIAN_POINT('Ctrl Pts',(-17.7886594980501,14.5668407202151,
132.325472650321)) ;
#129341=CARTESIAN_POINT('Ctrl Pts',(-17.6984985567359,14.5831863672356,
132.029126031664)) ;
#129342=CARTESIAN_POINT('Ctrl Pts',(-17.6096304985475,14.5160479467046,
131.736214040919)) ;
#129343=CARTESIAN_POINT('Ctrl Pts',(-17.5307892260312,14.371057406114,131.472871564187)) ;
#129344=CARTESIAN_POINT('Ctrl Pts',(-17.4674191397048,14.1586832935138,
131.254698279897)) ;
#129345=CARTESIAN_POINT('Ctrl Pts',(-17.4247767870597,13.8924169027706,
131.096926633318)) ;
#129346=CARTESIAN_POINT('Ctrl Pts',(-17.4069871935266,13.5934591668299,
131.01187365005)) ;
#129347=CARTESIAN_POINT('Ctrl Pts',(-17.4158629113068,13.2817950572783,
131.004657265815)) ;
#129348=CARTESIAN_POINT('Ctrl Pts',(-17.4515297582126,12.9807521840059,
131.07575753327)) ;
#129349=CARTESIAN_POINT('Ctrl Pts',(-17.5120221179879,12.7114089548823,
131.219401548135)) ;
#129350=CARTESIAN_POINT('Ctrl Pts',(-17.5942883632725,12.4920356351317,
131.426490532179)) ;
#129351=CARTESIAN_POINT('Ctrl Pts',(-17.6923381457244,12.3404092688171,
131.679857275332)) ;
#129352=CARTESIAN_POINT('Ctrl Pts',(-17.8005326892055,12.2658594334509,
131.962769942963)) ;
#129353=CARTESIAN_POINT('Ctrl Pts',(-17.9115353857862,12.2744067631739,
132.253913270118)) ;
#129354=CARTESIAN_POINT('Ctrl Pts',(-18.0181294194039,12.3651073313828,
132.532197896733)) ;
#129355=CARTESIAN_POINT('Ctrl Pts',(-18.1135581728837,12.5316552187529,
132.777840247102)) ;
#129356=CARTESIAN_POINT('Ctrl Pts',(-18.1916435512604,12.7621960771077,
132.972806338441)) ;
#129357=CARTESIAN_POINT('Ctrl Pts',(-18.2474496440388,13.0400248542652,
133.102701427836)) ;
#129358=CARTESIAN_POINT('Ctrl Pts',(-18.2777567173541,13.3449924415224,
133.158139314612)) ;
#129359=CARTESIAN_POINT('Ctrl Pts',(-18.2811288977963,13.6560823827408,
133.134834483101)) ;
#129360=CARTESIAN_POINT('Ctrl Pts',(-18.2581110947125,13.9495229886617,
133.034546912265)) ;
#129361=CARTESIAN_POINT('Ctrl Pts',(-18.2110303763221,14.2060601785511,
132.863887514519)) ;
#129362=CARTESIAN_POINT('Ctrl Pts',(-18.1437370687427,14.406853356067,132.63409799875)) ;
#129363=CARTESIAN_POINT('Ctrl Pts',(-18.0622395109045,14.5364834433348,
132.362928416151)) ;
#129364=CARTESIAN_POINT('Ctrl Pts',(-17.9728141363402,14.5865952299809,
132.068568266676)) ;
#129365=CARTESIAN_POINT('Ctrl Pts',(-17.8826496229748,14.5532896957255,
131.772047908953)) ;
#129366=CARTESIAN_POINT('Ctrl Pts',(-17.7989857572976,14.4391769984152,
131.494542329969)) ;
#129367=CARTESIAN_POINT('Ctrl Pts',(-17.7284523059313,14.2521193913653,
131.255364723917)) ;
#129368=CARTESIAN_POINT('Ctrl Pts',(-17.6769029344046,14.0064609984077,
131.07172935955)) ;
#129369=CARTESIAN_POINT('Ctrl Pts',(-17.6485455441953,13.7162751815943,
130.955532254004)) ;
#129370=CARTESIAN_POINT('Ctrl Pts',(-17.6465647200914,13.4088590373153,
130.916820567134)) ;
#129371=CARTESIAN_POINT('Ctrl Pts',(-17.6713883006356,13.1005339058846,
130.956196977989)) ;
#129372=CARTESIAN_POINT('Ctrl Pts',(-17.7223049769936,12.8153801533597,
131.071793160456)) ;
#129373=CARTESIAN_POINT('Ctrl Pts',(-17.7959144365943,12.5742829537778,
131.253789203923)) ;
#129374=CARTESIAN_POINT('Ctrl Pts',(-17.8889904476805,12.392420790546,131.492309375237)) ;
#129375=CARTESIAN_POINT('Ctrl Pts',(-17.9933039878901,12.2864008615048,
131.764116093955)) ;
#129376=CARTESIAN_POINT('Ctrl Pts',(-18.1044185442691,12.2608494064564,
132.055456688157)) ;
#129377=CARTESIAN_POINT('Ctrl Pts',(-18.2132410021539,12.3186106427626,
132.340370823926)) ;
#129378=CARTESIAN_POINT('Ctrl Pts',(-18.3141761412567,12.4554522853447,
132.602062304633)) ;
#129379=CARTESIAN_POINT('Ctrl Pts',(-18.4001753853872,12.6626734835884,
132.820045754456)) ;
#129380=CARTESIAN_POINT('Ctrl Pts',(-18.4651186131618,12.9221025323028,
132.97681686488)) ;
#129381=CARTESIAN_POINT('Ctrl Pts',(-18.506216134943,13.2188657935947,133.063721914555)) ;
#129382=CARTESIAN_POINT('Ctrl Pts',(-18.5205724335731,13.5309968714097,
133.072441184273)) ;
#129383=CARTESIAN_POINT('Ctrl Pts',(-18.5081122278569,13.833390940375,133.00304473488)) ;
#129384=CARTESIAN_POINT('Ctrl Pts',(-18.4702838423824,14.1082731705155,
132.859326713092)) ;
#129385=CARTESIAN_POINT('Ctrl Pts',(-18.4106469707941,14.3332733281916,
132.651988018231)) ;
#129386=CARTESIAN_POINT('Ctrl Pts',(-18.3341547682758,14.4930898845826,
132.395391176241)) ;
#129387=CARTESIAN_POINT('Ctrl Pts',(-18.2472492763834,14.5762694584335,
132.108457428325)) ;
#129388=CARTESIAN_POINT('Ctrl Pts',(-18.1560969095704,14.5766426622739,
131.80889569352)) ;
#129389=CARTESIAN_POINT('Ctrl Pts',(-18.0694735665927,14.4950562230295,
131.522934074583)) ;
#129390=CARTESIAN_POINT('Ctrl Pts',(-17.9924950396233,14.3357813404639,
131.264798925683)) ;
#129391=CARTESIAN_POINT('Ctrl Pts',(-17.9327493732592,14.1117727148765,
131.05719510321)) ;
#129392=CARTESIAN_POINT('Ctrl Pts',(-17.8945803168045,13.8385113362907,
130.912589041417)) ;
#129393=CARTESIAN_POINT('Ctrl Pts',(-17.8817102320289,13.5338963360909,
130.841724345729)) ;
#129394=CARTESIAN_POINT('Ctrl Pts',(-17.895635047292,13.2242576561067,130.849457214998)) ;
#129395=CARTESIAN_POINT('Ctrl Pts',(-17.9363339259406,12.9262819739174,
130.935110268932)) ;
#129396=CARTESIAN_POINT('Ctrl Pts',(-18.0011613255471,12.6654698991639,
131.091455088112)) ;
#129397=CARTESIAN_POINT('Ctrl Pts',(-18.0871709850437,12.4574146452965,
131.309403426712)) ;
#129398=CARTESIAN_POINT('Ctrl Pts',(-18.1869663728995,12.3205165730399,
131.56807852545)) ;
#129399=CARTESIAN_POINT('Ctrl Pts',(-18.2966682093311,12.2610390486759,
131.855260917825)) ;
#129400=CARTESIAN_POINT('Ctrl Pts',(-18.4069695860607,12.2851065048332,
132.144493068143)) ;
#129401=CARTESIAN_POINT('Ctrl Pts',(-18.5126034033374,12.3913707363663,
132.419764922562)) ;
#129402=CARTESIAN_POINT('Ctrl Pts',(-18.6047688956456,12.5705078611999,
132.656013947326)) ;
#129403=CARTESIAN_POINT('Ctrl Pts',(-18.6790012787559,12.8110530748773,
132.839741264095)) ;
#129404=CARTESIAN_POINT('Ctrl Pts',(-18.7302911873267,13.0958080893831,
132.956423482839)) ;
#129405=CARTESIAN_POINT('Ctrl Pts',(-18.7555799964295,13.4043791335754,
132.997109048956)) ;
#129406=CARTESIAN_POINT('Ctrl Pts',(-18.7539405429472,13.7127503625776,
132.959310086933)) ;
#129407=CARTESIAN_POINT('Ctrl Pts',(-18.7258293961936,14.003146544252,132.843838523491)) ;
#129408=CARTESIAN_POINT('Ctrl Pts',(-18.6749537414129,14.2480984913921,
132.662380092603)) ;
#129409=CARTESIAN_POINT('Ctrl Pts',(-18.6044230138764,14.4370589151547,
132.423074769983)) ;
#129410=CARTESIAN_POINT('Ctrl Pts',(-18.520996512227,14.5521322459825,132.146306985102)) ;
#129411=CARTESIAN_POINT('Ctrl Pts',(-18.4306794059455,14.5867077629414,
131.849264763677)) ;
#129412=CARTESIAN_POINT('Ctrl Pts',(-18.3413660662321,14.5378478997284,
131.555300337176)) ;
#129413=CARTESIAN_POINT('Ctrl Pts',(-18.2596531854169,14.4092030440239,
131.283472890356)) ;
#129414=CARTESIAN_POINT('Ctrl Pts',(-18.1923026345111,14.2102655467961,
131.053642197071)) ;
#129415=CARTESIAN_POINT('Ctrl Pts',(-18.1446121318789,13.9531165249686,
130.881020749285)) ;
#129416=CARTESIAN_POINT('Ctrl Pts',(-18.1213237510083,13.6605445823028,
130.780006916634)) ;
#129417=CARTESIAN_POINT('Ctrl Pts',(-18.1242927670225,13.3493860420966,
130.755504301991)) ;
#129418=CARTESIAN_POINT('Ctrl Pts',(-18.1541961965779,13.0444136066678,
130.809790357298)) ;
#129419=CARTESIAN_POINT('Ctrl Pts',(-18.2096856771492,12.7658509592001,
130.938737600815)) ;
#129420=CARTESIAN_POINT('Ctrl Pts',(-18.2874255648017,12.5346699181632,
131.132718784265)) ;
#129421=CARTESIAN_POINT('Ctrl Pts',(-18.3827232290827,12.3668713397562,
131.37794706254)) ;
#129422=CARTESIAN_POINT('Ctrl Pts',(-18.4894019331544,12.2750736667704,
131.656423092485)) ;
#129423=CARTESIAN_POINT('Ctrl Pts',(-18.5999461896796,12.2654123740739,
131.946360057731)) ;
#129424=CARTESIAN_POINT('Ctrl Pts',(-18.7082699182573,12.338500075334,132.229645795639)) ;
#129425=CARTESIAN_POINT('Ctrl Pts',(-18.8066956525215,12.4893940348924,
132.484046512348)) ;
#129426=CARTESIAN_POINT('Ctrl Pts',(-18.8890064060484,12.7071834548376,
132.691365787329)) ;
#129427=CARTESIAN_POINT('Ctrl Pts',(-18.9499792122234,12.9760085814995,
132.836382852014)) ;
#129428=CARTESIAN_POINT('Ctrl Pts',(-18.986083387819,13.2771670277102,132.908713665755)) ;
#129429=CARTESIAN_POINT('Ctrl Pts',(-18.9953771961304,13.5885362669385,
132.902752796309)) ;
#129430=CARTESIAN_POINT('Ctrl Pts',(-18.9779428841239,13.8883473983697,
132.818679469177)) ;
#129431=CARTESIAN_POINT('Ctrl Pts',(-18.935738241321,14.1546796544185,132.662259619512)) ;
#129432=CARTESIAN_POINT('Ctrl Pts',(-18.8726034800023,14.3683944607912,
132.444729796403)) ;
#129433=CARTESIAN_POINT('Ctrl Pts',(-18.7937232819521,14.5146640106003,
132.181190970799)) ;
#129434=CARTESIAN_POINT('Ctrl Pts',(-18.7051646808948,14.5827891509108,
131.889269134723)) ;
#129435=CARTESIAN_POINT('Ctrl Pts',(-18.6147024524246,14.5676066114005,
131.59193939095)) ;
#129436=CARTESIAN_POINT('Ctrl Pts',(-18.5290201629713,14.4706131467255,
131.308524406706)) ;
#129437=CARTESIAN_POINT('Ctrl Pts',(-18.4550931376209,14.2987449409649,
131.059463494934)) ;
#129438=CARTESIAN_POINT('Ctrl Pts',(-18.3987987744585,14.063095845739,130.861778311655)) ;
#129439=CARTESIAN_POINT('Ctrl Pts',(-18.3653036692505,13.783320877813,130.730918820104)) ;
#129440=CARTESIAN_POINT('Ctrl Pts',(-18.3573754310237,13.4754883561184,
130.674484167362)) ;
#129441=CARTESIAN_POINT('Ctrl Pts',(-18.3764169558807,13.1664273020677,
130.697118916392)) ;
#129442=CARTESIAN_POINT('Ctrl Pts',(-18.4217940683259,12.8743475374644,
130.796531690104)) ;
#129443=CARTESIAN_POINT('Ctrl Pts',(-18.4908985820318,12.6220180754337,
130.965320118566)) ;
#129444=CARTESIAN_POINT('Ctrl Pts',(-18.5798731137621,12.4263341505379,
131.192035756237)) ;
#129445=CARTESIAN_POINT('Ctrl Pts',(-18.6827398919646,12.3026056588691,
131.459379942869)) ;
#129446=CARTESIAN_POINT('Ctrl Pts',(-18.7925820657954,12.2593725245785,
131.747194451469)) ;
#129447=CARTESIAN_POINT('Ctrl Pts',(-18.902507639715,12.2987734031186,132.035285394968)) ;
#129448=CARTESIAN_POINT('Ctrl Pts',(-19.0064670714771,12.4202091784099,
132.305601611935)) ;
#129449=CARTESIAN_POINT('Ctrl Pts',(-19.0954848269158,12.6117736557302,
132.532691445471)) ;
#129450=CARTESIAN_POINT('Ctrl Pts',(-19.1658110426442,12.8626551517495,
132.704935652386)) ;
#129451=CARTESIAN_POINT('Ctrl Pts',(-19.2121697896248,13.1527448205317,
132.807303457746)) ;
#129452=CARTESIAN_POINT('Ctrl Pts',(-19.2324491817657,13.4624297632054,
132.833446100144)) ;
#129453=CARTESIAN_POINT('Ctrl Pts',(-19.225671158967,13.7701810558333,132.780451712219)) ;
#129454=CARTESIAN_POINT('Ctrl Pts',(-19.1932078332292,14.0517728078933,
132.65257011804)) ;
#129455=CARTESIAN_POINT('Ctrl Pts',(-19.1379946589808,14.2892526496134,
132.458138372292)) ;
#129456=CARTESIAN_POINT('Ctrl Pts',(-19.0644566698038,14.4648239971076,
132.210085328861)) ;
#129457=CARTESIAN_POINT('Ctrl Pts',(-18.9793343757348,14.5650402955601,
131.928386517091)) ;
#129458=CARTESIAN_POINT('Ctrl Pts',(-18.8886434300041,14.5837489624633,
131.630274823525)) ;
#129459=CARTESIAN_POINT('Ctrl Pts',(-18.8004173888174,14.5197168158782,
131.339551521014)) ;
#129460=CARTESIAN_POINT('Ctrl Pts',(-18.7206220160406,14.3763315271282,
131.073195599226)) ;
#129461=CARTESIAN_POINT('Ctrl Pts',(-18.6567617236485,14.1656646034779,
130.853606216677)) ;
#129462=CARTESIAN_POINT('Ctrl Pts',(-18.6133812442094,13.8999129369224,
130.693587403167)) ;
#129463=CARTESIAN_POINT('Ctrl Pts',(-18.5949518753934,13.6028236441132,
130.60680394849)) ;
#129464=CARTESIAN_POINT('Ctrl Pts',(-18.6029793109596,13.291184662554,130.597103250091)) ;
#129465=CARTESIAN_POINT('Ctrl Pts',(-18.6378459697723,12.9894031508225,
130.665859260079)) ;
#129466=CARTESIAN_POINT('Ctrl Pts',(-18.697941222039,12.7177660513116,130.808203300005)) ;
#129467=CARTESIAN_POINT('Ctrl Pts',(-18.7796120718618,12.4972590440602,
131.013603451076)) ;
#129468=CARTESIAN_POINT('Ctrl Pts',(-18.8769989032459,12.3438957808923,
131.265123551428)) ;
#129469=CARTESIAN_POINT('Ctrl Pts',(-18.9850989880041,12.2668705331881,
131.547727750457)) ;
#129470=CARTESIAN_POINT('Ctrl Pts',(-19.0959985748491,12.2729077976525,
131.838609074605)) ;
#129471=CARTESIAN_POINT('Ctrl Pts',(-19.20298136002,12.3614501040313,132.11797427254)) ;
#129472=CARTESIAN_POINT('Ctrl Pts',(-19.2985829203928,12.5253314471916,
132.364220122057)) ;
#129473=CARTESIAN_POINT('Ctrl Pts',(-19.3776055221514,12.7552769702176,
132.561768746383)) ;
#129474=CARTESIAN_POINT('Ctrl Pts',(-19.4338889635372,13.0310568986237,
132.693180609869)) ;
#129475=CARTESIAN_POINT('Ctrl Pts',(-19.4650400815724,13.3361216893249,
132.751012638428)) ;
#129476=CARTESIAN_POINT('Ctrl Pts',(-19.4692309832608,13.6463104400421,
132.730217010446)) ;
#129477=CARTESIAN_POINT('Ctrl Pts',(-19.4468478616773,13.9424873380838,
132.631569354452)) ;
#129478=CARTESIAN_POINT('Ctrl Pts',(-19.4002106692333,14.2002008792275,
132.462183820064)) ;
#129479=CARTESIAN_POINT('Ctrl Pts',(-19.3338735917494,14.4015262359145,
132.235406621368)) ;
#129480=CARTESIAN_POINT('Ctrl Pts',(-19.2525009705936,14.5339054889456,
131.964504538039)) ;
#129481=CARTESIAN_POINT('Ctrl Pts',(-19.1632581585291,14.5863178639959,
131.670702154855)) ;
#129482=CARTESIAN_POINT('Ctrl Pts',(-19.0727741133847,14.5553221796482,
131.373161193195)) ;
#129483=CARTESIAN_POINT('Ctrl Pts',(-18.9888934197537,14.4431215079252,
131.095027066642)) ;
#129484=CARTESIAN_POINT('Ctrl Pts',(-18.9181460716304,14.2589451950462,
130.855367504887)) ;
#129485=CARTESIAN_POINT('Ctrl Pts',(-18.8657380795338,14.0132050908334,
130.66902315173)) ;
#129486=CARTESIAN_POINT('Ctrl Pts',(-18.836868487838,13.7264814717307,130.551624398978)) ;
#129487=CARTESIAN_POINT('Ctrl Pts',(-18.8340276274913,13.4166671207193,
130.510102042886)) ;
#129488=CARTESIAN_POINT('Ctrl Pts',(-18.8581413024745,13.1090562113246,
130.54751765992)) ;
#129489=CARTESIAN_POINT('Ctrl Pts',(-18.9083034310326,12.8228936758021,
130.660907356979)) ;
#129490=CARTESIAN_POINT('Ctrl Pts',(-18.9813885580166,12.5803482632518,
130.841359582256)) ;
#129491=CARTESIAN_POINT('Ctrl Pts',(-19.0735507529948,12.3971382948885,
131.077360101158)) ;
#129492=CARTESIAN_POINT('Ctrl Pts',(-19.1781196028754,12.2881794831016,
131.349740136877)) ;
#129493=CARTESIAN_POINT('Ctrl Pts',(-19.2889977456715,12.260444772771,131.640444771833)) ;
#129494=CARTESIAN_POINT('Ctrl Pts',(-19.3981903193112,12.3158800352752,
131.926374136199)) ;
#129495=CARTESIAN_POINT('Ctrl Pts',(-19.4995415293124,12.4512315889953,
132.189227462612)) ;
#129496=CARTESIAN_POINT('Ctrl Pts',(-19.5853658796549,12.6546809056087,
132.406990274991)) ;
#129497=CARTESIAN_POINT('Ctrl Pts',(-19.6515319436579,12.9147730695688,
132.567062358423)) ;
#129498=CARTESIAN_POINT('Ctrl Pts',(-19.6931210807734,13.2095558762223,
132.655557138369)) ;
#129499=CARTESIAN_POINT('Ctrl Pts',(-19.7083399050478,13.5223873446286,
132.666701944993)) ;
#129500=CARTESIAN_POINT('Ctrl Pts',(-19.69663409254,13.8250174171808,132.599547279371)) ;
#129501=CARTESIAN_POINT('Ctrl Pts',(-19.6592874859553,14.1019894892023,
132.457105233325)) ;
#129502=CARTESIAN_POINT('Ctrl Pts',(-19.6004579577044,14.3273312033298,
132.252294538842)) ;
#129503=CARTESIAN_POINT('Ctrl Pts',(-19.5244720497105,14.4893435077641,
131.997198017204)) ;
#129504=CARTESIAN_POINT('Ctrl Pts',(-19.437681105912,14.5749599942803,131.710560595662)) ;
#129505=CARTESIAN_POINT('Ctrl Pts',(-19.3466336963598,14.5779281388509,
131.411346196059)) ;
#129506=CARTESIAN_POINT('Ctrl Pts',(-19.2595748253476,14.498336569716,131.124014432636)) ;
#129507=CARTESIAN_POINT('Ctrl Pts',(-19.1825234436999,14.3420896850988,
130.865828840705)) ;
#129508=CARTESIAN_POINT('Ctrl Pts',(-19.1217474070917,14.1180212398974,
130.65495238919)) ;
#129509=CARTESIAN_POINT('Ctrl Pts',(-19.0832131949706,13.8471809568527,
130.509458949016)) ;
#129510=CARTESIAN_POINT('Ctrl Pts',(-19.0694761171171,13.5439414016218,
130.436135704644)) ;
#129511=CARTESIAN_POINT('Ctrl Pts',(-19.0826209143411,13.2331635587154,
130.441478853736)) ;
#129512=CARTESIAN_POINT('Ctrl Pts',(-19.1225909328652,12.9343809245396,
130.524995993454)) ;
#129513=CARTESIAN_POINT('Ctrl Pts',(-19.1868549465641,12.6721978750302,
130.679668772817)) ;
#129514=CARTESIAN_POINT('Ctrl Pts',(-19.2718327033345,12.4632419957696,
130.894780682372)) ;
#129515=CARTESIAN_POINT('Ctrl Pts',(-19.3718814394105,12.3231158873288,
131.15398475223)) ;
#129516=CARTESIAN_POINT('Ctrl Pts',(-19.4814339775529,12.2616017925994,
131.440740961046)) ;
#129517=CARTESIAN_POINT('Ctrl Pts',(-19.5915908616456,12.2833201710628,
131.729606330629)) ;
#129518=CARTESIAN_POINT('Ctrl Pts',(-19.6972964626275,12.3868877150975,
132.005156858411)) ;
#129519=CARTESIAN_POINT('Ctrl Pts',(-19.7903372888288,12.5648231149356,
132.243814036882)) ;
#129520=CARTESIAN_POINT('Ctrl Pts',(-19.8650354915899,12.8039601972563,
132.428918682179)) ;
#129521=CARTESIAN_POINT('Ctrl Pts',(-19.9168574250491,13.0864728883471,
132.547293299101)) ;
#129522=CARTESIAN_POINT('Ctrl Pts',(-19.9430599792711,13.395723837035,132.590534558758)) ;
#129523=CARTESIAN_POINT('Ctrl Pts',(-19.9420838172202,13.7038340403903,
132.554720244707)) ;
#129524=CARTESIAN_POINT('Ctrl Pts',(-19.9150775602916,13.9936201443638,
132.442686741954)) ;
#129525=CARTESIAN_POINT('Ctrl Pts',(-19.8641327250296,14.2431366577781,
132.26059214858)) ;
#129526=CARTESIAN_POINT('Ctrl Pts',(-19.7947524623111,14.4318623943572,
132.025001777215)) ;
#129527=CARTESIAN_POINT('Ctrl Pts',(-19.7110993425975,14.5502397442867,
131.747339740325)) ;
#129528=CARTESIAN_POINT('Ctrl Pts',(-19.6210900248515,14.5868194741509,
131.45129107148)) ;
#129529=CARTESIAN_POINT('Ctrl Pts',(-19.5315525619792,14.5403267808585,
131.156626982103)) ;
#129530=CARTESIAN_POINT('Ctrl Pts',(-19.449546684465,14.4138414992085,130.883957172776)) ;
#129531=CARTESIAN_POINT('Ctrl Pts',(-19.3816932266418,14.2163547115684,
130.65261934202)) ;
#129532=CARTESIAN_POINT('Ctrl Pts',(-19.3336313323173,13.9624648084783,
130.479143370895)) ;
#129533=CARTESIAN_POINT('Ctrl Pts',(-19.3093924490461,13.6693367941651,
130.375182192518)) ;
#129534=CARTESIAN_POINT('Ctrl Pts',(-19.3116017990212,13.3586798877786,
130.34850063673)) ;
#129535=CARTESIAN_POINT('Ctrl Pts',(-19.3407729872782,13.0526930051948,
130.400586269807)) ;
#129536=CARTESIAN_POINT('Ctrl Pts',(-19.3955780422064,12.7731728607976,
130.527545202649)) ;
#129537=CARTESIAN_POINT('Ctrl Pts',(-19.4727496969172,12.5404162495143,
130.719864313944)) ;
#129538=CARTESIAN_POINT('Ctrl Pts',(-19.5675241391113,12.3707608334166,
130.963600443702)) ;
#129539=CARTESIAN_POINT('Ctrl Pts',(-19.6739461692788,12.2766729754023,
131.241329946705)) ;
#129540=CARTESIAN_POINT('Ctrl Pts',(-19.7844202480155,12.2643218379507,
131.531079921362)) ;
#129541=CARTESIAN_POINT('Ctrl Pts',(-19.8937077378551,12.3360206173623,
131.816927019485)) ;
#129542=CARTESIAN_POINT('Ctrl Pts',(-19.9915672517583,12.4836396452835,
132.069982162294)) ;
#129543=CARTESIAN_POINT('Ctrl Pts',(-20.0748105489094,12.7003318361734,
132.279890008997)) ;
#129544=CARTESIAN_POINT('Ctrl Pts',(-20.1363655459467,12.9678916740203,
132.426631430434)) ;
#129545=CARTESIAN_POINT('Ctrl Pts',(-20.1732514845702,13.2687868226262,
132.501204712146)) ;
#129546=CARTESIAN_POINT('Ctrl Pts',(-20.1832535485897,13.5800033962545,
132.497330904926)) ;
#129547=CARTESIAN_POINT('Ctrl Pts',(-20.1665976689407,13.8799728738773,
132.415585091986)) ;
#129548=CARTESIAN_POINT('Ctrl Pts',(-20.1250490907357,14.1476993247652,
132.261063926315)) ;
#129549=CARTESIAN_POINT('Ctrl Pts',(-20.0624312334712,14.3632524005006,
132.045033139331)) ;
#129550=CARTESIAN_POINT('Ctrl Pts',(-19.9836617187187,14.5119335521308,
131.781720626237)) ;
#129551=CARTESIAN_POINT('Ctrl Pts',(-19.8953363000053,14.5819602078055,
131.490511990821)) ;
#129552=CARTESIAN_POINT('Ctrl Pts',(-19.8051206025169,14.5692454474693,
131.19400539406)) ;
#129553=CARTESIAN_POINT('Ctrl Pts',(-19.7189975522154,14.4742855004693,
130.909223014787)) ;
#129554=CARTESIAN_POINT('Ctrl Pts',(-19.6448612455928,14.3047439678629,
130.659636036259)) ;
#129555=CARTESIAN_POINT('Ctrl Pts',(-19.5879650946849,14.0710831645145,
130.460223445624)) ;
#129556=CARTESIAN_POINT('Ctrl Pts',(-19.5536759796393,13.7914036967699,
130.326934250486)) ;
#129557=CARTESIAN_POINT('Ctrl Pts',(-19.5450263082221,13.4850123615767,
130.268502128271)) ;
#129558=CARTESIAN_POINT('Ctrl Pts',(-19.5632218429817,13.1755844342699,
130.28864920662)) ;
#129559=CARTESIAN_POINT('Ctrl Pts',(-19.6079242224571,12.8823157939158,
130.386049430084)) ;
#129560=CARTESIAN_POINT('Ctrl Pts',(-19.6763866082576,12.6284363118315,
130.552956035433)) ;
#129561=CARTESIAN_POINT('Ctrl Pts',(-19.7652804875288,12.430459524885,130.779306976383)) ;
#129562=CARTESIAN_POINT('Ctrl Pts',(-19.8670137067598,12.3053999545834,
131.043605735168)) ;
#129563=CARTESIAN_POINT('Ctrl Pts',(-19.9776324212504,12.259348439198,131.333414105612)) ;
#129564=CARTESIAN_POINT('Ctrl Pts',(-20.0871279899776,12.2965483927982,
131.620409141885)) ;
#129565=CARTESIAN_POINT('Ctrl Pts',(-20.1914568507578,12.4156949329505,
131.891780020066)) ;
#129566=CARTESIAN_POINT('Ctrl Pts',(-20.280854617759,12.6050470822163,132.120029243764)) ;
#129567=CARTESIAN_POINT('Ctrl Pts',(-20.3519885949918,12.8553420961893,
132.294524748666)) ;
#129568=CARTESIAN_POINT('Ctrl Pts',(-20.3988624504608,13.1429454488516,
132.398581522686)) ;
#129569=CARTESIAN_POINT('Ctrl Pts',(-20.4200768369222,13.454391681807,132.427234220689)) ;
#129570=CARTESIAN_POINT('Ctrl Pts',(-20.4140136595561,13.7614619706277,
132.376445903007)) ;
#129571=CARTESIAN_POINT('Ctrl Pts',(-20.382192794584,14.0447127899292,132.250363159201)) ;
#129572=CARTESIAN_POINT('Ctrl Pts',(-20.327675093214,14.2828872647388,132.058058028165)) ;
#129573=CARTESIAN_POINT('Ctrl Pts',(-20.2549076280567,14.4603132079677,
131.812365927047)) ;
#129574=CARTESIAN_POINT('Ctrl Pts',(-20.1693733796987,14.5634617296136,
131.529204042072)) ;
#129575=CARTESIAN_POINT('Ctrl Pts',(-20.0794263338298,14.5844329944993,
131.233527995781)) ;
#129576=CARTESIAN_POINT('Ctrl Pts',(-19.9904362428095,14.5225343745256,
130.94034258586)) ;
#129577=CARTESIAN_POINT('Ctrl Pts',(-19.910574928501,14.3815448921276,130.673908872332)) ;
#129578=CARTESIAN_POINT('Ctrl Pts',(-19.8461411447143,14.1725755942996,
130.452618521442)) ;
#129579=CARTESIAN_POINT('Ctrl Pts',(-19.8022333693109,13.9093042080622,
130.291199800478)) ;
#129580=CARTESIAN_POINT('Ctrl Pts',(-19.7828574602038,13.6121560169538,
130.201553405444)) ;
#129581=CARTESIAN_POINT('Ctrl Pts',(-19.7902297852299,13.2990172973707,
130.189775599945)) ;
#129582=CARTESIAN_POINT('Ctrl Pts',(-19.8242499060709,12.9981567008458,
130.256216408043)) ;
#129583=CARTESIAN_POINT('Ctrl Pts',(-19.8834591196413,12.7257034100229,
130.396033289139)) ;
#129584=CARTESIAN_POINT('Ctrl Pts',(-19.9646135502491,12.503075938083,130.599887232167)) ;
#129585=CARTESIAN_POINT('Ctrl Pts',(-20.061806489816,12.3471530516957,130.850770434248)) ;
#129586=CARTESIAN_POINT('Ctrl Pts',(-20.1701165293733,12.2678408813101,
131.133870309601)) ;
#129587=CARTESIAN_POINT('Ctrl Pts',(-20.2803843836627,12.2715868988579,
131.423098040257)) ;
#129588=CARTESIAN_POINT('Ctrl Pts',(-20.3877234956396,12.3575775425478,
131.703470304113)) ;
#129589=CARTESIAN_POINT('Ctrl Pts',(-20.4838861019967,12.519859116392,131.95129175679)) ;
#129590=CARTESIAN_POINT('Ctrl Pts',(-20.563259553875,12.7472699624983,132.149979635772)) ;
#129591=CARTESIAN_POINT('Ctrl Pts',(-20.6205129961937,13.0233713370029,
132.284051353102)) ;
#129592=CARTESIAN_POINT('Ctrl Pts',(-20.652239731686,13.3264774087469,132.343728948937)) ;
#129593=CARTESIAN_POINT('Ctrl Pts',(-20.6572910380726,13.6374828083211,
132.325371821783)) ;
#129594=CARTESIAN_POINT('Ctrl Pts',(-20.6356455845063,13.9340521911672,
132.228917738845)) ;
#129595=CARTESIAN_POINT('Ctrl Pts',(-20.589784029738,14.193123894667,132.061824915611)) ;
#129596=CARTESIAN_POINT('Ctrl Pts',(-20.5234609844462,14.3974304405376,
131.83486651278)) ;
#129597=CARTESIAN_POINT('Ctrl Pts',(-20.4428898145144,14.5309245304013,
131.566514750519)) ;
#129598=CARTESIAN_POINT('Ctrl Pts',(-20.3537343109642,14.5859814529116,
131.272940165148)) ;
#129599=CARTESIAN_POINT('Ctrl Pts',(-20.2633620898879,14.5574777921035,
130.975793218994)) ;
#129600=CARTESIAN_POINT('Ctrl Pts',(-20.179134864296,14.4480150679812,130.696649838046)) ;
#129601=CARTESIAN_POINT('Ctrl Pts',(-20.1074565079211,14.2640747016683,
130.454011423191)) ;
#129602=CARTESIAN_POINT('Ctrl Pts',(-20.0549222211513,14.0222278748094,
130.267625814599)) ;
#129603=CARTESIAN_POINT('Ctrl Pts',(-20.0250364103788,13.7339092268223,
130.146949963196)) ;
#129604=CARTESIAN_POINT('Ctrl Pts',(-20.0215334625323,13.4264443315917,
130.103724396133)) ;
#129605=CARTESIAN_POINT('Ctrl Pts',(-20.0448205353659,13.117933729061,130.138658618017)) ;
#129606=CARTESIAN_POINT('Ctrl Pts',(-20.0942215492142,12.8308236543942,
130.249839143416)) ;
#129607=CARTESIAN_POINT('Ctrl Pts',(-20.1670498129061,12.5859821244952,
130.429403729018)) ;
#129608=CARTESIAN_POINT('Ctrl Pts',(-20.2580898691565,12.4020104693658,
130.662363596137)) ;
#129609=CARTESIAN_POINT('Ctrl Pts',(-20.3630369251127,12.2899875702474,
130.935630330481)) ;
#129610=CARTESIAN_POINT('Ctrl Pts',(-20.4732695786483,12.2601247777389,
131.224628401923)) ;
#129611=CARTESIAN_POINT('Ctrl Pts',(-20.5827915134349,12.3130228920766,
131.511459590319)) ;
#129612=CARTESIAN_POINT('Ctrl Pts',(-20.6842801965026,12.4457555265159,
131.774790797317)) ;
#129613=CARTESIAN_POINT('Ctrl Pts',(-20.770956455244,12.6478748445304,131.994929810398)) ;
#129614=CARTESIAN_POINT('Ctrl Pts',(-20.8379046355006,12.90742344953,132.157201250892)) ;
#129615=CARTESIAN_POINT('Ctrl Pts',(-20.8801243826187,13.2015878623563,
132.247531865277)) ;
#129616=CARTESIAN_POINT('Ctrl Pts',(-20.8960762410322,13.513246132059,132.260932671934)) ;
#129617=CARTESIAN_POINT('Ctrl Pts',(-20.8850515631884,13.8170403560637,
132.195686938087)) ;
#129618=CARTESIAN_POINT('Ctrl Pts',(-20.8487392341801,14.0930903285622,
132.056526224254)) ;
#129619=CARTESIAN_POINT('Ctrl Pts',(-20.7903126425234,14.3215764376153,
131.852723944522)) ;
#129620=CARTESIAN_POINT('Ctrl Pts',(-20.71446322452,14.4860163871687,131.59792677398)) ;
#129621=CARTESIAN_POINT('Ctrl Pts',(-20.6277873026751,14.5737421831593,
131.31159505661)) ;
#129622=CARTESIAN_POINT('Ctrl Pts',(-20.5369992850468,14.5789283519424,
131.013226876598)) ;
#129623=CARTESIAN_POINT('Ctrl Pts',(-20.4496947481666,14.5018180781457,
130.725170263346)) ;
#129624=CARTESIAN_POINT('Ctrl Pts',(-20.3720331642646,14.3465572138388,
130.465061663831)) ;
#129625=CARTESIAN_POINT('Ctrl Pts',(-20.3113537180096,14.1268975859946,
130.254856603659)) ;
#129626=CARTESIAN_POINT('Ctrl Pts',(-20.2716879247288,13.8551173333083,
130.105766414134)) ;
#129627=CARTESIAN_POINT('Ctrl Pts',(-20.2572946011384,13.5530514979448,
130.030607450358)) ;
#129628=CARTESIAN_POINT('Ctrl Pts',(-20.2696946884832,13.2415865700778,
130.033701144829)) ;
#129629=CARTESIAN_POINT('Ctrl Pts',(-20.3087706449792,12.9431698181064,
130.114729825383)) ;
#129630=CARTESIAN_POINT('Ctrl Pts',(-20.372493414144,12.6789857022783,130.267737292984)) ;
#129631=CARTESIAN_POINT('Ctrl Pts',(-20.4568543797459,12.4685394355876,
130.481090280765)) ;
#129632=CARTESIAN_POINT('Ctrl Pts',(-20.5565334718935,12.3261975065515,
130.739212503641)) ;
#129633=CARTESIAN_POINT('Ctrl Pts',(-20.6658499559575,12.2622045944374,
131.025302791094)) ;
#129634=CARTESIAN_POINT('Ctrl Pts',(-20.7762684309206,12.2815898104216,
131.314866496193)) ;
#129635=CARTESIAN_POINT('Ctrl Pts',(-20.8819109420116,12.3824517320663,
131.590340001243)) ;
#129636=CARTESIAN_POINT('Ctrl Pts',(-20.9755580922554,12.5585396445524,
131.830713394656)) ;
#129637=CARTESIAN_POINT('Ctrl Pts',(-21.05082616022,12.7954954473237,132.017545647161)) ;
#129638=CARTESIAN_POINT('Ctrl Pts',(-21.1037227225579,13.0796939722615,
132.13875377845)) ;
#129639=CARTESIAN_POINT('Ctrl Pts',(-21.1303775268751,13.3852304092896,
132.18368355125)) ;
#129640=CARTESIAN_POINT('Ctrl Pts',(-21.1302868768095,13.6960444391784,
132.150191483003)) ;
#129641=CARTESIAN_POINT('Ctrl Pts',(-21.103907238212,13.9858667251667,132.040067449433)) ;
#129642=CARTESIAN_POINT('Ctrl Pts',(-21.0539056725473,14.2358877354541,
131.860875963079)) ;
#129643=CARTESIAN_POINT('Ctrl Pts',(-20.9847199038895,14.427599936546,131.625699111867)) ;
#129644=CARTESIAN_POINT('Ctrl Pts',(-20.9012106052768,14.5480862875162,
131.348413046553)) ;
#129645=CARTESIAN_POINT('Ctrl Pts',(-20.8116067569838,14.5868446714445,
131.053662003123)) ;
#129646=CARTESIAN_POINT('Ctrl Pts',(-20.722052724287,14.543035766912,130.758989112208)) ;
#129647=CARTESIAN_POINT('Ctrl Pts',(-20.6396161469712,14.4187440233768,
130.485021247634)) ;
#129648=CARTESIAN_POINT('Ctrl Pts',(-20.5711851083752,14.2230681699305,
130.251972524178)) ;
#129649=CARTESIAN_POINT('Ctrl Pts',(-20.5224081144402,13.9697197802327,
130.076309410298)) ;
#129650=CARTESIAN_POINT('Ctrl Pts',(-20.4975411592122,13.678752384422,129.970666296557)) ;
#129651=CARTESIAN_POINT('Ctrl Pts',(-20.49894769684,13.3668523493994,129.941483136126)) ;
#129652=CARTESIAN_POINT('Ctrl Pts',(-20.5274636510951,13.0606725524935,
129.991675831064)) ;
#129653=CARTESIAN_POINT('Ctrl Pts',(-20.5813628220163,12.7810811870564,
130.116105508458)) ;
#129654=CARTESIAN_POINT('Ctrl Pts',(-20.6578955627211,12.5467078049701,
130.306564715947)) ;
#129655=CARTESIAN_POINT('Ctrl Pts',(-20.7520317982675,12.3750360916392,
130.548492029394)) ;
#129656=CARTESIAN_POINT('Ctrl Pts',(-20.8588402085985,12.2779852659618,
130.827153760842)) ;
#129657=CARTESIAN_POINT('Ctrl Pts',(-20.9691322717098,12.2637459415924,
131.1164165131)) ;
#129658=CARTESIAN_POINT('Ctrl Pts',(-21.0778822448708,12.3321871278704,
131.400920874685)) ;
#129659=CARTESIAN_POINT('Ctrl Pts',(-21.1769911008549,12.4786899197398,
131.657345754661)) ;
#129660=CARTESIAN_POINT('Ctrl Pts',(-21.2606987378686,12.6941597985184,
131.86859423361)) ;
#129661=CARTESIAN_POINT('Ctrl Pts',(-21.3226675980762,12.95948963943,132.016669195354)) ;
#129662=CARTESIAN_POINT('Ctrl Pts',(-21.3603388309651,13.2597800757016,
132.09352869614)) ;
#129663=CARTESIAN_POINT('Ctrl Pts',(-21.3711243868775,13.570593176475,132.091985203962)) ;
#129664=CARTESIAN_POINT('Ctrl Pts',(-21.3552655780944,13.8717553022586,
132.01251606465)) ;
#129665=CARTESIAN_POINT('Ctrl Pts',(-21.3141032516413,14.1416795276356,
131.858976575639)) ;
#129666=CARTESIAN_POINT('Ctrl Pts',(-21.2523927513415,14.3575207602719,
131.645808023395)) ;
#129667=CARTESIAN_POINT('Ctrl Pts',(-21.1737881611546,14.5088742129947,
131.382873338965)) ;
#129668=CARTESIAN_POINT('Ctrl Pts',(-21.0858332477586,14.5810485747374,
131.092827440589)) ;
#129669=CARTESIAN_POINT('Ctrl Pts',(-20.9954536594014,14.5707018423974,
130.79578508898)) ;
#129670=CARTESIAN_POINT('Ctrl Pts',(-20.9093467237376,14.4785663086567,
130.511161766983)) ;
#129671=CARTESIAN_POINT('Ctrl Pts',(-20.8341838994325,14.3096046901172,
130.258300710511)) ;
#129672=CARTESIAN_POINT('Ctrl Pts',(-20.7769970988678,14.0777450848623,
130.058128817237)) ;
#129673=CARTESIAN_POINT('Ctrl Pts',(-20.7421466915136,13.8001342656759,
129.923313470881)) ;
#129674=CARTESIAN_POINT('Ctrl Pts',(-20.732652270712,13.4946153798022,129.862456562529)) ;
#129675=CARTESIAN_POINT('Ctrl Pts',(-20.7501719019214,13.1837407483122,
129.880489260335)) ;
#129676=CARTESIAN_POINT('Ctrl Pts',(-20.7940652768132,12.8901082923596,
129.975587652555)) ;
#129677=CARTESIAN_POINT('Ctrl Pts',(-20.8623834981418,12.6339161097821,
130.141896445246)) ;
#129678=CARTESIAN_POINT('Ctrl Pts',(-20.9494844728681,12.43659258656,130.363483556097)) ;
#129679=CARTESIAN_POINT('Ctrl Pts',(-21.0520547764074,12.3075969650438,
130.629826825371)) ;
#129680=CARTESIAN_POINT('Ctrl Pts',(-21.1615735908753,12.25954136932,130.916733851634)) ;
#129681=CARTESIAN_POINT('Ctrl Pts',(-21.2721798049417,12.2945981234014,
131.206652794523)) ;
#129682=CARTESIAN_POINT('Ctrl Pts',(-21.3757162896064,12.4101972587338,
131.476072258358)) ;
#129683=CARTESIAN_POINT('Ctrl Pts',(-21.4663327145782,12.5987159490307,
131.707623163194)) ;
#129684=CARTESIAN_POINT('Ctrl Pts',(-21.5377865787159,12.8461743758197,
131.883234522718)) ;
#129685=CARTESIAN_POINT('Ctrl Pts',(-21.5858655490026,13.135926237231,131.990455824353)) ;
#129686=CARTESIAN_POINT('Ctrl Pts',(-21.607580328873,13.4447581443412,132.020835164362)) ;
#129687=CARTESIAN_POINT('Ctrl Pts',(-21.602335125879,13.7530929006016,131.972334348118)) ;
#129688=CARTESIAN_POINT('Ctrl Pts',(-21.5713569064062,14.0362080227333,
131.84885121752)) ;
#129689=CARTESIAN_POINT('Ctrl Pts',(-21.5173330548251,14.2769559751065,
131.657874005784)) ;
#129690=CARTESIAN_POINT('Ctrl Pts',(-21.4448194217764,14.4563581668246,
131.412866120982)) ;
#129691=CARTESIAN_POINT('Ctrl Pts',(-21.3601256689141,14.5613193380967,
131.132376374339)) ;
#129692=CARTESIAN_POINT('Ctrl Pts',(-21.269633652782,14.5851466782009,130.834886668731)) ;
#129693=CARTESIAN_POINT('Ctrl Pts',(-21.1804456514604,14.5250094575114,
130.541092527295)) ;
#129694=CARTESIAN_POINT('Ctrl Pts',(-21.1006537832372,14.3871119607425,
130.275049733062)) ;
#129695=CARTESIAN_POINT('Ctrl Pts',(-21.0353501151795,14.1786614290351,
130.051020270923)) ;
#129696=CARTESIAN_POINT('Ctrl Pts',(-20.9910103803622,13.9181922877867,
129.888536140965)) ;
#129697=CARTESIAN_POINT('Ctrl Pts',(-20.9707895546845,13.6189924395308,
129.796111778833)) ;
#129698=CARTESIAN_POINT('Ctrl Pts',(-20.9774051303695,13.3089362850498,
129.782452006343)) ;
#129699=CARTESIAN_POINT('Ctrl Pts',(-21.0107344731984,13.0058326835249,
129.846693977316)) ;
#129700=CARTESIAN_POINT('Ctrl Pts',(-21.069523134724,12.7318653591864,129.985217546622)) ;
#129701=CARTESIAN_POINT('Ctrl Pts',(-21.150025441934,12.5082427552374,130.1872332646)) ;
#129702=CARTESIAN_POINT('Ctrl Pts',(-21.2465051340931,12.3508733005898,
130.436144552975)) ;
#129703=CARTESIAN_POINT('Ctrl Pts',(-21.3542476171135,12.269103663372,130.717689338765)) ;
#129704=CARTESIAN_POINT('Ctrl Pts',(-21.4650677342557,12.2702137118359,
131.008368653473)) ;
#129705=CARTESIAN_POINT('Ctrl Pts',(-21.5727573438248,12.3542929443511,
131.289715826593)) ;
#129706=CARTESIAN_POINT('Ctrl Pts',(-21.669031736396,12.5141175803543,131.537958518578)) ;
#129707=CARTESIAN_POINT('Ctrl Pts',(-21.7489177217398,12.7395233280602,
131.738178017608)) ;
#129708=CARTESIAN_POINT('Ctrl Pts',(-21.8069012464984,13.0142278391015,
131.87440155685)) ;
#129709=CARTESIAN_POINT('Ctrl Pts',(-21.8395149250998,13.3177661715459,
131.936564544412)) ;
#129710=CARTESIAN_POINT('Ctrl Pts',(-21.8452824715449,13.6286636556953,
131.920321738813)) ;
#129711=CARTESIAN_POINT('Ctrl Pts',(-21.8244882197182,13.925291797829,131.826438201563)) ;
#129712=CARTESIAN_POINT('Ctrl Pts',(-21.7792414631911,14.1860949206715,
131.661093526473)) ;
#129713=CARTESIAN_POINT('Ctrl Pts',(-21.7137062627427,14.3917323897328,
131.436549030154)) ;
#129714=CARTESIAN_POINT('Ctrl Pts',(-21.633156096691,14.5282787292637,131.168110047203)) ;
#129715=CARTESIAN_POINT('Ctrl Pts',(-21.5439567054312,14.5855538686264,
130.874346913366)) ;
#129716=CARTESIAN_POINT('Ctrl Pts',(-21.4537797537119,14.5594424276329,
130.57786442623)) ;
#129717=CARTESIAN_POINT('Ctrl Pts',(-21.3693530406536,14.4525338463175,
130.298172317477)) ;
#129718=CARTESIAN_POINT('Ctrl Pts',(-21.297068085247,14.2704302035547,130.053714472127)) ;
#129719=CARTESIAN_POINT('Ctrl Pts',(-21.2438867525861,14.0294404893197,
129.865368122404)) ;
#129720=CARTESIAN_POINT('Ctrl Pts',(-21.2134075430614,13.7439522566763,
129.743168596482)) ;
#129721=CARTESIAN_POINT('Ctrl Pts',(-21.2090247258927,13.4354033012877,
129.697210582902)) ;
#129722=CARTESIAN_POINT('Ctrl Pts',(-21.231516856981,13.1268757860435,129.729861443556)) ;
#129723=CARTESIAN_POINT('Ctrl Pts',(-21.2803840223732,12.8380942311381,
129.839381945022)) ;
#129724=CARTESIAN_POINT('Ctrl Pts',(-21.3521470268813,12.593020734814,130.016027287416)) ;
#129725=CARTESIAN_POINT('Ctrl Pts',(-21.4432776558791,12.406038864334,130.249044156356)) ;
#129726=CARTESIAN_POINT('Ctrl Pts',(-21.5470627584207,12.2925312393263,
130.519197721252)) ;
#129727=CARTESIAN_POINT('Ctrl Pts',(-21.6581297703892,12.2597001756507,
130.810350160136)) ;
#129728=CARTESIAN_POINT('Ctrl Pts',(-21.7675384937541,12.3104428480306,
131.096926129953)) ;
#129729=CARTESIAN_POINT('Ctrl Pts',(-21.8694603895899,12.4411375343228,
131.361483890895)) ;
#129730=CARTESIAN_POINT('Ctrl Pts',(-21.9564206697515,12.6410412260459,
131.582529425716)) ;
#129731=CARTESIAN_POINT('Ctrl Pts',(-22.0240617398326,12.8990709412412,
131.746830040607)) ;
#129732=CARTESIAN_POINT('Ctrl Pts',(-22.0670949130516,13.1932158422951,
131.839455119408)) ;
#129733=CARTESIAN_POINT('Ctrl Pts',(-22.083767292589,13.5039483153196,131.855045190033)) ;
#129734=CARTESIAN_POINT('Ctrl Pts',(-22.073536721884,13.8084629331276,131.792095553188)) ;
#129735=CARTESIAN_POINT('Ctrl Pts',(-22.0379189931258,14.0856214522983,
131.654965961301)) ;
#129736=CARTESIAN_POINT('Ctrl Pts',(-21.9800713891494,14.3156973723363,
131.452856515095)) ;
#129737=CARTESIAN_POINT('Ctrl Pts',(-21.9047961256862,14.4820692516826,
131.199796234368)) ;
#129738=CARTESIAN_POINT('Ctrl Pts',(-21.8181774390092,14.5722583226928,
130.913562740899)) ;
#129739=CARTESIAN_POINT('Ctrl Pts',(-21.7278611027354,14.5801737014987,
130.616744267121)) ;
#129740=CARTESIAN_POINT('Ctrl Pts',(-21.6397157180103,14.5050114292979,
130.325985083812)) ;
#129741=CARTESIAN_POINT('Ctrl Pts',(-21.5619498046495,14.3522166044366,
130.065688507051)) ;
#129742=CARTESIAN_POINT('Ctrl Pts',(-21.5006045705158,14.1339604328417,
129.853478179641)) ;
#129743=CARTESIAN_POINT('Ctrl Pts',(-21.4603340437159,13.8641114718027,
129.702710340301)) ;
#129744=CARTESIAN_POINT('Ctrl Pts',(-21.4451043217958,13.5616227135085,
129.624990432218)) ;
#129745=CARTESIAN_POINT('Ctrl Pts',(-21.4567589247854,13.2502936297686,
129.625929497814)) ;
#129746=CARTESIAN_POINT('Ctrl Pts',(-21.4951599834877,12.9509784394827,
129.704955381254)) ;
#129747=CARTESIAN_POINT('Ctrl Pts',(-21.5580080093365,12.6863950306147,
129.855517297843)) ;
#129748=CARTESIAN_POINT('Ctrl Pts',(-21.6420011592254,12.4734607184327,
130.067712328711)) ;
#129749=CARTESIAN_POINT('Ctrl Pts',(-21.7417791407559,12.3287824290801,
130.325991712342)) ;
#129750=CARTESIAN_POINT('Ctrl Pts',(-21.8504049263474,12.2629634188969,
130.610230387682)) ;
#129751=CARTESIAN_POINT('Ctrl Pts',(-21.9610518581756,12.2798963089147,
130.900404347138)) ;
#129752=CARTESIAN_POINT('Ctrl Pts',(-22.0669959746994,12.3786943596861,
131.176740574865)) ;
#129753=CARTESIAN_POINT('Ctrl Pts',(-22.1611710364992,12.5532636786749,
131.418606895266)) ;
#129754=CARTESIAN_POINT('Ctrl Pts',(-22.2366635856223,12.7879391419199,
131.606219865345)) ;
#129755=CARTESIAN_POINT('Ctrl Pts',(-22.290142211429,13.0695370930121,131.729290328247)) ;
#129756=CARTESIAN_POINT('Ctrl Pts',(-22.3178130052509,13.3764286772832,
131.776992915573)) ;
#129757=CARTESIAN_POINT('Ctrl Pts',(-22.318427864876,13.6873693589622,131.745572982122)) ;
#129758=CARTESIAN_POINT('Ctrl Pts',(-22.292826577029,13.9780097335569,131.637733892545)) ;
#129759=CARTESIAN_POINT('Ctrl Pts',(-22.2431790354703,14.2303816852456,
131.459436217296)) ;
#129760=CARTESIAN_POINT('Ctrl Pts',(-22.1746653892291,14.4229832269157,
131.226347148492)) ;
#129761=CARTESIAN_POINT('Ctrl Pts',(-22.0916752545479,14.5456071990929,
130.950650854282)) ;
#129762=CARTESIAN_POINT('Ctrl Pts',(-22.0020115166837,14.5869244372619,
130.655664977446)) ;
#129763=CARTESIAN_POINT('Ctrl Pts',(-21.9122878651958,14.545413997822,130.360474615968)) ;
#129764=CARTESIAN_POINT('Ctrl Pts',(-21.8295294436028,14.4231615321001,
130.085553182396)) ;
#129765=CARTESIAN_POINT('Ctrl Pts',(-21.7608250583823,14.2299646068936,
129.85180667101)) ;
#129766=CARTESIAN_POINT('Ctrl Pts',(-21.7113239372725,13.9782380541428,
129.674030463916)) ;
#129767=CARTESIAN_POINT('Ctrl Pts',(-21.6856792409941,13.6869897055948,
129.565991871631)) ;
#129768=CARTESIAN_POINT('Ctrl Pts',(-21.6862854845015,13.3772462796711,
129.534677574901)) ;
#129769=CARTESIAN_POINT('Ctrl Pts',(-21.7138953989796,13.0701027009942,
129.582174987858)) ;
#129770=CARTESIAN_POINT('Ctrl Pts',(-21.7673001378337,12.7883758458207,
129.705033082138)) ;
#129771=CARTESIAN_POINT('Ctrl Pts',(-21.8432513830499,12.5524788761833,
129.893799085058)) ;
#129772=CARTESIAN_POINT('Ctrl Pts',(-21.9371566394696,12.3787206471269,
130.134993378243)) ;
#129773=CARTESIAN_POINT('Ctrl Pts',(-22.0430755659619,12.2799428632339,
130.41125725332)) ;
#129774=CARTESIAN_POINT('Ctrl Pts',(-22.1535702808427,12.262781436098,130.701037365043)) ;
#129775=CARTESIAN_POINT('Ctrl Pts',(-22.2630782526847,12.3295043869385,
130.987573569498)) ;
#129776=CARTESIAN_POINT('Ctrl Pts',(-22.362016039896,12.473510372606,131.243655905125)) ;
#129777=CARTESIAN_POINT('Ctrl Pts',(-22.4459844694034,12.6859034724392,
131.455815775636)) ;
#129778=CARTESIAN_POINT('Ctrl Pts',(-22.5090028960007,12.9511126916242,
131.606796748372)) ;
#129779=CARTESIAN_POINT('Ctrl Pts',(-22.54743070579,13.2510040815984,131.685842769885)) ;
#129780=CARTESIAN_POINT('Ctrl Pts',(-22.558981890815,13.5624346911567,131.686468142538)) ;
#129781=CARTESIAN_POINT('Ctrl Pts',(-22.5438100294484,13.863434989198,131.609077935155)) ;
#129782=CARTESIAN_POINT('Ctrl Pts',(-22.5036818951076,14.1332612598468,
131.45875046159)) ;
#129783=CARTESIAN_POINT('Ctrl Pts',(-22.4420921893319,14.3526408923895,
131.245680127562)) ;
#129784=CARTESIAN_POINT('Ctrl Pts',(-22.3640058771557,14.5054039149979,
130.984345418318)) ;
#129785=CARTESIAN_POINT('Ctrl Pts',(-22.2766140050104,14.5799567514586,
130.696072024306)) ;
#129786=CARTESIAN_POINT('Ctrl Pts',(-22.1858591503502,14.5723714395277,
130.397811110958)) ;
#129787=CARTESIAN_POINT('Ctrl Pts',(-22.0992395687441,14.4818104958985,
130.111564075611)) ;
#129788=CARTESIAN_POINT('Ctrl Pts',(-22.024274176973,14.3163443663444,129.859558431675)) ;
#129789=CARTESIAN_POINT('Ctrl Pts',(-21.9662417141904,14.0859121454152,
129.656831575018)) ;
#129790=CARTESIAN_POINT('Ctrl Pts',(-21.9305828051363,13.8088759018265,
129.519593613112)) ;
#129791=CARTESIAN_POINT('Ctrl Pts',(-21.9203578742062,13.5028416968273,
129.456494956462)) ;
#129792=CARTESIAN_POINT('Ctrl Pts',(-21.9370262576808,13.1931031843273,
129.472184440752)) ;
#129793=CARTESIAN_POINT('Ctrl Pts',(-21.9802902593002,12.89795929161,129.565356630037)) ;
#129794=CARTESIAN_POINT('Ctrl Pts',(-22.047553588434,12.6415807135438,129.728760415045)) ;
#129795=CARTESIAN_POINT('Ctrl Pts',(-22.1347436150936,12.4408172344946,
129.950365899039)) ;
#129796=CARTESIAN_POINT('Ctrl Pts',(-22.2370229130925,12.3100401659206,
130.215871813637)) ;
#129797=CARTESIAN_POINT('Ctrl Pts',(-22.346187343475,12.2598615754433,130.501810053951)) ;
#129798=CARTESIAN_POINT('Ctrl Pts',(-22.4566401515678,12.2922205414055,
130.791357288347)) ;
#129799=CARTESIAN_POINT('Ctrl Pts',(-22.5610110970781,12.4062484922091,
131.063036431062)) ;
#129800=CARTESIAN_POINT('Ctrl Pts',(-22.6518356473151,12.5927140655513,
131.295269732808)) ;
#129801=CARTESIAN_POINT('Ctrl Pts',(-22.7237313097823,12.8381489007341,
131.472242088444)) ;
#129802=CARTESIAN_POINT('Ctrl Pts',(-22.7725207924835,13.1260095421298,
131.581638130057)) ;
#129803=CARTESIAN_POINT('Ctrl Pts',(-22.7951559321079,13.4367097246031,
131.614472327231)) ;
#129804=CARTESIAN_POINT('Ctrl Pts',(-22.7906542710234,13.7438376703634,
131.56831388168)) ;
#129805=CARTESIAN_POINT('Ctrl Pts',(-22.7603725677891,14.0287736404421,
131.44677384493)) ;
#129806=CARTESIAN_POINT('Ctrl Pts',(-22.7068886331561,14.270962157525,131.257369646946)) ;
#129807=CARTESIAN_POINT('Ctrl Pts',(-22.6349661679253,14.4520607782582,
131.014146425895)) ;
#129808=CARTESIAN_POINT('Ctrl Pts',(-22.5504033640329,14.5594794315335,
130.733986591008)) ;
#129809=CARTESIAN_POINT('Ctrl Pts',(-22.4601541297996,14.5855261775524,
130.437269710365)) ;
#129810=CARTESIAN_POINT('Ctrl Pts',(-22.3710288767078,14.5283738977508,
130.14375232629)) ;
#129811=CARTESIAN_POINT('Ctrl Pts',(-22.2903791078735,14.391653675229,129.874980130826)) ;
#129812=CARTESIAN_POINT('Ctrl Pts',(-22.2249495985923,14.1863633924956,
129.650800118023)) ;
#129813=CARTESIAN_POINT('Ctrl Pts',(-22.1796679930113,13.9255969369485,
129.48534839629)) ;
#129814=CARTESIAN_POINT('Ctrl Pts',(-22.1588481354936,13.6292801899933,
129.391421087479)) ;
#129815=CARTESIAN_POINT('Ctrl Pts',(-22.1645772032321,13.3179690921283,
129.375020864213)) ;
#129816=CARTESIAN_POINT('Ctrl Pts',(-22.1971947872982,13.0144329999001,
129.437196033629)) ;
#129817=CARTESIAN_POINT('Ctrl Pts',(-22.2550420413868,12.7401668642732,
129.573078522351)) ;
#129818=CARTESIAN_POINT('Ctrl Pts',(-22.3348838189612,12.5144107984142,
129.773156275244)) ;
#129819=CARTESIAN_POINT('Ctrl Pts',(-22.4315850270881,12.3540785091182,
130.022507063406)) ;
#129820=CARTESIAN_POINT('Ctrl Pts',(-22.5386180179821,12.2704506972946,
130.302139542132)) ;
#129821=CARTESIAN_POINT('Ctrl Pts',(-22.6497921880934,12.2689820751512,
130.593744024713)) ;
#129822=CARTESIAN_POINT('Ctrl Pts',(-22.7576074186186,12.3508509067205,
130.875481503016)) ;
#129823=CARTESIAN_POINT('Ctrl Pts',(-22.8543111531987,12.5086054650755,
131.124969484035)) ;
#129824=CARTESIAN_POINT('Ctrl Pts',(-22.9349375950158,12.7330676157862,
131.327264167781)) ;
#129825=CARTESIAN_POINT('Ctrl Pts',(-22.9934475007787,13.0066123030749,
131.465048783301)) ;
#129826=CARTESIAN_POINT('Ctrl Pts',(-23.0266870652074,13.3082724111724,
131.529183861315)) ;
#129827=CARTESIAN_POINT('Ctrl Pts',(-23.033311559833,13.6201711563921,131.515348886077)) ;
#129828=CARTESIAN_POINT('Ctrl Pts',(-23.0130972666971,13.9183339563094,
131.423061499097)) ;
#129829=CARTESIAN_POINT('Ctrl Pts',(-22.9684886216917,14.1797387152336,
131.259643342506)) ;
#129830=CARTESIAN_POINT('Ctrl Pts',(-22.9036845336627,14.3864986617501,
131.037342151647)) ;
#129831=CARTESIAN_POINT('Ctrl Pts',(-22.8235293433254,14.5252641386946,
130.77006712631)) ;
#129832=CARTESIAN_POINT('Ctrl Pts',(-22.7344573025139,14.5851720998815,
130.476667796814)) ;
#129833=CARTESIAN_POINT('Ctrl Pts',(-22.6437076364381,14.561066934574,130.178322236931)) ;
#129834=CARTESIAN_POINT('Ctrl Pts',(-22.5595163505151,14.4566510125324,
129.899496693664)) ;
#129835=CARTESIAN_POINT('Ctrl Pts',(-22.4868075776867,14.2771545547794,
129.653851802256)) ;
#129836=CARTESIAN_POINT('Ctrl Pts',(-22.4327702184639,14.0362065593723,
129.462817295921)) ;
#129837=CARTESIAN_POINT('Ctrl Pts',(-22.4017946730085,13.7533987365905,
129.339371688466)) ;
#129838=CARTESIAN_POINT('Ctrl Pts',(-22.3965076931407,13.444128366597,129.290651049899)) ;
#129839=CARTESIAN_POINT('Ctrl Pts',(-22.4184444031792,13.1346408962195,
129.321598554928)) ;
#129840=CARTESIAN_POINT('Ctrl Pts',(-22.4661569344923,12.8470251691959,
129.427998466394)) ;
#129841=CARTESIAN_POINT('Ctrl Pts',(-22.5378591493393,12.5984937822196,
129.604197721476)) ;
#129842=CARTESIAN_POINT('Ctrl Pts',(-22.6280348584897,12.4108688263379,
129.834624782045)) ;
#129843=CARTESIAN_POINT('Ctrl Pts',(-22.7317416641835,12.2946081111199,
130.104467076645)) ;
#129844=CARTESIAN_POINT('Ctrl Pts',(-22.8428132954771,12.2594450542174,
130.395612682579)) ;
#129845=CARTESIAN_POINT('Ctrl Pts',(-22.9524265076277,12.3080481401079,
130.682755174456)) ;
#129846=CARTESIAN_POINT('Ctrl Pts',(-23.0543320583707,12.4360760785603,
130.9473801658)) ;
#129847=CARTESIAN_POINT('Ctrl Pts',(-23.1419844807782,12.6345257825012,
131.170374346328)) ;
#129848=CARTESIAN_POINT('Ctrl Pts',(-23.2100400384086,12.8902136369556,
131.336008542892)) ;
#129849=CARTESIAN_POINT('Ctrl Pts',(-23.2539371077913,13.1836914556234,
131.431128041516)) ;
#129850=CARTESIAN_POINT('Ctrl Pts',(-23.2714654817158,13.4943233171344,
131.449212934784)) ;
#129851=CARTESIAN_POINT('Ctrl Pts',(-23.2619647848818,13.800844370543,131.388233267397)) ;
#129852=CARTESIAN_POINT('Ctrl Pts',(-23.2268232132927,14.0793169381169,
131.25243650753)) ;
#129853=CARTESIAN_POINT('Ctrl Pts',(-23.1698063741231,14.3098744283553,
131.052912529895)) ;
#129854=CARTESIAN_POINT('Ctrl Pts',(-23.0946065002962,14.4788323999099,
130.799928901127)) ;
#129855=CARTESIAN_POINT('Ctrl Pts',(-23.0086310860279,14.5706779805767,
130.51574571968)) ;
#129856=CARTESIAN_POINT('Ctrl Pts',(-22.9181540035114,14.5811216751553,
130.218385768939)) ;
#129857=CARTESIAN_POINT('Ctrl Pts',(-22.8299926049286,14.5082992229446,
129.927641015252)) ;
#129858=CARTESIAN_POINT('Ctrl Pts',(-22.7518958692624,14.3580059118444,
129.666415005834)) ;
#129859=CARTESIAN_POINT('Ctrl Pts',(-22.68973964975,14.1405258591395,129.451695647597)) ;
#129860=CARTESIAN_POINT('Ctrl Pts',(-22.6489474985288,13.8719963111484,
129.299439068749)) ;
#129861=CARTESIAN_POINT('Ctrl Pts',(-22.6329623427693,13.5716291757303,
129.219672143091)) ;
#129862=CARTESIAN_POINT('Ctrl Pts',(-22.6438299307625,13.2591264952113,
129.218186867551)) ;
#129863=CARTESIAN_POINT('Ctrl Pts',(-22.6813595982475,12.9599152981085,
129.294758434884)) ;
#129864=CARTESIAN_POINT('Ctrl Pts',(-22.7437268703939,12.6930802012435,
129.44379758794)) ;
#129865=CARTESIAN_POINT('Ctrl Pts',(-22.8271153369779,12.4788238742032,
129.654272485267)) ;
#129866=CARTESIAN_POINT('Ctrl Pts',(-22.9262087039054,12.3322479611375,
129.910645691407)) ;
#129867=CARTESIAN_POINT('Ctrl Pts',(-23.0347908804482,12.2636849703181,
130.194712650591)) ;
#129868=CARTESIAN_POINT('Ctrl Pts',(-23.1457780726912,12.2782423508481,
130.485793595157)) ;
#129869=CARTESIAN_POINT('Ctrl Pts',(-23.2518521138872,12.3748788138008,
130.762534585018)) ;
#129870=CARTESIAN_POINT('Ctrl Pts',(-23.3461191357027,12.5463734301239,
131.004816306225)) ;
#129871=CARTESIAN_POINT('Ctrl Pts',(-23.4227572575714,12.7810696053441,
131.195540562452)) ;
#129872=CARTESIAN_POINT('Ctrl Pts',(-23.4766900181559,13.0608632810621,
131.320045830173)) ;
#129873=CARTESIAN_POINT('Ctrl Pts',(-23.5051675153737,13.3671882377426,
131.37011185604)) ;
#129874=CARTESIAN_POINT('Ctrl Pts',(-23.5065949253369,13.6783220595412,
131.341073633408)) ;
#129875=CARTESIAN_POINT('Ctrl Pts',(-23.4816682311954,13.9701100472944,
131.235162424807)) ;
#129876=CARTESIAN_POINT('Ctrl Pts',(-23.4329222288376,14.2230345165602,
131.059637422382)) ;
#129877=CARTESIAN_POINT('Ctrl Pts',(-23.3645416427281,14.4186168854027,
130.826753646501)) ;
#129878=CARTESIAN_POINT('Ctrl Pts',(-23.2822390982612,14.5428705868712,
130.553224844874)) ;
#129879=CARTESIAN_POINT('Ctrl Pts',(-23.192506581194,14.5869069851008,130.257961717535)) ;
#129880=CARTESIAN_POINT('Ctrl Pts',(-23.1027575317741,14.5480013167689,
129.962735045499)) ;
#129881=CARTESIAN_POINT('Ctrl Pts',(-23.0192260399974,14.4271740757264,
129.685359875558)) ;
#129882=CARTESIAN_POINT('Ctrl Pts',(-22.9503502410774,14.2362638789622,
129.451230370321)) ;
#129883=CARTESIAN_POINT('Ctrl Pts',(-22.9002301505869,13.9863048422078,
129.271676603921)) ;
#129884=CARTESIAN_POINT('Ctrl Pts',(-22.8738614058396,13.6957298315302,
129.161501741172)) ;
#129885=CARTESIAN_POINT('Ctrl Pts',(-22.8736157044307,13.3866515918627,
129.127747431502)) ;
#129886=CARTESIAN_POINT('Ctrl Pts',(-22.9007309903636,13.0771469983457,
129.173578973472)) ;
#129887=CARTESIAN_POINT('Ctrl Pts',(-22.9531241560762,12.7963921312271,
129.29371262047)) ;
#129888=CARTESIAN_POINT('Ctrl Pts',(-23.0287907307986,12.5578779663261,
129.481500335553)) ;
#129889=CARTESIAN_POINT('Ctrl Pts',(-23.1219014006858,12.3830735911952,
129.720516205546)) ;
#129890=CARTESIAN_POINT('Ctrl Pts',(-23.2275724461705,12.2815115328469,
129.99604251459)) ;
#129891=CARTESIAN_POINT('Ctrl Pts',(-23.3388191343614,12.2623682351307,
130.287780389931)) ;
#129892=CARTESIAN_POINT('Ctrl Pts',(-23.4471188624795,12.3259183972767,
130.571207242919)) ;
#129893=CARTESIAN_POINT('Ctrl Pts',(-23.5471374646567,12.4680808771893,
130.830236267802)) ;
#129894=CARTESIAN_POINT('Ctrl Pts',(-23.6317831266168,12.6795622431896,
131.04428925764)) ;
#129895=CARTESIAN_POINT('Ctrl Pts',(-23.6952246631273,12.942589382418,131.196621763478)) ;
#129896=CARTESIAN_POINT('Ctrl Pts',(-23.7344524554603,13.2417281941733,
131.278005106931)) ;
#129897=CARTESIAN_POINT('Ctrl Pts',(-23.7468298790603,13.5531901597367,
131.281039111896)) ;
#129898=CARTESIAN_POINT('Ctrl Pts',(-23.7323614802831,13.8554127215433,
131.205630116186)) ;
#129899=CARTESIAN_POINT('Ctrl Pts',(-23.6929669829259,14.1261607802399,
131.05748848122)) ;
#129900=CARTESIAN_POINT('Ctrl Pts',(-23.631618534262,14.3478084011447,130.844991831341)) ;
#129901=CARTESIAN_POINT('Ctrl Pts',(-23.5546595857602,14.5013886239399,
130.587262450918)) ;
#129902=CARTESIAN_POINT('Ctrl Pts',(-23.4667489844287,14.5792262889595,
130.29719183709)) ;
#129903=CARTESIAN_POINT('Ctrl Pts',(-23.3761695508235,14.5735423486693,
129.999514469588)) ;
#129904=CARTESIAN_POINT('Ctrl Pts',(-23.289558304496,14.4859392632534,129.71339602831)) ;
#129905=CARTESIAN_POINT('Ctrl Pts',(-23.2136588166763,14.3210240501096,
129.458405866252)) ;
#129906=CARTESIAN_POINT('Ctrl Pts',(-23.1555173074775,14.0938130208259,
129.2556140445)) ;
#129907=CARTESIAN_POINT('Ctrl Pts',(-23.118997631847,13.8165580564643,129.115691388806)) ;
#129908=CARTESIAN_POINT('Ctrl Pts',(-23.1080276758516,13.5127265390552,
129.050612193546)) ;
#129909=CARTESIAN_POINT('Ctrl Pts',(-23.1241410108863,13.2000972464797,
129.064374981949)) ;
#129910=CARTESIAN_POINT('Ctrl Pts',(-23.1662601446052,12.9073427660881,
129.154562570437)) ;
#129911=CARTESIAN_POINT('Ctrl Pts',(-23.2331580385046,12.6479572947944,
129.316703386966)) ;
#129912=CARTESIAN_POINT('Ctrl Pts',(-23.3195943837913,12.4461100602533,
129.53621950267)) ;
#129913=CARTESIAN_POINT('Ctrl Pts',(-23.4215936463265,12.3127706355445,
129.800873866609)) ;
#129914=CARTESIAN_POINT('Ctrl Pts',(-23.530741294766,12.2601401093184,130.086732236641)) ;
#129915=CARTESIAN_POINT('Ctrl Pts',(-23.641295933381,12.2901733170219,130.37656641642)) ;
#129916=CARTESIAN_POINT('Ctrl Pts',(-23.7457667500472,12.4015832972313,
130.648604057112)) ;
#129917=CARTESIAN_POINT('Ctrl Pts',(-23.837320922193,12.5866483743453,130.882868179984)) ;
#129918=CARTESIAN_POINT('Ctrl Pts',(-23.9097809110176,12.8302723297284,
131.061533181026)) ;
#129919=CARTESIAN_POINT('Ctrl Pts',(-23.9594436984039,13.1192440323379,
131.17325973788)) ;
#129920=CARTESIAN_POINT('Ctrl Pts',(-23.9825588767331,13.4254781979924,
131.207947994022)) ;
#129921=CARTESIAN_POINT('Ctrl Pts',(-23.9789923334788,13.735359683146,131.164262668825)) ;
#129922=CARTESIAN_POINT('Ctrl Pts',(-23.9493638176101,14.0210481955409,
131.044652952135)) ;
#129923=CARTESIAN_POINT('Ctrl Pts',(-23.8964348750507,14.2649914593589,
130.856831392013)) ;
#129924=CARTESIAN_POINT('Ctrl Pts',(-23.8250858891093,14.4476746883627,
130.615345568459)) ;
#129925=CARTESIAN_POINT('Ctrl Pts',(-23.7408346035683,14.5574099930499,
130.3361027737)) ;
#129926=CARTESIAN_POINT('Ctrl Pts',(-23.6506254186035,14.5860647522522,
130.039495997294)) ;
#129927=CARTESIAN_POINT('Ctrl Pts',(-23.5609942892391,14.5307819491484,
129.744354946213)) ;
#129928=CARTESIAN_POINT('Ctrl Pts',(-23.4804650219021,14.3969445600344,
129.476125426802)) ;
#129929=CARTESIAN_POINT('Ctrl Pts',(-23.4142527293967,14.1927449819674,
129.249526011617)) ;
#129930=CARTESIAN_POINT('Ctrl Pts',(-23.3684848120887,13.9340125126876,
129.082756157156)) ;
#129931=CARTESIAN_POINT('Ctrl Pts',(-23.3468587978125,13.6381122428634,
128.986428754755)) ;
#129932=CARTESIAN_POINT('Ctrl Pts',(-23.3518116052348,13.3270743882958,
128.967779729988)) ;
#129933=CARTESIAN_POINT('Ctrl Pts',(-23.3836997037052,13.022510775008,129.027771986449)) ;
#129934=CARTESIAN_POINT('Ctrl Pts',(-23.4410446186167,12.7468021187138,
129.162131040852)) ;
#129935=CARTESIAN_POINT('Ctrl Pts',(-23.5199252416539,12.5205888533643,
129.359570203463)) ;
#129936=CARTESIAN_POINT('Ctrl Pts',(-23.6162103718271,12.3578210122937,
129.607688028642)) ;
#129937=CARTESIAN_POINT('Ctrl Pts',(-23.7233238649532,12.2716455027741,
129.887467974327)) ;
#129938=CARTESIAN_POINT('Ctrl Pts',(-23.8343750091978,12.2679542835663,
130.178745490843)) ;
#129939=CARTESIAN_POINT('Ctrl Pts',(-23.9420352985659,12.3469221374096,
130.460148975221)) ;
#129940=CARTESIAN_POINT('Ctrl Pts',(-24.0395306000166,12.5030897490068,
130.71181941671)) ;
#129941=CARTESIAN_POINT('Ctrl Pts',(-24.1204139007615,12.7250181142628,
130.914990286498)) ;
#129942=CARTESIAN_POINT('Ctrl Pts',(-24.1797612052318,12.997182712002,131.055216258735)) ;
#129943=CARTESIAN_POINT('Ctrl Pts',(-24.2139296280654,13.2997827331154,
131.121902223964)) ;
#129944=CARTESIAN_POINT('Ctrl Pts',(-24.2212467345928,13.6108909290664,
131.110180839414)) ;
#129945=CARTESIAN_POINT('Ctrl Pts',(-24.2019836667752,13.9087322628313,
131.020799333689)) ;
#129946=CARTESIAN_POINT('Ctrl Pts',(-24.1579858554531,14.1725575472539,
130.859051286282)) ;
#129947=CARTESIAN_POINT('Ctrl Pts',(-24.093541705692,14.3815587405522,130.637727194554)) ;
#129948=CARTESIAN_POINT('Ctrl Pts',(-24.0137360577577,14.5223295633007,
130.371479426055)) ;
#129949=CARTESIAN_POINT('Ctrl Pts',(-23.9250824711545,14.5844939623778,
130.079398354997)) ;
#129950=CARTESIAN_POINT('Ctrl Pts',(-23.8342900042102,14.5631534424975,
129.780935135738)) ;
#129951=CARTESIAN_POINT('Ctrl Pts',(-23.7494814898801,14.4606751322893,
129.500175677992)) ;
#129952=CARTESIAN_POINT('Ctrl Pts',(-23.6763381643652,14.2826954398612,
129.253230600252)) ;
#129953=CARTESIAN_POINT('Ctrl Pts',(-23.6219494390935,14.0447463788915,
129.061356272604)) ;
#129954=CARTESIAN_POINT('Ctrl Pts',(-23.5900786851126,13.7613771395104,
128.935107708196)) ;
#129955=CARTESIAN_POINT('Ctrl Pts',(-23.5840797714012,13.4542323467487,
128.884499268984)) ;
#129956=CARTESIAN_POINT('Ctrl Pts',(-23.6051135424781,13.1437994705374,
128.91274207276)) ;
#129957=CARTESIAN_POINT('Ctrl Pts',(-23.6524480707265,12.8538469195634,
129.017861949348)) ;
#129958=CARTESIAN_POINT('Ctrl Pts',(-23.7231470461455,12.6054873461084,
129.191328878648)) ;
#129959=CARTESIAN_POINT('Ctrl Pts',(-23.812834818571,12.4153273171675,129.420299880366)) ;
#129960=CARTESIAN_POINT('Ctrl Pts',(-23.9171324935436,12.2964112453651,
129.691604194727)) ;
#129961=CARTESIAN_POINT('Ctrl Pts',(-24.0268994581797,12.2594155907016,
129.979307926472)) ;
#129962=CARTESIAN_POINT('Ctrl Pts',(-24.1370680092537,12.3053349417689,
130.267942075581)) ;
#129963=CARTESIAN_POINT('Ctrl Pts',(-24.2392677005312,12.4312258982637,
130.533435968365)) ;
#129964=CARTESIAN_POINT('Ctrl Pts',(-24.3275283859303,12.627959699626,130.758169851058)) ;
#129965=CARTESIAN_POINT('Ctrl Pts',(-24.3962310838253,12.8824932642082,
130.925674503715)) ;
#129966=CARTESIAN_POINT('Ctrl Pts',(-24.4407733223245,13.1745455141317,
131.022746419222)) ;
#129967=CARTESIAN_POINT('Ctrl Pts',(-24.4591380272995,13.4851755332174,
131.043255013574)) ;
#129968=CARTESIAN_POINT('Ctrl Pts',(-24.4503750207915,13.7921378916297,
130.984426733776)) ;
#129969=CARTESIAN_POINT('Ctrl Pts',(-24.4161419214947,14.0710147358115,
130.851388646496)) ;
#129970=CARTESIAN_POINT('Ctrl Pts',(-24.3593113729837,14.3045451630866,
130.65219208029)) ;
#129971=CARTESIAN_POINT('Ctrl Pts',(-24.2852488197019,14.4740865668841,
130.402844051698)) ;
#129972=CARTESIAN_POINT('Ctrl Pts',(-24.1989871899202,14.5693022255178,
130.11759849223)) ;
#129973=CARTESIAN_POINT('Ctrl Pts',(-24.1085533561024,14.5820126404232,
129.820380804925)) ;
#129974=CARTESIAN_POINT('Ctrl Pts',(-24.0199963670256,14.511227148385,129.528389522944)) ;
#129975=CARTESIAN_POINT('Ctrl Pts',(-23.9418631026754,14.3635592095882,
129.267195284118)) ;
#129976=CARTESIAN_POINT('Ctrl Pts',(-23.8791136578675,14.1479540457657,
129.05073670007)) ;
#129977=CARTESIAN_POINT('Ctrl Pts',(-23.8375873211756,13.8806548150988,
128.896328674777)) ;
#129978=CARTESIAN_POINT('Ctrl Pts',(-23.8208085079993,13.5796274976099,
128.814103347584)) ;
#129979=CARTESIAN_POINT('Ctrl Pts',(-23.8309910040008,13.2675903207149,
128.810667211912)) ;
#129980=CARTESIAN_POINT('Ctrl Pts',(-23.8676460753912,12.9685393954342,
128.884773865646)) ;
#129981=CARTESIAN_POINT('Ctrl Pts',(-23.9293823518697,12.7001828412868,
129.031937184548)) ;
#129982=CARTESIAN_POINT('Ctrl Pts',(-24.0121193234782,12.484351447388,129.240548101327)) ;
#129983=CARTESIAN_POINT('Ctrl Pts',(-24.1109979057002,12.3354378229303,
129.496238790614)) ;
#129984=CARTESIAN_POINT('Ctrl Pts',(-24.2190824025548,12.2645466644513,
129.778950581268)) ;
#129985=CARTESIAN_POINT('Ctrl Pts',(-24.330609557235,12.2767400310682,130.071453555101)) ;
#129986=CARTESIAN_POINT('Ctrl Pts',(-24.4365405624164,12.3708038596253,
130.347899012378)) ;
#129987=CARTESIAN_POINT('Ctrl Pts',(-24.5314328322576,12.5405713719576,
130.591935712668)) ;
#129988=CARTESIAN_POINT('Ctrl Pts',(-24.6084325711965,12.7727635932404,
130.783833850884)) ;
#129989=CARTESIAN_POINT('Ctrl Pts',(-24.6634600795244,13.0532481868504,
130.911323007965)) ;
#129990=CARTESIAN_POINT('Ctrl Pts',(-24.692522529149,13.3594503322591,130.963076041083)) ;
#129991=CARTESIAN_POINT('Ctrl Pts',(-24.6947280405791,13.6687250263673,
130.936529774944)) ;
#129992=CARTESIAN_POINT('Ctrl Pts',(-24.6705282850378,13.9622483916866,
130.832644671573)) ;
#129993=CARTESIAN_POINT('Ctrl Pts',(-24.622436218567,14.216383713817,130.659054441099)) ;
#129994=CARTESIAN_POINT('Ctrl Pts',(-24.5543668513611,14.4143549366633,
130.426992649947)) ;
#129995=CARTESIAN_POINT('Ctrl Pts',(-24.4723486974786,14.5404303817965,
130.154299491946)) ;
#129996=CARTESIAN_POINT('Ctrl Pts',(-24.3831123163456,14.5868747918771,
129.860628601173)) ;
#129997=CARTESIAN_POINT('Ctrl Pts',(-24.2927557290999,14.5499212465235,
129.56342641909)) ;
#129998=CARTESIAN_POINT('Ctrl Pts',(-24.2096290003052,14.4324626280189,
129.287528296366)) ;
#129999=CARTESIAN_POINT('Ctrl Pts',(-24.1396226803011,14.2419356925952,
129.049797964534)) ;
#130000=CARTESIAN_POINT('Ctrl Pts',(-24.0891543308482,13.9939564781135,
128.869339869159)) ;
#130001=CARTESIAN_POINT('Ctrl Pts',(-24.0620213641921,13.704318184283,128.756930260385)) ;
#130002=CARTESIAN_POINT('Ctrl Pts',(-24.0610743558635,13.3953698080797,
128.721115144032)) ;
#130003=CARTESIAN_POINT('Ctrl Pts',(-24.0872215118966,13.0868084154143,
128.764268368717)) ;
#130004=CARTESIAN_POINT('Ctrl Pts',(-24.1391372778054,12.8035341969557,
128.882834895599)) ;
#130005=CARTESIAN_POINT('Ctrl Pts',(-24.2141316302003,12.5639567807414,
129.068713539452)) ;
#130006=CARTESIAN_POINT('Ctrl Pts',(-24.3069768980926,12.3867441637874,
129.306888123521)) ;
#130007=CARTESIAN_POINT('Ctrl Pts',(-24.4126054249827,12.2832559851663,
129.582236617727)) ;
#130008=CARTESIAN_POINT('Ctrl Pts',(-24.5228382226761,12.2616345605918,
129.871302925535)) ;
#130009=CARTESIAN_POINT('Ctrl Pts',(-24.6321785231031,12.3231638536054,
130.157498310678)) ;
#130010=CARTESIAN_POINT('Ctrl Pts',(-24.7320770324703,12.4627499394219,
130.41633010543)) ;
#130011=CARTESIAN_POINT('Ctrl Pts',(-24.8175012342038,12.6729052718455,
130.632563287353)) ;
#130012=CARTESIAN_POINT('Ctrl Pts',(-24.8815266149577,12.9344259227914,
130.786639358572)) ;
#130013=CARTESIAN_POINT('Ctrl Pts',(-24.9215855419147,13.2340773776093,
130.870319237765)) ;
#130014=CARTESIAN_POINT('Ctrl Pts',(-24.9345965993483,13.5439037579597,
130.875373791953)) ;
#130015=CARTESIAN_POINT('Ctrl Pts',(-24.9209872048283,13.8465580418888,
130.802495474506)) ;
#130016=CARTESIAN_POINT('Ctrl Pts',(-24.8822354446801,14.1188038713519,
130.656193145261)) ;
#130017=CARTESIAN_POINT('Ctrl Pts',(-24.8215520611578,14.3420290100945,
130.445680053042)) ;
#130018=CARTESIAN_POINT('Ctrl Pts',(-24.7447511412938,14.4980359942342,
130.188314463308)) ;
#130019=CARTESIAN_POINT('Ctrl Pts',(-24.6574682218922,14.5780642273586,
129.900239858161)) ;
#130020=CARTESIAN_POINT('Ctrl Pts',(-24.5661704406245,14.5747644826435,
129.600201361656)) ;
#130021=CARTESIAN_POINT('Ctrl Pts',(-24.4798397107362,14.4895501610045,
129.315081720064)) ;
#130022=CARTESIAN_POINT('Ctrl Pts',(-24.4036359268958,14.3274512492284,
129.059276795445)) ;
#130023=CARTESIAN_POINT('Ctrl Pts',(-24.3446920999538,14.1012132638127,
128.854030110214)) ;
#130024=CARTESIAN_POINT('Ctrl Pts',(-24.3074730021535,13.8249845460598,
128.712057536314)) ;
#130025=CARTESIAN_POINT('Ctrl Pts',(-24.2957931040204,13.5214322498008,
128.644878171936)) ;
#130026=CARTESIAN_POINT('Ctrl Pts',(-24.3109547722312,13.2103012906498,
128.656038921471)) ;
#130027=CARTESIAN_POINT('Ctrl Pts',(-24.3525323396269,12.9148532229271,
128.744433326594)) ;
#130028=CARTESIAN_POINT('Ctrl Pts',(-24.41885720721,12.6543478093024,128.904910138534)) ;
#130029=CARTESIAN_POINT('Ctrl Pts',(-24.5046482463071,12.4511189000955,
129.122596465375)) ;
#130030=CARTESIAN_POINT('Ctrl Pts',(-24.6060741915631,12.3156705580683,
129.385644993005)) ;
#130031=CARTESIAN_POINT('Ctrl Pts',(-24.7155785502479,12.2603783302423,
129.672396480643)) ;
#130032=CARTESIAN_POINT('Ctrl Pts',(-24.8261383061215,12.2883877203707,
129.962262156073)) ;
#130033=CARTESIAN_POINT('Ctrl Pts',(-24.9304589738136,12.396958249081,130.233999385643)) ;
#130034=CARTESIAN_POINT('Ctrl Pts',(-25.022824941926,12.5805839633338,130.470521381763)) ;
#130035=CARTESIAN_POINT('Ctrl Pts',(-25.0956897007076,12.8225431186843,
130.650415821546)) ;
#130036=CARTESIAN_POINT('Ctrl Pts',(-25.1459747153606,13.1085293603561,
130.764170454789)) ;
#130037=CARTESIAN_POINT('Ctrl Pts',(-25.1701258151212,13.4184312880114,
130.801450841833)) ;
#130038=CARTESIAN_POINT('Ctrl Pts',(-25.1672868025462,13.725396861632,130.760244966017)) ;
#130039=CARTESIAN_POINT('Ctrl Pts',(-25.1382759895552,14.0140710256624,
130.642207480891)) ;
#130040=CARTESIAN_POINT('Ctrl Pts',(-25.0860152986228,14.2586953044857,
130.45643248086)) ;
#130041=CARTESIAN_POINT('Ctrl Pts',(-25.0150543029557,14.4435712314573,
130.216035138787)) ;
#130042=CARTESIAN_POINT('Ctrl Pts',(-24.9310895100697,14.5554638006899,
129.93764282236)) ;
#130043=CARTESIAN_POINT('Ctrl Pts',(-24.8408606796343,14.5862678502932,
129.640940642294)) ;
#130044=CARTESIAN_POINT('Ctrl Pts',(-24.7516930753071,14.5339455436029,
129.347384079267)) ;
#130045=CARTESIAN_POINT('Ctrl Pts',(-24.6703799463621,14.4019055973539,
129.076694015721)) ;
#130046=CARTESIAN_POINT('Ctrl Pts',(-24.60374205745,14.1996929983724,128.848891564666)) ;
#130047=CARTESIAN_POINT('Ctrl Pts',(-24.5572296961542,13.9418840737313,
128.679885640708)) ;
#130048=CARTESIAN_POINT('Ctrl Pts',(-24.5348995734261,13.6467946760401,
128.581512428971)) ;
#130049=CARTESIAN_POINT('Ctrl Pts',(-24.5390899690228,13.3358858786889,
128.560634084449)) ;
#130050=CARTESIAN_POINT('Ctrl Pts',(-24.5701795719701,13.0311284856173,
128.618330046274)) ;
#130051=CARTESIAN_POINT('Ctrl Pts',(-24.6268180622581,12.7543596486341,
128.750628733576)) ;
#130052=CARTESIAN_POINT('Ctrl Pts',(-24.7050311793029,12.5263865010007,
128.946135952786)) ;
#130053=CARTESIAN_POINT('Ctrl Pts',(-24.8017020723011,12.3607018495905,
129.1951266527)) ;
#130054=CARTESIAN_POINT('Ctrl Pts',(-24.9076373162968,12.2732420345152,
129.471773127455)) ;
#130055=CARTESIAN_POINT('Ctrl Pts',(-25.019108352556,12.2668291057712,129.764141625486)) ;
#130056=CARTESIAN_POINT('Ctrl Pts',(-25.1268880991479,12.3436151679642,
130.045917699935)) ;
#130057=CARTESIAN_POINT('Ctrl Pts',(-25.2248793133505,12.4979166687538,
130.298995565544)) ;
#130058=CARTESIAN_POINT('Ctrl Pts',(-25.3062265907711,12.7181779713464,
130.503539894247)) ;
#130059=CARTESIAN_POINT('Ctrl Pts',(-25.3661555440321,12.9887183065796,
130.645518524112)) ;
#130060=CARTESIAN_POINT('Ctrl Pts',(-25.4011086939028,13.2908825887428,
130.714479030165)) ;
#130061=CARTESIAN_POINT('Ctrl Pts',(-25.4092132990991,13.6021682784688,
130.70504715979)) ;
#130062=CARTESIAN_POINT('Ctrl Pts',(-25.3905897140097,13.9015372403182,
130.617436728814)) ;
#130063=CARTESIAN_POINT('Ctrl Pts',(-25.3471895019976,14.1661756912177,
130.457466439887)) ;
#130064=CARTESIAN_POINT('Ctrl Pts',(-25.283475751484,14.3763136257562,130.238379001657)) ;
#130065=CARTESIAN_POINT('Ctrl Pts',(-25.2038316680715,14.5195378836765,
129.972523388979)) ;
#130066=CARTESIAN_POINT('Ctrl Pts',(-25.1155555814888,14.5837467686513,
129.681630393675)) ;
#130067=CARTESIAN_POINT('Ctrl Pts',(-25.0247905890407,14.5651055728363,
129.383278007598)) ;
#130068=CARTESIAN_POINT('Ctrl Pts',(-24.9394526693564,14.4645029027952,
129.100861825567)) ;
#130069=CARTESIAN_POINT('Ctrl Pts',(-24.8661197664223,14.2890440216263,
128.853472968967)) ;
#130070=CARTESIAN_POINT('Ctrl Pts',(-24.8110505251749,14.0526945141533,
128.659594364076)) ;
#130071=CARTESIAN_POINT('Ctrl Pts',(-24.7784342225117,13.769986617102,128.531126378095)) ;
#130072=CARTESIAN_POINT('Ctrl Pts',(-24.771626872808,13.4631529516268,128.478150286101)) ;
#130073=CARTESIAN_POINT('Ctrl Pts',(-24.7920899070549,13.1513621108982,
128.504596727791)) ;
#130074=CARTESIAN_POINT('Ctrl Pts',(-24.8382943929961,12.8627668355385,
128.606681449633)) ;
#130075=CARTESIAN_POINT('Ctrl Pts',(-24.9089211448075,12.6109028724027,
128.779662777081)) ;
#130076=CARTESIAN_POINT('Ctrl Pts',(-24.9977863342769,12.420019305974,129.006391048658)) ;
#130077=CARTESIAN_POINT('Ctrl Pts',(-25.1018228161412,12.2986947230639,
129.276907811114)) ;
#130078=CARTESIAN_POINT('Ctrl Pts',(-25.2113470557582,12.259272392657,129.563951755654)) ;
#130079=CARTESIAN_POINT('Ctrl Pts',(-25.3219618782627,12.3030853474754,
129.853781195152)) ;
#130080=CARTESIAN_POINT('Ctrl Pts',(-25.4239394298828,12.4259705757025,
130.118810360826)) ;
#130081=CARTESIAN_POINT('Ctrl Pts',(-25.5132843704644,12.6220549882292,
130.346490329366)) ;
#130082=CARTESIAN_POINT('Ctrl Pts',(-25.5823256886098,12.8744669108447,
130.515101999542)) ;
#130083=CARTESIAN_POINT('Ctrl Pts',(-25.6277091251102,13.1663405634683,
130.614553329165)) ;
#130084=CARTESIAN_POINT('Ctrl Pts',(-25.6467159933288,13.4758788255352,
130.637032806762)) ;
#130085=CARTESIAN_POINT('Ctrl Pts',(-25.638912605484,13.7823952267848,130.581117864475)) ;
#130086=CARTESIAN_POINT('Ctrl Pts',(-25.605083495813,14.0644181271455,130.4490002908)) ;
#130087=CARTESIAN_POINT('Ctrl Pts',(-25.5492735285762,14.2977470624668,
130.253047631057)) ;
#130088=CARTESIAN_POINT('Ctrl Pts',(-25.475180464955,14.470619356869,130.003380356877)) ;
#130089=CARTESIAN_POINT('Ctrl Pts',(-25.3894108294434,14.5675954870708,
129.719686882913)) ;
#130090=CARTESIAN_POINT('Ctrl Pts',(-25.2989629243675,14.5827756114501,
129.422402440643)) ;
#130091=CARTESIAN_POINT('Ctrl Pts',(-25.2105889079703,14.5148009028155,
129.131086132755)) ;
#130092=CARTESIAN_POINT('Ctrl Pts',(-25.1317819491608,14.369224395635,128.867826008019)) ;
#130093=CARTESIAN_POINT('Ctrl Pts',(-25.0682405512477,14.1540995770501,
128.648890563742)) ;
#130094=CARTESIAN_POINT('Ctrl Pts',(-25.0263127249798,13.8891947674814,
128.493467439993)) ;
#130095=CARTESIAN_POINT('Ctrl Pts',(-25.0087151808049,13.5894850421774,
128.408911577462)) ;
#130096=CARTESIAN_POINT('Ctrl Pts',(-25.0180502307985,13.2771023843451,
128.402962217407)) ;
#130097=CARTESIAN_POINT('Ctrl Pts',(-25.0539881461516,12.9767130862842,
128.474903380437)) ;
#130098=CARTESIAN_POINT('Ctrl Pts',(-25.1153594134085,12.7063603271624,
128.620882754512)) ;
#130099=CARTESIAN_POINT('Ctrl Pts',(-25.1971076916216,12.4901610418877,
128.826797301287)) ;
#130100=CARTESIAN_POINT('Ctrl Pts',(-25.2956565313931,12.3386882869186,
129.081490867723)) ;
#130101=CARTESIAN_POINT('Ctrl Pts',(-25.4037767211478,12.2654833410071,
129.364243566983)) ;
#130102=CARTESIAN_POINT('Ctrl Pts',(-25.5149608400151,12.2750423619251,
129.655858772134)) ;
#130103=CARTESIAN_POINT('Ctrl Pts',(-25.62166667954,12.3673308735559,129.934393950309)) ;
#130104=CARTESIAN_POINT('Ctrl Pts',(-25.7165022687578,12.5343468737747,
130.178429108854)) ;
#130105=CARTESIAN_POINT('Ctrl Pts',(-25.7943039636434,12.7652870390172,
130.372595003719)) ;
#130106=CARTESIAN_POINT('Ctrl Pts',(-25.8499392894425,13.0444118412715,
130.501898406253)) ;
#130107=CARTESIAN_POINT('Ctrl Pts',(-25.8798587035347,13.3498616588083,
130.556181727478)) ;
#130108=CARTESIAN_POINT('Ctrl Pts',(-25.8827771353525,13.6613614501294,
130.531495893468)) ;
#130109=CARTESIAN_POINT('Ctrl Pts',(-25.8593804684295,13.9537821761938,
130.430165894424)) ;
#130110=CARTESIAN_POINT('Ctrl Pts',(-25.8119584670191,14.2096141280325,
130.25850584693)) ;
#130111=CARTESIAN_POINT('Ctrl Pts',(-25.7445330464467,14.4090573125523,
130.028392541274)) ;
#130112=CARTESIAN_POINT('Ctrl Pts',(-25.6628970061439,14.5378227703646,
129.756818694175)) ;
#130113=CARTESIAN_POINT('Ctrl Pts',(-25.5730799531226,14.586641023904,129.461192374976)) ;
#130114=CARTESIAN_POINT('Ctrl Pts',(-25.483496675564,14.5524956993372,129.166576918439)) ;
#130115=CARTESIAN_POINT('Ctrl Pts',(-25.3993139751561,14.4363359778134,
128.887285569447)) ;
#130116=CARTESIAN_POINT('Ctrl Pts',(-25.3293572590476,14.2487612489542,
128.649931064422)) ;
#130117=CARTESIAN_POINT('Ctrl Pts',(-25.2781045437042,14.001996361713,128.467114957121)) ;
#130118=CARTESIAN_POINT('Ctrl Pts',(-25.250215263522,13.7133413728872,128.352510202207)) ;
#130119=CARTESIAN_POINT('Ctrl Pts',(-25.2485729664507,13.4034231145874,
128.31452669011)) ;
#130120=CARTESIAN_POINT('Ctrl Pts',(-25.2737311770127,13.096615616376,128.35502835555)) ;
#130121=CARTESIAN_POINT('Ctrl Pts',(-25.3252318166841,12.8104956483767,
128.472164048683)) ;
#130122=CARTESIAN_POINT('Ctrl Pts',(-25.399266285014,12.5707042667784,128.655417699095)) ;
#130123=CARTESIAN_POINT('Ctrl Pts',(-25.491768455404,12.391019395432,128.892529678587)) ;
#130124=CARTESIAN_POINT('Ctrl Pts',(-25.5968872536902,12.2853288824572,
129.166465407052)) ;
#130125=CARTESIAN_POINT('Ctrl Pts',(-25.7074275379451,12.2609818492728,
129.456317516163)) ;
#130126=CARTESIAN_POINT('Ctrl Pts',(-25.8172037544521,12.320475723284,129.74370091659)) ;
#130127=CARTESIAN_POINT('Ctrl Pts',(-25.9174068491702,12.4582515201719,
130.003416142013)) ;
#130128=CARTESIAN_POINT('Ctrl Pts',(-26.0030700444993,12.6658997536836,
130.220462101582)) ;
#130129=CARTESIAN_POINT('Ctrl Pts',(-26.0678508238643,12.9268094738204,
130.3766640491)) ;
#130130=CARTESIAN_POINT('Ctrl Pts',(-26.1084061300055,13.2233760165972,
130.462053917808)) ;
#130131=CARTESIAN_POINT('Ctrl Pts',(-26.1224375596645,13.5346575170046,
130.469920578644)) ;
#130132=CARTESIAN_POINT('Ctrl Pts',(-26.1094897742864,13.8387959699086,
130.398875623468)) ;
#130133=CARTESIAN_POINT('Ctrl Pts',(-26.0713053088302,14.1123016431052,
130.254200206036)) ;
#130134=CARTESIAN_POINT('Ctrl Pts',(-26.0113054939942,14.3364686131329,
130.045772465312)) ;
#130135=CARTESIAN_POINT('Ctrl Pts',(-25.9349000952512,14.4947707498965,
129.789555101611)) ;
#130136=CARTESIAN_POINT('Ctrl Pts',(-25.847424432091,14.5769227712613,129.500776994959)) ;
#130137=CARTESIAN_POINT('Ctrl Pts',(-25.7571700794344,14.5762675707607,
129.204175853418)) ;
#130138=CARTESIAN_POINT('Ctrl Pts',(-25.6698503685572,14.493055502163,128.915876035084)) ;
#130139=CARTESIAN_POINT('Ctrl Pts',(-25.593444376005,14.3331651665745,128.659561752647)) ;
#130140=CARTESIAN_POINT('Ctrl Pts',(-25.5338234294376,14.1081177718604,
128.452263061707)) ;
#130141=CARTESIAN_POINT('Ctrl Pts',(-25.4960451793118,13.8340180428126,
128.308780387983)) ;
#130142=CARTESIAN_POINT('Ctrl Pts',(-25.4835318306803,13.5302900584997,
128.239082101355)) ;
#130143=CARTESIAN_POINT('Ctrl Pts',(-25.4979122407888,13.2194243094674,
128.24800347794)) ;
#130144=CARTESIAN_POINT('Ctrl Pts',(-25.5387210538809,12.9232189359804,
128.334150129687)) ;
#130145=CARTESIAN_POINT('Ctrl Pts',(-25.6043090215129,12.6614613466154,
128.492497917721)) ;
#130146=CARTESIAN_POINT('Ctrl Pts',(-25.6897562965941,12.4560560790089,
128.709114179214)) ;
#130147=CARTESIAN_POINT('Ctrl Pts',(-25.7905081105,12.3187614770299,128.970300671274)) ;
#130148=CARTESIAN_POINT('Ctrl Pts',(-25.9000226576879,12.2608758941321,
129.257026905128)) ;
#130149=CARTESIAN_POINT('Ctrl Pts',(-26.0104797637691,12.2860567415008,
129.546655594556)) ;
#130150=CARTESIAN_POINT('Ctrl Pts',(-26.1159736762641,12.3936760642326,
129.821514421549)) ;
#130151=CARTESIAN_POINT('Ctrl Pts',(-26.2077752209374,12.5734426987992,
130.056754959979)) ;
#130152=CARTESIAN_POINT('Ctrl Pts',(-26.2819090991338,12.8155556665824,
130.240092263776)) ;
#130153=CARTESIAN_POINT('Ctrl Pts',(-26.3326381883263,13.1001458874772,
130.355223107769)) ;
#130154=CARTESIAN_POINT('Ctrl Pts',(-26.3575582974656,13.4082451870112,
130.394897541893)) ;
#130155=CARTESIAN_POINT('Ctrl Pts',(-26.3555548909241,13.7170001852575,
130.355978042951)) ;
#130156=CARTESIAN_POINT('Ctrl Pts',(-26.3271329019922,14.0068803460707,
130.239616500101)) ;
#130157=CARTESIAN_POINT('Ctrl Pts',(-26.2756477863993,14.2520830316222,
130.056220302137)) ;
#130158=CARTESIAN_POINT('Ctrl Pts',(-26.2052864210748,14.4388654813696,
129.817614241307)) ;
#130159=CARTESIAN_POINT('Ctrl Pts',(-26.1215233775957,14.5532758693692,
129.539771420139)) ;
#130160=CARTESIAN_POINT('Ctrl Pts',(-26.0313033647725,14.5866372914021,
129.243071371308)) ;
#130161=CARTESIAN_POINT('Ctrl Pts',(-25.9417632337185,14.536325428207,128.948328411036)) ;
#130162=CARTESIAN_POINT('Ctrl Pts',(-25.8604875007569,14.4070821895425,
128.677900419032)) ;
#130163=CARTESIAN_POINT('Ctrl Pts',(-25.7930114331716,14.2058492618622,
128.447493048992)) ;
#130164=CARTESIAN_POINT('Ctrl Pts',(-25.745989866581,13.9493210754263,128.277020775163)) ;
#130165=CARTESIAN_POINT('Ctrl Pts',(-25.7229926511202,13.6560817466226,
128.176815880105)) ;
#130166=CARTESIAN_POINT('Ctrl Pts',(-25.7263604626951,13.3454214916358,
128.153541083346)) ;
#130167=CARTESIAN_POINT('Ctrl Pts',(-25.75653203912,13.0405959101595,128.208610801399)) ;
#130168=CARTESIAN_POINT('Ctrl Pts',(-25.8127824032737,12.7610204461784,
128.339579180513)) ;
#130169=CARTESIAN_POINT('Ctrl Pts',(-25.8904302641907,12.5320805798767,
128.533479631004)) ;
#130170=CARTESIAN_POINT('Ctrl Pts',(-25.9859544465224,12.3651154017827,
128.779347978492)) ;
#130171=CARTESIAN_POINT('Ctrl Pts',(-26.092542096783,12.2743250187668,129.057620383868)) ;
#130172=CARTESIAN_POINT('Ctrl Pts',(-26.2040626873145,12.2660445050815,
129.350117816326)) ;
#130173=CARTESIAN_POINT('Ctrl Pts',(-26.3116128241466,12.3402670873944,
129.631347677385)) ;
#130174=CARTESIAN_POINT('Ctrl Pts',(-26.4100212191217,12.4924310818324,
129.885636405723)) ;
#130175=CARTESIAN_POINT('Ctrl Pts',(-26.4918260757063,12.7106680082788,
130.091558972653)) ;
#130176=CARTESIAN_POINT('Ctrl Pts',(-26.5525962863501,12.9803448576749,
130.235943356586)) ;
#130177=CARTESIAN_POINT('Ctrl Pts',(-26.5883391529532,13.2833169308344,
130.30706416664)) ;
#130178=CARTESIAN_POINT('Ctrl Pts',(-26.5971320647006,13.5926826730587,
130.299854627125)) ;
#130179=CARTESIAN_POINT('Ctrl Pts',(-26.5792466524351,13.8936496800992,
130.21429663377)) ;
#130180=CARTESIAN_POINT('Ctrl Pts',(-26.5365931556998,14.1589429573028,
130.056588090138)) ;
#130181=CARTESIAN_POINT('Ctrl Pts',(-26.4733112450839,14.371150690962,129.838705183338)) ;
#130182=CARTESIAN_POINT('Ctrl Pts',(-26.3943156088787,14.5162610236172,
129.574855837709)) ;
#130183=CARTESIAN_POINT('Ctrl Pts',(-26.3054716122965,14.5833063391636,
129.282028478141)) ;
#130184=CARTESIAN_POINT('Ctrl Pts',(-26.2149058148592,14.5665129861826,
128.984347754554)) ;
#130185=CARTESIAN_POINT('Ctrl Pts',(-26.1296349482658,14.4685224536154,
128.702240983504)) ;
#130186=CARTESIAN_POINT('Ctrl Pts',(-26.055901030885,14.2954966749806,128.453723607246)) ;
#130187=CARTESIAN_POINT('Ctrl Pts',(-26.000035182886,14.0596947072176,128.257378016009)) ;
#130188=CARTESIAN_POINT('Ctrl Pts',(-25.9667582155581,13.7784556667528,
128.12704153871)) ;
#130189=CARTESIAN_POINT('Ctrl Pts',(-25.9593349700014,13.4704205936671,
128.072089582602)) ;
#130190=CARTESIAN_POINT('Ctrl Pts',(-25.9786379348954,13.1626907214352,
128.095620872259)) ;
#130191=CARTESIAN_POINT('Ctrl Pts',(-26.024568251676,12.8697533437124,128.196503840888)) ;
#130192=CARTESIAN_POINT('Ctrl Pts',(-26.0939304436759,12.618666846953,128.366102809598)) ;
#130193=CARTESIAN_POINT('Ctrl Pts',(-26.1831183712039,12.424057056317,128.593453303362)) ;
#130194=CARTESIAN_POINT('Ctrl Pts',(-26.2857494091626,12.301712900972,128.860227719189)) ;
#130195=CARTESIAN_POINT('Ctrl Pts',(-26.3959672181736,12.2592124432014,
129.149039423007)) ;
#130196=CARTESIAN_POINT('Ctrl Pts',(-26.5061419238419,12.300200425655,129.437764546279)) ;
#130197=CARTESIAN_POINT('Ctrl Pts',(-26.6094954585518,12.4222100084694,
129.706457390739)) ;
#130198=CARTESIAN_POINT('Ctrl Pts',(-26.6985712830069,12.6151763749812,
129.93361606151)) ;
#130199=CARTESIAN_POINT('Ctrl Pts',(-26.7684896012397,12.8667635353633,
130.104687662764)) ;
#130200=CARTESIAN_POINT('Ctrl Pts',(-26.8144251071473,13.1566082723263,
130.205889756394)) ;
#130201=CARTESIAN_POINT('Ctrl Pts',(-26.834380951446,13.4669634672463,130.23102669691)) ;
#130202=CARTESIAN_POINT('Ctrl Pts',(-26.827214904313,13.7743605227785,130.176916300451)) ;
#130203=CARTESIAN_POINT('Ctrl Pts',(-26.7943756619693,14.0556835016132,
130.047907219521)) ;
#130204=CARTESIAN_POINT('Ctrl Pts',(-26.7388548120431,14.2923698001693,
129.852577489673)) ;
#130205=CARTESIAN_POINT('Ctrl Pts',(-26.6650281834544,14.4669397818909,
129.603657958846)) ;
#130206=CARTESIAN_POINT('Ctrl Pts',(-26.5799991592676,14.5658236939165,
129.322316054393)) ;
#130207=CARTESIAN_POINT('Ctrl Pts',(-26.4890730846777,14.5834030857371,
129.023436802721)) ;
#130208=CARTESIAN_POINT('Ctrl Pts',(-26.4010181587823,14.5182209911816,
128.733249100209)) ;
#130209=CARTESIAN_POINT('Ctrl Pts',(-26.3211717954855,14.3732473260144,
128.466642858011)) ;
#130210=CARTESIAN_POINT('Ctrl Pts',(-26.2577722791704,14.1617341890797,
128.248450584103)) ;
#130211=CARTESIAN_POINT('Ctrl Pts',(-26.2148585718976,13.8968740490593,
128.08996654976)) ;
#130212=CARTESIAN_POINT('Ctrl Pts',(-26.1966227215079,13.5970562228853,
128.003481258227)) ;
#130213=CARTESIAN_POINT('Ctrl Pts',(-26.2052628641563,13.2853499830191,
127.995568689957)) ;
#130214=CARTESIAN_POINT('Ctrl Pts',(-26.2403552083071,12.9854215224893,
128.065151386669)) ;
#130215=CARTESIAN_POINT('Ctrl Pts',(-26.3007530503343,12.7145027585382,
128.208390021964)) ;
#130216=CARTESIAN_POINT('Ctrl Pts',(-26.3823022410149,12.4953423449653,
128.413561260671)) ;
#130217=CARTESIAN_POINT('Ctrl Pts',(-26.4806652696605,12.3417858317011,
128.667663037527)) ;
#130218=CARTESIAN_POINT('Ctrl Pts',(-26.5882930356624,12.2665368316973,
128.949071919843)) ;
#130219=CARTESIAN_POINT('Ctrl Pts',(-26.6993769112587,12.2735361419267,
129.240428663002)) ;
#130220=CARTESIAN_POINT('Ctrl Pts',(-26.8062769983724,12.363229877568,129.519550348536)) ;
#130221=CARTESIAN_POINT('Ctrl Pts',(-26.9018479830977,12.5286846808382,
129.765628188398)) ;
#130222=CARTESIAN_POINT('Ctrl Pts',(-26.9801291972496,12.7579693374739,
129.961216881114)) ;
#130223=CARTESIAN_POINT('Ctrl Pts',(-27.0363720503262,13.0352201558529,
130.092378992134)) ;
#130224=CARTESIAN_POINT('Ctrl Pts',(-27.0671269832124,13.3405827861553,
130.149055244298)) ;
#130225=CARTESIAN_POINT('Ctrl Pts',(-27.0708970811726,13.6512270836361,
130.126969755603)) ;
#130226=CARTESIAN_POINT('Ctrl Pts',(-27.0482279288328,13.9458586294117,
130.027616439483)) ;
#130227=CARTESIAN_POINT('Ctrl Pts',(-27.0012885597917,14.2033946145398,
129.857305947176)) ;
#130228=CARTESIAN_POINT('Ctrl Pts',(-26.9345407993142,14.4040390929878,
129.629266290777)) ;
#130229=CARTESIAN_POINT('Ctrl Pts',(-26.85334590466,14.5350227299355,129.359015173723)) ;
#130230=CARTESIAN_POINT('Ctrl Pts',(-26.7635252041074,14.5864958770583,
129.06333080397)) ;
#130231=CARTESIAN_POINT('Ctrl Pts',(-26.6736873277468,14.5544169288515,
128.767901047483)) ;
#130232=CARTESIAN_POINT('Ctrl Pts',(-26.5897148721243,14.4414134411267,
128.489433678146)) ;
#130233=CARTESIAN_POINT('Ctrl Pts',(-26.5189024761237,14.2551029687745,
128.249417390294)) ;
#130234=CARTESIAN_POINT('Ctrl Pts',(-26.4670805480505,14.0100365363148,
128.064977335595)) ;
#130235=CARTESIAN_POINT('Ctrl Pts',(-26.4384400244146,13.7214335689568,
127.948077488775)) ;
#130236=CARTESIAN_POINT('Ctrl Pts',(-26.435974371304,13.4135493064467,127.907881396188)) ;
#130237=CARTESIAN_POINT('Ctrl Pts',(-26.4605255580527,13.1045553590735,
127.946402200391)) ;
#130238=CARTESIAN_POINT('Ctrl Pts',(-26.5108395176121,12.8197359183053,
128.060352490887)) ;
#130239=CARTESIAN_POINT('Ctrl Pts',(-26.5848090385455,12.5762135336046,
128.243133399849)) ;
#130240=CARTESIAN_POINT('Ctrl Pts',(-26.6767305633784,12.3952020079458,
128.478624662692)) ;
#130241=CARTESIAN_POINT('Ctrl Pts',(-26.7816921203493,12.2871509240411,
128.752062073402)) ;
#130242=CARTESIAN_POINT('Ctrl Pts',(-26.8919186056864,12.260566124011,129.041074313787)) ;
#130243=CARTESIAN_POINT('Ctrl Pts',(-27.0018360824349,12.3174695873532,
129.328875433493)) ;
#130244=CARTESIAN_POINT('Ctrl Pts',(-27.1026169626887,12.453509519007,129.590196755254)) ;
#130245=CARTESIAN_POINT('Ctrl Pts',(-27.1885697033625,12.6588730452131,
129.80817298517)) ;
#130246=CARTESIAN_POINT('Ctrl Pts',(-27.2540789212245,12.918573180631,129.966479194314)) ;
#130247=CARTESIAN_POINT('Ctrl Pts',(-27.2953789589594,13.2144046243544,
130.054046631809)) ;
#130248=CARTESIAN_POINT('Ctrl Pts',(-27.3101837233567,13.5255440796009,
130.064173865051)) ;
#130249=CARTESIAN_POINT('Ctrl Pts',(-27.2980790148711,13.829753908523,129.995651392622)) ;
#130250=CARTESIAN_POINT('Ctrl Pts',(-27.2605055755069,14.1049217078337,
129.852691968057)) ;
#130251=CARTESIAN_POINT('Ctrl Pts',(-27.201449003967,14.3298723137222,129.647191490044)) ;
#130252=CARTESIAN_POINT('Ctrl Pts',(-27.1249177570824,14.4915527560892,
129.390360258502)) ;
#130253=CARTESIAN_POINT('Ctrl Pts',(-27.0379228723855,14.5755974314799,
129.103103428759)) ;
#130254=CARTESIAN_POINT('Ctrl Pts',(-26.9475249321661,14.5774288452973,
128.806022504469)) ;
#130255=CARTESIAN_POINT('Ctrl Pts',(-26.8602123103374,14.4968431861705,
128.517832330982)) ;
#130256=CARTESIAN_POINT('Ctrl Pts',(-26.7831288401317,14.338559634622,128.259421353338)) ;
#130257=CARTESIAN_POINT('Ctrl Pts',(-26.7230100498861,14.1152211662258,
128.050691457082)) ;
#130258=CARTESIAN_POINT('Ctrl Pts',(-26.6845517589779,13.8419815633955,
127.905190962222)) ;
#130259=CARTESIAN_POINT('Ctrl Pts',(-26.6713188132477,13.5398086158385,
127.833500347495)) ;
#130260=CARTESIAN_POINT('Ctrl Pts',(-26.6848767081703,13.2280436814142,
127.839935470396)) ;
#130261=CARTESIAN_POINT('Ctrl Pts',(-26.7252319504286,12.9300591800615,
127.924625401279)) ;
#130262=CARTESIAN_POINT('Ctrl Pts',(-26.789898437,12.6684085006953,128.080447400552)) ;
#130263=CARTESIAN_POINT('Ctrl Pts',(-26.8749504447235,12.4608091979395,
128.295851853874)) ;
#130264=CARTESIAN_POINT('Ctrl Pts',(-26.9754442077812,12.3214093724075,
128.556266165395)) ;
#130265=CARTESIAN_POINT('Ctrl Pts',(-27.0849883594925,12.2613303026755,
128.843029640314)) ;
#130266=CARTESIAN_POINT('Ctrl Pts',(-27.1950704339796,12.2843254889888,
129.131687712862)) ;
#130267=CARTESIAN_POINT('Ctrl Pts',(-27.300365347957,12.3887269550652,129.406127183944)) ;
#130268=CARTESIAN_POINT('Ctrl Pts',(-27.3932129896385,12.5673627247375,
129.644228488839)) ;
#130269=CARTESIAN_POINT('Ctrl Pts',(-27.4678735203102,12.8080166646894,
129.829115438456)) ;
#130270=CARTESIAN_POINT('Ctrl Pts',(-27.5193391617637,13.0914774239872,
129.946409122059)) ;
#130271=CARTESIAN_POINT('Ctrl Pts',(-27.5450607387376,13.4005589621793,
129.988284468122)) ;
#130272=CARTESIAN_POINT('Ctrl Pts',(-27.543724962801,13.7083911586178,129.951439629823)) ;
#130273=CARTESIAN_POINT('Ctrl Pts',(-27.5161530969791,13.9985991401632,
129.837634676897)) ;
#130274=CARTESIAN_POINT('Ctrl Pts',(-27.4652173082198,14.2457812582848,
129.655783326903)) ;
#130275=CARTESIAN_POINT('Ctrl Pts',(-27.3952646502479,14.4345734163401,
129.418349238306)) ;
#130276=CARTESIAN_POINT('Ctrl Pts',(-27.3117425688963,14.5511370874347,
129.141196953696)) ;
#130277=CARTESIAN_POINT('Ctrl Pts',(-27.221888274012,14.5867802184263,128.845665992633)) ;
#130278=CARTESIAN_POINT('Ctrl Pts',(-27.1322077328839,14.5391948509929,
128.550515130345)) ;
#130279=CARTESIAN_POINT('Ctrl Pts',(-27.0503290364503,14.4115345503253,
128.278202231081)) ;
#130280=CARTESIAN_POINT('Ctrl Pts',(-26.9827628806094,14.2134356096031,
128.047738422895)) ;
#130281=CARTESIAN_POINT('Ctrl Pts',(-26.9348844871769,13.9582378109792,
127.874714631013)) ;
#130282=CARTESIAN_POINT('Ctrl Pts',(-26.9110599740153,13.6646543280563,
127.771965764763)) ;
#130283=CARTESIAN_POINT('Ctrl Pts',(-26.91366722638,13.3541837462344,127.746474671201)) ;
#130284=CARTESIAN_POINT('Ctrl Pts',(-26.9432027330941,13.0484270052538,
127.799627992835)) ;
#130285=CARTESIAN_POINT('Ctrl Pts',(-26.9984107380162,12.7694396720145,
127.927751926342)) ;
#130286=CARTESIAN_POINT('Ctrl Pts',(-27.0755390330106,12.5380418317107,
128.120059948438)) ;
#130287=CARTESIAN_POINT('Ctrl Pts',(-27.171221668837,12.3683286468607,128.366208709594)) ;
#130288=CARTESIAN_POINT('Ctrl Pts',(-27.2771022295698,12.276042045724,128.642572712994)) ;
#130289=CARTESIAN_POINT('Ctrl Pts',(-27.3880887650464,12.2649171865401,
128.933659578238)) ;
#130290=CARTESIAN_POINT('Ctrl Pts',(-27.4963674529684,12.3368690244089,
129.216857680154)) ;
#130291=CARTESIAN_POINT('Ctrl Pts',(-27.5952212736886,12.4871141807711,
129.472423974844)) ;
#130292=CARTESIAN_POINT('Ctrl Pts',(-27.6777148254917,12.7041604883304,
129.680290662464)) ;
#130293=CARTESIAN_POINT('Ctrl Pts',(-27.7389269911776,12.9721741232452,
129.826038291155)) ;
#130294=CARTESIAN_POINT('Ctrl Pts',(-27.7753612070752,13.2726901834042,
129.899369582598)) ;
#130295=CARTESIAN_POINT('Ctrl Pts',(-27.7850730785568,13.5844633646991,
129.894589911837)) ;
#130296=CARTESIAN_POINT('Ctrl Pts',(-27.7678692054937,13.8852369971297,
129.811108822555)) ;
#130297=CARTESIAN_POINT('Ctrl Pts',(-27.7261471250055,14.1508959663415,
129.656248903553)) ;
#130298=CARTESIAN_POINT('Ctrl Pts',(-27.6632436611501,14.3659569774688,
129.43934922914)) ;
#130299=CARTESIAN_POINT('Ctrl Pts',(-27.5842577970922,14.5133844128615,
129.175402290824)) ;
#130300=CARTESIAN_POINT('Ctrl Pts',(-27.4963291774889,14.5822824831324,
128.885527648374)) ;
#130301=CARTESIAN_POINT('Ctrl Pts',(-27.405500321609,14.5684017849453,128.586993900287)) ;
#130302=CARTESIAN_POINT('Ctrl Pts',(-27.319795130659,14.4726240674175,128.303557584134)) ;
#130303=CARTESIAN_POINT('Ctrl Pts',(-27.2454365186279,14.3009018680156,
128.053107574427)) ;
#130304=CARTESIAN_POINT('Ctrl Pts',(-27.1892164396155,14.06766624957,127.855870686258)) ;
#130305=CARTESIAN_POINT('Ctrl Pts',(-27.1551562261205,13.7867923876229,
127.723158502822)) ;
#130306=CARTESIAN_POINT('Ctrl Pts',(-27.1469288346791,13.4808116155242,
127.666034034963)) ;
#130307=CARTESIAN_POINT('Ctrl Pts',(-27.1655283118666,13.170617767173,127.687268480993)) ;
#130308=CARTESIAN_POINT('Ctrl Pts',(-27.2108436491157,12.8770484299103,
127.786367681697)) ;
#130309=CARTESIAN_POINT('Ctrl Pts',(-27.2794629869719,12.6251910653491,
127.95386304123)) ;
#130310=CARTESIAN_POINT('Ctrl Pts',(-27.3679175166217,12.4289584805404,
128.179147517579)) ;
#130311=CARTESIAN_POINT('Ctrl Pts',(-27.4707943397875,12.3038002389648,
128.446461935893)) ;
#130312=CARTESIAN_POINT('Ctrl Pts',(-27.5806821586256,12.2593442697271,
128.734384059874)) ;
#130313=CARTESIAN_POINT('Ctrl Pts',(-27.6906991544956,12.297889877657,129.022718858313)) ;
#130314=CARTESIAN_POINT('Ctrl Pts',(-27.7941126443979,12.4169444300621,
129.291685993974)) ;
#130315=CARTESIAN_POINT('Ctrl Pts',(-27.8842880110467,12.6093773199724,
129.521822960951)) ;
#130316=CARTESIAN_POINT('Ctrl Pts',(-27.9544400462606,12.858373409298,129.693747600172)) ;
#130317=CARTESIAN_POINT('Ctrl Pts',(-28.0012932497617,13.1480449631144,
129.797538916571)) ;
#130318=CARTESIAN_POINT('Ctrl Pts',(-28.0219611305027,13.4582417774946,
129.824751677157)) ;
#130319=CARTESIAN_POINT('Ctrl Pts',(-28.0155964008347,13.7655078893865,
129.773039846849)) ;
#130320=CARTESIAN_POINT('Ctrl Pts',(-27.9834174873497,14.0483169401814,
129.645907135585)) ;
#130321=CARTESIAN_POINT('Ctrl Pts',(-27.9285710178481,14.2859989758831,
129.45261104353)) ;
#130322=CARTESIAN_POINT('Ctrl Pts',(-27.855464240207,14.4624790270523,129.205887839955)) ;
#130323=CARTESIAN_POINT('Ctrl Pts',(-27.7701186641137,14.5642183790962,
128.923397956241)) ;
#130324=CARTESIAN_POINT('Ctrl Pts',(-27.6798082098764,14.5841609537885,
128.626534158212)) ;
#130325=CARTESIAN_POINT('Ctrl Pts',(-27.5910388931153,14.5209707585958,
128.334043392546)) ;
#130326=CARTESIAN_POINT('Ctrl Pts',(-27.5114075236351,14.3791779816594,
128.068312186743)) ;
#130327=CARTESIAN_POINT('Ctrl Pts',(-27.4471074600154,14.1688152035408,
127.847338449402)) ;
#130328=CARTESIAN_POINT('Ctrl Pts',(-27.4035904915364,13.905195794164,127.687104563405)) ;
#130329=CARTESIAN_POINT('Ctrl Pts',(-27.384611020138,13.6071501662918,127.598555977474)) ;
#130330=CARTESIAN_POINT('Ctrl Pts',(-27.3922962592168,13.2953844839231,
127.587845500422)) ;
#130331=CARTESIAN_POINT('Ctrl Pts',(-27.4268849846127,12.9930170511922,
127.655749387647)) ;
#130332=CARTESIAN_POINT('Ctrl Pts',(-27.4863412339869,12.7222274559466,
127.796397689186)) ;
#130333=CARTESIAN_POINT('Ctrl Pts',(-27.5675596487005,12.5005441594065,
128.000493530296)) ;
#130334=CARTESIAN_POINT('Ctrl Pts',(-27.6655029278047,12.3451353729422,
128.25339244165)) ;
#130335=CARTESIAN_POINT('Ctrl Pts',(-27.7729606560881,12.2674914409628,
128.534295667148)) ;
#130336=CARTESIAN_POINT('Ctrl Pts',(-27.8843595706386,12.2722652498167,
128.826484838542)) ;
#130337=CARTESIAN_POINT('Ctrl Pts',(-27.9913638557461,12.3599738059354,
129.105934292724)) ;
#130338=CARTESIAN_POINT('Ctrl Pts',(-28.0869339569718,12.5226377882888,
129.352153264961)) ;
#130339=CARTESIAN_POINT('Ctrl Pts',(-28.1660588301959,12.7508221881861,
129.550110967057)) ;
#130340=CARTESIAN_POINT('Ctrl Pts',(-28.2230720094142,13.0279564689842,
129.683425341747)) ;
#130341=CARTESIAN_POINT('Ctrl Pts',(-28.2544101794435,13.3323086828982,
129.741867809916)) ;
#130342=CARTESIAN_POINT('Ctrl Pts',(-28.2589445257815,13.6420773453948,
129.722122425532)) ;
#130343=CARTESIAN_POINT('Ctrl Pts',(-28.2370620629136,13.9374077798728,
129.625077365952)) ;
#130344=CARTESIAN_POINT('Ctrl Pts',(-28.1908166629315,14.1965319026708,
129.456785919999)) ;
#130345=CARTESIAN_POINT('Ctrl Pts',(-28.1241408657345,14.3999725565714,
129.228766463816)) ;
#130346=CARTESIAN_POINT('Ctrl Pts',(-28.0436674073878,14.5320840030957,
128.960801672885)) ;
#130347=CARTESIAN_POINT('Ctrl Pts',(-27.9541399262844,14.5862914480512,
128.666024910394)) ;
#130348=CARTESIAN_POINT('Ctrl Pts',(-27.8637234344466,14.5562373226541,
128.368717388047)) ;
#130349=CARTESIAN_POINT('Ctrl Pts',(-27.7799959913736,14.4460760144195,
128.091169611102)) ;
#130350=CARTESIAN_POINT('Ctrl Pts',(-27.7083901687493,14.2613118721967,
127.848714187468)) ;
#130351=CARTESIAN_POINT('Ctrl Pts',(-27.6559630033685,14.0168342944474,
127.662425250751)) ;
#130352=CARTESIAN_POINT('Ctrl Pts',(-27.6267508456225,13.7314084897265,
127.5441079102)) ;
#130353=CARTESIAN_POINT('Ctrl Pts',(-27.6234740932792,13.421392773908,127.501273878671)) ;
#130354=CARTESIAN_POINT('Ctrl Pts',(-27.6471850767089,13.1138964793829,
127.537539991659)) ;
#130355=CARTESIAN_POINT('Ctrl Pts',(-27.6968203365939,12.8273574977414,
127.649425077265)) ;
#130356=CARTESIAN_POINT('Ctrl Pts',(-27.7702606510501,12.5821904329902,
127.830639707684)) ;
#130357=CARTESIAN_POINT('Ctrl Pts',(-27.861839260569,12.3992406705926,128.065098381216)) ;
#130358=CARTESIAN_POINT('Ctrl Pts',(-27.9661679392864,12.289263542394,128.336801966784)) ;
#130359=CARTESIAN_POINT('Ctrl Pts',(-28.0765570656966,12.260188272694,128.626216040664)) ;
#130360=CARTESIAN_POINT('Ctrl Pts',(-28.1862199043233,12.3144490228481,
128.913396049941)) ;
#130361=CARTESIAN_POINT('Ctrl Pts',(-28.2874611534108,12.4481500069378,
129.176032982046)) ;
#130362=CARTESIAN_POINT('Ctrl Pts',(-28.3739963556883,12.6515764939739,
129.395704973391)) ;
#130363=CARTESIAN_POINT('Ctrl Pts',(-28.4404957092632,12.9112089841373,
129.556741445295)) ;
#130364=CARTESIAN_POINT('Ctrl Pts',(-28.4824385774787,13.2069679929226,
129.646128611396)) ;
#130365=CARTESIAN_POINT('Ctrl Pts',(-28.4979265928733,13.5165269909875,
129.658410386569)) ;
#130366=CARTESIAN_POINT('Ctrl Pts',(-28.4864805841876,13.8224960289794,
129.591668568529)) ;
#130367=CARTESIAN_POINT('Ctrl Pts',(-28.4497259503042,14.0973149318537,
129.451272234263)) ;
#130368=CARTESIAN_POINT('Ctrl Pts',(-28.3911415052306,14.3244517336708,
129.24707906695)) ;
#130369=CARTESIAN_POINT('Ctrl Pts',(-28.3151295314421,14.4877799140032,
128.99182597903)) ;
#130370=CARTESIAN_POINT('Ctrl Pts',(-28.2284706441736,14.5742904717488,
128.705587672482)) ;
#130371=CARTESIAN_POINT('Ctrl Pts',(-28.1376899133625,14.5785355539825,
128.407248586976)) ;
#130372=CARTESIAN_POINT('Ctrl Pts',(-28.0503077690536,14.4999983626793,
128.118890382677)) ;
#130373=CARTESIAN_POINT('Ctrl Pts',(-27.9731621173562,14.3447574910545,
127.860457559928)) ;
#130374=CARTESIAN_POINT('Ctrl Pts',(-27.9122294488622,14.1223925047645,
127.64922484791)) ;
#130375=CARTESIAN_POINT('Ctrl Pts',(-27.8731709084535,13.8510687474612,
127.502062113222)) ;
#130376=CARTESIAN_POINT('Ctrl Pts',(-27.8590929134541,13.5484337104113,
127.427784531783)) ;
#130377=CARTESIAN_POINT('Ctrl Pts',(-27.8719163776156,13.237024252248,127.432120494693)) ;
#130378=CARTESIAN_POINT('Ctrl Pts',(-27.9113445504404,12.9391312355254,
127.514195973746)) ;
#130379=CARTESIAN_POINT('Ctrl Pts',(-27.9753555068171,12.6756661013292,
127.668058674229)) ;
#130380=CARTESIAN_POINT('Ctrl Pts',(-28.0601115514291,12.465702834837,127.88251153638)) ;
#130381=CARTESIAN_POINT('Ctrl Pts',(-28.1601996212556,12.3244745737951,
128.141765929243)) ;
#130382=CARTESIAN_POINT('Ctrl Pts',(-28.2690911173844,12.261923279364,128.426769586932)) ;
#130383=CARTESIAN_POINT('Ctrl Pts',(-28.3800087348888,12.2825882232678,
128.717633267237)) ;
#130384=CARTESIAN_POINT('Ctrl Pts',(-28.4852015134817,12.3846500947886,
128.991882531666)) ;
#130385=CARTESIAN_POINT('Ctrl Pts',(-28.5784888744531,12.5611186866008,
129.231275217992)) ;
#130386=CARTESIAN_POINT('Ctrl Pts',(-28.6537672249704,12.8001288642586,
129.417975019435)) ;
#130387=CARTESIAN_POINT('Ctrl Pts',(-28.7059764335205,13.0829558196603,
129.537398073433)) ;
#130388=CARTESIAN_POINT('Ctrl Pts',(-28.7324492944742,13.3903655314665,
129.581607157294)) ;
#130389=CARTESIAN_POINT('Ctrl Pts',(-28.7319069972317,13.7001366120665,
129.546896868265)) ;
#130390=CARTESIAN_POINT('Ctrl Pts',(-28.7051802274337,13.9898881855453,
129.435719523823)) ;
#130391=CARTESIAN_POINT('Ctrl Pts',(-28.6548256890378,14.2391934633215,
129.255489830682)) ;
#130392=CARTESIAN_POINT('Ctrl Pts',(-28.5854484722084,14.4298567311308,
129.019774640516)) ;
#130393=CARTESIAN_POINT('Ctrl Pts',(-28.5017241019675,14.549247146468,128.741836021843)) ;
#130394=CARTESIAN_POINT('Ctrl Pts',(-28.4122620032697,14.5868020953667,
128.447568519666)) ;
#130395=CARTESIAN_POINT('Ctrl Pts',(-28.3225462061262,14.5417975168182,
128.15234527836)) ;
#130396=CARTESIAN_POINT('Ctrl Pts',(-28.2403119417274,14.4162088309709,
127.878972537112)) ;
#130397=CARTESIAN_POINT('Ctrl Pts',(-28.1722916779625,14.2204083444341,
127.647230902494)) ;
#130398=CARTESIAN_POINT('Ctrl Pts',(-28.1235425964528,13.9647701488693,
127.471442670808)) ;
#130399=CARTESIAN_POINT('Ctrl Pts',(-28.0992051057573,13.6739289079279,
127.367425886203)) ;
#130400=CARTESIAN_POINT('Ctrl Pts',(-28.1010246977608,13.3623285568061,
127.339487139088)) ;
#130401=CARTESIAN_POINT('Ctrl Pts',(-28.1297460934695,13.0574725166072,
127.39040500141)) ;
#130402=CARTESIAN_POINT('Ctrl Pts',(-28.1841421871714,12.7770677802999,
127.516143688262)) ;
#130403=CARTESIAN_POINT('Ctrl Pts',(-28.2613693483408,12.5427865648713,
127.708501576232)) ;
#130404=CARTESIAN_POINT('Ctrl Pts',(-28.3554333317346,12.3731888767337,
127.950342074124)) ;
#130405=CARTESIAN_POINT('Ctrl Pts',(-28.4616743353883,12.2773794535172,
128.227548370542)) ;
#130406=CARTESIAN_POINT('Ctrl Pts',(-28.5729382888434,12.2641879567031,
128.519360391861)) ;
#130407=CARTESIAN_POINT('Ctrl Pts',(-28.6810056913039,12.3335960199066,
128.802056791109)) ;
#130408=CARTESIAN_POINT('Ctrl Pts',(-28.7802524593645,12.481561593043,129.058771350839)) ;
#130409=CARTESIAN_POINT('Ctrl Pts',(-28.8633376120415,12.6968286383091,
129.268361232323)) ;
#130410=CARTESIAN_POINT('Ctrl Pts',(-28.9253336378422,12.9642189214816,
129.416324935008)) ;
#130411=CARTESIAN_POINT('Ctrl Pts',(-28.9624937310787,13.2637553890215,
129.491819397087)) ;
#130412=CARTESIAN_POINT('Ctrl Pts',(-28.972907528442,13.576692280422,129.488959145133)) ;
#130413=CARTESIAN_POINT('Ctrl Pts',(-28.9566596492702,13.8753721133811,
129.408582768456)) ;
#130414=CARTESIAN_POINT('Ctrl Pts',(-28.9153488774168,14.1446744627024,
129.254642514762)) ;
#130415=CARTESIAN_POINT('Ctrl Pts',(-28.8529986443521,14.36064855191,129.039430067817)) ;
#130416=CARTESIAN_POINT('Ctrl Pts',(-28.7746869988663,14.5100785493016,
128.777556943832)) ;
#130417=CARTESIAN_POINT('Ctrl Pts',(-28.6862473882598,14.5815775750292,
128.485933784396)) ;
#130418=CARTESIAN_POINT('Ctrl Pts',(-28.5960567042962,14.5700420013307,
128.189517892522)) ;
#130419=CARTESIAN_POINT('Ctrl Pts',(-28.5097083215572,14.4761038026697,
127.90403247577)) ;
#130420=CARTESIAN_POINT('Ctrl Pts',(-28.4353102169461,14.307434697937,127.653662973433)) ;
#130421=CARTESIAN_POINT('Ctrl Pts',(-28.3780629448932,14.0735726732338,
127.453120130801)) ;
#130422=CARTESIAN_POINT('Ctrl Pts',(-28.3437086879326,13.7966475167134,
127.319908828553)) ;
#130423=CARTESIAN_POINT('Ctrl Pts',(-28.3345516471301,13.4894705902725,
127.259873174334)) ;
#130424=CARTESIAN_POINT('Ctrl Pts',(-28.3523600420796,13.1800818840159,
127.278908994309)) ;
#130425=CARTESIAN_POINT('Ctrl Pts',(-28.3968933889525,12.8853356480997,
127.375690302013)) ;
#130426=CARTESIAN_POINT('Ctrl Pts',(-28.4649418587295,12.6318026190054,
127.541487159906)) ;
#130427=CARTESIAN_POINT('Ctrl Pts',(-28.5529364364977,12.4337108597235,
127.765417467458)) ;
#130428=CARTESIAN_POINT('Ctrl Pts',(-28.6552780292447,12.3064394733644,
128.031235084983)) ;
#130429=CARTESIAN_POINT('Ctrl Pts',(-28.7653696886047,12.2594672530152,
128.319652084352)) ;
#130430=CARTESIAN_POINT('Ctrl Pts',(-28.8753666720429,12.2954707768407,
128.607972520882)) ;
#130431=CARTESIAN_POINT('Ctrl Pts',(-28.979671778032,12.4135506766909,128.879323664204)) ;
#130432=CARTESIAN_POINT('Ctrl Pts',(-29.0691225992057,12.6014761735562,
129.10779578289)) ;
#130433=CARTESIAN_POINT('Ctrl Pts',(-29.1405896682972,12.8505488639341,
129.283303377178)) ;
#130434=CARTESIAN_POINT('Ctrl Pts',(-29.1880749546232,13.1393106596108,
129.388963361721)) ;
#130435=CARTESIAN_POINT('Ctrl Pts',(-29.2095406027946,13.4495612540633,
129.41846797085)) ;
#130436=CARTESIAN_POINT('Ctrl Pts',(-29.2039386729016,13.7566530786408,
129.369046592978)) ;
#130437=CARTESIAN_POINT('Ctrl Pts',(-29.1725100853546,14.0404143241467,
129.244112794232)) ;
#130438=CARTESIAN_POINT('Ctrl Pts',(-29.118290079075,14.2798567692648,129.052639875831)) ;
#130439=CARTESIAN_POINT('Ctrl Pts',(-29.0452671941991,14.458860759646,128.806015875749)) ;
#130440=CARTESIAN_POINT('Ctrl Pts',(-28.9606501594039,14.5622468001176,
128.525844912294)) ;
#130441=CARTESIAN_POINT('Ctrl Pts',(-28.8700482731633,14.5847589339645,
128.227997078051)) ;
#130442=CARTESIAN_POINT('Ctrl Pts',(-28.781392052291,14.5239999698819,127.935939206979)) ;
#130443=CARTESIAN_POINT('Ctrl Pts',(-28.7012903847953,14.3842926564904,
127.668789039323)) ;
#130444=CARTESIAN_POINT('Ctrl Pts',(-28.6365025896643,14.1758059968765,
127.446409369018)) ;
#130445=CARTESIAN_POINT('Ctrl Pts',(-28.5922392795345,13.9130885413349,
127.283943329095)) ;
#130446=CARTESIAN_POINT('Ctrl Pts',(-28.5725792909746,13.615158117942,127.193350804081)) ;
#130447=CARTESIAN_POINT('Ctrl Pts',(-28.5794652562286,13.3050555466183,
127.180474632891)) ;
#130448=CARTESIAN_POINT('Ctrl Pts',(-28.6132034548497,13.0018872896554,
127.245876417844)) ;
#130449=CARTESIAN_POINT('Ctrl Pts',(-28.6721407618882,12.7291798994599,
127.384921051073)) ;
#130450=CARTESIAN_POINT('Ctrl Pts',(-28.7527600784641,12.5061727549264,
127.587299193783)) ;
#130451=CARTESIAN_POINT('Ctrl Pts',(-28.8499185291111,12.3489726739453,
127.838024044716)) ;
#130452=CARTESIAN_POINT('Ctrl Pts',(-28.9575837943938,12.2685650260664,
128.119403625798)) ;
#130453=CARTESIAN_POINT('Ctrl Pts',(-29.0685724130936,12.2709027283838,
128.410520048629)) ;
#130454=CARTESIAN_POINT('Ctrl Pts',(-29.1758527905754,12.3558099877511,
128.690771136075)) ;
#130455=CARTESIAN_POINT('Ctrl Pts',(-29.2723093402486,12.5172181290402,
128.939417104886)) ;
#130456=CARTESIAN_POINT('Ctrl Pts',(-29.3517344944281,12.7432704544133,
129.138342295771)) ;
#130457=CARTESIAN_POINT('Ctrl Pts',(-29.4093349032086,13.0180146572784,
129.273499224363)) ;
#130458=CARTESIAN_POINT('Ctrl Pts',(-29.4416696464702,13.3228198676384,
129.334738648409)) ;
#130459=CARTESIAN_POINT('Ctrl Pts',(-29.4469785768553,13.6334361388998,
129.31718165255)) ;
#130460=CARTESIAN_POINT('Ctrl Pts',(-29.425802066603,13.9294162640336,129.222205017795)) ;
#130461=CARTESIAN_POINT('Ctrl Pts',(-29.3803607950668,14.1891569843553,
129.05635848618)) ;
#130462=CARTESIAN_POINT('Ctrl Pts',(-29.3142875101324,14.3946401780078,
128.830106500029)) ;
#130463=CARTESIAN_POINT('Ctrl Pts',(-29.2338335030574,14.529556883976,128.562067703441)) ;
#130464=CARTESIAN_POINT('Ctrl Pts',(-29.1443491687741,14.5858061305694,
128.267386240536)) ;
#130465=CARTESIAN_POINT('Ctrl Pts',(-29.0543546782956,14.5585141813688,
127.971498106513)) ;
#130466=CARTESIAN_POINT('Ctrl Pts',(-28.9698827692536,14.4500372288901,
127.691587731276)) ;
#130467=CARTESIAN_POINT('Ctrl Pts',(-28.8982435279839,14.2682020295539,
127.449226628376)) ;
#130468=CARTESIAN_POINT('Ctrl Pts',(-28.8449675977318,14.0250734212292,
127.260391247175)) ;
#130469=CARTESIAN_POINT('Ctrl Pts',(-28.8149686665018,13.7389393527222,
127.139599745821)) ;
#130470=CARTESIAN_POINT('Ctrl Pts',(-28.8110043888609,13.4311036991076,
127.094955672536)) ;
#130471=CARTESIAN_POINT('Ctrl Pts',(-28.8337924395339,13.1229020252546,
127.128494988837)) ;
#130472=CARTESIAN_POINT('Ctrl Pts',(-28.8832606513019,12.8333723826346,
127.239628018119)) ;
#130473=CARTESIAN_POINT('Ctrl Pts',(-28.9553257919547,12.5895126808553,
127.417194804428)) ;
#130474=CARTESIAN_POINT('Ctrl Pts',(-29.0466937510159,12.4035405044014,
127.650907478714)) ;
#130475=CARTESIAN_POINT('Ctrl Pts',(-29.1507398374928,12.2914040543739,
127.921795177575)) ;
#130476=CARTESIAN_POINT('Ctrl Pts',(-29.2611690696662,12.2598122660064,
128.2112892169)) ;
#130477=CARTESIAN_POINT('Ctrl Pts',(-29.3710266223058,12.3118570092467,
128.499018026177)) ;
#130478=CARTESIAN_POINT('Ctrl Pts',(-29.4723911564959,12.4430958477667,
128.762082814677)) ;
#130479=CARTESIAN_POINT('Ctrl Pts',(-29.5595187815204,12.6447072106669,
128.983465986791)) ;
#130480=CARTESIAN_POINT('Ctrl Pts',(-29.6266409499539,12.9030426443817,
129.146318264826)) ;
#130481=CARTESIAN_POINT('Ctrl Pts',(-29.6693091154689,13.1970328357363,
129.237929001175)) ;
#130482=CARTESIAN_POINT('Ctrl Pts',(-29.685629423096,13.508431210418,129.252425328306)) ;
#130483=CARTESIAN_POINT('Ctrl Pts',(-29.6750927790816,13.8121186853756,
129.18865319137)) ;
#130484=CARTESIAN_POINT('Ctrl Pts',(-29.6389283245049,14.0900961116511,
129.049754658892)) ;
#130485=CARTESIAN_POINT('Ctrl Pts',(-29.5808923584998,14.3187298480659,
128.847179665827)) ;
#130486=CARTESIAN_POINT('Ctrl Pts',(-29.5050756594598,14.4844226501879,
128.592406122416)) ;
#130487=CARTESIAN_POINT('Ctrl Pts',(-29.4189800280682,14.5727758610145,
128.307951714936)) ;
#130488=CARTESIAN_POINT('Ctrl Pts',(-29.3282101502383,14.5796460652876,
128.00963807517)) ;
#130489=CARTESIAN_POINT('Ctrl Pts',(-29.2405915893346,14.5035866280562,
127.720582538253)) ;
#130490=CARTESIAN_POINT('Ctrl Pts',(-29.1627463131859,14.3497064261521,
127.459966008998)) ;
#130491=CARTESIAN_POINT('Ctrl Pts',(-29.1014315581632,14.1291331402223,
127.247667595512)) ;
#130492=CARTESIAN_POINT('Ctrl Pts',(-29.0617835084594,13.8597728320795,
127.098872760759)) ;
#130493=CARTESIAN_POINT('Ctrl Pts',(-29.0469138734206,13.5574625507345,
127.022250060698)) ;
#130494=CARTESIAN_POINT('Ctrl Pts',(-29.0589124808749,13.2463367213565,
127.024215607838)) ;
#130495=CARTESIAN_POINT('Ctrl Pts',(-29.0976581896989,12.9472974934633,
127.104242355792)) ;
#130496=CARTESIAN_POINT('Ctrl Pts',(-29.1607751106638,12.6832079210241,
127.255592028414)) ;
#130497=CARTESIAN_POINT('Ctrl Pts',(-29.2453851104306,12.4704983369195,
127.469462912104)) ;
#130498=CARTESIAN_POINT('Ctrl Pts',(-29.3447716639353,12.3276823761117,
127.726790304496)) ;
#130499=CARTESIAN_POINT('Ctrl Pts',(-29.4537157894357,12.2625925296001,
128.011876171548)) ;
#130500=CARTESIAN_POINT('Ctrl Pts',(-29.5643047349069,12.2806191987991,
128.301897217799)) ;
#130501=CARTESIAN_POINT('Ctrl Pts',(-29.6704487959945,12.3809214254249,
128.57871127182)) ;
#130502=CARTESIAN_POINT('Ctrl Pts',(-29.76412340717,12.5560400663307,128.819213425397)) ;
#130503=CARTESIAN_POINT('Ctrl Pts',(-29.8395060734412,12.7918900929914,
129.006436877495)) ;
#130504=CARTESIAN_POINT('Ctrl Pts',(-29.8926354306049,13.0744209302394,
129.128450455972)) ;
#130505=CARTESIAN_POINT('Ctrl Pts',(-29.9198456862715,13.3812416408414,
129.174838109595)) ;
#130506=CARTESIAN_POINT('Ctrl Pts',(-29.9200785827897,13.6920796910028,
129.14230522542)) ;
#130507=CARTESIAN_POINT('Ctrl Pts',(-29.8939694883016,13.9824941646698,
129.032937034259)) ;
#130508=CARTESIAN_POINT('Ctrl Pts',(-29.8445055241324,14.2323227439513,
128.855452218984)) ;
#130509=CARTESIAN_POINT('Ctrl Pts',(-29.7751603262968,14.4258243504284,
128.619628402019)) ;
#130510=CARTESIAN_POINT('Ctrl Pts',(-29.6924818729896,14.5465247241855,
128.345045148463)) ;
#130511=CARTESIAN_POINT('Ctrl Pts',(-29.6022812245865,14.5869806831231,
128.048301947459)) ;
#130512=CARTESIAN_POINT('Ctrl Pts',(-29.5129647804047,14.5442058467449,
127.754432704675)) ;
#130513=CARTESIAN_POINT('Ctrl Pts',(-29.4302326997558,14.4209679616749,
127.479549414334)) ;
#130514=CARTESIAN_POINT('Ctrl Pts',(-29.361544244752,14.2257906653135,127.245713957041)) ;
#130515=CARTESIAN_POINT('Ctrl Pts',(-29.3126320686624,13.9741287874761,
127.06978287009)) ;
#130516=CARTESIAN_POINT('Ctrl Pts',(-29.2873078566729,13.6829512743861,
126.962726744081)) ;
#130517=CARTESIAN_POINT('Ctrl Pts',(-29.2883658599329,13.3714665722058,
126.9325602086)) ;
#130518=CARTESIAN_POINT('Ctrl Pts',(-29.3163871008899,13.0656059038766,
126.981368852155)) ;
#130519=CARTESIAN_POINT('Ctrl Pts',(-29.3699746758538,12.7850335054103,
127.104838856256)) ;
#130520=CARTESIAN_POINT('Ctrl Pts',(-29.4462187184721,12.54966734435,127.294443632792)) ;
#130521=CARTESIAN_POINT('Ctrl Pts',(-29.5405084491528,12.3766688899815,
127.536703010351)) ;
#130522=CARTESIAN_POINT('Ctrl Pts',(-29.6465183988453,12.2789529397111,
127.813246121849)) ;
#130523=CARTESIAN_POINT('Ctrl Pts',(-29.7575529820162,12.2634413447035,
128.104442432783)) ;
#130524=CARTESIAN_POINT('Ctrl Pts',(-29.8658142138442,12.3304156583785,
128.387703279497)) ;
#130525=CARTESIAN_POINT('Ctrl Pts',(-29.9657429019495,12.477034323666,128.646289139449)) ;
#130526=CARTESIAN_POINT('Ctrl Pts',(-30.04889523573,12.6896429302191,128.856241956516)) ;
#130527=CARTESIAN_POINT('Ctrl Pts',(-30.1115928889291,12.9554490393123,
129.006277363579)) ;
#130528=CARTESIAN_POINT('Ctrl Pts',(-30.1495545265171,13.2546654169279,
129.08407484375)) ;
#130529=CARTESIAN_POINT('Ctrl Pts',(-30.160795972007,13.5672373629207,129.08367315207)) ;
#130530=CARTESIAN_POINT('Ctrl Pts',(-30.1452246339684,13.867352650113,129.005175262755)) ;
#130531=CARTESIAN_POINT('Ctrl Pts',(-30.1048447842729,14.1367234867938,
128.854116866161)) ;
#130532=CARTESIAN_POINT('Ctrl Pts',(-30.042556700534,14.3561275745404,128.638823326171)) ;
#130533=CARTESIAN_POINT('Ctrl Pts',(-29.9649745078786,14.5065131149989,
128.379260463449)) ;
#130534=CARTESIAN_POINT('Ctrl Pts',(-29.8769584255218,14.5806176797064,
128.088948707526)) ;
#130535=CARTESIAN_POINT('Ctrl Pts',(-29.7864336038671,14.5715967155624,
127.791445629283)) ;
#130536=CARTESIAN_POINT('Ctrl Pts',(-29.69982662067,14.4799161202559,127.505198050496)) ;
#130537=CARTESIAN_POINT('Ctrl Pts',(-29.6249930783652,14.3130126833991,
127.253530278741)) ;
#130538=CARTESIAN_POINT('Ctrl Pts',(-29.5674004888477,14.0821692542283,
127.052156703191)) ;
#130539=CARTESIAN_POINT('Ctrl Pts',(-29.5320652904142,13.8046646113754,
126.915868687298)) ;
#130540=CARTESIAN_POINT('Ctrl Pts',(-29.522245757931,13.4979411637468,126.85390767621)) ;
#130541=CARTESIAN_POINT('Ctrl Pts',(-29.5392765293126,13.1889484555023,
126.870727175006)) ;
#130542=CARTESIAN_POINT('Ctrl Pts',(-29.5829152948127,12.8939178939325,
126.964964143682)) ;
#130543=CARTESIAN_POINT('Ctrl Pts',(-29.6506193843243,12.6378239616322,
127.129606070988)) ;
#130544=CARTESIAN_POINT('Ctrl Pts',(-29.738152535917,12.4382802323548,127.352204897437)) ;
#130545=CARTESIAN_POINT('Ctrl Pts',(-29.8397245266592,12.3092349725469,
127.615912819609)) ;
#130546=CARTESIAN_POINT('Ctrl Pts',(-29.9500722254853,12.2595575244022,
127.904963057869)) ;
#130547=CARTESIAN_POINT('Ctrl Pts',(-30.0599627030921,12.2934341290355,
128.193023554747)) ;
#130548=CARTESIAN_POINT('Ctrl Pts',(-30.1640305325771,12.4080333821748,
128.463876290564)) ;
#130549=CARTESIAN_POINT('Ctrl Pts',(-30.254996316276,12.5960960444092,128.696398341662)) ;
#130550=CARTESIAN_POINT('Ctrl Pts',(-30.3266379956478,12.8430835986194,
128.872552220836)) ;
#130551=CARTESIAN_POINT('Ctrl Pts',(-30.3747931066949,13.1299282695534,
128.980268604815)) ;
#130552=CARTESIAN_POINT('Ctrl Pts',(-30.3971261320801,13.4413370794651,
129.012154398595)) ;
#130553=CARTESIAN_POINT('Ctrl Pts',(-30.3922326048791,13.7480777708716,
128.96487811748)) ;
#130554=CARTESIAN_POINT('Ctrl Pts',(-30.3615407807411,14.0327532731281,
128.842104048057)) ;
#130555=CARTESIAN_POINT('Ctrl Pts',(-30.3079642325184,14.2736050674125,
128.652532725912)) ;
#130556=CARTESIAN_POINT('Ctrl Pts',(-30.2353404472758,14.4547314005176,
128.407048833985)) ;
#130557=CARTESIAN_POINT('Ctrl Pts',(-30.1511026849128,14.560267557326,128.128030852945)) ;
#130558=CARTESIAN_POINT('Ctrl Pts',(-30.0604947582532,14.5853381835963,
127.830140097985)) ;
#130559=CARTESIAN_POINT('Ctrl Pts',(-29.9715942466692,14.5268296207526,
127.537332693561)) ;
#130560=CARTESIAN_POINT('Ctrl Pts',(-29.8911967366192,14.3893358191871,
127.269338442133)) ;
#130561=CARTESIAN_POINT('Ctrl Pts',(-29.8258710176355,14.1825587760216,
127.045374761125)) ;
#130562=CARTESIAN_POINT('Ctrl Pts',(-29.7809873413325,13.9213689273391,
126.881125929181)) ;
#130563=CARTESIAN_POINT('Ctrl Pts',(-29.7605871063278,13.624244891243,126.788376072781)) ;
#130564=CARTESIAN_POINT('Ctrl Pts',(-29.7665958590195,13.3143405109537,
126.772954857604)) ;
#130565=CARTESIAN_POINT('Ctrl Pts',(-29.7999614019313,13.0084391813705,
126.837014109222)) ;
#130566=CARTESIAN_POINT('Ctrl Pts',(-29.8577439349117,12.7371910069822,
126.972993813021)) ;
#130567=CARTESIAN_POINT('Ctrl Pts',(-29.9380486306226,12.5114338941523,
127.174317241384)) ;
#130568=CARTESIAN_POINT('Ctrl Pts',(-30.0347895009958,12.3524150089363,
127.423845852049)) ;
#130569=CARTESIAN_POINT('Ctrl Pts',(-30.1423814173391,12.2696328223672,
127.704969894785)) ;
#130570=CARTESIAN_POINT('Ctrl Pts',(-30.2533143890773,12.2697667116298,
127.995941819015)) ;
#130571=CARTESIAN_POINT('Ctrl Pts',(-30.3606289089555,12.3522196481958,
128.276346153937)) ;
#130572=CARTESIAN_POINT('Ctrl Pts',(-30.4575418534214,12.5116176555494,
128.526307518704)) ;
#130573=CARTESIAN_POINT('Ctrl Pts',(-30.5375652450921,12.7360826079941,
128.726969342083)) ;
#130574=CARTESIAN_POINT('Ctrl Pts',(-30.5959763461482,13.0105745884039,
128.864397493548)) ;
#130575=CARTESIAN_POINT('Ctrl Pts',(-30.6289168911378,13.3146277352433,
128.927438637494)) ;
#130576=CARTESIAN_POINT('Ctrl Pts',(-30.6349932443909,13.6243830684314,
128.912226450868)) ;
#130577=CARTESIAN_POINT('Ctrl Pts',(-30.6145002172543,13.9217977302755,
128.819166633438)) ;
#130578=CARTESIAN_POINT('Ctrl Pts',(-30.5697865145131,14.182101761474,128.655530820559)) ;
#130579=CARTESIAN_POINT('Ctrl Pts',(-30.5043483601306,14.38941229378,128.431164790754)) ;
#130580=CARTESIAN_POINT('Ctrl Pts',(-30.4239598225637,14.5268848124279,
128.163207055914)) ;
#130581=CARTESIAN_POINT('Ctrl Pts',(-30.3349091733917,14.5852561632452,
127.869902527666)) ;
#130582=CARTESIAN_POINT('Ctrl Pts',(-30.2448016587935,14.5605921487245,
127.573667910456)) ;
#130583=CARTESIAN_POINT('Ctrl Pts',(-30.1599580712501,14.4542388685168,
127.292630282821)) ;
#130584=CARTESIAN_POINT('Ctrl Pts',(-30.0878192488777,14.2743936484204,
127.048803788339)) ;
#130585=CARTESIAN_POINT('Ctrl Pts',(-30.0338404841497,14.0316377347413,
126.857786097763)) ;
#130586=CARTESIAN_POINT('Ctrl Pts',(-30.0033296373907,13.748755621538,126.735765359026)) ;
#130587=CARTESIAN_POINT('Ctrl Pts',(-29.9985372111809,13.4387761369995,
126.688426657773)) ;
#130588=CARTESIAN_POINT('Ctrl Pts',(-30.0205594673105,13.1317846538023,
126.719892013202)) ;
#130589=CARTESIAN_POINT('Ctrl Pts',(-30.0693092770263,12.8410201849047,
126.828891131929)) ;
#130590=CARTESIAN_POINT('Ctrl Pts',(-30.1405833793293,12.5963885979045,
127.004236412401)) ;
#130591=CARTESIAN_POINT('Ctrl Pts',(-30.2312796308035,12.4083250169264,
127.236028455529)) ;
#130592=CARTESIAN_POINT('Ctrl Pts',(-30.335740326897,12.2932606250205,127.507907427166)) ;
#130593=CARTESIAN_POINT('Ctrl Pts',(-30.4455648003633,12.2596773195356,
127.795795732775)) ;
#130594=CARTESIAN_POINT('Ctrl Pts',(-30.5554887651398,12.3089369784701,
128.083738997651)) ;
#130595=CARTESIAN_POINT('Ctrl Pts',(-30.6576028767063,12.4384178929668,
128.348866404619)) ;
#130596=CARTESIAN_POINT('Ctrl Pts',(-30.7452784557848,12.6389284156292,
128.571788006726)) ;
#130597=CARTESIAN_POINT('Ctrl Pts',(-30.8125438621909,12.8936368315776,
128.735337806806)) ;
#130598=CARTESIAN_POINT('Ctrl Pts',(-30.8563542073147,13.189035253119,128.830024629578)) ;
#130599=CARTESIAN_POINT('Ctrl Pts',(-30.8733117963159,13.4997523048697,
128.846448825023)) ;
#130600=CARTESIAN_POINT('Ctrl Pts',(-30.8635035099321,13.80398082463,128.784788851022)) ;
#130601=CARTESIAN_POINT('Ctrl Pts',(-30.8281975796196,14.0820720991441,
128.648525909069)) ;
#130602=CARTESIAN_POINT('Ctrl Pts',(-30.7705950246315,14.3130040222785,
128.447121485095)) ;
#130603=CARTESIAN_POINT('Ctrl Pts',(-30.6955724619812,14.4800544799105,
128.194827012547)) ;
#130604=CARTESIAN_POINT('Ctrl Pts',(-30.6094796922681,14.5714591728311,
127.910278099775)) ;
#130605=CARTESIAN_POINT('Ctrl Pts',(-30.5182772146109,14.5804983969621,
127.610538709757)) ;
#130606=CARTESIAN_POINT('Ctrl Pts',(-30.4309086742145,14.5069052814483,
127.322370946456)) ;
#130607=CARTESIAN_POINT('Ctrl Pts',(-30.3527812954282,14.3557030567126,
127.060991610997)) ;
#130608=CARTESIAN_POINT('Ctrl Pts',(-30.290791764377,14.1367620675431,126.846684361694)) ;
#130609=CARTESIAN_POINT('Ctrl Pts',(-30.2503365492017,13.868069475113,126.695461101934)) ;
#130610=CARTESIAN_POINT('Ctrl Pts',(-30.2347621394633,13.5652243934133,
126.616661910851)) ;
#130611=CARTESIAN_POINT('Ctrl Pts',(-30.2459604354312,13.2558697743365,
126.616481401596)) ;
#130612=CARTESIAN_POINT('Ctrl Pts',(-30.2838897938117,12.9557647499979,
126.694089516615)) ;
#130613=CARTESIAN_POINT('Ctrl Pts',(-30.3465075080088,12.6900042913403,
126.843917515241)) ;
#130614=CARTESIAN_POINT('Ctrl Pts',(-30.4302612148162,12.4761056036643,
127.055401271101)) ;
#130615=CARTESIAN_POINT('Ctrl Pts',(-30.5298042611788,12.3304586966932,
127.313012046257)) ;
#130616=CARTESIAN_POINT('Ctrl Pts',(-30.6380631716033,12.2634381679405,
127.59626025709)) ;
#130617=CARTESIAN_POINT('Ctrl Pts',(-30.7489387888862,12.2788783439155,
127.887043779485)) ;
#130618=CARTESIAN_POINT('Ctrl Pts',(-30.8551974172725,12.3768659519767,
128.164231165451)) ;
#130619=CARTESIAN_POINT('Ctrl Pts',(-30.9493029249669,12.5495629773897,
128.406018950591)) ;
#130620=CARTESIAN_POINT('Ctrl Pts',(-31.0257192355162,12.7855771010426,
128.596039753622)) ;
#130621=CARTESIAN_POINT('Ctrl Pts',(-31.0791447785856,13.0654344689711,
128.719127640439)) ;
#130622=CARTESIAN_POINT('Ctrl Pts',(-31.10721979407,13.3720088898766,128.768014230976)) ;
#130623=CARTESIAN_POINT('Ctrl Pts',(-31.1082390144562,13.6824356605847,
128.737845756141)) ;
#130624=CARTESIAN_POINT('Ctrl Pts',(-31.0830160432829,13.9739144612511,
128.63106921161)) ;
#130625=CARTESIAN_POINT('Ctrl Pts',(-31.0337088291658,14.2268633656514,
128.453783206045)) ;
#130626=CARTESIAN_POINT('Ctrl Pts',(-30.9655242077267,14.4204385538483,
128.221677293176)) ;
#130627=CARTESIAN_POINT('Ctrl Pts',(-30.8824245353142,14.5445800995036,
127.94555557525)) ;
#130628=CARTESIAN_POINT('Ctrl Pts',(-30.7929153317515,14.5868220519023,
127.65106138528)) ;
#130629=CARTESIAN_POINT('Ctrl Pts',(-30.7033259864182,14.5468039096368,
127.356334978812)) ;
#130630=CARTESIAN_POINT('Ctrl Pts',(-30.6200169000235,14.4251034045477,
127.079648615156)) ;
#130631=CARTESIAN_POINT('Ctrl Pts',(-30.5511679459364,14.2325286601305,
126.845483441192)) ;
#130632=CARTESIAN_POINT('Ctrl Pts',(-30.5014922994488,13.9823226220566,
126.667300841302)) ;
#130633=CARTESIAN_POINT('Ctrl Pts',(-30.4754060797272,13.6900857926319,
126.55781575587)) ;
#130634=CARTESIAN_POINT('Ctrl Pts',(-30.4757515263436,13.3811330388435,
126.525818393865)) ;
#130635=CARTESIAN_POINT('Ctrl Pts',(-30.5029596486349,13.0742212515847,
126.572184425358)) ;
#130636=CARTESIAN_POINT('Ctrl Pts',(-30.5559456878785,12.7922256350364,
126.693851892319)) ;
#130637=CARTESIAN_POINT('Ctrl Pts',(-30.6318353087,12.5548594605115,126.882340820124)) ;
#130638=CARTESIAN_POINT('Ctrl Pts',(-30.7256332714889,12.3804086732527,
127.123208519804)) ;
#130639=CARTESIAN_POINT('Ctrl Pts',(-30.8308984098131,12.2809059933595,
127.397727950232)) ;
#130640=CARTESIAN_POINT('Ctrl Pts',(-30.9417668692838,12.2624888444475,
127.688477101505)) ;
#130641=CARTESIAN_POINT('Ctrl Pts',(-31.0508252577136,12.3276776788202,
127.973866698083)) ;
#130642=CARTESIAN_POINT('Ctrl Pts',(-31.1502685162055,12.4707928531316,
128.231326341888)) ;
#130643=CARTESIAN_POINT('Ctrl Pts',(-31.2345189994147,12.6823313434113,
128.444309921377)) ;
#130644=CARTESIAN_POINT('Ctrl Pts',(-31.2980256195684,12.9478030946643,
128.596611453119)) ;
#130645=CARTESIAN_POINT('Ctrl Pts',(-31.3366816217105,13.2466922642525,
128.676406435598)) ;
#130646=CARTESIAN_POINT('Ctrl Pts',(-31.348613489995,13.5583771774669,128.678110282587)) ;
#130647=CARTESIAN_POINT('Ctrl Pts',(-31.3338483463751,13.8592555730131,
128.601960259952)) ;
#130648=CARTESIAN_POINT('Ctrl Pts',(-31.2938314441516,14.130642447192,128.451821693927)) ;
#130649=CARTESIAN_POINT('Ctrl Pts',(-31.2328517776415,14.3493759206944,
128.240739607194)) ;
#130650=CARTESIAN_POINT('Ctrl Pts',(-31.1550554986113,14.5035317147663,
127.980260239585)) ;
#130651=CARTESIAN_POINT('Ctrl Pts',(-31.0673952128672,14.5795844939409,
127.691069205955)) ;
#130652=CARTESIAN_POINT('Ctrl Pts',(-30.9766712485968,14.5729335746648,
127.39291041864)) ;
#130653=CARTESIAN_POINT('Ctrl Pts',(-30.8901457754388,14.4838965301244,
127.10702428331)) ;
#130654=CARTESIAN_POINT('Ctrl Pts',(-30.814690482604,14.3187458157033,126.8534560206)) ;
#130655=CARTESIAN_POINT('Ctrl Pts',(-30.7566026297993,14.089767661644,126.65067853821)) ;
#130656=CARTESIAN_POINT('Ctrl Pts',(-30.7205507654139,13.8134083502436,
126.512294932625)) ;
#130657=CARTESIAN_POINT('Ctrl Pts',(-30.7099213905107,13.507393703558,126.447991813842)) ;
#130658=CARTESIAN_POINT('Ctrl Pts',(-30.7262164766661,13.1976577760434,
126.46259634103)) ;
#130659=CARTESIAN_POINT('Ctrl Pts',(-30.7689461273649,12.9027230155048,
126.554284830547)) ;
#130660=CARTESIAN_POINT('Ctrl Pts',(-30.8360682125386,12.6448108807206,
126.717171534774)) ;
#130661=CARTESIAN_POINT('Ctrl Pts',(-30.9228749815143,12.4434495892378,
126.937711355592)) ;
#130662=CARTESIAN_POINT('Ctrl Pts',(-31.0250861654557,12.3113759849424,
127.20298051609)) ;
#130663=CARTESIAN_POINT('Ctrl Pts',(-31.1341161240077,12.2599503304548,
127.488549607509)) ;
#130664=CARTESIAN_POINT('Ctrl Pts',(-31.2449686946706,12.2913693198197,
127.779152527576)) ;
#130665=CARTESIAN_POINT('Ctrl Pts',(-31.3490006777393,12.4038516007803,
128.049992695568)) ;
#130666=CARTESIAN_POINT('Ctrl Pts',(-31.4401686589773,12.589262648139,128.283203736203)) ;
#130667=CARTESIAN_POINT('Ctrl Pts',(-31.5125077640223,12.834296673012,128.461424138523)) ;
#130668=CARTESIAN_POINT('Ctrl Pts',(-31.5616695171324,13.122430570677,128.571832493846)) ;
#130669=CARTESIAN_POINT('Ctrl Pts',(-31.584572061778,13.4307504343076,128.60568665077)) ;
#130670=CARTESIAN_POINT('Ctrl Pts',(-31.5805716706129,13.7394115379672,
128.560850441774)) ;
#130671=CARTESIAN_POINT('Ctrl Pts',(-31.5505589696301,14.0250582462743,
128.440063952068)) ;
#130672=CARTESIAN_POINT('Ctrl Pts',(-31.4974778440457,14.267685746029,128.251885798625)) ;
#130673=CARTESIAN_POINT('Ctrl Pts',(-31.425639817206,14.4501343666904,128.008842210201)) ;
#130674=CARTESIAN_POINT('Ctrl Pts',(-31.3412464001568,14.5585281597601,
127.729196706468)) ;
#130675=CARTESIAN_POINT('Ctrl Pts',(-31.2509509298363,14.5857500281756,
127.432315546893)) ;
#130676=CARTESIAN_POINT('Ctrl Pts',(-31.1617583850195,14.5296138402308,
127.138599459681)) ;
#130677=CARTESIAN_POINT('Ctrl Pts',(-31.0810307993938,14.3940563949584,
126.869634324592)) ;
#130678=CARTESIAN_POINT('Ctrl Pts',(-31.015365639309,14.1896706789709,126.644769166929)) ;
#130679=CARTESIAN_POINT('Ctrl Pts',(-30.9697407804104,13.9296796265153,
126.478325815102)) ;
#130680=CARTESIAN_POINT('Ctrl Pts',(-30.9485581261753,13.632561455883,126.383213941901)) ;
#130681=CARTESIAN_POINT('Ctrl Pts',(-30.9539104538573,13.3229080728124,
126.365887442255)) ;
#130682=CARTESIAN_POINT('Ctrl Pts',(-30.9861601219692,13.0185267768755,
126.42692304573)) ;
#130683=CARTESIAN_POINT('Ctrl Pts',(-31.0436635658604,12.7436674784671,
126.561805226232)) ;
#130684=CARTESIAN_POINT('Ctrl Pts',(-31.1235774177391,12.516497959597,126.761971689529)) ;
#130685=CARTESIAN_POINT('Ctrl Pts',(-31.2195573192475,12.3560840678509,
127.009401681164)) ;
#130686=CARTESIAN_POINT('Ctrl Pts',(-31.3269550981851,12.2708854944156,
127.289950809879)) ;
#130687=CARTESIAN_POINT('Ctrl Pts',(-31.4377439150536,12.2685611985324,
127.580543137024)) ;
#130688=CARTESIAN_POINT('Ctrl Pts',(-31.5454598315593,12.3486009329829,
127.862068280233)) ;
#130689=CARTESIAN_POINT('Ctrl Pts',(-31.6431291831054,12.5069430119851,
128.114092641889)) ;
#130690=CARTESIAN_POINT('Ctrl Pts',(-31.7231801494414,12.7284058667927,
128.31504662471)) ;
#130691=CARTESIAN_POINT('Ctrl Pts',(-31.7824884513957,13.0024844630991,
128.454991776573)) ;
#130692=CARTESIAN_POINT('Ctrl Pts',(-31.8160995644744,13.3053155340302,
128.520072219864)) ;
#130693=CARTESIAN_POINT('Ctrl Pts',(-31.8229604762739,13.6156286046676,
128.507094948621)) ;
#130694=CARTESIAN_POINT('Ctrl Pts',(-31.8033478246911,13.9128849150777,
128.416718921952)) ;
#130695=CARTESIAN_POINT('Ctrl Pts',(-31.7589073492138,14.1766184698676,
128.253605928012)) ;
#130696=CARTESIAN_POINT('Ctrl Pts',(-31.6940252869537,14.3847398233907,
128.030954151065)) ;
#130697=CARTESIAN_POINT('Ctrl Pts',(-31.6142724237389,14.523836080727,127.764966919406)) ;
#130698=CARTESIAN_POINT('Ctrl Pts',(-31.5254919515761,14.5847742986496,
127.47249459861)) ;
#130699=CARTESIAN_POINT('Ctrl Pts',(-31.4349594358017,14.5623309512569,
127.174878551546)) ;
#130700=CARTESIAN_POINT('Ctrl Pts',(-31.3499799147985,14.4584178345544,
126.893505314748)) ;
#130701=CARTESIAN_POINT('Ctrl Pts',(-31.2771464293534,14.2791868966926,
126.647472840431)) ;
#130702=CARTESIAN_POINT('Ctrl Pts',(-31.2232355329482,14.0415187300811,
126.45712718632)) ;
#130703=CARTESIAN_POINT('Ctrl Pts',(-31.1915724331804,13.7564325475948,
126.33133935828)) ;
#130704=CARTESIAN_POINT('Ctrl Pts',(-31.1860350406004,13.4495648633329,
126.282136996625)) ;
#130705=CARTESIAN_POINT('Ctrl Pts',(-31.207465416303,13.139416785511,126.311549638386)) ;
#130706=CARTESIAN_POINT('Ctrl Pts',(-31.2549371688994,12.8508801252525,
126.417190090246)) ;
#130707=CARTESIAN_POINT('Ctrl Pts',(-31.3260883980019,12.6022770135179,
126.591874983273)) ;
#130708=CARTESIAN_POINT('Ctrl Pts',(-31.4162873476206,12.4127865766784,
126.822257067223)) ;
#130709=CARTESIAN_POINT('Ctrl Pts',(-31.5204129624464,12.2953916616204,
127.093162819959)) ;
#130710=CARTESIAN_POINT('Ctrl Pts',(-31.6303913905,12.2594835085984,127.381432512102)) ;
#130711=CARTESIAN_POINT('Ctrl Pts',(-31.7402120890356,12.3065006883116,
127.669135805987)) ;
#130712=CARTESIAN_POINT('Ctrl Pts',(-31.8423834591039,12.4331949818184,
127.934527475475)) ;
#130713=CARTESIAN_POINT('Ctrl Pts',(-31.9308910035952,12.6325250875222,
128.159756985898)) ;
#130714=CARTESIAN_POINT('Ctrl Pts',(-31.9986534951646,12.8854153645511,
128.324824636163)) ;
#130715=CARTESIAN_POINT('Ctrl Pts',(-32.0432416690704,13.1803566291491,
128.421740282294)) ;
#130716=CARTESIAN_POINT('Ctrl Pts',(-32.0609557105027,13.4893560631302,
128.440539890944)) ;
#130717=CARTESIAN_POINT('Ctrl Pts',(-32.0519920259812,13.7954469993451,
128.38120266347)) ;
#130718=CARTESIAN_POINT('Ctrl Pts',(-32.0172267567837,14.0751704523599,
128.246444081047)) ;
#130719=CARTESIAN_POINT('Ctrl Pts',(-31.9603465713458,14.3069079863902,
128.04724645239)) ;
#130720=CARTESIAN_POINT('Ctrl Pts',(-31.8858483293298,14.4762412630358,
127.796504873332)) ;
#130721=CARTESIAN_POINT('Ctrl Pts',(-31.7992735361296,14.5702449515651,
127.510285055868)) ;
#130722=CARTESIAN_POINT('Ctrl Pts',(-31.7089460812534,14.5813885782014,
127.213417952581)) ;
#130723=CARTESIAN_POINT('Ctrl Pts',(-31.6209134531669,14.5100797260329,
126.923132692913)) ;
#130724=CARTESIAN_POINT('Ctrl Pts',(-31.542314320007,14.3602445926638,126.660309566855)) ;
#130725=CARTESIAN_POINT('Ctrl Pts',(-31.4799830689848,14.1432533152037,
126.445071104613)) ;
#130726=CARTESIAN_POINT('Ctrl Pts',(-31.4390256574942,13.8766591291424,
126.292492402048)) ;
#130727=CARTESIAN_POINT('Ctrl Pts',(-31.4226243614274,13.5754713250829,
126.211380568243)) ;
#130728=CARTESIAN_POINT('Ctrl Pts',(-31.4330180261553,13.2645670010663,
126.208687793803)) ;
#130729=CARTESIAN_POINT('Ctrl Pts',(-31.4703430384628,12.9634278823174,
126.284481469812)) ;
#130730=CARTESIAN_POINT('Ctrl Pts',(-31.5321358860487,12.6972349900806,
126.431994498119)) ;
#130731=CARTESIAN_POINT('Ctrl Pts',(-31.6152291836202,12.481723120017,126.64158339994)) ;
#130732=CARTESIAN_POINT('Ctrl Pts',(-31.7143133014449,12.3338052298827,
126.897872583145)) ;
#130733=CARTESIAN_POINT('Ctrl Pts',(-31.8227437636715,12.2641456097446,
127.181516339519)) ;
#130734=CARTESIAN_POINT('Ctrl Pts',(-31.9335770129781,12.277353556164,127.472198089832)) ;
#130735=CARTESIAN_POINT('Ctrl Pts',(-32.0398281227222,12.3726334343567,
127.749447473408)) ;
#130736=CARTESIAN_POINT('Ctrl Pts',(-32.1345084762193,12.5434757962,127.992866694939)) ;
#130737=CARTESIAN_POINT('Ctrl Pts',(-32.2113206179641,12.7769497154647,
128.184156230134)) ;
#130738=CARTESIAN_POINT('Ctrl Pts',(-32.2657802289169,13.0568799295701,
128.31011632032)) ;
#130739=CARTESIAN_POINT('Ctrl Pts',(-32.2945922213593,13.3636449055978,
128.361095482394)) ;
#130740=CARTESIAN_POINT('Ctrl Pts',(-32.2963571044857,13.6733774156544,
128.333199277218)) ;
#130741=CARTESIAN_POINT('Ctrl Pts',(-32.271951381347,13.965438068356,128.228844280693)) ;
#130742=CARTESIAN_POINT('Ctrl Pts',(-32.2232530315277,14.2203012587836,
128.053289070133)) ;
#130743=CARTESIAN_POINT('Ctrl Pts',(-32.155372333444,14.4159470406951,127.82200217397)) ;
#130744=CARTESIAN_POINT('Ctrl Pts',(-32.0731102939308,14.5416943667992,
127.548530757984)) ;
#130745=CARTESIAN_POINT('Ctrl Pts',(-31.9833574865262,14.5869018903293,
127.253186867552)) ;
#130746=CARTESIAN_POINT('Ctrl Pts',(-31.8935389765681,14.5489491297832,
126.957740138225)) ;
#130747=CARTESIAN_POINT('Ctrl Pts',(-31.8102081714722,14.4300240433963,
126.681107926645)) ;
#130748=CARTESIAN_POINT('Ctrl Pts',(-31.7405903151456,14.2387296175427,
126.444572398836)) ;
#130749=CARTESIAN_POINT('Ctrl Pts',(-31.6904068259423,13.9899469029636,
126.264929854329)) ;
#130750=CARTESIAN_POINT('Ctrl Pts',(-31.6636696322021,13.7002922437487,
126.153725446933)) ;
#130751=CARTESIAN_POINT('Ctrl Pts',(-31.6630638330101,13.3909003280038,
126.118871837105)) ;
#130752=CARTESIAN_POINT('Ctrl Pts',(-31.68968990522,13.0819914624154,126.163364765764)) ;
#130753=CARTESIAN_POINT('Ctrl Pts',(-31.7418568854852,12.8000707590593,
126.282755069558)) ;
#130754=CARTESIAN_POINT('Ctrl Pts',(-31.816871195244,12.5616135129792,126.468774849614)) ;
#130755=CARTESIAN_POINT('Ctrl Pts',(-31.9103871654035,12.3844499171478,
126.708743358304)) ;
#130756=CARTESIAN_POINT('Ctrl Pts',(-32.0159352821582,12.2824628358376,
126.98393007406)) ;
#130757=CARTESIAN_POINT('Ctrl Pts',(-32.1261749285063,12.2618989558539,
127.27301807145)) ;
#130758=CARTESIAN_POINT('Ctrl Pts',(-32.2355321466552,12.3245801207235,
127.559239590374)) ;
#130759=CARTESIAN_POINT('Ctrl Pts',(-32.335338397919,12.4655889395947,127.817759618502)) ;
#130760=CARTESIAN_POINT('Ctrl Pts',(-32.4201013753358,12.6753257670411,
128.032242329175)) ;
#130761=CARTESIAN_POINT('Ctrl Pts',(-32.4842152329815,12.9389694466535,
128.186377249352)) ;
#130762=CARTESIAN_POINT('Ctrl Pts',(-32.5236900098666,13.2377440459955,
128.268495152112)) ;
#130763=CARTESIAN_POINT('Ctrl Pts',(-32.5364526740039,13.5478076708615,
128.272797762813)) ;
#130764=CARTESIAN_POINT('Ctrl Pts',(-32.5223947250415,13.8515134131997,
128.198467412285)) ;
#130765=CARTESIAN_POINT('Ctrl Pts',(-32.4831407710608,14.1231096251736,
128.050674414571)) ;
#130766=CARTESIAN_POINT('Ctrl Pts',(-32.4226347638806,14.3439545931311,
127.840915685831)) ;
#130767=CARTESIAN_POINT('Ctrl Pts',(-32.3454372578941,14.4998916589537,
127.58227442761)) ;
#130768=CARTESIAN_POINT('Ctrl Pts',(-32.2576768546008,14.5786386310749,
127.292673319528)) ;
#130769=CARTESIAN_POINT('Ctrl Pts',(-32.1669904917241,14.5742675213239,
126.9946475028)) ;
#130770=CARTESIAN_POINT('Ctrl Pts',(-32.0801842586365,14.4873447468798,
126.707909950738)) ;
#130771=CARTESIAN_POINT('Ctrl Pts',(-32.0045667910146,14.3247914484279,
126.453977737131)) ;
#130772=CARTESIAN_POINT('Ctrl Pts',(-31.9456990864337,14.0970302958978,
126.248838632102)) ;
#130773=CARTESIAN_POINT('Ctrl Pts',(-31.9089308570874,13.8204924579681,
126.108230614868)) ;
#130774=CARTESIAN_POINT('Ctrl Pts',(-31.8976597732386,13.5164550314446,
126.042218995313)) ;
#130775=CARTESIAN_POINT('Ctrl Pts',(-31.9131779382847,13.2060700526839,
126.054496803148)) ;
#130776=CARTESIAN_POINT('Ctrl Pts',(-31.9552445107061,12.9102233152311,
126.144229921165)) ;
#130777=CARTESIAN_POINT('Ctrl Pts',(-32.0218893865554,12.6507291998818,
126.305673327108)) ;
#130778=CARTESIAN_POINT('Ctrl Pts',(-32.1079190718772,12.448558591514,126.524068042123)) ;
#130779=CARTESIAN_POINT('Ctrl Pts',(-32.2092378807032,12.3145373927892,
126.78689226887)) ;
#130780=CARTESIAN_POINT('Ctrl Pts',(-32.3187653072149,12.2601564003865,
127.0737196005)) ;
#130781=CARTESIAN_POINT('Ctrl Pts',(-32.4296559654795,12.2893926143671,
127.364444314449)) ;
#130782=CARTESIAN_POINT('Ctrl Pts',(-32.5339447068146,12.399436637318,127.636048091739)) ;
#130783=CARTESIAN_POINT('Ctrl Pts',(-32.6259308163714,12.5839727968354,
127.871499758443)) ;
#130784=CARTESIAN_POINT('Ctrl Pts',(-32.6984702869464,12.8264918557582,
128.050463425862)) ;
#130785=CARTESIAN_POINT('Ctrl Pts',(-32.7484756801105,13.1141229255637,
128.163283725505)) ;
#130786=CARTESIAN_POINT('Ctrl Pts',(-32.7641874562103,13.3194868174309,
128.187142012586)) ;
#130787=CARTESIAN_POINT('Ctrl Pts',(-32.7676006247655,13.4222383333956,
128.186092009004)) ;
#130788=CARTESIAN_POINT('Ctrl Pts',(-11.2812798643659,13.1551399285885,
133.225361312885)) ;
#130789=CARTESIAN_POINT('Ctrl Pts',(-11.2820187647633,13.1489709609094,
133.226788867079)) ;
#130790=CARTESIAN_POINT('Ctrl Pts',(-11.2940725891313,13.0505878441039,
133.250318667877)) ;
#130791=CARTESIAN_POINT('Ctrl Pts',(-11.3268196692865,12.8648900473044,
133.323006215356)) ;
#130792=CARTESIAN_POINT('Ctrl Pts',(-11.3955581347561,12.6378996894465,
133.490786092827)) ;
#130793=CARTESIAN_POINT('Ctrl Pts',(-11.4818126038911,12.4661938442505,
133.709651137204)) ;
#130794=CARTESIAN_POINT('Ctrl Pts',(-11.5806418499012,12.3629468779938,
133.965082777503)) ;
#130795=CARTESIAN_POINT('Ctrl Pts',(-11.6840920756584,12.3360866578135,
134.234357728742)) ;
#130796=CARTESIAN_POINT('Ctrl Pts',(-11.7874232958009,12.3868467815327,
134.502988211751)) ;
#130797=CARTESIAN_POINT('Ctrl Pts',(-11.8826517586958,12.5118616193735,
134.748082512994)) ;
#130798=CARTESIAN_POINT('Ctrl Pts',(-11.9642364503466,12.7022376314793,
134.953268302114)) ;
#130799=CARTESIAN_POINT('Ctrl Pts',(-12.0268555159077,12.9442211340136,
135.103070944459)) ;
#130800=CARTESIAN_POINT('Ctrl Pts',(-12.0667868417897,13.2203922331636,
135.186606249474)) ;
#130801=CARTESIAN_POINT('Ctrl Pts',(-12.0819921567622,13.5109001041669,
135.197934267535)) ;
#130802=CARTESIAN_POINT('Ctrl Pts',(-12.0718871830781,13.7967277450532,
135.135125417403)) ;
#130803=CARTESIAN_POINT('Ctrl Pts',(-12.0382787552941,14.0531634695327,
135.003985075531)) ;
#130804=CARTESIAN_POINT('Ctrl Pts',(-11.984040511163,14.2659161102292,134.812412340654)) ;
#130805=CARTESIAN_POINT('Ctrl Pts',(-11.9138317313736,14.4182155312585,
134.574200139104)) ;
#130806=CARTESIAN_POINT('Ctrl Pts',(-11.8331828494072,14.4993926065239,
134.305392211434)) ;
#130807=CARTESIAN_POINT('Ctrl Pts',(-11.7490444838035,14.5030674016304,
134.026483130585)) ;
#130808=CARTESIAN_POINT('Ctrl Pts',(-11.6680809986179,14.4296658181567,
133.756898311423)) ;
#130809=CARTESIAN_POINT('Ctrl Pts',(-11.5965958202758,14.2842405620309,
133.514968656249)) ;
#130810=CARTESIAN_POINT('Ctrl Pts',(-11.5404239481228,14.0768885755418,
133.31772524141)) ;
#130811=CARTESIAN_POINT('Ctrl Pts',(-11.5044626643021,13.821937566696,133.179448820527)) ;
#130812=CARTESIAN_POINT('Ctrl Pts',(-11.492115437901,13.5404397832619,133.110400577556)) ;
#130813=CARTESIAN_POINT('Ctrl Pts',(-11.5046895368218,13.2491903771815,
133.113990718504)) ;
#130814=CARTESIAN_POINT('Ctrl Pts',(-11.5423996819585,12.9699188880577,
133.190943520196)) ;
#130815=CARTESIAN_POINT('Ctrl Pts',(-11.6027127193453,12.7245502986717,
133.33412175314)) ;
#130816=CARTESIAN_POINT('Ctrl Pts',(-11.6827307770101,12.5279694687298,
133.534676781188)) ;
#130817=CARTESIAN_POINT('Ctrl Pts',(-11.7767909409935,12.3961377043517,
133.7763823545)) ;
#130818=CARTESIAN_POINT('Ctrl Pts',(-11.8796482494039,12.3376103677892,
134.043626665423)) ;
#130819=CARTESIAN_POINT('Ctrl Pts',(-11.9835249356267,12.3569098529355,
134.314074542349)) ;
#130820=CARTESIAN_POINT('Ctrl Pts',(-12.0830151650733,12.452769019898,134.571498333322)) ;
#130821=CARTESIAN_POINT('Ctrl Pts',(-12.1707022339469,12.6179593573441,
134.794565234874)) ;
#130822=CARTESIAN_POINT('Ctrl Pts',(-12.2415306520725,12.8405880377693,
134.968374154773)) ;
#130823=CARTESIAN_POINT('Ctrl Pts',(-12.2912076318387,13.1065246421439,
135.080214865833)) ;
#130824=CARTESIAN_POINT('Ctrl Pts',(-12.3163775691246,13.3925179674891,
135.12078307657)) ;
#130825=CARTESIAN_POINT('Ctrl Pts',(-12.3166058496797,13.6819916651313,
135.088335546118)) ;
#130826=CARTESIAN_POINT('Ctrl Pts',(-12.2921472081091,13.9537242418059,
134.983669295533)) ;
#130827=CARTESIAN_POINT('Ctrl Pts',(-12.2457390773696,14.1863734291659,
134.815010882744)) ;
#130828=CARTESIAN_POINT('Ctrl Pts',(-12.1814800516644,14.3643807985693,
134.59423567404)) ;
#130829=CARTESIAN_POINT('Ctrl Pts',(-12.1044683457898,14.4754559850244,
134.336147922274)) ;
#130830=CARTESIAN_POINT('Ctrl Pts',(-12.0208090250937,14.5110246739577,
134.058551574174)) ;
#130831=CARTESIAN_POINT('Ctrl Pts',(-11.9378612224862,14.4687063588107,
133.783197368949)) ;
#130832=CARTESIAN_POINT('Ctrl Pts',(-11.8615647632541,14.3514018815055,
133.527145574601)) ;
#130833=CARTESIAN_POINT('Ctrl Pts',(-11.798502564401,14.1671964752596,133.309749293991)) ;
#130834=CARTESIAN_POINT('Ctrl Pts',(-11.754049052173,13.9308608041133,133.146872132253)) ;
#130835=CARTESIAN_POINT('Ctrl Pts',(-11.7316977644638,13.6570089999716,
133.048397750488)) ;
#130836=CARTESIAN_POINT('Ctrl Pts',(-11.7341180951435,13.3664659574419,
133.022308686926)) ;
#130837=CARTESIAN_POINT('Ctrl Pts',(-11.761720921654,13.0805681472547,133.069846022257)) ;
#130838=CARTESIAN_POINT('Ctrl Pts',(-11.8131936002259,12.8190539470386,
133.187112979174)) ;
#130839=CARTESIAN_POINT('Ctrl Pts',(-11.886092857491,12.5999338423892,133.366806137464)) ;
#130840=CARTESIAN_POINT('Ctrl Pts',(-11.9747587487869,12.4413957528131,
133.592859241921)) ;
#130841=CARTESIAN_POINT('Ctrl Pts',(-12.0748052338517,12.3520378265489,
133.85195165464)) ;
#130842=CARTESIAN_POINT('Ctrl Pts',(-12.1791704719716,12.339734386482,134.123710421306)) ;
#130843=CARTESIAN_POINT('Ctrl Pts',(-12.2811942198852,12.4049383167358,
134.388634754176)) ;
#130844=CARTESIAN_POINT('Ctrl Pts',(-12.3743104910804,12.5429634979505,
134.627548525017)) ;
#130845=CARTESIAN_POINT('Ctrl Pts',(-12.4527350962615,12.7443553986761,
134.823486021638)) ;
#130846=CARTESIAN_POINT('Ctrl Pts',(-12.5113245953194,12.9943521537239,
134.961502568807)) ;
#130847=CARTESIAN_POINT('Ctrl Pts',(-12.5466491191103,13.2741647768729,
135.031655728832)) ;
#130848=CARTESIAN_POINT('Ctrl Pts',(-12.557133530808,13.565720269456,135.029118946566)) ;
#130849=CARTESIAN_POINT('Ctrl Pts',(-12.5424084976818,13.8474315556546,
134.952884078473)) ;
#130850=CARTESIAN_POINT('Ctrl Pts',(-12.504658245782,14.0971649669908,134.809596596871)) ;
#130851=CARTESIAN_POINT('Ctrl Pts',(-12.4468015681524,14.3002122843455,
134.607345660129)) ;
#130852=CARTESIAN_POINT('Ctrl Pts',(-12.3740820116557,14.4394509674979,
134.361774496034)) ;
#130853=CARTESIAN_POINT('Ctrl Pts',(-12.2928286579386,14.5058688200503,
134.091445642351)) ;
#130854=CARTESIAN_POINT('Ctrl Pts',(-12.2085754911848,14.4952594831202,
133.812133112469)) ;
#130855=CARTESIAN_POINT('Ctrl Pts',(-12.1285286312613,14.4071576912799,
133.54505905862)) ;
#130856=CARTESIAN_POINT('Ctrl Pts',(-12.0595995840032,14.2488070341169,
133.310594609379)) ;
#130857=CARTESIAN_POINT('Ctrl Pts',(-12.007204001394,14.032332595662,133.124541926762)) ;
#130858=CARTESIAN_POINT('Ctrl Pts',(-11.9754518623539,13.7715185673777,
132.998664946929)) ;
#130859=CARTESIAN_POINT('Ctrl Pts',(-11.9676077024159,13.4849968555095,
132.942553623633)) ;
#130860=CARTESIAN_POINT('Ctrl Pts',(-11.9852141495617,13.1936954317484,
132.960744777079)) ;
#130861=CARTESIAN_POINT('Ctrl Pts',(-12.0270155274854,12.9217410981826,
133.049976934939)) ;
#130862=CARTESIAN_POINT('Ctrl Pts',(-12.0916442917843,12.6826993167214,
133.205531163459)) ;
#130863=CARTESIAN_POINT('Ctrl Pts',(-12.1748344849184,12.4976839220085,
133.415374259801)) ;
#130864=CARTESIAN_POINT('Ctrl Pts',(-12.2706003786281,12.3794711428103,
133.662174391645)) ;
#130865=CARTESIAN_POINT('Ctrl Pts',(-12.3744503899862,12.3351744196322,
133.932269165389)) ;
#130866=CARTESIAN_POINT('Ctrl Pts',(-12.4782650208009,12.3695012763354,
134.202412750315)) ;
#130867=CARTESIAN_POINT('Ctrl Pts',(-12.5754721648271,12.4786183736045,
134.453365352351)) ;
#130868=CARTESIAN_POINT('Ctrl Pts',(-12.6605578265862,12.6556201701116,
134.668788412585)) ;
#130869=CARTESIAN_POINT('Ctrl Pts',(-12.7278290779799,12.8885376957079,
134.832076052564)) ;
#130870=CARTESIAN_POINT('Ctrl Pts',(-12.7727942038789,13.1578672277872,
134.93044163856)) ;
#130871=CARTESIAN_POINT('Ctrl Pts',(-12.7935589960753,13.4488181058444,
134.957796140316)) ;
#130872=CARTESIAN_POINT('Ctrl Pts',(-12.7888443918457,13.7357351250712,
134.91097260511)) ;
#130873=CARTESIAN_POINT('Ctrl Pts',(-12.7602605916963,14.0000244154435,
134.794478626913)) ;
#130874=CARTESIAN_POINT('Ctrl Pts',(-12.7099141607957,14.2248063693443,
134.614145960045)) ;
#130875=CARTESIAN_POINT('Ctrl Pts',(-12.6428897963242,14.3907221531774,
134.385334239461)) ;
#130876=CARTESIAN_POINT('Ctrl Pts',(-12.5640447774941,14.4880878052934,
134.121834427977)) ;
#130877=CARTESIAN_POINT('Ctrl Pts',(-12.4802617689659,14.5090844515927,
133.844015139513)) ;
#130878=CARTESIAN_POINT('Ctrl Pts',(-12.3974642832698,14.4517331277302,
133.568827359843)) ;
#130879=CARTESIAN_POINT('Ctrl Pts',(-12.3236763447296,14.3213873494252,
133.320287858352)) ;
#130880=CARTESIAN_POINT('Ctrl Pts',(-12.2637347152158,14.1266126254878,
133.112060420808)) ;
#130881=CARTESIAN_POINT('Ctrl Pts',(-12.2229774667805,13.8801113803002,
132.959735466426)) ;
#130882=CARTESIAN_POINT('Ctrl Pts',(-12.2053838579744,13.6025840232108,
132.875302084043)) ;
#130883=CARTESIAN_POINT('Ctrl Pts',(-12.2124772397581,13.3122088978665,
132.862974191922)) ;
#130884=CARTESIAN_POINT('Ctrl Pts',(-12.2448145015933,13.0284665595888,
132.924236901387)) ;
#130885=CARTESIAN_POINT('Ctrl Pts',(-12.3005599019218,12.7739765033465,
133.053999198988)) ;
#130886=CARTESIAN_POINT('Ctrl Pts',(-12.3766445028271,12.5655228915478,
133.243117582921)) ;
#130887=CARTESIAN_POINT('Ctrl Pts',(-12.4681423855166,12.4188418488155,
133.47731500825)) ;
#130888=CARTESIAN_POINT('Ctrl Pts',(-12.5692422546882,12.3438198182334,
133.739584235759)) ;
#130889=CARTESIAN_POINT('Ctrl Pts',(-12.6740334889537,12.3461749880073,
134.012474638995)) ;
#130890=CARTESIAN_POINT('Ctrl Pts',(-12.7747162224539,12.4256199459212,
134.273532924423)) ;
#130891=CARTESIAN_POINT('Ctrl Pts',(-12.8655945356852,12.5766359900473,
134.505860328425)) ;
#130892=CARTESIAN_POINT('Ctrl Pts',(-12.9405208029623,12.7882864475543,
134.691614915467)) ;
#130893=CARTESIAN_POINT('Ctrl Pts',(-12.9949316879518,13.0452019382586,
134.817458837911)) ;
#130894=CARTESIAN_POINT('Ctrl Pts',(-13.025720643168,13.3293877258915,134.874271333741)) ;
#130895=CARTESIAN_POINT('Ctrl Pts',(-13.0313457796955,13.6204035856812,
134.857561997613)) ;
#130896=CARTESIAN_POINT('Ctrl Pts',(-13.0121238177563,13.8971496153171,
134.768280402699)) ;
#130897=CARTESIAN_POINT('Ctrl Pts',(-12.9702433337836,14.1397539052331,
134.612839445253)) ;
#130898=CARTESIAN_POINT('Ctrl Pts',(-12.9092683557999,14.3313464702874,
134.401559637406)) ;
#130899=CARTESIAN_POINT('Ctrl Pts',(-12.8346344667875,14.4574458616527,
134.150487900523)) ;
#130900=CARTESIAN_POINT('Ctrl Pts',(-12.7520232585293,14.5099723944026,
133.876034599555)) ;
#130901=CARTESIAN_POINT('Ctrl Pts',(-12.6680149991839,14.4843439695083,
133.597416296755)) ;
#130902=CARTESIAN_POINT('Ctrl Pts',(-12.5898605639027,14.3827749410654,
133.336012913517)) ;
#130903=CARTESIAN_POINT('Ctrl Pts',(-12.5235110131134,14.2124739950545,
133.109063094795)) ;
#130904=CARTESIAN_POINT('Ctrl Pts',(-12.47454385575,13.9855789386979,132.932891873958)) ;
#130905=CARTESIAN_POINT('Ctrl Pts',(-12.44718714331,13.7185805864342,132.819871229684)) ;
#130906=CARTESIAN_POINT('Ctrl Pts',(-12.4441083202369,13.4303185636673,
132.777757800251)) ;
#130907=CARTESIAN_POINT('Ctrl Pts',(-12.4662081675216,13.1417758325219,
132.809228396078)) ;
#130908=CARTESIAN_POINT('Ctrl Pts',(-12.5128438608682,12.8725286043858,
132.912265477798)) ;
#130909=CARTESIAN_POINT('Ctrl Pts',(-12.5811355936144,12.6435096258014,
133.078662360882)) ;
#130910=CARTESIAN_POINT('Ctrl Pts',(-12.6670557983815,12.4701546223289,
133.296533072804)) ;
#130911=CARTESIAN_POINT('Ctrl Pts',(-12.7650980875458,12.3650501876111,
133.549835459936)) ;
#130912=CARTESIAN_POINT('Ctrl Pts',(-12.8692895553206,12.3357586674927,
133.821013809302)) ;
#130913=CARTESIAN_POINT('Ctrl Pts',(-12.9722194636702,12.3843195509594,
134.088641190149)) ;
#130914=CARTESIAN_POINT('Ctrl Pts',(-13.0679235169665,12.5073666683789,
134.335069106556)) ;
#130915=CARTESIAN_POINT('Ctrl Pts',(-13.1498474421669,12.6958200369819,
134.541296314724)) ;
#130916=CARTESIAN_POINT('Ctrl Pts',(-13.2130846476701,12.9363649293222,
134.692916583502)) ;
#130917=CARTESIAN_POINT('Ctrl Pts',(-13.2537553284003,13.212046231595,134.778583028313)) ;
#130918=CARTESIAN_POINT('Ctrl Pts',(-13.2696867588976,13.5022481067603,
134.792052779991)) ;
#130919=CARTESIAN_POINT('Ctrl Pts',(-13.2603291226857,13.7884016128943,
134.731444216182)) ;
#130920=CARTESIAN_POINT('Ctrl Pts',(-13.2274358441086,14.045945075732,134.602400846472)) ;
#130921=CARTESIAN_POINT('Ctrl Pts',(-13.1734739345736,14.2610680704969,
134.41149155897)) ;
#130922=CARTESIAN_POINT('Ctrl Pts',(-13.1038966633744,14.4145624165552,
134.175255364668)) ;
#130923=CARTESIAN_POINT('Ctrl Pts',(-13.0234728088093,14.4980852125695,
133.907100960487)) ;
#130924=CARTESIAN_POINT('Ctrl Pts',(-12.939325995419,14.5041312739862,133.628163299805)) ;
#130925=CARTESIAN_POINT('Ctrl Pts',(-12.8580140805557,14.4326962339747,
133.357486536545)) ;
#130926=CARTESIAN_POINT('Ctrl Pts',(-12.7862358410937,14.289424830309,133.114743545619)) ;
#130927=CARTESIAN_POINT('Ctrl Pts',(-12.7294171395877,14.0826507854277,
132.915479459106)) ;
#130928=CARTESIAN_POINT('Ctrl Pts',(-12.6931113261045,13.8312291814697,
132.77650858526)) ;
#130929=CARTESIAN_POINT('Ctrl Pts',(-12.6798565616288,13.5479805821752,
132.704527307887)) ;
#130930=CARTESIAN_POINT('Ctrl Pts',(-12.6918329131031,13.2572981016289,
132.706442366543)) ;
#130931=CARTESIAN_POINT('Ctrl Pts',(-12.7286154648152,12.9781391944844,
132.780789668285)) ;
#130932=CARTESIAN_POINT('Ctrl Pts',(-12.788841308569,12.7298471383749,132.923457407859)) ;
#130933=CARTESIAN_POINT('Ctrl Pts',(-12.8678064119023,12.5331718510569,
133.121190067536)) ;
#130934=CARTESIAN_POINT('Ctrl Pts',(-12.9619860922532,12.3987050488903,
133.3630746114)) ;
#130935=CARTESIAN_POINT('Ctrl Pts',(-13.0641173669679,12.3381977133859,
133.628393862531)) ;
#130936=CARTESIAN_POINT('Ctrl Pts',(-13.1689636586994,12.3556285786372,
133.901368958815)) ;
#130937=CARTESIAN_POINT('Ctrl Pts',(-13.2676215267395,12.448498640132,134.156721062578)) ;
#130938=CARTESIAN_POINT('Ctrl Pts',(-13.3562794099848,12.6124651727369,
134.382428532808)) ;
#130939=CARTESIAN_POINT('Ctrl Pts',(-13.4274024159188,12.8330193864531,
134.55721035227)) ;
#130940=CARTESIAN_POINT('Ctrl Pts',(-13.4778657839761,13.0981216515098,
134.671314825157)) ;
#130941=CARTESIAN_POINT('Ctrl Pts',(-13.5037873702561,13.3840423616995,
134.714047923931)) ;
#130942=CARTESIAN_POINT('Ctrl Pts',(-13.5047230832927,13.6738043197191,
134.683656575562)) ;
#130943=CARTESIAN_POINT('Ctrl Pts',(-13.4810350619758,13.9458856450603,
134.581307831703)) ;
#130944=CARTESIAN_POINT('Ctrl Pts',(-13.4350850950003,14.1805609741337,
134.413888828413)) ;
#130945=CARTESIAN_POINT('Ctrl Pts',(-13.3713435625267,14.3602096703021,
134.19466352274)) ;
#130946=CARTESIAN_POINT('Ctrl Pts',(-13.2941228668166,14.4737146563849,
133.935766751957)) ;
#130947=CARTESIAN_POINT('Ctrl Pts',(-13.2111150371913,14.510981736058,133.660304806086)) ;
#130948=CARTESIAN_POINT('Ctrl Pts',(-13.1279555516473,14.4710234538019,
133.384286573336)) ;
#130949=CARTESIAN_POINT('Ctrl Pts',(-13.0514607207591,14.3558611755068,
133.127695259553)) ;
#130950=CARTESIAN_POINT('Ctrl Pts',(-12.987929872837,14.1736059642118,132.908940703681)) ;
#130951=CARTESIAN_POINT('Ctrl Pts',(-12.9427874558613,13.9381264816024,
132.743987191645)) ;
#130952=CARTESIAN_POINT('Ctrl Pts',(-12.9198159126567,13.665192099168,132.643720985883)) ;
#130953=CARTESIAN_POINT('Ctrl Pts',(-12.9214159568252,13.3755914984187,
132.615321479283)) ;
#130954=CARTESIAN_POINT('Ctrl Pts',(-12.9485033871058,13.0874857506397,
132.661141600498)) ;
#130955=CARTESIAN_POINT('Ctrl Pts',(-12.9991534842726,12.8264337657975,
132.776172659393)) ;
#130956=CARTESIAN_POINT('Ctrl Pts',(-13.0712502877118,12.6060974389448,
132.953593799865)) ;
#130957=CARTESIAN_POINT('Ctrl Pts',(-13.1597261697062,12.4450313389733,
133.179001034814)) ;
#130958=CARTESIAN_POINT('Ctrl Pts',(-13.2598221399245,12.3534666197661,
133.438152169847)) ;
#130959=CARTESIAN_POINT('Ctrl Pts',(-13.3638496997786,12.3390029903486,
133.709021457282)) ;
#130960=CARTESIAN_POINT('Ctrl Pts',(-13.466268319613,12.4020392430349,133.975026492123)) ;
#130961=CARTESIAN_POINT('Ctrl Pts',(-13.5598211640111,12.5385711173323,
134.215165246668)) ;
#130962=CARTESIAN_POINT('Ctrl Pts',(-13.6383382505058,12.737337324062,134.411540597844)) ;
#130963=CARTESIAN_POINT('Ctrl Pts',(-13.6976697861643,12.9861206892308,
134.551707741949)) ;
#130964=CARTESIAN_POINT('Ctrl Pts',(-13.7337928936498,13.2660910782566,
134.62410596592)) ;
#130965=CARTESIAN_POINT('Ctrl Pts',(-13.7449404119012,13.5573227840952,
134.623538746113)) ;
#130966=CARTESIAN_POINT('Ctrl Pts',(-13.731057609949,13.8386952169897,134.549882879065)) ;
#130967=CARTESIAN_POINT('Ctrl Pts',(-13.6938267710482,14.0906007554108,
134.407982826979)) ;
#130968=CARTESIAN_POINT('Ctrl Pts',(-13.6366983945426,14.2945039762926,
134.207985282423)) ;
#130969=CARTESIAN_POINT('Ctrl Pts',(-13.5643971905334,14.4361574187858,
133.963631330981)) ;
#130970=CARTESIAN_POINT('Ctrl Pts',(-13.4829079562931,14.5051117570611,
133.692450855681)) ;
#130971=CARTESIAN_POINT('Ctrl Pts',(-13.398865589322,14.496582620466,133.413844416583)) ;
#130972=CARTESIAN_POINT('Ctrl Pts',(-13.3188758691256,14.4113394819302,
133.147064384826)) ;
#130973=CARTESIAN_POINT('Ctrl Pts',(-13.2492482094451,14.2546479447355,
132.910444808226)) ;
#130974=CARTESIAN_POINT('Ctrl Pts',(-13.1961963849046,14.039143877786,132.722400695126)) ;
#130975=CARTESIAN_POINT('Ctrl Pts',(-13.1638347550569,13.7793416572316,
132.594749383636)) ;
#130976=CARTESIAN_POINT('Ctrl Pts',(-13.1552775077889,13.4941095874199,
132.536650789137)) ;
#130977=CARTESIAN_POINT('Ctrl Pts',(-13.1720447629105,13.2026874966814,
132.552397812081)) ;
#130978=CARTESIAN_POINT('Ctrl Pts',(-13.2133004298939,12.928833346161,132.639904988231)) ;
#130979=CARTESIAN_POINT('Ctrl Pts',(-13.2774801251183,12.6885083712283,
132.794116581438)) ;
#130980=CARTESIAN_POINT('Ctrl Pts',(-13.3597053837363,12.5026390795781,
133.001327621254)) ;
#130981=CARTESIAN_POINT('Ctrl Pts',(-13.455701350823,12.3816810236162,133.248611444686)) ;
#130982=CARTESIAN_POINT('Ctrl Pts',(-13.5588450701788,12.3354826595071,
133.516837122875)) ;
#130983=CARTESIAN_POINT('Ctrl Pts',(-13.662986257812,12.3671988660942,133.787859387829)) ;
#130984=CARTESIAN_POINT('Ctrl Pts',(-13.7608857501055,12.4748749581507,
134.040689706046)) ;
#130985=CARTESIAN_POINT('Ctrl Pts',(-13.8461189502053,12.6498955190515,
134.256626571108)) ;
#130986=CARTESIAN_POINT('Ctrl Pts',(-13.9137641762851,12.8801431332148,
134.421162047123)) ;
#130987=CARTESIAN_POINT('Ctrl Pts',(-13.959688118663,13.1504415297617,134.52210348875)) ;
#130988=CARTESIAN_POINT('Ctrl Pts',(-13.9810355826832,13.438739202615,134.551438413197)) ;
#130989=CARTESIAN_POINT('Ctrl Pts',(-13.9771509252308,13.7280473502378,
134.50680820225)) ;
#130990=CARTESIAN_POINT('Ctrl Pts',(-13.9490883356948,13.9932362064335,
134.391820118097)) ;
#130991=CARTESIAN_POINT('Ctrl Pts',(-13.899552383743,14.2186783745982,134.213988401194)) ;
#130992=CARTESIAN_POINT('Ctrl Pts',(-13.8326088799132,14.3872014330787,
133.985246691092)) ;
#130993=CARTESIAN_POINT('Ctrl Pts',(-13.754354251272,14.486216521528,133.723625961275)) ;
#130994=CARTESIAN_POINT('Ctrl Pts',(-13.6703274653614,14.5095010567365,
133.444968044136)) ;
#130995=CARTESIAN_POINT('Ctrl Pts',(-13.587915515568,14.4548476689191,133.171125957688)) ;
#130996=CARTESIAN_POINT('Ctrl Pts',(-13.5132496102258,14.3259646517619,
132.919798090487)) ;
#130997=CARTESIAN_POINT('Ctrl Pts',(-13.4528381497739,14.1320240566172,
132.710133322283)) ;
#130998=CARTESIAN_POINT('Ctrl Pts',(-13.4117984923924,13.8890687487633,
132.557286539592)) ;
#130999=CARTESIAN_POINT('Ctrl Pts',(-13.3933038950219,13.6109288487181,
132.470050146704)) ;
#131000=CARTESIAN_POINT('Ctrl Pts',(-13.3996927101153,13.3205780973656,
132.455665139994)) ;
#131001=CARTESIAN_POINT('Ctrl Pts',(-13.4314451231204,13.0356410236252,
132.515132416829)) ;
#131002=CARTESIAN_POINT('Ctrl Pts',(-13.4863521726588,12.7811568557338,
132.642583088239)) ;
#131003=CARTESIAN_POINT('Ctrl Pts',(-13.5618719439237,12.5709851276515,
132.830045482527)) ;
#131004=CARTESIAN_POINT('Ctrl Pts',(-13.6530001533805,12.4221766619671,
133.063156221214)) ;
#131005=CARTESIAN_POINT('Ctrl Pts',(-13.7543438242653,12.3447406812541,
133.325997758698)) ;
#131006=CARTESIAN_POINT('Ctrl Pts',(-13.858979447707,12.3451621602759,133.598484050117)) ;
#131007=CARTESIAN_POINT('Ctrl Pts',(-13.9595871058779,12.4221617733591,
133.859413033911)) ;
#131008=CARTESIAN_POINT('Ctrl Pts',(-14.0509368702114,12.5713293574021,
134.093085140404)) ;
#131009=CARTESIAN_POINT('Ctrl Pts',(-14.1263288360547,12.7811357471148,
134.280239363245)) ;
#131010=CARTESIAN_POINT('Ctrl Pts',(-14.181464730297,13.037385413305,134.408146154191)) ;
#131011=CARTESIAN_POINT('Ctrl Pts',(-14.2129289597319,13.3202247802994,
134.46702998844)) ;
#131012=CARTESIAN_POINT('Ctrl Pts',(-14.2193168783918,13.6126649497902,
134.452393596522)) ;
#131013=CARTESIAN_POINT('Ctrl Pts',(-14.2008364796894,13.889109539137,134.365400616144)) ;
#131014=CARTESIAN_POINT('Ctrl Pts',(-14.1595000662705,14.1334576219234,
134.211477497111)) ;
#131015=CARTESIAN_POINT('Ctrl Pts',(-14.0992466494206,14.3262010857029,
134.002423062281)) ;
#131016=CARTESIAN_POINT('Ctrl Pts',(-14.0244678789738,14.4552702241494,
133.750713932904)) ;
#131017=CARTESIAN_POINT('Ctrl Pts',(-13.9418997721999,14.5094659873619,
133.476364746001)) ;
#131018=CARTESIAN_POINT('Ctrl Pts',(-13.8583861168424,14.48627928254,133.199410244325)) ;
#131019=CARTESIAN_POINT('Ctrl Pts',(-13.7797353567973,14.3867194330965,
132.936459435104)) ;
#131020=CARTESIAN_POINT('Ctrl Pts',(-13.7130105219871,14.2183273389604,
132.708437979387)) ;
#131021=CARTESIAN_POINT('Ctrl Pts',(-13.6633479068396,13.9922441011096,
132.530147180322)) ;
#131022=CARTESIAN_POINT('Ctrl Pts',(-13.6354328184579,13.7260908863955,
132.415503205816)) ;
#131023=CARTESIAN_POINT('Ctrl Pts',(-13.6315996421401,13.4392990683917,
132.371317925094)) ;
#131024=CARTESIAN_POINT('Ctrl Pts',(-13.6531002743803,13.1491383926391,
132.400878674979)) ;
#131025=CARTESIAN_POINT('Ctrl Pts',(-13.6988895423874,12.880138144259,132.501583429181)) ;
#131026=CARTESIAN_POINT('Ctrl Pts',(-13.7669016038619,12.6488312040692,
132.66702117208)) ;
#131027=CARTESIAN_POINT('Ctrl Pts',(-13.8519661020191,12.4746173052797,
132.882564533349)) ;
#131028=CARTESIAN_POINT('Ctrl Pts',(-13.9499918537797,12.3669410581914,
133.13572242046)) ;
#131029=CARTESIAN_POINT('Ctrl Pts',(-14.0540803057466,12.3355244467329,
133.406613758036)) ;
#131030=CARTESIAN_POINT('Ctrl Pts',(-14.1570770496498,12.3818824637266,
133.674448586604)) ;
#131031=CARTESIAN_POINT('Ctrl Pts',(-14.2529156063067,12.502442440452,133.921340780179)) ;
#131032=CARTESIAN_POINT('Ctrl Pts',(-14.3357164299663,12.6900860359651,
134.129966525958)) ;
#131033=CARTESIAN_POINT('Ctrl Pts',(-14.3993556473891,12.9290693621117,
134.282824648329)) ;
#131034=CARTESIAN_POINT('Ctrl Pts',(-14.4406746427025,13.2033802627449,
134.370454904131)) ;
#131035=CARTESIAN_POINT('Ctrl Pts',(-14.4573570221151,13.493885424346,134.386064394722)) ;
#131036=CARTESIAN_POINT('Ctrl Pts',(-14.4487939272164,13.7798208359641,
134.327863613174)) ;
#131037=CARTESIAN_POINT('Ctrl Pts',(-14.4163591296665,14.0398147256928,
134.199973199807)) ;
#131038=CARTESIAN_POINT('Ctrl Pts',(-14.3630430477874,14.2555980954836,
134.011057985321)) ;
#131039=CARTESIAN_POINT('Ctrl Pts',(-14.2938516112464,14.4112165057251,
133.775932908363)) ;
#131040=CARTESIAN_POINT('Ctrl Pts',(-14.213327419341,14.4969135755094,133.50736843725)) ;
#131041=CARTESIAN_POINT('Ctrl Pts',(-14.1296189321524,14.5049696810031,
133.229876903082)) ;
#131042=CARTESIAN_POINT('Ctrl Pts',(-14.0481698596881,14.4360249735447,
132.958821806314)) ;
#131043=CARTESIAN_POINT('Ctrl Pts',(-13.9759487851369,14.2945754362065,
132.714746600477)) ;
#131044=CARTESIAN_POINT('Ctrl Pts',(-13.9186392005941,14.0897548858671,
132.514089317548)) ;
#131045=CARTESIAN_POINT('Ctrl Pts',(-13.8816283734556,13.8387001375239,
132.372961040856)) ;
#131046=CARTESIAN_POINT('Ctrl Pts',(-13.86765973633,13.5574044598577,132.299056743724)) ;
#131047=CARTESIAN_POINT('Ctrl Pts',(-13.8789956043886,13.2644130009093,
132.2988381339)) ;
#131048=CARTESIAN_POINT('Ctrl Pts',(-13.9149994984909,12.9862195730077,
132.371090109727)) ;
#131049=CARTESIAN_POINT('Ctrl Pts',(-13.9743502243685,12.7371111819008,
132.511275565875)) ;
#131050=CARTESIAN_POINT('Ctrl Pts',(-14.0530557762854,12.5380203242925,
132.708138925323)) ;
#131051=CARTESIAN_POINT('Ctrl Pts',(-14.1469276806553,12.4015272632005,
132.949117652525)) ;
#131052=CARTESIAN_POINT('Ctrl Pts',(-14.2489833656644,12.3389470103484,
133.214189844898)) ;
#131053=CARTESIAN_POINT('Ctrl Pts',(-14.3533226131928,12.3537864997403,
133.485861761893)) ;
#131054=CARTESIAN_POINT('Ctrl Pts',(-14.4528614890508,12.4449099176858,
133.743576395913)) ;
#131055=CARTESIAN_POINT('Ctrl Pts',(-14.5418561425685,12.6072327563546,
133.97027761533)) ;
#131056=CARTESIAN_POINT('Ctrl Pts',(-14.6133813155202,12.8259751420657,
134.146289595912)) ;
#131057=CARTESIAN_POINT('Ctrl Pts',(-14.6644626717837,13.0894865209779,
134.262268329824)) ;
#131058=CARTESIAN_POINT('Ctrl Pts',(-14.6912354788188,13.3763086244584,
134.307339213758)) ;
#131059=CARTESIAN_POINT('Ctrl Pts',(-14.6927780845657,13.666102426872,134.278737035569)) ;
#131060=CARTESIAN_POINT('Ctrl Pts',(-14.6699098049705,13.9378774393092,
134.178922193569)) ;
#131061=CARTESIAN_POINT('Ctrl Pts',(-14.6244200591529,14.174793298913,134.012730262355)) ;
#131062=CARTESIAN_POINT('Ctrl Pts',(-14.5612019536203,14.355667987911,133.795095051057)) ;
#131063=CARTESIAN_POINT('Ctrl Pts',(-14.4846906294762,14.4711053294092,
133.538428577137)) ;
#131064=CARTESIAN_POINT('Ctrl Pts',(-14.4011850462511,14.511170979715,133.261273870169)) ;
#131065=CARTESIAN_POINT('Ctrl Pts',(-14.3178410780268,14.4729025341711,
132.984673903261)) ;
#131066=CARTESIAN_POINT('Ctrl Pts',(-14.2414431710577,14.3605014183323,
132.728538157581)) ;
#131067=CARTESIAN_POINT('Ctrl Pts',(-14.1770966200207,14.1789799497678,
132.507210107387)) ;
#131068=CARTESIAN_POINT('Ctrl Pts',(-14.1315848885081,13.9453130755044,
132.341277366815)) ;
#131069=CARTESIAN_POINT('Ctrl Pts',(-14.1079390036142,13.673613297581,132.239086339493)) ;
#131070=CARTESIAN_POINT('Ctrl Pts',(-14.1087830481224,13.3843416477693,
132.208491884339)) ;
#131071=CARTESIAN_POINT('Ctrl Pts',(-14.1351400941846,13.0956424787648,
132.252157038047)) ;
#131072=CARTESIAN_POINT('Ctrl Pts',(-14.1851403795369,12.8335787485534,
132.365283706234)) ;
#131073=CARTESIAN_POINT('Ctrl Pts',(-14.2566883427613,12.6116522531053,
132.541092961402)) ;
#131074=CARTESIAN_POINT('Ctrl Pts',(-14.3449178102994,12.4486058050818,
132.765728820733)) ;
#131075=CARTESIAN_POINT('Ctrl Pts',(-14.4444094609299,12.3551665981467,
133.023238128206)) ;
#131076=CARTESIAN_POINT('Ctrl Pts',(-14.5487260750023,12.3383111368361,
133.294844327139)) ;
#131077=CARTESIAN_POINT('Ctrl Pts',(-14.651135777708,12.3991318667188,133.560878201396)) ;
#131078=CARTESIAN_POINT('Ctrl Pts',(-14.7450247980916,12.5336133546432,
133.801997324254)) ;
#131079=CARTESIAN_POINT('Ctrl Pts',(-14.8240658891889,12.7304747525644,
133.999922781035)) ;
#131080=CARTESIAN_POINT('Ctrl Pts',(-14.8843591623108,12.9801493565206,
134.142645016146)) ;
#131081=CARTESIAN_POINT('Ctrl Pts',(-14.9207776314118,13.2569930870622,
134.216214669517)) ;
#131082=CARTESIAN_POINT('Ctrl Pts',(-14.9327904526555,13.5493201067258,
134.218039568247)) ;
#131083=CARTESIAN_POINT('Ctrl Pts',(-14.9195608823309,13.8310609228274,
134.146315593606)) ;
#131084=CARTESIAN_POINT('Ctrl Pts',(-14.8829071658904,14.0843638099265,
134.006060198745)) ;
#131085=CARTESIAN_POINT('Ctrl Pts',(-14.8262774665716,14.2896244491401,
133.807537482938)) ;
#131086=CARTESIAN_POINT('Ctrl Pts',(-14.7544509561564,14.4330063116879,
133.564623744753)) ;
#131087=CARTESIAN_POINT('Ctrl Pts',(-14.6730981695364,14.5042107415309,
133.293824015626)) ;
#131088=CARTESIAN_POINT('Ctrl Pts',(-14.5890044461905,14.4979449999679,
133.015056574469)) ;
#131089=CARTESIAN_POINT('Ctrl Pts',(-14.5085811345525,14.4144601779744,
132.746912885546)) ;
#131090=CARTESIAN_POINT('Ctrl Pts',(-14.4386966820867,14.2595209902124,
132.509575163383)) ;
#131091=CARTESIAN_POINT('Ctrl Pts',(-14.3852681727933,14.046214919979,132.32053362023)) ;
#131092=CARTESIAN_POINT('Ctrl Pts',(-14.3521879692475,13.7868053449528,
132.190703349274)) ;
#131093=CARTESIAN_POINT('Ctrl Pts',(-14.3429850788203,13.5027357390144,
132.130803960272)) ;
#131094=CARTESIAN_POINT('Ctrl Pts',(-14.3589256787532,13.2114164567146,
132.144166678592)) ;
#131095=CARTESIAN_POINT('Ctrl Pts',(-14.3996479591576,12.9359342983456,
132.230005501464)) ;
#131096=CARTESIAN_POINT('Ctrl Pts',(-14.4630310316759,12.6951562018299,
132.381999972268)) ;
#131097=CARTESIAN_POINT('Ctrl Pts',(-14.5447779273386,12.5073061272103,
132.587797294127)) ;
#131098=CARTESIAN_POINT('Ctrl Pts',(-14.6405874915994,12.3841592686752,
132.834495044115)) ;
#131099=CARTESIAN_POINT('Ctrl Pts',(-14.7436396651289,12.3356200239572,
133.102447533053)) ;
#131100=CARTESIAN_POINT('Ctrl Pts',(-14.8482334000072,12.3655842279676,
133.374661826652)) ;
#131101=CARTESIAN_POINT('Ctrl Pts',(-14.9456378863924,12.4702048591763,
133.62631542447)) ;
#131102=CARTESIAN_POINT('Ctrl Pts',(-15.032031341998,12.6448837976238,133.845354670619)) ;
#131103=CARTESIAN_POINT('Ctrl Pts',(-15.0997909854076,12.872508423284,134.010430965611)) ;
#131104=CARTESIAN_POINT('Ctrl Pts',(-15.1466624677231,13.1434988331289,
134.11394299587)) ;
#131105=CARTESIAN_POINT('Ctrl Pts',(-15.1684830221252,13.4301737780494,
134.144821454034)) ;
#131106=CARTESIAN_POINT('Ctrl Pts',(-15.1655029363779,13.7187795914099,
134.102960274335)) ;
#131107=CARTESIAN_POINT('Ctrl Pts',(-15.137871807278,13.9870154433738,133.988964277523)) ;
#131108=CARTESIAN_POINT('Ctrl Pts',(-15.089103500937,14.2124398345738,133.813561355081)) ;
#131109=CARTESIAN_POINT('Ctrl Pts',(-15.0226861816082,14.3830654461858,
133.586365342099)) ;
#131110=CARTESIAN_POINT('Ctrl Pts',(-14.9442977084689,14.4846609541733,
133.324197217531)) ;
#131111=CARTESIAN_POINT('Ctrl Pts',(-14.8603045751173,14.5097913616969,
133.045629352813)) ;
#131112=CARTESIAN_POINT('Ctrl Pts',(-14.7781158124174,14.4576093080194,
132.772584210679)) ;
#131113=CARTESIAN_POINT('Ctrl Pts',(-14.7029379087114,14.3304831317374,
132.519675058584)) ;
#131114=CARTESIAN_POINT('Ctrl Pts',(-14.6421746060609,14.1386183822934,
132.309056084948)) ;
#131115=CARTESIAN_POINT('Ctrl Pts',(-14.6004669656827,13.8965846856625,
132.154209706835)) ;
#131116=CARTESIAN_POINT('Ctrl Pts',(-14.5812880337956,13.6198365630073,
132.065057969682)) ;
#131117=CARTESIAN_POINT('Ctrl Pts',(-14.5869544254102,13.3288844737818,
132.048478781958)) ;
#131118=CARTESIAN_POINT('Ctrl Pts',(-14.6178077703533,13.0447399832046,
132.105475686592)) ;
#131119=CARTESIAN_POINT('Ctrl Pts',(-14.6721136258845,12.7881836368688,
132.231068090543)) ;
#131120=CARTESIAN_POINT('Ctrl Pts',(-14.7475386699193,12.5755910115287,
132.418091523374)) ;
#131121=CARTESIAN_POINT('Ctrl Pts',(-14.8378940236856,12.4257574465567,
132.649102005788)) ;
#131122=CARTESIAN_POINT('Ctrl Pts',(-14.9388209084364,12.3460112405744,
132.910787274949)) ;
#131123=CARTESIAN_POINT('Ctrl Pts',(-15.0435737078647,12.3439532504127,
133.183578235088)) ;
#131124=CARTESIAN_POINT('Ctrl Pts',(-15.1446091167616,12.4188218900739,
133.445686307793)) ;
#131125=CARTESIAN_POINT('Ctrl Pts',(-15.2365998734713,12.5668341062151,
133.681113263233)) ;
#131126=CARTESIAN_POINT('Ctrl Pts',(-15.3120455807105,12.7739565310488,
133.868616342754)) ;
#131127=CARTESIAN_POINT('Ctrl Pts',(-15.3679671650309,13.0292275295923,
133.998784482597)) ;
#131128=CARTESIAN_POINT('Ctrl Pts',(-15.4001513908772,13.3121167714202,
134.059708256056)) ;
#131129=CARTESIAN_POINT('Ctrl Pts',(-15.407302294284,13.6036711588795,134.047415072482)) ;
#131130=CARTESIAN_POINT('Ctrl Pts',(-15.3894117903854,13.8822010088686,
133.961971555951)) ;
#131131=CARTESIAN_POINT('Ctrl Pts',(-15.3488581880954,14.126534024312,133.810499271449)) ;
#131132=CARTESIAN_POINT('Ctrl Pts',(-15.2890058404676,14.3215277156221,
133.602541497692)) ;
#131133=CARTESIAN_POINT('Ctrl Pts',(-15.2146261037101,14.4523872469144,
133.352036701433)) ;
#131134=CARTESIAN_POINT('Ctrl Pts',(-15.132276398967,14.509081269933,133.078352393805)) ;
#131135=CARTESIAN_POINT('Ctrl Pts',(-15.048156334803,14.4877530584647,132.799404216537)) ;
#131136=CARTESIAN_POINT('Ctrl Pts',(-14.9697741972722,14.3906972492053,
132.537447195776)) ;
#131137=CARTESIAN_POINT('Ctrl Pts',(-14.9025432118204,14.2242127265294,
132.307919886886)) ;
#131138=CARTESIAN_POINT('Ctrl Pts',(-14.8524134830202,14.0000453961231,
132.128331876439)) ;
#131139=CARTESIAN_POINT('Ctrl Pts',(-14.8236827135926,13.7349941187306,
132.011308130338)) ;
#131140=CARTESIAN_POINT('Ctrl Pts',(-14.8192110157222,13.4462938086935,
131.964998461715)) ;
#131141=CARTESIAN_POINT('Ctrl Pts',(-14.8397608257614,13.1586524064852,
131.992109164985)) ;
#131142=CARTESIAN_POINT('Ctrl Pts',(-14.8852506544382,12.8863235925418,
132.091631205511)) ;
#131143=CARTESIAN_POINT('Ctrl Pts',(-14.952306886852,12.6553854575325,132.254505839022)) ;
#131144=CARTESIAN_POINT('Ctrl Pts',(-15.036993538522,12.4787538591612,132.468885463633)) ;
#131145=CARTESIAN_POINT('Ctrl Pts',(-15.1351325127102,12.3688114822916,
132.722256615459)) ;
#131146=CARTESIAN_POINT('Ctrl Pts',(-15.2387002100067,12.3354319136936,
132.991765834986)) ;
#131147=CARTESIAN_POINT('Ctrl Pts',(-15.3419020299315,12.3792576310417,
133.260178529464)) ;
#131148=CARTESIAN_POINT('Ctrl Pts',(-15.4385746866519,12.4988398999205,
133.509304414363)) ;
#131149=CARTESIAN_POINT('Ctrl Pts',(-15.5211785051019,12.6835118512005,
133.71760539492)) ;
#131150=CARTESIAN_POINT('Ctrl Pts',(-15.585614912484,12.9214923912795,133.872725040323)) ;
#131151=CARTESIAN_POINT('Ctrl Pts',(-15.6276593796861,13.1954916424955,
133.96242929729)) ;
#131152=CARTESIAN_POINT('Ctrl Pts',(-15.6450448286836,13.4865485670219,
133.980012149667)) ;
#131153=CARTESIAN_POINT('Ctrl Pts',(-15.6370948847114,13.772471589557,133.923647448758)) ;
#131154=CARTESIAN_POINT('Ctrl Pts',(-15.6054576941134,14.0322259092952,
133.798239163953)) ;
#131155=CARTESIAN_POINT('Ctrl Pts',(-15.5528532090993,14.2496185339524,
133.611440842472)) ;
#131156=CARTESIAN_POINT('Ctrl Pts',(-15.483617346609,14.4079186586772,133.375986031408)) ;
#131157=CARTESIAN_POINT('Ctrl Pts',(-15.4040148005417,14.495128940057,133.110405781656)) ;
#131158=CARTESIAN_POINT('Ctrl Pts',(-15.3198980850125,14.5060206783235,
132.831544484233)) ;
#131159=CARTESIAN_POINT('Ctrl Pts',(-15.2380342056834,14.4388851972431,
132.55918054693)) ;
#131160=CARTESIAN_POINT('Ctrl Pts',(-15.1654389797841,14.2990479598781,
132.313981427395)) ;
#131161=CARTESIAN_POINT('Ctrl Pts',(-15.107816605712,14.096277092635,132.112499036057)) ;
#131162=CARTESIAN_POINT('Ctrl Pts',(-15.0701124492741,13.8463552274942,
131.969338122834)) ;
#131163=CARTESIAN_POINT('Ctrl Pts',(-15.05554407707,13.5643762793268,131.893541407323)) ;
#131164=CARTESIAN_POINT('Ctrl Pts',(-15.0659585050918,13.2747380866486,
131.891020251149)) ;
#131165=CARTESIAN_POINT('Ctrl Pts',(-15.101446630055,12.9934296976024,131.961474427387)) ;
#131166=CARTESIAN_POINT('Ctrl Pts',(-15.1601039100246,12.7438068041656,
132.099715492444)) ;
#131167=CARTESIAN_POINT('Ctrl Pts',(-15.2384724882155,12.5426943442427,
132.295520501906)) ;
#131168=CARTESIAN_POINT('Ctrl Pts',(-15.3316626347415,12.4046936236787,
132.534630966333)) ;
#131169=CARTESIAN_POINT('Ctrl Pts',(-15.4337983976848,12.3396331759052,
132.799852893319)) ;
#131170=CARTESIAN_POINT('Ctrl Pts',(-15.5380451833256,12.3522550875064,
133.071297592341)) ;
#131171=CARTESIAN_POINT('Ctrl Pts',(-15.6378149553019,12.441158614988,133.329684714748)) ;
#131172=CARTESIAN_POINT('Ctrl Pts',(-15.7271824288003,12.6013769713038,
133.55749869446)) ;
#131173=CARTESIAN_POINT('Ctrl Pts',(-15.799387164279,12.819071640269,133.735430014399)) ;
#131174=CARTESIAN_POINT('Ctrl Pts',(-15.8509954325536,13.0807346140254,
133.853055281245)) ;
#131175=CARTESIAN_POINT('Ctrl Pts',(-15.8785701981475,13.3675408612144,
133.900413861765)) ;
#131176=CARTESIAN_POINT('Ctrl Pts',(-15.880950069095,13.6570979280699,133.874320504545)) ;
#131177=CARTESIAN_POINT('Ctrl Pts',(-15.8584614917164,13.9319893911641,
133.775308859387)) ;
#131178=CARTESIAN_POINT('Ctrl Pts',(-15.8140300794619,14.1676085258846,
133.612576918087)) ;
#131179=CARTESIAN_POINT('Ctrl Pts',(-15.7508365618172,14.3519029604138,
133.394745430706)) ;
#131180=CARTESIAN_POINT('Ctrl Pts',(-15.6747542377325,14.4687263868581,
133.139424327783)) ;
#131181=CARTESIAN_POINT('Ctrl Pts',(-15.5916310901521,14.5110206744739,
132.86348513324)) ;
#131182=CARTESIAN_POINT('Ctrl Pts',(-15.5082277554707,14.4754839101951,
132.586740900539)) ;
#131183=CARTESIAN_POINT('Ctrl Pts',(-15.4310148106346,14.3641243881349,
132.327975519891)) ;
#131184=CARTESIAN_POINT('Ctrl Pts',(-15.366796148105,14.1859981150162,132.10732571318)) ;
#131185=CARTESIAN_POINT('Ctrl Pts',(-15.3203690301936,13.9527739629267,
131.938549874937)) ;
#131186=CARTESIAN_POINT('Ctrl Pts',(-15.2960642034895,13.6818171869407,
131.83443758756)) ;
#131187=CARTESIAN_POINT('Ctrl Pts',(-15.2962284106988,13.3923456599437,
131.801803057666)) ;
#131188=CARTESIAN_POINT('Ctrl Pts',(-15.3217088635482,13.1044625348289,
131.843052348479)) ;
#131189=CARTESIAN_POINT('Ctrl Pts',(-15.3712895624886,12.8400820200563,
131.954780479996)) ;
#131190=CARTESIAN_POINT('Ctrl Pts',(-15.4421215709794,12.6174283224968,
132.128595071256)) ;
#131191=CARTESIAN_POINT('Ctrl Pts',(-15.5300656767636,12.4521814963559,
132.352341736955)) ;
#131192=CARTESIAN_POINT('Ctrl Pts',(-15.6293654089259,12.3567835155047,
132.609283754024)) ;
#131193=CARTESIAN_POINT('Ctrl Pts',(-15.7333497867975,12.3377092271658,
132.880009523703)) ;
#131194=CARTESIAN_POINT('Ctrl Pts',(-15.8360089773108,12.3962076032604,
133.146742886939)) ;
#131195=CARTESIAN_POINT('Ctrl Pts',(-15.930453723468,12.5290432373042,133.389409066584)) ;
#131196=CARTESIAN_POINT('Ctrl Pts',(-16.009869584066,12.7244085230837,133.588441629327)) ;
#131197=CARTESIAN_POINT('Ctrl Pts',(-16.0704566796156,12.9709500550387,
133.732258312717)) ;
#131198=CARTESIAN_POINT('Ctrl Pts',(-16.1079755146477,13.2494402817627,
133.808760193825)) ;
#131199=CARTESIAN_POINT('Ctrl Pts',(-16.1205567949924,13.5418967084717,
133.812230503726)) ;
#131200=CARTESIAN_POINT('Ctrl Pts',(-16.1080660019669,13.8230883914708,
133.742789063125)) ;
#131201=CARTESIAN_POINT('Ctrl Pts',(-16.0720612901439,14.0775910910953,
133.604421793909)) ;
#131202=CARTESIAN_POINT('Ctrl Pts',(-16.016031312662,14.2842118886259,133.407692540579)) ;
#131203=CARTESIAN_POINT('Ctrl Pts',(-15.9444811188164,14.4299775435325,
133.165534218954)) ;
#131204=CARTESIAN_POINT('Ctrl Pts',(-15.8629277653847,14.503331032243,132.894001914259)) ;
#131205=CARTESIAN_POINT('Ctrl Pts',(-15.7793496289803,14.4992417837061,
132.616952244808)) ;
#131206=CARTESIAN_POINT('Ctrl Pts',(-15.6984734089822,14.4177939822546,
132.347381532007)) ;
#131207=CARTESIAN_POINT('Ctrl Pts',(-15.6283650852396,14.2650806147523,
132.109470216545)) ;
#131208=CARTESIAN_POINT('Ctrl Pts',(-15.5743268050137,14.0529681509037,
131.918590385591)) ;
#131209=CARTESIAN_POINT('Ctrl Pts',(-15.5406403700371,13.7955270319932,
131.787101135372)) ;
#131210=CARTESIAN_POINT('Ctrl Pts',(-15.5306638256876,13.5095709535078,
131.724666349948)) ;
#131211=CARTESIAN_POINT('Ctrl Pts',(-15.5460171831695,13.2189036520177,
131.736403340103)) ;
#131212=CARTESIAN_POINT('Ctrl Pts',(-15.5859137154081,12.9437120966298,
131.819943466577)) ;
#131213=CARTESIAN_POINT('Ctrl Pts',(-15.6485475179313,12.7018113312773,
131.969792071976)) ;
#131214=CARTESIAN_POINT('Ctrl Pts',(-15.7301725881226,12.5115374792667,
132.175093619939)) ;
#131215=CARTESIAN_POINT('Ctrl Pts',(-15.8255194984171,12.3865362509785,
132.420501324227)) ;
#131216=CARTESIAN_POINT('Ctrl Pts',(-15.9289904176059,12.3360647683775,
132.689500393083)) ;
#131217=CARTESIAN_POINT('Ctrl Pts',(-16.0322109432962,12.3630945002041,
132.958176956719)) ;
#131218=CARTESIAN_POINT('Ctrl Pts',(-16.1310535797055,12.4665769548229,
133.213630713827)) ;
#131219=CARTESIAN_POINT('Ctrl Pts',(-16.2171162898203,12.637873730405,133.432016347732)) ;
#131220=CARTESIAN_POINT('Ctrl Pts',(-16.2861070614099,12.8661806742055,
133.600365416687)) ;
#131221=CARTESIAN_POINT('Ctrl Pts',(-16.3331577984964,13.1333277515124,
133.704775971435)) ;
#131222=CARTESIAN_POINT('Ctrl Pts',(-16.3560616077762,13.4221934836715,
133.738517459493)) ;
#131223=CARTESIAN_POINT('Ctrl Pts',(-16.3536937500244,13.7107571318464,
133.698487549138)) ;
#131224=CARTESIAN_POINT('Ctrl Pts',(-16.3267795290435,13.9798563780996,
133.58659147111)) ;
#131225=CARTESIAN_POINT('Ctrl Pts',(-16.2784408821239,14.2070905580459,
133.412375341533)) ;
#131226=CARTESIAN_POINT('Ctrl Pts',(-16.2125397227886,14.3790287482914,
133.186748864503)) ;
#131227=CARTESIAN_POINT('Ctrl Pts',(-16.1346594708171,14.4826462514907,
132.926162382995)) ;
#131228=CARTESIAN_POINT('Ctrl Pts',(-16.0504302213959,14.5101765749395,
132.646782279628)) ;
#131229=CARTESIAN_POINT('Ctrl Pts',(-15.9682674268405,14.4602521093363,
132.373878730922)) ;
#131230=CARTESIAN_POINT('Ctrl Pts',(-15.892694390541,14.3349863303821,132.119771873462)) ;
#131231=CARTESIAN_POINT('Ctrl Pts',(-15.8317129503708,14.1459036519263,
131.908681279387)) ;
#131232=CARTESIAN_POINT('Ctrl Pts',(-15.7891216920241,13.9042674567381,
131.751109063095)) ;
#131233=CARTESIAN_POINT('Ctrl Pts',(-15.7692741641614,13.6274934121279,
131.659929127433)) ;
#131234=CARTESIAN_POINT('Ctrl Pts',(-15.774240842792,13.3375401227482,131.641402457855)) ;
#131235=CARTESIAN_POINT('Ctrl Pts',(-15.8042482653973,13.0529656397982,
131.695949415826)) ;
#131236=CARTESIAN_POINT('Ctrl Pts',(-15.8584516986935,12.793542004979,131.820979830249)) ;
#131237=CARTESIAN_POINT('Ctrl Pts',(-15.9326864597706,12.5815361452067,
132.004842248444)) ;
#131238=CARTESIAN_POINT('Ctrl Pts',(-16.0230837910625,12.4287258471182,
132.235797836759)) ;
#131239=CARTESIAN_POINT('Ctrl Pts',(-16.1240643432101,12.3470719994747,
132.497574210549)) ;
#131240=CARTESIAN_POINT('Ctrl Pts',(-16.2285925774014,12.3430683223392,
132.769776197563)) ;
#131241=CARTESIAN_POINT('Ctrl Pts',(-16.3294552263757,12.4155936091128,
133.031491197843)) ;
#131242=CARTESIAN_POINT('Ctrl Pts',(-16.42158697565,12.5608875783812,133.267432939441)) ;
#131243=CARTESIAN_POINT('Ctrl Pts',(-16.4979791687381,12.7672957855937,
133.457539227448)) ;
#131244=CARTESIAN_POINT('Ctrl Pts',(-16.5545469684218,13.0219896288371,
133.589546147221)) ;
#131245=CARTESIAN_POINT('Ctrl Pts',(-16.5873216769804,13.3035436342973,
133.652289558074)) ;
#131246=CARTESIAN_POINT('Ctrl Pts',(-16.5952372158022,13.5948422510341,
133.642264450776)) ;
#131247=CARTESIAN_POINT('Ctrl Pts',(-16.5781262828345,13.8739529691167,
133.559117325056)) ;
#131248=CARTESIAN_POINT('Ctrl Pts',(-16.5380768677347,14.1203174233417,
133.409012301568)) ;
#131249=CARTESIAN_POINT('Ctrl Pts',(-16.4787184094645,14.3167168643634,
133.20251930448)) ;
#131250=CARTESIAN_POINT('Ctrl Pts',(-16.4048795075091,14.4494066861711,
132.953678390524)) ;
#131251=CARTESIAN_POINT('Ctrl Pts',(-16.3225697948458,14.5084702688582,
132.680063070833)) ;
#131252=CARTESIAN_POINT('Ctrl Pts',(-16.2386731326133,14.489700746972,132.401879914645)) ;
#131253=CARTESIAN_POINT('Ctrl Pts',(-16.159666302226,14.3946106074975,132.13794942029)) ;
#131254=CARTESIAN_POINT('Ctrl Pts',(-16.0919372674924,14.2294635345246,
131.906906848158)) ;
#131255=CARTESIAN_POINT('Ctrl Pts',(-16.0414142644033,14.0073333887475,
131.726263966149)) ;
#131256=CARTESIAN_POINT('Ctrl Pts',(-16.0120005571222,13.7435828448799,
131.607279354952)) ;
#131257=CARTESIAN_POINT('Ctrl Pts',(-16.0067413555039,13.454824745877,131.558621231445)) ;
#131258=CARTESIAN_POINT('Ctrl Pts',(-16.0266816029947,13.1663898496403,
131.58388276017)) ;
#131259=CARTESIAN_POINT('Ctrl Pts',(-16.071174096646,12.8948251888563,131.680693404511)) ;
#131260=CARTESIAN_POINT('Ctrl Pts',(-16.1378143759152,12.6613614393991,
131.842219614895)) ;
#131261=CARTESIAN_POINT('Ctrl Pts',(-16.2222899580583,12.4827884864443,
132.055914031115)) ;
#131262=CARTESIAN_POINT('Ctrl Pts',(-16.3195947643377,12.3713198999723,
132.307032186213)) ;
#131263=CARTESIAN_POINT('Ctrl Pts',(-16.42316155049,12.3351536539427,132.576506572357)) ;
#131264=CARTESIAN_POINT('Ctrl Pts',(-16.5269587087536,12.3771106003778,
132.846499102918)) ;
#131265=CARTESIAN_POINT('Ctrl Pts',(-16.6232634802675,12.493746042562,133.094781650953)) ;
#131266=CARTESIAN_POINT('Ctrl Pts',(-16.7066715515362,12.6767291405437,
133.30534152523)) ;
#131267=CARTESIAN_POINT('Ctrl Pts',(-16.7719969184263,12.9147362953278,
133.462888792416)) ;
#131268=CARTESIAN_POINT('Ctrl Pts',(-16.8145117924752,13.1870897175325,
133.554081812245)) ;
#131269=CARTESIAN_POINT('Ctrl Pts',(-16.832664410647,13.4771402294594,133.573993886311)) ;
#131270=CARTESIAN_POINT('Ctrl Pts',(-16.8255195547471,13.7642376991577,
133.519905575425)) ;
#131271=CARTESIAN_POINT('Ctrl Pts',(-16.7943070458963,14.0261140050281,
133.395578546783)) ;
#131272=CARTESIAN_POINT('Ctrl Pts',(-16.7424882598997,14.2437566095146,
133.211251228587)) ;
#131273=CARTESIAN_POINT('Ctrl Pts',(-16.6736113908412,14.4043004510961,
132.976804095223)) ;
#131274=CARTESIAN_POINT('Ctrl Pts',(-16.5942186823598,14.4936451763547,
132.711836822872)) ;
#131275=CARTESIAN_POINT('Ctrl Pts',(-16.5101466580755,14.5067755223083,
132.433108081231)) ;
#131276=CARTESIAN_POINT('Ctrl Pts',(-16.4282410882398,14.4421251633059,
132.160681842967)) ;
#131277=CARTESIAN_POINT('Ctrl Pts',(-16.3551632521983,14.3039891726026,
131.914003956164)) ;
#131278=CARTESIAN_POINT('Ctrl Pts',(-16.2972497108617,14.1040922169467,
131.711842779145)) ;
#131279=CARTESIAN_POINT('Ctrl Pts',(-16.2585983326173,13.8535852347893,
131.565668552377)) ;
#131280=CARTESIAN_POINT('Ctrl Pts',(-16.243420453165,13.5730952435811,131.488208101679)) ;
#131281=CARTESIAN_POINT('Ctrl Pts',(-16.2531006198612,13.2829861782011,
131.483481649537)) ;
#131282=CARTESIAN_POINT('Ctrl Pts',(-16.2877661805878,13.0017737284941,
131.551621835108)) ;
#131283=CARTESIAN_POINT('Ctrl Pts',(-16.3459738367156,12.7500890797144,
131.688431825914)) ;
#131284=CARTESIAN_POINT('Ctrl Pts',(-16.4238184818004,12.5475577998432,
131.882729415997)) ;
#131285=CARTESIAN_POINT('Ctrl Pts',(-16.5167586194788,12.4075652478031,
132.121078295711)) ;
#131286=CARTESIAN_POINT('Ctrl Pts',(-16.6183907518262,12.3405227377109,
132.384938789592)) ;
#131287=CARTESIAN_POINT('Ctrl Pts',(-16.7229364475564,12.3506975715296,
132.657173213167)) ;
#131288=CARTESIAN_POINT('Ctrl Pts',(-16.8232859030364,12.438177489278,132.917122022405)) ;
#131289=CARTESIAN_POINT('Ctrl Pts',(-16.9125712124386,12.5958827964123,
133.1448620791)) ;
#131290=CARTESIAN_POINT('Ctrl Pts',(-16.9854582743437,12.8123887822574,
133.324729525533)) ;
#131291=CARTESIAN_POINT('Ctrl Pts',(-17.037709893631,13.0732934241726,133.444215844693)) ;
#131292=CARTESIAN_POINT('Ctrl Pts',(-17.0659638164382,13.3601444544887,
133.493509177191)) ;
#131293=CARTESIAN_POINT('Ctrl Pts',(-17.0689675284249,13.6487324697402,
133.469363185352)) ;
#131294=CARTESIAN_POINT('Ctrl Pts',(-17.0474035047278,13.9231969052117,
133.37321432911)) ;
#131295=CARTESIAN_POINT('Ctrl Pts',(-17.0033733673897,14.1616648845749,
133.211459633651)) ;
#131296=CARTESIAN_POINT('Ctrl Pts',(-16.9406158991401,14.3474885130478,
132.994912465869)) ;
#131297=CARTESIAN_POINT('Ctrl Pts',(-16.864876505793,14.4664584587802,132.740606759249)) ;
#131298=CARTESIAN_POINT('Ctrl Pts',(-16.7814776117931,14.5109046603937,
132.463712586271)) ;
#131299=CARTESIAN_POINT('Ctrl Pts',(-16.6983907346783,14.477538406395,132.188050973166)) ;
#131300=CARTESIAN_POINT('Ctrl Pts',(-16.6207705482251,14.3681997132881,
131.928042842248)) ;
#131301=CARTESIAN_POINT('Ctrl Pts',(-16.5561356079281,14.19161807787,131.706168442298)) ;
#131302=CARTESIAN_POINT('Ctrl Pts',(-16.5092308734292,13.9603524956053,
131.536079167786)) ;
#131303=CARTESIAN_POINT('Ctrl Pts',(-16.4841796106604,13.6895220911817,
131.429699941359)) ;
#131304=CARTESIAN_POINT('Ctrl Pts',(-16.4836919093705,13.4007319641459,
131.395211960917)) ;
#131305=CARTESIAN_POINT('Ctrl Pts',(-16.5082964988508,13.1132078283894,
131.433992211526)) ;
#131306=CARTESIAN_POINT('Ctrl Pts',(-16.5574784700436,12.8466068578935,
131.544388229293)) ;
#131307=CARTESIAN_POINT('Ctrl Pts',(-16.6273997075169,12.6236984730367,
131.715716955648)) ;
#131308=CARTESIAN_POINT('Ctrl Pts',(-16.7150468521775,12.4561011970055,
131.938529922164)) ;
#131309=CARTESIAN_POINT('Ctrl Pts',(-16.8139682824648,12.3585968124196,
132.194412407875)) ;
#131310=CARTESIAN_POINT('Ctrl Pts',(-16.9182265147246,12.3371246735504,
132.465833558649)) ;
#131311=CARTESIAN_POINT('Ctrl Pts',(-17.0209026074425,12.3935413485491,
132.732653318412)) ;
#131312=CARTESIAN_POINT('Ctrl Pts',(-17.1153756443262,12.5236723848828,
132.975519307564)) ;
#131313=CARTESIAN_POINT('Ctrl Pts',(-17.1956555914022,12.7179304240541,
133.176947444366)) ;
#131314=CARTESIAN_POINT('Ctrl Pts',(-17.2569924030211,12.9643000603806,
133.322838842009)) ;
#131315=CARTESIAN_POINT('Ctrl Pts',(-17.2949538933717,13.2410161239663,
133.400773057716)) ;
#131316=CARTESIAN_POINT('Ctrl Pts',(-17.3083412632257,13.5320326358814,
133.40675253041)) ;
#131317=CARTESIAN_POINT('Ctrl Pts',(-17.2965889183178,13.8151976332958,
133.339306952295)) ;
#131318=CARTESIAN_POINT('Ctrl Pts',(-17.2611712342104,14.070965110173,133.202631251777)) ;
#131319=CARTESIAN_POINT('Ctrl Pts',(-17.2055219190199,14.2795161854134,
133.006946181317)) ;
#131320=CARTESIAN_POINT('Ctrl Pts',(-17.1344526197165,14.4266233568165,
132.766264881813)) ;
#131321=CARTESIAN_POINT('Ctrl Pts',(-17.0535835623515,14.5021444966585,
132.496922447555)) ;
#131322=CARTESIAN_POINT('Ctrl Pts',(-16.9693534559784,14.5004799279669,
132.217713549754)) ;
#131323=CARTESIAN_POINT('Ctrl Pts',(-16.8885085804287,14.4210758361391,
131.948320350664)) ;
#131324=CARTESIAN_POINT('Ctrl Pts',(-16.818249196986,14.2711637356508,131.710095463003)) ;
#131325=CARTESIAN_POINT('Ctrl Pts',(-16.7633840110066,14.0600320259714,
131.516677712646)) ;
#131326=CARTESIAN_POINT('Ctrl Pts',(-16.729034656478,13.8025046463563,131.383125760343)) ;
#131327=CARTESIAN_POINT('Ctrl Pts',(-16.7184105236858,13.5194350300881,
131.319077858953)) ;
#131328=CARTESIAN_POINT('Ctrl Pts',(-16.7329082611137,13.227929848522,131.328230796269)) ;
#131329=CARTESIAN_POINT('Ctrl Pts',(-16.7721540100418,12.9514279979351,
131.409809044102)) ;
#131330=CARTESIAN_POINT('Ctrl Pts',(-16.834426980546,12.7076270254922,131.558495828173)) ;
#131331=CARTESIAN_POINT('Ctrl Pts',(-16.9152315370478,12.5164543914562,
131.761543944961)) ;
#131332=CARTESIAN_POINT('Ctrl Pts',(-17.0104958015721,12.3891143889345,
132.006622580848)) ;
#131333=CARTESIAN_POINT('Ctrl Pts',(-17.1132917121907,12.3364756158918,
132.273826383176)) ;
#131334=CARTESIAN_POINT('Ctrl Pts',(-17.2173332534644,12.3612642231578,
132.54465957405)) ;
#131335=CARTESIAN_POINT('Ctrl Pts',(-17.3163641429157,12.4629838840005,
132.800676032605)) ;
#131336=CARTESIAN_POINT('Ctrl Pts',(-17.4026407183266,12.6321971699934,
133.01975282772)) ;
#131337=CARTESIAN_POINT('Ctrl Pts',(-17.472100457449,12.8584558798932,133.189548524182)) ;
#131338=CARTESIAN_POINT('Ctrl Pts',(-17.5200564206003,13.1261648647243,
133.296424663186)) ;
#131339=CARTESIAN_POINT('Ctrl Pts',(-17.5435329958318,13.4141234552309,
133.331916813786)) ;
#131340=CARTESIAN_POINT('Ctrl Pts',(-17.5418705107985,13.7023852342343,
133.294006470842)) ;
#131341=CARTESIAN_POINT('Ctrl Pts',(-17.515866367185,13.9714212012371,133.184910655295)) ;
#131342=CARTESIAN_POINT('Ctrl Pts',(-17.4677121548387,14.202020081249,133.01095053406)) ;
#131343=CARTESIAN_POINT('Ctrl Pts',(-17.4023716167183,14.3750071736422,
132.787065724901)) ;
#131344=CARTESIAN_POINT('Ctrl Pts',(-17.3247668097447,14.4806351346196,
132.527282453733)) ;
#131345=CARTESIAN_POINT('Ctrl Pts',(-17.2410054869792,14.5105855297535,
132.24943004058)) ;
#131346=CARTESIAN_POINT('Ctrl Pts',(-17.1581501091636,14.4625550657111,
131.974268906069)) ;
#131347=CARTESIAN_POINT('Ctrl Pts',(-17.0827332780509,14.3400369417443,
131.720826863696)) ;
#131348=CARTESIAN_POINT('Ctrl Pts',(-17.0209888868574,14.1521957535254,
131.507380128005)) ;
#131349=CARTESIAN_POINT('Ctrl Pts',(-16.9778207788142,13.9116489154345,
131.348115653949)) ;
#131350=CARTESIAN_POINT('Ctrl Pts',(-16.9572990580186,13.6358544266559,
131.25499330384)) ;
#131351=CARTESIAN_POINT('Ctrl Pts',(-16.9615071381463,13.3459427675745,
131.23424300822)) ;
#131352=CARTESIAN_POINT('Ctrl Pts',(-16.9909211180614,13.0604649745041,
131.286996740778)) ;
#131353=CARTESIAN_POINT('Ctrl Pts',(-17.0441007990242,12.8015143832803,
131.409241549806)) ;
#131354=CARTESIAN_POINT('Ctrl Pts',(-17.1180304186239,12.586871423154,131.592073079015)) ;
#131355=CARTESIAN_POINT('Ctrl Pts',(-17.2080500636742,12.4323032180318,
131.821934768459)) ;
#131356=CARTESIAN_POINT('Ctrl Pts',(-17.3084611337155,12.348604012381,132.082157360211)) ;
#131357=CARTESIAN_POINT('Ctrl Pts',(-17.4130111461555,12.3418345254331,
132.3544143668)) ;
#131358=CARTESIAN_POINT('Ctrl Pts',(-17.5146765749007,12.4127257697425,
132.618266949295)) ;
#131359=CARTESIAN_POINT('Ctrl Pts',(-17.606721170884,12.5554430365515,132.854114383774)) ;
#131360=CARTESIAN_POINT('Ctrl Pts',(-17.6839111619126,12.7608029240068,
133.046442139626)) ;
#131361=CARTESIAN_POINT('Ctrl Pts',(-17.7410331806284,13.0143079229722,
133.180091411217)) ;
#131362=CARTESIAN_POINT('Ctrl Pts',(-17.7745360164768,13.2953661026702,
133.244952941826)) ;
#131363=CARTESIAN_POINT('Ctrl Pts',(-17.7831520054483,13.587499191953,133.236886150184)) ;
#131364=CARTESIAN_POINT('Ctrl Pts',(-17.7666348632763,13.8669338626205,
133.155497022517)) ;
#131365=CARTESIAN_POINT('Ctrl Pts',(-17.7273863718362,14.1134263503453,
133.007875421063)) ;
#131366=CARTESIAN_POINT('Ctrl Pts',(-17.6683893078491,14.3121780897716,
132.802342611055)) ;
#131367=CARTESIAN_POINT('Ctrl Pts',(-17.5946147982464,14.4470050265316,
132.553591742459)) ;
#131368=CARTESIAN_POINT('Ctrl Pts',(-17.5125911040324,14.5078086325279,
132.280874384855)) ;
#131369=CARTESIAN_POINT('Ctrl Pts',(-17.4289255794743,14.4913412737729,
132.003473976216)) ;
#131370=CARTESIAN_POINT('Ctrl Pts',(-17.3497030184291,14.3985299043882,
131.738923406222)) ;
#131371=CARTESIAN_POINT('Ctrl Pts',(-17.2814947859058,14.2353764928408,
131.506472748856)) ;
#131372=CARTESIAN_POINT('Ctrl Pts',(-17.2301833982271,14.0132824388172,
131.32333677435)) ;
#131373=CARTESIAN_POINT('Ctrl Pts',(-17.2003726149901,13.751770584179,131.203370984278)) ;
#131374=CARTESIAN_POINT('Ctrl Pts',(-17.1942692410409,13.4639004603942,
131.15229798358)) ;
#131375=CARTESIAN_POINT('Ctrl Pts',(-17.2136563233809,13.1736259559936,
131.175755585428)) ;
#131376=CARTESIAN_POINT('Ctrl Pts',(-17.2572199771084,12.9029494351804,
131.270058586451)) ;
#131377=CARTESIAN_POINT('Ctrl Pts',(-17.3234518657098,12.6670694829694,
131.430263375814)) ;
#131378=CARTESIAN_POINT('Ctrl Pts',(-17.4076950363158,12.4867414535482,
131.643224441991)) ;
#131379=CARTESIAN_POINT('Ctrl Pts',(-17.5042594533731,12.3736046950475,
131.892333562312)) ;
#131380=CARTESIAN_POINT('Ctrl Pts',(-17.6083225797878,12.3351061359291,
132.163067552705)) ;
#131381=CARTESIAN_POINT('Ctrl Pts',(-17.7115102747659,12.3747297412366,
132.431506046747)) ;
#131382=CARTESIAN_POINT('Ctrl Pts',(-17.80835655534,12.4890530273647,132.681306942846)) ;
#131383=CARTESIAN_POINT('Ctrl Pts',(-17.8927139370083,12.6718473822343,
132.894413198474)) ;
#131384=CARTESIAN_POINT('Ctrl Pts',(-17.9581348743092,12.9071471042355,
133.05245843071)) ;
#131385=CARTESIAN_POINT('Ctrl Pts',(-18.0014489044881,13.1791583633753,
133.145922177929)) ;
#131386=CARTESIAN_POINT('Ctrl Pts',(-18.020261151911,13.4685703303894,133.16781609884)) ;
#131387=CARTESIAN_POINT('Ctrl Pts',(-18.0138792132709,13.7556865610863,
133.115998787948)) ;
#131388=CARTESIAN_POINT('Ctrl Pts',(-17.9834392562243,14.0184520779736,
132.993960277943)) ;
#131389=CARTESIAN_POINT('Ctrl Pts',(-17.9319093006337,14.2386835545227,
132.810307624848)) ;
#131390=CARTESIAN_POINT('Ctrl Pts',(-17.8634196060343,14.4009245247973,
132.577005577925)) ;
#131391=CARTESIAN_POINT('Ctrl Pts',(-17.7839956342627,14.4923209079493,
132.311848278652)) ;
#131392=CARTESIAN_POINT('Ctrl Pts',(-17.7003715420016,14.5074993821674,
132.034597515729)) ;
#131393=CARTESIAN_POINT('Ctrl Pts',(-17.6179715693461,14.4446391320812,
131.760580504429)) ;
#131394=CARTESIAN_POINT('Ctrl Pts',(-17.5449472629492,14.309013886893,131.514230915999)) ;
#131395=CARTESIAN_POINT('Ctrl Pts',(-17.4863929079662,14.1104149351794,
131.310125649846)) ;
#131396=CARTESIAN_POINT('Ctrl Pts',(-17.4472233098488,13.8614588559076,
131.162498832848)) ;
#131397=CARTESIAN_POINT('Ctrl Pts',(-17.4312869960412,13.5819687002437,
131.082859767227)) ;
#131398=CARTESIAN_POINT('Ctrl Pts',(-17.4402797073093,13.2906279013141,
131.075985151787)) ;
#131399=CARTESIAN_POINT('Ctrl Pts',(-17.4743143198391,13.009243305788,131.142317233284)) ;
#131400=CARTESIAN_POINT('Ctrl Pts',(-17.5315517099284,12.7575168112921,
131.276452625469)) ;
#131401=CARTESIAN_POINT('Ctrl Pts',(-17.6091410096472,12.5525240138587,
131.469879021206)) ;
#131402=CARTESIAN_POINT('Ctrl Pts',(-17.7014737885802,12.4108770336832,
131.706544893167)) ;
#131403=CARTESIAN_POINT('Ctrl Pts',(-17.8032831969416,12.3412909140522,
131.97080490142)) ;
#131404=CARTESIAN_POINT('Ctrl Pts',(-17.9077079735701,12.3493861735078,
132.242732393973)) ;
#131405=CARTESIAN_POINT('Ctrl Pts',(-18.0080021312736,12.4342727909203,
132.502613425746)) ;
#131406=CARTESIAN_POINT('Ctrl Pts',(-18.097851259794,12.5900489009072,132.731956223757)) ;
#131407=CARTESIAN_POINT('Ctrl Pts',(-18.1714811565311,12.8056265995217,
132.913906681068)) ;
#131408=CARTESIAN_POINT('Ctrl Pts',(-18.2242791522083,13.0653848746049,
133.035014327401)) ;
#131409=CARTESIAN_POINT('Ctrl Pts',(-18.2532373491338,13.3504851063388,
133.086511791274)) ;
#131410=CARTESIAN_POINT('Ctrl Pts',(-18.2570176970517,13.6412798147236,
133.064399324168)) ;
#131411=CARTESIAN_POINT('Ctrl Pts',(-18.2361288879767,13.915548156852,132.970331104728)) ;
#131412=CARTESIAN_POINT('Ctrl Pts',(-18.1927521468012,14.1552942040558,
132.810491998612)) ;
#131413=CARTESIAN_POINT('Ctrl Pts',(-18.1304889717146,14.3429101935435,
132.595396822877)) ;
#131414=CARTESIAN_POINT('Ctrl Pts',(-18.0549535994053,14.4639893047867,
132.341644352442)) ;
#131415=CARTESIAN_POINT('Ctrl Pts',(-17.9720169774795,14.5107279953385,
132.066239556179)) ;
#131416=CARTESIAN_POINT('Ctrl Pts',(-17.88839874123,14.4794893752074,131.788842595817)) ;
#131417=CARTESIAN_POINT('Ctrl Pts',(-17.8108656194136,14.3727211578977,
131.529246532274)) ;
#131418=CARTESIAN_POINT('Ctrl Pts',(-17.7456151211965,14.1977799584113,
131.305501822006)) ;
#131419=CARTESIAN_POINT('Ctrl Pts',(-17.6981151394564,13.9680803032242,
131.13369579038)) ;
#131420=CARTESIAN_POINT('Ctrl Pts',(-17.6723054333923,13.6967826933105,
131.024941140418)) ;
#131421=CARTESIAN_POINT('Ctrl Pts',(-17.6711447708163,13.4094043760888,
130.98862536116)) ;
#131422=CARTESIAN_POINT('Ctrl Pts',(-17.6950445630246,13.1212039321583,
131.025303143358)) ;
#131423=CARTESIAN_POINT('Ctrl Pts',(-17.74333311896,12.8546896237207,131.133221894845)) ;
#131424=CARTESIAN_POINT('Ctrl Pts',(-17.81282756458,12.6293810356165,131.303196900116)) ;
#131425=CARTESIAN_POINT('Ctrl Pts',(-17.9005194706817,12.4594635396626,
131.525988684649)) ;
#131426=CARTESIAN_POINT('Ctrl Pts',(-17.9986989569018,12.3604529302704,
131.779876218196)) ;
#131427=CARTESIAN_POINT('Ctrl Pts',(-18.1032340963646,12.3366695079855,
132.05199660503)) ;
#131428=CARTESIAN_POINT('Ctrl Pts',(-18.2056125319901,12.3907630606801,
132.318086056791)) ;
#131429=CARTESIAN_POINT('Ctrl Pts',(-18.300613364825,12.5187717527639,132.562441868016)) ;
#131430=CARTESIAN_POINT('Ctrl Pts',(-18.3816465085652,12.7125553045139,
132.765918032423)) ;
#131431=CARTESIAN_POINT('Ctrl Pts',(-18.4429853099616,12.9551208485313,
132.912159665352)) ;
#131432=CARTESIAN_POINT('Ctrl Pts',(-18.4820336765163,13.2325620060974,
132.993078593711)) ;
#131433=CARTESIAN_POINT('Ctrl Pts',(-18.496084383933,13.5243419796884,133.00090515124)) ;
#131434=CARTESIAN_POINT('Ctrl Pts',(-18.4850639350324,13.8069926528057,
132.935714610325)) ;
#131435=CARTESIAN_POINT('Ctrl Pts',(-18.4503367662865,14.0639000199269,
132.801056058483)) ;
#131436=CARTESIAN_POINT('Ctrl Pts',(-18.3952268191814,14.2741558930926,
132.606941700926)) ;
#131437=CARTESIAN_POINT('Ctrl Pts',(-18.3243680288223,14.4234615625839,
132.366801537788)) ;
#131438=CARTESIAN_POINT('Ctrl Pts',(-18.2437816042926,14.5011170686614,
132.098327447916)) ;
#131439=CARTESIAN_POINT('Ctrl Pts',(-18.1592384984199,14.5013614779113,
131.81807310291)) ;
#131440=CARTESIAN_POINT('Ctrl Pts',(-18.0789307375107,14.4249956630962,
131.550560960519)) ;
#131441=CARTESIAN_POINT('Ctrl Pts',(-18.0076541118125,14.2760171565871,
131.309082565097)) ;
#131442=CARTESIAN_POINT('Ctrl Pts',(-17.9524899575172,14.0665442400002,
131.114862544505)) ;
#131443=CARTESIAN_POINT('Ctrl Pts',(-17.9175014310239,13.8110528410318,
130.979547647309)) ;
#131444=CARTESIAN_POINT('Ctrl Pts',(-17.9061688391216,13.5262786463887,
130.913174372637)) ;
#131445=CARTESIAN_POINT('Ctrl Pts',(-17.919877948496,13.2368369901033,130.920277108179)) ;
#131446=CARTESIAN_POINT('Ctrl Pts',(-17.9586197277239,12.9583255903659,
131.000212959745)) ;
#131447=CARTESIAN_POINT('Ctrl Pts',(-18.0199083066583,12.7145800096232,
131.146219952724)) ;
#131448=CARTESIAN_POINT('Ctrl Pts',(-18.1009974511921,12.5201730384604,
131.349794172582)) ;
#131449=CARTESIAN_POINT('Ctrl Pts',(-18.1949562384929,12.392297716127,131.59141902566)) ;
#131450=CARTESIAN_POINT('Ctrl Pts',(-18.2981754606917,12.3368042043637,
131.859663996403)) ;
#131451=CARTESIAN_POINT('Ctrl Pts',(-18.4019398290045,12.3594079574846,
132.129799825424)) ;
#131452=CARTESIAN_POINT('Ctrl Pts',(-18.5013383418749,12.4588426243277,
132.386856715267)) ;
#131453=CARTESIAN_POINT('Ctrl Pts',(-18.5881323912535,12.6263832935465,
132.607414342136)) ;
#131454=CARTESIAN_POINT('Ctrl Pts',(-18.6581587702516,12.8513078071139,
132.778854814353)) ;
#131455=CARTESIAN_POINT('Ctrl Pts',(-18.7067345904951,13.1175341941134,
132.887608467018)) ;
#131456=CARTESIAN_POINT('Ctrl Pts',(-18.731003412201,13.4059954970849,132.925314381533)) ;
#131457=CARTESIAN_POINT('Ctrl Pts',(-18.7300968071152,13.6942419645787,
132.889656262388)) ;
#131458=CARTESIAN_POINT('Ctrl Pts',(-18.7044541735128,13.9656571359195,
132.781395875164)) ;
#131459=CARTESIAN_POINT('Ctrl Pts',(-18.6575265026644,14.1945698215837,
132.611470543872)) ;
#131460=CARTESIAN_POINT('Ctrl Pts',(-18.5922406519204,14.3711224528334,
132.387486886082)) ;
#131461=CARTESIAN_POINT('Ctrl Pts',(-18.5149037393986,14.4785950091488,
132.128508392993)) ;
#131462=CARTESIAN_POINT('Ctrl Pts',(-18.4311371510558,14.5108133112394,
131.850601957705)) ;
#131463=CARTESIAN_POINT('Ctrl Pts',(-18.3483146549276,14.4650394200622,
131.575598992863)) ;
#131464=CARTESIAN_POINT('Ctrl Pts',(-18.2726066198908,14.3446919400874,
131.321313280288)) ;
#131465=CARTESIAN_POINT('Ctrl Pts',(-18.2103307361537,14.1586507898245,
131.106307024848)) ;
#131466=CARTESIAN_POINT('Ctrl Pts',(-18.1664432390162,13.9182142591253,
130.944795156692)) ;
#131467=CARTESIAN_POINT('Ctrl Pts',(-18.1453636366719,13.6446894301756,
130.850233747273)) ;
#131468=CARTESIAN_POINT('Ctrl Pts',(-18.1488348343508,13.3538163555555,
130.82719813754)) ;
#131469=CARTESIAN_POINT('Ctrl Pts',(-18.1774811245967,13.0687529323482,
130.877811758373)) ;
#131470=CARTESIAN_POINT('Ctrl Pts',(-18.2300437642224,12.8084025711039,
130.998208929724)) ;
#131471=CARTESIAN_POINT('Ctrl Pts',(-18.3034001053734,12.5923662507696,
131.179384620874)) ;
#131472=CARTESIAN_POINT('Ctrl Pts',(-18.3931634370597,12.4355966936421,
131.408445657945)) ;
#131473=CARTESIAN_POINT('Ctrl Pts',(-18.4935575860177,12.3498834173245,
131.668562849344)) ;
#131474=CARTESIAN_POINT('Ctrl Pts',(-18.5975530541275,12.3409542808635,
131.939369081028)) ;
#131475=CARTESIAN_POINT('Ctrl Pts',(-18.6994673351223,12.4093757248112,
132.203931136602)) ;
#131476=CARTESIAN_POINT('Ctrl Pts',(-18.7921201529756,12.5505196315372,
132.441467645947)) ;
#131477=CARTESIAN_POINT('Ctrl Pts',(-18.8697017731338,12.7541803006072,
132.634971878383)) ;
#131478=CARTESIAN_POINT('Ctrl Pts',(-18.9273307484839,13.0055267425044,
132.770220733639)) ;
#131479=CARTESIAN_POINT('Ctrl Pts',(-18.9617100390982,13.2870724884799,
132.83751270461)) ;
#131480=CARTESIAN_POINT('Ctrl Pts',(-18.9710255677151,13.5781354317469,
132.831615285865)) ;
#131481=CARTESIAN_POINT('Ctrl Pts',(-18.9553578084607,13.8583662507443,
132.752702523973)) ;
#131482=CARTESIAN_POINT('Ctrl Pts',(-18.9165383575917,14.1072755060793,
132.606171710367)) ;
#131483=CARTESIAN_POINT('Ctrl Pts',(-18.8581587772242,14.3069765889331,
132.4025330216)) ;
#131484=CARTESIAN_POINT('Ctrl Pts',(-18.7850681968336,14.443614067786,132.155907192059)) ;
#131485=CARTESIAN_POINT('Ctrl Pts',(-18.702941141321,14.5071928082345,131.882773592227)) ;
#131486=CARTESIAN_POINT('Ctrl Pts',(-18.6190408117616,14.4928945220509,
131.604612881179)) ;
#131487=CARTESIAN_POINT('Ctrl Pts',(-18.5396187459799,14.4021254936154,
131.339485656911)) ;
#131488=CARTESIAN_POINT('Ctrl Pts',(-18.4711933901986,14.2413770477371,
131.106496569037)) ;
#131489=CARTESIAN_POINT('Ctrl Pts',(-18.4192605637911,14.0210258594474,
130.921552581758)) ;
#131490=CARTESIAN_POINT('Ctrl Pts',(-18.3886405960536,13.7594508415378,
130.799092122936)) ;
#131491=CARTESIAN_POINT('Ctrl Pts',(-18.381928462571,13.4716753030503,130.746210031867)) ;
#131492=CARTESIAN_POINT('Ctrl Pts',(-18.4004216312574,13.18278007244,130.767242888151)) ;
#131493=CARTESIAN_POINT('Ctrl Pts',(-18.4435339670258,12.9097866347109,
130.860039653288)) ;
#131494=CARTESIAN_POINT('Ctrl Pts',(-18.5088204983959,12.6739761120234,
131.017674750893)) ;
#131495=CARTESIAN_POINT('Ctrl Pts',(-18.5926770612546,12.4911376353209,
131.229439455072)) ;
#131496=CARTESIAN_POINT('Ctrl Pts',(-18.6895108158381,12.3755758788311,
131.479159592622)) ;
#131497=CARTESIAN_POINT('Ctrl Pts',(-18.7928542788589,12.3352662329562,
131.747989657394)) ;
#131498=CARTESIAN_POINT('Ctrl Pts',(-18.8962659376777,12.3722006143293,
132.017051741353)) ;
#131499=CARTESIAN_POINT('Ctrl Pts',(-18.9940984306609,12.4858118722087,
132.26946955847)) ;
#131500=CARTESIAN_POINT('Ctrl Pts',(-19.0779483654093,12.6649628027199,
132.481462828409)) ;
#131501=CARTESIAN_POINT('Ctrl Pts',(-19.144324386781,12.8995424291904,132.64216747859)) ;
#131502=CARTESIAN_POINT('Ctrl Pts',(-19.1882893988472,13.1707489990253,
132.73754255469)) ;
#131503=CARTESIAN_POINT('Ctrl Pts',(-19.2078747746244,13.4602465419289,
132.76165779285)) ;
#131504=CARTESIAN_POINT('Ctrl Pts',(-19.2021695943243,13.7479094104328,
132.711797460233)) ;
#131505=CARTESIAN_POINT('Ctrl Pts',(-19.1724541288044,14.0110933638022,
132.591943088721)) ;
#131506=CARTESIAN_POINT('Ctrl Pts',(-19.1214789970609,14.2330195298938,
132.409891780119)) ;
#131507=CARTESIAN_POINT('Ctrl Pts',(-19.0533824116154,14.397056415232,132.177734508543)) ;
#131508=CARTESIAN_POINT('Ctrl Pts',(-18.9744610193818,14.4906410938832,
131.914150162339)) ;
#131509=CARTESIAN_POINT('Ctrl Pts',(-18.890345578861,14.5080280130628,131.635247249356)) ;
#131510=CARTESIAN_POINT('Ctrl Pts',(-18.8085392860132,14.4480725424633,
131.363277720596)) ;
#131511=CARTESIAN_POINT('Ctrl Pts',(-18.7346273925197,14.3139470607326,
131.114108989611)) ;
#131512=CARTESIAN_POINT('Ctrl Pts',(-18.6756142626322,14.1169437524237,
130.908679443903)) ;
#131513=CARTESIAN_POINT('Ctrl Pts',(-18.6357563526766,13.8684682048696,
130.758950982595)) ;
#131514=CARTESIAN_POINT('Ctrl Pts',(-18.6192189361488,13.5907243651,130.677694418299)) ;
#131515=CARTESIAN_POINT('Ctrl Pts',(-18.6274186795787,13.2994062522709,
130.668497076563)) ;
#131516=CARTESIAN_POINT('Ctrl Pts',(-18.6607053713449,13.0173302811176,
130.732637587237)) ;
#131517=CARTESIAN_POINT('Ctrl Pts',(-18.7175745221499,12.7634586998748,
130.865557336184)) ;
#131518=CARTESIAN_POINT('Ctrl Pts',(-18.7946062779487,12.5574053612187,
131.057405473283)) ;
#131519=CARTESIAN_POINT('Ctrl Pts',(-18.8863176363417,12.4141338116398,
131.292346024062)) ;
#131520=CARTESIAN_POINT('Ctrl Pts',(-18.9880396659882,12.342233208706,131.556318246303)) ;
#131521=CARTESIAN_POINT('Ctrl Pts',(-19.092367557879,12.3479816385131,131.828001920729)) ;
#131522=CARTESIAN_POINT('Ctrl Pts',(-19.1930265312653,12.4308508598937,
132.088893600864)) ;
#131523=CARTESIAN_POINT('Ctrl Pts',(-19.2830355733598,12.5841342714032,
132.318802233278)) ;
#131524=CARTESIAN_POINT('Ctrl Pts',(-19.3575448753726,12.7991564308112,
132.503166321675)) ;
#131525=CARTESIAN_POINT('Ctrl Pts',(-19.410786935153,13.0569999610756,132.625693509338)) ;
#131526=CARTESIAN_POINT('Ctrl Pts',(-19.4405356262244,13.3421921034464,
132.679428679679)) ;
#131527=CARTESIAN_POINT('Ctrl Pts',(-19.4450790880921,13.6321454574867,
132.659662972591)) ;
#131528=CARTESIAN_POINT('Ctrl Pts',(-19.4247875387373,13.9089725412032,
132.567125349093)) ;
#131529=CARTESIAN_POINT('Ctrl Pts',(-19.381825668748,14.1498188340954,132.408476398238)) ;
#131530=CARTESIAN_POINT('Ctrl Pts',(-19.3204518279194,14.3379335225619,
132.196198119276)) ;
#131531=CARTESIAN_POINT('Ctrl Pts',(-19.2450347897687,14.4615825769609,
131.942693860373)) ;
#131532=CARTESIAN_POINT('Ctrl Pts',(-19.162267963524,14.5104718339952,131.667809535155)) ;
#131533=CARTESIAN_POINT('Ctrl Pts',(-19.0783524563333,14.4813917081873,
131.389457000585)) ;
#131534=CARTESIAN_POINT('Ctrl Pts',(-19.0006162859046,14.3764101476522,
131.129272642533)) ;
#131535=CARTESIAN_POINT('Ctrl Pts',(-18.9351626104612,14.2041613001764,
130.905077291113)) ;
#131536=CARTESIAN_POINT('Ctrl Pts',(-18.8868641696125,13.9743839791119,
130.730738018104)) ;
#131537=CARTESIAN_POINT('Ctrl Pts',(-18.8605695212481,13.7063210401926,
130.620861352139)) ;
#131538=CARTESIAN_POINT('Ctrl Pts',(-18.8586114405782,13.416701167449,130.581917827711)) ;
#131539=CARTESIAN_POINT('Ctrl Pts',(-18.8818454285258,13.1291677758352,
130.616763647551)) ;
#131540=CARTESIAN_POINT('Ctrl Pts',(-18.9294289009308,12.86171027905,130.722620411742)) ;
#131541=CARTESIAN_POINT('Ctrl Pts',(-18.9984336324713,12.6350478480017,
130.891152728659)) ;
#131542=CARTESIAN_POINT('Ctrl Pts',(-19.0852684560724,12.4638699665219,
131.111590594525)) ;
#131543=CARTESIAN_POINT('Ctrl Pts',(-19.1836902605787,12.3621126869917,
131.366013493841)) ;
#131544=CARTESIAN_POINT('Ctrl Pts',(-19.2880034593845,12.336288293437,131.637540200635)) ;
#131545=CARTESIAN_POINT('Ctrl Pts',(-19.3907293591919,12.3882079133966,
131.9045787098)) ;
#131546=CARTESIAN_POINT('Ctrl Pts',(-19.4861202999562,12.5148240028862,
132.150020522081)) ;
#131547=CARTESIAN_POINT('Ctrl Pts',(-19.566984502277,12.7050812653244,132.353293437429)) ;
#131548=CARTESIAN_POINT('Ctrl Pts',(-19.6294717703468,12.9482677220772,
132.502618790391)) ;
#131549=CARTESIAN_POINT('Ctrl Pts',(-19.6689768655333,13.2238578222556,
132.585025535771)) ;
#131550=CARTESIAN_POINT('Ctrl Pts',(-19.6838357324499,13.5162932448957,
132.595118812429)) ;
#131551=CARTESIAN_POINT('Ctrl Pts',(-19.6735197937544,13.799165239793,132.532024333921)) ;
#131552=CARTESIAN_POINT('Ctrl Pts',(-19.6392454600331,14.0580267764743,
132.398557205212)) ;
#131553=CARTESIAN_POINT('Ctrl Pts',(-19.5848869196862,14.2686028129511,
132.206807442572)) ;
#131554=CARTESIAN_POINT('Ctrl Pts',(-19.5145008411043,14.4199618502008,
131.968069495771)) ;
#131555=CARTESIAN_POINT('Ctrl Pts',(-19.4340220268986,14.4998958219189,
131.699871465245)) ;
#131556=CARTESIAN_POINT('Ctrl Pts',(-19.3495759662661,14.5025664794371,
131.419941342377)) ;
#131557=CARTESIAN_POINT('Ctrl Pts',(-19.2688627445457,14.4280652825415,
131.151146889785)) ;
#131558=CARTESIAN_POINT('Ctrl Pts',(-19.197514432747,14.2819177513075,130.909621465088)) ;
#131559=CARTESIAN_POINT('Ctrl Pts',(-19.1413921728409,14.0723877227319,
130.712339919469)) ;
#131560=CARTESIAN_POINT('Ctrl Pts',(-19.1060584048045,13.8191595273478,
130.576195818314)) ;
#131561=CARTESIAN_POINT('Ctrl Pts',(-19.0939136018658,13.5356702848312,
130.507524027747)) ;
#131562=CARTESIAN_POINT('Ctrl Pts',(-19.1068958007053,13.2451626614465,
130.512392184105)) ;
#131563=CARTESIAN_POINT('Ctrl Pts',(-19.1449564065195,12.9658959397094,
130.5903314269)) ;
#131564=CARTESIAN_POINT('Ctrl Pts',(-19.2057189790489,12.720867949973,130.73477557543)) ;
#131565=CARTESIAN_POINT('Ctrl Pts',(-19.2858400354675,12.5256178596935,
130.935699785553)) ;
#131566=CARTESIAN_POINT('Ctrl Pts',(-19.3800402811628,12.3947249390078,
131.177818876414)) ;
#131567=CARTESIAN_POINT('Ctrl Pts',(-19.4831200353959,12.3373274128747,
131.445666380565)) ;
#131568=CARTESIAN_POINT('Ctrl Pts',(-19.5867485454506,12.3577351376061,
131.715460652154)) ;
#131569=CARTESIAN_POINT('Ctrl Pts',(-19.6862131801358,12.4546492514378,
131.972779675498)) ;
#131570=CARTESIAN_POINT('Ctrl Pts',(-19.7738286134021,12.6210676591383,
132.195587853881)) ;
#131571=CARTESIAN_POINT('Ctrl Pts',(-19.8442902702029,12.8446766854148,
132.368316433847)) ;
#131572=CARTESIAN_POINT('Ctrl Pts',(-19.8933608798738,13.108808163257,132.478653710118)) ;
#131573=CARTESIAN_POINT('Ctrl Pts',(-19.9184859283659,13.3979062620311,
132.518747291947)) ;
#131574=CARTESIAN_POINT('Ctrl Pts',(-19.9181983031023,13.6859097607706,
132.484944374893)) ;
#131575=CARTESIAN_POINT('Ctrl Pts',(-19.8935840118438,13.9567565280856,
132.379898432991)) ;
#131576=CARTESIAN_POINT('Ctrl Pts',(-19.8465997978561,14.1899349125241,
132.209373856163)) ;
#131577=CARTESIAN_POINT('Ctrl Pts',(-19.7823820361551,14.3662692626876,
131.988864508273)) ;
#131578=CARTESIAN_POINT('Ctrl Pts',(-19.7048377925854,14.4768289979695,
131.729048105592)) ;
#131579=CARTESIAN_POINT('Ctrl Pts',(-19.621356858463,14.5109207090365,131.452070562692)) ;
#131580=CARTESIAN_POINT('Ctrl Pts',(-19.5383256537918,14.4673589954117,
131.176412965102)) ;
#131581=CARTESIAN_POINT('Ctrl Pts',(-19.462343360731,14.3490298117359,130.921339630599)) ;
#131582=CARTESIAN_POINT('Ctrl Pts',(-19.399598094763,14.1643442573792,130.70492417211)) ;
#131583=CARTESIAN_POINT('Ctrl Pts',(-19.3553585530389,13.9269540764464,
130.542614298548)) ;
#131584=CARTESIAN_POINT('Ctrl Pts',(-19.3333939719036,13.6529087066834,
130.44529695513)) ;
#131585=CARTESIAN_POINT('Ctrl Pts',(-19.3361541913265,13.3625040426011,
130.420224634067)) ;
#131586=CARTESIAN_POINT('Ctrl Pts',(-19.3641172961552,13.0764917625792,
130.468781137817)) ;
#131587=CARTESIAN_POINT('Ctrl Pts',(-19.4160399610195,12.8152457852602,
130.587319851219)) ;
#131588=CARTESIAN_POINT('Ctrl Pts',(-19.4888652574942,12.5977360848388,
130.766942106929)) ;
#131589=CARTESIAN_POINT('Ctrl Pts',(-19.5781388686584,12.4392301767845,
130.994608862376)) ;
#131590=CARTESIAN_POINT('Ctrl Pts',(-19.6782931891438,12.3513755992719,
131.254028736787)) ;
#131591=CARTESIAN_POINT('Ctrl Pts',(-19.7822229405507,12.3399316332142,
131.524661009902)) ;
#131592=CARTESIAN_POINT('Ctrl Pts',(-19.88504344773,12.4070554351268,131.791616350641)) ;
#131593=CARTESIAN_POINT('Ctrl Pts',(-19.9771610745846,12.5451369869361,
132.027897931008)) ;
#131594=CARTESIAN_POINT('Ctrl Pts',(-20.0556173721215,12.7477726868892,
132.223821692675)) ;
#131595=CARTESIAN_POINT('Ctrl Pts',(-20.1137903255926,12.9979367372735,
132.360683275234)) ;
#131596=CARTESIAN_POINT('Ctrl Pts',(-20.1489013724765,13.2792370978739,
132.430071631305)) ;
#131597=CARTESIAN_POINT('Ctrl Pts',(-20.1588787384282,13.5701580555343,
132.426125674529)) ;
#131598=CARTESIAN_POINT('Ctrl Pts',(-20.143937682242,13.8505377724051,132.349389311992)) ;
#131599=CARTESIAN_POINT('Ctrl Pts',(-20.1057318059421,14.1007512372239,
132.20463305785)) ;
#131600=CARTESIAN_POINT('Ctrl Pts',(-20.0478354950526,14.3021715583994,
132.002395149785)) ;
#131601=CARTESIAN_POINT('Ctrl Pts',(-19.9748500391882,14.4410638226486,
131.755979394128)) ;
#131602=CARTESIAN_POINT('Ctrl Pts',(-19.892940104349,14.506420576945,131.483512074612)) ;
#131603=CARTESIAN_POINT('Ctrl Pts',(-19.8092678890523,14.4944296739133,
131.206120710523)) ;
#131604=CARTESIAN_POINT('Ctrl Pts',(-19.7294350859359,14.4055611915821,
130.939713797808)) ;
#131605=CARTESIAN_POINT('Ctrl Pts',(-19.66081208133,14.2469875620131,130.706232624641)) ;
#131606=CARTESIAN_POINT('Ctrl Pts',(-19.6083158027718,14.0284942715184,
130.519673218377)) ;
#131607=CARTESIAN_POINT('Ctrl Pts',(-19.5769557514165,13.7670074742828,
130.394940588624)) ;
#131608=CARTESIAN_POINT('Ctrl Pts',(-19.5695668686991,13.4805781215048,
130.340191561689)) ;
#131609=CARTESIAN_POINT('Ctrl Pts',(-19.5872696261961,13.1913388058783,
130.358899107894)) ;
#131610=CARTESIAN_POINT('Ctrl Pts',(-19.6297522740938,12.9172330933754,
130.449814911348)) ;
#131611=CARTESIAN_POINT('Ctrl Pts',(-19.6944389773908,12.6799728703758,
130.60569175476)) ;
#131612=CARTESIAN_POINT('Ctrl Pts',(-19.7782230780513,12.4949910418975,
130.817115688087)) ;
#131613=CARTESIAN_POINT('Ctrl Pts',(-19.8739923402946,12.3781840447206,
131.063992159593)) ;
#131614=CARTESIAN_POINT('Ctrl Pts',(-19.9780674608701,12.3352411023339,
131.33468497079)) ;
#131615=CARTESIAN_POINT('Ctrl Pts',(-20.0810744379286,12.3701183957634,
131.602725123913)) ;
#131616=CARTESIAN_POINT('Ctrl Pts',(-20.179252895713,12.4815908370187,131.85612905703)) ;
#131617=CARTESIAN_POINT('Ctrl Pts',(-20.2634570739637,12.6586744463426,
132.069206441814)) ;
#131618=CARTESIAN_POINT('Ctrl Pts',(-20.3305901520664,12.8927064505131,
132.232014267973)) ;
#131619=CARTESIAN_POINT('Ctrl Pts',(-20.3750331233153,13.1615895986342,
132.328969789793)) ;
#131620=CARTESIAN_POINT('Ctrl Pts',(-20.3954965997089,13.4527337961883,
132.355428882089)) ;
#131621=CARTESIAN_POINT('Ctrl Pts',(-20.3904573045894,13.7397606263225,
132.307631593907)) ;
#131622=CARTESIAN_POINT('Ctrl Pts',(-20.3613437715797,14.0044956878458,
132.189457679076)) ;
#131623=CARTESIAN_POINT('Ctrl Pts',(-20.3110168045734,14.2270717047825,
132.009394785638)) ;
#131624=CARTESIAN_POINT('Ctrl Pts',(-20.2436381751946,14.3928428531141,
131.779444891534)) ;
#131625=CARTESIAN_POINT('Ctrl Pts',(-20.164336633125,14.4891679896536,131.51449038135)) ;
#131626=CARTESIAN_POINT('Ctrl Pts',(-20.0809111882638,14.5086708936273,
131.237865647246)) ;
#131627=CARTESIAN_POINT('Ctrl Pts',(-19.9983950566067,14.4507091204102,
130.963592375788)) ;
#131628=CARTESIAN_POINT('Ctrl Pts',(-19.9244190141413,14.318823465338,130.714351089596)) ;
#131629=CARTESIAN_POINT('Ctrl Pts',(-19.8648700988791,14.1234067424229,
130.507330724768)) ;
#131630=CARTESIAN_POINT('Ctrl Pts',(-19.8245161746179,13.8772496577341,
130.356293737963)) ;
#131631=CARTESIAN_POINT('Ctrl Pts',(-19.8070957881005,13.5994498547175,
130.272359938913)) ;
#131632=CARTESIAN_POINT('Ctrl Pts',(-19.8146864693653,13.3067289539218,
130.261220009531)) ;
#131633=CARTESIAN_POINT('Ctrl Pts',(-19.8471784531872,13.025513208076,130.323196727465)) ;
#131634=CARTESIAN_POINT('Ctrl Pts',(-19.9032180692331,12.7708776887036,
130.453754380472)) ;
#131635=CARTESIAN_POINT('Ctrl Pts',(-19.9797679754465,12.5628412979246,
130.644157296538)) ;
#131636=CARTESIAN_POINT('Ctrl Pts',(-20.0712997390683,12.4171764122364,
130.878502714501)) ;
#131637=CARTESIAN_POINT('Ctrl Pts',(-20.173220666744,12.3431378359771,131.142938313351)) ;
#131638=CARTESIAN_POINT('Ctrl Pts',(-20.2769543623743,12.3467434972734,
131.413078047708)) ;
#131639=CARTESIAN_POINT('Ctrl Pts',(-20.3779474556413,12.4272274658185,
131.674911921515)) ;
#131640=CARTESIAN_POINT('Ctrl Pts',(-20.4684824931614,12.5790158149027,
131.906293765199)) ;
#131641=CARTESIAN_POINT('Ctrl Pts',(-20.5433178346082,12.7916687829571,
132.091724629749)) ;
#131642=CARTESIAN_POINT('Ctrl Pts',(-20.59747019779,13.0498138992039,132.216737279054)) ;
#131643=CARTESIAN_POINT('Ctrl Pts',(-20.6277539698486,13.3331756720239,
132.272199599018)) ;
#131644=CARTESIAN_POINT('Ctrl Pts',(-20.63310319697,13.6238935345468,132.254712776567)) ;
#131645=CARTESIAN_POINT('Ctrl Pts',(-20.6135004102223,13.9010885274901,
132.164225860573)) ;
#131646=CARTESIAN_POINT('Ctrl Pts',(-20.5712628793398,14.1432054793993,
132.007719764268)) ;
#131647=CARTESIAN_POINT('Ctrl Pts',(-20.5099062183509,14.3341070280144,
131.795269476235)) ;
#131648=CARTESIAN_POINT('Ctrl Pts',(-20.4352339689786,14.4587991787124,
131.544150012527)) ;
#131649=CARTESIAN_POINT('Ctrl Pts',(-20.3525489079931,14.5101605081857,
131.269477291802)) ;
#131650=CARTESIAN_POINT('Ctrl Pts',(-20.2687361872864,14.4834097576633,
130.991492371573)) ;
#131651=CARTESIAN_POINT('Ctrl Pts',(-20.1906756501309,14.380986704451,130.730363509583)) ;
#131652=CARTESIAN_POINT('Ctrl Pts',(-20.1243569260148,14.2089571607828,
130.503381990289)) ;
#131653=CARTESIAN_POINT('Ctrl Pts',(-20.0759333865454,13.9828180453883,
130.329004955831)) ;
#131654=CARTESIAN_POINT('Ctrl Pts',(-20.0486953445985,13.7132629209954,
130.216063933579)) ;
#131655=CARTESIAN_POINT('Ctrl Pts',(-20.0461136758052,13.42583764063,130.175529664949)) ;
#131656=CARTESIAN_POINT('Ctrl Pts',(-20.0685766436055,13.1374631065902,
130.208056459246)) ;
#131657=CARTESIAN_POINT('Ctrl Pts',(-20.1154485813734,12.8691197006536,
130.31184888817)) ;
#131658=CARTESIAN_POINT('Ctrl Pts',(-20.1842161886027,12.6403113443668,
130.479551228157)) ;
#131659=CARTESIAN_POINT('Ctrl Pts',(-20.2699974667944,12.468420702256,130.697148821309)) ;
#131660=CARTESIAN_POINT('Ctrl Pts',(-20.368777345651,12.3638000217504,130.952399609198)) ;
#131661=CARTESIAN_POINT('Ctrl Pts',(-20.4724837589939,12.3359859144704,
131.22233281641)) ;
#131662=CARTESIAN_POINT('Ctrl Pts',(-20.5755189014966,12.3855342690204,
131.490214378318)) ;
#131663=CARTESIAN_POINT('Ctrl Pts',(-20.6710370148352,12.5097023136888,
131.736103980719)) ;
#131664=CARTESIAN_POINT('Ctrl Pts',(-20.7526999022241,12.6987169895182,
131.941597617443)) ;
#131665=CARTESIAN_POINT('Ctrl Pts',(-20.8159200282362,12.9413958856346,
132.092978431002)) ;
#131666=CARTESIAN_POINT('Ctrl Pts',(-20.8560148207953,13.2164083911014,
132.177101494275)) ;
#131667=CARTESIAN_POINT('Ctrl Pts',(-20.8715568106971,13.5077476116907,
132.18930496735)) ;
#131668=CARTESIAN_POINT('Ctrl Pts',(-20.8618791478333,13.7917084995172,
132.127994218716)) ;
#131669=CARTESIAN_POINT('Ctrl Pts',(-20.8285666993428,14.0497089633418,
131.997596945122)) ;
#131670=CARTESIAN_POINT('Ctrl Pts',(-20.7745879228126,14.2632250030891,
131.806787903495)) ;
#131671=CARTESIAN_POINT('Ctrl Pts',(-20.7043311974277,14.4168537708596,
131.568328459368)) ;
#131672=CARTESIAN_POINT('Ctrl Pts',(-20.6239603167272,14.4987598986465,
131.300415425815)) ;
#131673=CARTESIAN_POINT('Ctrl Pts',(-20.539754785129,14.5035045718472,131.021276419093)) ;
#131674=CARTESIAN_POINT('Ctrl Pts',(-20.4588117616689,14.4313229997249,
130.751803459987)) ;
#131675=CARTESIAN_POINT('Ctrl Pts',(-20.3868956375626,14.286096674379,130.508478859911)) ;
#131676=CARTESIAN_POINT('Ctrl Pts',(-20.3308554449234,14.0806888556304,
130.311826279916)) ;
#131677=CARTESIAN_POINT('Ctrl Pts',(-20.2944696102375,13.8265805447723,
130.172317712221)) ;
#131678=CARTESIAN_POINT('Ctrl Pts',(-20.2817095072984,13.5441879409374,
130.101929815543)) ;
#131679=CARTESIAN_POINT('Ctrl Pts',(-20.2939970046262,13.2530370689606,
130.104694604891)) ;
#131680=CARTESIAN_POINT('Ctrl Pts',(-20.3312192505214,12.9741114175935,
130.18030810907)) ;
#131681=CARTESIAN_POINT('Ctrl Pts',(-20.391477731723,12.7272119216586,130.323195480133)) ;
#131682=CARTESIAN_POINT('Ctrl Pts',(-20.4710215017653,12.5305677659782,
130.522476172394)) ;
#131683=CARTESIAN_POINT('Ctrl Pts',(-20.5648765077218,12.3976028767503,
130.763584707341)) ;
#131684=CARTESIAN_POINT('Ctrl Pts',(-20.6677354645716,12.3378877564715,
131.030810858964)) ;
#131685=CARTESIAN_POINT('Ctrl Pts',(-20.771610142133,12.3561146457162,131.301258410359)) ;
#131686=CARTESIAN_POINT('Ctrl Pts',(-20.8710140356471,12.4504996091204,
131.558507272223)) ;
#131687=CARTESIAN_POINT('Ctrl Pts',(-20.9591976245712,12.6151918179393,
131.782920165643)) ;
#131688=CARTESIAN_POINT('Ctrl Pts',(-21.0301909969835,12.8367627956422,
131.957264907826)) ;
#131689=CARTESIAN_POINT('Ctrl Pts',(-21.0802720431719,13.102471284239,132.070248175628)) ;
#131690=CARTESIAN_POINT('Ctrl Pts',(-21.1058128562322,13.388098474674,132.11192368682)) ;
#131691=CARTESIAN_POINT('Ctrl Pts',(-21.1063578527298,13.6786302634614,
132.08028850925)) ;
#131692=CARTESIAN_POINT('Ctrl Pts',(-21.0823275663731,13.9495118019851,
131.977027551482)) ;
#131693=CARTESIAN_POINT('Ctrl Pts',(-21.0362217842379,14.1831630717315,
131.809216673534)) ;
#131694=CARTESIAN_POINT('Ctrl Pts',(-20.9721884045855,14.3622887251467,
131.589091305906)) ;
#131695=CARTESIAN_POINT('Ctrl Pts',(-20.8947792880245,14.4748192529362,
131.32962547702)) ;
#131696=CARTESIAN_POINT('Ctrl Pts',(-20.8116749026299,14.5109473630978,
131.053861074448)) ;
#131697=CARTESIAN_POINT('Ctrl Pts',(-20.7286272549608,14.46989386631,130.778195045776)) ;
#131698=CARTESIAN_POINT('Ctrl Pts',(-20.6522431108941,14.3536144736526,
130.521907930923)) ;
#131699=CARTESIAN_POINT('Ctrl Pts',(-20.5889583813436,14.17062113719,130.303892930056)) ;
#131700=CARTESIAN_POINT('Ctrl Pts',(-20.5440524129988,13.933736573907,130.13953810035)) ;
#131701=CARTESIAN_POINT('Ctrl Pts',(-20.5214975045223,13.6617104442443,
130.040649083481)) ;
#131702=CARTESIAN_POINT('Ctrl Pts',(-20.5235105668905,13.3701432171844,
130.013237741548)) ;
#131703=CARTESIAN_POINT('Ctrl Pts',(-20.5508607538459,13.0839501475181,
130.0600249237)) ;
#131704=CARTESIAN_POINT('Ctrl Pts',(-20.6019342296123,12.8226369063403,
130.176200002378)) ;
#131705=CARTESIAN_POINT('Ctrl Pts',(-20.674162245095,12.6036153158418,130.354083975274)) ;
#131706=CARTESIAN_POINT('Ctrl Pts',(-20.7628382753172,12.4432239429731,
130.580060592785)) ;
#131707=CARTESIAN_POINT('Ctrl Pts',(-20.8633579914741,12.3525997513282,
130.840351394468)) ;
#131708=CARTESIAN_POINT('Ctrl Pts',(-20.9671168641114,12.3393903655815,
131.110528978872)) ;
#131709=CARTESIAN_POINT('Ctrl Pts',(-21.0694306011919,12.403468098602,131.376231401918)) ;
#131710=CARTESIAN_POINT('Ctrl Pts',(-21.1627219404933,12.5405072085783,
131.615661785443)) ;
#131711=CARTESIAN_POINT('Ctrl Pts',(-21.2416127937835,12.7420005519616,
131.812839172161)) ;
#131712=CARTESIAN_POINT('Ctrl Pts',(-21.3001704333997,12.9900801149227,
131.950949061272)) ;
#131713=CARTESIAN_POINT('Ctrl Pts',(-21.3360159038547,13.2708158721555,
132.022475029764)) ;
#131714=CARTESIAN_POINT('Ctrl Pts',(-21.3467250085586,13.5613604134334,
132.020708203514)) ;
#131715=CARTESIAN_POINT('Ctrl Pts',(-21.332530072888,13.8428560081929,131.946099675255)) ;
#131716=CARTESIAN_POINT('Ctrl Pts',(-21.2946880005883,14.0951246502648,
131.802259522002)) ;
#131717=CARTESIAN_POINT('Ctrl Pts',(-21.2376357521135,14.2968154125605,
131.602698948677)) ;
#131718=CARTESIAN_POINT('Ctrl Pts',(-21.164806246768,14.4382062812648,131.356634806151)) ;
#131719=CARTESIAN_POINT('Ctrl Pts',(-21.0832408338308,14.5055713938207,
131.085254319312)) ;
#131720=CARTESIAN_POINT('Ctrl Pts',(-20.9994162423038,14.4957941932041,
130.807360837672)) ;
#131721=CARTESIAN_POINT('Ctrl Pts',(-20.9195959138854,14.4095662340998,
130.541102349046)) ;
#131722=CARTESIAN_POINT('Ctrl Pts',(-20.8500186277359,14.2515335127425,
130.304558118666)) ;
#131723=CARTESIAN_POINT('Ctrl Pts',(-20.7972486154139,14.0347236874785,
130.11728882556)) ;
#131724=CARTESIAN_POINT('Ctrl Pts',(-20.7653613268004,13.7751700114088,
129.991129528377)) ;
#131725=CARTESIAN_POINT('Ctrl Pts',(-20.7571817990629,13.489555102194,129.934113768398)) ;
#131726=CARTESIAN_POINT('Ctrl Pts',(-20.7742556911792,13.1989624545804,
129.950844344899)) ;
#131727=CARTESIAN_POINT('Ctrl Pts',(-20.8159809707414,12.9245155762064,
130.03960916018)) ;
#131728=CARTESIAN_POINT('Ctrl Pts',(-20.8805367450398,12.6850932088169,
130.194926855194)) ;
#131729=CARTESIAN_POINT('Ctrl Pts',(-20.9626356003938,12.5007200500438,
130.401901459438)) ;
#131730=CARTESIAN_POINT('Ctrl Pts',(-21.0591957946408,12.3802348015134,
130.650687618331)) ;
#131731=CARTESIAN_POINT('Ctrl Pts',(-21.1622370545661,12.3354177830535,
130.918672003733)) ;
#131732=CARTESIAN_POINT('Ctrl Pts',(-21.2662887681593,12.3682931650198,
131.189443526458)) ;
#131733=CARTESIAN_POINT('Ctrl Pts',(-21.3637199956931,12.4764500222757,
131.44102792815)) ;
#131734=CARTESIAN_POINT('Ctrl Pts',(-21.4490683123423,12.6527561756398,
131.657189302748)) ;
#131735=CARTESIAN_POINT('Ctrl Pts',(-21.5164968590452,12.8841372675975,
131.821041651181)) ;
#131736=CARTESIAN_POINT('Ctrl Pts',(-21.5620729321248,13.1550291136418,
131.920951331736)) ;
#131737=CARTESIAN_POINT('Ctrl Pts',(-21.5829990360394,13.4437302360126,
131.949026741888)) ;
#131738=CARTESIAN_POINT('Ctrl Pts',(-21.5787261653874,13.7319393007276,
131.903366364301)) ;
#131739=CARTESIAN_POINT('Ctrl Pts',(-21.5503975227815,13.9965481623833,
131.787623344815)) ;
#131740=CARTESIAN_POINT('Ctrl Pts',(-21.5005342471165,14.2215298170475,
131.608800269925)) ;
#131741=CARTESIAN_POINT('Ctrl Pts',(-21.4333938850247,14.3891483272759,
131.379489123203)) ;
#131742=CARTESIAN_POINT('Ctrl Pts',(-21.3548735774567,14.4871687024338,
131.117033634355)) ;
#131743=CARTESIAN_POINT('Ctrl Pts',(-21.2709428978837,14.5093408079897,
130.838711318976)) ;
#131744=CARTESIAN_POINT('Ctrl Pts',(-21.1882422406468,14.4530254583256,
130.563868416307)) ;
#131745=CARTESIAN_POINT('Ctrl Pts',(-21.1143270880585,14.3240305585518,
130.31499305445)) ;
#131746=CARTESIAN_POINT('Ctrl Pts',(-21.0539688868397,14.1290979717854,
130.105410602035)) ;
#131747=CARTESIAN_POINT('Ctrl Pts',(-21.0132069302916,13.8855604155571,
129.953378103653)) ;
#131748=CARTESIAN_POINT('Ctrl Pts',(-20.9950030451873,13.6058416707122,
129.866845755651)) ;
#131749=CARTESIAN_POINT('Ctrl Pts',(-21.0018793397198,13.3160021377259,
129.853947611582)) ;
#131750=CARTESIAN_POINT('Ctrl Pts',(-21.0337293398582,13.0326886676077,
129.913868033499)) ;
#131751=CARTESIAN_POINT('Ctrl Pts',(-21.0893772116349,12.7766372190837,
130.043216529831)) ;
#131752=CARTESIAN_POINT('Ctrl Pts',(-21.1653161877122,12.5676698161814,
130.231901557219)) ;
#131753=CARTESIAN_POINT('Ctrl Pts',(-21.2561790285771,12.4206517790888,
130.464404545457)) ;
#131754=CARTESIAN_POINT('Ctrl Pts',(-21.3575675366688,12.3443150505119,
130.727387699059)) ;
#131755=CARTESIAN_POINT('Ctrl Pts',(-21.4618210845223,12.3454567433165,
130.998884337509)) ;
#131756=CARTESIAN_POINT('Ctrl Pts',(-21.5631430702427,12.4241540146565,
131.261630006307)) ;
#131757=CARTESIAN_POINT('Ctrl Pts',(-21.6537810155053,12.5736454649868,
131.493407152973)) ;
#131758=CARTESIAN_POINT('Ctrl Pts',(-21.7290950924145,12.7844244258342,
131.680270904741)) ;
#131759=CARTESIAN_POINT('Ctrl Pts',(-21.7839298109933,13.041264478038,131.807295952736)) ;
#131760=CARTESIAN_POINT('Ctrl Pts',(-21.8150448539116,13.3250313838274,
131.865081031141)) ;
#131761=CARTESIAN_POINT('Ctrl Pts',(-21.8210632536644,13.6156492492809,
131.849571033927)) ;
#131762=CARTESIAN_POINT('Ctrl Pts',(-21.8022545212773,13.8929002803611,
131.761487721122)) ;
#131763=CARTESIAN_POINT('Ctrl Pts',(-21.7605924585031,14.1366366428793,
131.606614879296)) ;
#131764=CARTESIAN_POINT('Ctrl Pts',(-21.6999698317163,14.3287833833703,
131.396421302764)) ;
#131765=CARTESIAN_POINT('Ctrl Pts',(-21.6253197774301,14.4563288342089,
131.145218098165)) ;
#131766=CARTESIAN_POINT('Ctrl Pts',(-21.5425945750513,14.5097636463918,
130.870367772935)) ;
#131767=CARTESIAN_POINT('Ctrl Pts',(-21.4589621479375,14.4852491819093,
130.593003563587)) ;
#131768=CARTESIAN_POINT('Ctrl Pts',(-21.380714091029,14.385213180382,130.331360934625)) ;
#131769=CARTESIAN_POINT('Ctrl Pts',(-21.3138290434139,14.2148994362801,
130.102677640231)) ;
#131770=CARTESIAN_POINT('Ctrl Pts',(-21.264802027938,13.9895605141043,129.92646714371)) ;
#131771=CARTESIAN_POINT('Ctrl Pts',(-21.2370048320792,13.7226496289756,
129.812102485109)) ;
#131772=CARTESIAN_POINT('Ctrl Pts',(-21.2336042417307,13.4342098859693,
129.769013814372)) ;
#131773=CARTESIAN_POINT('Ctrl Pts',(-21.2553236046358,13.1458182759752,
129.799407215841)) ;
#131774=CARTESIAN_POINT('Ctrl Pts',(-21.3016988392798,12.8759127132536,
129.901648132077)) ;
#131775=CARTESIAN_POINT('Ctrl Pts',(-21.3694669987003,12.6468868556867,
130.066623481143)) ;
#131776=CARTESIAN_POINT('Ctrl Pts',(-21.4553373193102,12.4721832296684,
130.284273605613)) ;
#131777=CARTESIAN_POINT('Ctrl Pts',(-21.5530256217249,12.3661739274481,
130.536616813639)) ;
#131778=CARTESIAN_POINT('Ctrl Pts',(-21.6575177270796,12.3355863385396,
130.808562220896)) ;
#131779=CARTESIAN_POINT('Ctrl Pts',(-21.7604456918656,12.3831198658751,
131.076206190241)) ;
#131780=CARTESIAN_POINT('Ctrl Pts',(-21.8563696469902,12.5053833023315,
131.323242388746)) ;
#131781=CARTESIAN_POINT('Ctrl Pts',(-21.9382966693068,12.6923270702948,
131.529584453516)) ;
#131782=CARTESIAN_POINT('Ctrl Pts',(-22.0021645015312,12.9335865705139,
131.682862448256)) ;
#131783=CARTESIAN_POINT('Ctrl Pts',(-22.0430213128192,13.2085814539572,
131.769129801508)) ;
#131784=CARTESIAN_POINT('Ctrl Pts',(-22.0592352836556,13.4990557588074,
131.783380739882)) ;
#131785=CARTESIAN_POINT('Ctrl Pts',(-22.0503004073671,13.7836907462661,
131.724216167399)) ;
#131786=CARTESIAN_POINT('Ctrl Pts',(-22.0176371901026,14.0427281414566,
131.595717480909)) ;
#131787=CARTESIAN_POINT('Ctrl Pts',(-21.9641995370827,14.2577309750281,
131.406490661624)) ;
#131788=CARTESIAN_POINT('Ctrl Pts',(-21.8944782363852,14.4131664617501,
131.169654967239)) ;
#131789=CARTESIAN_POINT('Ctrl Pts',(-21.8141620072022,14.4973755702956,
130.901832610092)) ;
#131790=CARTESIAN_POINT('Ctrl Pts',(-21.7303937720881,14.5046724130054,
130.624142862364)) ;
#131791=CARTESIAN_POINT('Ctrl Pts',(-21.6486693225774,14.4343111747756,
130.352140919931)) ;
#131792=CARTESIAN_POINT('Ctrl Pts',(-21.5766530687314,14.2913904033354,
130.108640611113)) ;
#131793=CARTESIAN_POINT('Ctrl Pts',(-21.5199914526865,14.0872940403586,
129.910112364196)) ;
#131794=CARTESIAN_POINT('Ctrl Pts',(-21.4830382408884,13.8349907742835,
129.769035274606)) ;
#131795=CARTESIAN_POINT('Ctrl Pts',(-21.4694985396213,13.5522018199285,
129.696252361388)) ;
#131796=CARTESIAN_POINT('Ctrl Pts',(-21.4810885813508,13.2611771320633,
129.697002826515)) ;
#131797=CARTESIAN_POINT('Ctrl Pts',(-21.5176805732444,12.9814107201437,
129.770743949859)) ;
#131798=CARTESIAN_POINT('Ctrl Pts',(-21.5771191123903,12.7341369610279,
129.911345858839)) ;
#131799=CARTESIAN_POINT('Ctrl Pts',(-21.6563209788842,12.535166216503,130.109544290444)) ;
#131800=CARTESIAN_POINT('Ctrl Pts',(-21.7502713534583,12.4000170891871,
130.350799701057)) ;
#131801=CARTESIAN_POINT('Ctrl Pts',(-21.8524815344102,12.3385941106561,
130.616296707476)) ;
#131802=CARTESIAN_POINT('Ctrl Pts',(-21.9565712501459,12.3545286685026,
130.887315313701)) ;
#131803=CARTESIAN_POINT('Ctrl Pts',(-22.0562577481496,12.4469846430608,
131.14537139149)) ;
#131804=CARTESIAN_POINT('Ctrl Pts',(-22.1449360417052,12.6102579412087,
131.371180205731)) ;
#131805=CARTESIAN_POINT('Ctrl Pts',(-22.2161370464207,12.8296977311719,
131.546256445573)) ;
#131806=CARTESIAN_POINT('Ctrl Pts',(-22.2667592690025,13.0929763552362,
131.660982603106)) ;
#131807=CARTESIAN_POINT('Ctrl Pts',(-22.2932535098378,13.3798715107165,
131.705248169509)) ;
#131808=CARTESIAN_POINT('Ctrl Pts',(-22.2944576782056,13.6705227535771,
131.675549761758)) ;
#131809=CARTESIAN_POINT('Ctrl Pts',(-22.2711545117995,13.9421700423004,
131.57442408932)) ;
#131810=CARTESIAN_POINT('Ctrl Pts',(-22.2253820822901,14.1780191011813,
131.407446635602)) ;
#131811=CARTESIAN_POINT('Ctrl Pts',(-22.1619741826909,14.3579768124892,
131.189272795754)) ;
#131812=CARTESIAN_POINT('Ctrl Pts',(-22.0850483275451,14.4725057553617,
130.931291857228)) ;
#131813=CARTESIAN_POINT('Ctrl Pts',(-22.0018889458697,14.5110248787396,
130.655306915796)) ;
#131814=CARTESIAN_POINT('Ctrl Pts',(-21.9186831269904,14.4721191969269,
130.37915685792)) ;
#131815=CARTESIAN_POINT('Ctrl Pts',(-21.8419983594231,14.3577454336847,
130.121978165508)) ;
#131816=CARTESIAN_POINT('Ctrl Pts',(-21.7784559689967,14.1770688666527,
129.90331119887)) ;
#131817=CARTESIAN_POINT('Ctrl Pts',(-21.7328730623761,13.9416997327419,
129.73698112711)) ;
#131818=CARTESIAN_POINT('Ctrl Pts',(-21.7095937547817,13.6694104353782,
129.635852457523)) ;
#131819=CARTESIAN_POINT('Ctrl Pts',(-21.7108544164153,13.3798585935035,
129.60644988842)) ;
#131820=CARTESIAN_POINT('Ctrl Pts',(-21.7373587408651,13.0927640382574,
129.650717582232)) ;
#131821=CARTESIAN_POINT('Ctrl Pts',(-21.7879727694938,12.8294542733058,
129.765423278)) ;
#131822=CARTESIAN_POINT('Ctrl Pts',(-21.8596572059499,12.6090080043084,
129.941724810289)) ;
#131823=CARTESIAN_POINT('Ctrl Pts',(-21.9481186483126,12.4466659582347,
130.167016290758)) ;
#131824=CARTESIAN_POINT('Ctrl Pts',(-22.0478029406896,12.3544265354386,
130.425067159699)) ;
#131825=CARTESIAN_POINT('Ctrl Pts',(-22.1517530143636,12.338485550426,130.695728652991)) ;
#131826=CARTESIAN_POINT('Ctrl Pts',(-22.2547791723717,12.4009576070215,
130.963329774343)) ;
#131827=CARTESIAN_POINT('Ctrl Pts',(-22.3479076849026,12.5356622675021,
131.202441690569)) ;
#131828=CARTESIAN_POINT('Ctrl Pts',(-22.427039674185,12.7342792931547,131.400473047047)) ;
#131829=CARTESIAN_POINT('Ctrl Pts',(-22.4865817751364,12.9822470405306,
131.541298758196)) ;
#131830=CARTESIAN_POINT('Ctrl Pts',(-22.5231351067208,13.2626104241267,
131.614868935857)) ;
#131831=CARTESIAN_POINT('Ctrl Pts',(-22.5345613145019,13.5537330357078,
131.615129217148)) ;
#131832=CARTESIAN_POINT('Ctrl Pts',(-22.5210072175352,13.8350780443648,
131.542464925158)) ;
#131833=CARTESIAN_POINT('Ctrl Pts',(-22.4841282635127,14.0872562376869,
131.401629162015)) ;
#131834=CARTESIAN_POINT('Ctrl Pts',(-22.4271936380161,14.2922552735091,
131.202157542)) ;
#131835=CARTESIAN_POINT('Ctrl Pts',(-22.3548468095764,14.4349645919609,
130.957589374496)) ;
#131836=CARTESIAN_POINT('Ctrl Pts',(-22.2738049730186,14.5045540577175,
130.687866104784)) ;
#131837=CARTESIAN_POINT('Ctrl Pts',(-22.1896316409164,14.4973581396257,
130.408831550043)) ;
#131838=CARTESIAN_POINT('Ctrl Pts',(-22.1093343470203,14.4126016842873,
130.14105358009)) ;
#131839=CARTESIAN_POINT('Ctrl Pts',(-22.0399356599868,14.2578370889756,
129.905309744937)) ;
#131840=CARTESIAN_POINT('Ctrl Pts',(-21.9863765422796,14.0423606370671,
129.715650705837)) ;
#131841=CARTESIAN_POINT('Ctrl Pts',(-21.9537345461485,13.7833430848993,
129.58722594006)) ;
#131842=CARTESIAN_POINT('Ctrl Pts',(-21.9448743026681,13.4972454461382,
129.528113894271)) ;
#131843=CARTESIAN_POINT('Ctrl Pts',(-21.9611494569257,13.2077137971034,
129.542654652447)) ;
#131844=CARTESIAN_POINT('Ctrl Pts',(-22.002288346979,12.9318531124,129.629618831657)) ;
#131845=CARTESIAN_POINT('Ctrl Pts',(-22.0658546135328,12.6922552108513,
129.782222524194)) ;
#131846=CARTESIAN_POINT('Ctrl Pts',(-22.1480419825475,12.504666487009,129.989213929092)) ;
#131847=CARTESIAN_POINT('Ctrl Pts',(-22.2443302147763,12.3825157199122,
130.237218364436)) ;
#131848=CARTESIAN_POINT('Ctrl Pts',(-22.3470392380216,12.3357140444497,
130.504298662281)) ;
#131849=CARTESIAN_POINT('Ctrl Pts',(-22.4509464733217,12.3660679541908,
130.774724556597)) ;
#131850=CARTESIAN_POINT('Ctrl Pts',(-22.549161413923,12.4727573812884,131.028420389511)) ;
#131851=CARTESIAN_POINT('Ctrl Pts',(-22.6347030566716,12.6471452986828,
131.245220928735)) ;
#131852=CARTESIAN_POINT('Ctrl Pts',(-22.7025433269035,12.8766362181276,
131.410346416835)) ;
#131853=CARTESIAN_POINT('Ctrl Pts',(-22.7487814948906,13.1457609561308,
131.512289397035)) ;
#131854=CARTESIAN_POINT('Ctrl Pts',(-22.7705721874272,13.436208516762,131.542656742186)) ;
#131855=CARTESIAN_POINT('Ctrl Pts',(-22.7669909559281,13.7232902020091,
131.499187113643)) ;
#131856=CARTESIAN_POINT('Ctrl Pts',(-22.739314974999,13.9896012284326,131.385259077282)) ;
#131857=CARTESIAN_POINT('Ctrl Pts',(-22.6899563353196,14.2159296230216,
131.207905951156)) ;
#131858=CARTESIAN_POINT('Ctrl Pts',(-22.6233672864789,14.3851342144556,
130.980263042488)) ;
#131859=CARTESIAN_POINT('Ctrl Pts',(-22.5449702570784,14.4854516976048,
130.718115056966)) ;
#131860=CARTESIAN_POINT('Ctrl Pts',(-22.461265093064,14.5096986607512,130.440515127017)) ;
#131861=CARTESIAN_POINT('Ctrl Pts',(-22.378621004999,14.4561737731647,130.165930931039)) ;
#131862=CARTESIAN_POINT('Ctrl Pts',(-22.3039082628437,14.3282785458503,
129.914502352423)) ;
#131863=CARTESIAN_POINT('Ctrl Pts',(-22.2434277952934,14.1363003864466,
129.704779792514)) ;
#131864=CARTESIAN_POINT('Ctrl Pts',(-22.2017896977858,13.8924839857025,
129.549971716453)) ;
#131865=CARTESIAN_POINT('Ctrl Pts',(-22.1830205641406,13.6154602436594,
129.462035111654)) ;
#131866=CARTESIAN_POINT('Ctrl Pts',(-22.1890712067793,13.3244466531158,
129.446574293387)) ;
#131867=CARTESIAN_POINT('Ctrl Pts',(-22.2202555636145,13.0407282159145,
129.504562629151)) ;
#131868=CARTESIAN_POINT('Ctrl Pts',(-22.2750211321796,12.7843965627726,
129.631442703902)) ;
#131869=CARTESIAN_POINT('Ctrl Pts',(-22.3503429335631,12.5734338880589,
129.818316417424)) ;
#131870=CARTESIAN_POINT('Ctrl Pts',(-22.4414173268538,12.4236459559127,
130.051229799352)) ;
#131871=CARTESIAN_POINT('Ctrl Pts',(-22.5421394962141,12.3455712635568,
130.312426708327)) ;
#131872=CARTESIAN_POINT('Ctrl Pts',(-22.6467265172187,12.3443023671055,
130.584788395612)) ;
#131873=CARTESIAN_POINT('Ctrl Pts',(-22.7481657330948,12.420933178294,130.847899857883)) ;
#131874=CARTESIAN_POINT('Ctrl Pts',(-22.8392055009209,12.5684896870098,
131.080841902066)) ;
#131875=CARTESIAN_POINT('Ctrl Pts',(-22.9152137261507,12.7783872300958,
131.269645560269)) ;
#131876=CARTESIAN_POINT('Ctrl Pts',(-22.9705402435953,13.0341435528073,
131.398130661038)) ;
#131877=CARTESIAN_POINT('Ctrl Pts',(-23.0022377817911,13.3161552682329,
131.457761074721)) ;
#131878=CARTESIAN_POINT('Ctrl Pts',(-23.009059140071,13.6077102167408,131.444501189894)) ;
#131879=CARTESIAN_POINT('Ctrl Pts',(-22.9907943770449,13.8863966863271,
131.357908893058)) ;
#131880=CARTESIAN_POINT('Ctrl Pts',(-22.9497275238959,14.1306963082603,
131.204837242028)) ;
#131881=CARTESIAN_POINT('Ctrl Pts',(-22.8897860606364,14.3238933046915,
130.996741057129)) ;
#131882=CARTESIAN_POINT('Ctrl Pts',(-22.8155047276147,14.4535137780173,
130.746625113997)) ;
#131883=CARTESIAN_POINT('Ctrl Pts',(-22.7328983548189,14.5094099168095,
130.47211370142)) ;
#131884=CARTESIAN_POINT('Ctrl Pts',(-22.6487340748289,14.4867701673882,
130.193005786419)) ;
#131885=CARTESIAN_POINT('Ctrl Pts',(-22.5707021703194,14.3890643828725,
129.932173416396)) ;
#131886=CARTESIAN_POINT('Ctrl Pts',(-22.5034195621283,14.2211869107964,
129.70237977909)) ;
#131887=CARTESIAN_POINT('Ctrl Pts',(-22.4535961395973,13.9958858020985,
129.523655290175)) ;
#131888=CARTESIAN_POINT('Ctrl Pts',(-22.4253306349521,13.7314793548645,
129.40812642471)) ;
#131889=CARTESIAN_POINT('Ctrl Pts',(-22.4210875175899,13.4423639400344,
129.362455182987)) ;
#131890=CARTESIAN_POINT('Ctrl Pts',(-22.4422895478426,13.1530743203904,
129.391256495026)) ;
#131891=CARTESIAN_POINT('Ctrl Pts',(-22.487580667877,12.8842566111771,129.490582827144)) ;
#131892=CARTESIAN_POINT('Ctrl Pts',(-22.5552977498778,12.6519995362001,
129.655140460866)) ;
#131893=CARTESIAN_POINT('Ctrl Pts',(-22.6402716313289,12.4766942436469,
129.870371614395)) ;
#131894=CARTESIAN_POINT('Ctrl Pts',(-22.7378885944903,12.3681120678918,
130.122423877062)) ;
#131895=CARTESIAN_POINT('Ctrl Pts',(-22.8423855341256,12.3353450096833,
130.394363079284)) ;
#131896=CARTESIAN_POINT('Ctrl Pts',(-22.9455053804218,12.3808789292608,
130.66253674151)) ;
#131897=CARTESIAN_POINT('Ctrl Pts',(-23.0414119491019,12.5006496739186,
130.90963712832)) ;
#131898=CARTESIAN_POINT('Ctrl Pts',(-23.1239874820464,12.6862348924807,
131.117800379368)) ;
#131899=CARTESIAN_POINT('Ctrl Pts',(-23.1882404954987,12.9253055289241,
131.272326344278)) ;
#131900=CARTESIAN_POINT('Ctrl Pts',(-23.2299054869804,13.1996774467986,
131.360925356354)) ;
#131901=CARTESIAN_POINT('Ctrl Pts',(-23.2469197712831,13.4900583198245,
131.37750845876)) ;
#131902=CARTESIAN_POINT('Ctrl Pts',(-23.2386702442009,13.7765694769724,
131.320183787516)) ;
#131903=CARTESIAN_POINT('Ctrl Pts',(-23.2064532063664,14.036835662277,131.192930360202)) ;
#131904=CARTESIAN_POINT('Ctrl Pts',(-23.1537890318512,14.2522894974628,
131.006121661116)) ;
#131905=CARTESIAN_POINT('Ctrl Pts',(-23.0841408392017,14.410142650821,130.769355953609)) ;
#131906=CARTESIAN_POINT('Ctrl Pts',(-23.0044224542759,14.4959011359271,
130.503451200898)) ;
#131907=CARTESIAN_POINT('Ctrl Pts',(-22.9205051252153,14.5055615596735,
130.225254015656)) ;
#131908=CARTESIAN_POINT('Ctrl Pts',(-22.8387642579551,14.4373879166647,
129.953265322989)) ;
#131909=CARTESIAN_POINT('Ctrl Pts',(-22.7664377143828,14.2968056087925,
129.708895562602)) ;
#131910=CARTESIAN_POINT('Ctrl Pts',(-22.7090205846332,14.0934340145334,
129.508020332236)) ;
#131911=CARTESIAN_POINT('Ctrl Pts',(-22.6715788423865,13.8423638114029,
129.365551179356)) ;
#131912=CARTESIAN_POINT('Ctrl Pts',(-22.6573294356865,13.5615577206812,
129.290854833297)) ;
#131913=CARTESIAN_POINT('Ctrl Pts',(-22.6681862864359,13.2694348944804,
129.289338191419)) ;
#131914=CARTESIAN_POINT('Ctrl Pts',(-22.7039617574597,12.9897647818979,
129.360785289403)) ;
#131915=CARTESIAN_POINT('Ctrl Pts',(-22.7629534424542,12.7403852471457,
129.499963464368)) ;
#131916=CARTESIAN_POINT('Ctrl Pts',(-22.8415892215112,12.5401778472151,
129.696554511139)) ;
#131917=CARTESIAN_POINT('Ctrl Pts',(-22.9348979213409,12.4032538731495,
129.936029182917)) ;
#131918=CARTESIAN_POINT('Ctrl Pts',(-23.0370685674519,12.3392654765734,
130.201366375023)) ;
#131919=CARTESIAN_POINT('Ctrl Pts',(-23.141478431911,12.3529795705707,130.473233214815)) ;
#131920=CARTESIAN_POINT('Ctrl Pts',(-23.2412861780916,12.44341496887,130.731668708428)) ;
#131921=CARTESIAN_POINT('Ctrl Pts',(-23.330047912579,12.6038142404483,130.957868037024)) ;
#131922=CARTESIAN_POINT('Ctrl Pts',(-23.4023245485338,12.8232746698558,
131.135851245433)) ;
#131923=CARTESIAN_POINT('Ctrl Pts',(-23.4533693512746,13.0848674095602,
131.251920028465)) ;
#131924=CARTESIAN_POINT('Ctrl Pts',(-23.4806176034136,13.3712340427374,
131.298395105942)) ;
#131925=CARTESIAN_POINT('Ctrl Pts',(-23.4825810779044,13.6620670155129,
131.270922868641)) ;
#131926=CARTESIAN_POINT('Ctrl Pts',(-23.4599091408466,13.9347879219274,
131.171598398464)) ;
#131927=CARTESIAN_POINT('Ctrl Pts',(-23.4149763968351,14.1711547034761,
131.007212926626)) ;
#131928=CARTESIAN_POINT('Ctrl Pts',(-23.3516961209413,14.3538985958079,
130.789228498426)) ;
#131929=CARTESIAN_POINT('Ctrl Pts',(-23.2754093744269,14.4699515410886,
130.533273425003)) ;
#131930=CARTESIAN_POINT('Ctrl Pts',(-23.1921867842084,14.511011729743,130.257027506385)) ;
#131931=CARTESIAN_POINT('Ctrl Pts',(-23.1089561500767,14.4745400421894,
129.980842840064)) ;
#131932=CARTESIAN_POINT('Ctrl Pts',(-23.031552894356,14.3614974996119,129.721369859714)) ;
#131933=CARTESIAN_POINT('Ctrl Pts',(-22.9678477580129,14.1829580277845,
129.502345220066)) ;
#131934=CARTESIAN_POINT('Ctrl Pts',(-22.9216856506781,13.9492404929465,
129.334353763701)) ;
#131935=CARTESIAN_POINT('Ctrl Pts',(-22.8977300159152,13.6775800982586,
129.231228230102)) ;
#131936=CARTESIAN_POINT('Ctrl Pts',(-22.8981933527482,13.3886494635436,
129.19954520776)) ;
#131937=CARTESIAN_POINT('Ctrl Pts',(-22.9242400045738,13.0993478015478,
129.242254988579)) ;
#131938=CARTESIAN_POINT('Ctrl Pts',(-22.9739037222349,12.8369458310676,
129.354415199943)) ;
#131939=CARTESIAN_POINT('Ctrl Pts',(-23.0453252131747,12.6140529768099,
129.529801908795)) ;
#131940=CARTESIAN_POINT('Ctrl Pts',(-23.1330410816671,12.4507323341902,
129.753058144926)) ;
#131941=CARTESIAN_POINT('Ctrl Pts',(-23.2324941335687,12.3558899306528,
130.010420059215)) ;
#131942=CARTESIAN_POINT('Ctrl Pts',(-23.3371521212107,12.3380969081111,
130.282910607247)) ;
#131943=CARTESIAN_POINT('Ctrl Pts',(-23.4390406262999,12.3976016694818,
130.547608591386)) ;
#131944=CARTESIAN_POINT('Ctrl Pts',(-23.5331839274626,12.530583824708,130.789474316628)) ;
#131945=CARTESIAN_POINT('Ctrl Pts',(-23.6129508354768,12.7283490506027,
130.989275182951)) ;
#131946=CARTESIAN_POINT('Ctrl Pts',(-23.6728864226876,12.9742771227128,
131.13136588872)) ;
#131947=CARTESIAN_POINT('Ctrl Pts',(-23.71018774412,13.2539376227601,131.207121504005)) ;
#131948=CARTESIAN_POINT('Ctrl Pts',(-23.7223865299285,13.5450903335013,
131.209633661058)) ;
#131949=CARTESIAN_POINT('Ctrl Pts',(-23.7094914718236,13.8275787514848,
131.138820807372)) ;
#131950=CARTESIAN_POINT('Ctrl Pts',(-23.6732974807833,14.080619519853,131.000028693289)) ;
#131951=CARTESIAN_POINT('Ctrl Pts',(-23.616590785082,14.2877392133105,130.801091824847)) ;
#131952=CARTESIAN_POINT('Ctrl Pts',(-23.5452916636683,14.431213841156,130.559896288173)) ;
#131953=CARTESIAN_POINT('Ctrl Pts',(-23.4637700924587,14.5038738166411,
130.288489711948)) ;
#131954=CARTESIAN_POINT('Ctrl Pts',(-23.3797591259085,14.4984557576167,
130.010000564517)) ;
#131955=CARTESIAN_POINT('Ctrl Pts',(-23.2994671912968,14.4164646825051,
129.742342495005)) ;
#131956=CARTESIAN_POINT('Ctrl Pts',(-23.2292002172557,14.2622140461571,
129.503806387235)) ;
#131957=CARTESIAN_POINT('Ctrl Pts',(-23.1755337197615,14.0497489487789,
129.314087251754)) ;
#131958=CARTESIAN_POINT('Ctrl Pts',(-23.1420903990703,13.7905258352839,
129.183151437944)) ;
#131959=CARTESIAN_POINT('Ctrl Pts',(-23.1325295042077,13.506486494377,129.12218848079)) ;
#131960=CARTESIAN_POINT('Ctrl Pts',(-23.1482921851681,13.2142515667239,
129.134926916223)) ;
#131961=CARTESIAN_POINT('Ctrl Pts',(-23.188353413262,12.9406232851689,129.219102820939)) ;
#131962=CARTESIAN_POINT('Ctrl Pts',(-23.2515823582444,12.6982138740687,
129.370525672368)) ;
#131963=CARTESIAN_POINT('Ctrl Pts',(-23.3330631497147,12.5096112048297,
129.575565311669)) ;
#131964=CARTESIAN_POINT('Ctrl Pts',(-23.4290906890084,12.3850648620669,
129.822774700949)) ;
#131965=CARTESIAN_POINT('Ctrl Pts',(-23.531784997696,12.3359713268051,130.089781167871)) ;
#131966=CARTESIAN_POINT('Ctrl Pts',(-23.6357879798494,12.3641515700291,
130.360476235555)) ;
#131967=CARTESIAN_POINT('Ctrl Pts',(-23.7340953356143,12.4683944776065,
130.614508785511)) ;
#131968=CARTESIAN_POINT('Ctrl Pts',(-23.8203211365081,12.6414744910879,
130.833207334208)) ;
#131969=CARTESIAN_POINT('Ctrl Pts',(-23.8886881736005,12.8692739707259,
130.99991574651)) ;
#131970=CARTESIAN_POINT('Ctrl Pts',(-23.9357467861378,13.1394382839076,
131.104034823546)) ;
#131971=CARTESIAN_POINT('Ctrl Pts',(-23.9579774455155,13.4257125423889,
131.136139167156)) ;
#131972=CARTESIAN_POINT('Ctrl Pts',(-23.9552750237727,13.7153678926771,
131.094978168242)) ;
#131973=CARTESIAN_POINT('Ctrl Pts',(-23.9282090173285,13.9823826092166,
130.982854215722)) ;
#131974=CARTESIAN_POINT('Ctrl Pts',(-23.8793697422226,14.210351268189,130.806979650137)) ;
#131975=CARTESIAN_POINT('Ctrl Pts',(-23.8133153702057,14.3810373513132,
130.58096078673)) ;
#131976=CARTESIAN_POINT('Ctrl Pts',(-23.735209224892,14.4835203874639,130.319669563206)) ;
#131977=CARTESIAN_POINT('Ctrl Pts',(-23.6515414522142,14.5102051470099,
130.042171972968)) ;
#131978=CARTESIAN_POINT('Ctrl Pts',(-23.5684272969825,14.4584272467564,
129.766068717826)) ;
#131979=CARTESIAN_POINT('Ctrl Pts',(-23.4938231437372,14.3332271538461,
129.515148015428)) ;
#131980=CARTESIAN_POINT('Ctrl Pts',(-23.4326135115301,14.1422679027751,
129.303162687106)) ;
#131981=CARTESIAN_POINT('Ctrl Pts',(-23.3905185584406,13.9003526545792,
129.147122527455)) ;
#131982=CARTESIAN_POINT('Ctrl Pts',(-23.3709966570516,13.6237176044633,
129.056941792442)) ;
#131983=CARTESIAN_POINT('Ctrl Pts',(-23.3763211847102,13.3329588361478,
129.039378660403)) ;
#131984=CARTESIAN_POINT('Ctrl Pts',(-23.4068246825045,13.0482791472687,
129.095326134194)) ;
#131985=CARTESIAN_POINT('Ctrl Pts',(-23.4611218639704,12.7905984211716,
129.220781957599)) ;
#131986=CARTESIAN_POINT('Ctrl Pts',(-23.5355417145057,12.5792074314873,
129.405190030391)) ;
#131987=CARTESIAN_POINT('Ctrl Pts',(-23.6262276903051,12.4271420328258,
129.636951252849)) ;
#131988=CARTESIAN_POINT('Ctrl Pts',(-23.72702713312,12.3466854620337,129.898286196702)) ;
#131989=CARTESIAN_POINT('Ctrl Pts',(-23.8314987159718,12.3433384451733,
130.170343083653)) ;
#131990=CARTESIAN_POINT('Ctrl Pts',(-23.9327910170219,12.417256873973,130.433143999051)) ;
#131991=CARTESIAN_POINT('Ctrl Pts',(-24.0245736232509,12.5633304568432,
130.668126155051)) ;
#131992=CARTESIAN_POINT('Ctrl Pts',(-24.1008197720403,12.7708593905581,
130.857750684135)) ;
#131993=CARTESIAN_POINT('Ctrl Pts',(-24.1569294635632,13.025326349885,130.988518737243)) ;
#131994=CARTESIAN_POINT('Ctrl Pts',(-24.1894985627988,13.3082178025067,
131.05053265747)) ;
#131995=CARTESIAN_POINT('Ctrl Pts',(-24.196965740994,13.5990344955289,131.039249671657)) ;
#131996=CARTESIAN_POINT('Ctrl Pts',(-24.1795877670942,13.8774216043795,
130.955375021049)) ;
#131997=CARTESIAN_POINT('Ctrl Pts',(-24.1390939585473,14.1239848990119,
130.803863087357)) ;
#131998=CARTESIAN_POINT('Ctrl Pts',(-24.0794901932382,14.3192776170792,
130.596679031769)) ;
#131999=CARTESIAN_POINT('Ctrl Pts',(-24.0055352361048,14.4507732360595,
130.347522670003)) ;
#132000=CARTESIAN_POINT('Ctrl Pts',(-23.9233178114793,14.5087792678555,
130.074243320989)) ;
#132001=CARTESIAN_POINT('Ctrl Pts',(-23.8391129704671,14.4887238336712,
129.795024289797)) ;
#132002=CARTESIAN_POINT('Ctrl Pts',(-23.7605064372372,14.3928285084541,
129.532382450158)) ;
#132003=CARTESIAN_POINT('Ctrl Pts',(-23.6928180061624,14.2263682040696,
129.30137255382)) ;
#132004=CARTESIAN_POINT('Ctrl Pts',(-23.6426620351328,14.0038696460673,
129.121863214626)) ;
#132005=CARTESIAN_POINT('Ctrl Pts',(-23.613563581647,13.7389372008462,129.003713269081)) ;
#132006=CARTESIAN_POINT('Ctrl Pts',(-23.6086509708226,13.4518073715824,
128.956278206236)) ;
#132007=CARTESIAN_POINT('Ctrl Pts',(-23.6290105898186,13.1616327439453,
128.982551634326)) ;
#132008=CARTESIAN_POINT('Ctrl Pts',(-23.6739522585566,12.8906304372966,
129.080681338749)) ;
#132009=CARTESIAN_POINT('Ctrl Pts',(-23.7407279250101,12.6585325321797,
129.242687250476)) ;
#132010=CARTESIAN_POINT('Ctrl Pts',(-23.8252467089156,12.4808578746759,
129.456558276985)) ;
#132011=CARTESIAN_POINT('Ctrl Pts',(-23.9234212908845,12.369794968941,129.709975426016)) ;
#132012=CARTESIAN_POINT('Ctrl Pts',(-24.0266916219991,12.3353140243209,
129.978700782335)) ;
#132013=CARTESIAN_POINT('Ctrl Pts',(-24.1303332495694,12.3783402005982,
130.248268071055)) ;
#132014=CARTESIAN_POINT('Ctrl Pts',(-24.2265146825975,12.4961137906607,
130.496181048475)) ;
#132015=CARTESIAN_POINT('Ctrl Pts',(-24.3096595921357,12.6800956082709,
130.705970404282)) ;
#132016=CARTESIAN_POINT('Ctrl Pts',(-24.3745179631744,12.9180877152906,
130.862244767084)) ;
#132017=CARTESIAN_POINT('Ctrl Pts',(-24.4167847945233,13.1911275173993,
130.952669619891)) ;
#132018=CARTESIAN_POINT('Ctrl Pts',(-24.4345812423772,13.4815072415882,
130.971518185869)) ;
#132019=CARTESIAN_POINT('Ctrl Pts',(-24.4270213519574,13.7684314308885,
130.916204524826)) ;
#132020=CARTESIAN_POINT('Ctrl Pts',(-24.3956514842814,14.029076308477,130.791530690429)) ;
#132021=CARTESIAN_POINT('Ctrl Pts',(-24.343165506001,14.2473093926041,130.605025756878)) ;
#132022=CARTESIAN_POINT('Ctrl Pts',(-24.2745743047042,14.4057091519906,
130.371660986809)) ;
#132023=CARTESIAN_POINT('Ctrl Pts',(-24.1945925450092,14.4946178708306,
130.104760579953)) ;
#132024=CARTESIAN_POINT('Ctrl Pts',(-24.11071512251,14.5063975208026,129.826695894897)) ;
#132025=CARTESIAN_POINT('Ctrl Pts',(-24.0286060386776,14.4401278585609,
129.553540640394)) ;
#132026=CARTESIAN_POINT('Ctrl Pts',(-23.9562423178897,14.3020001323071,
129.309200756072)) ;
#132027=CARTESIAN_POINT('Ctrl Pts',(-23.8982704981956,14.100380875427,129.106698871819)) ;
#132028=CARTESIAN_POINT('Ctrl Pts',(-23.8601423404147,13.8504602239821,
128.962217821069)) ;
#132029=CARTESIAN_POINT('Ctrl Pts',(-23.8451537683981,13.5690360496352,
128.88522225926)) ;
#132030=CARTESIAN_POINT('Ctrl Pts',(-23.85536903869,13.277347744237,128.881881865911)) ;
#132031=CARTESIAN_POINT('Ctrl Pts',(-23.8903250024146,12.9978265767653,
128.951024979183)) ;
#132032=CARTESIAN_POINT('Ctrl Pts',(-23.9487275671782,12.747023860199,129.088449649182)) ;
#132033=CARTESIAN_POINT('Ctrl Pts',(-24.0267536508702,12.5453431667421,
129.283298823089)) ;
#132034=CARTESIAN_POINT('Ctrl Pts',(-24.1198629233628,12.4062333259034,
129.52213584094)) ;
#132035=CARTESIAN_POINT('Ctrl Pts',(-24.2215666079949,12.3400677949455,
129.786207600519)) ;
#132036=CARTESIAN_POINT('Ctrl Pts',(-24.3264846884265,12.3515722965719,
130.059403729799)) ;
#132037=CARTESIAN_POINT('Ctrl Pts',(-24.4261565993231,12.4396025465946,
130.317564726088)) ;
#132038=CARTESIAN_POINT('Ctrl Pts',(-24.515504520949,12.5983879462257,130.545404926639)) ;
#132039=CARTESIAN_POINT('Ctrl Pts',(-24.5881171815504,12.8155081778463,
130.724487254865)) ;
#132040=CARTESIAN_POINT('Ctrl Pts',(-24.6401896035301,13.0777480891852,
130.8433438272)) ;
#132041=CARTESIAN_POINT('Ctrl Pts',(-24.6679851185762,13.3640007134148,
130.891395810982)) ;
#132042=CARTESIAN_POINT('Ctrl Pts',(-24.6706717433523,13.6530970190172,
130.866255003353)) ;
#132043=CARTESIAN_POINT('Ctrl Pts',(-24.6486810155768,13.9274410550996,
130.768823051012)) ;
#132044=CARTESIAN_POINT('Ctrl Pts',(-24.6043588117149,14.1649405448642,
130.60624558075)) ;
#132045=CARTESIAN_POINT('Ctrl Pts',(-24.5413708101056,14.3499176915205,
130.389027795027)) ;
#132046=CARTESIAN_POINT('Ctrl Pts',(-24.4653494690363,14.4676736740884,
130.133852904625)) ;
#132047=CARTESIAN_POINT('Ctrl Pts',(-24.3825873013246,14.5109849198275,
129.859094894237)) ;
#132048=CARTESIAN_POINT('Ctrl Pts',(-24.2987925768636,14.4763368011369,
129.58106163939)) ;
#132049=CARTESIAN_POINT('Ctrl Pts',(-24.2217612201684,14.3664425274482,
129.322969701944)) ;
#132050=CARTESIAN_POINT('Ctrl Pts',(-24.1570057110458,14.1882602546085,
129.100578369949)) ;
#132051=CARTESIAN_POINT('Ctrl Pts',(-24.1105157071068,13.9563928712726,
128.931742068379)) ;
#132052=CARTESIAN_POINT('Ctrl Pts',(-24.0858458393616,13.6856075071528,
128.826527819527)) ;
#132053=CARTESIAN_POINT('Ctrl Pts',(-24.0856539585114,13.3967978155194,
128.792918629269)) ;
#132054=CARTESIAN_POINT('Ctrl Pts',(-24.1107926076059,13.1083772147109,
128.833125740032)) ;
#132055=CARTESIAN_POINT('Ctrl Pts',(-24.1600137825134,12.8436201216384,
128.943820657913)) ;
#132056=CARTESIAN_POINT('Ctrl Pts',(-24.2308058798189,12.6197329650473,
129.117423409396)) ;
#132057=CARTESIAN_POINT('Ctrl Pts',(-24.3182751718309,12.4541610182818,
129.339893353894)) ;
#132058=CARTESIAN_POINT('Ctrl Pts',(-24.4176896908462,12.3575181073951,
129.59708909666)) ;
#132059=CARTESIAN_POINT('Ctrl Pts',(-24.5213942641841,12.337407534574,129.86708474398)) ;
#132060=CARTESIAN_POINT('Ctrl Pts',(-24.6242611097352,12.3950240477661,
130.134369464736)) ;
#132061=CARTESIAN_POINT('Ctrl Pts',(-24.7182893080511,12.5255974682326,
130.376052536827)) ;
#132062=CARTESIAN_POINT('Ctrl Pts',(-24.7987860343519,12.7221236513144,
130.577891266987)) ;
#132063=CARTESIAN_POINT('Ctrl Pts',(-24.8592668458931,12.966643820031,130.721612719223)) ;
#132064=CARTESIAN_POINT('Ctrl Pts',(-24.8973477603996,13.2467842966359,
130.799514303858)) ;
#132065=CARTESIAN_POINT('Ctrl Pts',(-24.9101357439362,13.5364084867458,
130.803917200582)) ;
#132066=CARTESIAN_POINT('Ctrl Pts',(-24.8980433329888,13.819301352246,130.735470391269)) ;
#132067=CARTESIAN_POINT('Ctrl Pts',(-24.8624508729161,14.0737430594077,
130.598397208659)) ;
#132068=CARTESIAN_POINT('Ctrl Pts',(-24.8063650001413,14.2823383256047,
130.401314654759)) ;
#132069=CARTESIAN_POINT('Ctrl Pts',(-24.7352153152331,14.4280819786068,
130.160457808913)) ;
#132070=CARTESIAN_POINT('Ctrl Pts',(-24.654277110767,14.5027907188546,129.890917785084)) ;
#132071=CARTESIAN_POINT('Ctrl Pts',(-24.569599491767,14.4996009182714,129.610218523976)) ;
#132072=CARTESIAN_POINT('Ctrl Pts',(-24.4895659727805,14.4198435135005,
129.343494691889)) ;
#132073=CARTESIAN_POINT('Ctrl Pts',(-24.4190126879205,14.2682255575811,
129.104196361098)) ;
#132074=CARTESIAN_POINT('Ctrl Pts',(-24.364598178107,14.0566692320112,128.91218100257)) ;
#132075=CARTESIAN_POINT('Ctrl Pts',(-24.3305009683015,13.7984046917339,
128.779328284604)) ;
#132076=CARTESIAN_POINT('Ctrl Pts',(-24.3202768420663,13.5146255183712,
128.716401612773)) ;
#132077=CARTESIAN_POINT('Ctrl Pts',(-24.3351461344103,13.22379017507,128.726708255358)) ;
#132078=CARTESIAN_POINT('Ctrl Pts',(-24.3747056074861,12.9476430099182,
128.809207275973)) ;
#132079=CARTESIAN_POINT('Ctrl Pts',(-24.4373988447194,12.7041858709694,
128.959075140171)) ;
#132080=CARTESIAN_POINT('Ctrl Pts',(-24.5182754986541,12.5142908380612,
129.162405255088)) ;
#132081=CARTESIAN_POINT('Ctrl Pts',(-24.6137660742652,12.3877724329813,
129.408115006488)) ;
#132082=CARTESIAN_POINT('Ctrl Pts',(-24.7167971690515,12.3361912043238,
129.675956387308)) ;
#132083=CARTESIAN_POINT('Ctrl Pts',(-24.8208049085079,12.3624798224069,
129.946681899111)) ;
#132084=CARTESIAN_POINT('Ctrl Pts',(-24.9189695732058,12.4640688022784,
130.200435824458)) ;
#132085=CARTESIAN_POINT('Ctrl Pts',(-25.005956640633,12.6358046245907,130.421244636591)) ;
#132086=CARTESIAN_POINT('Ctrl Pts',(-25.0747012664645,12.862048858162,130.589103084132)) ;
#132087=CARTESIAN_POINT('Ctrl Pts',(-25.1223375525266,13.1294243703739,
130.69512008432)) ;
#132088=CARTESIAN_POINT('Ctrl Pts',(-25.1455445896858,13.419127554444,130.729642616116)) ;
#132089=CARTESIAN_POINT('Ctrl Pts',(-25.1435152363736,13.7060585256719,
130.690801967982)) ;
#132090=CARTESIAN_POINT('Ctrl Pts',(-25.1170308827865,13.9758635071568,
130.580144935401)) ;
#132091=CARTESIAN_POINT('Ctrl Pts',(-25.0688142460135,14.2044690811379,
130.40618368144)) ;
#132092=CARTESIAN_POINT('Ctrl Pts',(-25.003123247664,14.3772046466544,130.18118138791)) ;
#132093=CARTESIAN_POINT('Ctrl Pts',(-24.9252844700022,14.4817041640368,
129.920684773534)) ;
#132094=CARTESIAN_POINT('Ctrl Pts',(-24.8415989541778,14.5103977605507,
129.643097336818)) ;
#132095=CARTESIAN_POINT('Ctrl Pts',(-24.7589132492041,14.461387716176,129.368476107022)) ;
#132096=CARTESIAN_POINT('Ctrl Pts',(-24.6835796855055,14.3378670523305,
129.115253926662)) ;
#132097=CARTESIAN_POINT('Ctrl Pts',(-24.6219712562161,14.1487649480966,
128.902143850339)) ;
#132098=CARTESIAN_POINT('Ctrl Pts',(-24.5791815584349,13.9077124472436,
128.744012805924)) ;
#132099=CARTESIAN_POINT('Ctrl Pts',(-24.5590011432879,13.6318349091011,
128.651919455676)) ;
#132100=CARTESIAN_POINT('Ctrl Pts',(-24.5636129562954,13.3411961915081,
128.632272182411)) ;
#132101=CARTESIAN_POINT('Ctrl Pts',(-24.5933692421231,13.0563347009616,
128.686073174335)) ;
#132102=CARTESIAN_POINT('Ctrl Pts',(-24.6470060166101,12.7976622253545,
128.809603060301)) ;
#132103=CARTESIAN_POINT('Ctrl Pts',(-24.7208016129616,12.584625305209,128.992205539617)) ;
#132104=CARTESIAN_POINT('Ctrl Pts',(-24.8118536009071,12.429833286881,129.224781939929)) ;
#132105=CARTESIAN_POINT('Ctrl Pts',(-24.911545430168,12.3481748757021,129.483189757942)) ;
#132106=CARTESIAN_POINT('Ctrl Pts',(-25.0164125625319,12.3422836205948,
129.75626651559)) ;
#132107=CARTESIAN_POINT('Ctrl Pts',(-25.117816306108,12.414162317258,130.019416608038)) ;
#132108=CARTESIAN_POINT('Ctrl Pts',(-25.2100635855326,12.55849168118,130.255714929222)) ;
#132109=CARTESIAN_POINT('Ctrl Pts',(-25.2867433505999,12.7644624942609,
130.446624226534)) ;
#132110=CARTESIAN_POINT('Ctrl Pts',(-25.3433959651672,13.0174115077838,
130.579031809203)) ;
#132111=CARTESIAN_POINT('Ctrl Pts',(-25.3766991434267,13.2998964348547,
130.643172314106)) ;
#132112=CARTESIAN_POINT('Ctrl Pts',(-25.3849027762527,13.5908799629275,
130.634029729427)) ;
#132113=CARTESIAN_POINT('Ctrl Pts',(-25.3681244270798,13.8706960081611,
130.551809717868)) ;
#132114=CARTESIAN_POINT('Ctrl Pts',(-25.3281885696402,14.1180202656557,
130.401959719847)) ;
#132115=CARTESIAN_POINT('Ctrl Pts',(-25.2692654377525,14.3143765894564,
130.196866938718)) ;
#132116=CARTESIAN_POINT('Ctrl Pts',(-25.1954627990625,14.4481660809184,
129.948075722546)) ;
#132117=CARTESIAN_POINT('Ctrl Pts',(-25.1135963031033,14.5080838606745,
129.675906827394)) ;
#132118=CARTESIAN_POINT('Ctrl Pts',(-25.0294161558255,14.4905518531177,
129.396790506061)) ;
#132119=CARTESIAN_POINT('Ctrl Pts',(-24.9503166631056,14.3964092296967,
129.132598410075)) ;
#132120=CARTESIAN_POINT('Ctrl Pts',(-24.8824484698929,14.232304987228,128.901173407916)) ;
#132121=CARTESIAN_POINT('Ctrl Pts',(-24.831656485841,14.0113006854444,128.719789796304)) ;
#132122=CARTESIAN_POINT('Ctrl Pts',(-24.8018618709668,13.7469853282518,
128.599564702445)) ;
#132123=CARTESIAN_POINT('Ctrl Pts',(-24.7961937055128,13.4601451324146,
128.54991646717)) ;
#132124=CARTESIAN_POINT('Ctrl Pts',(-24.8160226315964,13.1687003200991,
128.574510511953)) ;
#132125=CARTESIAN_POINT('Ctrl Pts',(-24.859902739483,12.8989650919222,128.669805113981)) ;
#132126=CARTESIAN_POINT('Ctrl Pts',(-24.9266168659618,12.6635916504989,
128.831356633498)) ;
#132127=CARTESIAN_POINT('Ctrl Pts',(-25.0103639202873,12.485239800862,129.043133485935)) ;
#132128=CARTESIAN_POINT('Ctrl Pts',(-25.1082951885594,12.3719259500599,
129.295815313463)) ;
#132129=CARTESIAN_POINT('Ctrl Pts',(-25.2113378058678,12.3351771032852,
129.563924734244)) ;
#132130=CARTESIAN_POINT('Ctrl Pts',(-25.3153987713946,12.3762351050997,
129.834608633564)) ;
#132131=CARTESIAN_POINT('Ctrl Pts',(-25.4113691303234,12.4911992435135,
130.082089209234)) ;
#132132=CARTESIAN_POINT('Ctrl Pts',(-25.4955318190917,12.6745749260732,
130.29463045715)) ;
#132133=CARTESIAN_POINT('Ctrl Pts',(-25.560704508805,12.9105841176317,130.451940846143)) ;
#132134=CARTESIAN_POINT('Ctrl Pts',(-25.6037591586016,13.1834575472762,
130.544589177351)) ;
#132135=CARTESIAN_POINT('Ctrl Pts',(-25.6221540731369,13.4728172007292,
130.565280977399)) ;
#132136=CARTESIAN_POINT('Ctrl Pts',(-25.6154890774634,13.7593252111675,
130.512691578256)) ;
#132137=CARTESIAN_POINT('Ctrl Pts',(-25.5845017414514,14.0229111380707,
130.388875573167)) ;
#132138=CARTESIAN_POINT('Ctrl Pts',(-25.5329646548234,14.2409568530166,
130.205405121793)) ;
#132139=CARTESIAN_POINT('Ctrl Pts',(-25.4643492210366,14.4024702596202,
129.971739445436)) ;
#132140=CARTESIAN_POINT('Ctrl Pts',(-25.3848249850593,14.4930252918819,
129.706290426526)) ;
#132141=CARTESIAN_POINT('Ctrl Pts',(-25.3009346998094,14.5071138077779,
129.428162516891)) ;
#132142=CARTESIAN_POINT('Ctrl Pts',(-25.2189936227422,14.4434722304718,
129.155638517111)) ;
#132143=CARTESIAN_POINT('Ctrl Pts',(-25.1460018098747,14.3072991508372,
128.909365963459)) ;
#132144=CARTESIAN_POINT('Ctrl Pts',(-25.0872927957611,14.1061281755834,
128.704547183538)) ;
#132145=CARTESIAN_POINT('Ctrl Pts',(-25.0487858755379,13.8584458365122,
128.559117426276)) ;
#132146=CARTESIAN_POINT('Ctrl Pts',(-25.0330304801592,13.5782527615593,
128.479942965013)) ;
#132147=CARTESIAN_POINT('Ctrl Pts',(-25.0424542208566,13.2862405830432,
128.474252693863)) ;
#132148=CARTESIAN_POINT('Ctrl Pts',(-25.0767412324267,13.0054673407222,
128.541371132674)) ;
#132149=CARTESIAN_POINT('Ctrl Pts',(-25.1348051000407,12.7527978446706,
128.67768872235)) ;
#132150=CARTESIAN_POINT('Ctrl Pts',(-25.2119030388808,12.5507722085017,
128.870018404504)) ;
#132151=CARTESIAN_POINT('Ctrl Pts',(-25.3047050008252,12.4092693590586,
129.107923829017)) ;
#132152=CARTESIAN_POINT('Ctrl Pts',(-25.406443595545,12.3409406073707,129.37203421041)) ;
#132153=CARTESIAN_POINT('Ctrl Pts',(-25.5110390200225,12.3499819194409,
129.644402105975)) ;
#132154=CARTESIAN_POINT('Ctrl Pts',(-25.6114390222507,12.4363532158425,
129.904516274518)) ;
#132155=CARTESIAN_POINT('Ctrl Pts',(-25.7007310200177,12.5925663631045,
130.132357144071)) ;
#132156=CARTESIAN_POINT('Ctrl Pts',(-25.7740950725506,12.8085170384963,
130.313559518156)) ;
#132157=CARTESIAN_POINT('Ctrl Pts',(-25.8267351162025,13.0694866152918,
130.434112913458)) ;
#132158=CARTESIAN_POINT('Ctrl Pts',(-25.8553312907165,13.3550371201656,
130.48453070364)) ;
#132159=CARTESIAN_POINT('Ctrl Pts',(-25.8586885366147,13.6462143005165,
130.461126760816)) ;
#132160=CARTESIAN_POINT('Ctrl Pts',(-25.837444412916,13.9195287631536,130.366084906634)) ;
#132161=CARTESIAN_POINT('Ctrl Pts',(-25.7937488394422,14.1586150899391,
130.205310735235)) ;
#132162=CARTESIAN_POINT('Ctrl Pts',(-25.7313611315605,14.3449689837057,
129.989913913384)) ;
#132163=CARTESIAN_POINT('Ctrl Pts',(-25.6556964572195,14.465239738532,129.735783996914)) ;
#132164=CARTESIAN_POINT('Ctrl Pts',(-25.5723964230934,14.5107689866746,
129.459195604095)) ;
#132165=CARTESIAN_POINT('Ctrl Pts',(-25.4893174125801,14.4787461978325,
129.183580822489)) ;
#132166=CARTESIAN_POINT('Ctrl Pts',(-25.4113051186338,14.3700644324197,
128.922314853824)) ;
#132167=CARTESIAN_POINT('Ctrl Pts',(-25.3465909420863,14.1946408166751,
128.700275185896)) ;
#132168=CARTESIAN_POINT('Ctrl Pts',(-25.299369271165,13.963907732595,128.529234819729)) ;
#132169=CARTESIAN_POINT('Ctrl Pts',(-25.2739922523,13.6940409321305,128.421969041019)) ;
#132170=CARTESIAN_POINT('Ctrl Pts',(-25.2731534451911,13.4043243937501,
128.386332734542)) ;
#132171=CARTESIAN_POINT('Ctrl Pts',(-25.2973628386527,13.1175424358185,
128.424062655725)) ;
#132172=CARTESIAN_POINT('Ctrl Pts',(-25.3462006392316,12.8501254079525,
128.533419495547)) ;
#132173=CARTESIAN_POINT('Ctrl Pts',(-25.4160919098287,12.6260375389968,
128.704569775621)) ;
#132174=CARTESIAN_POINT('Ctrl Pts',(-25.5032418915579,12.4581545252769,
128.926046604269)) ;
#132175=CARTESIAN_POINT('Ctrl Pts',(-25.6021785519615,12.3594525497003,
129.181922681907)) ;
#132176=CARTESIAN_POINT('Ctrl Pts',(-25.7061730224389,12.3367944069397,
129.452652747223)) ;
#132177=CARTESIAN_POINT('Ctrl Pts',(-25.8094492173163,12.3925085409291,
129.721047874811)) ;
#132178=CARTESIAN_POINT('Ctrl Pts',(-25.9037624326914,12.5213898755188,
129.963557213451)) ;
#132179=CARTESIAN_POINT('Ctrl Pts',(-25.9844805178092,12.7155724021421,
130.166157205425)) ;
#132180=CARTESIAN_POINT('Ctrl Pts',(-26.0456691934443,12.9595220676015,
130.311865673155)) ;
#132181=CARTESIAN_POINT('Ctrl Pts',(-26.0842093042236,13.2367788940881,
130.391368626224)) ;
#132182=CARTESIAN_POINT('Ctrl Pts',(-26.0979544525776,13.5277643625836,
130.39839898417)) ;
#132183=CARTESIAN_POINT('Ctrl Pts',(-26.0864824258526,13.8120453761231,
130.331665108325)) ;
#132184=CARTESIAN_POINT('Ctrl Pts',(-26.05142082645,14.0676654739834,130.196112404188)) ;
#132185=CARTESIAN_POINT('Ctrl Pts',(-25.9959721958356,14.2771419928287,
130.000979869832)) ;
#132186=CARTESIAN_POINT('Ctrl Pts',(-25.9251922030581,14.425031880978,129.761195796767)) ;
#132187=CARTESIAN_POINT('Ctrl Pts',(-25.8440763649555,14.5017260060049,
129.490996412094)) ;
#132188=CARTESIAN_POINT('Ctrl Pts',(-25.7603662435499,14.5010099059246,
129.213512691512)) ;
#132189=CARTESIAN_POINT('Ctrl Pts',(-25.6794136560246,14.4231233705973,
128.943812915352)) ;
#132190=CARTESIAN_POINT('Ctrl Pts',(-25.6086694413268,14.2735700722065,
128.704038175328)) ;
#132191=CARTESIAN_POINT('Ctrl Pts',(-25.5536232001884,14.0631260843178,
128.510103402269)) ;
#132192=CARTESIAN_POINT('Ctrl Pts',(-25.5190005221295,13.8068513237717,
128.37583898455)) ;
#132193=CARTESIAN_POINT('Ctrl Pts',(-25.5079988886962,13.5229068768556,
128.310556815572)) ;
#132194=CARTESIAN_POINT('Ctrl Pts',(-25.522136912891,13.2323185296325,128.31877011903)) ;
#132195=CARTESIAN_POINT('Ctrl Pts',(-25.5609778387885,12.955462422634,128.399168054502)) ;
#132196=CARTESIAN_POINT('Ctrl Pts',(-25.622981897995,12.7108337306576,128.547046303102)) ;
#132197=CARTESIAN_POINT('Ctrl Pts',(-25.7035387876594,12.5189036902296,
128.749376462235)) ;
#132198=CARTESIAN_POINT('Ctrl Pts',(-25.7983973245378,12.3906586207823,
128.993347141695)) ;
#132199=CARTESIAN_POINT('Ctrl Pts',(-25.9014394205249,12.3366531336248,
129.261165642822)) ;
#132200=CARTESIAN_POINT('Ctrl Pts',(-26.0053503635526,12.360297772879,129.531671267842)) ;
#132201=CARTESIAN_POINT('Ctrl Pts',(-26.1046179703446,12.4609988515391,
129.788341417843)) ;
#132202=CARTESIAN_POINT('Ctrl Pts',(-26.1910706407531,12.6291274638668,
130.0079564874)) ;
#132203=CARTESIAN_POINT('Ctrl Pts',(-26.2610067862353,12.8555169755094,
130.179031109569)) ;
#132204=CARTESIAN_POINT('Ctrl Pts',(-26.3090567054831,13.1215885522129,
130.286335393292)) ;
#132205=CARTESIAN_POINT('Ctrl Pts',(-26.3329796835872,13.4096083938423,
130.323096945283)) ;
#132206=CARTESIAN_POINT('Ctrl Pts',(-26.3317340747676,13.698212942693,130.286391172774)) ;
#132207=CARTESIAN_POINT('Ctrl Pts',(-26.3058007346478,13.9691452295141,
130.177299627734)) ;
#132208=CARTESIAN_POINT('Ctrl Pts',(-26.2583066398341,14.1982918407705,
130.005562251346)) ;
#132209=CARTESIAN_POINT('Ctrl Pts',(-26.1931751350795,14.3728095621698,
129.782233989023)) ;
#132210=CARTESIAN_POINT('Ctrl Pts',(-26.1155255616385,14.479662285758,129.522250222093)) ;
#132211=CARTESIAN_POINT('Ctrl Pts',(-26.0318486038747,14.5107460879228,
129.244664158376)) ;
#132212=CARTESIAN_POINT('Ctrl Pts',(-25.9488165487381,14.4636147982726,
128.968932999966)) ;
#132213=CARTESIAN_POINT('Ctrl Pts',(-25.8735146658894,14.3427084720644,
128.715956195703)) ;
#132214=CARTESIAN_POINT('Ctrl Pts',(-25.811125852612,14.1545214106307,128.500410033898)) ;
#132215=CARTESIAN_POINT('Ctrl Pts',(-25.767859635489,13.914665784431,128.340908123874)) ;
#132216=CARTESIAN_POINT('Ctrl Pts',(-25.7470531048229,13.6405172708492,
128.247102795506)) ;
#132217=CARTESIAN_POINT('Ctrl Pts',(-25.7508957888745,13.3501102818962,
128.225215226321)) ;
#132218=CARTESIAN_POINT('Ctrl Pts',(-25.7797927372613,13.0651843315454,
128.276561420719)) ;
#132219=CARTESIAN_POINT('Ctrl Pts',(-25.8330708547357,12.80388772374,128.398847085602)) ;
#132220=CARTESIAN_POINT('Ctrl Pts',(-25.9063371941856,12.5899465270377,
128.579947959411)) ;
#132221=CARTESIAN_POINT('Ctrl Pts',(-25.9963126660368,12.4339563210189,
128.809607064104)) ;
#132222=CARTESIAN_POINT('Ctrl Pts',(-26.0966203558645,12.3491846989202,
129.069534053189)) ;
#132223=CARTESIAN_POINT('Ctrl Pts',(-26.2015343109458,12.3415474281895,
129.342731765695)) ;
#132224=CARTESIAN_POINT('Ctrl Pts',(-26.3027211617629,12.4110292201394,
129.60537279447)) ;
#132225=CARTESIAN_POINT('Ctrl Pts',(-26.3953588574291,12.5533605448057,
129.842803792173)) ;
#132226=CARTESIAN_POINT('Ctrl Pts',(-26.4724658228993,12.7574391512257,
130.035002583383)) ;
#132227=CARTESIAN_POINT('Ctrl Pts',(-26.5299060950814,13.0095817126533,
130.169659341123)) ;
#132228=CARTESIAN_POINT('Ctrl Pts',(-26.5639504532064,13.2928226801242,
130.235818361087)) ;
#132229=CARTESIAN_POINT('Ctrl Pts',(-26.5727935985865,13.5820119966617,
130.228755567199)) ;
#132230=CARTESIAN_POINT('Ctrl Pts',(-26.5567072828717,13.8633229249982,
130.148453208055)) ;
#132231=CARTESIAN_POINT('Ctrl Pts',(-26.5174678494182,14.1112602779132,
130.000718041267)) ;
#132232=CARTESIAN_POINT('Ctrl Pts',(-26.4589493371831,14.3095521754014,
129.79675027408)) ;
#132233=CARTESIAN_POINT('Ctrl Pts',(-26.3857504408749,14.4451057235358,
129.549834730436)) ;
#132234=CARTESIAN_POINT('Ctrl Pts',(-26.3033581527554,14.5076745769451,
129.275854508276)) ;
#132235=CARTESIAN_POINT('Ctrl Pts',(-26.2193621817028,14.4918702514085,
128.997365975633)) ;
#132236=CARTESIAN_POINT('Ctrl Pts',(-26.1403227598029,14.4001695900989,
128.733462893607)) ;
#132237=CARTESIAN_POINT('Ctrl Pts',(-26.0720785017029,14.238339270588,128.500982256028)) ;
#132238=CARTESIAN_POINT('Ctrl Pts',(-26.0205445494064,14.0178457541506,
128.317291271494)) ;
#132239=CARTESIAN_POINT('Ctrl Pts',(-25.9901309545097,13.7549024704848,
128.195319458128)) ;
#132240=CARTESIAN_POINT('Ctrl Pts',(-25.9838907425677,13.4669383655623,
128.143823454231)) ;
#132241=CARTESIAN_POINT('Ctrl Pts',(-26.002625472959,13.1792878389568,128.165694781332)) ;
#132242=CARTESIAN_POINT('Ctrl Pts',(-26.0462578585361,12.9054935275296,
128.259864888277)) ;
#132243=CARTESIAN_POINT('Ctrl Pts',(-26.1117838862911,12.6708451835732,
128.418257412013)) ;
#132244=CARTESIAN_POINT('Ctrl Pts',(-26.1958394673662,12.4890109361581,
128.630614971608)) ;
#132245=CARTESIAN_POINT('Ctrl Pts',(-26.292450313642,12.3747427440592,128.879802823841)) ;
#132246=CARTESIAN_POINT('Ctrl Pts',(-26.3961466629634,12.335118127865,129.149563628382)) ;
#132247=CARTESIAN_POINT('Ctrl Pts',(-26.4997927945682,12.3735357257966,
129.41921706946)) ;
#132248=CARTESIAN_POINT('Ctrl Pts',(-26.5970562066531,12.4876827050984,
129.670119063763)) ;
#132249=CARTESIAN_POINT('Ctrl Pts',(-26.6809623236233,12.668143871092,129.882175659137)) ;
#132250=CARTESIAN_POINT('Ctrl Pts',(-26.7469567383412,12.9033827829949,
130.041784506141)) ;
#132251=CARTESIAN_POINT('Ctrl Pts',(-26.7905248136644,13.1743601664502,
130.136070712378)) ;
#132252=CARTESIAN_POINT('Ctrl Pts',(-26.8098089341939,13.4644840041335,
130.159245371207)) ;
#132253=CARTESIAN_POINT('Ctrl Pts',(-26.8037407483827,13.7518155739233,
130.108342116625)) ;
#132254=CARTESIAN_POINT('Ctrl Pts',(-26.7736744947239,14.0147480425275,
129.987433665233)) ;
#132255=CARTESIAN_POINT('Ctrl Pts',(-26.7224117937105,14.2359322469135,
129.804543108639)) ;
#132256=CARTESIAN_POINT('Ctrl Pts',(-26.6540459121311,14.3990328419962,
129.571575856472)) ;
#132257=CARTESIAN_POINT('Ctrl Pts',(-26.5752101350165,14.4913721211862,
129.308326055989)) ;
#132258=CARTESIAN_POINT('Ctrl Pts',(-26.4908765753451,14.5077030613306,
129.028705274742)) ;
#132259=CARTESIAN_POINT('Ctrl Pts',(-26.4092296365473,14.4466726935246,
128.757236988289)) ;
#132260=CARTESIAN_POINT('Ctrl Pts',(-26.3352722351391,14.3110620977678,
128.507833953029)) ;
#132261=CARTESIAN_POINT('Ctrl Pts',(-26.2766889458892,14.1132680684101,
128.303711145387)) ;
#132262=CARTESIAN_POINT('Ctrl Pts',(-26.2372639174626,13.8656264960883,
128.15541845975)) ;
#132263=CARTESIAN_POINT('Ctrl Pts',(-26.2209130537975,13.5853317318957,
128.074439710367)) ;
#132264=CARTESIAN_POINT('Ctrl Pts',(-26.2296856924358,13.2939513094312,
128.066914197785)) ;
#132265=CARTESIAN_POINT('Ctrl Pts',(-26.2631798636915,13.0136081090702,
128.131828211089)) ;
#132266=CARTESIAN_POINT('Ctrl Pts',(-26.3203316415523,12.7604084565328,
128.265584239078)) ;
#132267=CARTESIAN_POINT('Ctrl Pts',(-26.397246993967,12.5556140537718,128.457218817256)) ;
#132268=CARTESIAN_POINT('Ctrl Pts',(-26.4898764488098,12.412162783817,128.694571316763)) ;
#132269=CARTESIAN_POINT('Ctrl Pts',(-26.5911530122536,12.3419224833159,
128.957426665658)) ;
#132270=CARTESIAN_POINT('Ctrl Pts',(-26.6956543409951,12.3485705631489,
129.229554057824)) ;
#132271=CARTESIAN_POINT('Ctrl Pts',(-26.7962358912617,12.4325162173742,
129.490217635024)) ;
#132272=CARTESIAN_POINT('Ctrl Pts',(-26.8862177213639,12.5872706018155,
129.719968083883)) ;
#132273=CARTESIAN_POINT('Ctrl Pts',(-26.9600298412944,12.8016741765326,
129.902501376654)) ;
#132274=CARTESIAN_POINT('Ctrl Pts',(-27.0132363984096,13.0608926757193,
130.024793668328)) ;
#132275=CARTESIAN_POINT('Ctrl Pts',(-27.0426146311277,13.3463627388947,
130.077448217005)) ;
#132276=CARTESIAN_POINT('Ctrl Pts',(-27.0467658686963,13.6367413735624,
130.056476137218)) ;
#132277=CARTESIAN_POINT('Ctrl Pts',(-27.0262045189193,13.912123441329,129.96328026669)) ;
#132278=CARTESIAN_POINT('Ctrl Pts',(-26.9829610646689,14.1528033236638,
129.803766513539)) ;
#132279=CARTESIAN_POINT('Ctrl Pts',(-26.9212047054132,14.3402810134416,
129.590308052972)) ;
#132280=CARTESIAN_POINT('Ctrl Pts',(-26.8459513519056,14.4626257099404,
129.33741374041)) ;
#132281=CARTESIAN_POINT('Ctrl Pts',(-26.7626484303445,14.5106364099982,
129.060769517447)) ;
#132282=CARTESIAN_POINT('Ctrl Pts',(-26.6793325739832,14.4805445966973,
128.784392296914)) ;
#132283=CARTESIAN_POINT('Ctrl Pts',(-26.6015120722546,14.3748126779467,
128.523896403084)) ;
#132284=CARTESIAN_POINT('Ctrl Pts',(-26.5360012381168,14.2005693776624,
128.299367371948)) ;
#132285=CARTESIAN_POINT('Ctrl Pts',(-26.4882466006821,13.9714224956824,
128.126808943075)) ;
#132286=CARTESIAN_POINT('Ctrl Pts',(-26.4621696395529,13.7016038456452,
128.017397936684)) ;
#132287=CARTESIAN_POINT('Ctrl Pts',(-26.4605573044593,13.4137877720204,
127.979694610522)) ;
#132288=CARTESIAN_POINT('Ctrl Pts',(-26.4842037814474,13.1249621059971,
128.015572519599)) ;
#132289=CARTESIAN_POINT('Ctrl Pts',(-26.5319266616535,12.858759801946,128.121953585796)) ;
#132290=CARTESIAN_POINT('Ctrl Pts',(-26.601763218089,12.6311849064932,128.292661018411)) ;
#132291=CARTESIAN_POINT('Ctrl Pts',(-26.6883690358658,12.4620614418067,
128.512623702752)) ;
#132292=CARTESIAN_POINT('Ctrl Pts',(-26.7871596601743,12.3611529243014,
128.768034196029)) ;
#132293=CARTESIAN_POINT('Ctrl Pts',(-26.8908594338048,12.336402737043,129.037980194775)) ;
#132294=CARTESIAN_POINT('Ctrl Pts',(-26.9942677499415,12.3896954767389,
129.30676634427)) ;
#132295=CARTESIAN_POINT('Ctrl Pts',(-27.0891228503658,12.5169545730866,
129.550776904504)) ;
#132296=CARTESIAN_POINT('Ctrl Pts',(-27.170110122641,12.7090014500136,129.754247695197)) ;
#132297=CARTESIAN_POINT('Ctrl Pts',(-27.2319803579197,12.9518209129291,
129.901923479105)) ;
#132298=CARTESIAN_POINT('Ctrl Pts',(-27.2712167263555,13.2283911259786,
129.983462395853)) ;
#132299=CARTESIAN_POINT('Ctrl Pts',(-27.2856848450787,13.5192444476926,
129.992606198651)) ;
#132300=CARTESIAN_POINT('Ctrl Pts',(-27.2749998341,13.8035929406365,129.928231036212)) ;
#132301=CARTESIAN_POINT('Ctrl Pts',(-27.2405107086992,14.0607675161601,
129.794281704174)) ;
#132302=CARTESIAN_POINT('Ctrl Pts',(-27.1859404561386,14.2709776513911,
129.601886944103)) ;
#132303=CARTESIAN_POINT('Ctrl Pts',(-27.1150473623168,14.4220258151157,
129.36152624086)) ;
#132304=CARTESIAN_POINT('Ctrl Pts',(-27.0343785010806,14.5004899933202,
129.09274938976)) ;
#132305=CARTESIAN_POINT('Ctrl Pts',(-26.950535069012,14.5020985766214,128.814815907977)) ;
#132306=CARTESIAN_POINT('Ctrl Pts',(-26.8695870479016,14.426667623352,128.545218407416)) ;
#132307=CARTESIAN_POINT('Ctrl Pts',(-26.798211588555,14.2786158189735,128.303482030973)) ;
#132308=CARTESIAN_POINT('Ctrl Pts',(-26.7426992360049,14.0697690186074,
128.108208750919)) ;
#132309=CARTESIAN_POINT('Ctrl Pts',(-26.7074412852036,13.8142976320865,
127.972057291302)) ;
#132310=CARTESIAN_POINT('Ctrl Pts',(-26.6957645215905,13.5318062075926,
127.904912693824)) ;
#132311=CARTESIAN_POINT('Ctrl Pts',(-26.7091353370237,13.2403761874523,
127.91080130822)) ;
#132312=CARTESIAN_POINT('Ctrl Pts',(-26.74755505738,12.9618561593774,127.989837070354)) ;
#132313=CARTESIAN_POINT('Ctrl Pts',(-26.8086943560285,12.7173263730279,
128.135355225743)) ;
#132314=CARTESIAN_POINT('Ctrl Pts',(-26.8888831517,12.5233446886838,128.33655295725)) ;
#132315=CARTESIAN_POINT('Ctrl Pts',(-26.9835011120047,12.3931312315505,
128.579802503126)) ;
#132316=CARTESIAN_POINT('Ctrl Pts',(-27.0865721816442,12.337075246258,128.847656402371)) ;
#132317=CARTESIAN_POINT('Ctrl Pts',(-27.1901303578273,12.3586764449227,
129.117256451724)) ;
#132318=CARTESIAN_POINT('Ctrl Pts',(-27.2892091804132,12.4563696314589,
129.373537084527)) ;
#132319=CARTESIAN_POINT('Ctrl Pts',(-27.3766437558911,12.6234424170359,
129.595825398964)) ;
#132320=CARTESIAN_POINT('Ctrl Pts',(-27.447072154312,12.8484690314232,129.768349176844)) ;
#132321=CARTESIAN_POINT('Ctrl Pts',(-27.4958104255805,13.1134860607375,
129.877675494575)) ;
#132322=CARTESIAN_POINT('Ctrl Pts',(-27.5204851717528,13.402425050447,129.916492772369)) ;
#132323=CARTESIAN_POINT('Ctrl Pts',(-27.5198611034755,13.6901681944769,
129.881727019293)) ;
#132324=CARTESIAN_POINT('Ctrl Pts',(-27.4947206170695,13.9614083380647,
129.775024765156)) ;
#132325=CARTESIAN_POINT('Ctrl Pts',(-27.4477408524357,14.1924050674132,
129.604730002262)) ;
#132326=CARTESIAN_POINT('Ctrl Pts',(-27.3829916295066,14.3688010159201,
129.382496516221)) ;
#132327=CARTESIAN_POINT('Ctrl Pts',(-27.305567395489,14.4776662097744,129.123157647789)) ;
#132328=CARTESIAN_POINT('Ctrl Pts',(-27.2222300887403,14.5108828480259,
128.84666452346)) ;
#132329=CARTESIAN_POINT('Ctrl Pts',(-27.1390665957671,14.4662997711349,
128.570551673275)) ;
#132330=CARTESIAN_POINT('Ctrl Pts',(-27.063203525044,14.3468724358185,128.315811999268)) ;
#132331=CARTESIAN_POINT('Ctrl Pts',(-27.000726116674,14.161614932188,128.10021376119)) ;
#132332=CARTESIAN_POINT('Ctrl Pts',(-26.9566598775861,13.9230022753498,
127.938326275104)) ;
#132333=CARTESIAN_POINT('Ctrl Pts',(-26.9350826150652,13.6485314062169,
127.842142219284)) ;
#132334=CARTESIAN_POINT('Ctrl Pts',(-26.9382141999983,13.3583011743042,
127.818182839235)) ;
#132335=CARTESIAN_POINT('Ctrl Pts',(-26.9665177873497,13.072504270402,127.867737400507)) ;
#132336=CARTESIAN_POINT('Ctrl Pts',(-27.0188173523961,12.8117566735177,
127.987365016217)) ;
#132337=CARTESIAN_POINT('Ctrl Pts',(-27.0915996802834,12.5955171582893,
128.166977325295)) ;
#132338=CARTESIAN_POINT('Ctrl Pts',(-27.1817271815024,12.4369580568928,
128.396898077135)) ;
#132339=CARTESIAN_POINT('Ctrl Pts',(-27.2813708056134,12.3507869630092,
128.655042348106)) ;
#132340=CARTESIAN_POINT('Ctrl Pts',(-27.3857827418417,12.3404899643528,
128.926923079581)) ;
#132341=CARTESIAN_POINT('Ctrl Pts',(-27.4876541467364,12.4078494476239,
129.191403822402)) ;
#132342=CARTESIAN_POINT('Ctrl Pts',(-27.5807089481865,12.5483871977687,
129.430029656426)) ;
#132343=CARTESIAN_POINT('Ctrl Pts',(-27.6584612758746,12.7513533086917,
129.624045981255)) ;
#132344=CARTESIAN_POINT('Ctrl Pts',(-27.7163134902441,13.001941318222,129.759978308328)) ;
#132345=CARTESIAN_POINT('Ctrl Pts',(-27.7510006841768,13.2828868274063,
129.828206089058)) ;
#132346=CARTESIAN_POINT('Ctrl Pts',(-27.7607078220157,13.5743278631276,
129.823412590067)) ;
#132347=CARTESIAN_POINT('Ctrl Pts',(-27.7452570064132,13.8554587804339,
129.745052642731)) ;
#132348=CARTESIAN_POINT('Ctrl Pts',(-27.7068857846591,14.103739100914,129.599981463497)) ;
#132349=CARTESIAN_POINT('Ctrl Pts',(-27.6487231943859,14.3046990175591,
129.396931127844)) ;
#132350=CARTESIAN_POINT('Ctrl Pts',(-27.5755356695319,14.4424188711516,
129.149922663509)) ;
#132351=CARTESIAN_POINT('Ctrl Pts',(-27.4939933548379,14.5067209234145,
128.878704097542)) ;
#132352=CARTESIAN_POINT('Ctrl Pts',(-27.4097527588653,14.4936392684735,
128.599416389571)) ;
#132353=CARTESIAN_POINT('Ctrl Pts',(-27.3303082230943,14.404006740505,128.334269093954)) ;
#132354=CARTESIAN_POINT('Ctrl Pts',(-27.2614819305869,14.2433942656814,
128.099980444704)) ;
#132355=CARTESIAN_POINT('Ctrl Pts',(-27.2096136486434,14.0252993056693,
127.915456300396)) ;
#132356=CARTESIAN_POINT('Ctrl Pts',(-27.178469556164,13.7626963119846,127.791262873367)) ;
#132357=CARTESIAN_POINT('Ctrl Pts',(-27.1714738989522,13.4766513624265,
127.737736625053)) ;
#132358=CARTESIAN_POINT('Ctrl Pts',(-27.1895561727833,13.1866966293381,
127.757460183878)) ;
#132359=CARTESIAN_POINT('Ctrl Pts',(-27.2326135994264,12.9123106961637,
127.849963433579)) ;
#132360=CARTESIAN_POINT('Ctrl Pts',(-27.2974441217088,12.6769408805555,
128.006390666055)) ;
#132361=CARTESIAN_POINT('Ctrl Pts',(-27.3808130116155,12.4935889535621,
128.216818650803)) ;
#132362=CARTESIAN_POINT('Ctrl Pts',(-27.4776575476475,12.3766908568814,
128.466511171481)) ;
#132363=CARTESIAN_POINT('Ctrl Pts',(-27.5810443505466,12.3352383862452,
128.735442117728)) ;
#132364=CARTESIAN_POINT('Ctrl Pts',(-27.6845420847214,12.3713736006973,
129.004732437811)) ;
#132365=CARTESIAN_POINT('Ctrl Pts',(-27.7818596677854,12.4827590293817,
129.255891826048)) ;
#132366=CARTESIAN_POINT('Ctrl Pts',(-27.8667979944307,12.6627224306716,
129.47073002161)) ;
#132367=CARTESIAN_POINT('Ctrl Pts',(-27.9330076414952,12.8955397849013,
129.631137908056)) ;
#132368=CARTESIAN_POINT('Ctrl Pts',(-27.9774352268445,13.1663558963296,
129.72784335586)) ;
#132369=CARTESIAN_POINT('Ctrl Pts',(-27.9973849513202,13.4563321062043,
129.752958193208)) ;
#132370=CARTESIAN_POINT('Ctrl Pts',(-27.9920646322741,13.74354179735,129.704297361198)) ;
#132371=CARTESIAN_POINT('Ctrl Pts',(-27.9626165416411,14.007863745204,129.585142101985)) ;
#132372=CARTESIAN_POINT('Ctrl Pts',(-27.9119828992553,14.2299792391956,
129.404152786278)) ;
#132373=CARTESIAN_POINT('Ctrl Pts',(-27.844287943155,14.3948659481182,129.173238937185)) ;
#132374=CARTESIAN_POINT('Ctrl Pts',(-27.7651604606475,14.4898740802148,
128.908913740689)) ;
#132375=CARTESIAN_POINT('Ctrl Pts',(-27.681397890891,14.5084149248409,128.631178035807)) ;
#132376=CARTESIAN_POINT('Ctrl Pts',(-27.5990872491488,14.4492459338564,
128.357554758999)) ;
#132377=CARTESIAN_POINT('Ctrl Pts',(-27.5253256223266,14.316609488643,128.108970615685)) ;
#132378=CARTESIAN_POINT('Ctrl Pts',(-27.4659033295799,14.1198900556279,
127.9022461303)) ;
#132379=CARTESIAN_POINT('Ctrl Pts',(-27.42591393932,13.8734079349303,127.752317228327)) ;
#132380=CARTESIAN_POINT('Ctrl Pts',(-27.408865491139,13.5947694158123,127.669409669264)) ;
#132381=CARTESIAN_POINT('Ctrl Pts',(-27.4167455300075,13.3033325180628,
127.659268253717)) ;
#132382=CARTESIAN_POINT('Ctrl Pts',(-27.4497732461264,13.0207084742087,
127.722612022269)) ;
#132383=CARTESIAN_POINT('Ctrl Pts',(-27.5060414733426,12.767628690545,127.853947272495)) ;
#132384=CARTESIAN_POINT('Ctrl Pts',(-27.5826500146593,12.5604751539345,
128.044576460787)) ;
#132385=CARTESIAN_POINT('Ctrl Pts',(-27.6748867687302,12.4152916729436,
128.280805111389)) ;
#132386=CARTESIAN_POINT('Ctrl Pts',(-27.7760048062591,12.3428120631862,
128.543188432493)) ;
#132387=CARTESIAN_POINT('Ctrl Pts',(-27.880802690774,12.3473797413046,128.816094258677)) ;
#132388=CARTESIAN_POINT('Ctrl Pts',(-27.9814814316689,12.4294695368143,
129.077065134186)) ;
#132389=CARTESIAN_POINT('Ctrl Pts',(-28.0714598999934,12.5816148375682,
129.306949475753)) ;
#132390=CARTESIAN_POINT('Ctrl Pts',(-28.1460628162166,12.7949907280796,
129.491697351825)) ;
#132391=CARTESIAN_POINT('Ctrl Pts',(-28.1999915303535,13.054101177031,129.616001192498)) ;
#132392=CARTESIAN_POINT('Ctrl Pts',(-28.2299138854955,13.3386274126212,
129.670307692816)) ;
#132393=CARTESIAN_POINT('Ctrl Pts',(-28.2347775216737,13.6281884734652,
129.651524250556)) ;
#132394=CARTESIAN_POINT('Ctrl Pts',(-28.2149512862949,13.9042249218154,
129.560485972219)) ;
#132395=CARTESIAN_POINT('Ctrl Pts',(-28.1723564864184,14.1463903457502,
129.402858889307)) ;
#132396=CARTESIAN_POINT('Ctrl Pts',(-28.1106708276455,14.3364819716926,
129.189416939951)) ;
#132397=CARTESIAN_POINT('Ctrl Pts',(-28.0360880693673,14.4598817702337,
128.938660433378)) ;
#132398=CARTESIAN_POINT('Ctrl Pts',(-27.953057765994,14.5104486170863,128.662863635966)) ;
#132399=CARTESIAN_POINT('Ctrl Pts',(-27.8692045369708,14.4822486369166,
128.384729130641)) ;
#132400=CARTESIAN_POINT('Ctrl Pts',(-27.791608538637,14.3791733041028,128.125092916574)) ;
#132401=CARTESIAN_POINT('Ctrl Pts',(-27.7253583208721,14.2063740303146,
127.898282623416)) ;
#132402=CARTESIAN_POINT('Ctrl Pts',(-27.6770395587882,13.9777765864427,
127.723995413382)) ;
#132403=CARTESIAN_POINT('Ctrl Pts',(-27.6504229397667,13.7109259499415,
127.613260324166)) ;
#132404=CARTESIAN_POINT('Ctrl Pts',(-27.6480583043497,13.4211174151953,
127.573090826099)) ;
#132405=CARTESIAN_POINT('Ctrl Pts',(-27.6709154004622,13.1336909339448,
127.606862509643)) ;
#132406=CARTESIAN_POINT('Ctrl Pts',(-27.7180057890291,12.8658812639418,
127.711313356748)) ;
#132407=CARTESIAN_POINT('Ctrl Pts',(-27.7873482366324,12.6367690190525,
127.880557040248)) ;
#132408=CARTESIAN_POINT('Ctrl Pts',(-27.8736342999947,12.4658337897599,
128.099554794345)) ;
#132409=CARTESIAN_POINT('Ctrl Pts',(-27.9718311891268,12.3631245211514,
128.353345809671)) ;
#132410=CARTESIAN_POINT('Ctrl Pts',(-28.0756846325717,12.3360466241608,
128.623667434511)) ;
#132411=CARTESIAN_POINT('Ctrl Pts',(-28.1788526517052,12.3868688002356,
128.891874367728)) ;
#132412=CARTESIAN_POINT('Ctrl Pts',(-28.2741388501772,12.5119418325269,
129.137115030646)) ;
#132413=CARTESIAN_POINT('Ctrl Pts',(-28.3556708751438,12.7021783709845,
129.342171425122)) ;
#132414=CARTESIAN_POINT('Ctrl Pts',(-28.4184699311589,12.9449353770794,
129.492398354652)) ;
#132415=CARTESIAN_POINT('Ctrl Pts',(-28.4583084084869,13.2214383784226,
129.575638041553)) ;
#132416=CARTESIAN_POINT('Ctrl Pts',(-28.4734122859081,13.5108147708277,
129.586797648768)) ;
#132417=CARTESIAN_POINT('Ctrl Pts',(-28.4633457731125,13.7968084175674,
129.524085701258)) ;
#132418=CARTESIAN_POINT('Ctrl Pts',(-28.4296187997626,14.0536576083437,
129.392533959943)) ;
#132419=CARTESIAN_POINT('Ctrl Pts',(-28.3754911658076,14.2659120564335,
129.201360310375)) ;
#132420=CARTESIAN_POINT('Ctrl Pts',(-28.3050821824441,14.4185012516542,
128.962475031458)) ;
#132421=CARTESIAN_POINT('Ctrl Pts',(-28.2247264730961,14.4992712221482,
128.694649965742)) ;
#132422=CARTESIAN_POINT('Ctrl Pts',(-28.1405276912772,14.5031360116066,
128.415538484686)) ;
#132423=CARTESIAN_POINT('Ctrl Pts',(-28.059513753469,14.4296202074177,128.145783486771)) ;
#132424=CARTESIAN_POINT('Ctrl Pts',(-27.9880766403289,14.2844131247839,
127.904026806799)) ;
#132425=CARTESIAN_POINT('Ctrl Pts',(-27.9318057397691,14.0764755685082,
127.706412345186)) ;
#132426=CARTESIAN_POINT('Ctrl Pts',(-27.8959845576815,13.8227947339683,
127.568706785711)) ;
#132427=CARTESIAN_POINT('Ctrl Pts',(-27.8835201350609,13.5398702989391,
127.499142873583)) ;
#132428=CARTESIAN_POINT('Ctrl Pts',(-27.8962033555758,13.2487717783427,
127.50306914783)) ;
#132429=CARTESIAN_POINT('Ctrl Pts',(-27.9337544855272,12.9703362151756,
127.579661290793)) ;
#132430=CARTESIAN_POINT('Ctrl Pts',(-27.9942820451289,12.7241092781338,
127.723348072863)) ;
#132431=CARTESIAN_POINT('Ctrl Pts',(-28.0741961867263,12.5279171433205,
127.923656462501)) ;
#132432=CARTESIAN_POINT('Ctrl Pts',(-28.1684346295129,12.3959938665945,
128.165822555878)) ;
#132433=CARTESIAN_POINT('Ctrl Pts',(-28.2708930006534,12.3376260980812,
128.432033363079)) ;
#132434=CARTESIAN_POINT('Ctrl Pts',(-28.3752372703154,12.3570497794023,
128.703694565037)) ;
#132435=CARTESIAN_POINT('Ctrl Pts',(-28.474218780803,12.4525559733436,128.959799081295)) ;
#132436=CARTESIAN_POINT('Ctrl Pts',(-28.5620645646479,12.6176036105847,
129.183295489253)) ;
#132437=CARTESIAN_POINT('Ctrl Pts',(-28.6330705369593,12.8410947019102,
129.357514549927)) ;
#132438=CARTESIAN_POINT('Ctrl Pts',(-28.6825047729054,13.1055203518464,
129.468831178845)) ;
#132439=CARTESIAN_POINT('Ctrl Pts',(-28.7078791143123,13.3928980327512,
129.509831198009)) ;
#132440=CARTESIAN_POINT('Ctrl Pts',(-28.7080000857972,13.6824543649216,
129.477058491295)) ;
#132441=CARTESIAN_POINT('Ctrl Pts',(-28.6836462060832,13.9532692757644,
129.372812982897)) ;
#132442=CARTESIAN_POINT('Ctrl Pts',(-28.637210824604,14.1862511235797,129.204032177995)) ;
#132443=CARTESIAN_POINT('Ctrl Pts',(-28.5729983268859,14.3643962082537,
128.983404490918)) ;
#132444=CARTESIAN_POINT('Ctrl Pts',(-28.4953888433576,14.4759024807437,
128.723329064892)) ;
#132445=CARTESIAN_POINT('Ctrl Pts',(-28.4124155755593,14.5109062464403,
128.448017144722)) ;
#132446=CARTESIAN_POINT('Ctrl Pts',(-28.3292183756258,14.4687351628052,
128.171836440681)) ;
#132447=CARTESIAN_POINT('Ctrl Pts',(-28.2530232843449,14.351243796897,127.916105712843)) ;
#132448=CARTESIAN_POINT('Ctrl Pts',(-28.19012029587,14.1681343550178,127.699312985571)) ;
#132449=CARTESIAN_POINT('Ctrl Pts',(-28.1452447510838,13.9291093552066,
127.534840373785)) ;
#132450=CARTESIAN_POINT('Ctrl Pts',(-28.123183101824,13.6572015399983,127.437471920795)) ;
#132451=CARTESIAN_POINT('Ctrl Pts',(-28.1255814706017,13.3659146668707,
127.411223933066)) ;
#132452=CARTESIAN_POINT('Ctrl Pts',(-28.1531210645832,13.0809591455927,
127.458689441797)) ;
#132453=CARTESIAN_POINT('Ctrl Pts',(-28.2046620168687,12.8188859308948,
127.576087509683)) ;
#132454=CARTESIAN_POINT('Ctrl Pts',(-28.277541817743,12.5999510440463,127.755745614815)) ;
#132455=CARTESIAN_POINT('Ctrl Pts',(-28.3661476402695,12.4414984825018,
127.981641389139)) ;
#132456=CARTESIAN_POINT('Ctrl Pts',(-28.4661327647063,12.3520343108791,
128.240572616874)) ;
#132457=CARTESIAN_POINT('Ctrl Pts',(-28.5708059444941,12.3398054622105,
128.513131254719)) ;
#132458=CARTESIAN_POINT('Ctrl Pts',(-28.6724777538977,12.4047865271677,
128.777144444355)) ;
#132459=CARTESIAN_POINT('Ctrl Pts',(-28.7659001413954,12.5431933869583,
129.016844456436)) ;
#132460=CARTESIAN_POINT('Ctrl Pts',(-28.8442058560459,12.7444965603529,
129.212472342267)) ;
#132461=CARTESIAN_POINT('Ctrl Pts',(-28.9027924661007,12.9945025224571,
129.350476244749)) ;
#132462=CARTESIAN_POINT('Ctrl Pts',(-28.9381575691283,13.2745329094811,
129.420727068277)) ;
#132463=CARTESIAN_POINT('Ctrl Pts',(-28.9485234575593,13.5670626370277,
129.417726861736)) ;
#132464=CARTESIAN_POINT('Ctrl Pts',(-28.933960447473,13.8462370772247,129.342272430857)) ;
#132465=CARTESIAN_POINT('Ctrl Pts',(-28.8959789907869,14.0979241250953,
129.198057982517)) ;
#132466=CARTESIAN_POINT('Ctrl Pts',(-28.838332105253,14.2997383418867,128.996585250886)) ;
#132467=CARTESIAN_POINT('Ctrl Pts',(-28.7657725957652,14.4393312193764,
128.7515156292)) ;
#132468=CARTESIAN_POINT('Ctrl Pts',(-28.6837573347161,14.5060643569228,
128.478659684657)) ;
#132469=CARTESIAN_POINT('Ctrl Pts',(-28.6001080114847,14.4951758782706,
128.201352828122)) ;
#132470=CARTESIAN_POINT('Ctrl Pts',(-28.5200653111137,14.4072623281432,
127.934287968157)) ;
#132471=CARTESIAN_POINT('Ctrl Pts',(-28.4511978062007,14.2495039694875,
127.70007480226)) ;
#132472=CARTESIAN_POINT('Ctrl Pts',(-28.3983753819167,14.0308221258824,
127.512458103752)) ;
#132473=CARTESIAN_POINT('Ctrl Pts',(-28.3669487720982,13.7719100664948,
127.38779922883)) ;
#132474=CARTESIAN_POINT('Ctrl Pts',(-28.3590881011533,13.4847456450531,
127.331550611793)) ;
#132475=CARTESIAN_POINT('Ctrl Pts',(-28.3764285791946,13.1955425031336,
127.349219523261)) ;
#132476=CARTESIAN_POINT('Ctrl Pts',(-28.4187558984065,12.9200552968874,
127.439556443674)) ;
#132477=CARTESIAN_POINT('Ctrl Pts',(-28.4830536897966,12.6831184385928,
127.594396583248)) ;
#132478=CARTESIAN_POINT('Ctrl Pts',(-28.5659931747335,12.4980281206389,
127.803559634745)) ;
#132479=CARTESIAN_POINT('Ctrl Pts',(-28.6623364928729,12.3791543430107,
128.051854714151)) ;
#132480=CARTESIAN_POINT('Ctrl Pts',(-28.7659162180442,12.3353503717386,
128.321248640665)) ;
#132481=CARTESIAN_POINT('Ctrl Pts',(-28.869394759317,12.3691099621928,128.590526992868)) ;
#132482=CARTESIAN_POINT('Ctrl Pts',(-28.9675502196224,12.4795856785055,
128.843913403417)) ;
#132483=CARTESIAN_POINT('Ctrl Pts',(-29.0518027446978,12.6553361009926,
129.057199931773)) ;
#132484=CARTESIAN_POINT('Ctrl Pts',(-29.1192464163454,12.8882259217544,
129.220954123798)) ;
#132485=CARTESIAN_POINT('Ctrl Pts',(-29.1642643498932,13.1581921393272,
129.319406321897)) ;
#132486=CARTESIAN_POINT('Ctrl Pts',(-29.1849604313943,13.4482190387101,
129.34666282445)) ;
#132487=CARTESIAN_POINT('Ctrl Pts',(-29.1803518618151,13.7352663202425,
129.300143313471)) ;
#132488=CARTESIAN_POINT('Ctrl Pts',(-29.1516048942262,14.0004787425337,
129.183043232165)) ;
#132489=CARTESIAN_POINT('Ctrl Pts',(-29.1015568370635,14.2242401467777,
129.003757674716)) ;
#132490=CARTESIAN_POINT('Ctrl Pts',(-29.0339430184054,14.391486003047,128.772934980117)) ;
#132491=CARTESIAN_POINT('Ctrl Pts',(-28.955492652777,14.4880341837757,128.510778479589)) ;
#132492=CARTESIAN_POINT('Ctrl Pts',(-28.8714600975796,14.5089767222778,
128.232121389573)) ;
#132493=CARTESIAN_POINT('Ctrl Pts',(-28.7892529362311,14.4520807364783,
127.958902917957)) ;
#132494=CARTESIAN_POINT('Ctrl Pts',(-28.7150523793816,14.3213934969356,
127.708991446956)) ;
#132495=CARTESIAN_POINT('Ctrl Pts',(-28.6551735760367,14.126427628205,127.500952233118)) ;
#132496=CARTESIAN_POINT('Ctrl Pts',(-28.6144873955634,13.8807880817665,
127.348935930026)) ;
#132497=CARTESIAN_POINT('Ctrl Pts',(-28.5968038371001,13.6022566506269,
127.264117077343)) ;
#132498=CARTESIAN_POINT('Ctrl Pts',(-28.6039330637587,13.3123739575692,
127.251951536785)) ;
#132499=CARTESIAN_POINT('Ctrl Pts',(-28.6361660227389,13.0290004002489,
127.312956120869)) ;
#132500=CARTESIAN_POINT('Ctrl Pts',(-28.6919510174919,12.7741270713226,
127.442792020744)) ;
#132501=CARTESIAN_POINT('Ctrl Pts',(-28.7679989254335,12.5657352250487,
127.631815876347)) ;
#132502=CARTESIAN_POINT('Ctrl Pts',(-28.8594997341221,12.4188762117679,
127.866013266875)) ;
#132503=CARTESIAN_POINT('Ctrl Pts',(-28.9608147014607,12.3438128452305,
128.128841957193)) ;
#132504=CARTESIAN_POINT('Ctrl Pts',(-29.0652267516056,12.3461025205116,
128.400746493264)) ;
#132505=CARTESIAN_POINT('Ctrl Pts',(-29.1661640470906,12.4255735874937,
128.662467769584)) ;
#132506=CARTESIAN_POINT('Ctrl Pts',(-29.2569746802431,12.5765456735502,
128.894620530997)) ;
#132507=CARTESIAN_POINT('Ctrl Pts',(-29.3318567873601,12.7879286592572,
129.080274286269)) ;
#132508=CARTESIAN_POINT('Ctrl Pts',(-29.3863322538626,13.0448054046113,
129.206302436344)) ;
#132509=CARTESIAN_POINT('Ctrl Pts',(-29.4171885363179,13.329756321322,129.26322288733)) ;
#132510=CARTESIAN_POINT('Ctrl Pts',(-29.4227776954555,13.6201107178654,
129.246484513251)) ;
#132511=CARTESIAN_POINT('Ctrl Pts',(-29.4036112081965,13.8967554382586,
129.157379684264)) ;
#132512=CARTESIAN_POINT('Ctrl Pts',(-29.3617661068054,14.1394983367384,
129.002038511481)) ;
#132513=CARTESIAN_POINT('Ctrl Pts',(-29.3006432267773,14.3315001569242,
128.790247960104)) ;
#132514=CARTESIAN_POINT('Ctrl Pts',(-29.2260808954585,14.4575222943013,
128.539420298087)) ;
#132515=CARTESIAN_POINT('Ctrl Pts',(-29.1430912249785,14.5099977938908,
128.263711456409)) ;
#132516=CARTESIAN_POINT('Ctrl Pts',(-29.0596283023754,14.4843800867397,
127.986903750172)) ;
#132517=CARTESIAN_POINT('Ctrl Pts',(-28.9813399566608,14.3828781461486,
127.725057189875)) ;
#132518=CARTESIAN_POINT('Ctrl Pts',(-28.9150542416882,14.212816168216,127.498335145429)) ;
#132519=CARTESIAN_POINT('Ctrl Pts',(-28.8659433323491,13.9854781681749,
127.321666885816)) ;
#132520=CARTESIAN_POINT('Ctrl Pts',(-28.8385949971052,13.7179644909653,
127.2086184725)) ;
#132521=CARTESIAN_POINT('Ctrl Pts',(-28.835583635112,13.4301920376034,127.166758116441)) ;
#132522=CARTESIAN_POINT('Ctrl Pts',(-28.8575789748189,13.1421055633853,
127.197981715462)) ;
#132523=CARTESIAN_POINT('Ctrl Pts',(-28.9045188244626,12.87150128464,127.301728733917)) ;
#132524=CARTESIAN_POINT('Ctrl Pts',(-28.9725684665303,12.6436097991943,
127.46756519262)) ;
#132525=CARTESIAN_POINT('Ctrl Pts',(-29.0586604842472,12.4698498437503,
127.68586545448)) ;
#132526=CARTESIAN_POINT('Ctrl Pts',(-29.1565931939368,12.3651221856613,
127.938894371706)) ;
#132527=CARTESIAN_POINT('Ctrl Pts',(-29.2604850351592,12.335692224637,128.209290972507)) ;
#132528=CARTESIAN_POINT('Ctrl Pts',(-29.3638355952977,12.3844432071478,
128.478011145159)) ;
#132529=CARTESIAN_POINT('Ctrl Pts',(-29.4592358664342,12.5072147901112,
128.723652752499)) ;
#132530=CARTESIAN_POINT('Ctrl Pts',(-29.5413221888135,12.6957550150873,
128.930308953615)) ;
#132531=CARTESIAN_POINT('Ctrl Pts',(-29.6047036187767,12.9372999479051,
129.082233550744)) ;
#132532=CARTESIAN_POINT('Ctrl Pts',(-29.6452182047899,13.2121499543988,
129.167553115)) ;
#132533=CARTESIAN_POINT('Ctrl Pts',(-29.6611042764023,13.5032465104466,
129.180780924663)) ;
#132534=CARTESIAN_POINT('Ctrl Pts',(-29.6518819161121,13.7871080328991,
129.120848156331)) ;
#132535=CARTESIAN_POINT('Ctrl Pts',(-29.6187108954398,14.0469104745439,
128.990694231868)) ;
#132536=CARTESIAN_POINT('Ctrl Pts',(-29.5650955851099,14.2605649124229,
128.801033137001)) ;
#132537=CARTESIAN_POINT('Ctrl Pts',(-29.494870755953,14.4153649488043,128.562594916595)) ;
#132538=CARTESIAN_POINT('Ctrl Pts',(-29.4150387131859,14.4978582783663,
128.296438099207)) ;
#132539=CARTESIAN_POINT('Ctrl Pts',(-29.3308499416307,14.5041773990225,
128.017349602118)) ;
#132540=CARTESIAN_POINT('Ctrl Pts',(-29.2496148451093,14.4329779197685,
127.746941843894)) ;
#132541=CARTESIAN_POINT('Ctrl Pts',(-29.1775262666222,14.2890422314917,
127.503142142852)) ;
#132542=CARTESIAN_POINT('Ctrl Pts',(-29.1208969337368,14.082779433517,127.304531079944)) ;
#132543=CARTESIAN_POINT('Ctrl Pts',(-29.0845225826136,13.8309337098099,
127.165299579887)) ;
#132544=CARTESIAN_POINT('Ctrl Pts',(-29.0713186329842,13.5483120187831,
127.093542785031)) ;
#132545=CARTESIAN_POINT('Ctrl Pts',(-29.083229857648,13.2574777531019,127.095253063998)) ;
#132546=CARTESIAN_POINT('Ctrl Pts',(-29.1201441678816,12.9779697529959,
127.169929814834)) ;
#132547=CARTESIAN_POINT('Ctrl Pts',(-29.1798340071233,12.7311580251373,
127.311268080156)) ;
#132548=CARTESIAN_POINT('Ctrl Pts',(-29.259615046753,12.5323980592304,127.511032300878)) ;
#132549=CARTESIAN_POINT('Ctrl Pts',(-29.3531954363121,12.3989897288854,
127.751398360947)) ;
#132550=CARTESIAN_POINT('Ctrl Pts',(-29.4557047728638,12.3382487603058,
128.017686516644)) ;
#132551=CARTESIAN_POINT('Ctrl Pts',(-29.5597398015999,12.3552058083452,
128.288561847953)) ;
#132552=CARTESIAN_POINT('Ctrl Pts',(-29.6596151268484,12.4490680703867,
128.547063275398)) ;
#132553=CARTESIAN_POINT('Ctrl Pts',(-29.747823539621,12.612854304799,128.771597225379)) ;
#132554=CARTESIAN_POINT('Ctrl Pts',(-29.8189230473542,12.8333918295054,
128.946308444558)) ;
#132555=CARTESIAN_POINT('Ctrl Pts',(-29.8692193933531,13.0975419155814,
129.060046052025)) ;
#132556=CARTESIAN_POINT('Ctrl Pts',(-29.8952825556904,13.3843701567211,
129.103082744144)) ;
#132557=CARTESIAN_POINT('Ctrl Pts',(-29.8961296754756,13.6749248626015,
129.072344167559)) ;
#132558=CARTESIAN_POINT('Ctrl Pts',(-29.872352875635,13.9463602578246,128.969789222471)) ;
#132559=CARTESIAN_POINT('Ctrl Pts',(-29.8267467901644,14.1798324379302,
128.803574285622)) ;
#132560=CARTESIAN_POINT('Ctrl Pts',(-29.762567848699,14.3606302769089,128.582842462436)) ;
#132561=CARTESIAN_POINT('Ctrl Pts',(-29.6859295100925,14.4733618864566,
128.325903972762)) ;
#132562=CARTESIAN_POINT('Ctrl Pts',(-29.6022723165312,14.5110756600993,
128.048275924638)) ;
#132563=CARTESIAN_POINT('Ctrl Pts',(-29.5194444158079,14.4709889009811,
127.773361424165)) ;
#132564=CARTESIAN_POINT('Ctrl Pts',(-29.4427850873383,14.3556941984043,
127.516218240476)) ;
#132565=CARTESIAN_POINT('Ctrl Pts',(-29.379260435332,14.1731666486328,127.297467610204)) ;
#132566=CARTESIAN_POINT('Ctrl Pts',(-29.3342254132114,13.9378584167298,
127.132862710005)) ;
#132567=CARTESIAN_POINT('Ctrl Pts',(-29.3112446912435,13.6656355311939,
127.03265253494)) ;
#132568=CARTESIAN_POINT('Ctrl Pts',(-29.3129312287784,13.3744563081115,
127.004322113587)) ;
#132569=CARTESIAN_POINT('Ctrl Pts',(-29.3398177129572,13.0885611803192,
127.049815834232)) ;
#132570=CARTESIAN_POINT('Ctrl Pts',(-29.3906009924672,12.8263306498725,
127.165093753781)) ;
#132571=CARTESIAN_POINT('Ctrl Pts',(-29.4625594349018,12.6063807769631,
127.342179164998)) ;
#132572=CARTESIAN_POINT('Ctrl Pts',(-29.5513814104012,12.4447492933123,
127.568465791526)) ;
#132573=CARTESIAN_POINT('Ctrl Pts',(-29.6511504516607,12.3535025882306,
127.826777567947)) ;
#132574=CARTESIAN_POINT('Ctrl Pts',(-29.7556083087904,12.3391045054194,
128.098761532225)) ;
#132575=CARTESIAN_POINT('Ctrl Pts',(-29.8574615889439,12.4018104241151,
128.363303066571)) ;
#132576=CARTESIAN_POINT('Ctrl Pts',(-29.9515240336887,12.5389586489687,
128.604752086664)) ;
#132577=CARTESIAN_POINT('Ctrl Pts',(-30.0298895040687,12.7377764458565,
128.800721216607)) ;
#132578=CARTESIAN_POINT('Ctrl Pts',(-30.0891318078393,12.9863019722805,
128.940662639121)) ;
#132579=CARTESIAN_POINT('Ctrl Pts',(-30.1252471064463,13.2660338630659,
129.013066477495)) ;
#132580=CARTESIAN_POINT('Ctrl Pts',(-30.1363860269831,13.5582232268191,
129.012365283493)) ;
#132581=CARTESIAN_POINT('Ctrl Pts',(-30.1224573425596,13.8387404070693,
128.9386660175)) ;
#132582=CARTESIAN_POINT('Ctrl Pts',(-30.0853429984546,14.0904925183414,
128.797147021732)) ;
#132583=CARTESIAN_POINT('Ctrl Pts',(-30.0277590711992,14.2955136011611,
128.595595560232)) ;
#132584=CARTESIAN_POINT('Ctrl Pts',(-29.9558778598522,14.4360006812449,
128.352686763533)) ;
#132585=CARTESIAN_POINT('Ctrl Pts',(-29.8742567679805,14.5051702931602,
128.081056456965)) ;
#132586=CARTESIAN_POINT('Ctrl Pts',(-29.7902969630137,14.4966323764384,
127.802731519334)) ;
#132587=CARTESIAN_POINT('Ctrl Pts',(-29.7100123387406,14.4108291399258,
127.534953213959)) ;
#132588=CARTESIAN_POINT('Ctrl Pts',(-29.6407380446541,14.2547209501546,
127.299525468516)) ;
#132589=CARTESIAN_POINT('Ctrl Pts',(-29.5875888674703,14.0388606089928,
127.111132269111)) ;
#132590=CARTESIAN_POINT('Ctrl Pts',(-29.5552494813085,13.779405578044,126.983595808789)) ;
#132591=CARTESIAN_POINT('Ctrl Pts',(-29.5467692399988,13.4926641580088,
126.925547219345)) ;
#132592=CARTESIAN_POINT('Ctrl Pts',(-29.5633816541989,13.2038302112353,
126.941144586643)) ;
#132593=CARTESIAN_POINT('Ctrl Pts',(-29.6048714410533,12.9280759931688,
127.02910382322)) ;
#132594=CARTESIAN_POINT('Ctrl Pts',(-29.6688506403303,12.6887447492448,
127.182864366148)) ;
#132595=CARTESIAN_POINT('Ctrl Pts',(-29.7513587249347,12.5022966343227,
127.39078364992)) ;
#132596=CARTESIAN_POINT('Ctrl Pts',(-29.8469802454942,12.381763978882,127.637108683278)) ;
#132597=CARTESIAN_POINT('Ctrl Pts',(-29.9508020024135,12.3354318114705,
127.907094928409)) ;
#132598=CARTESIAN_POINT('Ctrl Pts',(-30.0541803012317,12.3672035513488,
128.176131637916)) ;
#132599=CARTESIAN_POINT('Ctrl Pts',(-30.1521106585629,12.474426481286,128.429055203006)) ;
#132600=CARTESIAN_POINT('Ctrl Pts',(-30.2377865470727,12.6503068829769,
128.646124078682)) ;
#132601=CARTESIAN_POINT('Ctrl Pts',(-30.3053907898611,12.8812481424524,
128.810483543534)) ;
#132602=CARTESIAN_POINT('Ctrl Pts',(-30.3510328505262,13.1494231082653,
128.910858646302)) ;
#132603=CARTESIAN_POINT('Ctrl Pts',(-30.3725424728725,13.4405328283774,
128.94033906329)) ;
#132604=CARTESIAN_POINT('Ctrl Pts',(-30.3685945252647,13.7272524095848,
128.895825068985)) ;
#132605=CARTESIAN_POINT('Ctrl Pts',(-30.3405359677795,13.9933197786215,
128.780743464257)) ;
#132606=CARTESIAN_POINT('Ctrl Pts',(-30.2910888155488,14.2183989061991,
128.603235194175)) ;
#132607=CARTESIAN_POINT('Ctrl Pts',(-30.2238484293931,14.3876287517767,
128.373477627282)) ;
#132608=CARTESIAN_POINT('Ctrl Pts',(-30.1457515284424,14.4861870970875,
128.112398717919)) ;
#132609=CARTESIAN_POINT('Ctrl Pts',(-30.0617136501863,14.5095212297327,
127.833700802789)) ;
#132610=CARTESIAN_POINT('Ctrl Pts',(-29.9792786676799,14.4547287275128,
127.559780909732)) ;
#132611=CARTESIAN_POINT('Ctrl Pts',(-29.9048009680584,14.3261105544631,
127.309079981945)) ;
#132612=CARTESIAN_POINT('Ctrl Pts',(-29.844419395189,14.1327425032557,127.099559452458)) ;
#132613=CARTESIAN_POINT('Ctrl Pts',(-29.803152525388,13.8885306001009,126.945876263857)) ;
#132614=CARTESIAN_POINT('Ctrl Pts',(-29.7847767393562,13.6107524410049,
126.859040355574)) ;
#132615=CARTESIAN_POINT('Ctrl Pts',(-29.7910854802672,13.3210542583331,
126.844495484992)) ;
#132616=CARTESIAN_POINT('Ctrl Pts',(-29.8229753868191,13.0351251235983,
126.904244014759)) ;
#132617=CARTESIAN_POINT('Ctrl Pts',(-29.8776744286432,12.7816150209491,
127.031216029816)) ;
#132618=CARTESIAN_POINT('Ctrl Pts',(-29.9534311716552,12.5706518061014,
127.219253692065)) ;
#132619=CARTESIAN_POINT('Ctrl Pts',(-30.0445412838822,12.422091900903,127.452333377032)) ;
#132620=CARTESIAN_POINT('Ctrl Pts',(-30.1457887502779,12.3448083833829,
127.714923612566)) ;
#132621=CARTESIAN_POINT('Ctrl Pts',(-30.250148655895,12.3450375607664,127.986693881587)) ;
#132622=CARTESIAN_POINT('Ctrl Pts',(-30.3511170822601,12.4222140372622,
128.248559607977)) ;
#132623=CARTESIAN_POINT('Ctrl Pts',(-30.4423550067095,12.5713072693593,
128.481942746401)) ;
#132624=CARTESIAN_POINT('Ctrl Pts',(-30.5177968325665,12.7812068465324,
128.669220610782)) ;
#132625=CARTESIAN_POINT('Ctrl Pts',(-30.5730322088188,13.0378486801572,
128.797371634622)) ;
#132626=CARTESIAN_POINT('Ctrl Pts',(-30.6044543099339,13.3220972424203,
128.855977004469)) ;
#132627=CARTESIAN_POINT('Ctrl Pts',(-30.6107589621473,13.6116477161832,
128.841431739069)) ;
#132628=CARTESIAN_POINT('Ctrl Pts',(-30.5922328646922,13.8896343949454,
128.754117840507)) ;
#132629=CARTESIAN_POINT('Ctrl Pts',(-30.5510661396947,14.1329048293709,
128.60084368254)) ;
#132630=CARTESIAN_POINT('Ctrl Pts',(-30.4905361238725,14.3266157424045,
128.390815616408)) ;
#132631=CARTESIAN_POINT('Ctrl Pts',(-30.4160368539188,14.4550271923226,
128.140061981301)) ;
#132632=CARTESIAN_POINT('Ctrl Pts',(-30.333450058965,14.5094869156272,127.865640071397)) ;
#132633=CARTESIAN_POINT('Ctrl Pts',(-30.2498814405861,14.4863255111229,
127.588507289986)) ;
#132634=CARTESIAN_POINT('Ctrl Pts',(-30.1712461824057,14.3868080890416,
127.325605825376)) ;
#132635=CARTESIAN_POINT('Ctrl Pts',(-30.1044933380963,14.2186053771164,
127.097513189475)) ;
#132636=CARTESIAN_POINT('Ctrl Pts',(-30.0547280039428,13.9916146831158,
126.918804037804)) ;
#132637=CARTESIAN_POINT('Ctrl Pts',(-30.0268955041398,13.727139474133,126.804607454992)) ;
#132638=CARTESIAN_POINT('Ctrl Pts',(-30.0231159202939,13.437362164295,126.760227532608)) ;
#132639=CARTESIAN_POINT('Ctrl Pts',(-30.0443922432487,13.1504054531947,
126.789513820971)) ;
#132640=CARTESIAN_POINT('Ctrl Pts',(-30.0906616171445,12.8786465021209,
126.89126693415)) ;
#132641=CARTESIAN_POINT('Ctrl Pts',(-30.157970236125,12.6500332814425,127.055027994723)) ;
#132642=CARTESIAN_POINT('Ctrl Pts',(-30.2434337782595,12.4743183897028,
127.271533917434)) ;
#132643=CARTESIAN_POINT('Ctrl Pts',(-30.3417585829433,12.3668547922141,
127.525488336301)) ;
#132644=CARTESIAN_POINT('Ctrl Pts',(-30.4450821005495,12.335562941567,127.79438563983)) ;
#132645=CARTESIAN_POINT('Ctrl Pts',(-30.5484944936694,12.3817108072099,
128.063306891139)) ;
#132646=CARTESIAN_POINT('Ctrl Pts',(-30.6445980415539,12.502839824897,128.310875860644)) ;
#132647=CARTESIAN_POINT('Ctrl Pts',(-30.7271978616452,12.690351441453,128.518969835721)) ;
#132648=CARTESIAN_POINT('Ctrl Pts',(-30.7907079505213,12.9285059391321,
128.671549365572)) ;
#132649=CARTESIAN_POINT('Ctrl Pts',(-30.832295267727,13.2046731907038,128.75974213921)) ;
#132650=CARTESIAN_POINT('Ctrl Pts',(-30.8487758407748,13.4951333113011,
128.774772845728)) ;
#132651=CARTESIAN_POINT('Ctrl Pts',(-30.8402346447153,13.779501210584,128.716814376005)) ;
#132652=CARTESIAN_POINT('Ctrl Pts',(-30.8078637040687,14.0394108332529,
128.589125311067)) ;
#132653=CARTESIAN_POINT('Ctrl Pts',(-30.7546552751125,14.2552141196343,
128.400557285253)) ;
#132654=CARTESIAN_POINT('Ctrl Pts',(-30.6851696086428,14.4112842226695,
128.164437543065)) ;
#132655=CARTESIAN_POINT('Ctrl Pts',(-30.6053419982904,14.49663037618,127.89819080895)) ;
#132656=CARTESIAN_POINT('Ctrl Pts',(-30.520751800545,14.5049768783044,127.617767628039)) ;
#132657=CARTESIAN_POINT('Ctrl Pts',(-30.4397470692586,14.4360835729073,
127.348190225217)) ;
#132658=CARTESIAN_POINT('Ctrl Pts',(-30.3673932451776,14.2946513922982,
127.103676961857)) ;
#132659=CARTESIAN_POINT('Ctrl Pts',(-30.3101336108046,14.0899140100411,
126.903186984993)) ;
#132660=CARTESIAN_POINT('Ctrl Pts',(-30.2730059348416,13.8386917046902,
126.761684342598)) ;
#132661=CARTESIAN_POINT('Ctrl Pts',(-30.2591454609719,13.5555692125345,
126.687892009024)) ;
#132662=CARTESIAN_POINT('Ctrl Pts',(-30.2703044262027,13.2663901180779,
126.687596604313)) ;
#132663=CARTESIAN_POINT('Ctrl Pts',(-30.3064563015578,12.9858847333076,
126.760012223785)) ;
#132664=CARTESIAN_POINT('Ctrl Pts',(-30.3656808780386,12.7375102459871,
126.899927974495)) ;
#132665=CARTESIAN_POINT('Ctrl Pts',(-30.4446592433479,12.5376376287816,
127.097461701573)) ;
#132666=CARTESIAN_POINT('Ctrl Pts',(-30.5383897496922,12.4015826977934,
127.338092518212)) ;
#132667=CARTESIAN_POINT('Ctrl Pts',(-30.6402554773558,12.3390360902595,
127.602664560348)) ;
#132668=CARTESIAN_POINT('Ctrl Pts',(-30.7445603425615,12.353575403094,127.874253187337)) ;
#132669=CARTESIAN_POINT('Ctrl Pts',(-30.8445423217259,12.445274073871,128.133104829671)) ;
#132670=CARTESIAN_POINT('Ctrl Pts',(-30.9331533396269,12.6067971683827,
128.358841764631)) ;
#132671=CARTESIAN_POINT('Ctrl Pts',(-31.0052235518519,12.8274892534517,
128.536166471027)) ;
#132672=CARTESIAN_POINT('Ctrl Pts',(-31.0557929024469,13.0891408927057,
128.650910668167)) ;
#132673=CARTESIAN_POINT('Ctrl Pts',(-31.0826649707566,13.375740122579,128.696283133412)) ;
#132674=CARTESIAN_POINT('Ctrl Pts',(-31.0842457464183,13.6659116032671,
128.667755109105)) ;
#132675=CARTESIAN_POINT('Ctrl Pts',(-31.0612969342213,13.9383430672958,
128.567621981036)) ;
#132676=CARTESIAN_POINT('Ctrl Pts',(-31.0158421470532,14.1747318786697,
128.401589927848)) ;
#132677=CARTESIAN_POINT('Ctrl Pts',(-30.952741170991,14.3556000224366,128.184334680318)) ;
#132678=CARTESIAN_POINT('Ctrl Pts',(-30.8757148543573,14.4715471852787,
127.925954832144)) ;
#132679=CARTESIAN_POINT('Ctrl Pts',(-30.7926989079768,14.5109306884899,
127.650429154449)) ;
#132680=CARTESIAN_POINT('Ctrl Pts',(-30.7096170404131,14.4734197510009,
127.374712802353)) ;
#132681=CARTESIAN_POINT('Ctrl Pts',(-30.6324207964218,14.3595613312843,
127.115883659408)) ;
#132682=CARTESIAN_POINT('Ctrl Pts',(-30.5687431637558,14.179466171533,126.896825275717)) ;
#132683=CARTESIAN_POINT('Ctrl Pts',(-30.5229949276125,13.9455181185487,
126.730115674649)) ;
#132684=CARTESIAN_POINT('Ctrl Pts',(-30.4993062024708,13.6723045745694,
126.627634301698)) ;
#132685=CARTESIAN_POINT('Ctrl Pts',(-30.5003214317798,13.3834915874396,
126.597593551244)) ;
#132686=CARTESIAN_POINT('Ctrl Pts',(-30.5264493139276,13.0966134068724,
126.640803917263)) ;
#132687=CARTESIAN_POINT('Ctrl Pts',(-30.5766713219404,12.8330521051259,
126.754396922064)) ;
#132688=CARTESIAN_POINT('Ctrl Pts',(-30.6483002280116,12.6112324338377,
126.930439181463)) ;
#132689=CARTESIAN_POINT('Ctrl Pts',(-30.736661695068,12.4482429025448,127.155425447181)) ;
#132690=CARTESIAN_POINT('Ctrl Pts',(-30.8357315528907,12.3553252392396,
127.411846833704)) ;
#132691=CARTESIAN_POINT('Ctrl Pts',(-30.9400335857783,12.3382107107946,
127.683413725756)) ;
#132692=CARTESIAN_POINT('Ctrl Pts',(-31.042636248853,12.3992481458877,127.94994445052)) ;
#132693=CARTESIAN_POINT('Ctrl Pts',(-31.1362393771601,12.5331204758664,
128.190343537901)) ;
#132694=CARTESIAN_POINT('Ctrl Pts',(-31.215635139957,12.7309387918669,128.389145202128)) ;
#132695=CARTESIAN_POINT('Ctrl Pts',(-31.2756357249041,12.9791524410526,
128.53120468286)) ;
#132696=CARTESIAN_POINT('Ctrl Pts',(-31.312400854353,13.2585790598106,128.605475928875)) ;
#132697=CARTESIAN_POINT('Ctrl Pts',(-31.3241836080649,13.5499397896395,
128.606744173026)) ;
#132698=CARTESIAN_POINT('Ctrl Pts',(-31.3110087346716,13.8311712407388,
128.535239748079)) ;
#132699=CARTESIAN_POINT('Ctrl Pts',(-31.2742363093329,14.0848085651835,
128.394579152518)) ;
#132700=CARTESIAN_POINT('Ctrl Pts',(-31.2178679894401,14.2892041446737,
128.196968022278)) ;
#132701=CARTESIAN_POINT('Ctrl Pts',(-31.1457920021485,14.4332159069687,
127.953199131549)) ;
#132702=CARTESIAN_POINT('Ctrl Pts',(-31.064501704361,14.5042073782218,127.682616508337)) ;
#132703=CARTESIAN_POINT('Ctrl Pts',(-30.9803569070733,14.4978850554144,
127.403677198383)) ;
#132704=CARTESIAN_POINT('Ctrl Pts',(-30.9001457048563,14.4145534025925,
127.136236709374)) ;
#132705=CARTESIAN_POINT('Ctrl Pts',(-30.8302915857101,14.2600830965558,
126.899030948309)) ;
#132706=CARTESIAN_POINT('Ctrl Pts',(-30.7766783037662,14.0459659620245,
126.70932486434)) ;
#132707=CARTESIAN_POINT('Ctrl Pts',(-30.7436688177568,13.7875807752627,
126.579828846178)) ;
#132708=CARTESIAN_POINT('Ctrl Pts',(-30.7344309347098,13.5015008973902,
126.519590640979)) ;
#132709=CARTESIAN_POINT('Ctrl Pts',(-30.7503570117774,13.2119712102584,
126.533117195425)) ;
#132710=CARTESIAN_POINT('Ctrl Pts',(-30.7909948356034,12.9363053782512,
126.618694908227)) ;
#132711=CARTESIAN_POINT('Ctrl Pts',(-30.8544313460082,12.6952736602129,
126.770815078882)) ;
#132712=CARTESIAN_POINT('Ctrl Pts',(-30.936259477995,12.507125678723,126.976810991267)) ;
#132713=CARTESIAN_POINT('Ctrl Pts',(-31.0324849838793,12.3837628513247,
127.224594411425)) ;
#132714=CARTESIAN_POINT('Ctrl Pts',(-31.1350680188049,12.3357954087756,
127.491330342941)) ;
#132715=CARTESIAN_POINT('Ctrl Pts',(-31.23935127795,12.3652711251859,127.762742575844)) ;
#132716=CARTESIAN_POINT('Ctrl Pts',(-31.3372466101365,12.4705156806676,
128.015655972246)) ;
#132717=CARTESIAN_POINT('Ctrl Pts',(-31.4231098978925,12.6439184973371,
128.233370607722)) ;
#132718=CARTESIAN_POINT('Ctrl Pts',(-31.4913656157794,12.8730354055636,
128.399662361953)) ;
#132719=CARTESIAN_POINT('Ctrl Pts',(-31.5379531663441,13.1424159445997,
128.502550794473)) ;
#132720=CARTESIAN_POINT('Ctrl Pts',(-31.5599892196137,13.4306391754528,
128.533873702179)) ;
#132721=CARTESIAN_POINT('Ctrl Pts',(-31.5568791607716,13.7191539441457,
128.491638388163)) ;
#132722=CARTESIAN_POINT('Ctrl Pts',(-31.5294551877072,13.9861293896989,
128.378414253767)) ;
#132723=CARTESIAN_POINT('Ctrl Pts',(-31.4804720297221,14.2128684001206,
128.202207341774)) ;
#132724=CARTESIAN_POINT('Ctrl Pts',(-31.4139631417804,14.3833347965248,
127.974731570058)) ;
#132725=CARTESIAN_POINT('Ctrl Pts',(-31.3357239804157,14.4845639099252,
127.713064266216)) ;
#132726=CARTESIAN_POINT('Ctrl Pts',(-31.2519760904658,14.5099092471542,
127.435310311413)) ;
#132727=CARTESIAN_POINT('Ctrl Pts',(-31.169269063561,14.4573341215463,127.160540128222)) ;
#132728=CARTESIAN_POINT('Ctrl Pts',(-31.0944827944426,14.3305258270945,
126.908931141692)) ;
#132729=CARTESIAN_POINT('Ctrl Pts',(-31.0337818947545,14.1393930806654,
126.698567894651)) ;
#132730=CARTESIAN_POINT('Ctrl Pts',(-30.991822622221,13.8963012865058,126.542832684996)) ;
#132731=CARTESIAN_POINT('Ctrl Pts',(-30.9727169093987,13.618527952916,126.453788104164)) ;
#132732=CARTESIAN_POINT('Ctrl Pts',(-30.9784116943508,13.3290638567204,
126.43746201239)) ;
#132733=CARTESIAN_POINT('Ctrl Pts',(-31.0092534744897,13.0445549081066,
126.494384804869)) ;
#132734=CARTESIAN_POINT('Ctrl Pts',(-31.0636975928906,12.7876683953407,
126.620329890945)) ;
#132735=CARTESIAN_POINT('Ctrl Pts',(-31.1390893626737,12.5753843248543,
126.807286162987)) ;
#132736=CARTESIAN_POINT('Ctrl Pts',(-31.2294856731981,12.4255194566962,
127.038405016624)) ;
#132737=CARTESIAN_POINT('Ctrl Pts',(-31.3305520361071,12.3459765628223,
127.300458413669)) ;
#132738=CARTESIAN_POINT('Ctrl Pts',(-31.434776599086,12.3439073333341,127.571874828474)) ;
#132739=CARTESIAN_POINT('Ctrl Pts',(-31.5361216061782,12.4188279963137,
127.834788869403)) ;
#132740=CARTESIAN_POINT('Ctrl Pts',(-31.6280697762185,12.5669347456838,
128.070100154879)) ;
#132741=CARTESIAN_POINT('Ctrl Pts',(-31.7035334984892,12.7740276750078,
128.257653591068)) ;
#132742=CARTESIAN_POINT('Ctrl Pts',(-31.759609829367,13.0302839963835,128.388157305165)) ;
#132743=CARTESIAN_POINT('Ctrl Pts',(-31.7916573927032,13.3133908418281,
128.44867020828)) ;
#132744=CARTESIAN_POINT('Ctrl Pts',(-31.7986966116337,13.603463644202,128.436213818987)) ;
#132745=CARTESIAN_POINT('Ctrl Pts',(-31.7809913371395,13.8813033828735,
128.35140974243)) ;
#132746=CARTESIAN_POINT('Ctrl Pts',(-31.7400851389627,14.1277803353935,
128.198621302036)) ;
#132747=CARTESIAN_POINT('Ctrl Pts',(-31.6800730695565,14.3222499491186,
127.990196055143)) ;
#132748=CARTESIAN_POINT('Ctrl Pts',(-31.6061655491007,14.4521801137134,
127.741284607191)) ;
#132749=CARTESIAN_POINT('Ctrl Pts',(-31.5238300942761,14.5090397013049,
127.467639877269)) ;
#132750=CARTESIAN_POINT('Ctrl Pts',(-31.4398666707468,14.4879536383768,
127.189213876511)) ;
#132751=CARTESIAN_POINT('Ctrl Pts',(-31.3611027665607,14.3907169193799,
126.925998091316)) ;
#132752=CARTESIAN_POINT('Ctrl Pts',(-31.2937040056646,14.2230874926912,
126.695841876849)) ;
#132753=CARTESIAN_POINT('Ctrl Pts',(-31.2439920013192,14.0008521290395,
126.517762290878)) ;
#132754=CARTESIAN_POINT('Ctrl Pts',(-31.2150907661555,13.7343152663338,
126.400042595703)) ;
#132755=CARTESIAN_POINT('Ctrl Pts',(-31.2106083276963,13.4474451530714,
126.353922032443)) ;
#132756=CARTESIAN_POINT('Ctrl Pts',(-31.2313383311631,13.1575373599845,
126.381288702569)) ;
#132757=CARTESIAN_POINT('Ctrl Pts',(-31.2764056532061,12.8878586186382,
126.479905180231)) ;
#132758=CARTESIAN_POINT('Ctrl Pts',(-31.3436059924202,12.6555337160297,
126.643048484565)) ;
#132759=CARTESIAN_POINT('Ctrl Pts',(-31.4286039772841,12.4784852863875,
126.858237182344)) ;
#132760=CARTESIAN_POINT('Ctrl Pts',(-31.5266156330296,12.3688435126028,
127.11128245237)) ;
#132761=CARTESIAN_POINT('Ctrl Pts',(-31.630084559127,12.335379050582,127.380536177025)) ;
#132762=CARTESIAN_POINT('Ctrl Pts',(-31.7333993373061,12.3794309050292,
127.649233966248)) ;
#132763=CARTESIAN_POINT('Ctrl Pts',(-31.8295546512421,12.4979553005814,
127.897051153347)) ;
#132764=CARTESIAN_POINT('Ctrl Pts',(-31.9129345986958,12.6843641512771,
128.107301604166)) ;
#132765=CARTESIAN_POINT('Ctrl Pts',(-31.9769081760024,12.9208195190715,
128.261300839291)) ;
#132766=CARTESIAN_POINT('Ctrl Pts',(-32.0192234596835,13.1965599156971,
128.351576775379)) ;
#132767=CARTESIAN_POINT('Ctrl Pts',(-32.0364080377691,13.4854150034454,
128.36882968244)) ;
#132768=CARTESIAN_POINT('Ctrl Pts',(-32.0286590942519,13.7715245103546,
128.313041033143)) ;
#132769=CARTESIAN_POINT('Ctrl Pts',(-31.9967949405779,14.0329603333754,
128.186757372476)) ;
#132770=CARTESIAN_POINT('Ctrl Pts',(-31.9442598511563,14.2495174070446,
128.000252912401)) ;
#132771=CARTESIAN_POINT('Ctrl Pts',(-31.8752637456382,14.4077221355952,
127.765584521541)) ;
#132772=CARTESIAN_POINT('Ctrl Pts',(-31.7949904880439,14.4954974794661,
127.497773147365)) ;
#132773=CARTESIAN_POINT('Ctrl Pts',(-31.7112118667338,14.5058124227374,
127.220036909701)) ;
#132774=CARTESIAN_POINT('Ctrl Pts',(-31.6295895835472,14.4390540160987,
126.948477953836)) ;
#132775=CARTESIAN_POINT('Ctrl Pts',(-31.5567958768622,14.2988995016989,
126.702614005723)) ;
#132776=CARTESIAN_POINT('Ctrl Pts',(-31.4992152164798,14.0959846822767,
126.501253268444)) ;
#132777=CARTESIAN_POINT('Ctrl Pts',(-31.4616155663629,13.8467238077785,
126.358483470145)) ;
#132778=CARTESIAN_POINT('Ctrl Pts',(-31.4469797675735,13.5651499595772,
126.282529118317)) ;
#132779=CARTESIAN_POINT('Ctrl Pts',(-31.4573898379876,13.2745210705863,
126.279884269193)) ;
#132780=CARTESIAN_POINT('Ctrl Pts',(-31.4929777781403,12.9930481847516,
126.350603500459)) ;
#132781=CARTESIAN_POINT('Ctrl Pts',(-31.5514293278227,12.7442685275202,
126.488355718607)) ;
#132782=CARTESIAN_POINT('Ctrl Pts',(-31.629789771733,12.5428869624623,126.684118709821)) ;
#132783=CARTESIAN_POINT('Ctrl Pts',(-31.7230911251259,12.4047083280592,
126.923514916853)) ;
#132784=CARTESIAN_POINT('Ctrl Pts',(-31.8251196709966,12.3396945526809,
127.188456991403)) ;
#132785=CARTESIAN_POINT('Ctrl Pts',(-31.9293847768492,12.3521469576885,
127.459951466802)) ;
#132786=CARTESIAN_POINT('Ctrl Pts',(-32.0293584096416,12.441314353945,127.718862688757)) ;
#132787=CARTESIAN_POINT('Ctrl Pts',(-32.118508034267,12.6011043288198,127.946125196227)) ;
#132788=CARTESIAN_POINT('Ctrl Pts',(-32.1909463624357,12.8194224397463,
128.124637671274)) ;
#132789=CARTESIAN_POINT('Ctrl Pts',(-32.2424853469496,13.0811434342732,
128.242065843194)) ;
#132790=CARTESIAN_POINT('Ctrl Pts',(-32.2700475124695,13.3679217852881,
128.289393931887)) ;
#132791=CARTESIAN_POINT('Ctrl Pts',(-32.2723234688677,13.6574454003315,
128.262990706036)) ;
#132792=CARTESIAN_POINT('Ctrl Pts',(-32.2501377563472,13.9304218890574,
128.16512094437)) ;
#132793=CARTESIAN_POINT('Ctrl Pts',(-32.2052527136117,14.1686008595605,
128.000705406738)) ;
#132794=CARTESIAN_POINT('Ctrl Pts',(-32.1424368825761,14.3514046814191,
127.78421431945)) ;
#132795=CARTESIAN_POINT('Ctrl Pts',(-32.0661890017219,14.4688537010489,
127.528311842842)) ;
#132796=CARTESIAN_POINT('Ctrl Pts',(-31.9829477124764,14.5110084065472,
127.25198980975)) ;
#132797=CARTESIAN_POINT('Ctrl Pts',(-31.8996523370137,14.4754271659884,
126.975598872173)) ;
#132798=CARTESIAN_POINT('Ctrl Pts',(-31.8224332847297,14.3641624802179,
126.716820698264)) ;
#132799=CARTESIAN_POINT('Ctrl Pts',(-31.7580395500746,14.1852632695012,
126.495546204119)) ;
#132800=CARTESIAN_POINT('Ctrl Pts',(-31.7118161309124,13.9526451401233,
126.327472065972)) ;
#132801=CARTESIAN_POINT('Ctrl Pts',(-31.6875151171821,13.6818447118076,
126.223384381321)) ;
#132802=CARTESIAN_POINT('Ctrl Pts',(-31.6876428707132,13.3926206452482,
126.190673672069)) ;
#132803=CARTESIAN_POINT('Ctrl Pts',(-31.7132303697958,13.1038754923078,
126.232132655585)) ;
#132804=CARTESIAN_POINT('Ctrl Pts',(-31.7626844305404,12.8403836297391,
126.343597807942)) ;
#132805=CARTESIAN_POINT('Ctrl Pts',(-31.833493429736,12.6175434576375,126.517332769775)) ;
#132806=CARTESIAN_POINT('Ctrl Pts',(-31.9215930084005,12.4520178789147,
126.741478574285)) ;
#132807=CARTESIAN_POINT('Ctrl Pts',(-32.0209307914902,12.3567780608222,
126.998523271918)) ;
#132808=CARTESIAN_POINT('Ctrl Pts',(-32.1246416504795,12.3376561109864,
127.268538964137)) ;
#132809=CARTESIAN_POINT('Ctrl Pts',(-32.2275246940126,12.3963494804203,
127.535847716125)) ;
#132810=CARTESIAN_POINT('Ctrl Pts',(-32.3214673626583,12.5282529228556,
127.777238677115)) ;
#132811=CARTESIAN_POINT('Ctrl Pts',(-32.4013423719323,12.7243873042916,
127.977442347176)) ;
#132812=CARTESIAN_POINT('Ctrl Pts',(-32.4619096573449,12.9708923918956,
128.121216797039)) ;
#132813=CARTESIAN_POINT('Ctrl Pts',(-32.4994416556502,13.2502126197918,
128.197659332614)) ;
#132814=CARTESIAN_POINT('Ctrl Pts',(-32.5119978982385,13.5400583828972,
128.201358931735)) ;
#132815=CARTESIAN_POINT('Ctrl Pts',(-32.4994888167825,13.8239338286533,
128.131553230696)) ;
#132816=CARTESIAN_POINT('Ctrl Pts',(-32.4634273595897,14.0777676729547,
127.99308635593)) ;
#132817=CARTESIAN_POINT('Ctrl Pts',(-32.4075028614965,14.2841378500946,
127.796711420429)) ;
#132818=CARTESIAN_POINT('Ctrl Pts',(-32.3359847249591,14.429815657766,127.554661094343)) ;
#132819=CARTESIAN_POINT('Ctrl Pts',(-32.2546028623038,14.5033259168077,
127.283693381333)) ;
#132820=CARTESIAN_POINT('Ctrl Pts',(-32.1704924928081,14.499135115111,127.004877771061)) ;
#132821=CARTESIAN_POINT('Ctrl Pts',(-32.0900191687497,14.4177798325381,
126.736640312097)) ;
#132822=CARTESIAN_POINT('Ctrl Pts',(-32.0200109297833,14.2657377102023,
126.499094130843)) ;
#132823=CARTESIAN_POINT('Ctrl Pts',(-31.9656700623202,14.0527574173429,
126.30717910773)) ;
#132824=CARTESIAN_POINT('Ctrl Pts',(-31.9319934820835,13.7942044324148,
126.175602610685)) ;
#132825=CARTESIAN_POINT('Ctrl Pts',(-31.922152144827,13.509972220369,126.1137676569)) ;
#132826=CARTESIAN_POINT('Ctrl Pts',(-31.9373531303038,13.219834764377,126.12511889965)) ;
#132827=CARTESIAN_POINT('Ctrl Pts',(-31.9773715779164,12.9433154987134,
126.208868906181)) ;
#132828=CARTESIAN_POINT('Ctrl Pts',(-32.0403631928475,12.7008042356819,
126.359640175799)) ;
#132829=CARTESIAN_POINT('Ctrl Pts',(-32.1214625671299,12.5118988342583,
126.563632155226)) ;
#132830=CARTESIAN_POINT('Ctrl Pts',(-32.2168510067031,12.3867144480253,
126.809132213192)) ;
#132831=CARTESIAN_POINT('Ctrl Pts',(-32.3199033888381,12.3359851161897,
127.077044236849)) ;
#132832=CARTESIAN_POINT('Ctrl Pts',(-32.4242222709057,12.3634203970633,
127.348571063411)) ;
#132833=CARTESIAN_POINT('Ctrl Pts',(-32.5223579803355,12.4663876358086,
127.602200216398)) ;
#132834=CARTESIAN_POINT('Ctrl Pts',(-32.6089883742709,12.6389701182042,
127.82200642748)) ;
#132835=CARTESIAN_POINT('Ctrl Pts',(-32.6774297887948,12.8657474577828,
127.988998597794)) ;
#132836=CARTESIAN_POINT('Ctrl Pts',(-32.724805208469,13.1346343436699,128.094136048027)) ;
#132837=CARTESIAN_POINT('Ctrl Pts',(-32.7399114943369,13.3266512177486,
128.116225545094)) ;
#132838=CARTESIAN_POINT('Ctrl Pts',(-32.7433109767759,13.4226801736581,
128.115135559137)) ;
#132839=CARTESIAN_POINT('',(-11.2812798643659,13.1551399285885,133.225361312885)) ;
#132840=CARTESIAN_POINT('',(-21.9982570673691,12.9778651918053,129.622952131535)) ;
#132841=CARTESIAN_POINT('Ctrl Pts',(-11.2812798643659,13.1551399285885,
133.225361312885)) ;
#132842=CARTESIAN_POINT('Ctrl Pts',(-11.2820187647633,13.1489709609094,
133.226788867079)) ;
#132843=CARTESIAN_POINT('Ctrl Pts',(-11.2940725891313,13.0505878441039,
133.250318667877)) ;
#132844=CARTESIAN_POINT('Ctrl Pts',(-11.3268196692865,12.8648900473044,
133.323006215356)) ;
#132845=CARTESIAN_POINT('Ctrl Pts',(-11.3955581347561,12.6378996894465,
133.490786092827)) ;
#132846=CARTESIAN_POINT('Ctrl Pts',(-11.4818126038911,12.4661938442505,
133.709651137204)) ;
#132847=CARTESIAN_POINT('Ctrl Pts',(-11.5806418499012,12.3629468779938,
133.965082777503)) ;
#132848=CARTESIAN_POINT('Ctrl Pts',(-11.6840920756584,12.3360866578135,
134.234357728742)) ;
#132849=CARTESIAN_POINT('Ctrl Pts',(-11.7874232958009,12.3868467815327,
134.502988211751)) ;
#132850=CARTESIAN_POINT('Ctrl Pts',(-11.8826517586958,12.5118616193735,
134.748082512994)) ;
#132851=CARTESIAN_POINT('Ctrl Pts',(-11.9642364503466,12.7022376314793,
134.953268302114)) ;
#132852=CARTESIAN_POINT('Ctrl Pts',(-12.0268555159077,12.9442211340136,
135.103070944459)) ;
#132853=CARTESIAN_POINT('Ctrl Pts',(-12.0667868417897,13.2203922331636,
135.186606249474)) ;
#132854=CARTESIAN_POINT('Ctrl Pts',(-12.0819921567622,13.5109001041669,
135.197934267535)) ;
#132855=CARTESIAN_POINT('Ctrl Pts',(-12.0718871830781,13.7967277450532,
135.135125417403)) ;
#132856=CARTESIAN_POINT('Ctrl Pts',(-12.0382787552941,14.0531634695327,
135.003985075531)) ;
#132857=CARTESIAN_POINT('Ctrl Pts',(-11.984040511163,14.2659161102292,134.812412340654)) ;
#132858=CARTESIAN_POINT('Ctrl Pts',(-11.9138317313736,14.4182155312585,
134.574200139104)) ;
#132859=CARTESIAN_POINT('Ctrl Pts',(-11.8331828494072,14.4993926065239,
134.305392211434)) ;
#132860=CARTESIAN_POINT('Ctrl Pts',(-11.7490444838035,14.5030674016304,
134.026483130585)) ;
#132861=CARTESIAN_POINT('Ctrl Pts',(-11.6680809986179,14.4296658181567,
133.756898311423)) ;
#132862=CARTESIAN_POINT('Ctrl Pts',(-11.5965958202758,14.2842405620309,
133.514968656249)) ;
#132863=CARTESIAN_POINT('Ctrl Pts',(-11.5404239481228,14.0768885755418,
133.31772524141)) ;
#132864=CARTESIAN_POINT('Ctrl Pts',(-11.5044626643021,13.821937566696,133.179448820527)) ;
#132865=CARTESIAN_POINT('Ctrl Pts',(-11.492115437901,13.5404397832619,133.110400577556)) ;
#132866=CARTESIAN_POINT('Ctrl Pts',(-11.5046895368218,13.2491903771815,
133.113990718504)) ;
#132867=CARTESIAN_POINT('Ctrl Pts',(-11.5423996819585,12.9699188880577,
133.190943520196)) ;
#132868=CARTESIAN_POINT('Ctrl Pts',(-11.6027127193453,12.7245502986717,
133.33412175314)) ;
#132869=CARTESIAN_POINT('Ctrl Pts',(-11.6827307770101,12.5279694687298,
133.534676781188)) ;
#132870=CARTESIAN_POINT('Ctrl Pts',(-11.7767909409935,12.3961377043517,
133.7763823545)) ;
#132871=CARTESIAN_POINT('Ctrl Pts',(-11.8796482494039,12.3376103677892,
134.043626665423)) ;
#132872=CARTESIAN_POINT('Ctrl Pts',(-11.9835249356267,12.3569098529355,
134.314074542349)) ;
#132873=CARTESIAN_POINT('Ctrl Pts',(-12.0830151650733,12.452769019898,134.571498333322)) ;
#132874=CARTESIAN_POINT('Ctrl Pts',(-12.1707022339469,12.6179593573441,
134.794565234874)) ;
#132875=CARTESIAN_POINT('Ctrl Pts',(-12.2415306520725,12.8405880377693,
134.968374154773)) ;
#132876=CARTESIAN_POINT('Ctrl Pts',(-12.2912076318387,13.1065246421439,
135.080214865833)) ;
#132877=CARTESIAN_POINT('Ctrl Pts',(-12.3163775691246,13.3925179674891,
135.12078307657)) ;
#132878=CARTESIAN_POINT('Ctrl Pts',(-12.3166058496797,13.6819916651313,
135.088335546118)) ;
#132879=CARTESIAN_POINT('Ctrl Pts',(-12.2921472081091,13.9537242418059,
134.983669295533)) ;
#132880=CARTESIAN_POINT('Ctrl Pts',(-12.2457390773696,14.1863734291659,
134.815010882744)) ;
#132881=CARTESIAN_POINT('Ctrl Pts',(-12.1814800516644,14.3643807985693,
134.59423567404)) ;
#132882=CARTESIAN_POINT('Ctrl Pts',(-12.1044683457898,14.4754559850244,
134.336147922274)) ;
#132883=CARTESIAN_POINT('Ctrl Pts',(-12.0208090250937,14.5110246739577,
134.058551574174)) ;
#132884=CARTESIAN_POINT('Ctrl Pts',(-11.9378612224862,14.4687063588107,
133.783197368949)) ;
#132885=CARTESIAN_POINT('Ctrl Pts',(-11.8615647632541,14.3514018815055,
133.527145574601)) ;
#132886=CARTESIAN_POINT('Ctrl Pts',(-11.798502564401,14.1671964752596,133.309749293991)) ;
#132887=CARTESIAN_POINT('Ctrl Pts',(-11.754049052173,13.9308608041133,133.146872132253)) ;
#132888=CARTESIAN_POINT('Ctrl Pts',(-11.7316977644638,13.6570089999716,
133.048397750488)) ;
#132889=CARTESIAN_POINT('Ctrl Pts',(-11.7341180951435,13.3664659574419,
133.022308686926)) ;
#132890=CARTESIAN_POINT('Ctrl Pts',(-11.761720921654,13.0805681472547,133.069846022257)) ;
#132891=CARTESIAN_POINT('Ctrl Pts',(-11.8131936002259,12.8190539470386,
133.187112979174)) ;
#132892=CARTESIAN_POINT('Ctrl Pts',(-11.886092857491,12.5999338423892,133.366806137464)) ;
#132893=CARTESIAN_POINT('Ctrl Pts',(-11.9747587487869,12.4413957528131,
133.592859241921)) ;
#132894=CARTESIAN_POINT('Ctrl Pts',(-12.0748052338517,12.3520378265489,
133.85195165464)) ;
#132895=CARTESIAN_POINT('Ctrl Pts',(-12.1791704719716,12.339734386482,134.123710421306)) ;
#132896=CARTESIAN_POINT('Ctrl Pts',(-12.2811942198852,12.4049383167358,
134.388634754176)) ;
#132897=CARTESIAN_POINT('Ctrl Pts',(-12.3743104910804,12.5429634979505,
134.627548525017)) ;
#132898=CARTESIAN_POINT('Ctrl Pts',(-12.4527350962615,12.7443553986761,
134.823486021638)) ;
#132899=CARTESIAN_POINT('Ctrl Pts',(-12.5113245953194,12.9943521537239,
134.961502568807)) ;
#132900=CARTESIAN_POINT('Ctrl Pts',(-12.5466491191103,13.2741647768729,
135.031655728832)) ;
#132901=CARTESIAN_POINT('Ctrl Pts',(-12.557133530808,13.565720269456,135.029118946566)) ;
#132902=CARTESIAN_POINT('Ctrl Pts',(-12.5424084976818,13.8474315556546,
134.952884078473)) ;
#132903=CARTESIAN_POINT('Ctrl Pts',(-12.504658245782,14.0971649669908,134.809596596871)) ;
#132904=CARTESIAN_POINT('Ctrl Pts',(-12.4468015681524,14.3002122843455,
134.607345660129)) ;
#132905=CARTESIAN_POINT('Ctrl Pts',(-12.3740820116557,14.4394509674979,
134.361774496034)) ;
#132906=CARTESIAN_POINT('Ctrl Pts',(-12.2928286579386,14.5058688200503,
134.091445642351)) ;
#132907=CARTESIAN_POINT('Ctrl Pts',(-12.2085754911848,14.4952594831202,
133.812133112469)) ;
#132908=CARTESIAN_POINT('Ctrl Pts',(-12.1285286312613,14.4071576912799,
133.54505905862)) ;
#132909=CARTESIAN_POINT('Ctrl Pts',(-12.0595995840032,14.2488070341169,
133.310594609379)) ;
#132910=CARTESIAN_POINT('Ctrl Pts',(-12.007204001394,14.032332595662,133.124541926762)) ;
#132911=CARTESIAN_POINT('Ctrl Pts',(-11.9754518623539,13.7715185673777,
132.998664946929)) ;
#132912=CARTESIAN_POINT('Ctrl Pts',(-11.9676077024159,13.4849968555095,
132.942553623633)) ;
#132913=CARTESIAN_POINT('Ctrl Pts',(-11.9852141495617,13.1936954317484,
132.960744777079)) ;
#132914=CARTESIAN_POINT('Ctrl Pts',(-12.0270155274854,12.9217410981826,
133.049976934939)) ;
#132915=CARTESIAN_POINT('Ctrl Pts',(-12.0916442917843,12.6826993167214,
133.205531163459)) ;
#132916=CARTESIAN_POINT('Ctrl Pts',(-12.1748344849184,12.4976839220085,
133.415374259801)) ;
#132917=CARTESIAN_POINT('Ctrl Pts',(-12.2706003786281,12.3794711428103,
133.662174391645)) ;
#132918=CARTESIAN_POINT('Ctrl Pts',(-12.3744503899862,12.3351744196322,
133.932269165389)) ;
#132919=CARTESIAN_POINT('Ctrl Pts',(-12.4782650208009,12.3695012763354,
134.202412750315)) ;
#132920=CARTESIAN_POINT('Ctrl Pts',(-12.5754721648271,12.4786183736045,
134.453365352351)) ;
#132921=CARTESIAN_POINT('Ctrl Pts',(-12.6605578265862,12.6556201701116,
134.668788412585)) ;
#132922=CARTESIAN_POINT('Ctrl Pts',(-12.7278290779799,12.8885376957079,
134.832076052564)) ;
#132923=CARTESIAN_POINT('Ctrl Pts',(-12.7727942038789,13.1578672277872,
134.93044163856)) ;
#132924=CARTESIAN_POINT('Ctrl Pts',(-12.7935589960753,13.4488181058444,
134.957796140316)) ;
#132925=CARTESIAN_POINT('Ctrl Pts',(-12.7888443918457,13.7357351250712,
134.91097260511)) ;
#132926=CARTESIAN_POINT('Ctrl Pts',(-12.7602605916963,14.0000244154435,
134.794478626913)) ;
#132927=CARTESIAN_POINT('Ctrl Pts',(-12.7099141607957,14.2248063693443,
134.614145960045)) ;
#132928=CARTESIAN_POINT('Ctrl Pts',(-12.6428897963242,14.3907221531774,
134.385334239461)) ;
#132929=CARTESIAN_POINT('Ctrl Pts',(-12.5640447774941,14.4880878052934,
134.121834427977)) ;
#132930=CARTESIAN_POINT('Ctrl Pts',(-12.4802617689659,14.5090844515927,
133.844015139513)) ;
#132931=CARTESIAN_POINT('Ctrl Pts',(-12.3974642832698,14.4517331277302,
133.568827359843)) ;
#132932=CARTESIAN_POINT('Ctrl Pts',(-12.3236763447296,14.3213873494252,
133.320287858352)) ;
#132933=CARTESIAN_POINT('Ctrl Pts',(-12.2637347152158,14.1266126254878,
133.112060420808)) ;
#132934=CARTESIAN_POINT('Ctrl Pts',(-12.2229774667805,13.8801113803002,
132.959735466426)) ;
#132935=CARTESIAN_POINT('Ctrl Pts',(-12.2053838579744,13.6025840232108,
132.875302084043)) ;
#132936=CARTESIAN_POINT('Ctrl Pts',(-12.2124772397581,13.3122088978665,
132.862974191922)) ;
#132937=CARTESIAN_POINT('Ctrl Pts',(-12.2448145015933,13.0284665595888,
132.924236901387)) ;
#132938=CARTESIAN_POINT('Ctrl Pts',(-12.3005599019218,12.7739765033465,
133.053999198988)) ;
#132939=CARTESIAN_POINT('Ctrl Pts',(-12.3766445028271,12.5655228915478,
133.243117582921)) ;
#132940=CARTESIAN_POINT('Ctrl Pts',(-12.4681423855166,12.4188418488155,
133.47731500825)) ;
#132941=CARTESIAN_POINT('Ctrl Pts',(-12.5692422546882,12.3438198182334,
133.739584235759)) ;
#132942=CARTESIAN_POINT('Ctrl Pts',(-12.6740334889537,12.3461749880073,
134.012474638995)) ;
#132943=CARTESIAN_POINT('Ctrl Pts',(-12.7747162224539,12.4256199459212,
134.273532924423)) ;
#132944=CARTESIAN_POINT('Ctrl Pts',(-12.8655945356852,12.5766359900473,
134.505860328425)) ;
#132945=CARTESIAN_POINT('Ctrl Pts',(-12.9405208029623,12.7882864475543,
134.691614915467)) ;
#132946=CARTESIAN_POINT('Ctrl Pts',(-12.9949316879518,13.0452019382586,
134.817458837911)) ;
#132947=CARTESIAN_POINT('Ctrl Pts',(-13.025720643168,13.3293877258915,134.874271333741)) ;
#132948=CARTESIAN_POINT('Ctrl Pts',(-13.0313457796955,13.6204035856812,
134.857561997613)) ;
#132949=CARTESIAN_POINT('Ctrl Pts',(-13.0121238177563,13.8971496153171,
134.768280402699)) ;
#132950=CARTESIAN_POINT('Ctrl Pts',(-12.9702433337836,14.1397539052331,
134.612839445253)) ;
#132951=CARTESIAN_POINT('Ctrl Pts',(-12.9092683557999,14.3313464702874,
134.401559637406)) ;
#132952=CARTESIAN_POINT('Ctrl Pts',(-12.8346344667875,14.4574458616527,
134.150487900523)) ;
#132953=CARTESIAN_POINT('Ctrl Pts',(-12.7520232585293,14.5099723944026,
133.876034599555)) ;
#132954=CARTESIAN_POINT('Ctrl Pts',(-12.6680149991839,14.4843439695083,
133.597416296755)) ;
#132955=CARTESIAN_POINT('Ctrl Pts',(-12.5898605639027,14.3827749410654,
133.336012913517)) ;
#132956=CARTESIAN_POINT('Ctrl Pts',(-12.5235110131134,14.2124739950545,
133.109063094795)) ;
#132957=CARTESIAN_POINT('Ctrl Pts',(-12.47454385575,13.9855789386979,132.932891873958)) ;
#132958=CARTESIAN_POINT('Ctrl Pts',(-12.44718714331,13.7185805864342,132.819871229684)) ;
#132959=CARTESIAN_POINT('Ctrl Pts',(-12.4441083202369,13.4303185636673,
132.777757800251)) ;
#132960=CARTESIAN_POINT('Ctrl Pts',(-12.4662081675216,13.1417758325219,
132.809228396078)) ;
#132961=CARTESIAN_POINT('Ctrl Pts',(-12.5128438608682,12.8725286043858,
132.912265477798)) ;
#132962=CARTESIAN_POINT('Ctrl Pts',(-12.5811355936144,12.6435096258014,
133.078662360882)) ;
#132963=CARTESIAN_POINT('Ctrl Pts',(-12.6670557983815,12.4701546223289,
133.296533072804)) ;
#132964=CARTESIAN_POINT('Ctrl Pts',(-12.7650980875458,12.3650501876111,
133.549835459936)) ;
#132965=CARTESIAN_POINT('Ctrl Pts',(-12.8692895553206,12.3357586674927,
133.821013809302)) ;
#132966=CARTESIAN_POINT('Ctrl Pts',(-12.9722194636702,12.3843195509594,
134.088641190149)) ;
#132967=CARTESIAN_POINT('Ctrl Pts',(-13.0679235169665,12.5073666683789,
134.335069106556)) ;
#132968=CARTESIAN_POINT('Ctrl Pts',(-13.1498474421669,12.6958200369819,
134.541296314724)) ;
#132969=CARTESIAN_POINT('Ctrl Pts',(-13.2130846476701,12.9363649293222,
134.692916583502)) ;
#132970=CARTESIAN_POINT('Ctrl Pts',(-13.2537553284003,13.212046231595,134.778583028313)) ;
#132971=CARTESIAN_POINT('Ctrl Pts',(-13.2696867588976,13.5022481067603,
134.792052779991)) ;
#132972=CARTESIAN_POINT('Ctrl Pts',(-13.2603291226857,13.7884016128943,
134.731444216182)) ;
#132973=CARTESIAN_POINT('Ctrl Pts',(-13.2274358441086,14.045945075732,134.602400846472)) ;
#132974=CARTESIAN_POINT('Ctrl Pts',(-13.1734739345736,14.2610680704969,
134.41149155897)) ;
#132975=CARTESIAN_POINT('Ctrl Pts',(-13.1038966633744,14.4145624165552,
134.175255364668)) ;
#132976=CARTESIAN_POINT('Ctrl Pts',(-13.0234728088093,14.4980852125695,
133.907100960487)) ;
#132977=CARTESIAN_POINT('Ctrl Pts',(-12.939325995419,14.5041312739862,133.628163299805)) ;
#132978=CARTESIAN_POINT('Ctrl Pts',(-12.8580140805557,14.4326962339747,
133.357486536545)) ;
#132979=CARTESIAN_POINT('Ctrl Pts',(-12.7862358410937,14.289424830309,133.114743545619)) ;
#132980=CARTESIAN_POINT('Ctrl Pts',(-12.7294171395877,14.0826507854277,
132.915479459106)) ;
#132981=CARTESIAN_POINT('Ctrl Pts',(-12.6931113261045,13.8312291814697,
132.77650858526)) ;
#132982=CARTESIAN_POINT('Ctrl Pts',(-12.6798565616288,13.5479805821752,
132.704527307887)) ;
#132983=CARTESIAN_POINT('Ctrl Pts',(-12.6918329131031,13.2572981016289,
132.706442366543)) ;
#132984=CARTESIAN_POINT('Ctrl Pts',(-12.7286154648152,12.9781391944844,
132.780789668285)) ;
#132985=CARTESIAN_POINT('Ctrl Pts',(-12.788841308569,12.7298471383749,132.923457407859)) ;
#132986=CARTESIAN_POINT('Ctrl Pts',(-12.8678064119023,12.5331718510569,
133.121190067536)) ;
#132987=CARTESIAN_POINT('Ctrl Pts',(-12.9619860922532,12.3987050488903,
133.3630746114)) ;
#132988=CARTESIAN_POINT('Ctrl Pts',(-13.0641173669679,12.3381977133859,
133.628393862531)) ;
#132989=CARTESIAN_POINT('Ctrl Pts',(-13.1689636586994,12.3556285786372,
133.901368958815)) ;
#132990=CARTESIAN_POINT('Ctrl Pts',(-13.2676215267395,12.448498640132,134.156721062578)) ;
#132991=CARTESIAN_POINT('Ctrl Pts',(-13.3562794099848,12.6124651727369,
134.382428532808)) ;
#132992=CARTESIAN_POINT('Ctrl Pts',(-13.4274024159188,12.8330193864531,
134.55721035227)) ;
#132993=CARTESIAN_POINT('Ctrl Pts',(-13.4778657839761,13.0981216515098,
134.671314825157)) ;
#132994=CARTESIAN_POINT('Ctrl Pts',(-13.5037873702561,13.3840423616995,
134.714047923931)) ;
#132995=CARTESIAN_POINT('Ctrl Pts',(-13.5047230832927,13.6738043197191,
134.683656575562)) ;
#132996=CARTESIAN_POINT('Ctrl Pts',(-13.4810350619758,13.9458856450603,
134.581307831703)) ;
#132997=CARTESIAN_POINT('Ctrl Pts',(-13.4350850950003,14.1805609741337,
134.413888828413)) ;
#132998=CARTESIAN_POINT('Ctrl Pts',(-13.3713435625267,14.3602096703021,
134.19466352274)) ;
#132999=CARTESIAN_POINT('Ctrl Pts',(-13.2941228668166,14.4737146563849,
133.935766751957)) ;
#133000=CARTESIAN_POINT('Ctrl Pts',(-13.2111150371913,14.510981736058,133.660304806086)) ;
#133001=CARTESIAN_POINT('Ctrl Pts',(-13.1279555516473,14.4710234538019,
133.384286573336)) ;
#133002=CARTESIAN_POINT('Ctrl Pts',(-13.0514607207591,14.3558611755068,
133.127695259553)) ;
#133003=CARTESIAN_POINT('Ctrl Pts',(-12.987929872837,14.1736059642118,132.908940703681)) ;
#133004=CARTESIAN_POINT('Ctrl Pts',(-12.9427874558613,13.9381264816024,
132.743987191645)) ;
#133005=CARTESIAN_POINT('Ctrl Pts',(-12.9198159126567,13.665192099168,132.643720985883)) ;
#133006=CARTESIAN_POINT('Ctrl Pts',(-12.9214159568252,13.3755914984187,
132.615321479283)) ;
#133007=CARTESIAN_POINT('Ctrl Pts',(-12.9485033871058,13.0874857506397,
132.661141600498)) ;
#133008=CARTESIAN_POINT('Ctrl Pts',(-12.9991534842726,12.8264337657975,
132.776172659393)) ;
#133009=CARTESIAN_POINT('Ctrl Pts',(-13.0712502877118,12.6060974389448,
132.953593799865)) ;
#133010=CARTESIAN_POINT('Ctrl Pts',(-13.1597261697062,12.4450313389733,
133.179001034814)) ;
#133011=CARTESIAN_POINT('Ctrl Pts',(-13.2598221399245,12.3534666197661,
133.438152169847)) ;
#133012=CARTESIAN_POINT('Ctrl Pts',(-13.3638496997786,12.3390029903486,
133.709021457282)) ;
#133013=CARTESIAN_POINT('Ctrl Pts',(-13.466268319613,12.4020392430349,133.975026492123)) ;
#133014=CARTESIAN_POINT('Ctrl Pts',(-13.5598211640111,12.5385711173323,
134.215165246668)) ;
#133015=CARTESIAN_POINT('Ctrl Pts',(-13.6383382505058,12.737337324062,134.411540597844)) ;
#133016=CARTESIAN_POINT('Ctrl Pts',(-13.6976697861643,12.9861206892308,
134.551707741949)) ;
#133017=CARTESIAN_POINT('Ctrl Pts',(-13.7337928936498,13.2660910782566,
134.62410596592)) ;
#133018=CARTESIAN_POINT('Ctrl Pts',(-13.7449404119012,13.5573227840952,
134.623538746113)) ;
#133019=CARTESIAN_POINT('Ctrl Pts',(-13.731057609949,13.8386952169897,134.549882879065)) ;
#133020=CARTESIAN_POINT('Ctrl Pts',(-13.6938267710482,14.0906007554108,
134.407982826979)) ;
#133021=CARTESIAN_POINT('Ctrl Pts',(-13.6366983945426,14.2945039762926,
134.207985282423)) ;
#133022=CARTESIAN_POINT('Ctrl Pts',(-13.5643971905334,14.4361574187858,
133.963631330981)) ;
#133023=CARTESIAN_POINT('Ctrl Pts',(-13.4829079562931,14.5051117570611,
133.692450855681)) ;
#133024=CARTESIAN_POINT('Ctrl Pts',(-13.398865589322,14.496582620466,133.413844416583)) ;
#133025=CARTESIAN_POINT('Ctrl Pts',(-13.3188758691256,14.4113394819302,
133.147064384826)) ;
#133026=CARTESIAN_POINT('Ctrl Pts',(-13.2492482094451,14.2546479447355,
132.910444808226)) ;
#133027=CARTESIAN_POINT('Ctrl Pts',(-13.1961963849046,14.039143877786,132.722400695126)) ;
#133028=CARTESIAN_POINT('Ctrl Pts',(-13.1638347550569,13.7793416572316,
132.594749383636)) ;
#133029=CARTESIAN_POINT('Ctrl Pts',(-13.1552775077889,13.4941095874199,
132.536650789137)) ;
#133030=CARTESIAN_POINT('Ctrl Pts',(-13.1720447629105,13.2026874966814,
132.552397812081)) ;
#133031=CARTESIAN_POINT('Ctrl Pts',(-13.2133004298939,12.928833346161,132.639904988231)) ;
#133032=CARTESIAN_POINT('Ctrl Pts',(-13.2774801251183,12.6885083712283,
132.794116581438)) ;
#133033=CARTESIAN_POINT('Ctrl Pts',(-13.3597053837363,12.5026390795781,
133.001327621254)) ;
#133034=CARTESIAN_POINT('Ctrl Pts',(-13.455701350823,12.3816810236162,133.248611444686)) ;
#133035=CARTESIAN_POINT('Ctrl Pts',(-13.5588450701788,12.3354826595071,
133.516837122875)) ;
#133036=CARTESIAN_POINT('Ctrl Pts',(-13.662986257812,12.3671988660942,133.787859387829)) ;
#133037=CARTESIAN_POINT('Ctrl Pts',(-13.7608857501055,12.4748749581507,
134.040689706046)) ;
#133038=CARTESIAN_POINT('Ctrl Pts',(-13.8461189502053,12.6498955190515,
134.256626571108)) ;
#133039=CARTESIAN_POINT('Ctrl Pts',(-13.9137641762851,12.8801431332148,
134.421162047123)) ;
#133040=CARTESIAN_POINT('Ctrl Pts',(-13.959688118663,13.1504415297617,134.52210348875)) ;
#133041=CARTESIAN_POINT('Ctrl Pts',(-13.9810355826832,13.438739202615,134.551438413197)) ;
#133042=CARTESIAN_POINT('Ctrl Pts',(-13.9771509252308,13.7280473502378,
134.50680820225)) ;
#133043=CARTESIAN_POINT('Ctrl Pts',(-13.9490883356948,13.9932362064335,
134.391820118097)) ;
#133044=CARTESIAN_POINT('Ctrl Pts',(-13.899552383743,14.2186783745982,134.213988401194)) ;
#133045=CARTESIAN_POINT('Ctrl Pts',(-13.8326088799132,14.3872014330787,
133.985246691092)) ;
#133046=CARTESIAN_POINT('Ctrl Pts',(-13.754354251272,14.486216521528,133.723625961275)) ;
#133047=CARTESIAN_POINT('Ctrl Pts',(-13.6703274653614,14.5095010567365,
133.444968044136)) ;
#133048=CARTESIAN_POINT('Ctrl Pts',(-13.587915515568,14.4548476689191,133.171125957688)) ;
#133049=CARTESIAN_POINT('Ctrl Pts',(-13.5132496102258,14.3259646517619,
132.919798090487)) ;
#133050=CARTESIAN_POINT('Ctrl Pts',(-13.4528381497739,14.1320240566172,
132.710133322283)) ;
#133051=CARTESIAN_POINT('Ctrl Pts',(-13.4117984923924,13.8890687487633,
132.557286539592)) ;
#133052=CARTESIAN_POINT('Ctrl Pts',(-13.3933038950219,13.6109288487181,
132.470050146704)) ;
#133053=CARTESIAN_POINT('Ctrl Pts',(-13.3996927101153,13.3205780973656,
132.455665139994)) ;
#133054=CARTESIAN_POINT('Ctrl Pts',(-13.4314451231204,13.0356410236252,
132.515132416829)) ;
#133055=CARTESIAN_POINT('Ctrl Pts',(-13.4863521726588,12.7811568557338,
132.642583088239)) ;
#133056=CARTESIAN_POINT('Ctrl Pts',(-13.5618719439237,12.5709851276515,
132.830045482527)) ;
#133057=CARTESIAN_POINT('Ctrl Pts',(-13.6530001533805,12.4221766619671,
133.063156221214)) ;
#133058=CARTESIAN_POINT('Ctrl Pts',(-13.7543438242653,12.3447406812541,
133.325997758698)) ;
#133059=CARTESIAN_POINT('Ctrl Pts',(-13.858979447707,12.3451621602759,133.598484050117)) ;
#133060=CARTESIAN_POINT('Ctrl Pts',(-13.9595871058779,12.4221617733591,
133.859413033911)) ;
#133061=CARTESIAN_POINT('Ctrl Pts',(-14.0509368702114,12.5713293574021,
134.093085140404)) ;
#133062=CARTESIAN_POINT('Ctrl Pts',(-14.1263288360547,12.7811357471148,
134.280239363245)) ;
#133063=CARTESIAN_POINT('Ctrl Pts',(-14.181464730297,13.037385413305,134.408146154191)) ;
#133064=CARTESIAN_POINT('Ctrl Pts',(-14.2129289597319,13.3202247802994,
134.46702998844)) ;
#133065=CARTESIAN_POINT('Ctrl Pts',(-14.2193168783918,13.6126649497902,
134.452393596522)) ;
#133066=CARTESIAN_POINT('Ctrl Pts',(-14.2008364796894,13.889109539137,134.365400616144)) ;
#133067=CARTESIAN_POINT('Ctrl Pts',(-14.1595000662705,14.1334576219234,
134.211477497111)) ;
#133068=CARTESIAN_POINT('Ctrl Pts',(-14.0992466494206,14.3262010857029,
134.002423062281)) ;
#133069=CARTESIAN_POINT('Ctrl Pts',(-14.0244678789738,14.4552702241494,
133.750713932904)) ;
#133070=CARTESIAN_POINT('Ctrl Pts',(-13.9418997721999,14.5094659873619,
133.476364746001)) ;
#133071=CARTESIAN_POINT('Ctrl Pts',(-13.8583861168424,14.48627928254,133.199410244325)) ;
#133072=CARTESIAN_POINT('Ctrl Pts',(-13.7797353567973,14.3867194330965,
132.936459435104)) ;
#133073=CARTESIAN_POINT('Ctrl Pts',(-13.7130105219871,14.2183273389604,
132.708437979387)) ;
#133074=CARTESIAN_POINT('Ctrl Pts',(-13.6633479068396,13.9922441011096,
132.530147180322)) ;
#133075=CARTESIAN_POINT('Ctrl Pts',(-13.6354328184579,13.7260908863955,
132.415503205816)) ;
#133076=CARTESIAN_POINT('Ctrl Pts',(-13.6315996421401,13.4392990683917,
132.371317925094)) ;
#133077=CARTESIAN_POINT('Ctrl Pts',(-13.6531002743803,13.1491383926391,
132.400878674979)) ;
#133078=CARTESIAN_POINT('Ctrl Pts',(-13.6988895423874,12.880138144259,132.501583429181)) ;
#133079=CARTESIAN_POINT('Ctrl Pts',(-13.7669016038619,12.6488312040692,
132.66702117208)) ;
#133080=CARTESIAN_POINT('Ctrl Pts',(-13.8519661020191,12.4746173052797,
132.882564533349)) ;
#133081=CARTESIAN_POINT('Ctrl Pts',(-13.9499918537797,12.3669410581914,
133.13572242046)) ;
#133082=CARTESIAN_POINT('Ctrl Pts',(-14.0540803057466,12.3355244467329,
133.406613758036)) ;
#133083=CARTESIAN_POINT('Ctrl Pts',(-14.1570770496498,12.3818824637266,
133.674448586604)) ;
#133084=CARTESIAN_POINT('Ctrl Pts',(-14.2529156063067,12.502442440452,133.921340780179)) ;
#133085=CARTESIAN_POINT('Ctrl Pts',(-14.3357164299663,12.6900860359651,
134.129966525958)) ;
#133086=CARTESIAN_POINT('Ctrl Pts',(-14.3993556473891,12.9290693621117,
134.282824648329)) ;
#133087=CARTESIAN_POINT('Ctrl Pts',(-14.4406746427025,13.2033802627449,
134.370454904131)) ;
#133088=CARTESIAN_POINT('Ctrl Pts',(-14.4573570221151,13.493885424346,134.386064394722)) ;
#133089=CARTESIAN_POINT('Ctrl Pts',(-14.4487939272164,13.7798208359641,
134.327863613174)) ;
#133090=CARTESIAN_POINT('Ctrl Pts',(-14.4163591296665,14.0398147256928,
134.199973199807)) ;
#133091=CARTESIAN_POINT('Ctrl Pts',(-14.3630430477874,14.2555980954836,
134.011057985321)) ;
#133092=CARTESIAN_POINT('Ctrl Pts',(-14.2938516112464,14.4112165057251,
133.775932908363)) ;
#133093=CARTESIAN_POINT('Ctrl Pts',(-14.213327419341,14.4969135755094,133.50736843725)) ;
#133094=CARTESIAN_POINT('Ctrl Pts',(-14.1296189321524,14.5049696810031,
133.229876903082)) ;
#133095=CARTESIAN_POINT('Ctrl Pts',(-14.0481698596881,14.4360249735447,
132.958821806314)) ;
#133096=CARTESIAN_POINT('Ctrl Pts',(-13.9759487851369,14.2945754362065,
132.714746600477)) ;
#133097=CARTESIAN_POINT('Ctrl Pts',(-13.9186392005941,14.0897548858671,
132.514089317548)) ;
#133098=CARTESIAN_POINT('Ctrl Pts',(-13.8816283734556,13.8387001375239,
132.372961040856)) ;
#133099=CARTESIAN_POINT('Ctrl Pts',(-13.86765973633,13.5574044598577,132.299056743724)) ;
#133100=CARTESIAN_POINT('Ctrl Pts',(-13.8789956043886,13.2644130009093,
132.2988381339)) ;
#133101=CARTESIAN_POINT('Ctrl Pts',(-13.9149994984909,12.9862195730077,
132.371090109727)) ;
#133102=CARTESIAN_POINT('Ctrl Pts',(-13.9743502243685,12.7371111819008,
132.511275565875)) ;
#133103=CARTESIAN_POINT('Ctrl Pts',(-14.0530557762854,12.5380203242925,
132.708138925323)) ;
#133104=CARTESIAN_POINT('Ctrl Pts',(-14.1469276806553,12.4015272632005,
132.949117652525)) ;
#133105=CARTESIAN_POINT('Ctrl Pts',(-14.2489833656644,12.3389470103484,
133.214189844898)) ;
#133106=CARTESIAN_POINT('Ctrl Pts',(-14.3533226131928,12.3537864997403,
133.485861761893)) ;
#133107=CARTESIAN_POINT('Ctrl Pts',(-14.4528614890508,12.4449099176858,
133.743576395913)) ;
#133108=CARTESIAN_POINT('Ctrl Pts',(-14.5418561425685,12.6072327563546,
133.97027761533)) ;
#133109=CARTESIAN_POINT('Ctrl Pts',(-14.6133813155202,12.8259751420657,
134.146289595912)) ;
#133110=CARTESIAN_POINT('Ctrl Pts',(-14.6644626717837,13.0894865209779,
134.262268329824)) ;
#133111=CARTESIAN_POINT('Ctrl Pts',(-14.6912354788188,13.3763086244584,
134.307339213758)) ;
#133112=CARTESIAN_POINT('Ctrl Pts',(-14.6927780845657,13.666102426872,134.278737035569)) ;
#133113=CARTESIAN_POINT('Ctrl Pts',(-14.6699098049705,13.9378774393092,
134.178922193569)) ;
#133114=CARTESIAN_POINT('Ctrl Pts',(-14.6244200591529,14.174793298913,134.012730262355)) ;
#133115=CARTESIAN_POINT('Ctrl Pts',(-14.5612019536203,14.355667987911,133.795095051057)) ;
#133116=CARTESIAN_POINT('Ctrl Pts',(-14.4846906294762,14.4711053294092,
133.538428577137)) ;
#133117=CARTESIAN_POINT('Ctrl Pts',(-14.4011850462511,14.511170979715,133.261273870169)) ;
#133118=CARTESIAN_POINT('Ctrl Pts',(-14.3178410780268,14.4729025341711,
132.984673903261)) ;
#133119=CARTESIAN_POINT('Ctrl Pts',(-14.2414431710577,14.3605014183323,
132.728538157581)) ;
#133120=CARTESIAN_POINT('Ctrl Pts',(-14.1770966200207,14.1789799497678,
132.507210107387)) ;
#133121=CARTESIAN_POINT('Ctrl Pts',(-14.1315848885081,13.9453130755044,
132.341277366815)) ;
#133122=CARTESIAN_POINT('Ctrl Pts',(-14.1079390036142,13.673613297581,132.239086339493)) ;
#133123=CARTESIAN_POINT('Ctrl Pts',(-14.1087830481224,13.3843416477693,
132.208491884339)) ;
#133124=CARTESIAN_POINT('Ctrl Pts',(-14.1351400941846,13.0956424787648,
132.252157038047)) ;
#133125=CARTESIAN_POINT('Ctrl Pts',(-14.1851403795369,12.8335787485534,
132.365283706234)) ;
#133126=CARTESIAN_POINT('Ctrl Pts',(-14.2566883427613,12.6116522531053,
132.541092961402)) ;
#133127=CARTESIAN_POINT('Ctrl Pts',(-14.3449178102994,12.4486058050818,
132.765728820733)) ;
#133128=CARTESIAN_POINT('Ctrl Pts',(-14.4444094609299,12.3551665981467,
133.023238128206)) ;
#133129=CARTESIAN_POINT('Ctrl Pts',(-14.5487260750023,12.3383111368361,
133.294844327139)) ;
#133130=CARTESIAN_POINT('Ctrl Pts',(-14.651135777708,12.3991318667188,133.560878201396)) ;
#133131=CARTESIAN_POINT('Ctrl Pts',(-14.7450247980916,12.5336133546432,
133.801997324254)) ;
#133132=CARTESIAN_POINT('Ctrl Pts',(-14.8240658891889,12.7304747525644,
133.999922781035)) ;
#133133=CARTESIAN_POINT('Ctrl Pts',(-14.8843591623108,12.9801493565206,
134.142645016146)) ;
#133134=CARTESIAN_POINT('Ctrl Pts',(-14.9207776314118,13.2569930870622,
134.216214669517)) ;
#133135=CARTESIAN_POINT('Ctrl Pts',(-14.9327904526555,13.5493201067258,
134.218039568247)) ;
#133136=CARTESIAN_POINT('Ctrl Pts',(-14.9195608823309,13.8310609228274,
134.146315593606)) ;
#133137=CARTESIAN_POINT('Ctrl Pts',(-14.8829071658904,14.0843638099265,
134.006060198745)) ;
#133138=CARTESIAN_POINT('Ctrl Pts',(-14.8262774665716,14.2896244491401,
133.807537482938)) ;
#133139=CARTESIAN_POINT('Ctrl Pts',(-14.7544509561564,14.4330063116879,
133.564623744753)) ;
#133140=CARTESIAN_POINT('Ctrl Pts',(-14.6730981695364,14.5042107415309,
133.293824015626)) ;
#133141=CARTESIAN_POINT('Ctrl Pts',(-14.5890044461905,14.4979449999679,
133.015056574469)) ;
#133142=CARTESIAN_POINT('Ctrl Pts',(-14.5085811345525,14.4144601779744,
132.746912885546)) ;
#133143=CARTESIAN_POINT('Ctrl Pts',(-14.4386966820867,14.2595209902124,
132.509575163383)) ;
#133144=CARTESIAN_POINT('Ctrl Pts',(-14.3852681727933,14.046214919979,132.32053362023)) ;
#133145=CARTESIAN_POINT('Ctrl Pts',(-14.3521879692475,13.7868053449528,
132.190703349274)) ;
#133146=CARTESIAN_POINT('Ctrl Pts',(-14.3429850788203,13.5027357390144,
132.130803960272)) ;
#133147=CARTESIAN_POINT('Ctrl Pts',(-14.3589256787532,13.2114164567146,
132.144166678592)) ;
#133148=CARTESIAN_POINT('Ctrl Pts',(-14.3996479591576,12.9359342983456,
132.230005501464)) ;
#133149=CARTESIAN_POINT('Ctrl Pts',(-14.4630310316759,12.6951562018299,
132.381999972268)) ;
#133150=CARTESIAN_POINT('Ctrl Pts',(-14.5447779273386,12.5073061272103,
132.587797294127)) ;
#133151=CARTESIAN_POINT('Ctrl Pts',(-14.6405874915994,12.3841592686752,
132.834495044115)) ;
#133152=CARTESIAN_POINT('Ctrl Pts',(-14.7436396651289,12.3356200239572,
133.102447533053)) ;
#133153=CARTESIAN_POINT('Ctrl Pts',(-14.8482334000072,12.3655842279676,
133.374661826652)) ;
#133154=CARTESIAN_POINT('Ctrl Pts',(-14.9456378863924,12.4702048591763,
133.62631542447)) ;
#133155=CARTESIAN_POINT('Ctrl Pts',(-15.032031341998,12.6448837976238,133.845354670619)) ;
#133156=CARTESIAN_POINT('Ctrl Pts',(-15.0997909854076,12.872508423284,134.010430965611)) ;
#133157=CARTESIAN_POINT('Ctrl Pts',(-15.1466624677231,13.1434988331289,
134.11394299587)) ;
#133158=CARTESIAN_POINT('Ctrl Pts',(-15.1684830221252,13.4301737780494,
134.144821454034)) ;
#133159=CARTESIAN_POINT('Ctrl Pts',(-15.1655029363779,13.7187795914099,
134.102960274335)) ;
#133160=CARTESIAN_POINT('Ctrl Pts',(-15.137871807278,13.9870154433738,133.988964277523)) ;
#133161=CARTESIAN_POINT('Ctrl Pts',(-15.089103500937,14.2124398345738,133.813561355081)) ;
#133162=CARTESIAN_POINT('Ctrl Pts',(-15.0226861816082,14.3830654461858,
133.586365342099)) ;
#133163=CARTESIAN_POINT('Ctrl Pts',(-14.9442977084689,14.4846609541733,
133.324197217531)) ;
#133164=CARTESIAN_POINT('Ctrl Pts',(-14.8603045751173,14.5097913616969,
133.045629352813)) ;
#133165=CARTESIAN_POINT('Ctrl Pts',(-14.7781158124174,14.4576093080194,
132.772584210679)) ;
#133166=CARTESIAN_POINT('Ctrl Pts',(-14.7029379087114,14.3304831317374,
132.519675058584)) ;
#133167=CARTESIAN_POINT('Ctrl Pts',(-14.6421746060609,14.1386183822934,
132.309056084948)) ;
#133168=CARTESIAN_POINT('Ctrl Pts',(-14.6004669656827,13.8965846856625,
132.154209706835)) ;
#133169=CARTESIAN_POINT('Ctrl Pts',(-14.5812880337956,13.6198365630073,
132.065057969682)) ;
#133170=CARTESIAN_POINT('Ctrl Pts',(-14.5869544254102,13.3288844737818,
132.048478781958)) ;
#133171=CARTESIAN_POINT('Ctrl Pts',(-14.6178077703533,13.0447399832046,
132.105475686592)) ;
#133172=CARTESIAN_POINT('Ctrl Pts',(-14.6721136258845,12.7881836368688,
132.231068090543)) ;
#133173=CARTESIAN_POINT('Ctrl Pts',(-14.7475386699193,12.5755910115287,
132.418091523374)) ;
#133174=CARTESIAN_POINT('Ctrl Pts',(-14.8378940236856,12.4257574465567,
132.649102005788)) ;
#133175=CARTESIAN_POINT('Ctrl Pts',(-14.9388209084364,12.3460112405744,
132.910787274949)) ;
#133176=CARTESIAN_POINT('Ctrl Pts',(-15.0435737078647,12.3439532504127,
133.183578235088)) ;
#133177=CARTESIAN_POINT('Ctrl Pts',(-15.1446091167616,12.4188218900739,
133.445686307793)) ;
#133178=CARTESIAN_POINT('Ctrl Pts',(-15.2365998734713,12.5668341062151,
133.681113263233)) ;
#133179=CARTESIAN_POINT('Ctrl Pts',(-15.3120455807105,12.7739565310488,
133.868616342754)) ;
#133180=CARTESIAN_POINT('Ctrl Pts',(-15.3679671650309,13.0292275295923,
133.998784482597)) ;
#133181=CARTESIAN_POINT('Ctrl Pts',(-15.4001513908772,13.3121167714202,
134.059708256056)) ;
#133182=CARTESIAN_POINT('Ctrl Pts',(-15.407302294284,13.6036711588795,134.047415072482)) ;
#133183=CARTESIAN_POINT('Ctrl Pts',(-15.3894117903854,13.8822010088686,
133.961971555951)) ;
#133184=CARTESIAN_POINT('Ctrl Pts',(-15.3488581880954,14.126534024312,133.810499271449)) ;
#133185=CARTESIAN_POINT('Ctrl Pts',(-15.2890058404676,14.3215277156221,
133.602541497692)) ;
#133186=CARTESIAN_POINT('Ctrl Pts',(-15.2146261037101,14.4523872469144,
133.352036701433)) ;
#133187=CARTESIAN_POINT('Ctrl Pts',(-15.132276398967,14.509081269933,133.078352393805)) ;
#133188=CARTESIAN_POINT('Ctrl Pts',(-15.048156334803,14.4877530584647,132.799404216537)) ;
#133189=CARTESIAN_POINT('Ctrl Pts',(-14.9697741972722,14.3906972492053,
132.537447195776)) ;
#133190=CARTESIAN_POINT('Ctrl Pts',(-14.9025432118204,14.2242127265294,
132.307919886886)) ;
#133191=CARTESIAN_POINT('Ctrl Pts',(-14.8524134830202,14.0000453961231,
132.128331876439)) ;
#133192=CARTESIAN_POINT('Ctrl Pts',(-14.8236827135926,13.7349941187306,
132.011308130338)) ;
#133193=CARTESIAN_POINT('Ctrl Pts',(-14.8192110157222,13.4462938086935,
131.964998461715)) ;
#133194=CARTESIAN_POINT('Ctrl Pts',(-14.8397608257614,13.1586524064852,
131.992109164985)) ;
#133195=CARTESIAN_POINT('Ctrl Pts',(-14.8852506544382,12.8863235925418,
132.091631205511)) ;
#133196=CARTESIAN_POINT('Ctrl Pts',(-14.952306886852,12.6553854575325,132.254505839022)) ;
#133197=CARTESIAN_POINT('Ctrl Pts',(-15.036993538522,12.4787538591612,132.468885463633)) ;
#133198=CARTESIAN_POINT('Ctrl Pts',(-15.1351325127102,12.3688114822916,
132.722256615459)) ;
#133199=CARTESIAN_POINT('Ctrl Pts',(-15.2387002100067,12.3354319136936,
132.991765834986)) ;
#133200=CARTESIAN_POINT('Ctrl Pts',(-15.3419020299315,12.3792576310417,
133.260178529464)) ;
#133201=CARTESIAN_POINT('Ctrl Pts',(-15.4385746866519,12.4988398999205,
133.509304414363)) ;
#133202=CARTESIAN_POINT('Ctrl Pts',(-15.5211785051019,12.6835118512005,
133.71760539492)) ;
#133203=CARTESIAN_POINT('Ctrl Pts',(-15.585614912484,12.9214923912795,133.872725040323)) ;
#133204=CARTESIAN_POINT('Ctrl Pts',(-15.6276593796861,13.1954916424955,
133.96242929729)) ;
#133205=CARTESIAN_POINT('Ctrl Pts',(-15.6450448286836,13.4865485670219,
133.980012149667)) ;
#133206=CARTESIAN_POINT('Ctrl Pts',(-15.6370948847114,13.772471589557,133.923647448758)) ;
#133207=CARTESIAN_POINT('Ctrl Pts',(-15.6054576941134,14.0322259092952,
133.798239163953)) ;
#133208=CARTESIAN_POINT('Ctrl Pts',(-15.5528532090993,14.2496185339524,
133.611440842472)) ;
#133209=CARTESIAN_POINT('Ctrl Pts',(-15.483617346609,14.4079186586772,133.375986031408)) ;
#133210=CARTESIAN_POINT('Ctrl Pts',(-15.4040148005417,14.495128940057,133.110405781656)) ;
#133211=CARTESIAN_POINT('Ctrl Pts',(-15.3198980850125,14.5060206783235,
132.831544484233)) ;
#133212=CARTESIAN_POINT('Ctrl Pts',(-15.2380342056834,14.4388851972431,
132.55918054693)) ;
#133213=CARTESIAN_POINT('Ctrl Pts',(-15.1654389797841,14.2990479598781,
132.313981427395)) ;
#133214=CARTESIAN_POINT('Ctrl Pts',(-15.107816605712,14.096277092635,132.112499036057)) ;
#133215=CARTESIAN_POINT('Ctrl Pts',(-15.0701124492741,13.8463552274942,
131.969338122834)) ;
#133216=CARTESIAN_POINT('Ctrl Pts',(-15.05554407707,13.5643762793268,131.893541407323)) ;
#133217=CARTESIAN_POINT('Ctrl Pts',(-15.0659585050918,13.2747380866486,
131.891020251149)) ;
#133218=CARTESIAN_POINT('Ctrl Pts',(-15.101446630055,12.9934296976024,131.961474427387)) ;
#133219=CARTESIAN_POINT('Ctrl Pts',(-15.1601039100246,12.7438068041656,
132.099715492444)) ;
#133220=CARTESIAN_POINT('Ctrl Pts',(-15.2384724882155,12.5426943442427,
132.295520501906)) ;
#133221=CARTESIAN_POINT('Ctrl Pts',(-15.3316626347415,12.4046936236787,
132.534630966333)) ;
#133222=CARTESIAN_POINT('Ctrl Pts',(-15.4337983976848,12.3396331759052,
132.799852893319)) ;
#133223=CARTESIAN_POINT('Ctrl Pts',(-15.5380451833256,12.3522550875064,
133.071297592341)) ;
#133224=CARTESIAN_POINT('Ctrl Pts',(-15.6378149553019,12.441158614988,133.329684714748)) ;
#133225=CARTESIAN_POINT('Ctrl Pts',(-15.7271824288003,12.6013769713038,
133.55749869446)) ;
#133226=CARTESIAN_POINT('Ctrl Pts',(-15.799387164279,12.819071640269,133.735430014399)) ;
#133227=CARTESIAN_POINT('Ctrl Pts',(-15.8509954325536,13.0807346140254,
133.853055281245)) ;
#133228=CARTESIAN_POINT('Ctrl Pts',(-15.8785701981475,13.3675408612144,
133.900413861765)) ;
#133229=CARTESIAN_POINT('Ctrl Pts',(-15.880950069095,13.6570979280699,133.874320504545)) ;
#133230=CARTESIAN_POINT('Ctrl Pts',(-15.8584614917164,13.9319893911641,
133.775308859387)) ;
#133231=CARTESIAN_POINT('Ctrl Pts',(-15.8140300794619,14.1676085258846,
133.612576918087)) ;
#133232=CARTESIAN_POINT('Ctrl Pts',(-15.7508365618172,14.3519029604138,
133.394745430706)) ;
#133233=CARTESIAN_POINT('Ctrl Pts',(-15.6747542377325,14.4687263868581,
133.139424327783)) ;
#133234=CARTESIAN_POINT('Ctrl Pts',(-15.5916310901521,14.5110206744739,
132.86348513324)) ;
#133235=CARTESIAN_POINT('Ctrl Pts',(-15.5082277554707,14.4754839101951,
132.586740900539)) ;
#133236=CARTESIAN_POINT('Ctrl Pts',(-15.4310148106346,14.3641243881349,
132.327975519891)) ;
#133237=CARTESIAN_POINT('Ctrl Pts',(-15.366796148105,14.1859981150162,132.10732571318)) ;
#133238=CARTESIAN_POINT('Ctrl Pts',(-15.3203690301936,13.9527739629267,
131.938549874937)) ;
#133239=CARTESIAN_POINT('Ctrl Pts',(-15.2960642034895,13.6818171869407,
131.83443758756)) ;
#133240=CARTESIAN_POINT('Ctrl Pts',(-15.2962284106988,13.3923456599437,
131.801803057666)) ;
#133241=CARTESIAN_POINT('Ctrl Pts',(-15.3217088635482,13.1044625348289,
131.843052348479)) ;
#133242=CARTESIAN_POINT('Ctrl Pts',(-15.3712895624886,12.8400820200563,
131.954780479996)) ;
#133243=CARTESIAN_POINT('Ctrl Pts',(-15.4421215709794,12.6174283224968,
132.128595071256)) ;
#133244=CARTESIAN_POINT('Ctrl Pts',(-15.5300656767636,12.4521814963559,
132.352341736955)) ;
#133245=CARTESIAN_POINT('Ctrl Pts',(-15.6293654089259,12.3567835155047,
132.609283754024)) ;
#133246=CARTESIAN_POINT('Ctrl Pts',(-15.7333497867975,12.3377092271658,
132.880009523703)) ;
#133247=CARTESIAN_POINT('Ctrl Pts',(-15.8360089773108,12.3962076032604,
133.146742886939)) ;
#133248=CARTESIAN_POINT('Ctrl Pts',(-15.930453723468,12.5290432373042,133.389409066584)) ;
#133249=CARTESIAN_POINT('Ctrl Pts',(-16.009869584066,12.7244085230837,133.588441629327)) ;
#133250=CARTESIAN_POINT('Ctrl Pts',(-16.0704566796156,12.9709500550387,
133.732258312717)) ;
#133251=CARTESIAN_POINT('Ctrl Pts',(-16.1079755146477,13.2494402817627,
133.808760193825)) ;
#133252=CARTESIAN_POINT('Ctrl Pts',(-16.1205567949924,13.5418967084717,
133.812230503726)) ;
#133253=CARTESIAN_POINT('Ctrl Pts',(-16.1080660019669,13.8230883914708,
133.742789063125)) ;
#133254=CARTESIAN_POINT('Ctrl Pts',(-16.0720612901439,14.0775910910953,
133.604421793909)) ;
#133255=CARTESIAN_POINT('Ctrl Pts',(-16.016031312662,14.2842118886259,133.407692540579)) ;
#133256=CARTESIAN_POINT('Ctrl Pts',(-15.9444811188164,14.4299775435325,
133.165534218954)) ;
#133257=CARTESIAN_POINT('Ctrl Pts',(-15.8629277653847,14.503331032243,132.894001914259)) ;
#133258=CARTESIAN_POINT('Ctrl Pts',(-15.7793496289803,14.4992417837061,
132.616952244808)) ;
#133259=CARTESIAN_POINT('Ctrl Pts',(-15.6984734089822,14.4177939822546,
132.347381532007)) ;
#133260=CARTESIAN_POINT('Ctrl Pts',(-15.6283650852396,14.2650806147523,
132.109470216545)) ;
#133261=CARTESIAN_POINT('Ctrl Pts',(-15.5743268050137,14.0529681509037,
131.918590385591)) ;
#133262=CARTESIAN_POINT('Ctrl Pts',(-15.5406403700371,13.7955270319932,
131.787101135372)) ;
#133263=CARTESIAN_POINT('Ctrl Pts',(-15.5306638256876,13.5095709535078,
131.724666349948)) ;
#133264=CARTESIAN_POINT('Ctrl Pts',(-15.5460171831695,13.2189036520177,
131.736403340103)) ;
#133265=CARTESIAN_POINT('Ctrl Pts',(-15.5859137154081,12.9437120966298,
131.819943466577)) ;
#133266=CARTESIAN_POINT('Ctrl Pts',(-15.6485475179313,12.7018113312773,
131.969792071976)) ;
#133267=CARTESIAN_POINT('Ctrl Pts',(-15.7301725881226,12.5115374792667,
132.175093619939)) ;
#133268=CARTESIAN_POINT('Ctrl Pts',(-15.8255194984171,12.3865362509785,
132.420501324227)) ;
#133269=CARTESIAN_POINT('Ctrl Pts',(-15.9289904176059,12.3360647683775,
132.689500393083)) ;
#133270=CARTESIAN_POINT('Ctrl Pts',(-16.0322109432962,12.3630945002041,
132.958176956719)) ;
#133271=CARTESIAN_POINT('Ctrl Pts',(-16.1310535797055,12.4665769548229,
133.213630713827)) ;
#133272=CARTESIAN_POINT('Ctrl Pts',(-16.2171162898203,12.637873730405,133.432016347732)) ;
#133273=CARTESIAN_POINT('Ctrl Pts',(-16.2861070614099,12.8661806742055,
133.600365416687)) ;
#133274=CARTESIAN_POINT('Ctrl Pts',(-16.3331577984964,13.1333277515124,
133.704775971435)) ;
#133275=CARTESIAN_POINT('Ctrl Pts',(-16.3560616077762,13.4221934836715,
133.738517459493)) ;
#133276=CARTESIAN_POINT('Ctrl Pts',(-16.3536937500244,13.7107571318464,
133.698487549138)) ;
#133277=CARTESIAN_POINT('Ctrl Pts',(-16.3267795290435,13.9798563780996,
133.58659147111)) ;
#133278=CARTESIAN_POINT('Ctrl Pts',(-16.2784408821239,14.2070905580459,
133.412375341533)) ;
#133279=CARTESIAN_POINT('Ctrl Pts',(-16.2125397227886,14.3790287482914,
133.186748864503)) ;
#133280=CARTESIAN_POINT('Ctrl Pts',(-16.1346594708171,14.4826462514907,
132.926162382995)) ;
#133281=CARTESIAN_POINT('Ctrl Pts',(-16.0504302213959,14.5101765749395,
132.646782279628)) ;
#133282=CARTESIAN_POINT('Ctrl Pts',(-15.9682674268405,14.4602521093363,
132.373878730922)) ;
#133283=CARTESIAN_POINT('Ctrl Pts',(-15.892694390541,14.3349863303821,132.119771873462)) ;
#133284=CARTESIAN_POINT('Ctrl Pts',(-15.8317129503708,14.1459036519263,
131.908681279387)) ;
#133285=CARTESIAN_POINT('Ctrl Pts',(-15.7891216920241,13.9042674567381,
131.751109063095)) ;
#133286=CARTESIAN_POINT('Ctrl Pts',(-15.7692741641614,13.6274934121279,
131.659929127433)) ;
#133287=CARTESIAN_POINT('Ctrl Pts',(-15.774240842792,13.3375401227482,131.641402457855)) ;
#133288=CARTESIAN_POINT('Ctrl Pts',(-15.8042482653973,13.0529656397982,
131.695949415826)) ;
#133289=CARTESIAN_POINT('Ctrl Pts',(-15.8584516986935,12.793542004979,131.820979830249)) ;
#133290=CARTESIAN_POINT('Ctrl Pts',(-15.9326864597706,12.5815361452067,
132.004842248444)) ;
#133291=CARTESIAN_POINT('Ctrl Pts',(-16.0230837910625,12.4287258471182,
132.235797836759)) ;
#133292=CARTESIAN_POINT('Ctrl Pts',(-16.1240643432101,12.3470719994747,
132.497574210549)) ;
#133293=CARTESIAN_POINT('Ctrl Pts',(-16.2285925774014,12.3430683223392,
132.769776197563)) ;
#133294=CARTESIAN_POINT('Ctrl Pts',(-16.3294552263757,12.4155936091128,
133.031491197843)) ;
#133295=CARTESIAN_POINT('Ctrl Pts',(-16.42158697565,12.5608875783812,133.267432939441)) ;
#133296=CARTESIAN_POINT('Ctrl Pts',(-16.4979791687381,12.7672957855937,
133.457539227448)) ;
#133297=CARTESIAN_POINT('Ctrl Pts',(-16.5545469684218,13.0219896288371,
133.589546147221)) ;
#133298=CARTESIAN_POINT('Ctrl Pts',(-16.5873216769804,13.3035436342973,
133.652289558074)) ;
#133299=CARTESIAN_POINT('Ctrl Pts',(-16.5952372158022,13.5948422510341,
133.642264450776)) ;
#133300=CARTESIAN_POINT('Ctrl Pts',(-16.5781262828345,13.8739529691167,
133.559117325056)) ;
#133301=CARTESIAN_POINT('Ctrl Pts',(-16.5380768677347,14.1203174233417,
133.409012301568)) ;
#133302=CARTESIAN_POINT('Ctrl Pts',(-16.4787184094645,14.3167168643634,
133.20251930448)) ;
#133303=CARTESIAN_POINT('Ctrl Pts',(-16.4048795075091,14.4494066861711,
132.953678390524)) ;
#133304=CARTESIAN_POINT('Ctrl Pts',(-16.3225697948458,14.5084702688582,
132.680063070833)) ;
#133305=CARTESIAN_POINT('Ctrl Pts',(-16.2386731326133,14.489700746972,132.401879914645)) ;
#133306=CARTESIAN_POINT('Ctrl Pts',(-16.159666302226,14.3946106074975,132.13794942029)) ;
#133307=CARTESIAN_POINT('Ctrl Pts',(-16.0919372674924,14.2294635345246,
131.906906848158)) ;
#133308=CARTESIAN_POINT('Ctrl Pts',(-16.0414142644033,14.0073333887475,
131.726263966149)) ;
#133309=CARTESIAN_POINT('Ctrl Pts',(-16.0120005571222,13.7435828448799,
131.607279354952)) ;
#133310=CARTESIAN_POINT('Ctrl Pts',(-16.0067413555039,13.454824745877,131.558621231445)) ;
#133311=CARTESIAN_POINT('Ctrl Pts',(-16.0266816029947,13.1663898496403,
131.58388276017)) ;
#133312=CARTESIAN_POINT('Ctrl Pts',(-16.071174096646,12.8948251888563,131.680693404511)) ;
#133313=CARTESIAN_POINT('Ctrl Pts',(-16.1378143759152,12.6613614393991,
131.842219614895)) ;
#133314=CARTESIAN_POINT('Ctrl Pts',(-16.2222899580583,12.4827884864443,
132.055914031115)) ;
#133315=CARTESIAN_POINT('Ctrl Pts',(-16.3195947643377,12.3713198999723,
132.307032186213)) ;
#133316=CARTESIAN_POINT('Ctrl Pts',(-16.42316155049,12.3351536539427,132.576506572357)) ;
#133317=CARTESIAN_POINT('Ctrl Pts',(-16.5269587087536,12.3771106003778,
132.846499102918)) ;
#133318=CARTESIAN_POINT('Ctrl Pts',(-16.6232634802675,12.493746042562,133.094781650953)) ;
#133319=CARTESIAN_POINT('Ctrl Pts',(-16.7066715515362,12.6767291405437,
133.30534152523)) ;
#133320=CARTESIAN_POINT('Ctrl Pts',(-16.7719969184263,12.9147362953278,
133.462888792416)) ;
#133321=CARTESIAN_POINT('Ctrl Pts',(-16.8145117924752,13.1870897175325,
133.554081812245)) ;
#133322=CARTESIAN_POINT('Ctrl Pts',(-16.832664410647,13.4771402294594,133.573993886311)) ;
#133323=CARTESIAN_POINT('Ctrl Pts',(-16.8255195547471,13.7642376991577,
133.519905575425)) ;
#133324=CARTESIAN_POINT('Ctrl Pts',(-16.7943070458963,14.0261140050281,
133.395578546783)) ;
#133325=CARTESIAN_POINT('Ctrl Pts',(-16.7424882598997,14.2437566095146,
133.211251228587)) ;
#133326=CARTESIAN_POINT('Ctrl Pts',(-16.6736113908412,14.4043004510961,
132.976804095223)) ;
#133327=CARTESIAN_POINT('Ctrl Pts',(-16.5942186823598,14.4936451763547,
132.711836822872)) ;
#133328=CARTESIAN_POINT('Ctrl Pts',(-16.5101466580755,14.5067755223083,
132.433108081231)) ;
#133329=CARTESIAN_POINT('Ctrl Pts',(-16.4282410882398,14.4421251633059,
132.160681842967)) ;
#133330=CARTESIAN_POINT('Ctrl Pts',(-16.3551632521983,14.3039891726026,
131.914003956164)) ;
#133331=CARTESIAN_POINT('Ctrl Pts',(-16.2972497108617,14.1040922169467,
131.711842779145)) ;
#133332=CARTESIAN_POINT('Ctrl Pts',(-16.2585983326173,13.8535852347893,
131.565668552377)) ;
#133333=CARTESIAN_POINT('Ctrl Pts',(-16.243420453165,13.5730952435811,131.488208101679)) ;
#133334=CARTESIAN_POINT('Ctrl Pts',(-16.2531006198612,13.2829861782011,
131.483481649537)) ;
#133335=CARTESIAN_POINT('Ctrl Pts',(-16.2877661805878,13.0017737284941,
131.551621835108)) ;
#133336=CARTESIAN_POINT('Ctrl Pts',(-16.3459738367156,12.7500890797144,
131.688431825914)) ;
#133337=CARTESIAN_POINT('Ctrl Pts',(-16.4238184818004,12.5475577998432,
131.882729415997)) ;
#133338=CARTESIAN_POINT('Ctrl Pts',(-16.5167586194788,12.4075652478031,
132.121078295711)) ;
#133339=CARTESIAN_POINT('Ctrl Pts',(-16.6183907518262,12.3405227377109,
132.384938789592)) ;
#133340=CARTESIAN_POINT('Ctrl Pts',(-16.7229364475564,12.3506975715296,
132.657173213167)) ;
#133341=CARTESIAN_POINT('Ctrl Pts',(-16.8232859030364,12.438177489278,132.917122022405)) ;
#133342=CARTESIAN_POINT('Ctrl Pts',(-16.9125712124386,12.5958827964123,
133.1448620791)) ;
#133343=CARTESIAN_POINT('Ctrl Pts',(-16.9854582743437,12.8123887822574,
133.324729525533)) ;
#133344=CARTESIAN_POINT('Ctrl Pts',(-17.037709893631,13.0732934241726,133.444215844693)) ;
#133345=CARTESIAN_POINT('Ctrl Pts',(-17.0659638164382,13.3601444544887,
133.493509177191)) ;
#133346=CARTESIAN_POINT('Ctrl Pts',(-17.0689675284249,13.6487324697402,
133.469363185352)) ;
#133347=CARTESIAN_POINT('Ctrl Pts',(-17.0474035047278,13.9231969052117,
133.37321432911)) ;
#133348=CARTESIAN_POINT('Ctrl Pts',(-17.0033733673897,14.1616648845749,
133.211459633651)) ;
#133349=CARTESIAN_POINT('Ctrl Pts',(-16.9406158991401,14.3474885130478,
132.994912465869)) ;
#133350=CARTESIAN_POINT('Ctrl Pts',(-16.864876505793,14.4664584587802,132.740606759249)) ;
#133351=CARTESIAN_POINT('Ctrl Pts',(-16.7814776117931,14.5109046603937,
132.463712586271)) ;
#133352=CARTESIAN_POINT('Ctrl Pts',(-16.6983907346783,14.477538406395,132.188050973166)) ;
#133353=CARTESIAN_POINT('Ctrl Pts',(-16.6207705482251,14.3681997132881,
131.928042842248)) ;
#133354=CARTESIAN_POINT('Ctrl Pts',(-16.5561356079281,14.19161807787,131.706168442298)) ;
#133355=CARTESIAN_POINT('Ctrl Pts',(-16.5092308734292,13.9603524956053,
131.536079167786)) ;
#133356=CARTESIAN_POINT('Ctrl Pts',(-16.4841796106604,13.6895220911817,
131.429699941359)) ;
#133357=CARTESIAN_POINT('Ctrl Pts',(-16.4836919093705,13.4007319641459,
131.395211960917)) ;
#133358=CARTESIAN_POINT('Ctrl Pts',(-16.5082964988508,13.1132078283894,
131.433992211526)) ;
#133359=CARTESIAN_POINT('Ctrl Pts',(-16.5574784700436,12.8466068578935,
131.544388229293)) ;
#133360=CARTESIAN_POINT('Ctrl Pts',(-16.6273997075169,12.6236984730367,
131.715716955648)) ;
#133361=CARTESIAN_POINT('Ctrl Pts',(-16.7150468521775,12.4561011970055,
131.938529922164)) ;
#133362=CARTESIAN_POINT('Ctrl Pts',(-16.8139682824648,12.3585968124196,
132.194412407875)) ;
#133363=CARTESIAN_POINT('Ctrl Pts',(-16.9182265147246,12.3371246735504,
132.465833558649)) ;
#133364=CARTESIAN_POINT('Ctrl Pts',(-17.0209026074425,12.3935413485491,
132.732653318412)) ;
#133365=CARTESIAN_POINT('Ctrl Pts',(-17.1153756443262,12.5236723848828,
132.975519307564)) ;
#133366=CARTESIAN_POINT('Ctrl Pts',(-17.1956555914022,12.7179304240541,
133.176947444366)) ;
#133367=CARTESIAN_POINT('Ctrl Pts',(-17.2569924030211,12.9643000603806,
133.322838842009)) ;
#133368=CARTESIAN_POINT('Ctrl Pts',(-17.2949538933717,13.2410161239663,
133.400773057716)) ;
#133369=CARTESIAN_POINT('Ctrl Pts',(-17.3083412632257,13.5320326358814,
133.40675253041)) ;
#133370=CARTESIAN_POINT('Ctrl Pts',(-17.2965889183178,13.8151976332958,
133.339306952295)) ;
#133371=CARTESIAN_POINT('Ctrl Pts',(-17.2611712342104,14.070965110173,133.202631251777)) ;
#133372=CARTESIAN_POINT('Ctrl Pts',(-17.2055219190199,14.2795161854134,
133.006946181317)) ;
#133373=CARTESIAN_POINT('Ctrl Pts',(-17.1344526197165,14.4266233568165,
132.766264881813)) ;
#133374=CARTESIAN_POINT('Ctrl Pts',(-17.0535835623515,14.5021444966585,
132.496922447555)) ;
#133375=CARTESIAN_POINT('Ctrl Pts',(-16.9693534559784,14.5004799279669,
132.217713549754)) ;
#133376=CARTESIAN_POINT('Ctrl Pts',(-16.8885085804287,14.4210758361391,
131.948320350664)) ;
#133377=CARTESIAN_POINT('Ctrl Pts',(-16.818249196986,14.2711637356508,131.710095463003)) ;
#133378=CARTESIAN_POINT('Ctrl Pts',(-16.7633840110066,14.0600320259714,
131.516677712646)) ;
#133379=CARTESIAN_POINT('Ctrl Pts',(-16.729034656478,13.8025046463563,131.383125760343)) ;
#133380=CARTESIAN_POINT('Ctrl Pts',(-16.7184105236858,13.5194350300881,
131.319077858953)) ;
#133381=CARTESIAN_POINT('Ctrl Pts',(-16.7329082611137,13.227929848522,131.328230796269)) ;
#133382=CARTESIAN_POINT('Ctrl Pts',(-16.7721540100418,12.9514279979351,
131.409809044102)) ;
#133383=CARTESIAN_POINT('Ctrl Pts',(-16.834426980546,12.7076270254922,131.558495828173)) ;
#133384=CARTESIAN_POINT('Ctrl Pts',(-16.9152315370478,12.5164543914562,
131.761543944961)) ;
#133385=CARTESIAN_POINT('Ctrl Pts',(-17.0104958015721,12.3891143889345,
132.006622580848)) ;
#133386=CARTESIAN_POINT('Ctrl Pts',(-17.1132917121907,12.3364756158918,
132.273826383176)) ;
#133387=CARTESIAN_POINT('Ctrl Pts',(-17.2173332534644,12.3612642231578,
132.54465957405)) ;
#133388=CARTESIAN_POINT('Ctrl Pts',(-17.3163641429157,12.4629838840005,
132.800676032605)) ;
#133389=CARTESIAN_POINT('Ctrl Pts',(-17.4026407183266,12.6321971699934,
133.01975282772)) ;
#133390=CARTESIAN_POINT('Ctrl Pts',(-17.472100457449,12.8584558798932,133.189548524182)) ;
#133391=CARTESIAN_POINT('Ctrl Pts',(-17.5200564206003,13.1261648647243,
133.296424663186)) ;
#133392=CARTESIAN_POINT('Ctrl Pts',(-17.5435329958318,13.4141234552309,
133.331916813786)) ;
#133393=CARTESIAN_POINT('Ctrl Pts',(-17.5418705107985,13.7023852342343,
133.294006470842)) ;
#133394=CARTESIAN_POINT('Ctrl Pts',(-17.515866367185,13.9714212012371,133.184910655295)) ;
#133395=CARTESIAN_POINT('Ctrl Pts',(-17.4677121548387,14.202020081249,133.01095053406)) ;
#133396=CARTESIAN_POINT('Ctrl Pts',(-17.4023716167183,14.3750071736422,
132.787065724901)) ;
#133397=CARTESIAN_POINT('Ctrl Pts',(-17.3247668097447,14.4806351346196,
132.527282453733)) ;
#133398=CARTESIAN_POINT('Ctrl Pts',(-17.2410054869792,14.5105855297535,
132.24943004058)) ;
#133399=CARTESIAN_POINT('Ctrl Pts',(-17.1581501091636,14.4625550657111,
131.974268906069)) ;
#133400=CARTESIAN_POINT('Ctrl Pts',(-17.0827332780509,14.3400369417443,
131.720826863696)) ;
#133401=CARTESIAN_POINT('Ctrl Pts',(-17.0209888868574,14.1521957535254,
131.507380128005)) ;
#133402=CARTESIAN_POINT('Ctrl Pts',(-16.9778207788142,13.9116489154345,
131.348115653949)) ;
#133403=CARTESIAN_POINT('Ctrl Pts',(-16.9572990580186,13.6358544266559,
131.25499330384)) ;
#133404=CARTESIAN_POINT('Ctrl Pts',(-16.9615071381463,13.3459427675745,
131.23424300822)) ;
#133405=CARTESIAN_POINT('Ctrl Pts',(-16.9909211180614,13.0604649745041,
131.286996740778)) ;
#133406=CARTESIAN_POINT('Ctrl Pts',(-17.0441007990242,12.8015143832803,
131.409241549806)) ;
#133407=CARTESIAN_POINT('Ctrl Pts',(-17.1180304186239,12.586871423154,131.592073079015)) ;
#133408=CARTESIAN_POINT('Ctrl Pts',(-17.2080500636742,12.4323032180318,
131.821934768459)) ;
#133409=CARTESIAN_POINT('Ctrl Pts',(-17.3084611337155,12.348604012381,132.082157360211)) ;
#133410=CARTESIAN_POINT('Ctrl Pts',(-17.4130111461555,12.3418345254331,
132.3544143668)) ;
#133411=CARTESIAN_POINT('Ctrl Pts',(-17.5146765749007,12.4127257697425,
132.618266949295)) ;
#133412=CARTESIAN_POINT('Ctrl Pts',(-17.606721170884,12.5554430365515,132.854114383774)) ;
#133413=CARTESIAN_POINT('Ctrl Pts',(-17.6839111619126,12.7608029240068,
133.046442139626)) ;
#133414=CARTESIAN_POINT('Ctrl Pts',(-17.7410331806284,13.0143079229722,
133.180091411217)) ;
#133415=CARTESIAN_POINT('Ctrl Pts',(-17.7745360164768,13.2953661026702,
133.244952941826)) ;
#133416=CARTESIAN_POINT('Ctrl Pts',(-17.7831520054483,13.587499191953,133.236886150184)) ;
#133417=CARTESIAN_POINT('Ctrl Pts',(-17.7666348632763,13.8669338626205,
133.155497022517)) ;
#133418=CARTESIAN_POINT('Ctrl Pts',(-17.7273863718362,14.1134263503453,
133.007875421063)) ;
#133419=CARTESIAN_POINT('Ctrl Pts',(-17.6683893078491,14.3121780897716,
132.802342611055)) ;
#133420=CARTESIAN_POINT('Ctrl Pts',(-17.5946147982464,14.4470050265316,
132.553591742459)) ;
#133421=CARTESIAN_POINT('Ctrl Pts',(-17.5125911040324,14.5078086325279,
132.280874384855)) ;
#133422=CARTESIAN_POINT('Ctrl Pts',(-17.4289255794743,14.4913412737729,
132.003473976216)) ;
#133423=CARTESIAN_POINT('Ctrl Pts',(-17.3497030184291,14.3985299043882,
131.738923406222)) ;
#133424=CARTESIAN_POINT('Ctrl Pts',(-17.2814947859058,14.2353764928408,
131.506472748856)) ;
#133425=CARTESIAN_POINT('Ctrl Pts',(-17.2301833982271,14.0132824388172,
131.32333677435)) ;
#133426=CARTESIAN_POINT('Ctrl Pts',(-17.2003726149901,13.751770584179,131.203370984278)) ;
#133427=CARTESIAN_POINT('Ctrl Pts',(-17.1942692410409,13.4639004603942,
131.15229798358)) ;
#133428=CARTESIAN_POINT('Ctrl Pts',(-17.2136563233809,13.1736259559936,
131.175755585428)) ;
#133429=CARTESIAN_POINT('Ctrl Pts',(-17.2572199771084,12.9029494351804,
131.270058586451)) ;
#133430=CARTESIAN_POINT('Ctrl Pts',(-17.3234518657098,12.6670694829694,
131.430263375814)) ;
#133431=CARTESIAN_POINT('Ctrl Pts',(-17.4076950363158,12.4867414535482,
131.643224441991)) ;
#133432=CARTESIAN_POINT('Ctrl Pts',(-17.5042594533731,12.3736046950475,
131.892333562312)) ;
#133433=CARTESIAN_POINT('Ctrl Pts',(-17.6083225797878,12.3351061359291,
132.163067552705)) ;
#133434=CARTESIAN_POINT('Ctrl Pts',(-17.7115102747659,12.3747297412366,
132.431506046747)) ;
#133435=CARTESIAN_POINT('Ctrl Pts',(-17.80835655534,12.4890530273647,132.681306942846)) ;
#133436=CARTESIAN_POINT('Ctrl Pts',(-17.8927139370083,12.6718473822343,
132.894413198474)) ;
#133437=CARTESIAN_POINT('Ctrl Pts',(-17.9581348743092,12.9071471042355,
133.05245843071)) ;
#133438=CARTESIAN_POINT('Ctrl Pts',(-18.0014489044881,13.1791583633753,
133.145922177929)) ;
#133439=CARTESIAN_POINT('Ctrl Pts',(-18.020261151911,13.4685703303894,133.16781609884)) ;
#133440=CARTESIAN_POINT('Ctrl Pts',(-18.0138792132709,13.7556865610863,
133.115998787948)) ;
#133441=CARTESIAN_POINT('Ctrl Pts',(-17.9834392562243,14.0184520779736,
132.993960277943)) ;
#133442=CARTESIAN_POINT('Ctrl Pts',(-17.9319093006337,14.2386835545227,
132.810307624848)) ;
#133443=CARTESIAN_POINT('Ctrl Pts',(-17.8634196060343,14.4009245247973,
132.577005577925)) ;
#133444=CARTESIAN_POINT('Ctrl Pts',(-17.7839956342627,14.4923209079493,
132.311848278652)) ;
#133445=CARTESIAN_POINT('Ctrl Pts',(-17.7003715420016,14.5074993821674,
132.034597515729)) ;
#133446=CARTESIAN_POINT('Ctrl Pts',(-17.6179715693461,14.4446391320812,
131.760580504429)) ;
#133447=CARTESIAN_POINT('Ctrl Pts',(-17.5449472629492,14.309013886893,131.514230915999)) ;
#133448=CARTESIAN_POINT('Ctrl Pts',(-17.4863929079662,14.1104149351794,
131.310125649846)) ;
#133449=CARTESIAN_POINT('Ctrl Pts',(-17.4472233098488,13.8614588559076,
131.162498832848)) ;
#133450=CARTESIAN_POINT('Ctrl Pts',(-17.4312869960412,13.5819687002437,
131.082859767227)) ;
#133451=CARTESIAN_POINT('Ctrl Pts',(-17.4402797073093,13.2906279013141,
131.075985151787)) ;
#133452=CARTESIAN_POINT('Ctrl Pts',(-17.4743143198391,13.009243305788,131.142317233284)) ;
#133453=CARTESIAN_POINT('Ctrl Pts',(-17.5315517099284,12.7575168112921,
131.276452625469)) ;
#133454=CARTESIAN_POINT('Ctrl Pts',(-17.6091410096472,12.5525240138587,
131.469879021206)) ;
#133455=CARTESIAN_POINT('Ctrl Pts',(-17.7014737885802,12.4108770336832,
131.706544893167)) ;
#133456=CARTESIAN_POINT('Ctrl Pts',(-17.8032831969416,12.3412909140522,
131.97080490142)) ;
#133457=CARTESIAN_POINT('Ctrl Pts',(-17.9077079735701,12.3493861735078,
132.242732393973)) ;
#133458=CARTESIAN_POINT('Ctrl Pts',(-18.0080021312736,12.4342727909203,
132.502613425746)) ;
#133459=CARTESIAN_POINT('Ctrl Pts',(-18.097851259794,12.5900489009072,132.731956223757)) ;
#133460=CARTESIAN_POINT('Ctrl Pts',(-18.1714811565311,12.8056265995217,
132.913906681068)) ;
#133461=CARTESIAN_POINT('Ctrl Pts',(-18.2242791522083,13.0653848746049,
133.035014327401)) ;
#133462=CARTESIAN_POINT('Ctrl Pts',(-18.2532373491338,13.3504851063388,
133.086511791274)) ;
#133463=CARTESIAN_POINT('Ctrl Pts',(-18.2570176970517,13.6412798147236,
133.064399324168)) ;
#133464=CARTESIAN_POINT('Ctrl Pts',(-18.2361288879767,13.915548156852,132.970331104728)) ;
#133465=CARTESIAN_POINT('Ctrl Pts',(-18.1927521468012,14.1552942040558,
132.810491998612)) ;
#133466=CARTESIAN_POINT('Ctrl Pts',(-18.1304889717146,14.3429101935435,
132.595396822877)) ;
#133467=CARTESIAN_POINT('Ctrl Pts',(-18.0549535994053,14.4639893047867,
132.341644352442)) ;
#133468=CARTESIAN_POINT('Ctrl Pts',(-17.9720169774795,14.5107279953385,
132.066239556179)) ;
#133469=CARTESIAN_POINT('Ctrl Pts',(-17.88839874123,14.4794893752074,131.788842595817)) ;
#133470=CARTESIAN_POINT('Ctrl Pts',(-17.8108656194136,14.3727211578977,
131.529246532274)) ;
#133471=CARTESIAN_POINT('Ctrl Pts',(-17.7456151211965,14.1977799584113,
131.305501822006)) ;
#133472=CARTESIAN_POINT('Ctrl Pts',(-17.6981151394564,13.9680803032242,
131.13369579038)) ;
#133473=CARTESIAN_POINT('Ctrl Pts',(-17.6723054333923,13.6967826933105,
131.024941140418)) ;
#133474=CARTESIAN_POINT('Ctrl Pts',(-17.6711447708163,13.4094043760888,
130.98862536116)) ;
#133475=CARTESIAN_POINT('Ctrl Pts',(-17.6950445630246,13.1212039321583,
131.025303143358)) ;
#133476=CARTESIAN_POINT('Ctrl Pts',(-17.74333311896,12.8546896237207,131.133221894845)) ;
#133477=CARTESIAN_POINT('Ctrl Pts',(-17.81282756458,12.6293810356165,131.303196900116)) ;
#133478=CARTESIAN_POINT('Ctrl Pts',(-17.9005194706817,12.4594635396626,
131.525988684649)) ;
#133479=CARTESIAN_POINT('Ctrl Pts',(-17.9986989569018,12.3604529302704,
131.779876218196)) ;
#133480=CARTESIAN_POINT('Ctrl Pts',(-18.1032340963646,12.3366695079855,
132.05199660503)) ;
#133481=CARTESIAN_POINT('Ctrl Pts',(-18.2056125319901,12.3907630606801,
132.318086056791)) ;
#133482=CARTESIAN_POINT('Ctrl Pts',(-18.300613364825,12.5187717527639,132.562441868016)) ;
#133483=CARTESIAN_POINT('Ctrl Pts',(-18.3816465085652,12.7125553045139,
132.765918032423)) ;
#133484=CARTESIAN_POINT('Ctrl Pts',(-18.4429853099616,12.9551208485313,
132.912159665352)) ;
#133485=CARTESIAN_POINT('Ctrl Pts',(-18.4820336765163,13.2325620060974,
132.993078593711)) ;
#133486=CARTESIAN_POINT('Ctrl Pts',(-18.496084383933,13.5243419796884,133.00090515124)) ;
#133487=CARTESIAN_POINT('Ctrl Pts',(-18.4850639350324,13.8069926528057,
132.935714610325)) ;
#133488=CARTESIAN_POINT('Ctrl Pts',(-18.4503367662865,14.0639000199269,
132.801056058483)) ;
#133489=CARTESIAN_POINT('Ctrl Pts',(-18.3952268191814,14.2741558930926,
132.606941700926)) ;
#133490=CARTESIAN_POINT('Ctrl Pts',(-18.3243680288223,14.4234615625839,
132.366801537788)) ;
#133491=CARTESIAN_POINT('Ctrl Pts',(-18.2437816042926,14.5011170686614,
132.098327447916)) ;
#133492=CARTESIAN_POINT('Ctrl Pts',(-18.1592384984199,14.5013614779113,
131.81807310291)) ;
#133493=CARTESIAN_POINT('Ctrl Pts',(-18.0789307375107,14.4249956630962,
131.550560960519)) ;
#133494=CARTESIAN_POINT('Ctrl Pts',(-18.0076541118125,14.2760171565871,
131.309082565097)) ;
#133495=CARTESIAN_POINT('Ctrl Pts',(-17.9524899575172,14.0665442400002,
131.114862544505)) ;
#133496=CARTESIAN_POINT('Ctrl Pts',(-17.9175014310239,13.8110528410318,
130.979547647309)) ;
#133497=CARTESIAN_POINT('Ctrl Pts',(-17.9061688391216,13.5262786463887,
130.913174372637)) ;
#133498=CARTESIAN_POINT('Ctrl Pts',(-17.919877948496,13.2368369901033,130.920277108179)) ;
#133499=CARTESIAN_POINT('Ctrl Pts',(-17.9586197277239,12.9583255903659,
131.000212959745)) ;
#133500=CARTESIAN_POINT('Ctrl Pts',(-18.0199083066583,12.7145800096232,
131.146219952724)) ;
#133501=CARTESIAN_POINT('Ctrl Pts',(-18.1009974511921,12.5201730384604,
131.349794172582)) ;
#133502=CARTESIAN_POINT('Ctrl Pts',(-18.1949562384929,12.392297716127,131.59141902566)) ;
#133503=CARTESIAN_POINT('Ctrl Pts',(-18.2981754606917,12.3368042043637,
131.859663996403)) ;
#133504=CARTESIAN_POINT('Ctrl Pts',(-18.4019398290045,12.3594079574846,
132.129799825424)) ;
#133505=CARTESIAN_POINT('Ctrl Pts',(-18.5013383418749,12.4588426243277,
132.386856715267)) ;
#133506=CARTESIAN_POINT('Ctrl Pts',(-18.5881323912535,12.6263832935465,
132.607414342136)) ;
#133507=CARTESIAN_POINT('Ctrl Pts',(-18.6581587702516,12.8513078071139,
132.778854814353)) ;
#133508=CARTESIAN_POINT('Ctrl Pts',(-18.7067345904951,13.1175341941134,
132.887608467018)) ;
#133509=CARTESIAN_POINT('Ctrl Pts',(-18.731003412201,13.4059954970849,132.925314381533)) ;
#133510=CARTESIAN_POINT('Ctrl Pts',(-18.7300968071152,13.6942419645787,
132.889656262388)) ;
#133511=CARTESIAN_POINT('Ctrl Pts',(-18.7044541735128,13.9656571359195,
132.781395875164)) ;
#133512=CARTESIAN_POINT('Ctrl Pts',(-18.6575265026644,14.1945698215837,
132.611470543872)) ;
#133513=CARTESIAN_POINT('Ctrl Pts',(-18.5922406519204,14.3711224528334,
132.387486886082)) ;
#133514=CARTESIAN_POINT('Ctrl Pts',(-18.5149037393986,14.4785950091488,
132.128508392993)) ;
#133515=CARTESIAN_POINT('Ctrl Pts',(-18.4311371510558,14.5108133112394,
131.850601957705)) ;
#133516=CARTESIAN_POINT('Ctrl Pts',(-18.3483146549276,14.4650394200622,
131.575598992863)) ;
#133517=CARTESIAN_POINT('Ctrl Pts',(-18.2726066198908,14.3446919400874,
131.321313280288)) ;
#133518=CARTESIAN_POINT('Ctrl Pts',(-18.2103307361537,14.1586507898245,
131.106307024848)) ;
#133519=CARTESIAN_POINT('Ctrl Pts',(-18.1664432390162,13.9182142591253,
130.944795156692)) ;
#133520=CARTESIAN_POINT('Ctrl Pts',(-18.1453636366719,13.6446894301756,
130.850233747273)) ;
#133521=CARTESIAN_POINT('Ctrl Pts',(-18.1488348343508,13.3538163555555,
130.82719813754)) ;
#133522=CARTESIAN_POINT('Ctrl Pts',(-18.1774811245967,13.0687529323482,
130.877811758373)) ;
#133523=CARTESIAN_POINT('Ctrl Pts',(-18.2300437642224,12.8084025711039,
130.998208929724)) ;
#133524=CARTESIAN_POINT('Ctrl Pts',(-18.3034001053734,12.5923662507696,
131.179384620874)) ;
#133525=CARTESIAN_POINT('Ctrl Pts',(-18.3931634370597,12.4355966936421,
131.408445657945)) ;
#133526=CARTESIAN_POINT('Ctrl Pts',(-18.4935575860177,12.3498834173245,
131.668562849344)) ;
#133527=CARTESIAN_POINT('Ctrl Pts',(-18.5975530541275,12.3409542808635,
131.939369081028)) ;
#133528=CARTESIAN_POINT('Ctrl Pts',(-18.6994673351223,12.4093757248112,
132.203931136602)) ;
#133529=CARTESIAN_POINT('Ctrl Pts',(-18.7921201529756,12.5505196315372,
132.441467645947)) ;
#133530=CARTESIAN_POINT('Ctrl Pts',(-18.8697017731338,12.7541803006072,
132.634971878383)) ;
#133531=CARTESIAN_POINT('Ctrl Pts',(-18.9273307484839,13.0055267425044,
132.770220733639)) ;
#133532=CARTESIAN_POINT('Ctrl Pts',(-18.9617100390982,13.2870724884799,
132.83751270461)) ;
#133533=CARTESIAN_POINT('Ctrl Pts',(-18.9710255677151,13.5781354317469,
132.831615285865)) ;
#133534=CARTESIAN_POINT('Ctrl Pts',(-18.9553578084607,13.8583662507443,
132.752702523973)) ;
#133535=CARTESIAN_POINT('Ctrl Pts',(-18.9165383575917,14.1072755060793,
132.606171710367)) ;
#133536=CARTESIAN_POINT('Ctrl Pts',(-18.8581587772242,14.3069765889331,
132.4025330216)) ;
#133537=CARTESIAN_POINT('Ctrl Pts',(-18.7850681968336,14.443614067786,132.155907192059)) ;
#133538=CARTESIAN_POINT('Ctrl Pts',(-18.702941141321,14.5071928082345,131.882773592227)) ;
#133539=CARTESIAN_POINT('Ctrl Pts',(-18.6190408117616,14.4928945220509,
131.604612881179)) ;
#133540=CARTESIAN_POINT('Ctrl Pts',(-18.5396187459799,14.4021254936154,
131.339485656911)) ;
#133541=CARTESIAN_POINT('Ctrl Pts',(-18.4711933901986,14.2413770477371,
131.106496569037)) ;
#133542=CARTESIAN_POINT('Ctrl Pts',(-18.4192605637911,14.0210258594474,
130.921552581758)) ;
#133543=CARTESIAN_POINT('Ctrl Pts',(-18.3886405960536,13.7594508415378,
130.799092122936)) ;
#133544=CARTESIAN_POINT('Ctrl Pts',(-18.381928462571,13.4716753030503,130.746210031867)) ;
#133545=CARTESIAN_POINT('Ctrl Pts',(-18.4004216312574,13.18278007244,130.767242888151)) ;
#133546=CARTESIAN_POINT('Ctrl Pts',(-18.4435339670258,12.9097866347109,
130.860039653288)) ;
#133547=CARTESIAN_POINT('Ctrl Pts',(-18.5088204983959,12.6739761120234,
131.017674750893)) ;
#133548=CARTESIAN_POINT('Ctrl Pts',(-18.5926770612546,12.4911376353209,
131.229439455072)) ;
#133549=CARTESIAN_POINT('Ctrl Pts',(-18.6895108158381,12.3755758788311,
131.479159592622)) ;
#133550=CARTESIAN_POINT('Ctrl Pts',(-18.7928542788589,12.3352662329562,
131.747989657394)) ;
#133551=CARTESIAN_POINT('Ctrl Pts',(-18.8962659376777,12.3722006143293,
132.017051741353)) ;
#133552=CARTESIAN_POINT('Ctrl Pts',(-18.9940984306609,12.4858118722087,
132.26946955847)) ;
#133553=CARTESIAN_POINT('Ctrl Pts',(-19.0779483654093,12.6649628027199,
132.481462828409)) ;
#133554=CARTESIAN_POINT('Ctrl Pts',(-19.144324386781,12.8995424291904,132.64216747859)) ;
#133555=CARTESIAN_POINT('Ctrl Pts',(-19.1882893988472,13.1707489990253,
132.73754255469)) ;
#133556=CARTESIAN_POINT('Ctrl Pts',(-19.2078747746244,13.4602465419289,
132.76165779285)) ;
#133557=CARTESIAN_POINT('Ctrl Pts',(-19.2021695943243,13.7479094104328,
132.711797460233)) ;
#133558=CARTESIAN_POINT('Ctrl Pts',(-19.1724541288044,14.0110933638022,
132.591943088721)) ;
#133559=CARTESIAN_POINT('Ctrl Pts',(-19.1214789970609,14.2330195298938,
132.409891780119)) ;
#133560=CARTESIAN_POINT('Ctrl Pts',(-19.0533824116154,14.397056415232,132.177734508543)) ;
#133561=CARTESIAN_POINT('Ctrl Pts',(-18.9744610193818,14.4906410938832,
131.914150162339)) ;
#133562=CARTESIAN_POINT('Ctrl Pts',(-18.890345578861,14.5080280130628,131.635247249356)) ;
#133563=CARTESIAN_POINT('Ctrl Pts',(-18.8085392860132,14.4480725424633,
131.363277720596)) ;
#133564=CARTESIAN_POINT('Ctrl Pts',(-18.7346273925197,14.3139470607326,
131.114108989611)) ;
#133565=CARTESIAN_POINT('Ctrl Pts',(-18.6756142626322,14.1169437524237,
130.908679443903)) ;
#133566=CARTESIAN_POINT('Ctrl Pts',(-18.6357563526766,13.8684682048696,
130.758950982595)) ;
#133567=CARTESIAN_POINT('Ctrl Pts',(-18.6192189361488,13.5907243651,130.677694418299)) ;
#133568=CARTESIAN_POINT('Ctrl Pts',(-18.6274186795787,13.2994062522709,
130.668497076563)) ;
#133569=CARTESIAN_POINT('Ctrl Pts',(-18.6607053713449,13.0173302811176,
130.732637587237)) ;
#133570=CARTESIAN_POINT('Ctrl Pts',(-18.7175745221499,12.7634586998748,
130.865557336184)) ;
#133571=CARTESIAN_POINT('Ctrl Pts',(-18.7946062779487,12.5574053612187,
131.057405473283)) ;
#133572=CARTESIAN_POINT('Ctrl Pts',(-18.8863176363417,12.4141338116398,
131.292346024062)) ;
#133573=CARTESIAN_POINT('Ctrl Pts',(-18.9880396659882,12.342233208706,131.556318246303)) ;
#133574=CARTESIAN_POINT('Ctrl Pts',(-19.092367557879,12.3479816385131,131.828001920729)) ;
#133575=CARTESIAN_POINT('Ctrl Pts',(-19.1930265312653,12.4308508598937,
132.088893600864)) ;
#133576=CARTESIAN_POINT('Ctrl Pts',(-19.2830355733598,12.5841342714032,
132.318802233278)) ;
#133577=CARTESIAN_POINT('Ctrl Pts',(-19.3575448753726,12.7991564308112,
132.503166321675)) ;
#133578=CARTESIAN_POINT('Ctrl Pts',(-19.410786935153,13.0569999610756,132.625693509338)) ;
#133579=CARTESIAN_POINT('Ctrl Pts',(-19.4405356262244,13.3421921034464,
132.679428679679)) ;
#133580=CARTESIAN_POINT('Ctrl Pts',(-19.4450790880921,13.6321454574867,
132.659662972591)) ;
#133581=CARTESIAN_POINT('Ctrl Pts',(-19.4247875387373,13.9089725412032,
132.567125349093)) ;
#133582=CARTESIAN_POINT('Ctrl Pts',(-19.381825668748,14.1498188340954,132.408476398238)) ;
#133583=CARTESIAN_POINT('Ctrl Pts',(-19.3204518279194,14.3379335225619,
132.196198119276)) ;
#133584=CARTESIAN_POINT('Ctrl Pts',(-19.2450347897687,14.4615825769609,
131.942693860373)) ;
#133585=CARTESIAN_POINT('Ctrl Pts',(-19.162267963524,14.5104718339952,131.667809535155)) ;
#133586=CARTESIAN_POINT('Ctrl Pts',(-19.0783524563333,14.4813917081873,
131.389457000585)) ;
#133587=CARTESIAN_POINT('Ctrl Pts',(-19.0006162859046,14.3764101476522,
131.129272642533)) ;
#133588=CARTESIAN_POINT('Ctrl Pts',(-18.9351626104612,14.2041613001764,
130.905077291113)) ;
#133589=CARTESIAN_POINT('Ctrl Pts',(-18.8868641696125,13.9743839791119,
130.730738018104)) ;
#133590=CARTESIAN_POINT('Ctrl Pts',(-18.8605695212481,13.7063210401926,
130.620861352139)) ;
#133591=CARTESIAN_POINT('Ctrl Pts',(-18.8586114405782,13.416701167449,130.581917827711)) ;
#133592=CARTESIAN_POINT('Ctrl Pts',(-18.8818454285258,13.1291677758352,
130.616763647551)) ;
#133593=CARTESIAN_POINT('Ctrl Pts',(-18.9294289009308,12.86171027905,130.722620411742)) ;
#133594=CARTESIAN_POINT('Ctrl Pts',(-18.9984336324713,12.6350478480017,
130.891152728659)) ;
#133595=CARTESIAN_POINT('Ctrl Pts',(-19.0852684560724,12.4638699665219,
131.111590594525)) ;
#133596=CARTESIAN_POINT('Ctrl Pts',(-19.1836902605787,12.3621126869917,
131.366013493841)) ;
#133597=CARTESIAN_POINT('Ctrl Pts',(-19.2880034593845,12.336288293437,131.637540200635)) ;
#133598=CARTESIAN_POINT('Ctrl Pts',(-19.3907293591919,12.3882079133966,
131.9045787098)) ;
#133599=CARTESIAN_POINT('Ctrl Pts',(-19.4861202999562,12.5148240028862,
132.150020522081)) ;
#133600=CARTESIAN_POINT('Ctrl Pts',(-19.566984502277,12.7050812653244,132.353293437429)) ;
#133601=CARTESIAN_POINT('Ctrl Pts',(-19.6294717703468,12.9482677220772,
132.502618790391)) ;
#133602=CARTESIAN_POINT('Ctrl Pts',(-19.6689768655333,13.2238578222556,
132.585025535771)) ;
#133603=CARTESIAN_POINT('Ctrl Pts',(-19.6838357324499,13.5162932448957,
132.595118812429)) ;
#133604=CARTESIAN_POINT('Ctrl Pts',(-19.6735197937544,13.799165239793,132.532024333921)) ;
#133605=CARTESIAN_POINT('Ctrl Pts',(-19.6392454600331,14.0580267764743,
132.398557205212)) ;
#133606=CARTESIAN_POINT('Ctrl Pts',(-19.5848869196862,14.2686028129511,
132.206807442572)) ;
#133607=CARTESIAN_POINT('Ctrl Pts',(-19.5145008411043,14.4199618502008,
131.968069495771)) ;
#133608=CARTESIAN_POINT('Ctrl Pts',(-19.4340220268986,14.4998958219189,
131.699871465245)) ;
#133609=CARTESIAN_POINT('Ctrl Pts',(-19.3495759662661,14.5025664794371,
131.419941342377)) ;
#133610=CARTESIAN_POINT('Ctrl Pts',(-19.2688627445457,14.4280652825415,
131.151146889785)) ;
#133611=CARTESIAN_POINT('Ctrl Pts',(-19.197514432747,14.2819177513075,130.909621465088)) ;
#133612=CARTESIAN_POINT('Ctrl Pts',(-19.1413921728409,14.0723877227319,
130.712339919469)) ;
#133613=CARTESIAN_POINT('Ctrl Pts',(-19.1060584048045,13.8191595273478,
130.576195818314)) ;
#133614=CARTESIAN_POINT('Ctrl Pts',(-19.0939136018658,13.5356702848312,
130.507524027747)) ;
#133615=CARTESIAN_POINT('Ctrl Pts',(-19.1068958007053,13.2451626614465,
130.512392184105)) ;
#133616=CARTESIAN_POINT('Ctrl Pts',(-19.1449564065195,12.9658959397094,
130.5903314269)) ;
#133617=CARTESIAN_POINT('Ctrl Pts',(-19.2057189790489,12.720867949973,130.73477557543)) ;
#133618=CARTESIAN_POINT('Ctrl Pts',(-19.2858400354675,12.5256178596935,
130.935699785553)) ;
#133619=CARTESIAN_POINT('Ctrl Pts',(-19.3800402811628,12.3947249390078,
131.177818876414)) ;
#133620=CARTESIAN_POINT('Ctrl Pts',(-19.4831200353959,12.3373274128747,
131.445666380565)) ;
#133621=CARTESIAN_POINT('Ctrl Pts',(-19.5867485454506,12.3577351376061,
131.715460652154)) ;
#133622=CARTESIAN_POINT('Ctrl Pts',(-19.6862131801358,12.4546492514378,
131.972779675498)) ;
#133623=CARTESIAN_POINT('Ctrl Pts',(-19.7738286134021,12.6210676591383,
132.195587853881)) ;
#133624=CARTESIAN_POINT('Ctrl Pts',(-19.8442902702029,12.8446766854148,
132.368316433847)) ;
#133625=CARTESIAN_POINT('Ctrl Pts',(-19.8933608798738,13.108808163257,132.478653710118)) ;
#133626=CARTESIAN_POINT('Ctrl Pts',(-19.9184859283659,13.3979062620311,
132.518747291947)) ;
#133627=CARTESIAN_POINT('Ctrl Pts',(-19.9181983031023,13.6859097607706,
132.484944374893)) ;
#133628=CARTESIAN_POINT('Ctrl Pts',(-19.8935840118438,13.9567565280856,
132.379898432991)) ;
#133629=CARTESIAN_POINT('Ctrl Pts',(-19.8465997978561,14.1899349125241,
132.209373856163)) ;
#133630=CARTESIAN_POINT('Ctrl Pts',(-19.7823820361551,14.3662692626876,
131.988864508273)) ;
#133631=CARTESIAN_POINT('Ctrl Pts',(-19.7048377925854,14.4768289979695,
131.729048105592)) ;
#133632=CARTESIAN_POINT('Ctrl Pts',(-19.621356858463,14.5109207090365,131.452070562692)) ;
#133633=CARTESIAN_POINT('Ctrl Pts',(-19.5383256537918,14.4673589954117,
131.176412965102)) ;
#133634=CARTESIAN_POINT('Ctrl Pts',(-19.462343360731,14.3490298117359,130.921339630599)) ;
#133635=CARTESIAN_POINT('Ctrl Pts',(-19.399598094763,14.1643442573792,130.70492417211)) ;
#133636=CARTESIAN_POINT('Ctrl Pts',(-19.3553585530389,13.9269540764464,
130.542614298548)) ;
#133637=CARTESIAN_POINT('Ctrl Pts',(-19.3333939719036,13.6529087066834,
130.44529695513)) ;
#133638=CARTESIAN_POINT('Ctrl Pts',(-19.3361541913265,13.3625040426011,
130.420224634067)) ;
#133639=CARTESIAN_POINT('Ctrl Pts',(-19.3641172961552,13.0764917625792,
130.468781137817)) ;
#133640=CARTESIAN_POINT('Ctrl Pts',(-19.4160399610195,12.8152457852602,
130.587319851219)) ;
#133641=CARTESIAN_POINT('Ctrl Pts',(-19.4888652574942,12.5977360848388,
130.766942106929)) ;
#133642=CARTESIAN_POINT('Ctrl Pts',(-19.5781388686584,12.4392301767845,
130.994608862376)) ;
#133643=CARTESIAN_POINT('Ctrl Pts',(-19.6782931891438,12.3513755992719,
131.254028736787)) ;
#133644=CARTESIAN_POINT('Ctrl Pts',(-19.7822229405507,12.3399316332142,
131.524661009902)) ;
#133645=CARTESIAN_POINT('Ctrl Pts',(-19.88504344773,12.4070554351268,131.791616350641)) ;
#133646=CARTESIAN_POINT('Ctrl Pts',(-19.9771610745846,12.5451369869361,
132.027897931008)) ;
#133647=CARTESIAN_POINT('Ctrl Pts',(-20.0556173721215,12.7477726868892,
132.223821692675)) ;
#133648=CARTESIAN_POINT('Ctrl Pts',(-20.1137903255926,12.9979367372735,
132.360683275234)) ;
#133649=CARTESIAN_POINT('Ctrl Pts',(-20.1489013724765,13.2792370978739,
132.430071631305)) ;
#133650=CARTESIAN_POINT('Ctrl Pts',(-20.1588787384282,13.5701580555343,
132.426125674529)) ;
#133651=CARTESIAN_POINT('Ctrl Pts',(-20.143937682242,13.8505377724051,132.349389311992)) ;
#133652=CARTESIAN_POINT('Ctrl Pts',(-20.1057318059421,14.1007512372239,
132.20463305785)) ;
#133653=CARTESIAN_POINT('Ctrl Pts',(-20.0478354950526,14.3021715583994,
132.002395149785)) ;
#133654=CARTESIAN_POINT('Ctrl Pts',(-19.9748500391882,14.4410638226486,
131.755979394128)) ;
#133655=CARTESIAN_POINT('Ctrl Pts',(-19.892940104349,14.506420576945,131.483512074612)) ;
#133656=CARTESIAN_POINT('Ctrl Pts',(-19.8092678890523,14.4944296739133,
131.206120710523)) ;
#133657=CARTESIAN_POINT('Ctrl Pts',(-19.7294350859359,14.4055611915821,
130.939713797808)) ;
#133658=CARTESIAN_POINT('Ctrl Pts',(-19.66081208133,14.2469875620131,130.706232624641)) ;
#133659=CARTESIAN_POINT('Ctrl Pts',(-19.6083158027718,14.0284942715184,
130.519673218377)) ;
#133660=CARTESIAN_POINT('Ctrl Pts',(-19.5769557514165,13.7670074742828,
130.394940588624)) ;
#133661=CARTESIAN_POINT('Ctrl Pts',(-19.5695668686991,13.4805781215048,
130.340191561689)) ;
#133662=CARTESIAN_POINT('Ctrl Pts',(-19.5872696261961,13.1913388058783,
130.358899107894)) ;
#133663=CARTESIAN_POINT('Ctrl Pts',(-19.6297522740938,12.9172330933754,
130.449814911348)) ;
#133664=CARTESIAN_POINT('Ctrl Pts',(-19.6944389773908,12.6799728703758,
130.60569175476)) ;
#133665=CARTESIAN_POINT('Ctrl Pts',(-19.7782230780513,12.4949910418975,
130.817115688087)) ;
#133666=CARTESIAN_POINT('Ctrl Pts',(-19.8739923402946,12.3781840447206,
131.063992159593)) ;
#133667=CARTESIAN_POINT('Ctrl Pts',(-19.9780674608701,12.3352411023339,
131.33468497079)) ;
#133668=CARTESIAN_POINT('Ctrl Pts',(-20.0810744379286,12.3701183957634,
131.602725123913)) ;
#133669=CARTESIAN_POINT('Ctrl Pts',(-20.179252895713,12.4815908370187,131.85612905703)) ;
#133670=CARTESIAN_POINT('Ctrl Pts',(-20.2634570739637,12.6586744463426,
132.069206441814)) ;
#133671=CARTESIAN_POINT('Ctrl Pts',(-20.3305901520664,12.8927064505131,
132.232014267973)) ;
#133672=CARTESIAN_POINT('Ctrl Pts',(-20.3750331233153,13.1615895986342,
132.328969789793)) ;
#133673=CARTESIAN_POINT('Ctrl Pts',(-20.3954965997089,13.4527337961883,
132.355428882089)) ;
#133674=CARTESIAN_POINT('Ctrl Pts',(-20.3904573045894,13.7397606263225,
132.307631593907)) ;
#133675=CARTESIAN_POINT('Ctrl Pts',(-20.3613437715797,14.0044956878458,
132.189457679076)) ;
#133676=CARTESIAN_POINT('Ctrl Pts',(-20.3110168045734,14.2270717047825,
132.009394785638)) ;
#133677=CARTESIAN_POINT('Ctrl Pts',(-20.2436381751946,14.3928428531141,
131.779444891534)) ;
#133678=CARTESIAN_POINT('Ctrl Pts',(-20.164336633125,14.4891679896536,131.51449038135)) ;
#133679=CARTESIAN_POINT('Ctrl Pts',(-20.0809111882638,14.5086708936273,
131.237865647246)) ;
#133680=CARTESIAN_POINT('Ctrl Pts',(-19.9983950566067,14.4507091204102,
130.963592375788)) ;
#133681=CARTESIAN_POINT('Ctrl Pts',(-19.9244190141413,14.318823465338,130.714351089596)) ;
#133682=CARTESIAN_POINT('Ctrl Pts',(-19.8648700988791,14.1234067424229,
130.507330724768)) ;
#133683=CARTESIAN_POINT('Ctrl Pts',(-19.8245161746179,13.8772496577341,
130.356293737963)) ;
#133684=CARTESIAN_POINT('Ctrl Pts',(-19.8070957881005,13.5994498547175,
130.272359938913)) ;
#133685=CARTESIAN_POINT('Ctrl Pts',(-19.8146864693653,13.3067289539218,
130.261220009531)) ;
#133686=CARTESIAN_POINT('Ctrl Pts',(-19.8471784531872,13.025513208076,130.323196727465)) ;
#133687=CARTESIAN_POINT('Ctrl Pts',(-19.9032180692331,12.7708776887036,
130.453754380472)) ;
#133688=CARTESIAN_POINT('Ctrl Pts',(-19.9797679754465,12.5628412979246,
130.644157296538)) ;
#133689=CARTESIAN_POINT('Ctrl Pts',(-20.0712997390683,12.4171764122364,
130.878502714501)) ;
#133690=CARTESIAN_POINT('Ctrl Pts',(-20.173220666744,12.3431378359771,131.142938313351)) ;
#133691=CARTESIAN_POINT('Ctrl Pts',(-20.2769543623743,12.3467434972734,
131.413078047708)) ;
#133692=CARTESIAN_POINT('Ctrl Pts',(-20.3779474556413,12.4272274658185,
131.674911921515)) ;
#133693=CARTESIAN_POINT('Ctrl Pts',(-20.4684824931614,12.5790158149027,
131.906293765199)) ;
#133694=CARTESIAN_POINT('Ctrl Pts',(-20.5433178346082,12.7916687829571,
132.091724629749)) ;
#133695=CARTESIAN_POINT('Ctrl Pts',(-20.59747019779,13.0498138992039,132.216737279054)) ;
#133696=CARTESIAN_POINT('Ctrl Pts',(-20.6277539698486,13.3331756720239,
132.272199599018)) ;
#133697=CARTESIAN_POINT('Ctrl Pts',(-20.63310319697,13.6238935345468,132.254712776567)) ;
#133698=CARTESIAN_POINT('Ctrl Pts',(-20.6135004102223,13.9010885274901,
132.164225860573)) ;
#133699=CARTESIAN_POINT('Ctrl Pts',(-20.5712628793398,14.1432054793993,
132.007719764268)) ;
#133700=CARTESIAN_POINT('Ctrl Pts',(-20.5099062183509,14.3341070280144,
131.795269476235)) ;
#133701=CARTESIAN_POINT('Ctrl Pts',(-20.4352339689786,14.4587991787124,
131.544150012527)) ;
#133702=CARTESIAN_POINT('Ctrl Pts',(-20.3525489079931,14.5101605081857,
131.269477291802)) ;
#133703=CARTESIAN_POINT('Ctrl Pts',(-20.2687361872864,14.4834097576633,
130.991492371573)) ;
#133704=CARTESIAN_POINT('Ctrl Pts',(-20.1906756501309,14.380986704451,130.730363509583)) ;
#133705=CARTESIAN_POINT('Ctrl Pts',(-20.1243569260148,14.2089571607828,
130.503381990289)) ;
#133706=CARTESIAN_POINT('Ctrl Pts',(-20.0759333865454,13.9828180453883,
130.329004955831)) ;
#133707=CARTESIAN_POINT('Ctrl Pts',(-20.0486953445985,13.7132629209954,
130.216063933579)) ;
#133708=CARTESIAN_POINT('Ctrl Pts',(-20.0461136758052,13.42583764063,130.175529664949)) ;
#133709=CARTESIAN_POINT('Ctrl Pts',(-20.0685766436055,13.1374631065902,
130.208056459246)) ;
#133710=CARTESIAN_POINT('Ctrl Pts',(-20.1154485813734,12.8691197006536,
130.31184888817)) ;
#133711=CARTESIAN_POINT('Ctrl Pts',(-20.1842161886027,12.6403113443668,
130.479551228157)) ;
#133712=CARTESIAN_POINT('Ctrl Pts',(-20.2699974667944,12.468420702256,130.697148821309)) ;
#133713=CARTESIAN_POINT('Ctrl Pts',(-20.368777345651,12.3638000217504,130.952399609198)) ;
#133714=CARTESIAN_POINT('Ctrl Pts',(-20.4724837589939,12.3359859144704,
131.22233281641)) ;
#133715=CARTESIAN_POINT('Ctrl Pts',(-20.5755189014966,12.3855342690204,
131.490214378318)) ;
#133716=CARTESIAN_POINT('Ctrl Pts',(-20.6710370148352,12.5097023136888,
131.736103980719)) ;
#133717=CARTESIAN_POINT('Ctrl Pts',(-20.7526999022241,12.6987169895182,
131.941597617443)) ;
#133718=CARTESIAN_POINT('Ctrl Pts',(-20.8159200282362,12.9413958856346,
132.092978431002)) ;
#133719=CARTESIAN_POINT('Ctrl Pts',(-20.8560148207953,13.2164083911014,
132.177101494275)) ;
#133720=CARTESIAN_POINT('Ctrl Pts',(-20.8715568106971,13.5077476116907,
132.18930496735)) ;
#133721=CARTESIAN_POINT('Ctrl Pts',(-20.8618791478333,13.7917084995172,
132.127994218716)) ;
#133722=CARTESIAN_POINT('Ctrl Pts',(-20.8285666993428,14.0497089633418,
131.997596945122)) ;
#133723=CARTESIAN_POINT('Ctrl Pts',(-20.7745879228126,14.2632250030891,
131.806787903495)) ;
#133724=CARTESIAN_POINT('Ctrl Pts',(-20.7043311974277,14.4168537708596,
131.568328459368)) ;
#133725=CARTESIAN_POINT('Ctrl Pts',(-20.6239603167272,14.4987598986465,
131.300415425815)) ;
#133726=CARTESIAN_POINT('Ctrl Pts',(-20.539754785129,14.5035045718472,131.021276419093)) ;
#133727=CARTESIAN_POINT('Ctrl Pts',(-20.4588117616689,14.4313229997249,
130.751803459987)) ;
#133728=CARTESIAN_POINT('Ctrl Pts',(-20.3868956375626,14.286096674379,130.508478859911)) ;
#133729=CARTESIAN_POINT('Ctrl Pts',(-20.3308554449234,14.0806888556304,
130.311826279916)) ;
#133730=CARTESIAN_POINT('Ctrl Pts',(-20.2944696102375,13.8265805447723,
130.172317712221)) ;
#133731=CARTESIAN_POINT('Ctrl Pts',(-20.2817095072984,13.5441879409374,
130.101929815543)) ;
#133732=CARTESIAN_POINT('Ctrl Pts',(-20.2939970046262,13.2530370689606,
130.104694604891)) ;
#133733=CARTESIAN_POINT('Ctrl Pts',(-20.3312192505214,12.9741114175935,
130.18030810907)) ;
#133734=CARTESIAN_POINT('Ctrl Pts',(-20.391477731723,12.7272119216586,130.323195480133)) ;
#133735=CARTESIAN_POINT('Ctrl Pts',(-20.4710215017653,12.5305677659782,
130.522476172394)) ;
#133736=CARTESIAN_POINT('Ctrl Pts',(-20.5648765077218,12.3976028767503,
130.763584707341)) ;
#133737=CARTESIAN_POINT('Ctrl Pts',(-20.6677354645716,12.3378877564715,
131.030810858964)) ;
#133738=CARTESIAN_POINT('Ctrl Pts',(-20.771610142133,12.3561146457162,131.301258410359)) ;
#133739=CARTESIAN_POINT('Ctrl Pts',(-20.8710140356471,12.4504996091204,
131.558507272223)) ;
#133740=CARTESIAN_POINT('Ctrl Pts',(-20.9591976245712,12.6151918179393,
131.782920165643)) ;
#133741=CARTESIAN_POINT('Ctrl Pts',(-21.0301909969835,12.8367627956422,
131.957264907826)) ;
#133742=CARTESIAN_POINT('Ctrl Pts',(-21.0802720431719,13.102471284239,132.070248175628)) ;
#133743=CARTESIAN_POINT('Ctrl Pts',(-21.1058128562322,13.388098474674,132.11192368682)) ;
#133744=CARTESIAN_POINT('Ctrl Pts',(-21.1063578527298,13.6786302634614,
132.08028850925)) ;
#133745=CARTESIAN_POINT('Ctrl Pts',(-21.0823275663731,13.9495118019851,
131.977027551482)) ;
#133746=CARTESIAN_POINT('Ctrl Pts',(-21.0362217842379,14.1831630717315,
131.809216673534)) ;
#133747=CARTESIAN_POINT('Ctrl Pts',(-20.9721884045855,14.3622887251467,
131.589091305906)) ;
#133748=CARTESIAN_POINT('Ctrl Pts',(-20.8947792880245,14.4748192529362,
131.32962547702)) ;
#133749=CARTESIAN_POINT('Ctrl Pts',(-20.8116749026299,14.5109473630978,
131.053861074448)) ;
#133750=CARTESIAN_POINT('Ctrl Pts',(-20.7286272549608,14.46989386631,130.778195045776)) ;
#133751=CARTESIAN_POINT('Ctrl Pts',(-20.6522431108941,14.3536144736526,
130.521907930923)) ;
#133752=CARTESIAN_POINT('Ctrl Pts',(-20.5889583813436,14.17062113719,130.303892930056)) ;
#133753=CARTESIAN_POINT('Ctrl Pts',(-20.5440524129988,13.933736573907,130.13953810035)) ;
#133754=CARTESIAN_POINT('Ctrl Pts',(-20.5214975045223,13.6617104442443,
130.040649083481)) ;
#133755=CARTESIAN_POINT('Ctrl Pts',(-20.5235105668905,13.3701432171844,
130.013237741548)) ;
#133756=CARTESIAN_POINT('Ctrl Pts',(-20.5508607538459,13.0839501475181,
130.0600249237)) ;
#133757=CARTESIAN_POINT('Ctrl Pts',(-20.6019342296123,12.8226369063403,
130.176200002378)) ;
#133758=CARTESIAN_POINT('Ctrl Pts',(-20.674162245095,12.6036153158418,130.354083975274)) ;
#133759=CARTESIAN_POINT('Ctrl Pts',(-20.7628382753172,12.4432239429731,
130.580060592785)) ;
#133760=CARTESIAN_POINT('Ctrl Pts',(-20.8633579914741,12.3525997513282,
130.840351394468)) ;
#133761=CARTESIAN_POINT('Ctrl Pts',(-20.9671168641114,12.3393903655815,
131.110528978872)) ;
#133762=CARTESIAN_POINT('Ctrl Pts',(-21.0694306011919,12.403468098602,131.376231401918)) ;
#133763=CARTESIAN_POINT('Ctrl Pts',(-21.1627219404933,12.5405072085783,
131.615661785443)) ;
#133764=CARTESIAN_POINT('Ctrl Pts',(-21.2416127937835,12.7420005519616,
131.812839172161)) ;
#133765=CARTESIAN_POINT('Ctrl Pts',(-21.3001704333997,12.9900801149227,
131.950949061272)) ;
#133766=CARTESIAN_POINT('Ctrl Pts',(-21.3360159038547,13.2708158721555,
132.022475029764)) ;
#133767=CARTESIAN_POINT('Ctrl Pts',(-21.3467250085586,13.5613604134334,
132.020708203514)) ;
#133768=CARTESIAN_POINT('Ctrl Pts',(-21.332530072888,13.8428560081929,131.946099675255)) ;
#133769=CARTESIAN_POINT('Ctrl Pts',(-21.2946880005883,14.0951246502648,
131.802259522002)) ;
#133770=CARTESIAN_POINT('Ctrl Pts',(-21.2376357521135,14.2968154125605,
131.602698948677)) ;
#133771=CARTESIAN_POINT('Ctrl Pts',(-21.164806246768,14.4382062812648,131.356634806151)) ;
#133772=CARTESIAN_POINT('Ctrl Pts',(-21.0832408338308,14.5055713938207,
131.085254319312)) ;
#133773=CARTESIAN_POINT('Ctrl Pts',(-20.9994162423038,14.4957941932041,
130.807360837672)) ;
#133774=CARTESIAN_POINT('Ctrl Pts',(-20.9195959138854,14.4095662340998,
130.541102349046)) ;
#133775=CARTESIAN_POINT('Ctrl Pts',(-20.8500186277359,14.2515335127425,
130.304558118666)) ;
#133776=CARTESIAN_POINT('Ctrl Pts',(-20.7972486154139,14.0347236874785,
130.11728882556)) ;
#133777=CARTESIAN_POINT('Ctrl Pts',(-20.7653613268004,13.7751700114088,
129.991129528377)) ;
#133778=CARTESIAN_POINT('Ctrl Pts',(-20.7571817990629,13.489555102194,129.934113768398)) ;
#133779=CARTESIAN_POINT('Ctrl Pts',(-20.7742556911792,13.1989624545804,
129.950844344899)) ;
#133780=CARTESIAN_POINT('Ctrl Pts',(-20.8159809707414,12.9245155762064,
130.03960916018)) ;
#133781=CARTESIAN_POINT('Ctrl Pts',(-20.8805367450398,12.6850932088169,
130.194926855194)) ;
#133782=CARTESIAN_POINT('Ctrl Pts',(-20.9626356003938,12.5007200500438,
130.401901459438)) ;
#133783=CARTESIAN_POINT('Ctrl Pts',(-21.0591957946408,12.3802348015134,
130.650687618331)) ;
#133784=CARTESIAN_POINT('Ctrl Pts',(-21.1622370545661,12.3354177830535,
130.918672003733)) ;
#133785=CARTESIAN_POINT('Ctrl Pts',(-21.2662887681593,12.3682931650198,
131.189443526458)) ;
#133786=CARTESIAN_POINT('Ctrl Pts',(-21.3637199956931,12.4764500222757,
131.44102792815)) ;
#133787=CARTESIAN_POINT('Ctrl Pts',(-21.4490683123423,12.6527561756398,
131.657189302748)) ;
#133788=CARTESIAN_POINT('Ctrl Pts',(-21.5164968590452,12.8841372675975,
131.821041651181)) ;
#133789=CARTESIAN_POINT('Ctrl Pts',(-21.5620729321248,13.1550291136418,
131.920951331736)) ;
#133790=CARTESIAN_POINT('Ctrl Pts',(-21.5829990360394,13.4437302360126,
131.949026741888)) ;
#133791=CARTESIAN_POINT('Ctrl Pts',(-21.5787261653874,13.7319393007276,
131.903366364301)) ;
#133792=CARTESIAN_POINT('Ctrl Pts',(-21.5503975227815,13.9965481623833,
131.787623344815)) ;
#133793=CARTESIAN_POINT('Ctrl Pts',(-21.5005342471165,14.2215298170475,
131.608800269925)) ;
#133794=CARTESIAN_POINT('Ctrl Pts',(-21.4333938850247,14.3891483272759,
131.379489123203)) ;
#133795=CARTESIAN_POINT('Ctrl Pts',(-21.3548735774567,14.4871687024338,
131.117033634355)) ;
#133796=CARTESIAN_POINT('Ctrl Pts',(-21.2709428978837,14.5093408079897,
130.838711318976)) ;
#133797=CARTESIAN_POINT('Ctrl Pts',(-21.1882422406468,14.4530254583256,
130.563868416307)) ;
#133798=CARTESIAN_POINT('Ctrl Pts',(-21.1143270880585,14.3240305585518,
130.31499305445)) ;
#133799=CARTESIAN_POINT('Ctrl Pts',(-21.0539688868397,14.1290979717854,
130.105410602035)) ;
#133800=CARTESIAN_POINT('Ctrl Pts',(-21.0132069302916,13.8855604155571,
129.953378103653)) ;
#133801=CARTESIAN_POINT('Ctrl Pts',(-20.9950030451873,13.6058416707122,
129.866845755651)) ;
#133802=CARTESIAN_POINT('Ctrl Pts',(-21.0018793397198,13.3160021377259,
129.853947611582)) ;
#133803=CARTESIAN_POINT('Ctrl Pts',(-21.0337293398582,13.0326886676077,
129.913868033499)) ;
#133804=CARTESIAN_POINT('Ctrl Pts',(-21.0893772116349,12.7766372190837,
130.043216529831)) ;
#133805=CARTESIAN_POINT('Ctrl Pts',(-21.1653161877122,12.5676698161814,
130.231901557219)) ;
#133806=CARTESIAN_POINT('Ctrl Pts',(-21.2561790285771,12.4206517790888,
130.464404545457)) ;
#133807=CARTESIAN_POINT('Ctrl Pts',(-21.3575675366688,12.3443150505119,
130.727387699059)) ;
#133808=CARTESIAN_POINT('Ctrl Pts',(-21.4618210845223,12.3454567433165,
130.998884337509)) ;
#133809=CARTESIAN_POINT('Ctrl Pts',(-21.5631430702427,12.4241540146565,
131.261630006307)) ;
#133810=CARTESIAN_POINT('Ctrl Pts',(-21.6537810155053,12.5736454649868,
131.493407152973)) ;
#133811=CARTESIAN_POINT('Ctrl Pts',(-21.7290950924145,12.7844244258342,
131.680270904741)) ;
#133812=CARTESIAN_POINT('Ctrl Pts',(-21.7839298109933,13.041264478038,131.807295952736)) ;
#133813=CARTESIAN_POINT('Ctrl Pts',(-21.8150448539116,13.3250313838274,
131.865081031141)) ;
#133814=CARTESIAN_POINT('Ctrl Pts',(-21.8210632536644,13.6156492492809,
131.849571033927)) ;
#133815=CARTESIAN_POINT('Ctrl Pts',(-21.8022545212773,13.8929002803611,
131.761487721122)) ;
#133816=CARTESIAN_POINT('Ctrl Pts',(-21.7605924585031,14.1366366428793,
131.606614879296)) ;
#133817=CARTESIAN_POINT('Ctrl Pts',(-21.6999698317163,14.3287833833703,
131.396421302764)) ;
#133818=CARTESIAN_POINT('Ctrl Pts',(-21.6253197774301,14.4563288342089,
131.145218098165)) ;
#133819=CARTESIAN_POINT('Ctrl Pts',(-21.5425945750513,14.5097636463918,
130.870367772935)) ;
#133820=CARTESIAN_POINT('Ctrl Pts',(-21.4589621479375,14.4852491819093,
130.593003563587)) ;
#133821=CARTESIAN_POINT('Ctrl Pts',(-21.380714091029,14.385213180382,130.331360934625)) ;
#133822=CARTESIAN_POINT('Ctrl Pts',(-21.3138290434139,14.2148994362801,
130.102677640231)) ;
#133823=CARTESIAN_POINT('Ctrl Pts',(-21.264802027938,13.9895605141043,129.92646714371)) ;
#133824=CARTESIAN_POINT('Ctrl Pts',(-21.2370048320792,13.7226496289756,
129.812102485109)) ;
#133825=CARTESIAN_POINT('Ctrl Pts',(-21.2336042417307,13.4342098859693,
129.769013814372)) ;
#133826=CARTESIAN_POINT('Ctrl Pts',(-21.2553236046358,13.1458182759752,
129.799407215841)) ;
#133827=CARTESIAN_POINT('Ctrl Pts',(-21.3016988392798,12.8759127132536,
129.901648132077)) ;
#133828=CARTESIAN_POINT('Ctrl Pts',(-21.3694669987003,12.6468868556867,
130.066623481143)) ;
#133829=CARTESIAN_POINT('Ctrl Pts',(-21.4553373193102,12.4721832296684,
130.284273605613)) ;
#133830=CARTESIAN_POINT('Ctrl Pts',(-21.5530256217249,12.3661739274481,
130.536616813639)) ;
#133831=CARTESIAN_POINT('Ctrl Pts',(-21.6575177270796,12.3355863385396,
130.808562220896)) ;
#133832=CARTESIAN_POINT('Ctrl Pts',(-21.7604456918656,12.3831198658751,
131.076206190241)) ;
#133833=CARTESIAN_POINT('Ctrl Pts',(-21.8563696469902,12.5053833023315,
131.323242388746)) ;
#133834=CARTESIAN_POINT('Ctrl Pts',(-21.9382966693068,12.6923270702948,
131.529584453516)) ;
#133835=CARTESIAN_POINT('Ctrl Pts',(-22.0021645015312,12.9335865705139,
131.682862448256)) ;
#133836=CARTESIAN_POINT('Ctrl Pts',(-22.0430213128192,13.2085814539572,
131.769129801508)) ;
#133837=CARTESIAN_POINT('Ctrl Pts',(-22.0592352836556,13.4990557588074,
131.783380739882)) ;
#133838=CARTESIAN_POINT('Ctrl Pts',(-22.0503004073671,13.7836907462661,
131.724216167399)) ;
#133839=CARTESIAN_POINT('Ctrl Pts',(-22.0176371901026,14.0427281414566,
131.595717480909)) ;
#133840=CARTESIAN_POINT('Ctrl Pts',(-21.9641995370827,14.2577309750281,
131.406490661624)) ;
#133841=CARTESIAN_POINT('Ctrl Pts',(-21.8944782363852,14.4131664617501,
131.169654967239)) ;
#133842=CARTESIAN_POINT('Ctrl Pts',(-21.8141620072022,14.4973755702956,
130.901832610092)) ;
#133843=CARTESIAN_POINT('Ctrl Pts',(-21.7303937720881,14.5046724130054,
130.624142862364)) ;
#133844=CARTESIAN_POINT('Ctrl Pts',(-21.6486693225774,14.4343111747756,
130.352140919931)) ;
#133845=CARTESIAN_POINT('Ctrl Pts',(-21.5766530687314,14.2913904033354,
130.108640611113)) ;
#133846=CARTESIAN_POINT('Ctrl Pts',(-21.5199914526865,14.0872940403586,
129.910112364196)) ;
#133847=CARTESIAN_POINT('Ctrl Pts',(-21.4830382408884,13.8349907742835,
129.769035274606)) ;
#133848=CARTESIAN_POINT('Ctrl Pts',(-21.4694985396213,13.5522018199285,
129.696252361388)) ;
#133849=CARTESIAN_POINT('Ctrl Pts',(-21.4810885813508,13.2611771320633,
129.697002826515)) ;
#133850=CARTESIAN_POINT('Ctrl Pts',(-21.5176805732444,12.9814107201437,
129.770743949859)) ;
#133851=CARTESIAN_POINT('Ctrl Pts',(-21.5771191123903,12.7341369610279,
129.911345858839)) ;
#133852=CARTESIAN_POINT('Ctrl Pts',(-21.6563209788842,12.535166216503,130.109544290444)) ;
#133853=CARTESIAN_POINT('Ctrl Pts',(-21.7502713534583,12.4000170891871,
130.350799701057)) ;
#133854=CARTESIAN_POINT('Ctrl Pts',(-21.8524815344102,12.3385941106561,
130.616296707476)) ;
#133855=CARTESIAN_POINT('Ctrl Pts',(-21.9565712501459,12.3545286685026,
130.887315313701)) ;
#133856=CARTESIAN_POINT('Ctrl Pts',(-22.0562577481496,12.4469846430608,
131.14537139149)) ;
#133857=CARTESIAN_POINT('Ctrl Pts',(-22.1449360417052,12.6102579412087,
131.371180205731)) ;
#133858=CARTESIAN_POINT('Ctrl Pts',(-22.2161370464207,12.8296977311719,
131.546256445573)) ;
#133859=CARTESIAN_POINT('Ctrl Pts',(-22.2667592690025,13.0929763552362,
131.660982603106)) ;
#133860=CARTESIAN_POINT('Ctrl Pts',(-22.2932535098378,13.3798715107165,
131.705248169509)) ;
#133861=CARTESIAN_POINT('Ctrl Pts',(-22.2944576782056,13.6705227535771,
131.675549761758)) ;
#133862=CARTESIAN_POINT('Ctrl Pts',(-22.2711545117995,13.9421700423004,
131.57442408932)) ;
#133863=CARTESIAN_POINT('Ctrl Pts',(-22.2253820822901,14.1780191011813,
131.407446635602)) ;
#133864=CARTESIAN_POINT('Ctrl Pts',(-22.1619741826909,14.3579768124892,
131.189272795754)) ;
#133865=CARTESIAN_POINT('Ctrl Pts',(-22.0850483275451,14.4725057553617,
130.931291857228)) ;
#133866=CARTESIAN_POINT('Ctrl Pts',(-22.0018889458697,14.5110248787396,
130.655306915796)) ;
#133867=CARTESIAN_POINT('Ctrl Pts',(-21.9186831269904,14.4721191969269,
130.37915685792)) ;
#133868=CARTESIAN_POINT('Ctrl Pts',(-21.8419983594231,14.3577454336847,
130.121978165508)) ;
#133869=CARTESIAN_POINT('Ctrl Pts',(-21.7784559689967,14.1770688666527,
129.90331119887)) ;
#133870=CARTESIAN_POINT('Ctrl Pts',(-21.7328730623761,13.9416997327419,
129.73698112711)) ;
#133871=CARTESIAN_POINT('Ctrl Pts',(-21.7095937547817,13.6694104353782,
129.635852457523)) ;
#133872=CARTESIAN_POINT('Ctrl Pts',(-21.7108544164153,13.3798585935035,
129.60644988842)) ;
#133873=CARTESIAN_POINT('Ctrl Pts',(-21.7373587408651,13.0927640382574,
129.650717582232)) ;
#133874=CARTESIAN_POINT('Ctrl Pts',(-21.7879727694938,12.8294542733058,
129.765423278)) ;
#133875=CARTESIAN_POINT('Ctrl Pts',(-21.8596572059499,12.6090080043084,
129.941724810289)) ;
#133876=CARTESIAN_POINT('Ctrl Pts',(-21.9481186483126,12.4466659582347,
130.167016290758)) ;
#133877=CARTESIAN_POINT('Ctrl Pts',(-22.0478029406896,12.3544265354386,
130.425067159699)) ;
#133878=CARTESIAN_POINT('Ctrl Pts',(-22.1517530143636,12.338485550426,130.695728652991)) ;
#133879=CARTESIAN_POINT('Ctrl Pts',(-22.2547791723717,12.4009576070215,
130.963329774343)) ;
#133880=CARTESIAN_POINT('Ctrl Pts',(-22.3479076849026,12.5356622675021,
131.202441690569)) ;
#133881=CARTESIAN_POINT('Ctrl Pts',(-22.427039674185,12.7342792931547,131.400473047047)) ;
#133882=CARTESIAN_POINT('Ctrl Pts',(-22.4865817751364,12.9822470405306,
131.541298758196)) ;
#133883=CARTESIAN_POINT('Ctrl Pts',(-22.5231351067208,13.2626104241267,
131.614868935857)) ;
#133884=CARTESIAN_POINT('Ctrl Pts',(-22.5345613145019,13.5537330357078,
131.615129217148)) ;
#133885=CARTESIAN_POINT('Ctrl Pts',(-22.5210072175352,13.8350780443648,
131.542464925158)) ;
#133886=CARTESIAN_POINT('Ctrl Pts',(-22.4841282635127,14.0872562376869,
131.401629162015)) ;
#133887=CARTESIAN_POINT('Ctrl Pts',(-22.4271936380161,14.2922552735091,
131.202157542)) ;
#133888=CARTESIAN_POINT('Ctrl Pts',(-22.3548468095764,14.4349645919609,
130.957589374496)) ;
#133889=CARTESIAN_POINT('Ctrl Pts',(-22.2738049730186,14.5045540577175,
130.687866104784)) ;
#133890=CARTESIAN_POINT('Ctrl Pts',(-22.1896316409164,14.4973581396257,
130.408831550043)) ;
#133891=CARTESIAN_POINT('Ctrl Pts',(-22.1093343470203,14.4126016842873,
130.14105358009)) ;
#133892=CARTESIAN_POINT('Ctrl Pts',(-22.0399356599868,14.2578370889756,
129.905309744937)) ;
#133893=CARTESIAN_POINT('Ctrl Pts',(-21.9863765422796,14.0423606370671,
129.715650705837)) ;
#133894=CARTESIAN_POINT('Ctrl Pts',(-21.9537345461485,13.7833430848993,
129.58722594006)) ;
#133895=CARTESIAN_POINT('Ctrl Pts',(-21.9448743026681,13.4972454461382,
129.528113894271)) ;
#133896=CARTESIAN_POINT('Ctrl Pts',(-21.960316850898,13.2225256872019,129.541910774833)) ;
#133897=CARTESIAN_POINT('Ctrl Pts',(-21.984463817368,13.0520853568101,129.592017243009)) ;
#133898=CARTESIAN_POINT('Ctrl Pts',(-21.9982570673691,12.9778651918053,
129.622952131535)) ;
#133899=CARTESIAN_POINT('',(-11.3761033793275,13.1734341962953,133.269779676638)) ;
#133900=CARTESIAN_POINT('Origin',(-11.3525470049302,13.1551399285885,133.200965310447)) ;
#133901=CARTESIAN_POINT('',(-11.3289906305328,13.1368456608817,133.132150944256)) ;
#133902=CARTESIAN_POINT('Origin',(-11.3525470049302,13.1551399285885,133.200965310447)) ;
#133903=CARTESIAN_POINT('Origin',(-11.3525470049302,13.1551399285885,133.200965310447)) ;
#133904=CARTESIAN_POINT('',(-22.3151378869403,14.5729486686832,130.548644361977)) ;
#133905=CARTESIAN_POINT('Ctrl Pts',(-22.3151379480645,14.5729486667267,
130.548644337297)) ;
#133906=CARTESIAN_POINT('Ctrl Pts',(-22.3011761799316,14.5730368300439,
130.507858330238)) ;
#133907=CARTESIAN_POINT('Ctrl Pts',(-22.287200210088,14.5706665958407,130.467031058799)) ;
#133908=CARTESIAN_POINT('Ctrl Pts',(-22.2733078271729,14.5658273790944,
130.42644775387)) ;
#133909=CARTESIAN_POINT('Ctrl Pts',(-22.2675381995131,14.5638176102188,
130.409593153758)) ;
#133910=CARTESIAN_POINT('Ctrl Pts',(-22.2617824711753,14.5613818550179,
130.392779157221)) ;
#133911=CARTESIAN_POINT('Ctrl Pts',(-22.2560476493669,14.5585193175848,
130.376026234156)) ;
#133912=CARTESIAN_POINT('Ctrl Pts',(-22.2292231059487,14.545129841464,130.297664686553)) ;
#133913=CARTESIAN_POINT('Ctrl Pts',(-22.2028658648278,14.5224036480338,
130.220668467657)) ;
#133914=CARTESIAN_POINT('Ctrl Pts',(-22.1776957713426,14.4911112211587,
130.147139851903)) ;
#133915=CARTESIAN_POINT('Ctrl Pts',(-22.1719521385364,14.4839705162705,
130.130361154999)) ;
#133916=CARTESIAN_POINT('Ctrl Pts',(-22.166270291937,14.4763839522868,130.113762956894)) ;
#133917=CARTESIAN_POINT('Ctrl Pts',(-22.1606587249298,14.4683610330769,
130.097370093526)) ;
#133918=CARTESIAN_POINT('Ctrl Pts',(-22.1355483985991,14.4324605227158,
130.024016224965)) ;
#133919=CARTESIAN_POINT('Ctrl Pts',(-22.1118463317427,14.3878194900747,
129.954775802407)) ;
#133920=CARTESIAN_POINT('Ctrl Pts',(-22.0900768461573,14.3354941538269,
129.891181728977)) ;
#133921=CARTESIAN_POINT('Ctrl Pts',(-22.0856561856623,14.3248686135067,
129.878267881885)) ;
#133922=CARTESIAN_POINT('Ctrl Pts',(-22.0813151982726,14.3139263466192,
129.865586780601)) ;
#133923=CARTESIAN_POINT('Ctrl Pts',(-22.0770582501623,14.3026764237554,
129.853151115368)) ;
#133924=CARTESIAN_POINT('Ctrl Pts',(-22.0575007470533,14.2509914147575,
129.796018504125)) ;
#133925=CARTESIAN_POINT('Ctrl Pts',(-22.0397191593872,14.1928134151899,
129.744072096327)) ;
#133926=CARTESIAN_POINT('Ctrl Pts',(-22.0241540809177,14.1296950731463,
129.698603459873)) ;
#133927=CARTESIAN_POINT('Ctrl Pts',(-22.0196338868241,14.1113651201392,
129.685399089439)) ;
#133928=CARTESIAN_POINT('Ctrl Pts',(-22.015300592828,14.0926186905485,129.672740752753)) ;
#133929=CARTESIAN_POINT('Ctrl Pts',(-22.0111649071197,14.0734942173741,
129.660659326894)) ;
#133930=CARTESIAN_POINT('Ctrl Pts',(-21.9979065378246,14.0121841116736,
129.621928142528)) ;
#133931=CARTESIAN_POINT('Ctrl Pts',(-21.9866821734794,13.9469968841568,
129.589133277344)) ;
#133932=CARTESIAN_POINT('Ctrl Pts',(-21.977674302844,13.8791719111513,129.562821710652)) ;
#133933=CARTESIAN_POINT('Ctrl Pts',(-21.9741790940785,13.8528546548578,
129.552612370148)) ;
#133934=CARTESIAN_POINT('Ctrl Pts',(-21.9710176873156,13.8261405468838,
129.543378736997)) ;
#133935=CARTESIAN_POINT('Ctrl Pts',(-21.9682011481905,13.799103138409,129.535150885313)) ;
#133936=CARTESIAN_POINT('Ctrl Pts',(-21.9656494606323,13.774608176419,129.527696734726)) ;
#133937=CARTESIAN_POINT('Ctrl Pts',(-21.9633468396246,13.7495103406013,
129.520970042987)) ;
#133938=CARTESIAN_POINT('Ctrl Pts',(-21.961330695701,13.7240463055939,129.515080342888)) ;
#133939=CARTESIAN_POINT('Ctrl Pts',(-21.9593134014791,13.6985677422408,
129.509187282458)) ;
#133940=CARTESIAN_POINT('Ctrl Pts',(-21.9575829900595,13.6727232379291,
129.504132378895)) ;
#133941=CARTESIAN_POINT('Ctrl Pts',(-21.9561611043169,13.6467675495469,
129.49997876671)) ;
#133942=CARTESIAN_POINT('Ctrl Pts',(-21.9547385696093,13.6208000146897,
129.495823258767)) ;
#133943=CARTESIAN_POINT('Ctrl Pts',(-21.953624881802,13.5947219208531,129.492569954795)) ;
#133944=CARTESIAN_POINT('Ctrl Pts',(-21.9528249799405,13.5687954659883,
129.490233200648)) ;
#133945=CARTESIAN_POINT('Ctrl Pts',(-21.9521162979408,13.545825633356,129.488162927178)) ;
#133946=CARTESIAN_POINT('Ctrl Pts',(-21.9516536736589,13.5229752443421,
129.486811359342)) ;
#133947=CARTESIAN_POINT('Ctrl Pts',(-21.9514293963157,13.5004244329661,
129.486156186226)) ;
#133948=CARTESIAN_POINT('Ctrl Pts',(-21.9512381070114,13.481190528375,129.485597379848)) ;
#133949=CARTESIAN_POINT('Ctrl Pts',(-21.9512130944036,13.4613698797395,
129.485523580215)) ;
#133950=CARTESIAN_POINT('Ctrl Pts',(-21.9513804892,13.4412408608151,129.486012294124)) ;
#133951=CARTESIAN_POINT('Ctrl Pts',(-21.9515476082074,13.421145005191,129.48650020286)) ;
#133952=CARTESIAN_POINT('Ctrl Pts',(-21.9519065972143,13.4007422200765,
129.48754900886)) ;
#133953=CARTESIAN_POINT('Ctrl Pts',(-21.9524666030812,13.3803126577523,
129.489185369577)) ;
#133954=CARTESIAN_POINT('Ctrl Pts',(-21.9530180572326,13.3601950703844,
129.490796741821)) ;
#133955=CARTESIAN_POINT('Ctrl Pts',(-21.9537644170884,13.3400519549877,
129.492977752401)) ;
#133956=CARTESIAN_POINT('Ctrl Pts',(-21.9546975614041,13.3201474123098,
129.49570416507)) ;
#133957=CARTESIAN_POINT('Ctrl Pts',(-21.9556524119253,13.2997798629067,
129.498493997805)) ;
#133958=CARTESIAN_POINT('Ctrl Pts',(-21.9568028587807,13.2796626021651,
129.501854897454)) ;
#133959=CARTESIAN_POINT('Ctrl Pts',(-21.9581222304844,13.2600678710264,
129.505708828523)) ;
#133960=CARTESIAN_POINT('Ctrl Pts',(-21.9594416021881,13.2404731398877,
129.509562759592)) ;
#133961=CARTESIAN_POINT('Ctrl Pts',(-21.960929776014,13.2214012994025,129.513909294428)) ;
#133962=CARTESIAN_POINT('Ctrl Pts',(-21.96254318369,13.2031075416911,129.518622482662)) ;
#133963=CARTESIAN_POINT('Ctrl Pts',(-21.963701302918,13.1899761100796,129.522005653574)) ;
#133964=CARTESIAN_POINT('Ctrl Pts',(-21.9649923328492,13.1764783865927,
129.525776897949)) ;
#133965=CARTESIAN_POINT('Ctrl Pts',(-21.9663999656187,13.1629676618293,
129.529889010867)) ;
#133966=CARTESIAN_POINT('Ctrl Pts',(-21.9678179998417,13.1493571019527,
129.534031509516)) ;
#133967=CARTESIAN_POINT('Ctrl Pts',(-21.9693544131974,13.1357338594016,
129.53851997682)) ;
#133968=CARTESIAN_POINT('Ctrl Pts',(-21.9709759033026,13.1224444824642,
129.543256827227)) ;
#133969=CARTESIAN_POINT('Ctrl Pts',(-21.9725973934077,13.1091551055269,
129.547993677634)) ;
#133970=CARTESIAN_POINT('Ctrl Pts',(-21.9743038518766,13.096199960817,129.552978488115)) ;
#133971=CARTESIAN_POINT('Ctrl Pts',(-21.976045911875,13.0839043074199,129.558067503624)) ;
#133972=CARTESIAN_POINT('Ctrl Pts',(-21.9773237439476,13.0748852264019,
129.561800387246)) ;
#133973=CARTESIAN_POINT('Ctrl Pts',(-21.9787131003971,13.065573564542,129.565858984562)) ;
#133974=CARTESIAN_POINT('Ctrl Pts',(-21.9801662380091,13.056419673348,129.570104049804)) ;
#133975=CARTESIAN_POINT('Ctrl Pts',(-21.9816281570041,13.0472104647332,
129.574374768186)) ;
#133976=CARTESIAN_POINT('Ctrl Pts',(-21.9831546331542,13.0381613456531,
129.578833998246)) ;
#133977=CARTESIAN_POINT('Ctrl Pts',(-21.984681663157,13.0297062023895,129.583294812552)) ;
#133978=CARTESIAN_POINT('Ctrl Pts',(-21.9848487129258,13.0287812502109,
129.583782804272)) ;
#133979=CARTESIAN_POINT('Ctrl Pts',(-21.9850157546884,13.0278633792237,
129.584270774027)) ;
#133980=CARTESIAN_POINT('Ctrl Pts',(-21.9851826941415,13.0269531373025,
129.584758448084)) ;
#133981=CARTESIAN_POINT('Ctrl Pts',(-21.9863339740107,13.0206757524139,
129.588121639429)) ;
#133982=CARTESIAN_POINT('Ctrl Pts',(-21.9875828769642,13.0142106156177,
129.591770024712)) ;
#133983=CARTESIAN_POINT('Ctrl Pts',(-21.9888478967941,13.008138163139,129.595465492)) ;
#133984=CARTESIAN_POINT('Ctrl Pts',(-21.989454280972,13.0052273478162,129.597236905255)) ;
#133985=CARTESIAN_POINT('Ctrl Pts',(-21.990064156824,13.0024063418278,129.599018484663)) ;
#133986=CARTESIAN_POINT('Ctrl Pts',(-21.9906674065461,12.9997366350286,
129.600780735788)) ;
#133987=CARTESIAN_POINT('Ctrl Pts',(-21.9916964541652,12.9951825418823,
129.603786854577)) ;
#133988=CARTESIAN_POINT('Ctrl Pts',(-21.9928080155907,12.9906247701674,
129.607034017901)) ;
#133989=CARTESIAN_POINT('Ctrl Pts',(-21.9938748908751,12.9868577736952,
129.610150641252)) ;
#133990=CARTESIAN_POINT('Ctrl Pts',(-21.9945019204265,12.984643814723,129.611982359513)) ;
#133991=CARTESIAN_POINT('Ctrl Pts',(-21.995149121453,12.9825760105869,129.613873003867)) ;
#133992=CARTESIAN_POINT('Ctrl Pts',(-21.9957649760313,12.9809630503241,
129.615672077092)) ;
#133993=CARTESIAN_POINT('Ctrl Pts',(-21.996719473855,12.9784631629888,129.618460416319)) ;
#133994=CARTESIAN_POINT('Ctrl Pts',(-21.997623841344,12.9769886520828,129.621102311744)) ;
#133995=CARTESIAN_POINT('Ctrl Pts',(-21.9982570673691,12.9778651918053,
129.622952131536)) ;
#133996=CARTESIAN_POINT('',(-22.3151378869403,14.423223846854,130.548644361977)) ;
#133997=CARTESIAN_POINT('Ctrl Pts',(-22.3151378869416,14.5729486706397,
130.548644361981)) ;
#133998=CARTESIAN_POINT('Ctrl Pts',(-22.3536131995393,14.5727057162824,
130.661040871128)) ;
#133999=CARTESIAN_POINT('Ctrl Pts',(-22.3917725975218,14.5537967295509,
130.772514510611)) ;
#134000=CARTESIAN_POINT('Ctrl Pts',(-22.4651692698086,14.4793817119497,
130.986925497581)) ;
#134001=CARTESIAN_POINT('Ctrl Pts',(-22.4997692262472,14.4241005029474,
131.088001071933)) ;
#134002=CARTESIAN_POINT('Ctrl Pts',(-22.5689108472644,14.2666151380171,
131.289981934841)) ;
#134003=CARTESIAN_POINT('Ctrl Pts',(-22.6011767967328,14.1573235247065,
131.38423926092)) ;
#134004=CARTESIAN_POINT('Ctrl Pts',(-22.6488987494123,13.9114366623006,
131.523647638104)) ;
#134005=CARTESIAN_POINT('Ctrl Pts',(-22.6645996619435,13.7782522629318,
131.569514133756)) ;
#134006=CARTESIAN_POINT('Ctrl Pts',(-22.6786331937249,13.4898377655437,
131.610509771653)) ;
#134007=CARTESIAN_POINT('Ctrl Pts',(-22.6736768274188,13.3672753503854,
131.596030921988)) ;
#134008=CARTESIAN_POINT('Ctrl Pts',(-22.6651145627851,13.2574016528032,
131.571018294663)) ;
#134009=CARTESIAN_POINT('Ctrl Pts',(-22.6619233775539,13.2306316253481,
131.561696003049)) ;
#134010=CARTESIAN_POINT('Ctrl Pts',(-22.658869062641,13.2145328967425,131.552773545741)) ;
#134011=CARTESIAN_POINT('Ctrl Pts',(-22.658166921974,13.2113394407781,131.550722408079)) ;
#134012=CARTESIAN_POINT('Ctrl Pts',(-22.6572747831006,13.2091027938622,
131.54811623575)) ;
#134013=CARTESIAN_POINT('Ctrl Pts',(-22.6570602137521,13.2086648958779,
131.547489422314)) ;
#134014=CARTESIAN_POINT('Ctrl Pts',(-22.6566971522605,13.2082608228121,
131.546428824192)) ;
#134015=CARTESIAN_POINT('Ctrl Pts',(-22.6565542868357,13.2081743378001,
131.546011476705)) ;
#134016=CARTESIAN_POINT('Ctrl Pts',(-22.6562872703243,13.2082090859895,
131.545231451236)) ;
#134017=CARTESIAN_POINT('Ctrl Pts',(-22.656171236643,13.2082979781244,131.54489248633)) ;
#134018=CARTESIAN_POINT('Ctrl Pts',(-22.6559368182774,13.2086342290079,
131.54420768862)) ;
#134019=CARTESIAN_POINT('Ctrl Pts',(-22.6558268749173,13.2088894196119,
131.543886515144)) ;
#134020=CARTESIAN_POINT('Ctrl Pts',(-22.6555685283304,13.2096748296436,
131.543131816805)) ;
#134021=CARTESIAN_POINT('Ctrl Pts',(-22.6554365161173,13.2102931177128,
131.542746174404)) ;
#134022=CARTESIAN_POINT('Ctrl Pts',(-22.6550858617799,13.2123135011588,
131.541721820844)) ;
#134023=CARTESIAN_POINT('Ctrl Pts',(-22.6549030747436,13.2141115604459,
131.541187851828)) ;
#134024=CARTESIAN_POINT('Ctrl Pts',(-22.6543256425256,13.2215607234665,
131.539501020424)) ;
#134025=CARTESIAN_POINT('Ctrl Pts',(-22.6541135690987,13.2297469423957,
131.538881498157)) ;
#134026=CARTESIAN_POINT('Ctrl Pts',(-22.6532410800261,13.2936995343114,
131.536332728065)) ;
#134027=CARTESIAN_POINT('Ctrl Pts',(-22.6556996367525,13.4112788385444,
131.543514818452)) ;
#134028=CARTESIAN_POINT('Ctrl Pts',(-22.6382336783187,13.6947112909237,
131.492492159393)) ;
#134029=CARTESIAN_POINT('Ctrl Pts',(-22.6221628124986,13.8232128942525,
131.445544933384)) ;
#134030=CARTESIAN_POINT('Ctrl Pts',(-22.5744365803075,14.0563340831041,
131.306124054621)) ;
#134031=CARTESIAN_POINT('Ctrl Pts',(-22.5435243363485,14.1569964530154,
131.21582125845)) ;
#134032=CARTESIAN_POINT('Ctrl Pts',(-22.4791435871951,14.2967160993782,
131.027748154618)) ;
#134033=CARTESIAN_POINT('Ctrl Pts',(-22.4480466097423,14.3443721936477,
130.936905703363)) ;
#134034=CARTESIAN_POINT('Ctrl Pts',(-22.3828566010413,14.4076338778508,
130.746468539515)) ;
#134035=CARTESIAN_POINT('Ctrl Pts',(-22.3491318413627,14.4234782772114,
130.647949645059)) ;
#134036=CARTESIAN_POINT('Ctrl Pts',(-22.3151378869407,14.4232238463042,
130.548644361978)) ;
#134037=CARTESIAN_POINT('Ctrl Pts',(-21.9982570673691,12.9778651918053,
129.622952131535)) ;
#134038=CARTESIAN_POINT('Ctrl Pts',(-21.9983740357125,12.9780271046061,
129.623293826836)) ;
#134039=CARTESIAN_POINT('Ctrl Pts',(-21.9984729623435,12.9782537499198,
129.623582817547)) ;
#134040=CARTESIAN_POINT('Ctrl Pts',(-21.9986619517152,12.9788663176289,
129.624134905217)) ;
#134041=CARTESIAN_POINT('Ctrl Pts',(-21.9987422359044,12.9792529318713,
129.624369436452)) ;
#134042=CARTESIAN_POINT('Ctrl Pts',(-21.9989688888416,12.9806654239707,
129.625031549303)) ;
#134043=CARTESIAN_POINT('Ctrl Pts',(-21.9990592680355,12.9819390751646,
129.625295570703)) ;
#134044=CARTESIAN_POINT('Ctrl Pts',(-21.9992344695967,12.9863682734796,
129.625807380551)) ;
#134045=CARTESIAN_POINT('Ctrl Pts',(-21.9991646228976,12.9906967702327,
129.62560333997)) ;
#134046=CARTESIAN_POINT('Ctrl Pts',(-21.998493398505,13.0076193276443,129.623642516951)) ;
#134047=CARTESIAN_POINT('Ctrl Pts',(-21.9973112343386,13.024361696837,129.620189104446)) ;
#134048=CARTESIAN_POINT('Ctrl Pts',(-21.9922385267737,13.093661183053,129.605370391257)) ;
#134049=CARTESIAN_POINT('Ctrl Pts',(-21.9869683786663,13.1624395523346,
129.58997490231)) ;
#134050=CARTESIAN_POINT('Ctrl Pts',(-21.9792387916176,13.3897587207603,
129.567394745249)) ;
#134051=CARTESIAN_POINT('Ctrl Pts',(-21.9832458177027,13.5079529375974,
129.579100322505)) ;
#134052=CARTESIAN_POINT('Ctrl Pts',(-21.9990289638202,13.7299217778491,
129.625207044119)) ;
#134053=CARTESIAN_POINT('Ctrl Pts',(-22.0148314797799,13.8477898854171,
129.671370350136)) ;
#134054=CARTESIAN_POINT('Ctrl Pts',(-22.0613345650186,14.0688613754809,
129.807218094897)) ;
#134055=CARTESIAN_POINT('Ctrl Pts',(-22.0926080464121,14.1680229125909,
129.898576160635)) ;
#134056=CARTESIAN_POINT('Ctrl Pts',(-22.1569266233532,14.3035692712769,
130.08646764308)) ;
#134057=CARTESIAN_POINT('Ctrl Pts',(-22.1873142259314,14.3485547863788,
130.175237823827)) ;
#134058=CARTESIAN_POINT('Ctrl Pts',(-22.2505095483839,14.4080651754862,
130.359847984435)) ;
#134059=CARTESIAN_POINT('Ctrl Pts',(-22.282659459403,14.4229807584986,130.45376633159)) ;
#134060=CARTESIAN_POINT('Ctrl Pts',(-22.3151378869407,14.4232238463042,
130.548644361978)) ;
#134061=CARTESIAN_POINT('Ctrl Pts',(-11.2812798643659,13.1551399285885,
133.225361312885)) ;
#134062=CARTESIAN_POINT('Ctrl Pts',(-11.3048362387632,13.1734341962953,
133.294175679076)) ;
#134063=CARTESIAN_POINT('Ctrl Pts',(-11.3761033793275,13.1734341962953,
133.269779676638)) ;
#134064=CARTESIAN_POINT('Ctrl Pts',(-11.4473705198918,13.1734341962953,
133.2453836742)) ;
#134065=CARTESIAN_POINT('Ctrl Pts',(-11.4238141454945,13.1551399285885,
133.176569308009)) ;
#134066=CARTESIAN_POINT('Ctrl Pts',(-11.4002577710971,13.1368456608817,
133.107754941818)) ;
#134067=CARTESIAN_POINT('Ctrl Pts',(-11.3289906305328,13.1368456608817,
133.132150944256)) ;
#134068=CARTESIAN_POINT('Ctrl Pts',(-11.2577234899685,13.1368456608817,
133.156546946693)) ;
#134069=CARTESIAN_POINT('Ctrl Pts',(-11.2812798643659,13.1551399285885,
133.225361312885)) ;
#134070=CARTESIAN_POINT('Ctrl Pts',(-11.2798493008599,13.191264605624,133.215535474837)) ;
#134071=CARTESIAN_POINT('Ctrl Pts',(-11.3038195704943,13.1991216594078,
133.286995970946)) ;
#134072=CARTESIAN_POINT('Ctrl Pts',(-11.3749383182286,13.2028260557706,
133.262162005045)) ;
#134073=CARTESIAN_POINT('Ctrl Pts',(-11.4460570659629,13.2065304521335,
133.237328039145)) ;
#134074=CARTESIAN_POINT('Ctrl Pts',(-11.4220867963285,13.1986733983497,
133.165867543036)) ;
#134075=CARTESIAN_POINT('Ctrl Pts',(-11.398116526694,13.1908163445659,133.094407046927)) ;
#134076=CARTESIAN_POINT('Ctrl Pts',(-11.3269977789597,13.1871119482031,
133.119241012827)) ;
#134077=CARTESIAN_POINT('Ctrl Pts',(-11.2558790312254,13.1834075518402,
133.144074978727)) ;
#134078=CARTESIAN_POINT('Ctrl Pts',(-11.2798493008599,13.191264605624,133.215535474837)) ;
#134079=CARTESIAN_POINT('Ctrl Pts',(-11.27675499221,13.268036520819,133.2128184295)) ;
#134080=CARTESIAN_POINT('Ctrl Pts',(-11.3016167838991,13.2538025217343,
133.284678753642)) ;
#134081=CARTESIAN_POINT('Ctrl Pts',(-11.3724255895565,13.2651134066728,
133.260704367766)) ;
#134082=CARTESIAN_POINT('Ctrl Pts',(-11.4432343952138,13.2764242916113,
133.23672998189)) ;
#134083=CARTESIAN_POINT('Ctrl Pts',(-11.4183726035248,13.290658290696,133.164869657748)) ;
#134084=CARTESIAN_POINT('Ctrl Pts',(-11.3935108118358,13.3048922897807,
133.093009333607)) ;
#134085=CARTESIAN_POINT('Ctrl Pts',(-11.3227020061784,13.2935814048422,
133.116983719482)) ;
#134086=CARTESIAN_POINT('Ctrl Pts',(-11.251893200521,13.2822705199037,133.140958105358)) ;
#134087=CARTESIAN_POINT('Ctrl Pts',(-11.27675499221,13.268036520819,133.2128184295)) ;
#134088=CARTESIAN_POINT('Ctrl Pts',(-11.2723617392628,13.3732912215196,
133.259787303242)) ;
#134089=CARTESIAN_POINT('Ctrl Pts',(-11.298479063893,13.3290215614615,133.317617538259)) ;
#134090=CARTESIAN_POINT('Ctrl Pts',(-11.3688780671425,13.3500184403787,
133.299818088917)) ;
#134091=CARTESIAN_POINT('Ctrl Pts',(-11.439277070392,13.371015319296,133.282018639574)) ;
#134092=CARTESIAN_POINT('Ctrl Pts',(-11.4131597457618,13.4152849793541,
133.224188404558)) ;
#134093=CARTESIAN_POINT('Ctrl Pts',(-11.3870424211316,13.4595546394122,
133.166358169541)) ;
#134094=CARTESIAN_POINT('Ctrl Pts',(-11.3166434178821,13.4385577604949,
133.184157618883)) ;
#134095=CARTESIAN_POINT('Ctrl Pts',(-11.2462444146326,13.4175608815777,
133.201957068225)) ;
#134096=CARTESIAN_POINT('Ctrl Pts',(-11.2723617392628,13.3732912215196,
133.259787303242)) ;
#134097=CARTESIAN_POINT('Ctrl Pts',(-11.2691148403661,13.4471111688333,
133.348383186297)) ;
#134098=CARTESIAN_POINT('Ctrl Pts',(-11.2961492330365,13.3820520008154,
133.380368710749)) ;
#134099=CARTESIAN_POINT('Ctrl Pts',(-11.3662774333647,13.409026910249,133.37238538732)) ;
#134100=CARTESIAN_POINT('Ctrl Pts',(-11.436405633693,13.4360018196825,133.364402063892)) ;
#134101=CARTESIAN_POINT('Ctrl Pts',(-11.4093712410226,13.5010609877004,
133.33241653944)) ;
#134102=CARTESIAN_POINT('Ctrl Pts',(-11.3823368483522,13.5661201557183,
133.300431014988)) ;
#134103=CARTESIAN_POINT('Ctrl Pts',(-11.312208648024,13.5391452462847,133.308414338417)) ;
#134104=CARTESIAN_POINT('Ctrl Pts',(-11.2420804476957,13.5121703368512,
133.316397661845)) ;
#134105=CARTESIAN_POINT('Ctrl Pts',(-11.2691148403661,13.4471111688333,
133.348383186297)) ;
#134106=CARTESIAN_POINT('Ctrl Pts',(-11.26815235584,13.4654248347116,133.423083801914)) ;
#134107=CARTESIAN_POINT('Ctrl Pts',(-11.295448841143,13.3954694274565,133.433496373216)) ;
#134108=CARTESIAN_POINT('Ctrl Pts',(-11.3655255940352,13.4231551632892,
133.433144549366)) ;
#134109=CARTESIAN_POINT('Ctrl Pts',(-11.4356023469274,13.4508408991218,
133.432792725516)) ;
#134110=CARTESIAN_POINT('Ctrl Pts',(-11.4083058616244,13.5207963063769,
133.422380154214)) ;
#134111=CARTESIAN_POINT('Ctrl Pts',(-11.3810093763214,13.5907517136319,
133.411967582912)) ;
#134112=CARTESIAN_POINT('Ctrl Pts',(-11.3109326234292,13.5630659777992,
133.412319406762)) ;
#134113=CARTESIAN_POINT('Ctrl Pts',(-11.240855870537,13.5353802419666,133.412671230612)) ;
#134114=CARTESIAN_POINT('Ctrl Pts',(-11.26815235584,13.4654248347116,133.423083801914)) ;
#134115=CARTESIAN_POINT('Ctrl Pts',(-11.2680244517119,13.4658285122696,
133.460562426083)) ;
#134116=CARTESIAN_POINT('Ctrl Pts',(-11.2953502173512,13.3959427988304,
133.460195119767)) ;
#134117=CARTESIAN_POINT('Ctrl Pts',(-11.3654365304336,13.4231193515827,
133.463543154982)) ;
#134118=CARTESIAN_POINT('Ctrl Pts',(-11.435522843516,13.4502959043349,133.466891190198)) ;
#134119=CARTESIAN_POINT('Ctrl Pts',(-11.4081970778768,13.5201816177741,
133.467258496514)) ;
#134120=CARTESIAN_POINT('Ctrl Pts',(-11.3808713122375,13.5900673312133,
133.467625802831)) ;
#134121=CARTESIAN_POINT('Ctrl Pts',(-11.3107849991551,13.562890778461,133.464277767615)) ;
#134122=CARTESIAN_POINT('Ctrl Pts',(-11.2406986860726,13.5357142257088,
133.4609297324)) ;
#134123=CARTESIAN_POINT('Ctrl Pts',(-11.2680244517119,13.4658285122696,
133.460562426083)) ;
#134124=CARTESIAN_POINT('',(-11.2680244517119,13.4658285122696,133.460562426083)) ;
#134125=CARTESIAN_POINT('Ctrl Pts',(-11.2812798643659,13.1551399285885,
133.225361312885)) ;
#134126=CARTESIAN_POINT('Ctrl Pts',(-11.2798493008599,13.191264605624,133.215535474837)) ;
#134127=CARTESIAN_POINT('Ctrl Pts',(-11.27675499221,13.268036520819,133.2128184295)) ;
#134128=CARTESIAN_POINT('Ctrl Pts',(-11.2723617392628,13.3732912215196,
133.259787303242)) ;
#134129=CARTESIAN_POINT('Ctrl Pts',(-11.2691148403661,13.4471111688333,
133.348383186297)) ;
#134130=CARTESIAN_POINT('Ctrl Pts',(-11.26815235584,13.4654248347116,133.423083801914)) ;
#134131=CARTESIAN_POINT('Ctrl Pts',(-11.2680244517119,13.4658285122696,
133.460562426083)) ;
#134132=CARTESIAN_POINT('Origin',(-11.3381107647943,13.4930050650219,133.463910461299)) ;
#134133=CARTESIAN_POINT('Ctrl Pts',(-11.2680244517119,13.4658285122696,
133.460562426083)) ;
#134134=CARTESIAN_POINT('Ctrl Pts',(-11.2953502173512,13.3959427988304,
133.460195119767)) ;
#134135=CARTESIAN_POINT('Ctrl Pts',(-11.3654365304336,13.4231193515827,
133.463543154982)) ;
#134136=CARTESIAN_POINT('Ctrl Pts',(-11.435522843516,13.4502959043349,133.466891190198)) ;
#134137=CARTESIAN_POINT('Ctrl Pts',(-11.4081970778768,13.5201816177741,
133.467258496514)) ;
#134138=CARTESIAN_POINT('Ctrl Pts',(-11.3808713122375,13.5900673312133,
133.467625802831)) ;
#134139=CARTESIAN_POINT('Ctrl Pts',(-11.3107849991551,13.562890778461,133.464277767615)) ;
#134140=CARTESIAN_POINT('Ctrl Pts',(-11.2406986860726,13.5357142257088,
133.4609297324)) ;
#134141=CARTESIAN_POINT('Ctrl Pts',(-11.2680244517119,13.4658285122696,
133.460562426083)) ;
#134142=CARTESIAN_POINT('Ctrl Pts',(-11.2668676693348,13.4658294080177,
133.842542306898)) ;
#134143=CARTESIAN_POINT('Ctrl Pts',(-11.294193434974,13.3959436945786,133.842175000581)) ;
#134144=CARTESIAN_POINT('Ctrl Pts',(-11.3642797480564,13.4231202473308,
133.845523035796)) ;
#134145=CARTESIAN_POINT('Ctrl Pts',(-11.4343660611389,13.4502968000831,
133.848871071012)) ;
#134146=CARTESIAN_POINT('Ctrl Pts',(-11.4070402954996,13.5201825135223,
133.849238377328)) ;
#134147=CARTESIAN_POINT('Ctrl Pts',(-11.3797145298603,13.5900682269615,
133.849605683645)) ;
#134148=CARTESIAN_POINT('Ctrl Pts',(-11.3096282167779,13.5628916742092,
133.84625764843)) ;
#134149=CARTESIAN_POINT('Ctrl Pts',(-11.2395419036955,13.5357151214569,
133.842909613214)) ;
#134150=CARTESIAN_POINT('Ctrl Pts',(-11.2668676693348,13.4658294080177,
133.842542306898)) ;
#134151=CARTESIAN_POINT('Ctrl Pts',(-11.2657108869576,13.4658303037659,
134.224522187712)) ;
#134152=CARTESIAN_POINT('Ctrl Pts',(-11.2930366525969,13.3959445903267,
134.224154881395)) ;
#134153=CARTESIAN_POINT('Ctrl Pts',(-11.3631229656793,13.423121143079,134.227502916611)) ;
#134154=CARTESIAN_POINT('Ctrl Pts',(-11.4332092787617,13.4502976958313,
134.230850951826)) ;
#134155=CARTESIAN_POINT('Ctrl Pts',(-11.4058835131224,13.5201834092705,
134.231218258142)) ;
#134156=CARTESIAN_POINT('Ctrl Pts',(-11.3785577474832,13.5900691227097,
134.231585564459)) ;
#134157=CARTESIAN_POINT('Ctrl Pts',(-11.3084714344008,13.5628925699574,
134.228237529244)) ;
#134158=CARTESIAN_POINT('Ctrl Pts',(-11.2383851213183,13.5357160172051,
134.224889494028)) ;
#134159=CARTESIAN_POINT('Ctrl Pts',(-11.2657108869576,13.4658303037659,
134.224522187712)) ;
#134160=CARTESIAN_POINT('Ctrl Pts',(-11.2645541045804,13.4658311995141,
134.606502068526)) ;
#134161=CARTESIAN_POINT('Ctrl Pts',(-11.2918798702197,13.3959454860749,
134.606134762209)) ;
#134162=CARTESIAN_POINT('Ctrl Pts',(-11.3619661833021,13.4231220388272,
134.609482797425)) ;
#134163=CARTESIAN_POINT('Ctrl Pts',(-11.4320524963845,13.4502985915795,
134.61283083264)) ;
#134164=CARTESIAN_POINT('Ctrl Pts',(-11.4047267307453,13.5201843050187,
134.613198138957)) ;
#134165=CARTESIAN_POINT('Ctrl Pts',(-11.377400965106,13.5900700184578,134.613565445273)) ;
#134166=CARTESIAN_POINT('Ctrl Pts',(-11.3073146520236,13.5628934657056,
134.610217410058)) ;
#134167=CARTESIAN_POINT('Ctrl Pts',(-11.2372283389412,13.5357169129533,
134.606869374843)) ;
#134168=CARTESIAN_POINT('Ctrl Pts',(-11.2645541045804,13.4658311995141,
134.606502068526)) ;
#134169=CARTESIAN_POINT('',(-11.2645541045804,13.4658311995141,134.606502068526)) ;
#134170=CARTESIAN_POINT('',(-11.2680244517119,13.4658285122696,133.460562426083)) ;
#134171=CARTESIAN_POINT('',(-11.3347092035438,13.4180239009611,134.608294431335)) ;
#134172=CARTESIAN_POINT('Origin',(-11.3346404176629,13.4930077522664,134.609850103741)) ;
#134173=CARTESIAN_POINT('',(-11.3345717668412,13.5679916035759,134.611405781511)) ;
#134174=CARTESIAN_POINT('Origin',(-11.3346404176629,13.4930077522664,134.609850103741)) ;
#134175=CARTESIAN_POINT('Origin',(-11.3346404176629,13.4930077522664,134.609850103741)) ;
#134176=CARTESIAN_POINT('Ctrl Pts',(-11.2645541045804,13.4658311995141,
134.606502068526)) ;
#134177=CARTESIAN_POINT('Ctrl Pts',(-11.2918798702197,13.3959454860749,
134.606134762209)) ;
#134178=CARTESIAN_POINT('Ctrl Pts',(-11.3619661833021,13.4231220388272,
134.609482797425)) ;
#134179=CARTESIAN_POINT('Ctrl Pts',(-11.4320524963845,13.4502985915795,
134.61283083264)) ;
#134180=CARTESIAN_POINT('Ctrl Pts',(-11.4047267307453,13.5201843050187,
134.613198138957)) ;
#134181=CARTESIAN_POINT('Ctrl Pts',(-11.377400965106,13.5900700184578,134.613565445273)) ;
#134182=CARTESIAN_POINT('Ctrl Pts',(-11.3073146520236,13.5628934657056,
134.610217410058)) ;
#134183=CARTESIAN_POINT('Ctrl Pts',(-11.2372283389412,13.5357169129533,
134.606869374843)) ;
#134184=CARTESIAN_POINT('Ctrl Pts',(-11.2645541045804,13.4658311995141,
134.606502068526)) ;
#134185=CARTESIAN_POINT('Ctrl Pts',(-11.25920483017,13.4658311995141,134.672131214346)) ;
#134186=CARTESIAN_POINT('Ctrl Pts',(-11.2865612947575,13.3959454860749,
134.6745078611)) ;
#134187=CARTESIAN_POINT('Ctrl Pts',(-11.3562925573149,13.4231220388272,
134.68489500114)) ;
#134188=CARTESIAN_POINT('Ctrl Pts',(-11.4260238198722,13.4502985915795,
134.69528214118)) ;
#134189=CARTESIAN_POINT('Ctrl Pts',(-11.3986673552847,13.5201843050187,
134.692905494426)) ;
#134190=CARTESIAN_POINT('Ctrl Pts',(-11.3713108906971,13.5900700184579,
134.690528847672)) ;
#134191=CARTESIAN_POINT('Ctrl Pts',(-11.3015796281398,13.5628934657056,
134.680141707632)) ;
#134192=CARTESIAN_POINT('Ctrl Pts',(-11.2318483655824,13.5357169129533,
134.669754567592)) ;
#134193=CARTESIAN_POINT('Ctrl Pts',(-11.25920483017,13.4658311995141,134.672131214346)) ;
#134194=CARTESIAN_POINT('Ctrl Pts',(-11.2276030587525,13.4658311995141,
134.805074979322)) ;
#134195=CARTESIAN_POINT('Ctrl Pts',(-11.2541595398934,13.3959454860749,
134.813089440493)) ;
#134196=CARTESIAN_POINT('Ctrl Pts',(-11.3209495279222,13.4231220388272,
134.837803867739)) ;
#134197=CARTESIAN_POINT('Ctrl Pts',(-11.3877395159509,13.4502985915795,
134.862518294986)) ;
#134198=CARTESIAN_POINT('Ctrl Pts',(-11.36118303481,13.5201843050187,134.854503833814)) ;
#134199=CARTESIAN_POINT('Ctrl Pts',(-11.3346265536691,13.5900700184578,
134.846489372643)) ;
#134200=CARTESIAN_POINT('Ctrl Pts',(-11.2678365656403,13.5628934657056,
134.821774945397)) ;
#134201=CARTESIAN_POINT('Ctrl Pts',(-11.2010465776116,13.5357169129533,
134.79706051815)) ;
#134202=CARTESIAN_POINT('Ctrl Pts',(-11.2276030587525,13.4658311995141,
134.805074979322)) ;
#134203=CARTESIAN_POINT('Ctrl Pts',(-11.1205249516122,13.4658311995141,
134.982414797281)) ;
#134204=CARTESIAN_POINT('Ctrl Pts',(-11.1433187808326,13.3959454860749,
134.998198158856)) ;
#134205=CARTESIAN_POINT('Ctrl Pts',(-11.1992381575979,13.4231220388272,
135.042237953121)) ;
#134206=CARTESIAN_POINT('Ctrl Pts',(-11.2551575343632,13.4502985915795,
135.086277747385)) ;
#134207=CARTESIAN_POINT('Ctrl Pts',(-11.2323637051428,13.5201843050187,
135.07049438581)) ;
#134208=CARTESIAN_POINT('Ctrl Pts',(-11.2095698759223,13.5900700184579,
135.054711024235)) ;
#134209=CARTESIAN_POINT('Ctrl Pts',(-11.1536504991571,13.5628934657056,
135.01067122997)) ;
#134210=CARTESIAN_POINT('Ctrl Pts',(-11.0977311223918,13.5357169129533,
134.966631435705)) ;
#134211=CARTESIAN_POINT('Ctrl Pts',(-11.1205249516122,13.4658311995141,
134.982414797281)) ;
#134212=CARTESIAN_POINT('Ctrl Pts',(-10.9633031492974,13.4658311995141,
135.117701111297)) ;
#134213=CARTESIAN_POINT('Ctrl Pts',(-10.9800904444232,13.3959454860749,
135.139700051809)) ;
#134214=CARTESIAN_POINT('Ctrl Pts',(-11.0196342967342,13.4231220388272,
135.198730933269)) ;
#134215=CARTESIAN_POINT('Ctrl Pts',(-11.0591781490452,13.4502985915795,
135.257761814729)) ;
#134216=CARTESIAN_POINT('Ctrl Pts',(-11.0423908539194,13.5201843050187,
135.235762874218)) ;
#134217=CARTESIAN_POINT('Ctrl Pts',(-11.0256035587936,13.5900700184578,
135.213763933706)) ;
#134218=CARTESIAN_POINT('Ctrl Pts',(-10.9860597064826,13.5628934657056,
135.154733052246)) ;
#134219=CARTESIAN_POINT('Ctrl Pts',(-10.9465158541716,13.5357169129533,
135.095702170786)) ;
#134220=CARTESIAN_POINT('Ctrl Pts',(-10.9633031492974,13.4658311995141,
135.117701111297)) ;
#134221=CARTESIAN_POINT('Ctrl Pts',(-10.7756218068419,13.4658311995141,
135.197451240537)) ;
#134222=CARTESIAN_POINT('Ctrl Pts',(-10.7849240119387,13.3959454860749,
135.223477631156)) ;
#134223=CARTESIAN_POINT('Ctrl Pts',(-10.8046490834956,13.4231220388272,
135.291658096106)) ;
#134224=CARTESIAN_POINT('Ctrl Pts',(-10.8243741550525,13.4502985915795,
135.359838561057)) ;
#134225=CARTESIAN_POINT('Ctrl Pts',(-10.8150719499557,13.5201843050187,
135.333812170438)) ;
#134226=CARTESIAN_POINT('Ctrl Pts',(-10.8057697448589,13.5900700184579,
135.30778577982)) ;
#134227=CARTESIAN_POINT('Ctrl Pts',(-10.786044673302,13.5628934657056,135.239605314869)) ;
#134228=CARTESIAN_POINT('Ctrl Pts',(-10.7663196017452,13.5357169129533,
135.171424849918)) ;
#134229=CARTESIAN_POINT('Ctrl Pts',(-10.7756218068419,13.4658311995141,
135.197451240537)) ;
#134230=CARTESIAN_POINT('Ctrl Pts',(-10.572784802571,13.4658311995141,135.217973355629)) ;
#134231=CARTESIAN_POINT('Ctrl Pts',(-10.5737445376646,13.3959454860749,
135.245627319145)) ;
#134232=CARTESIAN_POINT('Ctrl Pts',(-10.5718329415469,13.4231220388272,
135.3166705477)) ;
#134233=CARTESIAN_POINT('Ctrl Pts',(-10.5699213454292,13.4502985915795,
135.387713776254)) ;
#134234=CARTESIAN_POINT('Ctrl Pts',(-10.5689616103356,13.5201843050187,
135.360059812739)) ;
#134235=CARTESIAN_POINT('Ctrl Pts',(-10.5680018752419,13.5900700184579,
135.332405849223)) ;
#134236=CARTESIAN_POINT('Ctrl Pts',(-10.5699134713596,13.5628934657056,
135.261362620669)) ;
#134237=CARTESIAN_POINT('Ctrl Pts',(-10.5718250674773,13.5357169129533,
135.190319392114)) ;
#134238=CARTESIAN_POINT('Ctrl Pts',(-10.572784802571,13.4658311995141,135.217973355629)) ;
#134239=CARTESIAN_POINT('Ctrl Pts',(-10.3699582950185,13.4658311995141,
135.175134903948)) ;
#134240=CARTESIAN_POINT('Ctrl Pts',(-10.362331940556,13.3959454860749,135.201787052399)) ;
#134241=CARTESIAN_POINT('Ctrl Pts',(-10.3385749628922,13.4231220388272,
135.268914209501)) ;
#134242=CARTESIAN_POINT('Ctrl Pts',(-10.3148179852285,13.4502985915795,
135.336041366603)) ;
#134243=CARTESIAN_POINT('Ctrl Pts',(-10.322444339691,13.5201843050187,135.309389218153)) ;
#134244=CARTESIAN_POINT('Ctrl Pts',(-10.3300706941535,13.5900700184579,
135.282737069703)) ;
#134245=CARTESIAN_POINT('Ctrl Pts',(-10.3538276718172,13.5628934657056,
135.2156099126)) ;
#134246=CARTESIAN_POINT('Ctrl Pts',(-10.377584649481,13.5357169129533,135.148482755498)) ;
#134247=CARTESIAN_POINT('Ctrl Pts',(-10.3699582950185,13.4658311995141,
135.175134903948)) ;
#134248=CARTESIAN_POINT('Ctrl Pts',(-10.1908705742325,13.4658311995141,
135.071278506368)) ;
#134249=CARTESIAN_POINT('Ctrl Pts',(-10.1754087005963,13.3959454860749,
135.094305894918)) ;
#134250=CARTESIAN_POINT('Ctrl Pts',(-10.132144438372,13.4231220388272,135.150910732527)) ;
#134251=CARTESIAN_POINT('Ctrl Pts',(-10.0888801761478,13.4502985915795,
135.207515570136)) ;
#134252=CARTESIAN_POINT('Ctrl Pts',(-10.1043420497839,13.5201843050187,
135.184488181586)) ;
#134253=CARTESIAN_POINT('Ctrl Pts',(-10.11980392342,13.5900700184578,135.161460793036)) ;
#134254=CARTESIAN_POINT('Ctrl Pts',(-10.1630681856443,13.5628934657056,
135.104855955427)) ;
#134255=CARTESIAN_POINT('Ctrl Pts',(-10.2063324478686,13.5357169129533,
135.048251117818)) ;
#134256=CARTESIAN_POINT('Ctrl Pts',(-10.1908705742325,13.4658311995141,
135.071278506368)) ;
#134257=CARTESIAN_POINT('Ctrl Pts',(-10.0546595912401,13.4658311995141,
134.920519441332)) ;
#134258=CARTESIAN_POINT('Ctrl Pts',(-10.0329617205844,13.3959454860749,
134.937811672168)) ;
#134259=CARTESIAN_POINT('Ctrl Pts',(-9.97462287968318,13.4231220388272,
134.978735156726)) ;
#134260=CARTESIAN_POINT('Ctrl Pts',(-9.91628403878198,13.4502985915795,
135.019658641283)) ;
#134261=CARTESIAN_POINT('Ctrl Pts',(-9.93798190943768,13.5201843050187,
135.002366410447)) ;
#134262=CARTESIAN_POINT('Ctrl Pts',(-9.95967978009337,13.5900700184578,
134.985074179611)) ;
#134263=CARTESIAN_POINT('Ctrl Pts',(-10.0180186209946,13.5628934657056,
134.944150695053)) ;
#134264=CARTESIAN_POINT('Ctrl Pts',(-10.0763574618958,13.5357169129533,
134.903227210496)) ;
#134265=CARTESIAN_POINT('Ctrl Pts',(-10.0546595912401,13.4658311995141,
134.920519441332)) ;
#134266=CARTESIAN_POINT('Ctrl Pts',(-9.96976593511389,13.4658311995141,
134.736076962611)) ;
#134267=CARTESIAN_POINT('Ctrl Pts',(-9.94383295001097,13.3959454860749,
134.746039923768)) ;
#134268=CARTESIAN_POINT('Ctrl Pts',(-9.87579920343744,13.4231220388272,
134.767509557221)) ;
#134269=CARTESIAN_POINT('Ctrl Pts',(-9.8077654568639,13.4502985915795,134.788979190673)) ;
#134270=CARTESIAN_POINT('Ctrl Pts',(-9.83369844196683,13.5201843050187,
134.779016229516)) ;
#134271=CARTESIAN_POINT('Ctrl Pts',(-9.85963142706976,13.5900700184578,
134.769053268359)) ;
#134272=CARTESIAN_POINT('Ctrl Pts',(-9.92766517364329,13.5628934657056,
134.747583634906)) ;
#134273=CARTESIAN_POINT('Ctrl Pts',(-9.99569892021682,13.5357169129533,
134.726114001454)) ;
#134274=CARTESIAN_POINT('Ctrl Pts',(-9.96976593511389,13.4658311995141,
134.736076962611)) ;
#134275=CARTESIAN_POINT('Ctrl Pts',(-9.9450022707828,13.4658311995141,134.530889401624)) ;
#134276=CARTESIAN_POINT('Ctrl Pts',(-9.91725078023896,13.3959454860749,
134.532432185862)) ;
#134277=CARTESIAN_POINT('Ctrl Pts',(-9.84588765184722,13.4231220388272,
134.532030726634)) ;
#134278=CARTESIAN_POINT('Ctrl Pts',(-9.7745245234555,13.4502985915795,134.531629267406)) ;
#134279=CARTESIAN_POINT('Ctrl Pts',(-9.80227601399935,13.5201843050187,
134.530086483168)) ;
#134280=CARTESIAN_POINT('Ctrl Pts',(-9.83002750454321,13.5900700184579,
134.52854369893)) ;
#134281=CARTESIAN_POINT('Ctrl Pts',(-9.90139063293494,13.5628934657056,
134.528945158158)) ;
#134282=CARTESIAN_POINT('Ctrl Pts',(-9.97275376132666,13.5357169129533,
134.529346617386)) ;
#134283=CARTESIAN_POINT('Ctrl Pts',(-9.9450022707828,13.4658311995141,134.530889401624)) ;
#134284=CARTESIAN_POINT('Ctrl Pts',(-9.98579846627996,13.4658311995141,
134.328087474358)) ;
#134285=CARTESIAN_POINT('Ctrl Pts',(-9.95895961611388,13.3959454860749,
134.321058285225)) ;
#134286=CARTESIAN_POINT('Ctrl Pts',(-9.89129025850839,13.4231220388272,
134.298825334214)) ;
#134287=CARTESIAN_POINT('Ctrl Pts',(-9.8236209009029,13.4502985915795,134.276592383203)) ;
#134288=CARTESIAN_POINT('Ctrl Pts',(-9.85045975106899,13.5201843050187,
134.283621572337)) ;
#134289=CARTESIAN_POINT('Ctrl Pts',(-9.87729860123505,13.5900700184579,
134.29065076147)) ;
#134290=CARTESIAN_POINT('Ctrl Pts',(-9.94496795884055,13.5628934657056,
134.312883712481)) ;
#134291=CARTESIAN_POINT('Ctrl Pts',(-10.012637316446,13.5357169129533,134.335116663492)) ;
#134292=CARTESIAN_POINT('Ctrl Pts',(-9.98579846627996,13.4658311995141,
134.328087474358)) ;
#134293=CARTESIAN_POINT('Ctrl Pts',(-10.084932132731,13.4658311995141,134.150331039369)) ;
#134294=CARTESIAN_POINT('Ctrl Pts',(-10.0615244873061,13.3959454860749,
134.135546052038)) ;
#134295=CARTESIAN_POINT('Ctrl Pts',(-10.0038742640268,13.4231220388272,
134.093969291127)) ;
#134296=CARTESIAN_POINT('Ctrl Pts',(-9.94622404074765,13.4502985915795,
134.052392530217)) ;
#134297=CARTESIAN_POINT('Ctrl Pts',(-9.96963168617264,13.5201843050187,
134.067177517548)) ;
#134298=CARTESIAN_POINT('Ctrl Pts',(-9.99303933159763,13.5900700184578,
134.08196250488)) ;
#134299=CARTESIAN_POINT('Ctrl Pts',(-10.0506895548768,13.5628934657056,
134.12353926579)) ;
#134300=CARTESIAN_POINT('Ctrl Pts',(-10.108339778156,13.5357169129533,134.165116026701)) ;
#134301=CARTESIAN_POINT('Ctrl Pts',(-10.084932132731,13.4658311995141,134.150331039369)) ;
#134302=CARTESIAN_POINT('Ctrl Pts',(-10.2325806005316,13.4658311995141,
134.009906610499)) ;
#134303=CARTESIAN_POINT('Ctrl Pts',(-10.2147622260544,13.3959454860749,
133.98872944415)) ;
#134304=CARTESIAN_POINT('Ctrl Pts',(-10.1724461134115,13.4231220388272,
133.931643368614)) ;
#134305=CARTESIAN_POINT('Ctrl Pts',(-10.1301300007686,13.4502985915795,
133.874557293077)) ;
#134306=CARTESIAN_POINT('Ctrl Pts',(-10.1479483752457,13.5201843050187,
133.895734459426)) ;
#134307=CARTESIAN_POINT('Ctrl Pts',(-10.1657667497229,13.5900700184578,
133.916911625774)) ;
#134308=CARTESIAN_POINT('Ctrl Pts',(-10.2080828623658,13.5628934657056,
133.973997701311)) ;
#134309=CARTESIAN_POINT('Ctrl Pts',(-10.2503989750087,13.5357169129533,
134.031083776847)) ;
#134310=CARTESIAN_POINT('Ctrl Pts',(-10.2325806005316,13.4658311995141,
134.009906610499)) ;
#134311=CARTESIAN_POINT('Ctrl Pts',(-10.4193096302539,13.4658311995141,
133.919352405347)) ;
#134312=CARTESIAN_POINT('Ctrl Pts',(-10.4088951913955,13.3959454860749,
133.893703082496)) ;
#134313=CARTESIAN_POINT('Ctrl Pts',(-10.3862601761435,13.4231220388272,
133.826314652615)) ;
#134314=CARTESIAN_POINT('Ctrl Pts',(-10.3636251608916,13.4502985915795,
133.758926222735)) ;
#134315=CARTESIAN_POINT('Ctrl Pts',(-10.37403959975,13.5201843050187,133.784575545586)) ;
#134316=CARTESIAN_POINT('Ctrl Pts',(-10.3844540386085,13.5900700184579,
133.810224868437)) ;
#134317=CARTESIAN_POINT('Ctrl Pts',(-10.4070890538605,13.5628934657056,
133.877613298317)) ;
#134318=CARTESIAN_POINT('Ctrl Pts',(-10.4297240691124,13.5357169129533,
133.945001728198)) ;
#134319=CARTESIAN_POINT('Ctrl Pts',(-10.4193096302539,13.4658311995141,
133.919352405347)) ;
#134320=CARTESIAN_POINT('Ctrl Pts',(-10.6249148927388,13.4658311995141,
133.891382896145)) ;
#134321=CARTESIAN_POINT('Ctrl Pts',(-10.62292917198,13.3959454860749,133.863786357312)) ;
#134322=CARTESIAN_POINT('Ctrl Pts',(-10.6222023784514,13.4231220388272,
133.79272927929)) ;
#134323=CARTESIAN_POINT('Ctrl Pts',(-10.6214755849228,13.4502985915795,
133.721672201269)) ;
#134324=CARTESIAN_POINT('Ctrl Pts',(-10.6234613056815,13.5201843050187,
133.749268740102)) ;
#134325=CARTESIAN_POINT('Ctrl Pts',(-10.6254470264403,13.5900700184578,
133.776865278935)) ;
#134326=CARTESIAN_POINT('Ctrl Pts',(-10.6261738199689,13.5628934657056,
133.847922356956)) ;
#134327=CARTESIAN_POINT('Ctrl Pts',(-10.6269006134975,13.5357169129533,
133.918979434977)) ;
#134328=CARTESIAN_POINT('Ctrl Pts',(-10.6249148927388,13.4658311995141,
133.891382896145)) ;
#134329=CARTESIAN_POINT('Ctrl Pts',(-10.7598002515905,13.4658311995141,
133.915014269252)) ;
#134330=CARTESIAN_POINT('Ctrl Pts',(-10.763505813003,13.3959454860749,133.887882392195)) ;
#134331=CARTESIAN_POINT('Ctrl Pts',(-10.7772907287654,13.4231220388272,
133.818909929522)) ;
#134332=CARTESIAN_POINT('Ctrl Pts',(-10.7910756445278,13.4502985915795,
133.74993746685)) ;
#134333=CARTESIAN_POINT('Ctrl Pts',(-10.7873700831153,13.5201843050187,
133.777069343907)) ;
#134334=CARTESIAN_POINT('Ctrl Pts',(-10.7836645217028,13.5900700184578,
133.804201220964)) ;
#134335=CARTESIAN_POINT('Ctrl Pts',(-10.7698796059404,13.5628934657056,
133.873173683637)) ;
#134336=CARTESIAN_POINT('Ctrl Pts',(-10.756094690178,13.5357169129533,133.942146146309)) ;
#134337=CARTESIAN_POINT('Ctrl Pts',(-10.7598002515905,13.4658311995141,
133.915014269252)) ;
#134338=CARTESIAN_POINT('Ctrl Pts',(-10.8223318974888,13.4658311995141,
133.936074466937)) ;
#134339=CARTESIAN_POINT('Ctrl Pts',(-10.8287148089814,13.3959454860749,
133.909577338005)) ;
#134340=CARTESIAN_POINT('Ctrl Pts',(-10.849260688724,13.4231220388272,133.842652384728)) ;
#134341=CARTESIAN_POINT('Ctrl Pts',(-10.8698065684665,13.4502985915795,
133.77572743145)) ;
#134342=CARTESIAN_POINT('Ctrl Pts',(-10.8634236569739,13.5201843050187,
133.802224560383)) ;
#134343=CARTESIAN_POINT('Ctrl Pts',(-10.8570407454813,13.5900700184578,
133.828721689315)) ;
#134344=CARTESIAN_POINT('Ctrl Pts',(-10.8364948657388,13.5628934657056,
133.895646642592)) ;
#134345=CARTESIAN_POINT('Ctrl Pts',(-10.8159489859962,13.5357169129533,
133.96257159587)) ;
#134346=CARTESIAN_POINT('Ctrl Pts',(-10.8223318974888,13.4658311995141,
133.936074466937)) ;
#134347=CARTESIAN_POINT('Ctrl Pts',(-11.2645541045804,13.4658311995141,
134.606502068526)) ;
#134348=CARTESIAN_POINT('Ctrl Pts',(-11.25920483017,13.4658311995141,134.672131214346)) ;
#134349=CARTESIAN_POINT('Ctrl Pts',(-11.2276030587525,13.4658311995141,
134.805074979322)) ;
#134350=CARTESIAN_POINT('Ctrl Pts',(-11.1205249516122,13.4658311995141,
134.982414797281)) ;
#134351=CARTESIAN_POINT('Ctrl Pts',(-10.9633031492974,13.4658311995141,
135.117701111297)) ;
#134352=CARTESIAN_POINT('Ctrl Pts',(-10.7756218068419,13.4658311995141,
135.197451240537)) ;
#134353=CARTESIAN_POINT('Ctrl Pts',(-10.572784802571,13.4658311995141,135.217973355629)) ;
#134354=CARTESIAN_POINT('Ctrl Pts',(-10.3699582950185,13.4658311995141,
135.175134903948)) ;
#134355=CARTESIAN_POINT('Ctrl Pts',(-10.1908705742325,13.4658311995141,
135.071278506368)) ;
#134356=CARTESIAN_POINT('Ctrl Pts',(-10.0546595912401,13.4658311995141,
134.920519441332)) ;
#134357=CARTESIAN_POINT('Ctrl Pts',(-9.96976593511389,13.4658311995141,
134.736076962611)) ;
#134358=CARTESIAN_POINT('Ctrl Pts',(-9.9450022707828,13.4658311995141,134.530889401624)) ;
#134359=CARTESIAN_POINT('Ctrl Pts',(-9.98579846627996,13.4658311995141,
134.328087474358)) ;
#134360=CARTESIAN_POINT('Ctrl Pts',(-10.084932132731,13.4658311995141,134.150331039369)) ;
#134361=CARTESIAN_POINT('Ctrl Pts',(-10.2325806005316,13.4658311995141,
134.009906610499)) ;
#134362=CARTESIAN_POINT('Ctrl Pts',(-10.4193096302539,13.4658311995141,
133.919352405347)) ;
#134363=CARTESIAN_POINT('Ctrl Pts',(-10.6249148927388,13.4658311995141,
133.891382896145)) ;
#134364=CARTESIAN_POINT('Ctrl Pts',(-10.7598002515905,13.4658311995141,
133.915014269252)) ;
#134365=CARTESIAN_POINT('Ctrl Pts',(-10.8223318974888,13.4658311995141,
133.936074466937)) ;
#134366=CARTESIAN_POINT('Origin',(-33.7895361580819,13.385947639229,127.22876720957)) ;
#134367=CARTESIAN_POINT('',(-33.8079438763917,13.4658311995141,127.161214257016)) ;
#134368=CARTESIAN_POINT('Origin',(-33.7873979966492,13.4930077522664,127.228139210294)) ;
#134369=CARTESIAN_POINT('Ctrl Pts',(-33.3489959095147,13.1551399285885,
127.871927411069)) ;
#134370=CARTESIAN_POINT('Ctrl Pts',(-33.3482570091173,13.1489709609094,
127.870499856875)) ;
#134371=CARTESIAN_POINT('Ctrl Pts',(-33.3362031847492,13.0505878441039,
127.846970056077)) ;
#134372=CARTESIAN_POINT('Ctrl Pts',(-33.303456104594,12.8648900473044,127.774282508598)) ;
#134373=CARTESIAN_POINT('Ctrl Pts',(-33.2347176391245,12.6378996894465,
127.606502631126)) ;
#134374=CARTESIAN_POINT('Ctrl Pts',(-33.1484631699894,12.4661938442505,
127.38763758675)) ;
#134375=CARTESIAN_POINT('Ctrl Pts',(-33.0496339239794,12.3629468779938,
127.132205946451)) ;
#134376=CARTESIAN_POINT('Ctrl Pts',(-32.9461836982222,12.3360866578135,
126.862930995212)) ;
#134377=CARTESIAN_POINT('Ctrl Pts',(-32.8428524780797,12.3868467815327,
126.594300512203)) ;
#134378=CARTESIAN_POINT('Ctrl Pts',(-32.7476240151848,12.5118616193735,
126.34920621096)) ;
#134379=CARTESIAN_POINT('Ctrl Pts',(-32.6660393235339,12.7022376314793,
126.14402042184)) ;
#134380=CARTESIAN_POINT('Ctrl Pts',(-32.6034202579729,12.9442211340136,
125.994217779495)) ;
#134381=CARTESIAN_POINT('Ctrl Pts',(-32.5634889320909,13.2203922331636,
125.91068247448)) ;
#134382=CARTESIAN_POINT('Ctrl Pts',(-32.5482836171183,13.5109001041669,
125.899354456419)) ;
#134383=CARTESIAN_POINT('Ctrl Pts',(-32.5583885908025,13.7967277450532,
125.962163306551)) ;
#134384=CARTESIAN_POINT('Ctrl Pts',(-32.5919970185865,14.0531634695327,
126.093303648423)) ;
#134385=CARTESIAN_POINT('Ctrl Pts',(-32.6462352627175,14.2659161102292,
126.2848763833)) ;
#134386=CARTESIAN_POINT('Ctrl Pts',(-32.7164440425069,14.4182155312585,
126.52308858485)) ;
#134387=CARTESIAN_POINT('Ctrl Pts',(-32.7970929244734,14.4993926065239,
126.791896512519)) ;
#134388=CARTESIAN_POINT('Ctrl Pts',(-32.8812312900771,14.5030674016304,
127.070805593369)) ;
#134389=CARTESIAN_POINT('Ctrl Pts',(-32.9621947752627,14.4296658181567,
127.340390412531)) ;
#134390=CARTESIAN_POINT('Ctrl Pts',(-33.0336799536047,14.2842405620309,
127.582320067705)) ;
#134391=CARTESIAN_POINT('Ctrl Pts',(-33.0898518257578,14.0768885755418,
127.779563482544)) ;
#134392=CARTESIAN_POINT('Ctrl Pts',(-33.1258131095785,13.821937566696,127.917839903426)) ;
#134393=CARTESIAN_POINT('Ctrl Pts',(-33.1381603359796,13.5404397832619,
127.986888146398)) ;
#134394=CARTESIAN_POINT('Ctrl Pts',(-33.1255862370588,13.2491903771815,
127.98329800545)) ;
#134395=CARTESIAN_POINT('Ctrl Pts',(-33.0878760919221,12.9699188880577,
127.906345203758)) ;
#134396=CARTESIAN_POINT('Ctrl Pts',(-33.0275630545352,12.7245502986717,
127.763166970814)) ;
#134397=CARTESIAN_POINT('Ctrl Pts',(-32.9475449968705,12.5279694687298,
127.562611942766)) ;
#134398=CARTESIAN_POINT('Ctrl Pts',(-32.853484832887,12.3961377043517,127.320906369453)) ;
#134399=CARTESIAN_POINT('Ctrl Pts',(-32.7506275244767,12.3376103677892,
127.053662058531)) ;
#134400=CARTESIAN_POINT('Ctrl Pts',(-32.6467508382538,12.3569098529355,
126.783214181605)) ;
#134401=CARTESIAN_POINT('Ctrl Pts',(-32.5472606088073,12.452769019898,126.525790390631)) ;
#134402=CARTESIAN_POINT('Ctrl Pts',(-32.4595735399336,12.6179593573441,
126.30272348908)) ;
#134403=CARTESIAN_POINT('Ctrl Pts',(-32.388745121808,12.8405880377693,126.12891456918)) ;
#134404=CARTESIAN_POINT('Ctrl Pts',(-32.3390681420419,13.1065246421439,
126.017073858121)) ;
#134405=CARTESIAN_POINT('Ctrl Pts',(-32.313898204756,13.3925179674891,125.976505647384)) ;
#134406=CARTESIAN_POINT('Ctrl Pts',(-32.3136699242009,13.6819916651313,
126.008953177836)) ;
#134407=CARTESIAN_POINT('Ctrl Pts',(-32.3381285657715,13.9537242418059,
126.113619428421)) ;
#134408=CARTESIAN_POINT('Ctrl Pts',(-32.384536696511,14.1863734291659,126.28227784121)) ;
#134409=CARTESIAN_POINT('Ctrl Pts',(-32.4487957222161,14.3643807985693,
126.503053049914)) ;
#134410=CARTESIAN_POINT('Ctrl Pts',(-32.5258074280907,14.4754559850244,
126.761140801679)) ;
#134411=CARTESIAN_POINT('Ctrl Pts',(-32.6094667487868,14.5110246739577,
127.038737149779)) ;
#134412=CARTESIAN_POINT('Ctrl Pts',(-32.6924145513944,14.4687063588107,
127.314091355005)) ;
#134413=CARTESIAN_POINT('Ctrl Pts',(-32.7687110106265,14.3514018815055,
127.570143149353)) ;
#134414=CARTESIAN_POINT('Ctrl Pts',(-32.8317732094795,14.1671964752596,
127.787539429963)) ;
#134415=CARTESIAN_POINT('Ctrl Pts',(-32.8762267217076,13.9308608041133,
127.950416591701)) ;
#134416=CARTESIAN_POINT('Ctrl Pts',(-32.8985780094168,13.6570089999716,
128.048890973466)) ;
#134417=CARTESIAN_POINT('Ctrl Pts',(-32.896157678737,13.3664659574419,128.074980037028)) ;
#134418=CARTESIAN_POINT('Ctrl Pts',(-32.8685548522265,13.0805681472547,
128.027442701697)) ;
#134419=CARTESIAN_POINT('Ctrl Pts',(-32.8170821736547,12.8190539470386,
127.91017574478)) ;
#134420=CARTESIAN_POINT('Ctrl Pts',(-32.7441829163896,12.5999338423892,
127.73048258649)) ;
#134421=CARTESIAN_POINT('Ctrl Pts',(-32.6555170250936,12.4413957528131,
127.504429482033)) ;
#134422=CARTESIAN_POINT('Ctrl Pts',(-32.5554705400289,12.3520378265489,
127.245337069314)) ;
#134423=CARTESIAN_POINT('Ctrl Pts',(-32.4511053019089,12.339734386482,126.973578302647)) ;
#134424=CARTESIAN_POINT('Ctrl Pts',(-32.3490815539954,12.4049383167358,
126.708653969777)) ;
#134425=CARTESIAN_POINT('Ctrl Pts',(-32.2559652828001,12.5429634979505,
126.469740198936)) ;
#134426=CARTESIAN_POINT('Ctrl Pts',(-32.1775406776191,12.7443553986761,
126.273802702315)) ;
#134427=CARTESIAN_POINT('Ctrl Pts',(-32.1189511785612,12.9943521537239,
126.135786155147)) ;
#134428=CARTESIAN_POINT('Ctrl Pts',(-32.0836266547703,13.2741647768729,
126.065632995122)) ;
#134429=CARTESIAN_POINT('Ctrl Pts',(-32.0731422430725,13.565720269456,126.068169777388)) ;
#134430=CARTESIAN_POINT('Ctrl Pts',(-32.0878672761987,13.8474315556546,
126.144404645481)) ;
#134431=CARTESIAN_POINT('Ctrl Pts',(-32.1256175280986,14.0971649669908,
126.287692127083)) ;
#134432=CARTESIAN_POINT('Ctrl Pts',(-32.1834742057281,14.3002122843455,
126.489943063825)) ;
#134433=CARTESIAN_POINT('Ctrl Pts',(-32.2561937622249,14.4394509674979,
126.73551422792)) ;
#134434=CARTESIAN_POINT('Ctrl Pts',(-32.3374471159419,14.5058688200503,
127.005843081603)) ;
#134435=CARTESIAN_POINT('Ctrl Pts',(-32.4217002826958,14.4952594831202,
127.285155611484)) ;
#134436=CARTESIAN_POINT('Ctrl Pts',(-32.5017471426193,14.4071576912799,
127.552229665334)) ;
#134437=CARTESIAN_POINT('Ctrl Pts',(-32.5706761898774,14.2488070341169,
127.786694114575)) ;
#134438=CARTESIAN_POINT('Ctrl Pts',(-32.6230717724866,14.032332595662,127.972746797191)) ;
#134439=CARTESIAN_POINT('Ctrl Pts',(-32.6548239115267,13.7715185673777,
128.098623777025)) ;
#134440=CARTESIAN_POINT('Ctrl Pts',(-32.6626680714647,13.4849968555095,
128.154735100321)) ;
#134441=CARTESIAN_POINT('Ctrl Pts',(-32.6450616243189,13.1936954317484,
128.136543946875)) ;
#134442=CARTESIAN_POINT('Ctrl Pts',(-32.6032602463952,12.9217410981826,
128.047311789015)) ;
#134443=CARTESIAN_POINT('Ctrl Pts',(-32.5386314820962,12.6826993167214,
127.891757560495)) ;
#134444=CARTESIAN_POINT('Ctrl Pts',(-32.4554412889622,12.4976839220085,
127.681914464153)) ;
#134445=CARTESIAN_POINT('Ctrl Pts',(-32.3596753952525,12.3794711428103,
127.435114332308)) ;
#134446=CARTESIAN_POINT('Ctrl Pts',(-32.2558253838943,12.3351744196322,
127.165019558565)) ;
#134447=CARTESIAN_POINT('Ctrl Pts',(-32.1520107530796,12.3695012763354,
126.894875973638)) ;
#134448=CARTESIAN_POINT('Ctrl Pts',(-32.0548036090535,12.4786183736045,
126.643923371603)) ;
#134449=CARTESIAN_POINT('Ctrl Pts',(-31.9697179472944,12.6556201701116,
126.428500311369)) ;
#134450=CARTESIAN_POINT('Ctrl Pts',(-31.9024466959007,12.8885376957079,
126.26521267139)) ;
#134451=CARTESIAN_POINT('Ctrl Pts',(-31.8574815700017,13.1578672277872,
126.166847085394)) ;
#134452=CARTESIAN_POINT('Ctrl Pts',(-31.8367167778053,13.4488181058444,
126.139492583638)) ;
#134453=CARTESIAN_POINT('Ctrl Pts',(-31.8414313820349,13.7357351250712,
126.186316118843)) ;
#134454=CARTESIAN_POINT('Ctrl Pts',(-31.8700151821842,14.0000244154435,
126.30281009704)) ;
#134455=CARTESIAN_POINT('Ctrl Pts',(-31.9203616130848,14.2248063693443,
126.483142763909)) ;
#134456=CARTESIAN_POINT('Ctrl Pts',(-31.9873859775564,14.3907221531774,
126.711954484493)) ;
#134457=CARTESIAN_POINT('Ctrl Pts',(-32.0662309963865,14.4880878052934,
126.975454295977)) ;
#134458=CARTESIAN_POINT('Ctrl Pts',(-32.1500140049146,14.5090844515927,
127.253273584441)) ;
#134459=CARTESIAN_POINT('Ctrl Pts',(-32.2328114906108,14.4517331277302,
127.528461364111)) ;
#134460=CARTESIAN_POINT('Ctrl Pts',(-32.306599429151,14.3213873494252,127.777000865602)) ;
#134461=CARTESIAN_POINT('Ctrl Pts',(-32.3665410586647,14.1266126254878,
127.985228303146)) ;
#134462=CARTESIAN_POINT('Ctrl Pts',(-32.4072983071001,13.8801113803002,
128.137553257528)) ;
#134463=CARTESIAN_POINT('Ctrl Pts',(-32.4248919159062,13.6025840232108,
128.221986639911)) ;
#134464=CARTESIAN_POINT('Ctrl Pts',(-32.4177985341224,13.3122088978665,
128.234314532032)) ;
#134465=CARTESIAN_POINT('Ctrl Pts',(-32.3854612722872,13.0284665595888,
128.173051822567)) ;
#134466=CARTESIAN_POINT('Ctrl Pts',(-32.3297158719588,12.7739765033465,
128.043289524966)) ;
#134467=CARTESIAN_POINT('Ctrl Pts',(-32.2536312710535,12.5655228915478,
127.854171141032)) ;
#134468=CARTESIAN_POINT('Ctrl Pts',(-32.1621333883639,12.4188418488155,
127.619973715704)) ;
#134469=CARTESIAN_POINT('Ctrl Pts',(-32.0610335191924,12.3438198182334,
127.357704488195)) ;
#134470=CARTESIAN_POINT('Ctrl Pts',(-31.9562422849269,12.3461749880073,
127.084814084959)) ;
#134471=CARTESIAN_POINT('Ctrl Pts',(-31.8555595514267,12.4256199459212,
126.823755799531)) ;
#134472=CARTESIAN_POINT('Ctrl Pts',(-31.7646812381954,12.5766359900473,
126.591428395529)) ;
#134473=CARTESIAN_POINT('Ctrl Pts',(-31.6897549709183,12.7882864475543,
126.405673808487)) ;
#134474=CARTESIAN_POINT('Ctrl Pts',(-31.6353440859288,13.0452019382586,
126.279829886042)) ;
#134475=CARTESIAN_POINT('Ctrl Pts',(-31.6045551307125,13.3293877258915,
126.223017390213)) ;
#134476=CARTESIAN_POINT('Ctrl Pts',(-31.598929994185,13.6204035856812,126.239726726341)) ;
#134477=CARTESIAN_POINT('Ctrl Pts',(-31.6181519561243,13.8971496153171,
126.329008321255)) ;
#134478=CARTESIAN_POINT('Ctrl Pts',(-31.660032440097,14.1397539052331,126.4844492787)) ;
#134479=CARTESIAN_POINT('Ctrl Pts',(-31.7210074180807,14.3313464702874,
126.695729086547)) ;
#134480=CARTESIAN_POINT('Ctrl Pts',(-31.7956413070931,14.4574458616527,
126.94680082343)) ;
#134481=CARTESIAN_POINT('Ctrl Pts',(-31.8782525153513,14.5099723944026,
127.221254124399)) ;
#134482=CARTESIAN_POINT('Ctrl Pts',(-31.9622607746967,14.4843439695083,
127.499872427198)) ;
#134483=CARTESIAN_POINT('Ctrl Pts',(-32.0404152099778,14.3827749410654,
127.761275810437)) ;
#134484=CARTESIAN_POINT('Ctrl Pts',(-32.1067647607671,14.2124739950545,
127.988225629159)) ;
#134485=CARTESIAN_POINT('Ctrl Pts',(-32.1557319181306,13.9855789386979,
128.164396849995)) ;
#134486=CARTESIAN_POINT('Ctrl Pts',(-32.1830886305706,13.7185805864342,
128.27741749427)) ;
#134487=CARTESIAN_POINT('Ctrl Pts',(-32.1861674536437,13.4303185636673,
128.319530923703)) ;
#134488=CARTESIAN_POINT('Ctrl Pts',(-32.164067606359,13.1417758325219,128.288060327875)) ;
#134489=CARTESIAN_POINT('Ctrl Pts',(-32.1174319130124,12.8725286043858,
128.185023246156)) ;
#134490=CARTESIAN_POINT('Ctrl Pts',(-32.0491401802662,12.6435096258014,
128.018626363072)) ;
#134491=CARTESIAN_POINT('Ctrl Pts',(-31.9632199754991,12.4701546223289,
127.800755651149)) ;
#134492=CARTESIAN_POINT('Ctrl Pts',(-31.8651776863348,12.3650501876111,
127.547453264018)) ;
#134493=CARTESIAN_POINT('Ctrl Pts',(-31.7609862185599,12.3357586674927,
127.276274914652)) ;
#134494=CARTESIAN_POINT('Ctrl Pts',(-31.6580563102104,12.3843195509594,
127.008647533804)) ;
#134495=CARTESIAN_POINT('Ctrl Pts',(-31.5623522569141,12.5073666683789,
126.762219617398)) ;
#134496=CARTESIAN_POINT('Ctrl Pts',(-31.4804283317136,12.6958200369819,
126.55599240923)) ;
#134497=CARTESIAN_POINT('Ctrl Pts',(-31.4171911262104,12.9363649293222,
126.404372140452)) ;
#134498=CARTESIAN_POINT('Ctrl Pts',(-31.3765204454803,13.212046231595,126.318705695641)) ;
#134499=CARTESIAN_POINT('Ctrl Pts',(-31.3605890149829,13.5022481067603,
126.305235943963)) ;
#134500=CARTESIAN_POINT('Ctrl Pts',(-31.3699466511949,13.7884016128943,
126.365844507772)) ;
#134501=CARTESIAN_POINT('Ctrl Pts',(-31.402839929772,14.045945075732,126.494887877481)) ;
#134502=CARTESIAN_POINT('Ctrl Pts',(-31.456801839307,14.2610680704969,126.685797164984)) ;
#134503=CARTESIAN_POINT('Ctrl Pts',(-31.5263791105061,14.4145624165552,
126.922033359285)) ;
#134504=CARTESIAN_POINT('Ctrl Pts',(-31.6068029650713,14.4980852125695,
127.190187763467)) ;
#134505=CARTESIAN_POINT('Ctrl Pts',(-31.6909497784616,14.5041312739862,
127.469125424148)) ;
#134506=CARTESIAN_POINT('Ctrl Pts',(-31.7722616933248,14.4326962339747,
127.739802187408)) ;
#134507=CARTESIAN_POINT('Ctrl Pts',(-31.8440399327869,14.289424830309,127.982545178335)) ;
#134508=CARTESIAN_POINT('Ctrl Pts',(-31.9008586342929,14.0826507854277,
128.181809264848)) ;
#134509=CARTESIAN_POINT('Ctrl Pts',(-31.9371644477761,13.8312291814697,
128.320780138694)) ;
#134510=CARTESIAN_POINT('Ctrl Pts',(-31.9504192122518,13.5479805821752,
128.392761416066)) ;
#134511=CARTESIAN_POINT('Ctrl Pts',(-31.9384428607775,13.2572981016289,
128.390846357411)) ;
#134512=CARTESIAN_POINT('Ctrl Pts',(-31.9016603090654,12.9781391944844,
128.316499055668)) ;
#134513=CARTESIAN_POINT('Ctrl Pts',(-31.8414344653115,12.7298471383749,
128.173831316095)) ;
#134514=CARTESIAN_POINT('Ctrl Pts',(-31.7624693619783,12.5331718510569,
127.976098656417)) ;
#134515=CARTESIAN_POINT('Ctrl Pts',(-31.6682896816273,12.3987050488903,
127.734214112554)) ;
#134516=CARTESIAN_POINT('Ctrl Pts',(-31.5661584069127,12.3381977133859,
127.468894861423)) ;
#134517=CARTESIAN_POINT('Ctrl Pts',(-31.4613121151811,12.3556285786372,
127.195919765139)) ;
#134518=CARTESIAN_POINT('Ctrl Pts',(-31.3626542471411,12.448498640132,126.940567661376)) ;
#134519=CARTESIAN_POINT('Ctrl Pts',(-31.2739963638957,12.6124651727369,
126.714860191145)) ;
#134520=CARTESIAN_POINT('Ctrl Pts',(-31.2028733579617,12.8330193864531,
126.540078371683)) ;
#134521=CARTESIAN_POINT('Ctrl Pts',(-31.1524099899045,13.0981216515098,
126.425973898796)) ;
#134522=CARTESIAN_POINT('Ctrl Pts',(-31.1264884036244,13.3840423616995,
126.383240800023)) ;
#134523=CARTESIAN_POINT('Ctrl Pts',(-31.1255526905879,13.6738043197191,
126.413632148392)) ;
#134524=CARTESIAN_POINT('Ctrl Pts',(-31.1492407119047,13.9458856450603,
126.515980892251)) ;
#134525=CARTESIAN_POINT('Ctrl Pts',(-31.1951906788803,14.1805609741337,
126.683399895541)) ;
#134526=CARTESIAN_POINT('Ctrl Pts',(-31.2589322113538,14.3602096703021,
126.902625201214)) ;
#134527=CARTESIAN_POINT('Ctrl Pts',(-31.336152907064,14.4737146563849,127.161521971997)) ;
#134528=CARTESIAN_POINT('Ctrl Pts',(-31.4191607366893,14.510981736058,127.436983917868)) ;
#134529=CARTESIAN_POINT('Ctrl Pts',(-31.5023202222332,14.4710234538019,
127.713002150618)) ;
#134530=CARTESIAN_POINT('Ctrl Pts',(-31.5788150531214,14.3558611755068,
127.9695934644)) ;
#134531=CARTESIAN_POINT('Ctrl Pts',(-31.6423459010436,14.1736059642118,
128.188348020273)) ;
#134532=CARTESIAN_POINT('Ctrl Pts',(-31.6874883180192,13.9381264816024,
128.353301532308)) ;
#134533=CARTESIAN_POINT('Ctrl Pts',(-31.7104598612239,13.665192099168,128.453567738071)) ;
#134534=CARTESIAN_POINT('Ctrl Pts',(-31.7088598170554,13.3755914984187,
128.481967244671)) ;
#134535=CARTESIAN_POINT('Ctrl Pts',(-31.6817723867748,13.0874857506397,
128.436147123456)) ;
#134536=CARTESIAN_POINT('Ctrl Pts',(-31.6311222896079,12.8264337657975,
128.32111606456)) ;
#134537=CARTESIAN_POINT('Ctrl Pts',(-31.5590254861687,12.6060974389448,
128.143694924089)) ;
#134538=CARTESIAN_POINT('Ctrl Pts',(-31.4705496041744,12.4450313389733,
127.91828768914)) ;
#134539=CARTESIAN_POINT('Ctrl Pts',(-31.3704536339561,12.3534666197661,
127.659136554107)) ;
#134540=CARTESIAN_POINT('Ctrl Pts',(-31.2664260741019,12.3390029903486,
127.388267266672)) ;
#134541=CARTESIAN_POINT('Ctrl Pts',(-31.1640074542676,12.4020392430349,
127.122262231831)) ;
#134542=CARTESIAN_POINT('Ctrl Pts',(-31.0704546098695,12.5385711173323,
126.882123477286)) ;
#134543=CARTESIAN_POINT('Ctrl Pts',(-30.9919375233747,12.737337324062,126.685748126109)) ;
#134544=CARTESIAN_POINT('Ctrl Pts',(-30.9326059877163,12.9861206892308,
126.545580982005)) ;
#134545=CARTESIAN_POINT('Ctrl Pts',(-30.8964828802307,13.2660910782566,
126.473182758033)) ;
#134546=CARTESIAN_POINT('Ctrl Pts',(-30.8853353619794,13.5573227840952,
126.473749977841)) ;
#134547=CARTESIAN_POINT('Ctrl Pts',(-30.8992181639316,13.8386952169897,
126.547405844888)) ;
#134548=CARTESIAN_POINT('Ctrl Pts',(-30.9364490028324,14.0906007554108,
126.689305896974)) ;
#134549=CARTESIAN_POINT('Ctrl Pts',(-30.993577379338,14.2945039762926,126.889303441531)) ;
#134550=CARTESIAN_POINT('Ctrl Pts',(-31.0658785833472,14.4361574187858,
127.133657392973)) ;
#134551=CARTESIAN_POINT('Ctrl Pts',(-31.1473678175875,14.5051117570611,
127.404837868273)) ;
#134552=CARTESIAN_POINT('Ctrl Pts',(-31.2314101845586,14.496582620466,127.68344430737)) ;
#134553=CARTESIAN_POINT('Ctrl Pts',(-31.3113999047549,14.4113394819302,
127.950224339128)) ;
#134554=CARTESIAN_POINT('Ctrl Pts',(-31.3810275644355,14.2546479447355,
128.186843915728)) ;
#134555=CARTESIAN_POINT('Ctrl Pts',(-31.434079388976,14.039143877786,128.374888028828)) ;
#134556=CARTESIAN_POINT('Ctrl Pts',(-31.4664410188237,13.7793416572316,
128.502539340318)) ;
#134557=CARTESIAN_POINT('Ctrl Pts',(-31.4749982660917,13.4941095874199,
128.560637934817)) ;
#134558=CARTESIAN_POINT('Ctrl Pts',(-31.4582310109701,13.2026874966814,
128.544890911873)) ;
#134559=CARTESIAN_POINT('Ctrl Pts',(-31.4169753439866,12.928833346161,128.457383735722)) ;
#134560=CARTESIAN_POINT('Ctrl Pts',(-31.3527956487623,12.6885083712283,
128.303172142516)) ;
#134561=CARTESIAN_POINT('Ctrl Pts',(-31.2705703901443,12.5026390795781,
128.0959611027)) ;
#134562=CARTESIAN_POINT('Ctrl Pts',(-31.1745744230575,12.3816810236162,
127.848677279268)) ;
#134563=CARTESIAN_POINT('Ctrl Pts',(-31.0714307037018,12.3354826595071,
127.580451601079)) ;
#134564=CARTESIAN_POINT('Ctrl Pts',(-30.9672895160686,12.3671988660942,
127.309429336125)) ;
#134565=CARTESIAN_POINT('Ctrl Pts',(-30.8693900237751,12.4748749581507,
127.056599017908)) ;
#134566=CARTESIAN_POINT('Ctrl Pts',(-30.7841568236753,12.6498955190515,
126.840662152846)) ;
#134567=CARTESIAN_POINT('Ctrl Pts',(-30.7165115975955,12.8801431332148,
126.67612667683)) ;
#134568=CARTESIAN_POINT('Ctrl Pts',(-30.6705876552176,13.1504415297617,
126.575185235204)) ;
#134569=CARTESIAN_POINT('Ctrl Pts',(-30.6492401911973,13.438739202615,126.545850310757)) ;
#134570=CARTESIAN_POINT('Ctrl Pts',(-30.6531248486497,13.7280473502378,
126.590480521703)) ;
#134571=CARTESIAN_POINT('Ctrl Pts',(-30.6811874381857,13.9932362064335,
126.705468605857)) ;
#134572=CARTESIAN_POINT('Ctrl Pts',(-30.7307233901376,14.2186783745982,
126.88330032276)) ;
#134573=CARTESIAN_POINT('Ctrl Pts',(-30.7976668939673,14.3872014330787,
127.112042032862)) ;
#134574=CARTESIAN_POINT('Ctrl Pts',(-30.8759215226086,14.486216521528,127.373662762679)) ;
#134575=CARTESIAN_POINT('Ctrl Pts',(-30.9599483085192,14.5095010567365,
127.652320679818)) ;
#134576=CARTESIAN_POINT('Ctrl Pts',(-31.0423602583126,14.4548476689191,
127.926162766265)) ;
#134577=CARTESIAN_POINT('Ctrl Pts',(-31.1170261636548,14.3259646517619,
128.177490633467)) ;
#134578=CARTESIAN_POINT('Ctrl Pts',(-31.1774376241067,14.1320240566172,
128.38715540167)) ;
#134579=CARTESIAN_POINT('Ctrl Pts',(-31.2184772814882,13.8890687487633,
128.540002184362)) ;
#134580=CARTESIAN_POINT('Ctrl Pts',(-31.2369718788586,13.6109288487181,
128.62723857725)) ;
#134581=CARTESIAN_POINT('Ctrl Pts',(-31.2305830637653,13.3205780973656,
128.64162358396)) ;
#134582=CARTESIAN_POINT('Ctrl Pts',(-31.1988306507602,13.0356410236252,
128.582156307125)) ;
#134583=CARTESIAN_POINT('Ctrl Pts',(-31.1439236012217,12.7811568557338,
128.454705635715)) ;
#134584=CARTESIAN_POINT('Ctrl Pts',(-31.0684038299569,12.5709851276515,
128.267243241426)) ;
#134585=CARTESIAN_POINT('Ctrl Pts',(-30.9772756205,12.4221766619671,128.03413250274)) ;
#134586=CARTESIAN_POINT('Ctrl Pts',(-30.8759319496152,12.3447406812541,
127.771290965256)) ;
#134587=CARTESIAN_POINT('Ctrl Pts',(-30.7712963261735,12.3451621602759,
127.498804673837)) ;
#134588=CARTESIAN_POINT('Ctrl Pts',(-30.6706886680026,12.4221617733591,
127.237875690043)) ;
#134589=CARTESIAN_POINT('Ctrl Pts',(-30.5793389036692,12.5713293574021,
127.00420358355)) ;
#134590=CARTESIAN_POINT('Ctrl Pts',(-30.5039469378259,12.7811357471148,
126.817049360709)) ;
#134591=CARTESIAN_POINT('Ctrl Pts',(-30.4488110435835,13.037385413305,126.689142569762)) ;
#134592=CARTESIAN_POINT('Ctrl Pts',(-30.4173468141487,13.3202247802994,
126.630258735514)) ;
#134593=CARTESIAN_POINT('Ctrl Pts',(-30.4109588954888,13.6126649497902,
126.644895127432)) ;
#134594=CARTESIAN_POINT('Ctrl Pts',(-30.4294392941911,13.889109539137,126.731888107809)) ;
#134595=CARTESIAN_POINT('Ctrl Pts',(-30.47077570761,14.1334576219234,126.885811226843)) ;
#134596=CARTESIAN_POINT('Ctrl Pts',(-30.53102912446,14.3262010857029,127.094865661672)) ;
#134597=CARTESIAN_POINT('Ctrl Pts',(-30.6058078949067,14.4552702241494,
127.346574791049)) ;
#134598=CARTESIAN_POINT('Ctrl Pts',(-30.6883760016807,14.5094659873619,
127.620923977953)) ;
#134599=CARTESIAN_POINT('Ctrl Pts',(-30.7718896570381,14.48627928254,127.897878479629)) ;
#134600=CARTESIAN_POINT('Ctrl Pts',(-30.8505404170833,14.3867194330965,
128.16082928885)) ;
#134601=CARTESIAN_POINT('Ctrl Pts',(-30.9172652518935,14.2183273389604,
128.388850744567)) ;
#134602=CARTESIAN_POINT('Ctrl Pts',(-30.966927867041,13.9922441011096,128.567141543632)) ;
#134603=CARTESIAN_POINT('Ctrl Pts',(-30.9948429554227,13.7260908863955,
128.681785518138)) ;
#134604=CARTESIAN_POINT('Ctrl Pts',(-30.9986761317404,13.4392990683917,
128.725970798859)) ;
#134605=CARTESIAN_POINT('Ctrl Pts',(-30.9771754995003,13.1491383926391,
128.696410048975)) ;
#134606=CARTESIAN_POINT('Ctrl Pts',(-30.9313862314932,12.880138144259,128.595705294773)) ;
#134607=CARTESIAN_POINT('Ctrl Pts',(-30.8633741700187,12.6488312040692,
128.430267551873)) ;
#134608=CARTESIAN_POINT('Ctrl Pts',(-30.7783096718615,12.4746173052797,
128.214724190605)) ;
#134609=CARTESIAN_POINT('Ctrl Pts',(-30.6802839201009,12.3669410581914,
127.961566303494)) ;
#134610=CARTESIAN_POINT('Ctrl Pts',(-30.5761954681339,12.3355244467329,
127.690674965918)) ;
#134611=CARTESIAN_POINT('Ctrl Pts',(-30.4731987242308,12.3818824637266,
127.42284013735)) ;
#134612=CARTESIAN_POINT('Ctrl Pts',(-30.3773601675738,12.502442440452,127.175947943775)) ;
#134613=CARTESIAN_POINT('Ctrl Pts',(-30.2945593439143,12.6900860359651,
126.967322197996)) ;
#134614=CARTESIAN_POINT('Ctrl Pts',(-30.2309201264915,12.9290693621117,
126.814464075625)) ;
#134615=CARTESIAN_POINT('Ctrl Pts',(-30.1896011311781,13.2033802627449,
126.726833819823)) ;
#134616=CARTESIAN_POINT('Ctrl Pts',(-30.1729187517655,13.493885424346,126.711224329232)) ;
#134617=CARTESIAN_POINT('Ctrl Pts',(-30.1814818466642,13.7798208359641,
126.769425110779)) ;
#134618=CARTESIAN_POINT('Ctrl Pts',(-30.2139166442141,14.0398147256928,
126.897315524147)) ;
#134619=CARTESIAN_POINT('Ctrl Pts',(-30.2672327260932,14.2555980954836,
127.086230738633)) ;
#134620=CARTESIAN_POINT('Ctrl Pts',(-30.3364241626342,14.4112165057251,
127.321355815591)) ;
#134621=CARTESIAN_POINT('Ctrl Pts',(-30.4169483545396,14.4969135755094,
127.589920286704)) ;
#134622=CARTESIAN_POINT('Ctrl Pts',(-30.5006568417281,14.5049696810031,
127.867411820872)) ;
#134623=CARTESIAN_POINT('Ctrl Pts',(-30.5821059141925,14.4360249735447,
128.13846691764)) ;
#134624=CARTESIAN_POINT('Ctrl Pts',(-30.6543269887437,14.2945754362065,
128.382542123477)) ;
#134625=CARTESIAN_POINT('Ctrl Pts',(-30.7116365732865,14.0897548858671,
128.583199406406)) ;
#134626=CARTESIAN_POINT('Ctrl Pts',(-30.7486474004249,13.8387001375239,
128.724327683098)) ;
#134627=CARTESIAN_POINT('Ctrl Pts',(-30.7626160375506,13.5574044598577,
128.79823198023)) ;
#134628=CARTESIAN_POINT('Ctrl Pts',(-30.751280169492,13.2644130009093,128.798450590054)) ;
#134629=CARTESIAN_POINT('Ctrl Pts',(-30.7152762753897,12.9862195730077,
128.726198614227)) ;
#134630=CARTESIAN_POINT('Ctrl Pts',(-30.6559255495121,12.7371111819008,
128.586013158079)) ;
#134631=CARTESIAN_POINT('Ctrl Pts',(-30.5772199975952,12.5380203242925,
128.389149798631)) ;
#134632=CARTESIAN_POINT('Ctrl Pts',(-30.4833480932253,12.4015272632005,
128.148171071429)) ;
#134633=CARTESIAN_POINT('Ctrl Pts',(-30.3812924082162,12.3389470103484,
127.883098879055)) ;
#134634=CARTESIAN_POINT('Ctrl Pts',(-30.2769531606877,12.3537864997403,
127.611426962061)) ;
#134635=CARTESIAN_POINT('Ctrl Pts',(-30.1774142848297,12.4449099176858,
127.353712328041)) ;
#134636=CARTESIAN_POINT('Ctrl Pts',(-30.0884196313121,12.6072327563546,
127.127011108624)) ;
#134637=CARTESIAN_POINT('Ctrl Pts',(-30.0168944583603,12.8259751420657,
126.950999128042)) ;
#134638=CARTESIAN_POINT('Ctrl Pts',(-29.9658131020968,13.0894865209779,
126.835020394129)) ;
#134639=CARTESIAN_POINT('Ctrl Pts',(-29.9390402950618,13.3763086244584,
126.789949510195)) ;
#134640=CARTESIAN_POINT('Ctrl Pts',(-29.9374976893148,13.666102426872,126.818551688385)) ;
#134641=CARTESIAN_POINT('Ctrl Pts',(-29.9603659689101,13.9378774393092,
126.918366530385)) ;
#134642=CARTESIAN_POINT('Ctrl Pts',(-30.0058557147277,14.174793298913,127.084558461599)) ;
#134643=CARTESIAN_POINT('Ctrl Pts',(-30.0690738202602,14.355667987911,127.302193672896)) ;
#134644=CARTESIAN_POINT('Ctrl Pts',(-30.1455851444044,14.4711053294092,
127.558860146817)) ;
#134645=CARTESIAN_POINT('Ctrl Pts',(-30.2290907276294,14.511170979715,127.836014853784)) ;
#134646=CARTESIAN_POINT('Ctrl Pts',(-30.3124346958538,14.4729025341711,
128.112614820692)) ;
#134647=CARTESIAN_POINT('Ctrl Pts',(-30.3888326028229,14.3605014183323,
128.368750566373)) ;
#134648=CARTESIAN_POINT('Ctrl Pts',(-30.4531791538599,14.1789799497678,
128.590078616567)) ;
#134649=CARTESIAN_POINT('Ctrl Pts',(-30.4986908853725,13.9453130755044,
128.756011357139)) ;
#134650=CARTESIAN_POINT('Ctrl Pts',(-30.5223367702664,13.673613297581,128.858202384461)) ;
#134651=CARTESIAN_POINT('Ctrl Pts',(-30.5214927257582,13.3843416477693,
128.888796839614)) ;
#134652=CARTESIAN_POINT('Ctrl Pts',(-30.4951356796959,13.0956424787648,
128.845131685907)) ;
#134653=CARTESIAN_POINT('Ctrl Pts',(-30.4451353943437,12.8335787485534,
128.73200501772)) ;
#134654=CARTESIAN_POINT('Ctrl Pts',(-30.3735874311193,12.6116522531053,
128.556195762552)) ;
#134655=CARTESIAN_POINT('Ctrl Pts',(-30.2853579635812,12.4486058050818,
128.33155990322)) ;
#134656=CARTESIAN_POINT('Ctrl Pts',(-30.1858663129506,12.3551665981467,
128.074050595748)) ;
#134657=CARTESIAN_POINT('Ctrl Pts',(-30.0815496988783,12.3383111368361,
127.802444396815)) ;
#134658=CARTESIAN_POINT('Ctrl Pts',(-29.9791399961725,12.3991318667188,
127.536410522558)) ;
#134659=CARTESIAN_POINT('Ctrl Pts',(-29.885250975789,12.5336133546432,127.2952913997)) ;
#134660=CARTESIAN_POINT('Ctrl Pts',(-29.8062098846917,12.7304747525644,
127.097365942919)) ;
#134661=CARTESIAN_POINT('Ctrl Pts',(-29.7459166115697,12.9801493565206,
126.954643707808)) ;
#134662=CARTESIAN_POINT('Ctrl Pts',(-29.7094981424688,13.2569930870622,
126.881074054437)) ;
#134663=CARTESIAN_POINT('Ctrl Pts',(-29.697485321225,13.5493201067258,126.879249155707)) ;
#134664=CARTESIAN_POINT('Ctrl Pts',(-29.7107148915496,13.8310609228274,
126.950973130347)) ;
#134665=CARTESIAN_POINT('Ctrl Pts',(-29.7473686079901,14.0843638099265,
127.091228525209)) ;
#134666=CARTESIAN_POINT('Ctrl Pts',(-29.8039983073089,14.2896244491401,
127.289751241016)) ;
#134667=CARTESIAN_POINT('Ctrl Pts',(-29.8758248177242,14.4330063116879,
127.5326649792)) ;
#134668=CARTESIAN_POINT('Ctrl Pts',(-29.9571776043441,14.5042107415309,
127.803464708327)) ;
#134669=CARTESIAN_POINT('Ctrl Pts',(-30.0412713276901,14.4979449999679,
128.082232149485)) ;
#134670=CARTESIAN_POINT('Ctrl Pts',(-30.121694639328,14.4144601779744,128.350375838408)) ;
#134671=CARTESIAN_POINT('Ctrl Pts',(-30.1915790917938,14.2595209902124,
128.587713560571)) ;
#134672=CARTESIAN_POINT('Ctrl Pts',(-30.2450076010872,14.046214919979,128.776755103724)) ;
#134673=CARTESIAN_POINT('Ctrl Pts',(-30.2780878046331,13.7868053449528,
128.906585374679)) ;
#134674=CARTESIAN_POINT('Ctrl Pts',(-30.2872906950602,13.5027357390144,
128.966484763682)) ;
#134675=CARTESIAN_POINT('Ctrl Pts',(-30.2713500951273,13.2114164567146,
128.953122045362)) ;
#134676=CARTESIAN_POINT('Ctrl Pts',(-30.230627814723,12.9359342983456,128.86728322249)) ;
#134677=CARTESIAN_POINT('Ctrl Pts',(-30.1672447422047,12.6951562018299,
128.715288751686)) ;
#134678=CARTESIAN_POINT('Ctrl Pts',(-30.0854978465419,12.5073061272103,
128.509491429827)) ;
#134679=CARTESIAN_POINT('Ctrl Pts',(-29.9896882822811,12.3841592686752,
128.262793679839)) ;
#134680=CARTESIAN_POINT('Ctrl Pts',(-29.8866361087517,12.3356200239572,
127.994841190901)) ;
#134681=CARTESIAN_POINT('Ctrl Pts',(-29.7820423738734,12.3655842279676,
127.722626897302)) ;
#134682=CARTESIAN_POINT('Ctrl Pts',(-29.6846378874882,12.4702048591763,
127.470973299483)) ;
#134683=CARTESIAN_POINT('Ctrl Pts',(-29.5982444318826,12.6448837976238,
127.251934053335)) ;
#134684=CARTESIAN_POINT('Ctrl Pts',(-29.530484788473,12.872508423284,127.086857758343)) ;
#134685=CARTESIAN_POINT('Ctrl Pts',(-29.4836133061575,13.1434988331289,
126.983345728084)) ;
#134686=CARTESIAN_POINT('Ctrl Pts',(-29.4617927517553,13.4301737780494,
126.952467269919)) ;
#134687=CARTESIAN_POINT('Ctrl Pts',(-29.4647728375027,13.7187795914099,
126.994328449619)) ;
#134688=CARTESIAN_POINT('Ctrl Pts',(-29.4924039666026,13.9870154433738,
127.108324446431)) ;
#134689=CARTESIAN_POINT('Ctrl Pts',(-29.5411722729436,14.2124398345738,
127.283727368873)) ;
#134690=CARTESIAN_POINT('Ctrl Pts',(-29.6075895922723,14.3830654461858,
127.510923381855)) ;
#134691=CARTESIAN_POINT('Ctrl Pts',(-29.6859780654117,14.4846609541733,
127.773091506423)) ;
#134692=CARTESIAN_POINT('Ctrl Pts',(-29.7699711987632,14.5097913616969,
128.051659371141)) ;
#134693=CARTESIAN_POINT('Ctrl Pts',(-29.8521599614632,14.4576093080194,
128.324704513275)) ;
#134694=CARTESIAN_POINT('Ctrl Pts',(-29.9273378651692,14.3304831317374,
128.57761366537)) ;
#134695=CARTESIAN_POINT('Ctrl Pts',(-29.9881011678196,14.1386183822934,
128.788232639006)) ;
#134696=CARTESIAN_POINT('Ctrl Pts',(-30.0298088081978,13.8965846856625,
128.943079017119)) ;
#134697=CARTESIAN_POINT('Ctrl Pts',(-30.048987740085,13.6198365630073,129.032230754272)) ;
#134698=CARTESIAN_POINT('Ctrl Pts',(-30.0433213484704,13.3288844737818,
129.048809941996)) ;
#134699=CARTESIAN_POINT('Ctrl Pts',(-30.0124680035273,13.0447399832046,
128.991813037362)) ;
#134700=CARTESIAN_POINT('Ctrl Pts',(-29.958162147996,12.7881836368688,128.866220633411)) ;
#134701=CARTESIAN_POINT('Ctrl Pts',(-29.8827371039613,12.5755910115287,
128.67919720058)) ;
#134702=CARTESIAN_POINT('Ctrl Pts',(-29.7923817501949,12.4257574465567,
128.448186718166)) ;
#134703=CARTESIAN_POINT('Ctrl Pts',(-29.6914548654442,12.3460112405744,
128.186501449005)) ;
#134704=CARTESIAN_POINT('Ctrl Pts',(-29.5867020660159,12.3439532504127,
127.913710488866)) ;
#134705=CARTESIAN_POINT('Ctrl Pts',(-29.485666657119,12.4188218900739,127.651602416161)) ;
#134706=CARTESIAN_POINT('Ctrl Pts',(-29.3936759004092,12.5668341062151,
127.416175460721)) ;
#134707=CARTESIAN_POINT('Ctrl Pts',(-29.3182301931701,12.7739565310488,
127.2286723812)) ;
#134708=CARTESIAN_POINT('Ctrl Pts',(-29.2623086088496,13.0292275295923,
127.098504241357)) ;
#134709=CARTESIAN_POINT('Ctrl Pts',(-29.2301243830033,13.3121167714202,
127.037580467898)) ;
#134710=CARTESIAN_POINT('Ctrl Pts',(-29.2229734795966,13.6036711588795,
127.049873651472)) ;
#134711=CARTESIAN_POINT('Ctrl Pts',(-29.2408639834952,13.8822010088686,
127.135317168003)) ;
#134712=CARTESIAN_POINT('Ctrl Pts',(-29.2814175857852,14.126534024312,127.286789452504)) ;
#134713=CARTESIAN_POINT('Ctrl Pts',(-29.341269933413,14.3215277156221,127.494747226261)) ;
#134714=CARTESIAN_POINT('Ctrl Pts',(-29.4156496701704,14.4523872469144,
127.745252022521)) ;
#134715=CARTESIAN_POINT('Ctrl Pts',(-29.4979993749135,14.509081269933,128.018936330148)) ;
#134716=CARTESIAN_POINT('Ctrl Pts',(-29.5821194390776,14.4877530584647,
128.297884507417)) ;
#134717=CARTESIAN_POINT('Ctrl Pts',(-29.6605015766084,14.3906972492053,
128.559841528178)) ;
#134718=CARTESIAN_POINT('Ctrl Pts',(-29.7277325620602,14.2242127265294,
128.789368837068)) ;
#134719=CARTESIAN_POINT('Ctrl Pts',(-29.7778622908604,14.0000453961231,
128.968956847515)) ;
#134720=CARTESIAN_POINT('Ctrl Pts',(-29.8065930602879,13.7349941187306,
129.085980593616)) ;
#134721=CARTESIAN_POINT('Ctrl Pts',(-29.8110647581583,13.4462938086935,
129.132290262238)) ;
#134722=CARTESIAN_POINT('Ctrl Pts',(-29.7905149481192,13.1586524064852,
129.105179558969)) ;
#134723=CARTESIAN_POINT('Ctrl Pts',(-29.7450251194424,12.8863235925418,
129.005657518442)) ;
#134724=CARTESIAN_POINT('Ctrl Pts',(-29.6779688870286,12.6553854575325,
128.842782884932)) ;
#134725=CARTESIAN_POINT('Ctrl Pts',(-29.5932822353585,12.4787538591612,
128.628403260321)) ;
#134726=CARTESIAN_POINT('Ctrl Pts',(-29.4951432611704,12.3688114822916,
128.375032108495)) ;
#134727=CARTESIAN_POINT('Ctrl Pts',(-29.3915755638739,12.3354319136936,
128.105522888968)) ;
#134728=CARTESIAN_POINT('Ctrl Pts',(-29.2883737439491,12.3792576310417,
127.83711019449)) ;
#134729=CARTESIAN_POINT('Ctrl Pts',(-29.1917010872287,12.4988398999205,
127.587984309591)) ;
#134730=CARTESIAN_POINT('Ctrl Pts',(-29.1090972687786,12.6835118512005,
127.379683329034)) ;
#134731=CARTESIAN_POINT('Ctrl Pts',(-29.0446608613966,12.9214923912795,
127.224563683631)) ;
#134732=CARTESIAN_POINT('Ctrl Pts',(-29.0026163941945,13.1954916424955,
127.134859426664)) ;
#134733=CARTESIAN_POINT('Ctrl Pts',(-28.985230945197,13.4865485670219,127.117276574287)) ;
#134734=CARTESIAN_POINT('Ctrl Pts',(-28.9931808891691,13.772471589557,127.173641275195)) ;
#134735=CARTESIAN_POINT('Ctrl Pts',(-29.0248180797672,14.0322259092952,
127.299049560001)) ;
#134736=CARTESIAN_POINT('Ctrl Pts',(-29.0774225647813,14.2496185339524,
127.485847881482)) ;
#134737=CARTESIAN_POINT('Ctrl Pts',(-29.1466584272716,14.4079186586772,
127.721302692546)) ;
#134738=CARTESIAN_POINT('Ctrl Pts',(-29.2262609733389,14.495128940057,127.986882942297)) ;
#134739=CARTESIAN_POINT('Ctrl Pts',(-29.310377688868,14.5060206783235,128.265744239721)) ;
#134740=CARTESIAN_POINT('Ctrl Pts',(-29.3922415681972,14.4388851972431,
128.538108177024)) ;
#134741=CARTESIAN_POINT('Ctrl Pts',(-29.4648367940965,14.2990479598781,
128.783307296558)) ;
#134742=CARTESIAN_POINT('Ctrl Pts',(-29.5224591681686,14.096277092635,128.984789687897)) ;
#134743=CARTESIAN_POINT('Ctrl Pts',(-29.5601633246064,13.8463552274942,
129.12795060112)) ;
#134744=CARTESIAN_POINT('Ctrl Pts',(-29.5747316968106,13.5643762793268,
129.203747316631)) ;
#134745=CARTESIAN_POINT('Ctrl Pts',(-29.5643172687888,13.2747380866486,
129.206268472805)) ;
#134746=CARTESIAN_POINT('Ctrl Pts',(-29.5288291438255,12.9934296976024,
129.135814296567)) ;
#134747=CARTESIAN_POINT('Ctrl Pts',(-29.470171863856,12.7438068041656,128.99757323151)) ;
#134748=CARTESIAN_POINT('Ctrl Pts',(-29.391803285665,12.5426943442427,128.801768222048)) ;
#134749=CARTESIAN_POINT('Ctrl Pts',(-29.2986131391391,12.4046936236787,
128.56265775762)) ;
#134750=CARTESIAN_POINT('Ctrl Pts',(-29.1964773761958,12.3396331759052,
128.297435830634)) ;
#134751=CARTESIAN_POINT('Ctrl Pts',(-29.092230590555,12.3522550875064,128.025991131613)) ;
#134752=CARTESIAN_POINT('Ctrl Pts',(-28.9924608185787,12.441158614988,127.767604009206)) ;
#134753=CARTESIAN_POINT('Ctrl Pts',(-28.9030933450802,12.6013769713038,
127.539790029494)) ;
#134754=CARTESIAN_POINT('Ctrl Pts',(-28.8308886096015,12.819071640269,127.361858709555)) ;
#134755=CARTESIAN_POINT('Ctrl Pts',(-28.779280341327,13.0807346140254,127.244233442709)) ;
#134756=CARTESIAN_POINT('Ctrl Pts',(-28.7517055757331,13.3675408612144,
127.196874862189)) ;
#134757=CARTESIAN_POINT('Ctrl Pts',(-28.7493257047856,13.6570979280699,
127.222968219409)) ;
#134758=CARTESIAN_POINT('Ctrl Pts',(-28.7718142821641,13.9319893911641,
127.321979864566)) ;
#134759=CARTESIAN_POINT('Ctrl Pts',(-28.8162456944187,14.1676085258846,
127.484711805867)) ;
#134760=CARTESIAN_POINT('Ctrl Pts',(-28.8794392120634,14.3519029604138,
127.702543293248)) ;
#134761=CARTESIAN_POINT('Ctrl Pts',(-28.955521536148,14.4687263868581,127.957864396171)) ;
#134762=CARTESIAN_POINT('Ctrl Pts',(-29.0386446837284,14.5110206744739,
128.233803590714)) ;
#134763=CARTESIAN_POINT('Ctrl Pts',(-29.1220480184099,14.4754839101951,
128.510547823415)) ;
#134764=CARTESIAN_POINT('Ctrl Pts',(-29.1992609632459,14.3641243881349,
128.769313204063)) ;
#134765=CARTESIAN_POINT('Ctrl Pts',(-29.2634796257756,14.1859981150162,
128.989963010774)) ;
#134766=CARTESIAN_POINT('Ctrl Pts',(-29.309906743687,13.9527739629267,129.158738849017)) ;
#134767=CARTESIAN_POINT('Ctrl Pts',(-29.3342115703911,13.6818171869407,
129.262851136394)) ;
#134768=CARTESIAN_POINT('Ctrl Pts',(-29.3340473631818,13.3923456599437,
129.295485666288)) ;
#134769=CARTESIAN_POINT('Ctrl Pts',(-29.3085669103323,13.1044625348289,
129.254236375475)) ;
#134770=CARTESIAN_POINT('Ctrl Pts',(-29.258986211392,12.8400820200563,129.142508243958)) ;
#134771=CARTESIAN_POINT('Ctrl Pts',(-29.1881542029012,12.6174283224968,
128.968693652698)) ;
#134772=CARTESIAN_POINT('Ctrl Pts',(-29.1002100971169,12.4521814963559,
128.744946986999)) ;
#134773=CARTESIAN_POINT('Ctrl Pts',(-29.0009103649547,12.3567835155047,
128.48800496993)) ;
#134774=CARTESIAN_POINT('Ctrl Pts',(-28.896925987083,12.3377092271658,128.21727920025)) ;
#134775=CARTESIAN_POINT('Ctrl Pts',(-28.7942667965697,12.3962076032604,
127.950545837014)) ;
#134776=CARTESIAN_POINT('Ctrl Pts',(-28.6998220504126,12.5290432373042,
127.70787965737)) ;
#134777=CARTESIAN_POINT('Ctrl Pts',(-28.6204061898145,12.7244085230837,
127.508847094626)) ;
#134778=CARTESIAN_POINT('Ctrl Pts',(-28.559819094265,12.9709500550387,127.365030411237)) ;
#134779=CARTESIAN_POINT('Ctrl Pts',(-28.5223002592329,13.2494402817627,
127.288528530129)) ;
#134780=CARTESIAN_POINT('Ctrl Pts',(-28.5097189788881,13.5418967084717,
127.285058220228)) ;
#134781=CARTESIAN_POINT('Ctrl Pts',(-28.5222097719137,13.8230883914708,
127.354499660829)) ;
#134782=CARTESIAN_POINT('Ctrl Pts',(-28.5582144837367,14.0775910910953,
127.492866930045)) ;
#134783=CARTESIAN_POINT('Ctrl Pts',(-28.6142444612186,14.2842118886259,
127.689596183375)) ;
#134784=CARTESIAN_POINT('Ctrl Pts',(-28.6857946550641,14.4299775435325,
127.931754504999)) ;
#134785=CARTESIAN_POINT('Ctrl Pts',(-28.7673480084958,14.503331032243,128.203286809695)) ;
#134786=CARTESIAN_POINT('Ctrl Pts',(-28.8509261449003,14.4992417837061,
128.480336479146)) ;
#134787=CARTESIAN_POINT('Ctrl Pts',(-28.9318023648984,14.4177939822546,
128.749907191947)) ;
#134788=CARTESIAN_POINT('Ctrl Pts',(-29.001910688641,14.2650806147523,128.987818507409)) ;
#134789=CARTESIAN_POINT('Ctrl Pts',(-29.0559489688668,14.0529681509037,
129.178698338362)) ;
#134790=CARTESIAN_POINT('Ctrl Pts',(-29.0896354038435,13.7955270319932,
129.310187588582)) ;
#134791=CARTESIAN_POINT('Ctrl Pts',(-29.099611948193,13.5095709535078,129.372622374006)) ;
#134792=CARTESIAN_POINT('Ctrl Pts',(-29.0842585907111,13.2189036520177,
129.360885383851)) ;
#134793=CARTESIAN_POINT('Ctrl Pts',(-29.0443620584725,12.9437120966298,
129.277345257376)) ;
#134794=CARTESIAN_POINT('Ctrl Pts',(-28.9817282559493,12.7018113312773,
129.127496651977)) ;
#134795=CARTESIAN_POINT('Ctrl Pts',(-28.900103185758,12.5115374792667,128.922195104015)) ;
#134796=CARTESIAN_POINT('Ctrl Pts',(-28.8047562754635,12.3865362509785,
128.676787399727)) ;
#134797=CARTESIAN_POINT('Ctrl Pts',(-28.7012853562746,12.3360647683775,
128.40778833087)) ;
#134798=CARTESIAN_POINT('Ctrl Pts',(-28.5980648305844,12.3630945002041,
128.139111767235)) ;
#134799=CARTESIAN_POINT('Ctrl Pts',(-28.4992221941751,12.4665769548229,
127.883658010127)) ;
#134800=CARTESIAN_POINT('Ctrl Pts',(-28.4131594840602,12.637873730405,127.665272376222)) ;
#134801=CARTESIAN_POINT('Ctrl Pts',(-28.3441687124707,12.8661806742055,
127.496923307267)) ;
#134802=CARTESIAN_POINT('Ctrl Pts',(-28.2971179753842,13.1333277515124,
127.392512752519)) ;
#134803=CARTESIAN_POINT('Ctrl Pts',(-28.2742141661044,13.4221934836715,
127.358771264461)) ;
#134804=CARTESIAN_POINT('Ctrl Pts',(-28.2765820238562,13.7107571318464,
127.398801174816)) ;
#134805=CARTESIAN_POINT('Ctrl Pts',(-28.3034962448371,13.9798563780996,
127.510697252844)) ;
#134806=CARTESIAN_POINT('Ctrl Pts',(-28.3518348917567,14.2070905580459,
127.684913382421)) ;
#134807=CARTESIAN_POINT('Ctrl Pts',(-28.417736051092,14.3790287482914,127.910539859451)) ;
#134808=CARTESIAN_POINT('Ctrl Pts',(-28.4956163030634,14.4826462514907,
128.171126340958)) ;
#134809=CARTESIAN_POINT('Ctrl Pts',(-28.5798455524846,14.5101765749395,
128.450506444325)) ;
#134810=CARTESIAN_POINT('Ctrl Pts',(-28.66200834704,14.4602521093363,128.723409993032)) ;
#134811=CARTESIAN_POINT('Ctrl Pts',(-28.7375813833395,14.3349863303821,
128.977516850491)) ;
#134812=CARTESIAN_POINT('Ctrl Pts',(-28.7985628235098,14.1459036519263,
129.188607444567)) ;
#134813=CARTESIAN_POINT('Ctrl Pts',(-28.8411540818564,13.9042674567381,
129.346179660859)) ;
#134814=CARTESIAN_POINT('Ctrl Pts',(-28.8610016097192,13.6274934121279,
129.437359596521)) ;
#134815=CARTESIAN_POINT('Ctrl Pts',(-28.8560349310886,13.3375401227482,
129.455886266098)) ;
#134816=CARTESIAN_POINT('Ctrl Pts',(-28.8260275084833,13.0529656397982,
129.401339308127)) ;
#134817=CARTESIAN_POINT('Ctrl Pts',(-28.7718240751871,12.793542004979,129.276308893705)) ;
#134818=CARTESIAN_POINT('Ctrl Pts',(-28.69758931411,12.5815361452067,129.09244647551)) ;
#134819=CARTESIAN_POINT('Ctrl Pts',(-28.607191982818,12.4287258471182,128.861490887195)) ;
#134820=CARTESIAN_POINT('Ctrl Pts',(-28.5062114306704,12.3470719994747,
128.599714513405)) ;
#134821=CARTESIAN_POINT('Ctrl Pts',(-28.4016831964791,12.3430683223392,
128.327512526391)) ;
#134822=CARTESIAN_POINT('Ctrl Pts',(-28.3008205475048,12.4155936091128,
128.065797526111)) ;
#134823=CARTESIAN_POINT('Ctrl Pts',(-28.2086887982306,12.5608875783812,
127.829855784513)) ;
#134824=CARTESIAN_POINT('Ctrl Pts',(-28.1322966051425,12.7672957855937,
127.639749496506)) ;
#134825=CARTESIAN_POINT('Ctrl Pts',(-28.0757288054588,13.0219896288371,
127.507742576733)) ;
#134826=CARTESIAN_POINT('Ctrl Pts',(-28.0429540969002,13.3035436342973,
127.44499916588)) ;
#134827=CARTESIAN_POINT('Ctrl Pts',(-28.0350385580784,13.5948422510341,
127.455024273178)) ;
#134828=CARTESIAN_POINT('Ctrl Pts',(-28.0521494910461,13.8739529691167,
127.538171398898)) ;
#134829=CARTESIAN_POINT('Ctrl Pts',(-28.0921989061459,14.1203174233417,
127.688276422386)) ;
#134830=CARTESIAN_POINT('Ctrl Pts',(-28.151557364416,14.3167168643634,127.894769419474)) ;
#134831=CARTESIAN_POINT('Ctrl Pts',(-28.2253962663715,14.4494066861711,
128.14361033343)) ;
#134832=CARTESIAN_POINT('Ctrl Pts',(-28.3077059790347,14.5084702688582,
128.41722565312)) ;
#134833=CARTESIAN_POINT('Ctrl Pts',(-28.3916026412673,14.489700746972,128.695408809309)) ;
#134834=CARTESIAN_POINT('Ctrl Pts',(-28.4706094716546,14.3946106074975,
128.959339303664)) ;
#134835=CARTESIAN_POINT('Ctrl Pts',(-28.5383385063881,14.2294635345246,
129.190381875795)) ;
#134836=CARTESIAN_POINT('Ctrl Pts',(-28.5888615094772,14.0073333887475,
129.371024757805)) ;
#134837=CARTESIAN_POINT('Ctrl Pts',(-28.6182752167583,13.7435828448799,
129.490009369002)) ;
#134838=CARTESIAN_POINT('Ctrl Pts',(-28.6235344183767,13.454824745877,129.538667492509)) ;
#134839=CARTESIAN_POINT('Ctrl Pts',(-28.6035941708859,13.1663898496403,
129.513405963783)) ;
#134840=CARTESIAN_POINT('Ctrl Pts',(-28.5591016772346,12.8948251888563,
129.416595319443)) ;
#134841=CARTESIAN_POINT('Ctrl Pts',(-28.4924613979654,12.6613614393991,
129.255069109059)) ;
#134842=CARTESIAN_POINT('Ctrl Pts',(-28.4079858158223,12.4827884864443,
129.041374692839)) ;
#134843=CARTESIAN_POINT('Ctrl Pts',(-28.3106810095428,12.3713198999723,
128.790256537741)) ;
#134844=CARTESIAN_POINT('Ctrl Pts',(-28.2071142233906,12.3351536539427,
128.520782151597)) ;
#134845=CARTESIAN_POINT('Ctrl Pts',(-28.1033170651269,12.3771106003778,
128.250789621036)) ;
#134846=CARTESIAN_POINT('Ctrl Pts',(-28.0070122936131,12.493746042562,128.002507073001)) ;
#134847=CARTESIAN_POINT('Ctrl Pts',(-27.9236042223444,12.6767291405437,
127.791947198724)) ;
#134848=CARTESIAN_POINT('Ctrl Pts',(-27.8582788554542,12.9147362953278,
127.634399931538)) ;
#134849=CARTESIAN_POINT('Ctrl Pts',(-27.8157639814054,13.1870897175325,
127.543206911709)) ;
#134850=CARTESIAN_POINT('Ctrl Pts',(-27.7976113632335,13.4771402294594,
127.523294837643)) ;
#134851=CARTESIAN_POINT('Ctrl Pts',(-27.8047562191335,13.7642376991577,
127.577383148529)) ;
#134852=CARTESIAN_POINT('Ctrl Pts',(-27.8359687279842,14.0261140050281,
127.701710177171)) ;
#134853=CARTESIAN_POINT('Ctrl Pts',(-27.8877875139809,14.2437566095146,
127.886037495367)) ;
#134854=CARTESIAN_POINT('Ctrl Pts',(-27.9566643830394,14.4043004510961,
128.12048462873)) ;
#134855=CARTESIAN_POINT('Ctrl Pts',(-28.0360570915207,14.4936451763547,
128.385451901082)) ;
#134856=CARTESIAN_POINT('Ctrl Pts',(-28.120129115805,14.5067755223083,128.664180642723)) ;
#134857=CARTESIAN_POINT('Ctrl Pts',(-28.2020346856407,14.4421251633059,
128.936606880987)) ;
#134858=CARTESIAN_POINT('Ctrl Pts',(-28.2751125216823,14.3039891726026,
129.183284767789)) ;
#134859=CARTESIAN_POINT('Ctrl Pts',(-28.3330260630189,14.1040922169467,
129.385445944809)) ;
#134860=CARTESIAN_POINT('Ctrl Pts',(-28.3716774412633,13.8535852347893,
129.531620171577)) ;
#134861=CARTESIAN_POINT('Ctrl Pts',(-28.3868553207156,13.5730952435811,
129.609080622274)) ;
#134862=CARTESIAN_POINT('Ctrl Pts',(-28.3771751540194,13.2829861782011,
129.613807074417)) ;
#134863=CARTESIAN_POINT('Ctrl Pts',(-28.3425095932928,13.0017737284941,
129.545666888846)) ;
#134864=CARTESIAN_POINT('Ctrl Pts',(-28.284301937165,12.7500890797144,129.408856898039)) ;
#134865=CARTESIAN_POINT('Ctrl Pts',(-28.2064572920802,12.5475577998432,
129.214559307957)) ;
#134866=CARTESIAN_POINT('Ctrl Pts',(-28.1135171544018,12.4075652478031,
128.976210428243)) ;
#134867=CARTESIAN_POINT('Ctrl Pts',(-28.0118850220544,12.3405227377109,
128.712349934362)) ;
#134868=CARTESIAN_POINT('Ctrl Pts',(-27.9073393263242,12.3506975715296,
128.440115510787)) ;
#134869=CARTESIAN_POINT('Ctrl Pts',(-27.8069898708441,12.438177489278,128.180166701549)) ;
#134870=CARTESIAN_POINT('Ctrl Pts',(-27.7177045614419,12.5958827964123,
127.952426644854)) ;
#134871=CARTESIAN_POINT('Ctrl Pts',(-27.6448174995369,12.8123887822574,
127.772559198421)) ;
#134872=CARTESIAN_POINT('Ctrl Pts',(-27.5925658802496,13.0732934241726,
127.653072879261)) ;
#134873=CARTESIAN_POINT('Ctrl Pts',(-27.5643119574423,13.3601444544887,
127.603779546763)) ;
#134874=CARTESIAN_POINT('Ctrl Pts',(-27.5613082454556,13.6487324697402,
127.627925538602)) ;
#134875=CARTESIAN_POINT('Ctrl Pts',(-27.5828722691528,13.9231969052117,
127.724074394844)) ;
#134876=CARTESIAN_POINT('Ctrl Pts',(-27.6269024064909,14.1616648845749,
127.885829090303)) ;
#134877=CARTESIAN_POINT('Ctrl Pts',(-27.6896598747405,14.3474885130478,
128.102376258084)) ;
#134878=CARTESIAN_POINT('Ctrl Pts',(-27.7653992680876,14.4664584587802,
128.356681964705)) ;
#134879=CARTESIAN_POINT('Ctrl Pts',(-27.8487981620875,14.5109046603937,
128.633576137683)) ;
#134880=CARTESIAN_POINT('Ctrl Pts',(-27.9318850392023,14.477538406395,128.909237750788)) ;
#134881=CARTESIAN_POINT('Ctrl Pts',(-28.0095052256554,14.3681997132881,
129.169245881706)) ;
#134882=CARTESIAN_POINT('Ctrl Pts',(-28.0741401659524,14.19161807787,129.391120281656)) ;
#134883=CARTESIAN_POINT('Ctrl Pts',(-28.1210449004513,13.9603524956053,
129.561209556167)) ;
#134884=CARTESIAN_POINT('Ctrl Pts',(-28.1460961632202,13.6895220911817,
129.667588782595)) ;
#134885=CARTESIAN_POINT('Ctrl Pts',(-28.1465838645101,13.4007319641459,
129.702076763037)) ;
#134886=CARTESIAN_POINT('Ctrl Pts',(-28.1219792750298,13.1132078283894,
129.663296512428)) ;
#134887=CARTESIAN_POINT('Ctrl Pts',(-28.072797303837,12.8466068578935,129.552900494661)) ;
#134888=CARTESIAN_POINT('Ctrl Pts',(-28.0028760663637,12.6236984730367,
129.381571768306)) ;
#134889=CARTESIAN_POINT('Ctrl Pts',(-27.9152289217031,12.4561011970055,
129.15875880179)) ;
#134890=CARTESIAN_POINT('Ctrl Pts',(-27.8163074914158,12.3585968124196,
128.902876316079)) ;
#134891=CARTESIAN_POINT('Ctrl Pts',(-27.7120492591559,12.3371246735504,
128.631455165304)) ;
#134892=CARTESIAN_POINT('Ctrl Pts',(-27.6093731664381,12.3935413485491,
128.364635405542)) ;
#134893=CARTESIAN_POINT('Ctrl Pts',(-27.5149001295544,12.5236723848828,
128.121769416389)) ;
#134894=CARTESIAN_POINT('Ctrl Pts',(-27.4346201824783,12.7179304240541,
127.920341279588)) ;
#134895=CARTESIAN_POINT('Ctrl Pts',(-27.3732833708595,12.9643000603806,
127.774449881944)) ;
#134896=CARTESIAN_POINT('Ctrl Pts',(-27.3353218805088,13.2410161239663,
127.696515666237)) ;
#134897=CARTESIAN_POINT('Ctrl Pts',(-27.3219345106549,13.5320326358814,
127.690536193544)) ;
#134898=CARTESIAN_POINT('Ctrl Pts',(-27.3336868555628,13.8151976332958,
127.757981771659)) ;
#134899=CARTESIAN_POINT('Ctrl Pts',(-27.3691045396702,14.070965110173,127.894657472177)) ;
#134900=CARTESIAN_POINT('Ctrl Pts',(-27.4247538548607,14.2795161854134,
128.090342542637)) ;
#134901=CARTESIAN_POINT('Ctrl Pts',(-27.495823154164,14.4266233568165,128.331023842141)) ;
#134902=CARTESIAN_POINT('Ctrl Pts',(-27.5766922115291,14.5021444966585,
128.600366276399)) ;
#134903=CARTESIAN_POINT('Ctrl Pts',(-27.6609223179021,14.5004799279669,
128.8795751742)) ;
#134904=CARTESIAN_POINT('Ctrl Pts',(-27.7417671934519,14.4210758361391,
129.14896837329)) ;
#134905=CARTESIAN_POINT('Ctrl Pts',(-27.8120265768946,14.2711637356508,
129.38719326095)) ;
#134906=CARTESIAN_POINT('Ctrl Pts',(-27.866891762874,14.0600320259714,129.580611011308)) ;
#134907=CARTESIAN_POINT('Ctrl Pts',(-27.9012411174026,13.8025046463563,
129.714162963611)) ;
#134908=CARTESIAN_POINT('Ctrl Pts',(-27.9118652501947,13.5194350300881,
129.778210865001)) ;
#134909=CARTESIAN_POINT('Ctrl Pts',(-27.8973675127668,13.227929848522,129.769057927685)) ;
#134910=CARTESIAN_POINT('Ctrl Pts',(-27.8581217638387,12.9514279979351,
129.687479679852)) ;
#134911=CARTESIAN_POINT('Ctrl Pts',(-27.7958487933346,12.7076270254922,
129.538792895781)) ;
#134912=CARTESIAN_POINT('Ctrl Pts',(-27.7150442368328,12.5164543914562,
129.335744778992)) ;
#134913=CARTESIAN_POINT('Ctrl Pts',(-27.6197799723084,12.3891143889345,
129.090666143106)) ;
#134914=CARTESIAN_POINT('Ctrl Pts',(-27.5169840616899,12.3364756158918,
128.823462340777)) ;
#134915=CARTESIAN_POINT('Ctrl Pts',(-27.4129425204162,12.3612642231578,
128.552629149903)) ;
#134916=CARTESIAN_POINT('Ctrl Pts',(-27.3139116309648,12.4629838840005,
128.296612691349)) ;
#134917=CARTESIAN_POINT('Ctrl Pts',(-27.2276350555539,12.6321971699934,
128.077535896234)) ;
#134918=CARTESIAN_POINT('Ctrl Pts',(-27.1581753164316,12.8584558798932,
127.907740199772)) ;
#134919=CARTESIAN_POINT('Ctrl Pts',(-27.1102193532803,13.1261648647243,
127.800864060768)) ;
#134920=CARTESIAN_POINT('Ctrl Pts',(-27.0867427780488,13.4141234552309,
127.765371910168)) ;
#134921=CARTESIAN_POINT('Ctrl Pts',(-27.088405263082,13.7023852342343,127.803282253112)) ;
#134922=CARTESIAN_POINT('Ctrl Pts',(-27.1144094066955,13.9714212012371,
127.912378068659)) ;
#134923=CARTESIAN_POINT('Ctrl Pts',(-27.1625636190418,14.202020081249,128.086338189894)) ;
#134924=CARTESIAN_POINT('Ctrl Pts',(-27.2279041571622,14.3750071736422,
128.310222999053)) ;
#134925=CARTESIAN_POINT('Ctrl Pts',(-27.3055089641359,14.4806351346196,
128.570006270221)) ;
#134926=CARTESIAN_POINT('Ctrl Pts',(-27.3892702869014,14.5105855297535,
128.847858683373)) ;
#134927=CARTESIAN_POINT('Ctrl Pts',(-27.4721256647169,14.4625550657111,
129.123019817885)) ;
#134928=CARTESIAN_POINT('Ctrl Pts',(-27.5475424958297,14.3400369417443,
129.376461860258)) ;
#134929=CARTESIAN_POINT('Ctrl Pts',(-27.6092868870231,14.1521957535254,
129.589908595948)) ;
#134930=CARTESIAN_POINT('Ctrl Pts',(-27.6524549950664,13.9116489154345,
129.749173070005)) ;
#134931=CARTESIAN_POINT('Ctrl Pts',(-27.6729767158619,13.6358544266559,
129.842295420114)) ;
#134932=CARTESIAN_POINT('Ctrl Pts',(-27.6687686357343,13.3459427675745,
129.863045715734)) ;
#134933=CARTESIAN_POINT('Ctrl Pts',(-27.6393546558192,13.0604649745041,
129.810291983176)) ;
#134934=CARTESIAN_POINT('Ctrl Pts',(-27.5861749748563,12.8015143832803,
129.688047174148)) ;
#134935=CARTESIAN_POINT('Ctrl Pts',(-27.5122453552566,12.586871423154,129.505215644939)) ;
#134936=CARTESIAN_POINT('Ctrl Pts',(-27.4222257102063,12.4323032180318,
129.275353955494)) ;
#134937=CARTESIAN_POINT('Ctrl Pts',(-27.321814640165,12.348604012381,129.015131363742)) ;
#134938=CARTESIAN_POINT('Ctrl Pts',(-27.2172646277251,12.3418345254331,
128.742874357153)) ;
#134939=CARTESIAN_POINT('Ctrl Pts',(-27.1155991989799,12.4127257697425,
128.479021774659)) ;
#134940=CARTESIAN_POINT('Ctrl Pts',(-27.0235546029965,12.5554430365515,
128.24317434018)) ;
#134941=CARTESIAN_POINT('Ctrl Pts',(-26.946364611968,12.7608029240068,128.050846584327)) ;
#134942=CARTESIAN_POINT('Ctrl Pts',(-26.8892425932522,13.0143079229722,
127.917197312737)) ;
#134943=CARTESIAN_POINT('Ctrl Pts',(-26.8557397574038,13.2953661026702,
127.852335782128)) ;
#134944=CARTESIAN_POINT('Ctrl Pts',(-26.8471237684322,13.587499191953,127.86040257377)) ;
#134945=CARTESIAN_POINT('Ctrl Pts',(-26.8636409106043,13.8669338626205,
127.941791701437)) ;
#134946=CARTESIAN_POINT('Ctrl Pts',(-26.9028894020443,14.1134263503453,
128.089413302891)) ;
#134947=CARTESIAN_POINT('Ctrl Pts',(-26.9618864660315,14.3121780897716,
128.294946112899)) ;
#134948=CARTESIAN_POINT('Ctrl Pts',(-27.0356609756341,14.4470050265316,
128.543696981495)) ;
#134949=CARTESIAN_POINT('Ctrl Pts',(-27.1176846698481,14.5078086325279,
128.816414339099)) ;
#134950=CARTESIAN_POINT('Ctrl Pts',(-27.2013501944063,14.4913412737729,
129.093814747738)) ;
#134951=CARTESIAN_POINT('Ctrl Pts',(-27.2805727554514,14.3985299043882,
129.358365317732)) ;
#134952=CARTESIAN_POINT('Ctrl Pts',(-27.3487809879748,14.2353764928408,
129.590815975098)) ;
#134953=CARTESIAN_POINT('Ctrl Pts',(-27.4000923756535,14.0132824388172,
129.773951949604)) ;
#134954=CARTESIAN_POINT('Ctrl Pts',(-27.4299031588905,13.751770584179,129.893917739675)) ;
#134955=CARTESIAN_POINT('Ctrl Pts',(-27.4360065328396,13.4639004603942,
129.944990740374)) ;
#134956=CARTESIAN_POINT('Ctrl Pts',(-27.4166194504997,13.1736259559936,
129.921533138526)) ;
#134957=CARTESIAN_POINT('Ctrl Pts',(-27.3730557967721,12.9029494351804,
129.827230137503)) ;
#134958=CARTESIAN_POINT('Ctrl Pts',(-27.3068239081708,12.6670694829694,
129.667025348139)) ;
#134959=CARTESIAN_POINT('Ctrl Pts',(-27.2225807375648,12.4867414535482,
129.454064281963)) ;
#134960=CARTESIAN_POINT('Ctrl Pts',(-27.1260163205075,12.3736046950475,
129.204955161642)) ;
#134961=CARTESIAN_POINT('Ctrl Pts',(-27.0219531940928,12.3351061359291,
128.934221171249)) ;
#134962=CARTESIAN_POINT('Ctrl Pts',(-26.9187654991147,12.3747297412366,
128.665782677207)) ;
#134963=CARTESIAN_POINT('Ctrl Pts',(-26.8219192185406,12.4890530273647,
128.415981781108)) ;
#134964=CARTESIAN_POINT('Ctrl Pts',(-26.7375618368722,12.6718473822343,
128.20287552548)) ;
#134965=CARTESIAN_POINT('Ctrl Pts',(-26.6721408995713,12.9071471042355,
128.044830293244)) ;
#134966=CARTESIAN_POINT('Ctrl Pts',(-26.6288268693924,13.1791583633753,
127.951366546025)) ;
#134967=CARTESIAN_POINT('Ctrl Pts',(-26.6100146219695,13.4685703303894,
127.929472625113)) ;
#134968=CARTESIAN_POINT('Ctrl Pts',(-26.6163965606096,13.7556865610863,
127.981289936006)) ;
#134969=CARTESIAN_POINT('Ctrl Pts',(-26.6468365176563,14.0184520779736,
128.103328446011)) ;
#134970=CARTESIAN_POINT('Ctrl Pts',(-26.6983664732469,14.2386835545227,
128.286981099105)) ;
#134971=CARTESIAN_POINT('Ctrl Pts',(-26.7668561678463,14.4009245247973,
128.520283146029)) ;
#134972=CARTESIAN_POINT('Ctrl Pts',(-26.8462801396179,14.4923209079493,
128.785440445302)) ;
#134973=CARTESIAN_POINT('Ctrl Pts',(-26.9299042318789,14.5074993821674,
129.062691208225)) ;
#134974=CARTESIAN_POINT('Ctrl Pts',(-27.0123042045344,14.4446391320812,
129.336708219525)) ;
#134975=CARTESIAN_POINT('Ctrl Pts',(-27.0853285109314,14.309013886893,129.583057807955)) ;
#134976=CARTESIAN_POINT('Ctrl Pts',(-27.1438828659143,14.1104149351794,
129.787163074108)) ;
#134977=CARTESIAN_POINT('Ctrl Pts',(-27.1830524640317,13.8614588559076,
129.934789891105)) ;
#134978=CARTESIAN_POINT('Ctrl Pts',(-27.1989887778394,13.5819687002437,
130.014428956727)) ;
#134979=CARTESIAN_POINT('Ctrl Pts',(-27.1899960665713,13.2906279013141,
130.021303572167)) ;
#134980=CARTESIAN_POINT('Ctrl Pts',(-27.1559614540415,13.009243305788,129.95497149067)) ;
#134981=CARTESIAN_POINT('Ctrl Pts',(-27.0987240639522,12.7575168112921,
129.820836098485)) ;
#134982=CARTESIAN_POINT('Ctrl Pts',(-27.0211347642334,12.5525240138587,
129.627409702748)) ;
#134983=CARTESIAN_POINT('Ctrl Pts',(-26.9288019853003,12.4108770336832,
129.390743830787)) ;
#134984=CARTESIAN_POINT('Ctrl Pts',(-26.8269925769389,12.3412909140522,
129.126483822534)) ;
#134985=CARTESIAN_POINT('Ctrl Pts',(-26.7225678003105,12.3493861735078,
128.854556329981)) ;
#134986=CARTESIAN_POINT('Ctrl Pts',(-26.6222736426069,12.4342727909203,
128.594675298208)) ;
#134987=CARTESIAN_POINT('Ctrl Pts',(-26.5324245140866,12.5900489009072,
128.365332500197)) ;
#134988=CARTESIAN_POINT('Ctrl Pts',(-26.4587946173494,12.8056265995217,
128.183382042886)) ;
#134989=CARTESIAN_POINT('Ctrl Pts',(-26.4059966216722,13.0653848746049,
128.062274396553)) ;
#134990=CARTESIAN_POINT('Ctrl Pts',(-26.3770384247468,13.3504851063388,
128.01077693268)) ;
#134991=CARTESIAN_POINT('Ctrl Pts',(-26.3732580768289,13.6412798147236,
128.032889399786)) ;
#134992=CARTESIAN_POINT('Ctrl Pts',(-26.3941468859038,13.915548156852,128.126957619226)) ;
#134993=CARTESIAN_POINT('Ctrl Pts',(-26.4375236270793,14.1552942040558,
128.286796725341)) ;
#134994=CARTESIAN_POINT('Ctrl Pts',(-26.499786802166,14.3429101935435,128.501891901076)) ;
#134995=CARTESIAN_POINT('Ctrl Pts',(-26.5753221744753,14.4639893047867,
128.755644371512)) ;
#134996=CARTESIAN_POINT('Ctrl Pts',(-26.658258796401,14.5107279953385,129.031049167775)) ;
#134997=CARTESIAN_POINT('Ctrl Pts',(-26.7418770326506,14.4794893752074,
129.308446128137)) ;
#134998=CARTESIAN_POINT('Ctrl Pts',(-26.819410154467,14.3727211578977,129.56804219168)) ;
#134999=CARTESIAN_POINT('Ctrl Pts',(-26.884660652684,14.1977799584113,129.791786901947)) ;
#135000=CARTESIAN_POINT('Ctrl Pts',(-26.9321606344241,13.9680803032242,
129.963592933574)) ;
#135001=CARTESIAN_POINT('Ctrl Pts',(-26.9579703404882,13.6967826933105,
130.072347583536)) ;
#135002=CARTESIAN_POINT('Ctrl Pts',(-26.9591310030642,13.4094043760888,
130.108663362794)) ;
#135003=CARTESIAN_POINT('Ctrl Pts',(-26.935231210856,13.1212039321583,130.071985580596)) ;
#135004=CARTESIAN_POINT('Ctrl Pts',(-26.8869426549206,12.8546896237207,
129.964066829109)) ;
#135005=CARTESIAN_POINT('Ctrl Pts',(-26.8174482093006,12.6293810356165,
129.794091823838)) ;
#135006=CARTESIAN_POINT('Ctrl Pts',(-26.7297563031988,12.4594635396626,
129.571300039305)) ;
#135007=CARTESIAN_POINT('Ctrl Pts',(-26.6315768169788,12.3604529302704,
129.317412505758)) ;
#135008=CARTESIAN_POINT('Ctrl Pts',(-26.527041677516,12.3366695079855,129.045292118923)) ;
#135009=CARTESIAN_POINT('Ctrl Pts',(-26.4246632418904,12.3907630606801,
128.779202667163)) ;
#135010=CARTESIAN_POINT('Ctrl Pts',(-26.3296624090555,12.5187717527639,
128.534846855937)) ;
#135011=CARTESIAN_POINT('Ctrl Pts',(-26.2486292653153,12.7125553045139,
128.331370691531)) ;
#135012=CARTESIAN_POINT('Ctrl Pts',(-26.187290463919,12.9551208485313,128.185129058602)) ;
#135013=CARTESIAN_POINT('Ctrl Pts',(-26.1482420973643,13.2325620060974,
128.104210130242)) ;
#135014=CARTESIAN_POINT('Ctrl Pts',(-26.1341913899476,13.5243419796884,
128.096383572714)) ;
#135015=CARTESIAN_POINT('Ctrl Pts',(-26.1452118388481,13.8069926528057,
128.161574113629)) ;
#135016=CARTESIAN_POINT('Ctrl Pts',(-26.1799390075941,14.0639000199269,
128.296232665471)) ;
#135017=CARTESIAN_POINT('Ctrl Pts',(-26.2350489546991,14.2741558930926,
128.490347023028)) ;
#135018=CARTESIAN_POINT('Ctrl Pts',(-26.3059077450582,14.4234615625839,
128.730487186166)) ;
#135019=CARTESIAN_POINT('Ctrl Pts',(-26.386494169588,14.5011170686614,128.998961276038)) ;
#135020=CARTESIAN_POINT('Ctrl Pts',(-26.4710372754606,14.5013614779113,
129.279215621043)) ;
#135021=CARTESIAN_POINT('Ctrl Pts',(-26.5513450363698,14.4249956630962,
129.546727763435)) ;
#135022=CARTESIAN_POINT('Ctrl Pts',(-26.6226216620681,14.2760171565871,
129.788206158856)) ;
#135023=CARTESIAN_POINT('Ctrl Pts',(-26.6777858163634,14.0665442400002,
129.982426179449)) ;
#135024=CARTESIAN_POINT('Ctrl Pts',(-26.7127743428566,13.8110528410318,
130.117741076645)) ;
#135025=CARTESIAN_POINT('Ctrl Pts',(-26.7241069347589,13.5262786463887,
130.184114351317)) ;
#135026=CARTESIAN_POINT('Ctrl Pts',(-26.7103978253846,13.2368369901033,
130.177011615775)) ;
#135027=CARTESIAN_POINT('Ctrl Pts',(-26.6716560461567,12.9583255903659,
130.097075764209)) ;
#135028=CARTESIAN_POINT('Ctrl Pts',(-26.6103674672222,12.7145800096232,
129.95106877123)) ;
#135029=CARTESIAN_POINT('Ctrl Pts',(-26.5292783226885,12.5201730384604,
129.747494551372)) ;
#135030=CARTESIAN_POINT('Ctrl Pts',(-26.4353195353877,12.392297716127,129.505869698294)) ;
#135031=CARTESIAN_POINT('Ctrl Pts',(-26.3321003131888,12.3368042043637,
129.23762472755)) ;
#135032=CARTESIAN_POINT('Ctrl Pts',(-26.2283359448761,12.3594079574846,
128.967488898529)) ;
#135033=CARTESIAN_POINT('Ctrl Pts',(-26.1289374320057,12.4588426243277,
128.710432008687)) ;
#135034=CARTESIAN_POINT('Ctrl Pts',(-26.0421433826271,12.6263832935465,
128.489874381818)) ;
#135035=CARTESIAN_POINT('Ctrl Pts',(-25.9721170036289,12.8513078071139,
128.318433909601)) ;
#135036=CARTESIAN_POINT('Ctrl Pts',(-25.9235411833855,13.1175341941134,
128.209680256936)) ;
#135037=CARTESIAN_POINT('Ctrl Pts',(-25.8992723616796,13.4059954970849,
128.171974342421)) ;
#135038=CARTESIAN_POINT('Ctrl Pts',(-25.9001789667653,13.6942419645787,
128.207632461566)) ;
#135039=CARTESIAN_POINT('Ctrl Pts',(-25.9258216003677,13.9656571359195,
128.31589284879)) ;
#135040=CARTESIAN_POINT('Ctrl Pts',(-25.9727492712161,14.1945698215837,
128.485818180082)) ;
#135041=CARTESIAN_POINT('Ctrl Pts',(-26.0380351219601,14.3711224528334,
128.709801837872)) ;
#135042=CARTESIAN_POINT('Ctrl Pts',(-26.115372034482,14.4785950091488,128.968780330961)) ;
#135043=CARTESIAN_POINT('Ctrl Pts',(-26.1991386228248,14.5108133112394,
129.246686766249)) ;
#135044=CARTESIAN_POINT('Ctrl Pts',(-26.281961118953,14.4650394200622,129.521689731091)) ;
#135045=CARTESIAN_POINT('Ctrl Pts',(-26.3576691539897,14.3446919400874,
129.775975443665)) ;
#135046=CARTESIAN_POINT('Ctrl Pts',(-26.4199450377268,14.1586507898245,
129.990981699106)) ;
#135047=CARTESIAN_POINT('Ctrl Pts',(-26.4638325348643,13.9182142591253,
130.152493567261)) ;
#135048=CARTESIAN_POINT('Ctrl Pts',(-26.4849121372087,13.6446894301756,
130.247054976681)) ;
#135049=CARTESIAN_POINT('Ctrl Pts',(-26.4814409395297,13.3538163555555,
130.270090586414)) ;
#135050=CARTESIAN_POINT('Ctrl Pts',(-26.4527946492839,13.0687529323482,
130.219476965581)) ;
#135051=CARTESIAN_POINT('Ctrl Pts',(-26.4002320096581,12.8084025711039,
130.099079794229)) ;
#135052=CARTESIAN_POINT('Ctrl Pts',(-26.3268756685072,12.5923662507696,
129.91790410308)) ;
#135053=CARTESIAN_POINT('Ctrl Pts',(-26.2371123368209,12.4355966936421,
129.688843066008)) ;
#135054=CARTESIAN_POINT('Ctrl Pts',(-26.1367181878628,12.3498834173245,
129.42872587461)) ;
#135055=CARTESIAN_POINT('Ctrl Pts',(-26.032722719753,12.3409542808635,129.157919642926)) ;
#135056=CARTESIAN_POINT('Ctrl Pts',(-25.9308084387583,12.4093757248112,
128.893357587352)) ;
#135057=CARTESIAN_POINT('Ctrl Pts',(-25.838155620905,12.5505196315372,128.655821078007)) ;
#135058=CARTESIAN_POINT('Ctrl Pts',(-25.7605740007468,12.7541803006072,
128.462316845571)) ;
#135059=CARTESIAN_POINT('Ctrl Pts',(-25.7029450253967,13.0055267425044,
128.327067990315)) ;
#135060=CARTESIAN_POINT('Ctrl Pts',(-25.6685657347824,13.2870724884799,
128.259776019344)) ;
#135061=CARTESIAN_POINT('Ctrl Pts',(-25.6592502061655,13.5781354317469,
128.265673438089)) ;
#135062=CARTESIAN_POINT('Ctrl Pts',(-25.6749179654199,13.8583662507443,
128.344586199981)) ;
#135063=CARTESIAN_POINT('Ctrl Pts',(-25.7137374162889,14.1072755060793,
128.491117013587)) ;
#135064=CARTESIAN_POINT('Ctrl Pts',(-25.7721169966564,14.3069765889331,
128.694755702354)) ;
#135065=CARTESIAN_POINT('Ctrl Pts',(-25.845207577047,14.443614067786,128.941381531894)) ;
#135066=CARTESIAN_POINT('Ctrl Pts',(-25.9273346325596,14.5071928082345,
129.214515131727)) ;
#135067=CARTESIAN_POINT('Ctrl Pts',(-26.011234962119,14.4928945220509,129.492675842775)) ;
#135068=CARTESIAN_POINT('Ctrl Pts',(-26.0906570279007,14.4021254936154,
129.757803067043)) ;
#135069=CARTESIAN_POINT('Ctrl Pts',(-26.159082383682,14.2413770477371,129.990792154917)) ;
#135070=CARTESIAN_POINT('Ctrl Pts',(-26.2110152100895,14.0210258594474,
130.175736142196)) ;
#135071=CARTESIAN_POINT('Ctrl Pts',(-26.241635177827,13.7594508415378,130.298196601018)) ;
#135072=CARTESIAN_POINT('Ctrl Pts',(-26.2483473113095,13.4716753030503,
130.351078692086)) ;
#135073=CARTESIAN_POINT('Ctrl Pts',(-26.2298541426232,13.18278007244,130.330045835803)) ;
#135074=CARTESIAN_POINT('Ctrl Pts',(-26.1867418068547,12.9097866347109,
130.237249070666)) ;
#135075=CARTESIAN_POINT('Ctrl Pts',(-26.1214552754847,12.6739761120234,
130.079613973061)) ;
#135076=CARTESIAN_POINT('Ctrl Pts',(-26.037598712626,12.4911376353209,129.867849268882)) ;
#135077=CARTESIAN_POINT('Ctrl Pts',(-25.9407649580424,12.3755758788311,
129.618129131331)) ;
#135078=CARTESIAN_POINT('Ctrl Pts',(-25.8374214950217,12.3352662329562,
129.34929906656)) ;
#135079=CARTESIAN_POINT('Ctrl Pts',(-25.7340098362028,12.3722006143293,
129.0802369826)) ;
#135080=CARTESIAN_POINT('Ctrl Pts',(-25.6361773432197,12.4858118722087,
128.827819165484)) ;
#135081=CARTESIAN_POINT('Ctrl Pts',(-25.5523274084712,12.6649628027199,
128.615825895545)) ;
#135082=CARTESIAN_POINT('Ctrl Pts',(-25.4859513870995,12.8995424291904,
128.455121245363)) ;
#135083=CARTESIAN_POINT('Ctrl Pts',(-25.4419863750333,13.1707489990253,
128.359746169264)) ;
#135084=CARTESIAN_POINT('Ctrl Pts',(-25.4224009992562,13.4602465419289,
128.335630931104)) ;
#135085=CARTESIAN_POINT('Ctrl Pts',(-25.4281061795563,13.7479094104328,
128.385491263721)) ;
#135086=CARTESIAN_POINT('Ctrl Pts',(-25.4578216450762,14.0110933638022,
128.505345635233)) ;
#135087=CARTESIAN_POINT('Ctrl Pts',(-25.5087967768197,14.2330195298938,
128.687396943834)) ;
#135088=CARTESIAN_POINT('Ctrl Pts',(-25.5768933622651,14.397056415232,128.919554215411)) ;
#135089=CARTESIAN_POINT('Ctrl Pts',(-25.6558147544988,14.4906410938832,
129.183138561615)) ;
#135090=CARTESIAN_POINT('Ctrl Pts',(-25.7399301950195,14.5080280130628,
129.462041474598)) ;
#135091=CARTESIAN_POINT('Ctrl Pts',(-25.8217364878674,14.4480725424633,
129.734011003358)) ;
#135092=CARTESIAN_POINT('Ctrl Pts',(-25.8956483813608,14.3139470607326,
129.983179734343)) ;
#135093=CARTESIAN_POINT('Ctrl Pts',(-25.9546615112484,14.1169437524237,
130.188609280051)) ;
#135094=CARTESIAN_POINT('Ctrl Pts',(-25.994519421204,13.8684682048696,130.338337741358)) ;
#135095=CARTESIAN_POINT('Ctrl Pts',(-26.0110568377318,13.5907243651,130.419594305655)) ;
#135096=CARTESIAN_POINT('Ctrl Pts',(-26.0028570943019,13.2994062522709,
130.428791647391)) ;
#135097=CARTESIAN_POINT('Ctrl Pts',(-25.9695704025357,13.0173302811176,
130.364651136717)) ;
#135098=CARTESIAN_POINT('Ctrl Pts',(-25.9127012517306,12.7634586998748,
130.23173138777)) ;
#135099=CARTESIAN_POINT('Ctrl Pts',(-25.8356694959319,12.5574053612187,
130.039883250671)) ;
#135100=CARTESIAN_POINT('Ctrl Pts',(-25.7439581375389,12.4141338116398,
129.804942699892)) ;
#135101=CARTESIAN_POINT('Ctrl Pts',(-25.6422361078924,12.342233208706,129.540970477651)) ;
#135102=CARTESIAN_POINT('Ctrl Pts',(-25.5379082160016,12.3479816385131,
129.269286803224)) ;
#135103=CARTESIAN_POINT('Ctrl Pts',(-25.4372492426153,12.4308508598937,
129.00839512309)) ;
#135104=CARTESIAN_POINT('Ctrl Pts',(-25.3472402005208,12.5841342714032,
128.778486490676)) ;
#135105=CARTESIAN_POINT('Ctrl Pts',(-25.272730898508,12.7991564308112,128.594122402279)) ;
#135106=CARTESIAN_POINT('Ctrl Pts',(-25.2194888387276,13.0569999610756,
128.471595214616)) ;
#135107=CARTESIAN_POINT('Ctrl Pts',(-25.1897401476562,13.3421921034464,
128.417860044275)) ;
#135108=CARTESIAN_POINT('Ctrl Pts',(-25.1851966857885,13.6321454574867,
128.437625751363)) ;
#135109=CARTESIAN_POINT('Ctrl Pts',(-25.2054882351433,13.9089725412032,
128.530163374861)) ;
#135110=CARTESIAN_POINT('Ctrl Pts',(-25.2484501051326,14.1498188340954,
128.688812325716)) ;
#135111=CARTESIAN_POINT('Ctrl Pts',(-25.3098239459612,14.3379335225619,
128.901090604678)) ;
#135112=CARTESIAN_POINT('Ctrl Pts',(-25.3852409841119,14.4615825769609,
129.154594863581)) ;
#135113=CARTESIAN_POINT('Ctrl Pts',(-25.4680078103566,14.5104718339952,
129.429479188798)) ;
#135114=CARTESIAN_POINT('Ctrl Pts',(-25.5519233175472,14.4813917081873,
129.707831723369)) ;
#135115=CARTESIAN_POINT('Ctrl Pts',(-25.6296594879759,14.3764101476522,
129.968016081421)) ;
#135116=CARTESIAN_POINT('Ctrl Pts',(-25.6951131634194,14.2041613001764,
130.192211432841)) ;
#135117=CARTESIAN_POINT('Ctrl Pts',(-25.7434116042681,13.9743839791119,
130.36655070585)) ;
#135118=CARTESIAN_POINT('Ctrl Pts',(-25.7697062526325,13.7063210401926,
130.476427371815)) ;
#135119=CARTESIAN_POINT('Ctrl Pts',(-25.7716643333024,13.416701167449,130.515370896243)) ;
#135120=CARTESIAN_POINT('Ctrl Pts',(-25.7484303453548,13.1291677758352,
130.480525076402)) ;
#135121=CARTESIAN_POINT('Ctrl Pts',(-25.7008468729498,12.86171027905,130.374668312212)) ;
#135122=CARTESIAN_POINT('Ctrl Pts',(-25.6318421414092,12.6350478480017,
130.206135995294)) ;
#135123=CARTESIAN_POINT('Ctrl Pts',(-25.5450073178082,12.4638699665219,
129.985698129429)) ;
#135124=CARTESIAN_POINT('Ctrl Pts',(-25.4465855133018,12.3621126869917,
129.731275230113)) ;
#135125=CARTESIAN_POINT('Ctrl Pts',(-25.3422723144961,12.336288293437,129.459748523319)) ;
#135126=CARTESIAN_POINT('Ctrl Pts',(-25.2395464146887,12.3882079133966,
129.192710014154)) ;
#135127=CARTESIAN_POINT('Ctrl Pts',(-25.1441554739243,12.5148240028862,
128.947268201873)) ;
#135128=CARTESIAN_POINT('Ctrl Pts',(-25.0632912716036,12.7050812653244,
128.743995286524)) ;
#135129=CARTESIAN_POINT('Ctrl Pts',(-25.0008040035337,12.9482677220772,
128.594669933562)) ;
#135130=CARTESIAN_POINT('Ctrl Pts',(-24.9612989083473,13.2238578222556,
128.512263188183)) ;
#135131=CARTESIAN_POINT('Ctrl Pts',(-24.9464400414306,13.5162932448957,
128.502169911524)) ;
#135132=CARTESIAN_POINT('Ctrl Pts',(-24.9567559801261,13.799165239793,128.565264390033)) ;
#135133=CARTESIAN_POINT('Ctrl Pts',(-24.9910303138475,14.0580267764743,
128.698731518742)) ;
#135134=CARTESIAN_POINT('Ctrl Pts',(-25.0453888541943,14.2686028129511,
128.890481281382)) ;
#135135=CARTESIAN_POINT('Ctrl Pts',(-25.1157749327763,14.4199618502008,
129.129219228183)) ;
#135136=CARTESIAN_POINT('Ctrl Pts',(-25.1962537469819,14.4998958219189,
129.397417258709)) ;
#135137=CARTESIAN_POINT('Ctrl Pts',(-25.2806998076144,14.5025664794371,
129.677347381576)) ;
#135138=CARTESIAN_POINT('Ctrl Pts',(-25.3614130293349,14.4280652825415,
129.946141834169)) ;
#135139=CARTESIAN_POINT('Ctrl Pts',(-25.4327613411336,14.2819177513075,
130.187667258866)) ;
#135140=CARTESIAN_POINT('Ctrl Pts',(-25.4888836010397,14.0723877227319,
130.384948804485)) ;
#135141=CARTESIAN_POINT('Ctrl Pts',(-25.524217369076,13.8191595273478,130.52109290564)) ;
#135142=CARTESIAN_POINT('Ctrl Pts',(-25.5363621720147,13.5356702848312,
130.589764696207)) ;
#135143=CARTESIAN_POINT('Ctrl Pts',(-25.5233799731752,13.2451626614465,
130.584896539849)) ;
#135144=CARTESIAN_POINT('Ctrl Pts',(-25.4853193673611,12.9658959397094,
130.506957297054)) ;
#135145=CARTESIAN_POINT('Ctrl Pts',(-25.4245567948317,12.720867949973,130.362513148524)) ;
#135146=CARTESIAN_POINT('Ctrl Pts',(-25.3444357384131,12.5256178596935,
130.161588938401)) ;
#135147=CARTESIAN_POINT('Ctrl Pts',(-25.2502354927177,12.3947249390078,
129.91946984754)) ;
#135148=CARTESIAN_POINT('Ctrl Pts',(-25.1471557384846,12.3373274128747,
129.651622343389)) ;
#135149=CARTESIAN_POINT('Ctrl Pts',(-25.04352722843,12.3577351376061,129.3818280718)) ;
#135150=CARTESIAN_POINT('Ctrl Pts',(-24.9440625937448,12.4546492514378,
129.124509048456)) ;
#135151=CARTESIAN_POINT('Ctrl Pts',(-24.8564471604785,12.6210676591383,
128.901700870073)) ;
#135152=CARTESIAN_POINT('Ctrl Pts',(-24.7859855036776,12.8446766854148,
128.728972290107)) ;
#135153=CARTESIAN_POINT('Ctrl Pts',(-24.7369148940067,13.108808163257,128.618635013836)) ;
#135154=CARTESIAN_POINT('Ctrl Pts',(-24.7117898455147,13.3979062620311,
128.578541432007)) ;
#135155=CARTESIAN_POINT('Ctrl Pts',(-24.7120774707783,13.6859097607706,
128.612344349061)) ;
#135156=CARTESIAN_POINT('Ctrl Pts',(-24.7366917620368,13.9567565280856,
128.717390290963)) ;
#135157=CARTESIAN_POINT('Ctrl Pts',(-24.7836759760245,14.1899349125241,
128.887914867791)) ;
#135158=CARTESIAN_POINT('Ctrl Pts',(-24.8478937377255,14.3662692626876,
129.10842421568)) ;
#135159=CARTESIAN_POINT('Ctrl Pts',(-24.9254379812952,14.4768289979695,
129.368240618362)) ;
#135160=CARTESIAN_POINT('Ctrl Pts',(-25.0089189154175,14.5109207090365,
129.645218161262)) ;
#135161=CARTESIAN_POINT('Ctrl Pts',(-25.0919501200887,14.4673589954117,
129.920875758852)) ;
#135162=CARTESIAN_POINT('Ctrl Pts',(-25.1679324131496,14.3490298117359,
130.175949093355)) ;
#135163=CARTESIAN_POINT('Ctrl Pts',(-25.2306776791176,14.1643442573792,
130.392364551844)) ;
#135164=CARTESIAN_POINT('Ctrl Pts',(-25.2749172208417,13.9269540764464,
130.554674425406)) ;
#135165=CARTESIAN_POINT('Ctrl Pts',(-25.296881801977,13.6529087066834,130.651991768824)) ;
#135166=CARTESIAN_POINT('Ctrl Pts',(-25.294121582554,13.3625040426011,130.677064089887)) ;
#135167=CARTESIAN_POINT('Ctrl Pts',(-25.2661584777254,13.0764917625792,
130.628507586136)) ;
#135168=CARTESIAN_POINT('Ctrl Pts',(-25.2142358128611,12.8152457852602,
130.509968872735)) ;
#135169=CARTESIAN_POINT('Ctrl Pts',(-25.1414105163864,12.5977360848388,
130.330346617025)) ;
#135170=CARTESIAN_POINT('Ctrl Pts',(-25.0521369052221,12.4392301767845,
130.102679861577)) ;
#135171=CARTESIAN_POINT('Ctrl Pts',(-24.9519825847367,12.3513755992719,
129.843259987167)) ;
#135172=CARTESIAN_POINT('Ctrl Pts',(-24.8480528333298,12.3399316332142,
129.572627714051)) ;
#135173=CARTESIAN_POINT('Ctrl Pts',(-24.7452323261505,12.4070554351268,
129.305672373312)) ;
#135174=CARTESIAN_POINT('Ctrl Pts',(-24.653114699296,12.5451369869361,129.069390792946)) ;
#135175=CARTESIAN_POINT('Ctrl Pts',(-24.574658401759,12.7477726868892,128.873467031278)) ;
#135176=CARTESIAN_POINT('Ctrl Pts',(-24.516485448288,12.9979367372735,128.736605448719)) ;
#135177=CARTESIAN_POINT('Ctrl Pts',(-24.4813744014041,13.2792370978739,
128.667217092649)) ;
#135178=CARTESIAN_POINT('Ctrl Pts',(-24.4713970354524,13.5701580555343,
128.671163049425)) ;
#135179=CARTESIAN_POINT('Ctrl Pts',(-24.4863380916386,13.8505377724051,
128.747899411962)) ;
#135180=CARTESIAN_POINT('Ctrl Pts',(-24.5245439679385,14.1007512372239,
128.892655666103)) ;
#135181=CARTESIAN_POINT('Ctrl Pts',(-24.5824402788279,14.3021715583994,
129.094893574169)) ;
#135182=CARTESIAN_POINT('Ctrl Pts',(-24.6554257346924,14.4410638226486,
129.341309329826)) ;
#135183=CARTESIAN_POINT('Ctrl Pts',(-24.7373356695316,14.506420576945,129.613776649341)) ;
#135184=CARTESIAN_POINT('Ctrl Pts',(-24.8210078848283,14.4944296739133,
129.89116801343)) ;
#135185=CARTESIAN_POINT('Ctrl Pts',(-24.9008406879447,14.4055611915821,
130.157574926146)) ;
#135186=CARTESIAN_POINT('Ctrl Pts',(-24.9694636925505,14.2469875620131,
130.391056099313)) ;
#135187=CARTESIAN_POINT('Ctrl Pts',(-25.0219599711088,14.0284942715184,
130.577615505577)) ;
#135188=CARTESIAN_POINT('Ctrl Pts',(-25.053320022464,13.7670074742828,130.70234813533)) ;
#135189=CARTESIAN_POINT('Ctrl Pts',(-25.0607089051815,13.4805781215048,
130.757097162265)) ;
#135190=CARTESIAN_POINT('Ctrl Pts',(-25.0430061476845,13.1913388058783,
130.73838961606)) ;
#135191=CARTESIAN_POINT('Ctrl Pts',(-25.0005234997867,12.9172330933754,
130.647473812606)) ;
#135192=CARTESIAN_POINT('Ctrl Pts',(-24.9358367964898,12.6799728703758,
130.491596969194)) ;
#135193=CARTESIAN_POINT('Ctrl Pts',(-24.8520526958292,12.4949910418975,
130.280173035867)) ;
#135194=CARTESIAN_POINT('Ctrl Pts',(-24.756283433586,12.3781840447206,130.033296564361)) ;
#135195=CARTESIAN_POINT('Ctrl Pts',(-24.6522083130104,12.3352411023339,
129.762603753164)) ;
#135196=CARTESIAN_POINT('Ctrl Pts',(-24.5492013359519,12.3701183957634,
129.494563600041)) ;
#135197=CARTESIAN_POINT('Ctrl Pts',(-24.4510228781676,12.4815908370187,
129.241159666924)) ;
#135198=CARTESIAN_POINT('Ctrl Pts',(-24.3668186999168,12.6586744463426,
129.02808228214)) ;
#135199=CARTESIAN_POINT('Ctrl Pts',(-24.2996856218142,12.8927064505131,
128.86527445598)) ;
#135200=CARTESIAN_POINT('Ctrl Pts',(-24.2552426505653,13.1615895986342,
128.768318934161)) ;
#135201=CARTESIAN_POINT('Ctrl Pts',(-24.2347791741716,13.4527337961883,
128.741859841865)) ;
#135202=CARTESIAN_POINT('Ctrl Pts',(-24.2398184692911,13.7397606263225,
128.789657130047)) ;
#135203=CARTESIAN_POINT('Ctrl Pts',(-24.2689320023009,14.0044956878458,
128.907831044878)) ;
#135204=CARTESIAN_POINT('Ctrl Pts',(-24.3192589693072,14.2270717047825,
129.087893938316)) ;
#135205=CARTESIAN_POINT('Ctrl Pts',(-24.386637598686,14.3928428531141,129.31784383242)) ;
#135206=CARTESIAN_POINT('Ctrl Pts',(-24.4659391407555,14.4891679896536,
129.582798342604)) ;
#135207=CARTESIAN_POINT('Ctrl Pts',(-24.5493645856168,14.5086708936273,
129.859423076708)) ;
#135208=CARTESIAN_POINT('Ctrl Pts',(-24.6318807172738,14.4507091204102,
130.133696348165)) ;
#135209=CARTESIAN_POINT('Ctrl Pts',(-24.7058567597393,14.318823465338,130.382937634357)) ;
#135210=CARTESIAN_POINT('Ctrl Pts',(-24.7654056750014,14.1234067424229,
130.589957999186)) ;
#135211=CARTESIAN_POINT('Ctrl Pts',(-24.8057595992627,13.8772496577341,
130.740994985991)) ;
#135212=CARTESIAN_POINT('Ctrl Pts',(-24.8231799857801,13.5994498547175,
130.82492878504)) ;
#135213=CARTESIAN_POINT('Ctrl Pts',(-24.8155893045152,13.3067289539218,
130.836068714423)) ;
#135214=CARTESIAN_POINT('Ctrl Pts',(-24.7830973206933,13.025513208076,130.774091996489)) ;
#135215=CARTESIAN_POINT('Ctrl Pts',(-24.7270577046474,12.7708776887036,
130.643534343482)) ;
#135216=CARTESIAN_POINT('Ctrl Pts',(-24.6505077984341,12.5628412979246,
130.453131427416)) ;
#135217=CARTESIAN_POINT('Ctrl Pts',(-24.5589760348122,12.4171764122364,
130.218786009453)) ;
#135218=CARTESIAN_POINT('Ctrl Pts',(-24.4570551071365,12.3431378359771,
129.954350410602)) ;
#135219=CARTESIAN_POINT('Ctrl Pts',(-24.3533214115063,12.3467434972734,
129.684210676246)) ;
#135220=CARTESIAN_POINT('Ctrl Pts',(-24.2523283182393,12.4272274658185,
129.422376802438)) ;
#135221=CARTESIAN_POINT('Ctrl Pts',(-24.1617932807192,12.5790158149027,
129.190994958755)) ;
#135222=CARTESIAN_POINT('Ctrl Pts',(-24.0869579392724,12.7916687829571,
129.005564094205)) ;
#135223=CARTESIAN_POINT('Ctrl Pts',(-24.0328055760906,13.0498138992039,
128.8805514449)) ;
#135224=CARTESIAN_POINT('Ctrl Pts',(-24.002521804032,13.3331756720239,128.825089124936)) ;
#135225=CARTESIAN_POINT('Ctrl Pts',(-23.9971725769105,13.6238935345468,
128.842575947387)) ;
#135226=CARTESIAN_POINT('Ctrl Pts',(-24.0167753636582,13.9010885274901,
128.933062863381)) ;
#135227=CARTESIAN_POINT('Ctrl Pts',(-24.0590128945408,14.1432054793993,
129.089568959686)) ;
#135228=CARTESIAN_POINT('Ctrl Pts',(-24.1203695555296,14.3341070280144,
129.302019247719)) ;
#135229=CARTESIAN_POINT('Ctrl Pts',(-24.1950418049019,14.4587991787124,
129.553138711427)) ;
#135230=CARTESIAN_POINT('Ctrl Pts',(-24.2777268658875,14.5101605081857,
129.827811432152)) ;
#135231=CARTESIAN_POINT('Ctrl Pts',(-24.3615395865942,14.4834097576633,
130.105796352381)) ;
#135232=CARTESIAN_POINT('Ctrl Pts',(-24.4396001237497,14.380986704451,130.366925214371)) ;
#135233=CARTESIAN_POINT('Ctrl Pts',(-24.5059188478657,14.2089571607828,
130.593906733665)) ;
#135234=CARTESIAN_POINT('Ctrl Pts',(-24.5543423873352,13.9828180453883,
130.768283768123)) ;
#135235=CARTESIAN_POINT('Ctrl Pts',(-24.5815804292821,13.7132629209954,
130.881224790375)) ;
#135236=CARTESIAN_POINT('Ctrl Pts',(-24.5841620980753,13.42583764063,130.921759059005)) ;
#135237=CARTESIAN_POINT('Ctrl Pts',(-24.5616991302751,13.1374631065902,
130.889232264708)) ;
#135238=CARTESIAN_POINT('Ctrl Pts',(-24.5148271925072,12.8691197006536,
130.785439835784)) ;
#135239=CARTESIAN_POINT('Ctrl Pts',(-24.4460595852779,12.6403113443668,
130.617737495797)) ;
#135240=CARTESIAN_POINT('Ctrl Pts',(-24.3602783070861,12.468420702256,130.400139902644)) ;
#135241=CARTESIAN_POINT('Ctrl Pts',(-24.2614984282295,12.3638000217504,
130.144889114756)) ;
#135242=CARTESIAN_POINT('Ctrl Pts',(-24.1577920148866,12.3359859144704,
129.874955907544)) ;
#135243=CARTESIAN_POINT('Ctrl Pts',(-24.054756872384,12.3855342690204,129.607074345636)) ;
#135244=CARTESIAN_POINT('Ctrl Pts',(-23.9592387590454,12.5097023136888,
129.361184743235)) ;
#135245=CARTESIAN_POINT('Ctrl Pts',(-23.8775758716564,12.6987169895182,
129.155691106511)) ;
#135246=CARTESIAN_POINT('Ctrl Pts',(-23.8143557456443,12.9413958856346,
129.004310292951)) ;
#135247=CARTESIAN_POINT('Ctrl Pts',(-23.7742609530853,13.2164083911014,
128.920187229679)) ;
#135248=CARTESIAN_POINT('Ctrl Pts',(-23.7587189631835,13.5077476116907,
128.907983756604)) ;
#135249=CARTESIAN_POINT('Ctrl Pts',(-23.7683966260473,13.7917084995172,
128.969294505237)) ;
#135250=CARTESIAN_POINT('Ctrl Pts',(-23.8017090745378,14.0497089633418,
129.099691778832)) ;
#135251=CARTESIAN_POINT('Ctrl Pts',(-23.855687851068,14.2632250030891,129.290500820459)) ;
#135252=CARTESIAN_POINT('Ctrl Pts',(-23.9259445764529,14.4168537708596,
129.528960264585)) ;
#135253=CARTESIAN_POINT('Ctrl Pts',(-24.0063154571533,14.4987598986465,
129.796873298139)) ;
#135254=CARTESIAN_POINT('Ctrl Pts',(-24.0905209887515,14.5035045718472,
130.07601230486)) ;
#135255=CARTESIAN_POINT('Ctrl Pts',(-24.1714640122117,14.4313229997249,
130.345485263966)) ;
#135256=CARTESIAN_POINT('Ctrl Pts',(-24.243380136318,14.286096674379,130.588809864043)) ;
#135257=CARTESIAN_POINT('Ctrl Pts',(-24.2994203289572,14.0806888556304,
130.785462444038)) ;
#135258=CARTESIAN_POINT('Ctrl Pts',(-24.3358061636431,13.8265805447723,
130.924971011733)) ;
#135259=CARTESIAN_POINT('Ctrl Pts',(-24.3485662665821,13.5441879409374,
130.995358908411)) ;
#135260=CARTESIAN_POINT('Ctrl Pts',(-24.3362787692544,13.2530370689606,
130.992594119063)) ;
#135261=CARTESIAN_POINT('Ctrl Pts',(-24.2990565233592,12.9741114175935,
130.916980614884)) ;
#135262=CARTESIAN_POINT('Ctrl Pts',(-24.2387980421576,12.7272119216586,
130.774093243821)) ;
#135263=CARTESIAN_POINT('Ctrl Pts',(-24.1592542721153,12.5305677659782,
130.57481255156)) ;
#135264=CARTESIAN_POINT('Ctrl Pts',(-24.0653992661587,12.3976028767503,
130.333704016612)) ;
#135265=CARTESIAN_POINT('Ctrl Pts',(-23.9625403093089,12.3378877564715,
130.06647786499)) ;
#135266=CARTESIAN_POINT('Ctrl Pts',(-23.8586656317476,12.3561146457162,
129.796030313594)) ;
#135267=CARTESIAN_POINT('Ctrl Pts',(-23.7592617382335,12.4504996091204,
129.538781451731)) ;
#135268=CARTESIAN_POINT('Ctrl Pts',(-23.6710781493093,12.6151918179393,
129.314368558311)) ;
#135269=CARTESIAN_POINT('Ctrl Pts',(-23.6000847768971,12.8367627956422,
129.140023816127)) ;
#135270=CARTESIAN_POINT('Ctrl Pts',(-23.5500037307086,13.102471284239,129.027040548326)) ;
#135271=CARTESIAN_POINT('Ctrl Pts',(-23.5244629176484,13.388098474674,128.985365037134)) ;
#135272=CARTESIAN_POINT('Ctrl Pts',(-23.5239179211507,13.6786302634614,
129.017000214703)) ;
#135273=CARTESIAN_POINT('Ctrl Pts',(-23.5479482075075,13.9495118019851,
129.120261172471)) ;
#135274=CARTESIAN_POINT('Ctrl Pts',(-23.5940539896427,14.1831630717315,
129.28807205042)) ;
#135275=CARTESIAN_POINT('Ctrl Pts',(-23.658087369295,14.3622887251467,129.508197418047)) ;
#135276=CARTESIAN_POINT('Ctrl Pts',(-23.7354964858561,14.4748192529362,
129.767663246934)) ;
#135277=CARTESIAN_POINT('Ctrl Pts',(-23.8186008712506,14.5109473630978,
130.043427649505)) ;
#135278=CARTESIAN_POINT('Ctrl Pts',(-23.9016485189198,14.46989386631,130.319093678178)) ;
#135279=CARTESIAN_POINT('Ctrl Pts',(-23.9780326629865,14.3536144736526,
130.57538079303)) ;
#135280=CARTESIAN_POINT('Ctrl Pts',(-24.041317392537,14.17062113719,130.793395793898)) ;
#135281=CARTESIAN_POINT('Ctrl Pts',(-24.0862233608817,13.933736573907,130.957750623604)) ;
#135282=CARTESIAN_POINT('Ctrl Pts',(-24.1087782693582,13.6617104442443,
131.056639640472)) ;
#135283=CARTESIAN_POINT('Ctrl Pts',(-24.1067652069901,13.3701432171844,
131.084050982405)) ;
#135284=CARTESIAN_POINT('Ctrl Pts',(-24.0794150200347,13.0839501475181,
131.037263800254)) ;
#135285=CARTESIAN_POINT('Ctrl Pts',(-24.0283415442683,12.8226369063403,
130.921088721576)) ;
#135286=CARTESIAN_POINT('Ctrl Pts',(-23.9561135287856,12.6036153158418,
130.74320474868)) ;
#135287=CARTESIAN_POINT('Ctrl Pts',(-23.8674374985634,12.4432239429731,
130.517228131168)) ;
#135288=CARTESIAN_POINT('Ctrl Pts',(-23.7669177824065,12.3525997513282,
130.256937329486)) ;
#135289=CARTESIAN_POINT('Ctrl Pts',(-23.6631589097691,12.3393903655815,
129.986759745082)) ;
#135290=CARTESIAN_POINT('Ctrl Pts',(-23.5608451726887,12.403468098602,129.721057322036)) ;
#135291=CARTESIAN_POINT('Ctrl Pts',(-23.4675538333872,12.5405072085783,
129.481626938511)) ;
#135292=CARTESIAN_POINT('Ctrl Pts',(-23.388662980097,12.7420005519616,129.284449551793)) ;
#135293=CARTESIAN_POINT('Ctrl Pts',(-23.3301053404809,12.9900801149227,
129.146339662681)) ;
#135294=CARTESIAN_POINT('Ctrl Pts',(-23.2942598700259,13.2708158721555,
129.07481369419)) ;
#135295=CARTESIAN_POINT('Ctrl Pts',(-23.2835507653219,13.5613604134334,
129.07658052044)) ;
#135296=CARTESIAN_POINT('Ctrl Pts',(-23.2977457009926,13.8428560081929,
129.151189048699)) ;
#135297=CARTESIAN_POINT('Ctrl Pts',(-23.3355877732922,14.0951246502648,
129.295029201952)) ;
#135298=CARTESIAN_POINT('Ctrl Pts',(-23.392640021767,14.2968154125605,129.494589775277)) ;
#135299=CARTESIAN_POINT('Ctrl Pts',(-23.4654695271126,14.4382062812648,
129.740653917803)) ;
#135300=CARTESIAN_POINT('Ctrl Pts',(-23.5470349400498,14.5055713938207,
130.012034404642)) ;
#135301=CARTESIAN_POINT('Ctrl Pts',(-23.6308595315768,14.4957941932041,
130.289927886282)) ;
#135302=CARTESIAN_POINT('Ctrl Pts',(-23.7106798599952,14.4095662340998,
130.556186374908)) ;
#135303=CARTESIAN_POINT('Ctrl Pts',(-23.7802571461447,14.2515335127425,
130.792730605287)) ;
#135304=CARTESIAN_POINT('Ctrl Pts',(-23.8330271584667,14.0347236874785,
130.979999898394)) ;
#135305=CARTESIAN_POINT('Ctrl Pts',(-23.8649144470802,13.7751700114088,
131.106159195577)) ;
#135306=CARTESIAN_POINT('Ctrl Pts',(-23.8730939748177,13.489555102194,131.163174955555)) ;
#135307=CARTESIAN_POINT('Ctrl Pts',(-23.8560200827014,13.1989624545804,
131.146444379055)) ;
#135308=CARTESIAN_POINT('Ctrl Pts',(-23.8142948031392,12.9245155762064,
131.057679563774)) ;
#135309=CARTESIAN_POINT('Ctrl Pts',(-23.7497390288408,12.6850932088169,
130.90236186876)) ;
#135310=CARTESIAN_POINT('Ctrl Pts',(-23.6676401734867,12.5007200500438,
130.695387264516)) ;
#135311=CARTESIAN_POINT('Ctrl Pts',(-23.5710799792398,12.3802348015134,
130.446601105623)) ;
#135312=CARTESIAN_POINT('Ctrl Pts',(-23.4680387193144,12.3354177830535,
130.178616720221)) ;
#135313=CARTESIAN_POINT('Ctrl Pts',(-23.3639870057212,12.3682931650198,
129.907845197495)) ;
#135314=CARTESIAN_POINT('Ctrl Pts',(-23.2665557781875,12.4764500222757,
129.656260795804)) ;
#135315=CARTESIAN_POINT('Ctrl Pts',(-23.1812074615382,12.6527561756398,
129.440099421206)) ;
#135316=CARTESIAN_POINT('Ctrl Pts',(-23.1137789148354,12.8841372675975,
129.276247072773)) ;
#135317=CARTESIAN_POINT('Ctrl Pts',(-23.0682028417558,13.1550291136418,
129.176337392218)) ;
#135318=CARTESIAN_POINT('Ctrl Pts',(-23.0472767378411,13.4437302360126,
129.148261982065)) ;
#135319=CARTESIAN_POINT('Ctrl Pts',(-23.0515496084932,13.7319393007276,
129.193922359653)) ;
#135320=CARTESIAN_POINT('Ctrl Pts',(-23.079878251099,13.9965481623833,129.309665379139)) ;
#135321=CARTESIAN_POINT('Ctrl Pts',(-23.129741526764,14.2215298170475,129.488488454029)) ;
#135322=CARTESIAN_POINT('Ctrl Pts',(-23.1968818888558,14.3891483272759,
129.717799600751)) ;
#135323=CARTESIAN_POINT('Ctrl Pts',(-23.2754021964238,14.4871687024338,
129.980255089599)) ;
#135324=CARTESIAN_POINT('Ctrl Pts',(-23.3593328759968,14.5093408079897,
130.258577404978)) ;
#135325=CARTESIAN_POINT('Ctrl Pts',(-23.4420335332337,14.4530254583256,
130.533420307647)) ;
#135326=CARTESIAN_POINT('Ctrl Pts',(-23.5159486858221,14.3240305585518,
130.782295669503)) ;
#135327=CARTESIAN_POINT('Ctrl Pts',(-23.5763068870408,14.1290979717854,
130.991878121919)) ;
#135328=CARTESIAN_POINT('Ctrl Pts',(-23.617068843589,13.8855604155571,131.143910620301)) ;
#135329=CARTESIAN_POINT('Ctrl Pts',(-23.6352727286933,13.6058416707122,
131.230442968303)) ;
#135330=CARTESIAN_POINT('Ctrl Pts',(-23.6283964341607,13.3160021377259,
131.243341112372)) ;
#135331=CARTESIAN_POINT('Ctrl Pts',(-23.5965464340223,13.0326886676077,
131.183420690455)) ;
#135332=CARTESIAN_POINT('Ctrl Pts',(-23.5408985622457,12.7766372190837,
131.054072194123)) ;
#135333=CARTESIAN_POINT('Ctrl Pts',(-23.4649595861684,12.5676698161814,
130.865387166735)) ;
#135334=CARTESIAN_POINT('Ctrl Pts',(-23.3740967453034,12.4206517790888,
130.632884178497)) ;
#135335=CARTESIAN_POINT('Ctrl Pts',(-23.2727082372118,12.3443150505119,
130.369901024895)) ;
#135336=CARTESIAN_POINT('Ctrl Pts',(-23.1684546893583,12.3454567433165,
130.098404386445)) ;
#135337=CARTESIAN_POINT('Ctrl Pts',(-23.0671327036379,12.4241540146565,
129.835658717647)) ;
#135338=CARTESIAN_POINT('Ctrl Pts',(-22.9764947583752,12.5736454649868,
129.60388157098)) ;
#135339=CARTESIAN_POINT('Ctrl Pts',(-22.9011806814661,12.7844244258342,
129.417017819213)) ;
#135340=CARTESIAN_POINT('Ctrl Pts',(-22.8463459628872,13.041264478038,129.289992771218)) ;
#135341=CARTESIAN_POINT('Ctrl Pts',(-22.815230919969,13.3250313838274,129.232207692813)) ;
#135342=CARTESIAN_POINT('Ctrl Pts',(-22.8092125202162,13.6156492492809,
129.247717690027)) ;
#135343=CARTESIAN_POINT('Ctrl Pts',(-22.8280212526032,13.8929002803611,
129.335801002832)) ;
#135344=CARTESIAN_POINT('Ctrl Pts',(-22.8696833153775,14.1366366428793,
129.490673844657)) ;
#135345=CARTESIAN_POINT('Ctrl Pts',(-22.9303059421642,14.3287833833703,
129.70086742119)) ;
#135346=CARTESIAN_POINT('Ctrl Pts',(-23.0049559964505,14.4563288342089,
129.952070625789)) ;
#135347=CARTESIAN_POINT('Ctrl Pts',(-23.0876811988293,14.5097636463918,
130.226920951019)) ;
#135348=CARTESIAN_POINT('Ctrl Pts',(-23.171313625943,14.4852491819093,130.504285160366)) ;
#135349=CARTESIAN_POINT('Ctrl Pts',(-23.2495616828516,14.385213180382,130.765927789329)) ;
#135350=CARTESIAN_POINT('Ctrl Pts',(-23.3164467304666,14.2148994362801,
130.994611083723)) ;
#135351=CARTESIAN_POINT('Ctrl Pts',(-23.3654737459425,13.9895605141043,
131.170821580244)) ;
#135352=CARTESIAN_POINT('Ctrl Pts',(-23.3932709418014,13.7226496289756,
131.285186238845)) ;
#135353=CARTESIAN_POINT('Ctrl Pts',(-23.3966715321499,13.4342098859693,
131.328274909581)) ;
#135354=CARTESIAN_POINT('Ctrl Pts',(-23.3749521692447,13.1458182759752,
131.297881508113)) ;
#135355=CARTESIAN_POINT('Ctrl Pts',(-23.3285769346008,12.8759127132536,
131.195640591877)) ;
#135356=CARTESIAN_POINT('Ctrl Pts',(-23.2608087751802,12.6468868556867,
131.030665242811)) ;
#135357=CARTESIAN_POINT('Ctrl Pts',(-23.1749384545703,12.4721832296684,
130.81301511834)) ;
#135358=CARTESIAN_POINT('Ctrl Pts',(-23.0772501521557,12.3661739274481,
130.560671910315)) ;
#135359=CARTESIAN_POINT('Ctrl Pts',(-22.972758046801,12.3355863385396,130.288726503058)) ;
#135360=CARTESIAN_POINT('Ctrl Pts',(-22.8698300820149,12.3831198658751,
130.021082533712)) ;
#135361=CARTESIAN_POINT('Ctrl Pts',(-22.7739061268904,12.5053833023315,
129.774046335208)) ;
#135362=CARTESIAN_POINT('Ctrl Pts',(-22.6919791045737,12.6923270702948,
129.567704270438)) ;
#135363=CARTESIAN_POINT('Ctrl Pts',(-22.6281112723494,12.9335865705139,
129.414426275698)) ;
#135364=CARTESIAN_POINT('Ctrl Pts',(-22.5872544610613,13.2085814539572,
129.328158922446)) ;
#135365=CARTESIAN_POINT('Ctrl Pts',(-22.5710404902249,13.4990557588074,
129.313907984072)) ;
#135366=CARTESIAN_POINT('Ctrl Pts',(-22.5799753665134,13.7836907462661,
129.373072556554)) ;
#135367=CARTESIAN_POINT('Ctrl Pts',(-22.612638583778,14.0427281414566,129.501571243045)) ;
#135368=CARTESIAN_POINT('Ctrl Pts',(-22.6660762367978,14.2577309750281,
129.69079806233)) ;
#135369=CARTESIAN_POINT('Ctrl Pts',(-22.7357975374954,14.4131664617501,
129.927633756715)) ;
#135370=CARTESIAN_POINT('Ctrl Pts',(-22.8161137666784,14.4973755702956,
130.195456113862)) ;
#135371=CARTESIAN_POINT('Ctrl Pts',(-22.8998820017925,14.5046724130054,
130.47314586159)) ;
#135372=CARTESIAN_POINT('Ctrl Pts',(-22.9816064513032,14.4343111747756,
130.745147804022)) ;
#135373=CARTESIAN_POINT('Ctrl Pts',(-23.0536227051492,14.2913904033354,
130.98864811284)) ;
#135374=CARTESIAN_POINT('Ctrl Pts',(-23.1102843211941,14.0872940403586,
131.187176359758)) ;
#135375=CARTESIAN_POINT('Ctrl Pts',(-23.1472375329922,13.8349907742835,
131.328253449348)) ;
#135376=CARTESIAN_POINT('Ctrl Pts',(-23.1607772342592,13.5522018199285,
131.401036362566)) ;
#135377=CARTESIAN_POINT('Ctrl Pts',(-23.1491871925298,13.2611771320633,
131.400285897439)) ;
#135378=CARTESIAN_POINT('Ctrl Pts',(-23.1125952006362,12.9814107201437,
131.326544774095)) ;
#135379=CARTESIAN_POINT('Ctrl Pts',(-23.0531566614903,12.7341369610279,
131.185942865115)) ;
#135380=CARTESIAN_POINT('Ctrl Pts',(-22.9739547949964,12.535166216503,130.98774443351)) ;
#135381=CARTESIAN_POINT('Ctrl Pts',(-22.8800044204222,12.4000170891871,
130.746489022896)) ;
#135382=CARTESIAN_POINT('Ctrl Pts',(-22.7777942394703,12.3385941106561,
130.480992016477)) ;
#135383=CARTESIAN_POINT('Ctrl Pts',(-22.6737045237347,12.3545286685026,
130.209973410253)) ;
#135384=CARTESIAN_POINT('Ctrl Pts',(-22.574018025731,12.4469846430608,129.951917332464)) ;
#135385=CARTESIAN_POINT('Ctrl Pts',(-22.4853397321754,12.6102579412087,
129.726108518223)) ;
#135386=CARTESIAN_POINT('Ctrl Pts',(-22.4141387274598,12.8296977311719,
129.551032278381)) ;
#135387=CARTESIAN_POINT('Ctrl Pts',(-22.3635165048781,13.0929763552362,
129.436306120848)) ;
#135388=CARTESIAN_POINT('Ctrl Pts',(-22.3370222640428,13.3798715107165,
129.392040554444)) ;
#135389=CARTESIAN_POINT('Ctrl Pts',(-22.3358180956749,13.6705227535771,
129.421738962196)) ;
#135390=CARTESIAN_POINT('Ctrl Pts',(-22.359121262081,13.9421700423004,129.522864634634)) ;
#135391=CARTESIAN_POINT('Ctrl Pts',(-22.4048936915904,14.1780191011813,
129.689842088352)) ;
#135392=CARTESIAN_POINT('Ctrl Pts',(-22.4683015911897,14.3579768124892,
129.908015928199)) ;
#135393=CARTESIAN_POINT('Ctrl Pts',(-22.5452274463354,14.4725057553617,
130.165996866725)) ;
#135394=CARTESIAN_POINT('Ctrl Pts',(-22.6283868280108,14.5110248787396,
130.441981808158)) ;
#135395=CARTESIAN_POINT('Ctrl Pts',(-22.7115926468901,14.4721191969269,
130.718131866034)) ;
#135396=CARTESIAN_POINT('Ctrl Pts',(-22.7882774144574,14.3577454336847,
130.975310558445)) ;
#135397=CARTESIAN_POINT('Ctrl Pts',(-22.8518198048839,14.1770688666527,
131.193977525084)) ;
#135398=CARTESIAN_POINT('Ctrl Pts',(-22.8974027115045,13.9416997327419,
131.360307596844)) ;
#135399=CARTESIAN_POINT('Ctrl Pts',(-22.9206820190988,13.6694104353782,
131.461436266431)) ;
#135400=CARTESIAN_POINT('Ctrl Pts',(-22.9194213574652,13.3798585935035,
131.490838835533)) ;
#135401=CARTESIAN_POINT('Ctrl Pts',(-22.8929170330155,13.0927640382574,
131.446571141722)) ;
#135402=CARTESIAN_POINT('Ctrl Pts',(-22.8423030043868,12.8294542733058,
131.331865445954)) ;
#135403=CARTESIAN_POINT('Ctrl Pts',(-22.7706185679307,12.6090080043084,
131.155563913664)) ;
#135404=CARTESIAN_POINT('Ctrl Pts',(-22.6821571255679,12.4466659582347,
130.930272433196)) ;
#135405=CARTESIAN_POINT('Ctrl Pts',(-22.5824728331909,12.3544265354386,
130.672221564255)) ;
#135406=CARTESIAN_POINT('Ctrl Pts',(-22.478522759517,12.338485550426,130.401560070963)) ;
#135407=CARTESIAN_POINT('Ctrl Pts',(-22.3754966015088,12.4009576070215,
130.133958949611)) ;
#135408=CARTESIAN_POINT('Ctrl Pts',(-22.2823680889779,12.5356622675021,
129.894847033385)) ;
#135409=CARTESIAN_POINT('Ctrl Pts',(-22.2032360996956,12.7342792931547,
129.696815676907)) ;
#135410=CARTESIAN_POINT('Ctrl Pts',(-22.1436939987442,12.9822470405306,
129.555989965758)) ;
#135411=CARTESIAN_POINT('Ctrl Pts',(-22.1071406671597,13.2626104241267,
129.482419788097)) ;
#135412=CARTESIAN_POINT('Ctrl Pts',(-22.0957144593787,13.5537330357078,
129.482159506806)) ;
#135413=CARTESIAN_POINT('Ctrl Pts',(-22.1092685563454,13.8350780443648,
129.554823798795)) ;
#135414=CARTESIAN_POINT('Ctrl Pts',(-22.1461475103679,14.0872562376869,
129.695659561939)) ;
#135415=CARTESIAN_POINT('Ctrl Pts',(-22.2030821358645,14.2922552735091,
129.895131181954)) ;
#135416=CARTESIAN_POINT('Ctrl Pts',(-22.2754289643042,14.4349645919609,
130.139699349458)) ;
#135417=CARTESIAN_POINT('Ctrl Pts',(-22.3564708008619,14.5045540577175,
130.40942261917)) ;
#135418=CARTESIAN_POINT('Ctrl Pts',(-22.4406441329642,14.4973581396257,
130.688457173911)) ;
#135419=CARTESIAN_POINT('Ctrl Pts',(-22.5209414268602,14.4126016842873,
130.956235143864)) ;
#135420=CARTESIAN_POINT('Ctrl Pts',(-22.5903401138937,14.2578370889756,
131.191978979017)) ;
#135421=CARTESIAN_POINT('Ctrl Pts',(-22.643899231601,14.0423606370671,131.381638018117)) ;
#135422=CARTESIAN_POINT('Ctrl Pts',(-22.676541227732,13.7833430848993,131.510062783894)) ;
#135423=CARTESIAN_POINT('Ctrl Pts',(-22.6854014712124,13.4972454461382,
131.569174829683)) ;
#135424=CARTESIAN_POINT('Ctrl Pts',(-22.6691263169549,13.2077137971034,
131.554634071507)) ;
#135425=CARTESIAN_POINT('Ctrl Pts',(-22.6279874269016,12.9318531124,131.467669892297)) ;
#135426=CARTESIAN_POINT('Ctrl Pts',(-22.5644211603477,12.6922552108513,
131.31506619976)) ;
#135427=CARTESIAN_POINT('Ctrl Pts',(-22.4822337913331,12.504666487009,131.108074794862)) ;
#135428=CARTESIAN_POINT('Ctrl Pts',(-22.3859455591042,12.3825157199122,
130.860070359518)) ;
#135429=CARTESIAN_POINT('Ctrl Pts',(-22.283236535859,12.3357140444497,130.592990061673)) ;
#135430=CARTESIAN_POINT('Ctrl Pts',(-22.1793293005588,12.3660679541908,
130.322564167356)) ;
#135431=CARTESIAN_POINT('Ctrl Pts',(-22.0811143599576,12.4727573812884,
130.068868334442)) ;
#135432=CARTESIAN_POINT('Ctrl Pts',(-21.995572717209,12.6471452986828,129.852067795218)) ;
#135433=CARTESIAN_POINT('Ctrl Pts',(-21.9277324469771,12.8766362181276,
129.686942307119)) ;
#135434=CARTESIAN_POINT('Ctrl Pts',(-21.88149427899,13.1457609561308,129.584999326918)) ;
#135435=CARTESIAN_POINT('Ctrl Pts',(-21.8597035864534,13.436208516762,129.554631981768)) ;
#135436=CARTESIAN_POINT('Ctrl Pts',(-21.8632848179525,13.7232902020091,
129.598101610311)) ;
#135437=CARTESIAN_POINT('Ctrl Pts',(-21.8909607988816,13.9896012284326,
129.712029646671)) ;
#135438=CARTESIAN_POINT('Ctrl Pts',(-21.9403194385609,14.2159296230216,
129.889382772798)) ;
#135439=CARTESIAN_POINT('Ctrl Pts',(-22.0069084874016,14.3851342144556,
130.117025681466)) ;
#135440=CARTESIAN_POINT('Ctrl Pts',(-22.0853055168022,14.4854516976048,
130.379173666988)) ;
#135441=CARTESIAN_POINT('Ctrl Pts',(-22.1690106808166,14.5096986607512,
130.656773596937)) ;
#135442=CARTESIAN_POINT('Ctrl Pts',(-22.2516547688815,14.4561737731647,
130.931357792915)) ;
#135443=CARTESIAN_POINT('Ctrl Pts',(-22.3263675110369,14.3282785458503,
131.182786371531)) ;
#135444=CARTESIAN_POINT('Ctrl Pts',(-22.3868479785871,14.1363003864466,
131.392508931439)) ;
#135445=CARTESIAN_POINT('Ctrl Pts',(-22.4284860760948,13.8924839857025,
131.547317007501)) ;
#135446=CARTESIAN_POINT('Ctrl Pts',(-22.44725520974,13.6154602436594,131.6352536123)) ;
#135447=CARTESIAN_POINT('Ctrl Pts',(-22.4412045671012,13.3244466531158,
131.650714430567)) ;
#135448=CARTESIAN_POINT('Ctrl Pts',(-22.4100202102661,13.0407282159145,
131.592726094803)) ;
#135449=CARTESIAN_POINT('Ctrl Pts',(-22.3552546417009,12.7843965627726,
131.465846020052)) ;
#135450=CARTESIAN_POINT('Ctrl Pts',(-22.2799328403175,12.5734338880589,
131.27897230653)) ;
#135451=CARTESIAN_POINT('Ctrl Pts',(-22.1888584470267,12.4236459559127,
131.046058924602)) ;
#135452=CARTESIAN_POINT('Ctrl Pts',(-22.0881362776665,12.3455712635568,
130.784862015627)) ;
#135453=CARTESIAN_POINT('Ctrl Pts',(-21.9835492566618,12.3443023671055,
130.512500328341)) ;
#135454=CARTESIAN_POINT('Ctrl Pts',(-21.8821100407858,12.420933178294,130.249388866071)) ;
#135455=CARTESIAN_POINT('Ctrl Pts',(-21.7910702729597,12.5684896870098,
130.016446821888)) ;
#135456=CARTESIAN_POINT('Ctrl Pts',(-21.7150620477299,12.7783872300958,
129.827643163685)) ;
#135457=CARTESIAN_POINT('Ctrl Pts',(-21.6597355302853,13.0341435528073,
129.699158062916)) ;
#135458=CARTESIAN_POINT('Ctrl Pts',(-21.6280379920894,13.3161552682329,
129.639527649233)) ;
#135459=CARTESIAN_POINT('Ctrl Pts',(-21.6212166338096,13.6077102167408,
129.65278753406)) ;
#135460=CARTESIAN_POINT('Ctrl Pts',(-21.6394813968357,13.8863966863271,
129.739379830896)) ;
#135461=CARTESIAN_POINT('Ctrl Pts',(-21.6805482499846,14.1306963082603,
129.892451481926)) ;
#135462=CARTESIAN_POINT('Ctrl Pts',(-21.7404897132441,14.3238933046915,
130.100547666824)) ;
#135463=CARTESIAN_POINT('Ctrl Pts',(-21.8147710462659,14.4535137780173,
130.350663609957)) ;
#135464=CARTESIAN_POINT('Ctrl Pts',(-21.8973774190617,14.5094099168095,
130.625175022534)) ;
#135465=CARTESIAN_POINT('Ctrl Pts',(-21.9815416990517,14.4867701673882,
130.904282937535)) ;
#135466=CARTESIAN_POINT('Ctrl Pts',(-22.0595736035611,14.3890643828725,
131.165115307558)) ;
#135467=CARTESIAN_POINT('Ctrl Pts',(-22.1268562117523,14.2211869107964,
131.394908944864)) ;
#135468=CARTESIAN_POINT('Ctrl Pts',(-22.1766796342833,13.9958858020985,
131.573633433779)) ;
#135469=CARTESIAN_POINT('Ctrl Pts',(-22.2049451389284,13.7314793548645,
131.689162299244)) ;
#135470=CARTESIAN_POINT('Ctrl Pts',(-22.2091882562906,13.4423639400344,
131.734833540967)) ;
#135471=CARTESIAN_POINT('Ctrl Pts',(-22.187986226038,13.1530743203904,131.706032228928)) ;
#135472=CARTESIAN_POINT('Ctrl Pts',(-22.1426951060036,12.8842566111771,
131.60670589681)) ;
#135473=CARTESIAN_POINT('Ctrl Pts',(-22.0749780240027,12.6519995362001,
131.442148263088)) ;
#135474=CARTESIAN_POINT('Ctrl Pts',(-21.9900041425516,12.4766942436469,
131.226917109559)) ;
#135475=CARTESIAN_POINT('Ctrl Pts',(-21.8923871793902,12.3681120678918,
130.974864846892)) ;
#135476=CARTESIAN_POINT('Ctrl Pts',(-21.787890239755,12.3353450096833,130.70292564467)) ;
#135477=CARTESIAN_POINT('Ctrl Pts',(-21.6847703934588,12.3808789292608,
130.434751982444)) ;
#135478=CARTESIAN_POINT('Ctrl Pts',(-21.5888638247786,12.5006496739186,
130.187651595634)) ;
#135479=CARTESIAN_POINT('Ctrl Pts',(-21.5062882918341,12.6862348924807,
129.979488344586)) ;
#135480=CARTESIAN_POINT('Ctrl Pts',(-21.4420352783819,12.9253055289241,
129.824962379676)) ;
#135481=CARTESIAN_POINT('Ctrl Pts',(-21.4003702869002,13.1996774467986,
129.7363633676)) ;
#135482=CARTESIAN_POINT('Ctrl Pts',(-21.3833560025974,13.4900583198245,
129.719780265193)) ;
#135483=CARTESIAN_POINT('Ctrl Pts',(-21.3916055296796,13.7765694769724,
129.777104936438)) ;
#135484=CARTESIAN_POINT('Ctrl Pts',(-21.4238225675142,14.036835662277,129.904358363752)) ;
#135485=CARTESIAN_POINT('Ctrl Pts',(-21.4764867420294,14.2522894974628,
130.091167062838)) ;
#135486=CARTESIAN_POINT('Ctrl Pts',(-21.5461349346789,14.410142650821,130.327932770345)) ;
#135487=CARTESIAN_POINT('Ctrl Pts',(-21.6258533196047,14.4959011359271,
130.593837523055)) ;
#135488=CARTESIAN_POINT('Ctrl Pts',(-21.7097706486653,14.5055615596735,
130.872034708298)) ;
#135489=CARTESIAN_POINT('Ctrl Pts',(-21.7915115159255,14.4373879166647,
131.144023400965)) ;
#135490=CARTESIAN_POINT('Ctrl Pts',(-21.8638380594977,14.2968056087925,
131.388393161352)) ;
#135491=CARTESIAN_POINT('Ctrl Pts',(-21.9212551892473,14.0934340145334,
131.589268391717)) ;
#135492=CARTESIAN_POINT('Ctrl Pts',(-21.9586969314941,13.8423638114029,
131.731737544598)) ;
#135493=CARTESIAN_POINT('Ctrl Pts',(-21.9729463381941,13.5615577206812,
131.806433890657)) ;
#135494=CARTESIAN_POINT('Ctrl Pts',(-21.9620894874447,13.2694348944804,
131.807950532534)) ;
#135495=CARTESIAN_POINT('Ctrl Pts',(-21.9263140164209,12.9897647818979,
131.73650343455)) ;
#135496=CARTESIAN_POINT('Ctrl Pts',(-21.8673223314263,12.7403852471457,
131.597325259585)) ;
#135497=CARTESIAN_POINT('Ctrl Pts',(-21.7886865523693,12.5401778472151,
131.400734212814)) ;
#135498=CARTESIAN_POINT('Ctrl Pts',(-21.6953778525397,12.4032538731495,
131.161259541037)) ;
#135499=CARTESIAN_POINT('Ctrl Pts',(-21.5932072064287,12.3392654765734,
130.895922348931)) ;
#135500=CARTESIAN_POINT('Ctrl Pts',(-21.4887973419696,12.3529795705707,
130.624055509138)) ;
#135501=CARTESIAN_POINT('Ctrl Pts',(-21.3889895957889,12.44341496887,130.365620015526)) ;
#135502=CARTESIAN_POINT('Ctrl Pts',(-21.3002278613015,12.6038142404483,
130.13942068693)) ;
#135503=CARTESIAN_POINT('Ctrl Pts',(-21.2279512253468,12.8232746698558,
129.96143747852)) ;
#135504=CARTESIAN_POINT('Ctrl Pts',(-21.1769064226059,13.0848674095602,
129.845368695489)) ;
#135505=CARTESIAN_POINT('Ctrl Pts',(-21.149658170467,13.3712340427374,129.798893618011)) ;
#135506=CARTESIAN_POINT('Ctrl Pts',(-21.1476946959762,13.6620670155129,
129.826365855313)) ;
#135507=CARTESIAN_POINT('Ctrl Pts',(-21.1703666330339,13.9347879219274,
129.92569032549)) ;
#135508=CARTESIAN_POINT('Ctrl Pts',(-21.2152993770454,14.1711547034761,
130.090075797328)) ;
#135509=CARTESIAN_POINT('Ctrl Pts',(-21.2785796529392,14.3538985958079,
130.308060225528)) ;
#135510=CARTESIAN_POINT('Ctrl Pts',(-21.3548663994536,14.4699515410886,
130.564015298951)) ;
#135511=CARTESIAN_POINT('Ctrl Pts',(-21.4380889896721,14.511011729743,130.840261217569)) ;
#135512=CARTESIAN_POINT('Ctrl Pts',(-21.5213196238039,14.4745400421894,
131.116445883889)) ;
#135513=CARTESIAN_POINT('Ctrl Pts',(-21.5987228795245,14.3614974996119,
131.37591886424)) ;
#135514=CARTESIAN_POINT('Ctrl Pts',(-21.6624280158677,14.1829580277845,
131.594943503888)) ;
#135515=CARTESIAN_POINT('Ctrl Pts',(-21.7085901232024,13.9492404929465,
131.762934960253)) ;
#135516=CARTESIAN_POINT('Ctrl Pts',(-21.7325457579653,13.6775800982586,
131.866060493852)) ;
#135517=CARTESIAN_POINT('Ctrl Pts',(-21.7320824211323,13.3886494635436,
131.897743516193)) ;
#135518=CARTESIAN_POINT('Ctrl Pts',(-21.7060357693068,13.0993478015478,
131.855033735375)) ;
#135519=CARTESIAN_POINT('Ctrl Pts',(-21.6563720516456,12.8369458310676,
131.74287352401)) ;
#135520=CARTESIAN_POINT('Ctrl Pts',(-21.5849505607058,12.6140529768099,
131.567486815159)) ;
#135521=CARTESIAN_POINT('Ctrl Pts',(-21.4972346922135,12.4507323341902,
131.344230579028)) ;
#135522=CARTESIAN_POINT('Ctrl Pts',(-21.3977816403119,12.3558899306528,
131.086868664739)) ;
#135523=CARTESIAN_POINT('Ctrl Pts',(-21.2931236526698,12.3380969081111,
130.814378116707)) ;
#135524=CARTESIAN_POINT('Ctrl Pts',(-21.1912351475806,12.3976016694818,
130.549680132567)) ;
#135525=CARTESIAN_POINT('Ctrl Pts',(-21.0970918464179,12.530583824708,130.307814407326)) ;
#135526=CARTESIAN_POINT('Ctrl Pts',(-21.0173249384038,12.7283490506027,
130.108013541003)) ;
#135527=CARTESIAN_POINT('Ctrl Pts',(-20.9573893511929,12.9742771227128,
129.965922835233)) ;
#135528=CARTESIAN_POINT('Ctrl Pts',(-20.9200880297606,13.2539376227601,
129.890167219948)) ;
#135529=CARTESIAN_POINT('Ctrl Pts',(-20.907889243952,13.5450903335013,129.887655062896)) ;
#135530=CARTESIAN_POINT('Ctrl Pts',(-20.920784302057,13.8275787514848,129.958467916581)) ;
#135531=CARTESIAN_POINT('Ctrl Pts',(-20.9569782930972,14.080619519853,130.097260030665)) ;
#135532=CARTESIAN_POINT('Ctrl Pts',(-21.0136849887986,14.2877392133105,
130.296196899106)) ;
#135533=CARTESIAN_POINT('Ctrl Pts',(-21.0849841102122,14.431213841156,130.537392435781)) ;
#135534=CARTESIAN_POINT('Ctrl Pts',(-21.1665056814218,14.5038738166411,
130.808799012005)) ;
#135535=CARTESIAN_POINT('Ctrl Pts',(-21.2505166479721,14.4984557576167,
131.087288159437)) ;
#135536=CARTESIAN_POINT('Ctrl Pts',(-21.3308085825838,14.4164646825051,
131.354946228948)) ;
#135537=CARTESIAN_POINT('Ctrl Pts',(-21.4010755566249,14.2622140461571,
131.593482336718)) ;
#135538=CARTESIAN_POINT('Ctrl Pts',(-21.4547420541191,14.0497489487789,
131.7832014722)) ;
#135539=CARTESIAN_POINT('Ctrl Pts',(-21.4881853748102,13.7905258352839,
131.91413728601)) ;
#135540=CARTESIAN_POINT('Ctrl Pts',(-21.4977462696728,13.506486494377,131.975100243164)) ;
#135541=CARTESIAN_POINT('Ctrl Pts',(-21.4819835887124,13.2142515667239,
131.96236180773)) ;
#135542=CARTESIAN_POINT('Ctrl Pts',(-21.4419223606185,12.9406232851689,
131.878185903014)) ;
#135543=CARTESIAN_POINT('Ctrl Pts',(-21.3786934156362,12.6982138740687,
131.726763051586)) ;
#135544=CARTESIAN_POINT('Ctrl Pts',(-21.2972126241658,12.5096112048297,
131.521723412285)) ;
#135545=CARTESIAN_POINT('Ctrl Pts',(-21.2011850848722,12.3850648620669,
131.274514023005)) ;
#135546=CARTESIAN_POINT('Ctrl Pts',(-21.0984907761846,12.3359713268051,
131.007507556083)) ;
#135547=CARTESIAN_POINT('Ctrl Pts',(-20.9944877940312,12.3641515700291,
130.736812488399)) ;
#135548=CARTESIAN_POINT('Ctrl Pts',(-20.8961804382662,12.4683944776065,
130.482779938443)) ;
#135549=CARTESIAN_POINT('Ctrl Pts',(-20.8099546373725,12.6414744910879,
130.264081389746)) ;
#135550=CARTESIAN_POINT('Ctrl Pts',(-20.7415876002801,12.8692739707259,
130.097372977444)) ;
#135551=CARTESIAN_POINT('Ctrl Pts',(-20.6945289877427,13.1394382839076,
129.993253900407)) ;
#135552=CARTESIAN_POINT('Ctrl Pts',(-20.672298328365,13.4257125423889,129.961149556797)) ;
#135553=CARTESIAN_POINT('Ctrl Pts',(-20.6750007501078,13.7153678926771,
130.002310555712)) ;
#135554=CARTESIAN_POINT('Ctrl Pts',(-20.7020667565521,13.9823826092166,
130.114434508231)) ;
#135555=CARTESIAN_POINT('Ctrl Pts',(-20.7509060316579,14.210351268189,130.290309073817)) ;
#135556=CARTESIAN_POINT('Ctrl Pts',(-20.8169604036749,14.3810373513132,
130.516327937223)) ;
#135557=CARTESIAN_POINT('Ctrl Pts',(-20.8950665489886,14.4835203874639,
130.777619160747)) ;
#135558=CARTESIAN_POINT('Ctrl Pts',(-20.9787343216663,14.5102051470099,
131.055116750985)) ;
#135559=CARTESIAN_POINT('Ctrl Pts',(-21.0618484768981,14.4584272467564,
131.331220006128)) ;
#135560=CARTESIAN_POINT('Ctrl Pts',(-21.1364526301434,14.3332271538461,
131.582140708526)) ;
#135561=CARTESIAN_POINT('Ctrl Pts',(-21.1976622623504,14.1422679027751,
131.794126036847)) ;
#135562=CARTESIAN_POINT('Ctrl Pts',(-21.23975721544,13.9003526545792,131.950166196499)) ;
#135563=CARTESIAN_POINT('Ctrl Pts',(-21.2592791168289,13.6237176044633,
132.040346931511)) ;
#135564=CARTESIAN_POINT('Ctrl Pts',(-21.2539545891703,13.3329588361478,
132.057910063551)) ;
#135565=CARTESIAN_POINT('Ctrl Pts',(-21.2234510913761,13.0482791472687,
132.00196258976)) ;
#135566=CARTESIAN_POINT('Ctrl Pts',(-21.1691539099102,12.7905984211716,
131.876506766355)) ;
#135567=CARTESIAN_POINT('Ctrl Pts',(-21.0947340593749,12.5792074314873,
131.692098693563)) ;
#135568=CARTESIAN_POINT('Ctrl Pts',(-21.0040480835755,12.4271420328258,
131.460337471105)) ;
#135569=CARTESIAN_POINT('Ctrl Pts',(-20.9032486407606,12.3466854620337,
131.199002527252)) ;
#135570=CARTESIAN_POINT('Ctrl Pts',(-20.7987770579087,12.3433384451733,
130.926945640301)) ;
#135571=CARTESIAN_POINT('Ctrl Pts',(-20.6974847568586,12.417256873973,130.664144724903)) ;
#135572=CARTESIAN_POINT('Ctrl Pts',(-20.6057021506296,12.5633304568432,
130.429162568903)) ;
#135573=CARTESIAN_POINT('Ctrl Pts',(-20.5294560018403,12.7708593905581,
130.239538039818)) ;
#135574=CARTESIAN_POINT('Ctrl Pts',(-20.4733463103174,13.025326349885,130.108769986711)) ;
#135575=CARTESIAN_POINT('Ctrl Pts',(-20.4407772110818,13.3082178025067,
130.046756066484)) ;
#135576=CARTESIAN_POINT('Ctrl Pts',(-20.4333100328866,13.5990344955289,
130.058039052296)) ;
#135577=CARTESIAN_POINT('Ctrl Pts',(-20.4506880067864,13.8774216043795,
130.141913702905)) ;
#135578=CARTESIAN_POINT('Ctrl Pts',(-20.4911818153333,14.1239848990119,
130.293425636597)) ;
#135579=CARTESIAN_POINT('Ctrl Pts',(-20.5507855806424,14.3192776170792,
130.500609692184)) ;
#135580=CARTESIAN_POINT('Ctrl Pts',(-20.6247405377758,14.4507732360595,
130.749766053951)) ;
#135581=CARTESIAN_POINT('Ctrl Pts',(-20.7069579624013,14.5087792678555,
131.023045402965)) ;
#135582=CARTESIAN_POINT('Ctrl Pts',(-20.7911628034135,14.4887238336712,
131.302264434157)) ;
#135583=CARTESIAN_POINT('Ctrl Pts',(-20.8697693366433,14.3928285084541,
131.564906273796)) ;
#135584=CARTESIAN_POINT('Ctrl Pts',(-20.9374577677181,14.2263682040696,
131.795916170133)) ;
#135585=CARTESIAN_POINT('Ctrl Pts',(-20.9876137387477,14.0038696460673,
131.975425509327)) ;
#135586=CARTESIAN_POINT('Ctrl Pts',(-21.0167121922335,13.7389372008462,
132.093575454873)) ;
#135587=CARTESIAN_POINT('Ctrl Pts',(-21.021624803058,13.4518073715824,132.141010517718)) ;
#135588=CARTESIAN_POINT('Ctrl Pts',(-21.001265184062,13.1616327439453,132.114737089628)) ;
#135589=CARTESIAN_POINT('Ctrl Pts',(-20.9563235153239,12.8906304372966,
132.016607385205)) ;
#135590=CARTESIAN_POINT('Ctrl Pts',(-20.8895478488704,12.6585325321797,
131.854601473478)) ;
#135591=CARTESIAN_POINT('Ctrl Pts',(-20.8050290649649,12.4808578746759,
131.640730446969)) ;
#135592=CARTESIAN_POINT('Ctrl Pts',(-20.706854482996,12.369794968941,131.387313297938)) ;
#135593=CARTESIAN_POINT('Ctrl Pts',(-20.6035841518815,12.3353140243209,
131.118587941619)) ;
#135594=CARTESIAN_POINT('Ctrl Pts',(-20.4999425243112,12.3783402005982,
130.849020652898)) ;
#135595=CARTESIAN_POINT('Ctrl Pts',(-20.4037610912831,12.4961137906607,
130.601107675479)) ;
#135596=CARTESIAN_POINT('Ctrl Pts',(-20.3206161817449,12.6800956082709,
130.391318319672)) ;
#135597=CARTESIAN_POINT('Ctrl Pts',(-20.2557578107062,12.9180877152906,
130.235043956869)) ;
#135598=CARTESIAN_POINT('Ctrl Pts',(-20.2134909793572,13.1911275173993,
130.144619104063)) ;
#135599=CARTESIAN_POINT('Ctrl Pts',(-20.1956945315034,13.4815072415882,
130.125770538085)) ;
#135600=CARTESIAN_POINT('Ctrl Pts',(-20.2032544219231,13.7684314308885,
130.181084199128)) ;
#135601=CARTESIAN_POINT('Ctrl Pts',(-20.2346242895992,14.029076308477,130.305758033525)) ;
#135602=CARTESIAN_POINT('Ctrl Pts',(-20.2871102678795,14.2473093926041,
130.492262967075)) ;
#135603=CARTESIAN_POINT('Ctrl Pts',(-20.3557014691764,14.4057091519906,
130.725627737145)) ;
#135604=CARTESIAN_POINT('Ctrl Pts',(-20.4356832288713,14.4946178708306,
130.992528144001)) ;
#135605=CARTESIAN_POINT('Ctrl Pts',(-20.5195606513706,14.5063975208026,
131.270592829057)) ;
#135606=CARTESIAN_POINT('Ctrl Pts',(-20.601669735203,14.4401278585609,131.543748083559)) ;
#135607=CARTESIAN_POINT('Ctrl Pts',(-20.6740334559909,14.3020001323071,
131.788087967881)) ;
#135608=CARTESIAN_POINT('Ctrl Pts',(-20.7320052756849,14.100380875427,131.990589852135)) ;
#135609=CARTESIAN_POINT('Ctrl Pts',(-20.7701334334659,13.8504602239821,
132.135070902885)) ;
#135610=CARTESIAN_POINT('Ctrl Pts',(-20.7851220054825,13.5690360496352,
132.212066464694)) ;
#135611=CARTESIAN_POINT('Ctrl Pts',(-20.7749067351906,13.277347744237,132.215406858043)) ;
#135612=CARTESIAN_POINT('Ctrl Pts',(-20.739950771466,12.9978265767653,132.146263744771)) ;
#135613=CARTESIAN_POINT('Ctrl Pts',(-20.6815482067024,12.747023860199,132.008839074771)) ;
#135614=CARTESIAN_POINT('Ctrl Pts',(-20.6035221230103,12.5453431667421,
131.813989900865)) ;
#135615=CARTESIAN_POINT('Ctrl Pts',(-20.5104128505178,12.4062333259034,
131.575152883014)) ;
#135616=CARTESIAN_POINT('Ctrl Pts',(-20.4087091658857,12.3400677949455,
131.311081123435)) ;
#135617=CARTESIAN_POINT('Ctrl Pts',(-20.303791085454,12.3515722965719,131.037884994155)) ;
#135618=CARTESIAN_POINT('Ctrl Pts',(-20.2041191745575,12.4396025465946,
130.779723997866)) ;
#135619=CARTESIAN_POINT('Ctrl Pts',(-20.1147712529316,12.5983879462257,
130.551883797315)) ;
#135620=CARTESIAN_POINT('Ctrl Pts',(-20.0421585923302,12.8155081778463,
130.372801469089)) ;
#135621=CARTESIAN_POINT('Ctrl Pts',(-19.9900861703505,13.0777480891852,
130.253944896754)) ;
#135622=CARTESIAN_POINT('Ctrl Pts',(-19.9622906553043,13.3640007134148,
130.205892912972)) ;
#135623=CARTESIAN_POINT('Ctrl Pts',(-19.9596040305283,13.6530970190172,
130.231033720601)) ;
#135624=CARTESIAN_POINT('Ctrl Pts',(-19.9815947583038,13.9274410550996,
130.328465672942)) ;
#135625=CARTESIAN_POINT('Ctrl Pts',(-20.0259169621657,14.1649405448642,
130.491043143204)) ;
#135626=CARTESIAN_POINT('Ctrl Pts',(-20.0889049637749,14.3499176915205,
130.708260928926)) ;
#135627=CARTESIAN_POINT('Ctrl Pts',(-20.1649263048442,14.4676736740884,
130.963435819328)) ;
#135628=CARTESIAN_POINT('Ctrl Pts',(-20.247688472556,14.5109849198275,131.238193829716)) ;
#135629=CARTESIAN_POINT('Ctrl Pts',(-20.331483197017,14.4763368011369,131.516227084564)) ;
#135630=CARTESIAN_POINT('Ctrl Pts',(-20.4085145537121,14.3664425274482,
131.774319022009)) ;
#135631=CARTESIAN_POINT('Ctrl Pts',(-20.4732700628347,14.1882602546085,
131.996710354005)) ;
#135632=CARTESIAN_POINT('Ctrl Pts',(-20.5197600667737,13.9563928712726,
132.165546655575)) ;
#135633=CARTESIAN_POINT('Ctrl Pts',(-20.544429934519,13.6856075071528,132.270760904427)) ;
#135634=CARTESIAN_POINT('Ctrl Pts',(-20.5446218153691,13.3967978155194,
132.304370094684)) ;
#135635=CARTESIAN_POINT('Ctrl Pts',(-20.5194831662747,13.1083772147109,
132.264162983921)) ;
#135636=CARTESIAN_POINT('Ctrl Pts',(-20.4702619913672,12.8436201216384,
132.15346806604)) ;
#135637=CARTESIAN_POINT('Ctrl Pts',(-20.3994698940617,12.6197329650473,
131.979865314557)) ;
#135638=CARTESIAN_POINT('Ctrl Pts',(-20.3120006020497,12.4541610182818,
131.75739537006)) ;
#135639=CARTESIAN_POINT('Ctrl Pts',(-20.2125860830344,12.3575181073951,
131.500199627294)) ;
#135640=CARTESIAN_POINT('Ctrl Pts',(-20.1088815096965,12.337407534574,131.230203979974)) ;
#135641=CARTESIAN_POINT('Ctrl Pts',(-20.0060146641454,12.3950240477661,
130.962919259217)) ;
#135642=CARTESIAN_POINT('Ctrl Pts',(-19.9119864658295,12.5255974682326,
130.721236187127)) ;
#135643=CARTESIAN_POINT('Ctrl Pts',(-19.8314897395286,12.7221236513144,
130.519397456966)) ;
#135644=CARTESIAN_POINT('Ctrl Pts',(-19.7710089279874,12.966643820031,130.375676004731)) ;
#135645=CARTESIAN_POINT('Ctrl Pts',(-19.732928013481,13.2467842966359,130.297774420096)) ;
#135646=CARTESIAN_POINT('Ctrl Pts',(-19.7201400299444,13.5364084867458,
130.293371523372)) ;
#135647=CARTESIAN_POINT('Ctrl Pts',(-19.7322324408918,13.819301352246,130.361818332685)) ;
#135648=CARTESIAN_POINT('Ctrl Pts',(-19.7678249009645,14.0737430594077,
130.498891515294)) ;
#135649=CARTESIAN_POINT('Ctrl Pts',(-19.8239107737393,14.2823383256047,
130.695974069195)) ;
#135650=CARTESIAN_POINT('Ctrl Pts',(-19.8950604586474,14.4280819786068,
130.936830915041)) ;
#135651=CARTESIAN_POINT('Ctrl Pts',(-19.9759986631136,14.5027907188546,
131.20637093887)) ;
#135652=CARTESIAN_POINT('Ctrl Pts',(-20.0606762821136,14.4996009182714,
131.487070199978)) ;
#135653=CARTESIAN_POINT('Ctrl Pts',(-20.1407098011001,14.4198435135005,
131.753794032065)) ;
#135654=CARTESIAN_POINT('Ctrl Pts',(-20.2112630859601,14.2682255575811,
131.993092362855)) ;
#135655=CARTESIAN_POINT('Ctrl Pts',(-20.2656775957736,14.0566692320112,
132.185107721384)) ;
#135656=CARTESIAN_POINT('Ctrl Pts',(-20.2997748055791,13.7984046917339,
132.317960439349)) ;
#135657=CARTESIAN_POINT('Ctrl Pts',(-20.3099989318143,13.5146255183712,
132.38088711118)) ;
#135658=CARTESIAN_POINT('Ctrl Pts',(-20.2951296394703,13.22379017507,132.370580468596)) ;
#135659=CARTESIAN_POINT('Ctrl Pts',(-20.2555701663945,12.9476430099182,
132.288081447981)) ;
#135660=CARTESIAN_POINT('Ctrl Pts',(-20.1928769291611,12.7041858709694,
132.138213583783)) ;
#135661=CARTESIAN_POINT('Ctrl Pts',(-20.1120002752265,12.5142908380612,
131.934883468866)) ;
#135662=CARTESIAN_POINT('Ctrl Pts',(-20.0165096996154,12.3877724329813,
131.689173717466)) ;
#135663=CARTESIAN_POINT('Ctrl Pts',(-19.913478604829,12.3361912043238,131.421332336646)) ;
#135664=CARTESIAN_POINT('Ctrl Pts',(-19.8094708653727,12.3624798224069,
131.150606824843)) ;
#135665=CARTESIAN_POINT('Ctrl Pts',(-19.7113062006748,12.4640688022784,
130.896852899496)) ;
#135666=CARTESIAN_POINT('Ctrl Pts',(-19.6243191332476,12.6358046245907,
130.676044087363)) ;
#135667=CARTESIAN_POINT('Ctrl Pts',(-19.5555745074161,12.862048858162,130.508185639822)) ;
#135668=CARTESIAN_POINT('Ctrl Pts',(-19.5079382213539,13.1294243703739,
130.402168639634)) ;
#135669=CARTESIAN_POINT('Ctrl Pts',(-19.4847311841948,13.419127554444,130.367646107838)) ;
#135670=CARTESIAN_POINT('Ctrl Pts',(-19.486760537507,13.7060585256719,130.406486755971)) ;
#135671=CARTESIAN_POINT('Ctrl Pts',(-19.5132448910941,13.9758635071568,
130.517143788552)) ;
#135672=CARTESIAN_POINT('Ctrl Pts',(-19.561461527867,14.2044690811379,130.691105042514)) ;
#135673=CARTESIAN_POINT('Ctrl Pts',(-19.6271525262166,14.3772046466544,
130.916107336043)) ;
#135674=CARTESIAN_POINT('Ctrl Pts',(-19.7049913038784,14.4817041640368,
131.17660395042)) ;
#135675=CARTESIAN_POINT('Ctrl Pts',(-19.7886768197028,14.5103977605507,
131.454191387136)) ;
#135676=CARTESIAN_POINT('Ctrl Pts',(-19.8713625246764,14.461387716176,131.728812616932)) ;
#135677=CARTESIAN_POINT('Ctrl Pts',(-19.9466960883751,14.3378670523305,
131.982034797292)) ;
#135678=CARTESIAN_POINT('Ctrl Pts',(-20.0083045176645,14.1487649480966,
132.195144873615)) ;
#135679=CARTESIAN_POINT('Ctrl Pts',(-20.0510942154457,13.9077124472436,
132.35327591803)) ;
#135680=CARTESIAN_POINT('Ctrl Pts',(-20.0712746305926,13.6318349091011,
132.445369268278)) ;
#135681=CARTESIAN_POINT('Ctrl Pts',(-20.0666628175852,13.3411961915081,
132.465016541542)) ;
#135682=CARTESIAN_POINT('Ctrl Pts',(-20.0369065317575,13.0563347009616,
132.411215549619)) ;
#135683=CARTESIAN_POINT('Ctrl Pts',(-19.9832697572704,12.7976622253545,
132.287685663652)) ;
#135684=CARTESIAN_POINT('Ctrl Pts',(-19.909474160919,12.584625305209,132.105083184337)) ;
#135685=CARTESIAN_POINT('Ctrl Pts',(-19.8184221729735,12.429833286881,131.872506784025)) ;
#135686=CARTESIAN_POINT('Ctrl Pts',(-19.7187303437125,12.3481748757021,
131.614098966012)) ;
#135687=CARTESIAN_POINT('Ctrl Pts',(-19.6138632113487,12.3422836205948,
131.341022208364)) ;
#135688=CARTESIAN_POINT('Ctrl Pts',(-19.5124594677726,12.414162317258,131.077872115915)) ;
#135689=CARTESIAN_POINT('Ctrl Pts',(-19.420212188348,12.55849168118,130.841573794732)) ;
#135690=CARTESIAN_POINT('Ctrl Pts',(-19.3435324232807,12.7644624942609,
130.65066449742)) ;
#135691=CARTESIAN_POINT('Ctrl Pts',(-19.2868798087134,13.0174115077838,
130.518256914751)) ;
#135692=CARTESIAN_POINT('Ctrl Pts',(-19.2535766304538,13.2998964348547,
130.454116409847)) ;
#135693=CARTESIAN_POINT('Ctrl Pts',(-19.2453729976278,13.5908799629275,
130.463258994527)) ;
#135694=CARTESIAN_POINT('Ctrl Pts',(-19.2621513468008,13.8706960081611,
130.545479006086)) ;
#135695=CARTESIAN_POINT('Ctrl Pts',(-19.3020872042403,14.1180202656557,
130.695329004107)) ;
#135696=CARTESIAN_POINT('Ctrl Pts',(-19.3610103361281,14.3143765894564,
130.900421785235)) ;
#135697=CARTESIAN_POINT('Ctrl Pts',(-19.434812974818,14.4481660809184,131.149213001408)) ;
#135698=CARTESIAN_POINT('Ctrl Pts',(-19.5166794707772,14.5080838606745,
131.421381896559)) ;
#135699=CARTESIAN_POINT('Ctrl Pts',(-19.6008596180551,14.4905518531177,
131.700498217892)) ;
#135700=CARTESIAN_POINT('Ctrl Pts',(-19.679959110775,14.3964092296967,131.964690313878)) ;
#135701=CARTESIAN_POINT('Ctrl Pts',(-19.7478273039877,14.232304987228,132.196115316038)) ;
#135702=CARTESIAN_POINT('Ctrl Pts',(-19.7986192880396,14.0113006854444,
132.37749892765)) ;
#135703=CARTESIAN_POINT('Ctrl Pts',(-19.8284139029138,13.7469853282518,
132.497724021509)) ;
#135704=CARTESIAN_POINT('Ctrl Pts',(-19.8340820683678,13.4601451324146,
132.547372256783)) ;
#135705=CARTESIAN_POINT('Ctrl Pts',(-19.8142531422841,13.1687003200991,
132.522778212001)) ;
#135706=CARTESIAN_POINT('Ctrl Pts',(-19.7703730343976,12.8989650919222,
132.427483609972)) ;
#135707=CARTESIAN_POINT('Ctrl Pts',(-19.7036589079187,12.6635916504989,
132.265932090456)) ;
#135708=CARTESIAN_POINT('Ctrl Pts',(-19.6199118535932,12.485239800862,132.054155238019)) ;
#135709=CARTESIAN_POINT('Ctrl Pts',(-19.5219805853211,12.3719259500599,
131.801473410491)) ;
#135710=CARTESIAN_POINT('Ctrl Pts',(-19.4189379680128,12.3351771032852,
131.53336398971)) ;
#135711=CARTESIAN_POINT('Ctrl Pts',(-19.3148770024859,12.3762351050997,
131.26268009039)) ;
#135712=CARTESIAN_POINT('Ctrl Pts',(-19.2189066435572,12.4911992435135,
131.01519951472)) ;
#135713=CARTESIAN_POINT('Ctrl Pts',(-19.1347439547889,12.6745749260732,
130.802658266804)) ;
#135714=CARTESIAN_POINT('Ctrl Pts',(-19.0695712650756,12.9105841176317,
130.64534787781)) ;
#135715=CARTESIAN_POINT('Ctrl Pts',(-19.026516615279,13.1834575472762,130.552699546602)) ;
#135716=CARTESIAN_POINT('Ctrl Pts',(-19.0081217007437,13.4728172007292,
130.532007746554)) ;
#135717=CARTESIAN_POINT('Ctrl Pts',(-19.0147866964172,13.7593252111675,
130.584597145698)) ;
#135718=CARTESIAN_POINT('Ctrl Pts',(-19.0457740324292,14.0229111380707,
130.708413150787)) ;
#135719=CARTESIAN_POINT('Ctrl Pts',(-19.0973111190571,14.2409568530166,
130.891883602161)) ;
#135720=CARTESIAN_POINT('Ctrl Pts',(-19.165926552844,14.4024702596202,131.125549278518)) ;
#135721=CARTESIAN_POINT('Ctrl Pts',(-19.2454507888212,14.4930252918819,
131.390998297428)) ;
#135722=CARTESIAN_POINT('Ctrl Pts',(-19.3293410740711,14.5071138077779,
131.669126207063)) ;
#135723=CARTESIAN_POINT('Ctrl Pts',(-19.4112821511384,14.4434722304718,
131.941650206842)) ;
#135724=CARTESIAN_POINT('Ctrl Pts',(-19.4842739640058,14.3072991508372,
132.187922760495)) ;
#135725=CARTESIAN_POINT('Ctrl Pts',(-19.5429829781195,14.1061281755834,
132.392741540416)) ;
#135726=CARTESIAN_POINT('Ctrl Pts',(-19.5814898983426,13.8584458365122,
132.538171297678)) ;
#135727=CARTESIAN_POINT('Ctrl Pts',(-19.5972452937213,13.5782527615593,
132.617345758941)) ;
#135728=CARTESIAN_POINT('Ctrl Pts',(-19.587821553024,13.2862405830432,132.623036030091)) ;
#135729=CARTESIAN_POINT('Ctrl Pts',(-19.5535345414538,13.0054673407222,
132.55591759128)) ;
#135730=CARTESIAN_POINT('Ctrl Pts',(-19.4954706738399,12.7527978446706,
132.419600001604)) ;
#135731=CARTESIAN_POINT('Ctrl Pts',(-19.4183727349997,12.5507722085017,
132.227270319449)) ;
#135732=CARTESIAN_POINT('Ctrl Pts',(-19.3255707730553,12.4092693590586,
131.989364894937)) ;
#135733=CARTESIAN_POINT('Ctrl Pts',(-19.2238321783356,12.3409406073707,
131.725254513543)) ;
#135734=CARTESIAN_POINT('Ctrl Pts',(-19.119236753858,12.3499819194409,131.452886617979)) ;
#135735=CARTESIAN_POINT('Ctrl Pts',(-19.0188367516298,12.4363532158425,
131.192772449436)) ;
#135736=CARTESIAN_POINT('Ctrl Pts',(-18.9295447538629,12.5925663631045,
130.964931579883)) ;
#135737=CARTESIAN_POINT('Ctrl Pts',(-18.85618070133,12.8085170384963,130.783729205798)) ;
#135738=CARTESIAN_POINT('Ctrl Pts',(-18.8035406576781,13.0694866152918,
130.663175810496)) ;
#135739=CARTESIAN_POINT('Ctrl Pts',(-18.774944483164,13.3550371201656,130.612758020313)) ;
#135740=CARTESIAN_POINT('Ctrl Pts',(-18.7715872372659,13.6462143005165,
130.636161963138)) ;
#135741=CARTESIAN_POINT('Ctrl Pts',(-18.7928313609646,13.9195287631536,
130.73120381732)) ;
#135742=CARTESIAN_POINT('Ctrl Pts',(-18.8365269344384,14.1586150899391,
130.891977988719)) ;
#135743=CARTESIAN_POINT('Ctrl Pts',(-18.8989146423201,14.3449689837057,
131.10737481057)) ;
#135744=CARTESIAN_POINT('Ctrl Pts',(-18.9745793166611,14.465239738532,131.36150472704)) ;
#135745=CARTESIAN_POINT('Ctrl Pts',(-19.0578793507872,14.5107689866746,
131.638093119859)) ;
#135746=CARTESIAN_POINT('Ctrl Pts',(-19.1409583613005,14.4787461978325,
131.913707901465)) ;
#135747=CARTESIAN_POINT('Ctrl Pts',(-19.2189706552468,14.3700644324197,
132.17497387013)) ;
#135748=CARTESIAN_POINT('Ctrl Pts',(-19.2836848317943,14.1946408166751,
132.397013538057)) ;
#135749=CARTESIAN_POINT('Ctrl Pts',(-19.3309065027156,13.963907732595,132.568053904224)) ;
#135750=CARTESIAN_POINT('Ctrl Pts',(-19.3562835215805,13.6940409321305,
132.675319682935)) ;
#135751=CARTESIAN_POINT('Ctrl Pts',(-19.3571223286895,13.4043243937501,
132.710955989412)) ;
#135752=CARTESIAN_POINT('Ctrl Pts',(-19.3329129352278,13.1175424358185,
132.673226068229)) ;
#135753=CARTESIAN_POINT('Ctrl Pts',(-19.284075134649,12.8501254079525,132.563869228407)) ;
#135754=CARTESIAN_POINT('Ctrl Pts',(-19.2141838640519,12.6260375389968,
132.392718948333)) ;
#135755=CARTESIAN_POINT('Ctrl Pts',(-19.1270338823226,12.4581545252769,
132.171242119684)) ;
#135756=CARTESIAN_POINT('Ctrl Pts',(-19.0280972219191,12.3594525497003,
131.915366042047)) ;
#135757=CARTESIAN_POINT('Ctrl Pts',(-18.9241027514417,12.3367944069397,
131.644635976731)) ;
#135758=CARTESIAN_POINT('Ctrl Pts',(-18.8208265565642,12.3925085409291,
131.376240849143)) ;
#135759=CARTESIAN_POINT('Ctrl Pts',(-18.7265133411892,12.5213898755188,
131.133731510503)) ;
#135760=CARTESIAN_POINT('Ctrl Pts',(-18.6457952560714,12.7155724021421,
130.931131518529)) ;
#135761=CARTESIAN_POINT('Ctrl Pts',(-18.5846065804363,12.9595220676015,
130.785423050799)) ;
#135762=CARTESIAN_POINT('Ctrl Pts',(-18.546066469657,13.2367788940881,130.70592009773)) ;
#135763=CARTESIAN_POINT('Ctrl Pts',(-18.5323213213029,13.5277643625836,
130.698889739784)) ;
#135764=CARTESIAN_POINT('Ctrl Pts',(-18.543793348028,13.8120453761231,130.765623615628)) ;
#135765=CARTESIAN_POINT('Ctrl Pts',(-18.5788549474306,14.0676654739834,
130.901176319765)) ;
#135766=CARTESIAN_POINT('Ctrl Pts',(-18.6343035780449,14.2771419928287,
131.096308854122)) ;
#135767=CARTESIAN_POINT('Ctrl Pts',(-18.7050835708224,14.425031880978,131.336092927187)) ;
#135768=CARTESIAN_POINT('Ctrl Pts',(-18.7861994089251,14.5017260060049,
131.60629231186)) ;
#135769=CARTESIAN_POINT('Ctrl Pts',(-18.8699095303306,14.5010099059246,
131.883776032442)) ;
#135770=CARTESIAN_POINT('Ctrl Pts',(-18.950862117856,14.4231233705973,132.153475808602)) ;
#135771=CARTESIAN_POINT('Ctrl Pts',(-19.0216063325537,14.2735700722065,
132.393250548626)) ;
#135772=CARTESIAN_POINT('Ctrl Pts',(-19.0766525736922,14.0631260843178,
132.587185321685)) ;
#135773=CARTESIAN_POINT('Ctrl Pts',(-19.1112752517511,13.8068513237717,
132.721449739404)) ;
#135774=CARTESIAN_POINT('Ctrl Pts',(-19.1222768851844,13.5229068768556,
132.786731908381)) ;
#135775=CARTESIAN_POINT('Ctrl Pts',(-19.1081388609896,13.2323185296325,
132.778518604924)) ;
#135776=CARTESIAN_POINT('Ctrl Pts',(-19.0692979350921,12.955462422634,132.698120669452)) ;
#135777=CARTESIAN_POINT('Ctrl Pts',(-19.0072938758856,12.7108337306576,
132.550242420851)) ;
#135778=CARTESIAN_POINT('Ctrl Pts',(-18.9267369862212,12.5189036902296,
132.347912261719)) ;
#135779=CARTESIAN_POINT('Ctrl Pts',(-18.8318784493428,12.3906586207823,
132.103941582259)) ;
#135780=CARTESIAN_POINT('Ctrl Pts',(-18.7288363533557,12.3366531336248,
131.836123081131)) ;
#135781=CARTESIAN_POINT('Ctrl Pts',(-18.624925410328,12.360297772879,131.565617456112)) ;
#135782=CARTESIAN_POINT('Ctrl Pts',(-18.5256578035359,12.4609988515391,
131.308947306111)) ;
#135783=CARTESIAN_POINT('Ctrl Pts',(-18.4392051331275,12.6291274638668,
131.089332236554)) ;
#135784=CARTESIAN_POINT('Ctrl Pts',(-18.3692689876453,12.8555169755094,
130.918257614385)) ;
#135785=CARTESIAN_POINT('Ctrl Pts',(-18.3212190683975,13.1215885522129,
130.810953330662)) ;
#135786=CARTESIAN_POINT('Ctrl Pts',(-18.2972960902934,13.4096083938423,
130.774191778671)) ;
#135787=CARTESIAN_POINT('Ctrl Pts',(-18.2985416991129,13.698212942693,130.810897551179)) ;
#135788=CARTESIAN_POINT('Ctrl Pts',(-18.3244750392328,13.9691452295141,
130.91998909622)) ;
#135789=CARTESIAN_POINT('Ctrl Pts',(-18.3719691340465,14.1982918407705,
131.091726472608)) ;
#135790=CARTESIAN_POINT('Ctrl Pts',(-18.437100638801,14.3728095621698,131.315054734931)) ;
#135791=CARTESIAN_POINT('Ctrl Pts',(-18.5147502122421,14.479662285758,131.575038501861)) ;
#135792=CARTESIAN_POINT('Ctrl Pts',(-18.5984271700058,14.5107460879228,
131.852624565577)) ;
#135793=CARTESIAN_POINT('Ctrl Pts',(-18.6814592251425,14.4636147982726,
132.128355723987)) ;
#135794=CARTESIAN_POINT('Ctrl Pts',(-18.7567611079911,14.3427084720644,
132.38133252825)) ;
#135795=CARTESIAN_POINT('Ctrl Pts',(-18.8191499212685,14.1545214106307,
132.596878690056)) ;
#135796=CARTESIAN_POINT('Ctrl Pts',(-18.8624161383915,13.914665784431,132.756380600079)) ;
#135797=CARTESIAN_POINT('Ctrl Pts',(-18.8832226690577,13.6405172708492,
132.850185928448)) ;
#135798=CARTESIAN_POINT('Ctrl Pts',(-18.879379985006,13.3501102818962,132.872073497633)) ;
#135799=CARTESIAN_POINT('Ctrl Pts',(-18.8504830366193,13.0651843315454,
132.820727303234)) ;
#135800=CARTESIAN_POINT('Ctrl Pts',(-18.7972049191449,12.80388772374,132.698441638351)) ;
#135801=CARTESIAN_POINT('Ctrl Pts',(-18.723938579695,12.5899465270377,132.517340764542)) ;
#135802=CARTESIAN_POINT('Ctrl Pts',(-18.6339631078438,12.4339563210189,
132.28768165985)) ;
#135803=CARTESIAN_POINT('Ctrl Pts',(-18.533655418016,12.3491846989202,132.027754670765)) ;
#135804=CARTESIAN_POINT('Ctrl Pts',(-18.4287414629348,12.3415474281895,
131.754556958259)) ;
#135805=CARTESIAN_POINT('Ctrl Pts',(-18.3275546121177,12.4110292201394,
131.491915929484)) ;
#135806=CARTESIAN_POINT('Ctrl Pts',(-18.2349169164515,12.5533605448057,
131.254484931781)) ;
#135807=CARTESIAN_POINT('Ctrl Pts',(-18.1578099509812,12.7574391512257,
131.062286140571)) ;
#135808=CARTESIAN_POINT('Ctrl Pts',(-18.1003696787992,13.0095817126533,
130.92762938283)) ;
#135809=CARTESIAN_POINT('Ctrl Pts',(-18.0663253206741,13.2928226801242,
130.861470362866)) ;
#135810=CARTESIAN_POINT('Ctrl Pts',(-18.0574821752941,13.5820119966617,
130.868533156755)) ;
#135811=CARTESIAN_POINT('Ctrl Pts',(-18.0735684910089,13.8633229249982,
130.948835515899)) ;
#135812=CARTESIAN_POINT('Ctrl Pts',(-18.1128079244624,14.1112602779132,
131.096570682687)) ;
#135813=CARTESIAN_POINT('Ctrl Pts',(-18.1713264366975,14.3095521754014,
131.300538449874)) ;
#135814=CARTESIAN_POINT('Ctrl Pts',(-18.2445253330056,14.4451057235358,
131.547453993518)) ;
#135815=CARTESIAN_POINT('Ctrl Pts',(-18.3269176211252,14.5076745769451,
131.821434215678)) ;
#135816=CARTESIAN_POINT('Ctrl Pts',(-18.4109135921778,14.4918702514085,
132.09992274832)) ;
#135817=CARTESIAN_POINT('Ctrl Pts',(-18.4899530140776,14.4001695900989,
132.363825830347)) ;
#135818=CARTESIAN_POINT('Ctrl Pts',(-18.5581972721776,14.238339270588,132.596306467926)) ;
#135819=CARTESIAN_POINT('Ctrl Pts',(-18.6097312244741,14.0178457541506,
132.77999745246)) ;
#135820=CARTESIAN_POINT('Ctrl Pts',(-18.6401448193709,13.7549024704848,
132.901969265826)) ;
#135821=CARTESIAN_POINT('Ctrl Pts',(-18.6463850313128,13.4669383655623,
132.953465269722)) ;
#135822=CARTESIAN_POINT('Ctrl Pts',(-18.6276503009215,13.1792878389568,
132.931593942622)) ;
#135823=CARTESIAN_POINT('Ctrl Pts',(-18.5840179153444,12.9054935275296,
132.837423835677)) ;
#135824=CARTESIAN_POINT('Ctrl Pts',(-18.5184918875895,12.6708451835732,
132.679031311941)) ;
#135825=CARTESIAN_POINT('Ctrl Pts',(-18.4344363065144,12.4890109361581,
132.466673752346)) ;
#135826=CARTESIAN_POINT('Ctrl Pts',(-18.3378254602386,12.3747427440592,
132.217485900113)) ;
#135827=CARTESIAN_POINT('Ctrl Pts',(-18.2341291109171,12.335118127865,131.947725095572)) ;
#135828=CARTESIAN_POINT('Ctrl Pts',(-18.1304829793124,12.3735357257966,
131.678071654494)) ;
#135829=CARTESIAN_POINT('Ctrl Pts',(-18.0332195672274,12.4876827050984,
131.427169660191)) ;
#135830=CARTESIAN_POINT('Ctrl Pts',(-17.9493134502573,12.668143871092,131.215113064817)) ;
#135831=CARTESIAN_POINT('Ctrl Pts',(-17.8833190355393,12.9033827829949,
131.055504217813)) ;
#135832=CARTESIAN_POINT('Ctrl Pts',(-17.8397509602161,13.1743601664502,
130.961218011576)) ;
#135833=CARTESIAN_POINT('Ctrl Pts',(-17.8204668396867,13.4644840041335,
130.938043352746)) ;
#135834=CARTESIAN_POINT('Ctrl Pts',(-17.8265350254978,13.7518155739233,
130.988946607329)) ;
#135835=CARTESIAN_POINT('Ctrl Pts',(-17.8566012791567,14.0147480425275,
131.109855058721)) ;
#135836=CARTESIAN_POINT('Ctrl Pts',(-17.90786398017,14.2359322469135,131.292745615315)) ;
#135837=CARTESIAN_POINT('Ctrl Pts',(-17.9762298617494,14.3990328419962,
131.525712867481)) ;
#135838=CARTESIAN_POINT('Ctrl Pts',(-18.055065638864,14.4913721211862,131.788962667964)) ;
#135839=CARTESIAN_POINT('Ctrl Pts',(-18.1393991985355,14.5077030613306,
132.068583449212)) ;
#135840=CARTESIAN_POINT('Ctrl Pts',(-18.2210461373333,14.4466726935246,
132.340051735665)) ;
#135841=CARTESIAN_POINT('Ctrl Pts',(-18.2950035387414,14.3110620977678,
132.589454770925)) ;
#135842=CARTESIAN_POINT('Ctrl Pts',(-18.3535868279914,14.1132680684101,
132.793577578567)) ;
#135843=CARTESIAN_POINT('Ctrl Pts',(-18.393011856418,13.8656264960883,132.941870264204)) ;
#135844=CARTESIAN_POINT('Ctrl Pts',(-18.4093627200831,13.5853317318957,
133.022849013586)) ;
#135845=CARTESIAN_POINT('Ctrl Pts',(-18.4005900814448,13.2939513094312,
133.030374526169)) ;
#135846=CARTESIAN_POINT('Ctrl Pts',(-18.3670959101891,13.0136081090702,
132.965460512865)) ;
#135847=CARTESIAN_POINT('Ctrl Pts',(-18.3099441323283,12.7604084565328,
132.831704484875)) ;
#135848=CARTESIAN_POINT('Ctrl Pts',(-18.2330287799136,12.5556140537718,
132.640069906698)) ;
#135849=CARTESIAN_POINT('Ctrl Pts',(-18.1403993250708,12.412162783817,132.402717407191)) ;
#135850=CARTESIAN_POINT('Ctrl Pts',(-18.039122761627,12.3419224833159,132.139862058296)) ;
#135851=CARTESIAN_POINT('Ctrl Pts',(-17.9346214328855,12.3485705631489,
131.867734666129)) ;
#135852=CARTESIAN_POINT('Ctrl Pts',(-17.8340398826189,12.4325162173742,
131.60707108893)) ;
#135853=CARTESIAN_POINT('Ctrl Pts',(-17.7440580525167,12.5872706018155,
131.377320640071)) ;
#135854=CARTESIAN_POINT('Ctrl Pts',(-17.6702459325862,12.8016741765326,
131.1947873473)) ;
#135855=CARTESIAN_POINT('Ctrl Pts',(-17.6170393754709,13.0608926757193,
131.072495055625)) ;
#135856=CARTESIAN_POINT('Ctrl Pts',(-17.5876611427528,13.3463627388947,
131.019840506949)) ;
#135857=CARTESIAN_POINT('Ctrl Pts',(-17.5835099051843,13.6367413735624,
131.040812586735)) ;
#135858=CARTESIAN_POINT('Ctrl Pts',(-17.6040712549613,13.912123441329,131.134008457263)) ;
#135859=CARTESIAN_POINT('Ctrl Pts',(-17.6473147092117,14.1528033236638,
131.293522210415)) ;
#135860=CARTESIAN_POINT('Ctrl Pts',(-17.7090710684674,14.3402810134416,
131.506980670982)) ;
#135861=CARTESIAN_POINT('Ctrl Pts',(-17.784324421975,14.4626257099404,131.759874983544)) ;
#135862=CARTESIAN_POINT('Ctrl Pts',(-17.8676273435361,14.5106364099982,
132.036519206507)) ;
#135863=CARTESIAN_POINT('Ctrl Pts',(-17.9509431998974,14.4805445966973,
132.31289642704)) ;
#135864=CARTESIAN_POINT('Ctrl Pts',(-18.0287637016259,14.3748126779467,
132.57339232087)) ;
#135865=CARTESIAN_POINT('Ctrl Pts',(-18.0942745357637,14.2005693776624,
132.797921352006)) ;
#135866=CARTESIAN_POINT('Ctrl Pts',(-18.1420291731984,13.9714224956824,
132.970479780879)) ;
#135867=CARTESIAN_POINT('Ctrl Pts',(-18.1681061343277,13.7016038456452,
133.07989078727)) ;
#135868=CARTESIAN_POINT('Ctrl Pts',(-18.1697184694213,13.4137877720204,
133.117594113432)) ;
#135869=CARTESIAN_POINT('Ctrl Pts',(-18.1460719924332,13.1249621059971,
133.081716204354)) ;
#135870=CARTESIAN_POINT('Ctrl Pts',(-18.098349112227,12.858759801946,132.975335138158)) ;
#135871=CARTESIAN_POINT('Ctrl Pts',(-18.0285125557916,12.6311849064932,
132.804627705542)) ;
#135872=CARTESIAN_POINT('Ctrl Pts',(-17.9419067380147,12.4620614418067,
132.584665021202)) ;
#135873=CARTESIAN_POINT('Ctrl Pts',(-17.8431161137062,12.3611529243014,
132.329254527925)) ;
#135874=CARTESIAN_POINT('Ctrl Pts',(-17.7394163400758,12.336402737043,132.059308529178)) ;
#135875=CARTESIAN_POINT('Ctrl Pts',(-17.636008023939,12.3896954767389,131.790522379684)) ;
#135876=CARTESIAN_POINT('Ctrl Pts',(-17.5411529235148,12.5169545730866,
131.54651181945)) ;
#135877=CARTESIAN_POINT('Ctrl Pts',(-17.4601656512396,12.7090014500136,
131.343041028757)) ;
#135878=CARTESIAN_POINT('Ctrl Pts',(-17.3982954159609,12.9518209129291,
131.195365244849)) ;
#135879=CARTESIAN_POINT('Ctrl Pts',(-17.3590590475251,13.2283911259786,
131.113826328101)) ;
#135880=CARTESIAN_POINT('Ctrl Pts',(-17.3445909288019,13.5192444476926,
131.104682525303)) ;
#135881=CARTESIAN_POINT('Ctrl Pts',(-17.3552759397806,13.8035929406365,
131.169057687742)) ;
#135882=CARTESIAN_POINT('Ctrl Pts',(-17.3897650651813,14.0607675161601,
131.30300701978)) ;
#135883=CARTESIAN_POINT('Ctrl Pts',(-17.4443353177419,14.2709776513911,
131.49540177985)) ;
#135884=CARTESIAN_POINT('Ctrl Pts',(-17.5152284115638,14.4220258151157,
131.735762483094)) ;
#135885=CARTESIAN_POINT('Ctrl Pts',(-17.5958972727999,14.5004899933202,
132.004539334194)) ;
#135886=CARTESIAN_POINT('Ctrl Pts',(-17.6797407048686,14.5020985766214,
132.282472815977)) ;
#135887=CARTESIAN_POINT('Ctrl Pts',(-17.7606887259789,14.426667623352,132.552070316538)) ;
#135888=CARTESIAN_POINT('Ctrl Pts',(-17.8320641853255,14.2786158189735,
132.79380669298)) ;
#135889=CARTESIAN_POINT('Ctrl Pts',(-17.8875765378756,14.0697690186074,
132.989079973035)) ;
#135890=CARTESIAN_POINT('Ctrl Pts',(-17.922834488677,13.8142976320865,133.125231432651)) ;
#135891=CARTESIAN_POINT('Ctrl Pts',(-17.9345112522901,13.5318062075926,
133.19237603013)) ;
#135892=CARTESIAN_POINT('Ctrl Pts',(-17.9211404368569,13.2403761874523,
133.186487415733)) ;
#135893=CARTESIAN_POINT('Ctrl Pts',(-17.8827207165006,12.9618561593774,
133.107451653599)) ;
#135894=CARTESIAN_POINT('Ctrl Pts',(-17.821581417852,12.7173263730279,132.96193349821)) ;
#135895=CARTESIAN_POINT('Ctrl Pts',(-17.7413926221805,12.5233446886838,
132.760735766704)) ;
#135896=CARTESIAN_POINT('Ctrl Pts',(-17.6467746618759,12.3931312315505,
132.517486220828)) ;
#135897=CARTESIAN_POINT('Ctrl Pts',(-17.5437035922363,12.337075246258,132.249632321582)) ;
#135898=CARTESIAN_POINT('Ctrl Pts',(-17.4401454160532,12.3586764449227,
131.98003227223)) ;
#135899=CARTESIAN_POINT('Ctrl Pts',(-17.3410665934673,12.4563696314589,
131.723751639427)) ;
#135900=CARTESIAN_POINT('Ctrl Pts',(-17.2536320179894,12.6234424170359,
131.50146332499)) ;
#135901=CARTESIAN_POINT('Ctrl Pts',(-17.1832036195686,12.8484690314232,
131.32893954711)) ;
#135902=CARTESIAN_POINT('Ctrl Pts',(-17.1344653483001,13.1134860607375,
131.219613229379)) ;
#135903=CARTESIAN_POINT('Ctrl Pts',(-17.1097906021278,13.402425050447,131.180795951585)) ;
#135904=CARTESIAN_POINT('Ctrl Pts',(-17.1104146704051,13.6901681944769,
131.215561704661)) ;
#135905=CARTESIAN_POINT('Ctrl Pts',(-17.1355551568111,13.9614083380647,
131.322263958797)) ;
#135906=CARTESIAN_POINT('Ctrl Pts',(-17.1825349214449,14.1924050674132,
131.492558721692)) ;
#135907=CARTESIAN_POINT('Ctrl Pts',(-17.247284144374,14.3688010159201,131.714792207733)) ;
#135908=CARTESIAN_POINT('Ctrl Pts',(-17.3247083783915,14.4776662097744,
131.974131076165)) ;
#135909=CARTESIAN_POINT('Ctrl Pts',(-17.4080456851403,14.5108828480259,
132.250624200494)) ;
#135910=CARTESIAN_POINT('Ctrl Pts',(-17.4912091781135,14.4662997711349,
132.526737050679)) ;
#135911=CARTESIAN_POINT('Ctrl Pts',(-17.5670722488366,14.3468724358185,
132.781476724685)) ;
#135912=CARTESIAN_POINT('Ctrl Pts',(-17.6295496572066,14.161614932188,132.997074962764)) ;
#135913=CARTESIAN_POINT('Ctrl Pts',(-17.6736158962945,13.9230022753498,
133.158962448849)) ;
#135914=CARTESIAN_POINT('Ctrl Pts',(-17.6951931588153,13.6485314062169,
133.25514650467)) ;
#135915=CARTESIAN_POINT('Ctrl Pts',(-17.6920615738823,13.3583011743042,
133.279105884718)) ;
#135916=CARTESIAN_POINT('Ctrl Pts',(-17.6637579865309,13.072504270402,133.229551323447)) ;
#135917=CARTESIAN_POINT('Ctrl Pts',(-17.6114584214845,12.8117566735177,
133.109923707737)) ;
#135918=CARTESIAN_POINT('Ctrl Pts',(-17.5386760935971,12.5955171582893,
132.930311398659)) ;
#135919=CARTESIAN_POINT('Ctrl Pts',(-17.4485485923782,12.4369580568928,
132.700390646819)) ;
#135920=CARTESIAN_POINT('Ctrl Pts',(-17.3489049682672,12.3507869630092,
132.442246375848)) ;
#135921=CARTESIAN_POINT('Ctrl Pts',(-17.2444930320388,12.3404899643528,
132.170365644373)) ;
#135922=CARTESIAN_POINT('Ctrl Pts',(-17.1426216271441,12.4078494476239,
131.905884901552)) ;
#135923=CARTESIAN_POINT('Ctrl Pts',(-17.0495668256941,12.5483871977687,
131.667259067528)) ;
#135924=CARTESIAN_POINT('Ctrl Pts',(-16.971814498006,12.7513533086917,131.473242742698)) ;
#135925=CARTESIAN_POINT('Ctrl Pts',(-16.9139622836365,13.001941318222,131.337310415625)) ;
#135926=CARTESIAN_POINT('Ctrl Pts',(-16.8792750897038,13.2828868274063,
131.269082634896)) ;
#135927=CARTESIAN_POINT('Ctrl Pts',(-16.8695679518648,13.5743278631276,
131.273876133887)) ;
#135928=CARTESIAN_POINT('Ctrl Pts',(-16.8850187674673,13.8554587804339,
131.352236081223)) ;
#135929=CARTESIAN_POINT('Ctrl Pts',(-16.9233899892215,14.103739100914,131.497307260457)) ;
#135930=CARTESIAN_POINT('Ctrl Pts',(-16.9815525794946,14.3046990175591,
131.70035759611)) ;
#135931=CARTESIAN_POINT('Ctrl Pts',(-17.0547401043487,14.4424188711516,
131.947366060444)) ;
#135932=CARTESIAN_POINT('Ctrl Pts',(-17.1362824190426,14.5067209234145,
132.218584626412)) ;
#135933=CARTESIAN_POINT('Ctrl Pts',(-17.2205230150152,14.4936392684735,
132.497872334383)) ;
#135934=CARTESIAN_POINT('Ctrl Pts',(-17.2999675507863,14.404006740505,132.76301963)) ;
#135935=CARTESIAN_POINT('Ctrl Pts',(-17.3687938432936,14.2433942656814,
132.99730827925)) ;
#135936=CARTESIAN_POINT('Ctrl Pts',(-17.4206621252372,14.0252993056693,
133.181832423558)) ;
#135937=CARTESIAN_POINT('Ctrl Pts',(-17.4518062177166,13.7626963119846,
133.306025850587)) ;
#135938=CARTESIAN_POINT('Ctrl Pts',(-17.4588018749284,13.4766513624265,
133.3595520989)) ;
#135939=CARTESIAN_POINT('Ctrl Pts',(-17.4407196010973,13.1866966293381,
133.339828540076)) ;
#135940=CARTESIAN_POINT('Ctrl Pts',(-17.3976621744542,12.9123106961637,
133.247325290375)) ;
#135941=CARTESIAN_POINT('Ctrl Pts',(-17.3328316521718,12.6769408805555,
133.090898057899)) ;
#135942=CARTESIAN_POINT('Ctrl Pts',(-17.2494627622651,12.4935889535621,
132.880470073151)) ;
#135943=CARTESIAN_POINT('Ctrl Pts',(-17.152618226233,12.3766908568814,132.630777552473)) ;
#135944=CARTESIAN_POINT('Ctrl Pts',(-17.049231423334,12.3352383862452,132.361846606225)) ;
#135945=CARTESIAN_POINT('Ctrl Pts',(-16.9457336891591,12.3713736006973,
132.092556286143)) ;
#135946=CARTESIAN_POINT('Ctrl Pts',(-16.8484161060952,12.4827590293817,
131.841396897906)) ;
#135947=CARTESIAN_POINT('Ctrl Pts',(-16.7634777794498,12.6627224306716,
131.626558702344)) ;
#135948=CARTESIAN_POINT('Ctrl Pts',(-16.6972681323854,12.8955397849013,
131.466150815898)) ;
#135949=CARTESIAN_POINT('Ctrl Pts',(-16.652840547036,13.1663558963296,131.369445368094)) ;
#135950=CARTESIAN_POINT('Ctrl Pts',(-16.6328908225603,13.4563321062043,
131.344330530745)) ;
#135951=CARTESIAN_POINT('Ctrl Pts',(-16.6382111416064,13.74354179735,131.392991362756)) ;
#135952=CARTESIAN_POINT('Ctrl Pts',(-16.6676592322395,14.007863745204,131.512146621969)) ;
#135953=CARTESIAN_POINT('Ctrl Pts',(-16.7182928746253,14.2299792391956,
131.693135937676)) ;
#135954=CARTESIAN_POINT('Ctrl Pts',(-16.7859878307255,14.3948659481182,
131.924049786769)) ;
#135955=CARTESIAN_POINT('Ctrl Pts',(-16.8651153132331,14.4898740802148,
132.188374983265)) ;
#135956=CARTESIAN_POINT('Ctrl Pts',(-16.9488778829896,14.5084149248409,
132.466110688147)) ;
#135957=CARTESIAN_POINT('Ctrl Pts',(-17.0311885247318,14.4492459338564,
132.739733964955)) ;
#135958=CARTESIAN_POINT('Ctrl Pts',(-17.104950151554,14.316609488643,132.988318108268)) ;
#135959=CARTESIAN_POINT('Ctrl Pts',(-17.1643724443007,14.1198900556279,
133.195042593654)) ;
#135960=CARTESIAN_POINT('Ctrl Pts',(-17.2043618345605,13.8734079349303,
133.344971495627)) ;
#135961=CARTESIAN_POINT('Ctrl Pts',(-17.2214102827416,13.5947694158123,
133.42787905469)) ;
#135962=CARTESIAN_POINT('Ctrl Pts',(-17.2135302438731,13.3033325180628,
133.438020470237)) ;
#135963=CARTESIAN_POINT('Ctrl Pts',(-17.1805025277542,13.0207084742087,
133.374676701685)) ;
#135964=CARTESIAN_POINT('Ctrl Pts',(-17.124234300538,12.767628690545,133.243341451459)) ;
#135965=CARTESIAN_POINT('Ctrl Pts',(-17.0476257592213,12.5604751539345,
133.052712263167)) ;
#135966=CARTESIAN_POINT('Ctrl Pts',(-16.9553890051503,12.4152916729436,
132.816483612565)) ;
#135967=CARTESIAN_POINT('Ctrl Pts',(-16.8542709676215,12.3428120631862,
132.554100291461)) ;
#135968=CARTESIAN_POINT('Ctrl Pts',(-16.7494730831066,12.3473797413046,
132.281194465277)) ;
#135969=CARTESIAN_POINT('Ctrl Pts',(-16.6487943422117,12.4294695368143,
132.020223589768)) ;
#135970=CARTESIAN_POINT('Ctrl Pts',(-16.5588158738871,12.5816148375682,
131.790339248201)) ;
#135971=CARTESIAN_POINT('Ctrl Pts',(-16.4842129576639,12.7949907280796,
131.605591372129)) ;
#135972=CARTESIAN_POINT('Ctrl Pts',(-16.4302842435271,13.054101177031,131.481287531456)) ;
#135973=CARTESIAN_POINT('Ctrl Pts',(-16.4003618883851,13.3386274126212,
131.426981031138)) ;
#135974=CARTESIAN_POINT('Ctrl Pts',(-16.3954982522069,13.6281884734652,
131.445764473398)) ;
#135975=CARTESIAN_POINT('Ctrl Pts',(-16.4153244875857,13.9042249218154,
131.536802751734)) ;
#135976=CARTESIAN_POINT('Ctrl Pts',(-16.4579192874622,14.1463903457502,
131.694429834647)) ;
#135977=CARTESIAN_POINT('Ctrl Pts',(-16.519604946235,14.3364819716926,131.907871784003)) ;
#135978=CARTESIAN_POINT('Ctrl Pts',(-16.5941877045133,14.4598817702337,
132.158628290576)) ;
#135979=CARTESIAN_POINT('Ctrl Pts',(-16.6772180078865,14.5104486170863,
132.434425087988)) ;
#135980=CARTESIAN_POINT('Ctrl Pts',(-16.7610712369098,14.4822486369166,
132.712559593312)) ;
#135981=CARTESIAN_POINT('Ctrl Pts',(-16.8386672352436,14.3791733041028,
132.97219580738)) ;
#135982=CARTESIAN_POINT('Ctrl Pts',(-16.9049174530084,14.2063740303146,
133.199006100538)) ;
#135983=CARTESIAN_POINT('Ctrl Pts',(-16.9532362150924,13.9777765864427,
133.373293310572)) ;
#135984=CARTESIAN_POINT('Ctrl Pts',(-16.9798528341138,13.7109259499415,
133.484028399788)) ;
#135985=CARTESIAN_POINT('Ctrl Pts',(-16.9822174695309,13.4211174151953,
133.524197897855)) ;
#135986=CARTESIAN_POINT('Ctrl Pts',(-16.9593603734184,13.1336909339448,
133.490426214311)) ;
#135987=CARTESIAN_POINT('Ctrl Pts',(-16.9122699848515,12.8658812639418,
133.385975367206)) ;
#135988=CARTESIAN_POINT('Ctrl Pts',(-16.8429275372481,12.6367690190525,
133.216731683706)) ;
#135989=CARTESIAN_POINT('Ctrl Pts',(-16.7566414738858,12.4658337897599,
132.997733929609)) ;
#135990=CARTESIAN_POINT('Ctrl Pts',(-16.6584445847538,12.3631245211514,
132.743942914283)) ;
#135991=CARTESIAN_POINT('Ctrl Pts',(-16.5545911413088,12.3360466241608,
132.473621289443)) ;
#135992=CARTESIAN_POINT('Ctrl Pts',(-16.4514231221753,12.3868688002356,
132.205414356226)) ;
#135993=CARTESIAN_POINT('Ctrl Pts',(-16.3561369237034,12.5119418325269,
131.960173693308)) ;
#135994=CARTESIAN_POINT('Ctrl Pts',(-16.2746048987367,12.7021783709845,
131.755117298832)) ;
#135995=CARTESIAN_POINT('Ctrl Pts',(-16.2118058427217,12.9449353770794,
131.604890369302)) ;
#135996=CARTESIAN_POINT('Ctrl Pts',(-16.1719673653937,13.2214383784226,
131.521650682401)) ;
#135997=CARTESIAN_POINT('Ctrl Pts',(-16.1568634879724,13.5108147708277,
131.510491075186)) ;
#135998=CARTESIAN_POINT('Ctrl Pts',(-16.1669300007681,13.7968084175674,
131.573203022695)) ;
#135999=CARTESIAN_POINT('Ctrl Pts',(-16.2006569741179,14.0536576083437,
131.704754764011)) ;
#136000=CARTESIAN_POINT('Ctrl Pts',(-16.254784608073,14.2659120564335,131.895928413579)) ;
#136001=CARTESIAN_POINT('Ctrl Pts',(-16.3251935914364,14.4185012516542,
132.134813692496)) ;
#136002=CARTESIAN_POINT('Ctrl Pts',(-16.4055493007845,14.4992712221482,
132.402638758212)) ;
#136003=CARTESIAN_POINT('Ctrl Pts',(-16.4897480826034,14.5031360116066,
132.681750239267)) ;
#136004=CARTESIAN_POINT('Ctrl Pts',(-16.5707620204115,14.4296202074177,
132.951505237183)) ;
#136005=CARTESIAN_POINT('Ctrl Pts',(-16.6421991335516,14.2844131247839,
133.193261917155)) ;
#136006=CARTESIAN_POINT('Ctrl Pts',(-16.6984700341114,14.0764755685082,
133.390876378768)) ;
#136007=CARTESIAN_POINT('Ctrl Pts',(-16.7342912161991,13.8227947339683,
133.528581938243)) ;
#136008=CARTESIAN_POINT('Ctrl Pts',(-16.7467556388197,13.5398702989391,
133.59814585037)) ;
#136009=CARTESIAN_POINT('Ctrl Pts',(-16.7340724183047,13.2487717783427,
133.594219576124)) ;
#136010=CARTESIAN_POINT('Ctrl Pts',(-16.6965212883533,12.9703362151756,
133.517627433161)) ;
#136011=CARTESIAN_POINT('Ctrl Pts',(-16.6359937287517,12.7241092781338,
133.373940651091)) ;
#136012=CARTESIAN_POINT('Ctrl Pts',(-16.5560795871543,12.5279171433205,
133.173632261453)) ;
#136013=CARTESIAN_POINT('Ctrl Pts',(-16.4618411443677,12.3959938665945,
132.931466168076)) ;
#136014=CARTESIAN_POINT('Ctrl Pts',(-16.3593827732272,12.3376260980812,
132.665255360874)) ;
#136015=CARTESIAN_POINT('Ctrl Pts',(-16.2550385035652,12.3570497794023,
132.393594158916)) ;
#136016=CARTESIAN_POINT('Ctrl Pts',(-16.1560569930776,12.4525559733436,
132.137489642659)) ;
#136017=CARTESIAN_POINT('Ctrl Pts',(-16.0682112092327,12.6176036105847,
131.9139932347)) ;
#136018=CARTESIAN_POINT('Ctrl Pts',(-15.9972052369213,12.8410947019102,
131.739774174027)) ;
#136019=CARTESIAN_POINT('Ctrl Pts',(-15.9477710009751,13.1055203518464,
131.628457545108)) ;
#136020=CARTESIAN_POINT('Ctrl Pts',(-15.9223966595682,13.3928980327512,
131.587457525944)) ;
#136021=CARTESIAN_POINT('Ctrl Pts',(-15.9222756880834,13.6824543649216,
131.620230232659)) ;
#136022=CARTESIAN_POINT('Ctrl Pts',(-15.9466295677973,13.9532692757644,
131.724475741057)) ;
#136023=CARTESIAN_POINT('Ctrl Pts',(-15.9930649492766,14.1862511235797,
131.893256545959)) ;
#136024=CARTESIAN_POINT('Ctrl Pts',(-16.0572774469947,14.3643962082537,
132.113884233036)) ;
#136025=CARTESIAN_POINT('Ctrl Pts',(-16.1348869305229,14.4759024807437,
132.373959659061)) ;
#136026=CARTESIAN_POINT('Ctrl Pts',(-16.2178601983213,14.5109062464403,
132.649271579231)) ;
#136027=CARTESIAN_POINT('Ctrl Pts',(-16.3010573982548,14.4687351628052,
132.925452283273)) ;
#136028=CARTESIAN_POINT('Ctrl Pts',(-16.3772524895357,14.351243796897,133.18118301111)) ;
#136029=CARTESIAN_POINT('Ctrl Pts',(-16.4401554780105,14.1681343550178,
133.397975738382)) ;
#136030=CARTESIAN_POINT('Ctrl Pts',(-16.4850310227968,13.9291093552066,
133.562448350169)) ;
#136031=CARTESIAN_POINT('Ctrl Pts',(-16.5070926720565,13.6572015399983,
133.659816803159)) ;
#136032=CARTESIAN_POINT('Ctrl Pts',(-16.5046943032788,13.3659146668707,
133.686064790888)) ;
#136033=CARTESIAN_POINT('Ctrl Pts',(-16.4771547092974,13.0809591455927,
133.638599282157)) ;
#136034=CARTESIAN_POINT('Ctrl Pts',(-16.4256137570119,12.8188859308948,
133.521201214271)) ;
#136035=CARTESIAN_POINT('Ctrl Pts',(-16.3527339561376,12.5999510440463,
133.341543109138)) ;
#136036=CARTESIAN_POINT('Ctrl Pts',(-16.2641281336111,12.4414984825018,
133.115647334815)) ;
#136037=CARTESIAN_POINT('Ctrl Pts',(-16.1641430091743,12.3520343108791,
132.85671610708)) ;
#136038=CARTESIAN_POINT('Ctrl Pts',(-16.0594698293865,12.3398054622105,
132.584157469235)) ;
#136039=CARTESIAN_POINT('Ctrl Pts',(-15.9577980199829,12.4047865271677,
132.320144279598)) ;
#136040=CARTESIAN_POINT('Ctrl Pts',(-15.8643756324851,12.5431933869583,
132.080444267518)) ;
#136041=CARTESIAN_POINT('Ctrl Pts',(-15.7860699178347,12.7444965603529,
131.884816381687)) ;
#136042=CARTESIAN_POINT('Ctrl Pts',(-15.7274833077799,12.9945025224571,
131.746812479205)) ;
#136043=CARTESIAN_POINT('Ctrl Pts',(-15.6921182047523,13.2745329094811,
131.676561655677)) ;
#136044=CARTESIAN_POINT('Ctrl Pts',(-15.6817523163213,13.5670626370277,
131.679561862218)) ;
#136045=CARTESIAN_POINT('Ctrl Pts',(-15.6963153264075,13.8462370772247,
131.755016293096)) ;
#136046=CARTESIAN_POINT('Ctrl Pts',(-15.7342967830937,14.0979241250953,
131.899230741437)) ;
#136047=CARTESIAN_POINT('Ctrl Pts',(-15.7919436686276,14.2997383418867,
132.100703473067)) ;
#136048=CARTESIAN_POINT('Ctrl Pts',(-15.8645031781154,14.4393312193764,
132.345773094754)) ;
#136049=CARTESIAN_POINT('Ctrl Pts',(-15.9465184391645,14.5060643569228,
132.618629039297)) ;
#136050=CARTESIAN_POINT('Ctrl Pts',(-16.0301677623958,14.4951758782706,
132.895935895831)) ;
#136051=CARTESIAN_POINT('Ctrl Pts',(-16.1102104627669,14.4072623281432,
133.163000755797)) ;
#136052=CARTESIAN_POINT('Ctrl Pts',(-16.1790779676799,14.2495039694875,
133.397213921694)) ;
#136053=CARTESIAN_POINT('Ctrl Pts',(-16.2319003919638,14.0308221258824,
133.584830620202)) ;
#136054=CARTESIAN_POINT('Ctrl Pts',(-16.2633270017823,13.7719100664948,
133.709489495124)) ;
#136055=CARTESIAN_POINT('Ctrl Pts',(-16.2711876727272,13.4847456450531,
133.765738112161)) ;
#136056=CARTESIAN_POINT('Ctrl Pts',(-16.253847194686,13.1955425031336,133.748069200693)) ;
#136057=CARTESIAN_POINT('Ctrl Pts',(-16.2115198754741,12.9200552968874,
133.65773228028)) ;
#136058=CARTESIAN_POINT('Ctrl Pts',(-16.147222084084,12.6831184385928,133.502892140705)) ;
#136059=CARTESIAN_POINT('Ctrl Pts',(-16.064282599147,12.4980281206389,133.293729089209)) ;
#136060=CARTESIAN_POINT('Ctrl Pts',(-15.9679392810076,12.3791543430107,
133.045434009803)) ;
#136061=CARTESIAN_POINT('Ctrl Pts',(-15.8643595558364,12.3353503717386,
132.776040083288)) ;
#136062=CARTESIAN_POINT('Ctrl Pts',(-15.7608810145636,12.3691099621928,
132.506761731086)) ;
#136063=CARTESIAN_POINT('Ctrl Pts',(-15.6627255542582,12.4795856785055,
132.253375320536)) ;
#136064=CARTESIAN_POINT('Ctrl Pts',(-15.5784730291827,12.6553361009926,
132.040088792181)) ;
#136065=CARTESIAN_POINT('Ctrl Pts',(-15.5110293575352,12.8882259217544,
131.876334600156)) ;
#136066=CARTESIAN_POINT('Ctrl Pts',(-15.4660114239873,13.1581921393272,
131.777882402057)) ;
#136067=CARTESIAN_POINT('Ctrl Pts',(-15.4453153424862,13.4482190387101,
131.750625899504)) ;
#136068=CARTESIAN_POINT('Ctrl Pts',(-15.4499239120655,13.7352663202425,
131.797145410483)) ;
#136069=CARTESIAN_POINT('Ctrl Pts',(-15.4786708796544,14.0004787425337,
131.914245491789)) ;
#136070=CARTESIAN_POINT('Ctrl Pts',(-15.528718936817,14.2242401467777,132.093531049238)) ;
#136071=CARTESIAN_POINT('Ctrl Pts',(-15.5963327554751,14.391486003047,132.324353743837)) ;
#136072=CARTESIAN_POINT('Ctrl Pts',(-15.6747831211035,14.4880341837757,
132.586510244365)) ;
#136073=CARTESIAN_POINT('Ctrl Pts',(-15.7588156763009,14.5089767222778,
132.865167334381)) ;
#136074=CARTESIAN_POINT('Ctrl Pts',(-15.8410228376495,14.4520807364783,
133.138385805997)) ;
#136075=CARTESIAN_POINT('Ctrl Pts',(-15.9152233944989,14.3213934969356,
133.388297276998)) ;
#136076=CARTESIAN_POINT('Ctrl Pts',(-15.9751021978438,14.126427628205,133.596336490836)) ;
#136077=CARTESIAN_POINT('Ctrl Pts',(-16.0157883783172,13.8807880817665,
133.748352793927)) ;
#136078=CARTESIAN_POINT('Ctrl Pts',(-16.0334719367804,13.6022566506269,
133.833171646611)) ;
#136079=CARTESIAN_POINT('Ctrl Pts',(-16.0263427101219,13.3123739575692,
133.845337187169)) ;
#136080=CARTESIAN_POINT('Ctrl Pts',(-15.9941097511416,13.0290004002489,
133.784332603085)) ;
#136081=CARTESIAN_POINT('Ctrl Pts',(-15.9383247563886,12.7741270713226,
133.65449670321)) ;
#136082=CARTESIAN_POINT('Ctrl Pts',(-15.8622768484471,12.5657352250487,
133.465472847607)) ;
#136083=CARTESIAN_POINT('Ctrl Pts',(-15.7707760397584,12.4188762117679,
133.231275457079)) ;
#136084=CARTESIAN_POINT('Ctrl Pts',(-15.6694610724198,12.3438128452305,
132.968446766761)) ;
#136085=CARTESIAN_POINT('Ctrl Pts',(-15.5650490222749,12.3461025205116,
132.696542230689)) ;
#136086=CARTESIAN_POINT('Ctrl Pts',(-15.4641117267899,12.4255735874937,
132.43482095437)) ;
#136087=CARTESIAN_POINT('Ctrl Pts',(-15.3733010936375,12.5765456735502,
132.202668192957)) ;
#136088=CARTESIAN_POINT('Ctrl Pts',(-15.2984189865204,12.7879286592572,
132.017014437685)) ;
#136089=CARTESIAN_POINT('Ctrl Pts',(-15.243943520018,13.0448054046113,131.89098628761)) ;
#136090=CARTESIAN_POINT('Ctrl Pts',(-15.2130872375626,13.329756321322,131.834065836623)) ;
#136091=CARTESIAN_POINT('Ctrl Pts',(-15.207498078425,13.6201107178654,131.850804210703)) ;
#136092=CARTESIAN_POINT('Ctrl Pts',(-15.226664565684,13.8967554382586,131.93990903969)) ;
#136093=CARTESIAN_POINT('Ctrl Pts',(-15.2685096670752,14.1394983367384,
132.095250212473)) ;
#136094=CARTESIAN_POINT('Ctrl Pts',(-15.3296325471033,14.3315001569242,
132.307040763849)) ;
#136095=CARTESIAN_POINT('Ctrl Pts',(-15.4041948784221,14.4575222943013,
132.557868425866)) ;
#136096=CARTESIAN_POINT('Ctrl Pts',(-15.4871845489021,14.5099977938908,
132.833577267545)) ;
#136097=CARTESIAN_POINT('Ctrl Pts',(-15.5706474715052,14.4843800867397,
133.110384973781)) ;
#136098=CARTESIAN_POINT('Ctrl Pts',(-15.6489358172198,14.3828781461486,
133.372231534079)) ;
#136099=CARTESIAN_POINT('Ctrl Pts',(-15.7152215321923,14.212816168216,133.598953578525)) ;
#136100=CARTESIAN_POINT('Ctrl Pts',(-15.7643324415315,13.9854781681749,
133.775621838138)) ;
#136101=CARTESIAN_POINT('Ctrl Pts',(-15.7916807767753,13.7179644909653,
133.888670251454)) ;
#136102=CARTESIAN_POINT('Ctrl Pts',(-15.7946921387686,13.4301920376034,
133.930530607513)) ;
#136103=CARTESIAN_POINT('Ctrl Pts',(-15.7726967990617,13.1421055633853,
133.899307008492)) ;
#136104=CARTESIAN_POINT('Ctrl Pts',(-15.725756949418,12.87150128464,133.795559990037)) ;
#136105=CARTESIAN_POINT('Ctrl Pts',(-15.6577073073503,12.6436097991943,
133.629723531333)) ;
#136106=CARTESIAN_POINT('Ctrl Pts',(-15.5716152896333,12.4698498437503,
133.411423269474)) ;
#136107=CARTESIAN_POINT('Ctrl Pts',(-15.4736825799438,12.3651221856613,
133.158394352247)) ;
#136108=CARTESIAN_POINT('Ctrl Pts',(-15.3697907387214,12.335692224637,132.887997751447)) ;
#136109=CARTESIAN_POINT('Ctrl Pts',(-15.2664401785828,12.3844432071478,
132.619277578795)) ;
#136110=CARTESIAN_POINT('Ctrl Pts',(-15.1710399074463,12.5072147901112,
132.373635971455)) ;
#136111=CARTESIAN_POINT('Ctrl Pts',(-15.0889535850671,12.6957550150873,
132.166979770339)) ;
#136112=CARTESIAN_POINT('Ctrl Pts',(-15.0255721551039,12.9372999479051,
132.01505517321)) ;
#136113=CARTESIAN_POINT('Ctrl Pts',(-14.9850575690906,13.2121499543988,
131.929735608954)) ;
#136114=CARTESIAN_POINT('Ctrl Pts',(-14.9691714974783,13.5032465104466,
131.91650779929)) ;
#136115=CARTESIAN_POINT('Ctrl Pts',(-14.9783938577685,13.7871080328991,
131.976440567623)) ;
#136116=CARTESIAN_POINT('Ctrl Pts',(-15.0115648784408,14.0469104745439,
132.106594492085)) ;
#136117=CARTESIAN_POINT('Ctrl Pts',(-15.0651801887707,14.2605649124229,
132.296255586953)) ;
#136118=CARTESIAN_POINT('Ctrl Pts',(-15.1354050179275,14.4153649488043,
132.534693807358)) ;
#136119=CARTESIAN_POINT('Ctrl Pts',(-15.2152370606947,14.4978582783663,
132.800850624746)) ;
#136120=CARTESIAN_POINT('Ctrl Pts',(-15.2994258322498,14.5041773990225,
133.079939121836)) ;
#136121=CARTESIAN_POINT('Ctrl Pts',(-15.3806609287712,14.4329779197685,
133.350346880059)) ;
#136122=CARTESIAN_POINT('Ctrl Pts',(-15.4527495072584,14.2890422314917,
133.594146581102)) ;
#136123=CARTESIAN_POINT('Ctrl Pts',(-15.5093788401438,14.082779433517,133.79275764401)) ;
#136124=CARTESIAN_POINT('Ctrl Pts',(-15.545753191267,13.8309337098099,133.931989144067)) ;
#136125=CARTESIAN_POINT('Ctrl Pts',(-15.5589571408963,13.5483120187831,
134.003745938923)) ;
#136126=CARTESIAN_POINT('Ctrl Pts',(-15.5470459162325,13.2574777531019,
134.002035659956)) ;
#136127=CARTESIAN_POINT('Ctrl Pts',(-15.510131605999,12.9779697529959,133.92735890912)) ;
#136128=CARTESIAN_POINT('Ctrl Pts',(-15.4504417667573,12.7311580251373,
133.786020643798)) ;
#136129=CARTESIAN_POINT('Ctrl Pts',(-15.3706607271275,12.5323980592304,
133.586256423076)) ;
#136130=CARTESIAN_POINT('Ctrl Pts',(-15.2770803375685,12.3989897288854,
133.345890363007)) ;
#136131=CARTESIAN_POINT('Ctrl Pts',(-15.1745710010167,12.3382487603058,
133.079602207309)) ;
#136132=CARTESIAN_POINT('Ctrl Pts',(-15.0705359722807,12.3552058083452,
132.808726876001)) ;
#136133=CARTESIAN_POINT('Ctrl Pts',(-14.9706606470321,12.4490680703867,
132.550225448555)) ;
#136134=CARTESIAN_POINT('Ctrl Pts',(-14.8824522342596,12.612854304799,132.325691498574)) ;
#136135=CARTESIAN_POINT('Ctrl Pts',(-14.8113527265263,12.8333918295054,
132.150980279395)) ;
#136136=CARTESIAN_POINT('Ctrl Pts',(-14.7610563805274,13.0975419155814,
132.037242671929)) ;
#136137=CARTESIAN_POINT('Ctrl Pts',(-14.7349932181902,13.3843701567211,
131.99420597981)) ;
#136138=CARTESIAN_POINT('Ctrl Pts',(-14.7341460984049,13.6749248626015,
132.024944556395)) ;
#136139=CARTESIAN_POINT('Ctrl Pts',(-14.7579228982456,13.9463602578246,
132.127499501483)) ;
#136140=CARTESIAN_POINT('Ctrl Pts',(-14.8035289837161,14.1798324379302,
132.293714438332)) ;
#136141=CARTESIAN_POINT('Ctrl Pts',(-14.8677079251816,14.3606302769089,
132.514446261517)) ;
#136142=CARTESIAN_POINT('Ctrl Pts',(-14.9443462637881,14.4733618864566,
132.771384751192)) ;
#136143=CARTESIAN_POINT('Ctrl Pts',(-15.0280034573494,14.5110756600993,
133.049012799316)) ;
#136144=CARTESIAN_POINT('Ctrl Pts',(-15.1108313580727,14.4709889009811,
133.323927299789)) ;
#136145=CARTESIAN_POINT('Ctrl Pts',(-15.1874906865422,14.3556941984043,
133.581070483478)) ;
#136146=CARTESIAN_POINT('Ctrl Pts',(-15.2510153385486,14.1731666486328,
133.79982111375)) ;
#136147=CARTESIAN_POINT('Ctrl Pts',(-15.2960503606692,13.9378584167298,
133.964426013949)) ;
#136148=CARTESIAN_POINT('Ctrl Pts',(-15.3190310826371,13.6656355311939,
134.064636189014)) ;
#136149=CARTESIAN_POINT('Ctrl Pts',(-15.3173445451022,13.3744563081115,
134.092966610367)) ;
#136150=CARTESIAN_POINT('Ctrl Pts',(-15.2904580609234,13.0885611803192,
134.047472889722)) ;
#136151=CARTESIAN_POINT('Ctrl Pts',(-15.2396747814133,12.8263306498725,
133.932194970172)) ;
#136152=CARTESIAN_POINT('Ctrl Pts',(-15.1677163389787,12.6063807769631,
133.755109558956)) ;
#136153=CARTESIAN_POINT('Ctrl Pts',(-15.0788943634793,12.4447492933123,
133.528822932428)) ;
#136154=CARTESIAN_POINT('Ctrl Pts',(-14.9791253222199,12.3535025882306,
133.270511156007)) ;
#136155=CARTESIAN_POINT('Ctrl Pts',(-14.8746674650902,12.3391045054194,
132.998527191728)) ;
#136156=CARTESIAN_POINT('Ctrl Pts',(-14.7728141849366,12.4018104241151,
132.733985657383)) ;
#136157=CARTESIAN_POINT('Ctrl Pts',(-14.6787517401919,12.5389586489687,
132.49253663729)) ;
#136158=CARTESIAN_POINT('Ctrl Pts',(-14.6003862698118,12.7377764458565,
132.296567507347)) ;
#136159=CARTESIAN_POINT('Ctrl Pts',(-14.5411439660413,12.9863019722805,
132.156626084833)) ;
#136160=CARTESIAN_POINT('Ctrl Pts',(-14.5050286674343,13.2660338630659,
132.084222246459)) ;
#136161=CARTESIAN_POINT('Ctrl Pts',(-14.4938897468974,13.5582232268191,
132.08492344046)) ;
#136162=CARTESIAN_POINT('Ctrl Pts',(-14.507818431321,13.8387404070693,132.158622706454)) ;
#136163=CARTESIAN_POINT('Ctrl Pts',(-14.5449327754259,14.0904925183414,
132.300141702221)) ;
#136164=CARTESIAN_POINT('Ctrl Pts',(-14.6025167026814,14.2955136011611,
132.501693163721)) ;
#136165=CARTESIAN_POINT('Ctrl Pts',(-14.6743979140284,14.4360006812449,
132.744601960421)) ;
#136166=CARTESIAN_POINT('Ctrl Pts',(-14.7560190059001,14.5051702931602,
133.016232266989)) ;
#136167=CARTESIAN_POINT('Ctrl Pts',(-14.8399788108669,14.4966323764384,
133.29455720462)) ;
#136168=CARTESIAN_POINT('Ctrl Pts',(-14.92026343514,14.4108291399258,133.562335509995)) ;
#136169=CARTESIAN_POINT('Ctrl Pts',(-14.9895377292265,14.2547209501546,
133.797763255438)) ;
#136170=CARTESIAN_POINT('Ctrl Pts',(-15.0426869064103,14.0388606089928,
133.986156454842)) ;
#136171=CARTESIAN_POINT('Ctrl Pts',(-15.0750262925721,13.779405578044,134.113692915164)) ;
#136172=CARTESIAN_POINT('Ctrl Pts',(-15.0835065338818,13.4926641580088,
134.171741504609)) ;
#136173=CARTESIAN_POINT('Ctrl Pts',(-15.0668941196817,13.2038302112353,
134.156144137311)) ;
#136174=CARTESIAN_POINT('Ctrl Pts',(-15.0254043328273,12.9280759931688,
134.068184900734)) ;
#136175=CARTESIAN_POINT('Ctrl Pts',(-14.9614251335503,12.6887447492448,
133.914424357805)) ;
#136176=CARTESIAN_POINT('Ctrl Pts',(-14.8789170489459,12.5022966343227,
133.706505074034)) ;
#136177=CARTESIAN_POINT('Ctrl Pts',(-14.7832955283864,12.381763978882,133.460180040676)) ;
#136178=CARTESIAN_POINT('Ctrl Pts',(-14.6794737714671,12.3354318114705,
133.190193795545)) ;
#136179=CARTESIAN_POINT('Ctrl Pts',(-14.5760954726489,12.3672035513488,
132.921157086038)) ;
#136180=CARTESIAN_POINT('Ctrl Pts',(-14.4781651153176,12.474426481286,132.668233520948)) ;
#136181=CARTESIAN_POINT('Ctrl Pts',(-14.3924892268079,12.6503068829769,
132.451164645272)) ;
#136182=CARTESIAN_POINT('Ctrl Pts',(-14.3248849840194,12.8812481424524,
132.28680518042)) ;
#136183=CARTESIAN_POINT('Ctrl Pts',(-14.2792429233544,13.1494231082653,
132.186430077652)) ;
#136184=CARTESIAN_POINT('Ctrl Pts',(-14.2577333010081,13.4405328283774,
132.156949660664)) ;
#136185=CARTESIAN_POINT('Ctrl Pts',(-14.2616812486159,13.7272524095848,
132.201463654968)) ;
#136186=CARTESIAN_POINT('Ctrl Pts',(-14.2897398061011,13.9933197786215,
132.316545259697)) ;
#136187=CARTESIAN_POINT('Ctrl Pts',(-14.3391869583318,14.2183989061991,
132.494053529779)) ;
#136188=CARTESIAN_POINT('Ctrl Pts',(-14.4064273444875,14.3876287517767,
132.723811096672)) ;
#136189=CARTESIAN_POINT('Ctrl Pts',(-14.4845242454382,14.4861870970875,
132.984890006035)) ;
#136190=CARTESIAN_POINT('Ctrl Pts',(-14.5685621236943,14.5095212297327,
133.263587921165)) ;
#136191=CARTESIAN_POINT('Ctrl Pts',(-14.6509971062007,14.4547287275128,
133.537507814222)) ;
#136192=CARTESIAN_POINT('Ctrl Pts',(-14.7254748058222,14.3261105544631,
133.788208742009)) ;
#136193=CARTESIAN_POINT('Ctrl Pts',(-14.7858563786915,14.1327425032557,
133.997729271496)) ;
#136194=CARTESIAN_POINT('Ctrl Pts',(-14.8271232484926,13.8885306001009,
134.151412460096)) ;
#136195=CARTESIAN_POINT('Ctrl Pts',(-14.8454990345243,13.6107524410049,
134.23824836838)) ;
#136196=CARTESIAN_POINT('Ctrl Pts',(-14.8391902936134,13.3210542583331,
134.252793238962)) ;
#136197=CARTESIAN_POINT('Ctrl Pts',(-14.8073003870615,13.0351251235983,
134.193044709195)) ;
#136198=CARTESIAN_POINT('Ctrl Pts',(-14.7526013452373,12.7816150209491,
134.066072694138)) ;
#136199=CARTESIAN_POINT('Ctrl Pts',(-14.6768446022253,12.5706518061014,
133.878035031889)) ;
#136200=CARTESIAN_POINT('Ctrl Pts',(-14.5857344899984,12.422091900903,133.644955346922)) ;
#136201=CARTESIAN_POINT('Ctrl Pts',(-14.4844870236026,12.3448083833829,
133.382365111388)) ;
#136202=CARTESIAN_POINT('Ctrl Pts',(-14.3801271179856,12.3450375607664,
133.110594842367)) ;
#136203=CARTESIAN_POINT('Ctrl Pts',(-14.2791586916205,12.4222140372622,
132.848729115977)) ;
#136204=CARTESIAN_POINT('Ctrl Pts',(-14.1879207671711,12.5713072693593,
132.615345977553)) ;
#136205=CARTESIAN_POINT('Ctrl Pts',(-14.1124789413141,12.7812068465324,
132.428068113172)) ;
#136206=CARTESIAN_POINT('Ctrl Pts',(-14.0572435650617,13.0378486801572,
132.299917089332)) ;
#136207=CARTESIAN_POINT('Ctrl Pts',(-14.0258214639467,13.3220972424203,
132.241311719484)) ;
#136208=CARTESIAN_POINT('Ctrl Pts',(-14.0195168117333,13.6116477161832,
132.255856984885)) ;
#136209=CARTESIAN_POINT('Ctrl Pts',(-14.0380429091883,13.8896343949454,
132.343170883447)) ;
#136210=CARTESIAN_POINT('Ctrl Pts',(-14.0792096341859,14.1329048293709,
132.496445041414)) ;
#136211=CARTESIAN_POINT('Ctrl Pts',(-14.139739650008,14.3266157424045,132.706473107546)) ;
#136212=CARTESIAN_POINT('Ctrl Pts',(-14.2142389199618,14.4550271923226,
132.957226742653)) ;
#136213=CARTESIAN_POINT('Ctrl Pts',(-14.2968257149156,14.5094869156272,
133.231648652557)) ;
#136214=CARTESIAN_POINT('Ctrl Pts',(-14.3803943332945,14.4863255111229,
133.508781433968)) ;
#136215=CARTESIAN_POINT('Ctrl Pts',(-14.4590295914748,14.3868080890416,
133.771682898577)) ;
#136216=CARTESIAN_POINT('Ctrl Pts',(-14.5257824357843,14.2186053771164,
133.999775534479)) ;
#136217=CARTESIAN_POINT('Ctrl Pts',(-14.5755477699378,13.9916146831158,
134.17848468615)) ;
#136218=CARTESIAN_POINT('Ctrl Pts',(-14.6033802697407,13.727139474133,134.292681268961)) ;
#136219=CARTESIAN_POINT('Ctrl Pts',(-14.6071598535866,13.437362164295,134.337061191346)) ;
#136220=CARTESIAN_POINT('Ctrl Pts',(-14.5858835306319,13.1504054531947,
134.307774902983)) ;
#136221=CARTESIAN_POINT('Ctrl Pts',(-14.5396141567361,12.8786465021209,
134.206021789804)) ;
#136222=CARTESIAN_POINT('Ctrl Pts',(-14.4723055377556,12.6500332814425,
134.042260729231)) ;
#136223=CARTESIAN_POINT('Ctrl Pts',(-14.386841995621,12.4743183897028,133.825754806519)) ;
#136224=CARTESIAN_POINT('Ctrl Pts',(-14.2885171909372,12.3668547922141,
133.571800387653)) ;
#136225=CARTESIAN_POINT('Ctrl Pts',(-14.1851936733311,12.335562941567,133.302903084124)) ;
#136226=CARTESIAN_POINT('Ctrl Pts',(-14.0817812802112,12.3817108072099,
133.033981832815)) ;
#136227=CARTESIAN_POINT('Ctrl Pts',(-13.9856777323266,12.502839824897,132.78641286331)) ;
#136228=CARTESIAN_POINT('Ctrl Pts',(-13.9030779122353,12.690351441453,132.578318888232)) ;
#136229=CARTESIAN_POINT('Ctrl Pts',(-13.8395678233593,12.9285059391321,
132.425739358382)) ;
#136230=CARTESIAN_POINT('Ctrl Pts',(-13.7979805061536,13.2046731907038,
132.337546584743)) ;
#136231=CARTESIAN_POINT('Ctrl Pts',(-13.7814999331058,13.4951333113011,
132.322515878226)) ;
#136232=CARTESIAN_POINT('Ctrl Pts',(-13.7900411291653,13.779501210584,132.380474347949)) ;
#136233=CARTESIAN_POINT('Ctrl Pts',(-13.8224120698119,14.0394108332529,
132.508163412887)) ;
#136234=CARTESIAN_POINT('Ctrl Pts',(-13.8756204987681,14.2552141196343,
132.696731438701)) ;
#136235=CARTESIAN_POINT('Ctrl Pts',(-13.9451061652378,14.4112842226695,
132.932851180889)) ;
#136236=CARTESIAN_POINT('Ctrl Pts',(-14.0249337755901,14.49663037618,133.199097915004)) ;
#136237=CARTESIAN_POINT('Ctrl Pts',(-14.1095239733355,14.5049768783044,
133.479521095915)) ;
#136238=CARTESIAN_POINT('Ctrl Pts',(-14.190528704622,14.4360835729073,133.749098498737)) ;
#136239=CARTESIAN_POINT('Ctrl Pts',(-14.262882528703,14.2946513922982,133.993611762097)) ;
#136240=CARTESIAN_POINT('Ctrl Pts',(-14.320142163076,14.0899140100411,134.194101738961)) ;
#136241=CARTESIAN_POINT('Ctrl Pts',(-14.3572698390389,13.8386917046902,
134.335604381356)) ;
#136242=CARTESIAN_POINT('Ctrl Pts',(-14.3711303129086,13.5555692125345,
134.40939671493)) ;
#136243=CARTESIAN_POINT('Ctrl Pts',(-14.3599713476779,13.2663901180779,
134.409692119641)) ;
#136244=CARTESIAN_POINT('Ctrl Pts',(-14.3238194723227,12.9858847333076,
134.337276500168)) ;
#136245=CARTESIAN_POINT('Ctrl Pts',(-14.2645948958419,12.7375102459871,
134.197360749458)) ;
#136246=CARTESIAN_POINT('Ctrl Pts',(-14.1856165305326,12.5376376287816,
133.99982702238)) ;
#136247=CARTESIAN_POINT('Ctrl Pts',(-14.0918860241884,12.4015826977934,
133.759196205742)) ;
#136248=CARTESIAN_POINT('Ctrl Pts',(-13.9900202965247,12.3390360902595,
133.494624163606)) ;
#136249=CARTESIAN_POINT('Ctrl Pts',(-13.885715431319,12.353575403094,133.223035536617)) ;
#136250=CARTESIAN_POINT('Ctrl Pts',(-13.7857334521546,12.445274073871,132.964183894283)) ;
#136251=CARTESIAN_POINT('Ctrl Pts',(-13.6971224342536,12.6067971683827,
132.738446959323)) ;
#136252=CARTESIAN_POINT('Ctrl Pts',(-13.6250522220287,12.8274892534517,
132.561122252927)) ;
#136253=CARTESIAN_POINT('Ctrl Pts',(-13.5744828714336,13.0891408927057,
132.446378055787)) ;
#136254=CARTESIAN_POINT('Ctrl Pts',(-13.547610803124,13.375740122579,132.401005590542)) ;
#136255=CARTESIAN_POINT('Ctrl Pts',(-13.5460300274622,13.6659116032671,
132.429533614848)) ;
#136256=CARTESIAN_POINT('Ctrl Pts',(-13.5689788396593,13.9383430672958,
132.529666742918)) ;
#136257=CARTESIAN_POINT('Ctrl Pts',(-13.6144336268274,14.1747318786697,
132.695698796106)) ;
#136258=CARTESIAN_POINT('Ctrl Pts',(-13.6775346028895,14.3556000224366,
132.912954043635)) ;
#136259=CARTESIAN_POINT('Ctrl Pts',(-13.7545609195232,14.4715471852787,
133.171333891809)) ;
#136260=CARTESIAN_POINT('Ctrl Pts',(-13.8375768659038,14.5109306884899,
133.446859569505)) ;
#136261=CARTESIAN_POINT('Ctrl Pts',(-13.9206587334674,14.4734197510009,
133.722575921601)) ;
#136262=CARTESIAN_POINT('Ctrl Pts',(-13.9978549774587,14.3595613312843,
133.981405064546)) ;
#136263=CARTESIAN_POINT('Ctrl Pts',(-14.0615326101247,14.179466171533,134.200463448237)) ;
#136264=CARTESIAN_POINT('Ctrl Pts',(-14.1072808462681,13.9455181185487,
134.367173049305)) ;
#136265=CARTESIAN_POINT('Ctrl Pts',(-14.1309695714097,13.6723045745694,
134.469654422256)) ;
#136266=CARTESIAN_POINT('Ctrl Pts',(-14.1299543421008,13.3834915874396,
134.49969517271)) ;
#136267=CARTESIAN_POINT('Ctrl Pts',(-14.103826459953,13.0966134068724,134.456484806691)) ;
#136268=CARTESIAN_POINT('Ctrl Pts',(-14.0536044519402,12.8330521051259,
134.342891801889)) ;
#136269=CARTESIAN_POINT('Ctrl Pts',(-13.9819755458689,12.6112324338377,
134.166849542491)) ;
#136270=CARTESIAN_POINT('Ctrl Pts',(-13.8936140788126,12.4482429025448,
133.941863276773)) ;
#136271=CARTESIAN_POINT('Ctrl Pts',(-13.7945442209898,12.3553252392396,
133.68544189025)) ;
#136272=CARTESIAN_POINT('Ctrl Pts',(-13.6902421881023,12.3382107107946,
133.413874998198)) ;
#136273=CARTESIAN_POINT('Ctrl Pts',(-13.5876395250276,12.3992481458877,
133.147344273434)) ;
#136274=CARTESIAN_POINT('Ctrl Pts',(-13.4940363967205,12.5331204758664,
132.906945186053)) ;
#136275=CARTESIAN_POINT('Ctrl Pts',(-13.4146406339235,12.7309387918669,
132.708143521826)) ;
#136276=CARTESIAN_POINT('Ctrl Pts',(-13.3546400489765,12.9791524410526,
132.566084041094)) ;
#136277=CARTESIAN_POINT('Ctrl Pts',(-13.3178749195276,13.2585790598106,
132.491812795079)) ;
#136278=CARTESIAN_POINT('Ctrl Pts',(-13.3060921658157,13.5499397896395,
132.490544550928)) ;
#136279=CARTESIAN_POINT('Ctrl Pts',(-13.319267039209,13.8311712407388,132.562048975874)) ;
#136280=CARTESIAN_POINT('Ctrl Pts',(-13.3560394645477,14.0848085651835,
132.702709571436)) ;
#136281=CARTESIAN_POINT('Ctrl Pts',(-13.4124077844404,14.2892041446737,
132.900320701676)) ;
#136282=CARTESIAN_POINT('Ctrl Pts',(-13.4844837717321,14.4332159069687,
133.144089592404)) ;
#136283=CARTESIAN_POINT('Ctrl Pts',(-13.5657740695195,14.5042073782218,
133.414672215616)) ;
#136284=CARTESIAN_POINT('Ctrl Pts',(-13.6499188668072,14.4978850554144,
133.693611525571)) ;
#136285=CARTESIAN_POINT('Ctrl Pts',(-13.7301300690243,14.4145534025925,
133.96105201458)) ;
#136286=CARTESIAN_POINT('Ctrl Pts',(-13.7999841881705,14.2600830965558,
134.198257775645)) ;
#136287=CARTESIAN_POINT('Ctrl Pts',(-13.8535974701144,14.0459659620245,
134.387963859614)) ;
#136288=CARTESIAN_POINT('Ctrl Pts',(-13.8866069561238,13.7875807752627,
134.517459877776)) ;
#136289=CARTESIAN_POINT('Ctrl Pts',(-13.8958448391708,13.5015008973902,
134.577698082975)) ;
#136290=CARTESIAN_POINT('Ctrl Pts',(-13.8799187621032,13.2119712102584,
134.564171528529)) ;
#136291=CARTESIAN_POINT('Ctrl Pts',(-13.8392809382772,12.9363053782512,
134.478593815727)) ;
#136292=CARTESIAN_POINT('Ctrl Pts',(-13.7758444278724,12.6952736602129,
134.326473645072)) ;
#136293=CARTESIAN_POINT('Ctrl Pts',(-13.6940162958856,12.507125678723,134.120477732686)) ;
#136294=CARTESIAN_POINT('Ctrl Pts',(-13.5977907900013,12.3837628513247,
133.872694312529)) ;
#136295=CARTESIAN_POINT('Ctrl Pts',(-13.4952077550757,12.3357954087756,
133.605958381013)) ;
#136296=CARTESIAN_POINT('Ctrl Pts',(-13.3909244959306,12.3652711251859,
133.33454614811)) ;
#136297=CARTESIAN_POINT('Ctrl Pts',(-13.2930291637441,12.4705156806676,
133.081632751708)) ;
#136298=CARTESIAN_POINT('Ctrl Pts',(-13.2071658759881,12.6439184973371,
132.863918116231)) ;
#136299=CARTESIAN_POINT('Ctrl Pts',(-13.1389101581012,12.8730354055636,
132.697626362)) ;
#136300=CARTESIAN_POINT('Ctrl Pts',(-13.0923226075365,13.1424159445997,
132.594737929481)) ;
#136301=CARTESIAN_POINT('Ctrl Pts',(-13.0702865542668,13.4306391754528,
132.563415021775)) ;
#136302=CARTESIAN_POINT('Ctrl Pts',(-13.0733966131089,13.7191539441457,
132.605650335791)) ;
#136303=CARTESIAN_POINT('Ctrl Pts',(-13.1008205861734,13.9861293896989,
132.718874470187)) ;
#136304=CARTESIAN_POINT('Ctrl Pts',(-13.1498037441585,14.2128684001206,
132.89508138218)) ;
#136305=CARTESIAN_POINT('Ctrl Pts',(-13.2163126321001,14.3833347965248,
133.122557153896)) ;
#136306=CARTESIAN_POINT('Ctrl Pts',(-13.2945517934649,14.4845639099252,
133.384224457738)) ;
#136307=CARTESIAN_POINT('Ctrl Pts',(-13.3782996834148,14.5099092471542,
133.66197841254)) ;
#136308=CARTESIAN_POINT('Ctrl Pts',(-13.4610067103196,14.4573341215463,
133.936748595732)) ;
#136309=CARTESIAN_POINT('Ctrl Pts',(-13.535792979438,14.3305258270945,134.188357582262)) ;
#136310=CARTESIAN_POINT('Ctrl Pts',(-13.5964938791261,14.1393930806654,
134.398720829303)) ;
#136311=CARTESIAN_POINT('Ctrl Pts',(-13.6384531516596,13.8963012865058,
134.554456038958)) ;
#136312=CARTESIAN_POINT('Ctrl Pts',(-13.6575588644819,13.618527952916,134.64350061979)) ;
#136313=CARTESIAN_POINT('Ctrl Pts',(-13.6518640795297,13.3290638567204,
134.659826711564)) ;
#136314=CARTESIAN_POINT('Ctrl Pts',(-13.6210222993908,13.0445549081066,
134.602903919085)) ;
#136315=CARTESIAN_POINT('Ctrl Pts',(-13.5665781809899,12.7876683953407,
134.476958833009)) ;
#136316=CARTESIAN_POINT('Ctrl Pts',(-13.4911864112069,12.5753843248543,
134.290002560966)) ;
#136317=CARTESIAN_POINT('Ctrl Pts',(-13.4007901006825,12.4255194566962,
134.05888370733)) ;
#136318=CARTESIAN_POINT('Ctrl Pts',(-13.2997237377735,12.3459765628223,
133.796830310285)) ;
#136319=CARTESIAN_POINT('Ctrl Pts',(-13.1954991747945,12.3439073333341,
133.52541389548)) ;
#136320=CARTESIAN_POINT('Ctrl Pts',(-13.0941541677024,12.4188279963137,
133.262499854551)) ;
#136321=CARTESIAN_POINT('Ctrl Pts',(-13.002205997662,12.5669347456838,133.027188569075)) ;
#136322=CARTESIAN_POINT('Ctrl Pts',(-12.9267422753913,12.7740276750078,
132.839635132885)) ;
#136323=CARTESIAN_POINT('Ctrl Pts',(-12.8706659445136,13.0302839963835,
132.709131418789)) ;
#136324=CARTESIAN_POINT('Ctrl Pts',(-12.8386183811773,13.3133908418281,
132.648618515674)) ;
#136325=CARTESIAN_POINT('Ctrl Pts',(-12.8315791622469,13.603463644202,132.661074904967)) ;
#136326=CARTESIAN_POINT('Ctrl Pts',(-12.8492844367411,13.8813033828735,
132.745878981524)) ;
#136327=CARTESIAN_POINT('Ctrl Pts',(-12.8901906349179,14.1277803353935,
132.898667421918)) ;
#136328=CARTESIAN_POINT('Ctrl Pts',(-12.9502027043241,14.3222499491186,
133.107092668811)) ;
#136329=CARTESIAN_POINT('Ctrl Pts',(-13.0241102247799,14.4521801137134,
133.356004116762)) ;
#136330=CARTESIAN_POINT('Ctrl Pts',(-13.1064456796044,14.5090397013049,
133.629648846685)) ;
#136331=CARTESIAN_POINT('Ctrl Pts',(-13.1904091031337,14.4879536383768,
133.908074847443)) ;
#136332=CARTESIAN_POINT('Ctrl Pts',(-13.2691730073198,14.3907169193799,
134.171290632638)) ;
#136333=CARTESIAN_POINT('Ctrl Pts',(-13.3365717682159,14.2230874926912,
134.401446847104)) ;
#136334=CARTESIAN_POINT('Ctrl Pts',(-13.3862837725614,14.0008521290395,
134.579526433076)) ;
#136335=CARTESIAN_POINT('Ctrl Pts',(-13.4151850077251,13.7343152663338,
134.697246128251)) ;
#136336=CARTESIAN_POINT('Ctrl Pts',(-13.4196674461843,13.4474451530714,
134.74336669151)) ;
#136337=CARTESIAN_POINT('Ctrl Pts',(-13.3989374427175,13.1575373599845,
134.716000021385)) ;
#136338=CARTESIAN_POINT('Ctrl Pts',(-13.3538701206744,12.8878586186382,
134.617383543723)) ;
#136339=CARTESIAN_POINT('Ctrl Pts',(-13.2866697814604,12.6555337160297,
134.454240239388)) ;
#136340=CARTESIAN_POINT('Ctrl Pts',(-13.2016717965965,12.4784852863875,
134.239051541609)) ;
#136341=CARTESIAN_POINT('Ctrl Pts',(-13.103660140851,12.3688435126028,133.986006271584)) ;
#136342=CARTESIAN_POINT('Ctrl Pts',(-13.0001912147535,12.335379050582,133.716752546929)) ;
#136343=CARTESIAN_POINT('Ctrl Pts',(-12.8968764365744,12.3794309050292,
133.448054757706)) ;
#136344=CARTESIAN_POINT('Ctrl Pts',(-12.8007211226384,12.4979553005814,
133.200237570607)) ;
#136345=CARTESIAN_POINT('Ctrl Pts',(-12.7173411751848,12.6843641512771,
132.989987119788)) ;
#136346=CARTESIAN_POINT('Ctrl Pts',(-12.6533675978781,12.9208195190715,
132.835987884663)) ;
#136347=CARTESIAN_POINT('Ctrl Pts',(-12.6110523141971,13.1965599156971,
132.745711948575)) ;
#136348=CARTESIAN_POINT('Ctrl Pts',(-12.5938677361115,13.4854150034454,
132.728459041513)) ;
#136349=CARTESIAN_POINT('Ctrl Pts',(-12.6016166796287,13.7715245103546,
132.784247690811)) ;
#136350=CARTESIAN_POINT('Ctrl Pts',(-12.6334808333027,14.0329603333754,
132.910531351478)) ;
#136351=CARTESIAN_POINT('Ctrl Pts',(-12.6860159227242,14.2495174070446,
133.097035811552)) ;
#136352=CARTESIAN_POINT('Ctrl Pts',(-12.7550120282424,14.4077221355952,
133.331704202413)) ;
#136353=CARTESIAN_POINT('Ctrl Pts',(-12.8352852858367,14.4954974794661,
133.599515576589)) ;
#136354=CARTESIAN_POINT('Ctrl Pts',(-12.9190639071468,14.5058124227374,
133.877251814252)) ;
#136355=CARTESIAN_POINT('Ctrl Pts',(-13.0006861903333,14.4390540160987,
134.148810770118)) ;
#136356=CARTESIAN_POINT('Ctrl Pts',(-13.0734798970183,14.2988995016989,
134.394674718231)) ;
#136357=CARTESIAN_POINT('Ctrl Pts',(-13.1310605574008,14.0959846822767,
134.59603545551)) ;
#136358=CARTESIAN_POINT('Ctrl Pts',(-13.1686602075177,13.8467238077785,
134.738805253809)) ;
#136359=CARTESIAN_POINT('Ctrl Pts',(-13.1832960063071,13.5651499595772,
134.814759605636)) ;
#136360=CARTESIAN_POINT('Ctrl Pts',(-13.1728859358929,13.2745210705863,
134.817404454761)) ;
#136361=CARTESIAN_POINT('Ctrl Pts',(-13.1372979957402,12.9930481847516,
134.746685223495)) ;
#136362=CARTESIAN_POINT('Ctrl Pts',(-13.0788464460579,12.7442685275202,
134.608933005347)) ;
#136363=CARTESIAN_POINT('Ctrl Pts',(-13.0004860021476,12.5428869624623,
134.413170014133)) ;
#136364=CARTESIAN_POINT('Ctrl Pts',(-12.9071846487547,12.4047083280592,
134.173773807101)) ;
#136365=CARTESIAN_POINT('Ctrl Pts',(-12.8051561028839,12.3396945526809,
133.90883173255)) ;
#136366=CARTESIAN_POINT('Ctrl Pts',(-12.7008909970313,12.3521469576885,
133.637337257152)) ;
#136367=CARTESIAN_POINT('Ctrl Pts',(-12.6009173642389,12.441314353945,133.378426035197)) ;
#136368=CARTESIAN_POINT('Ctrl Pts',(-12.5117677396135,12.6011043288198,
133.151163527727)) ;
#136369=CARTESIAN_POINT('Ctrl Pts',(-12.4393294114449,12.8194224397463,
132.97265105268)) ;
#136370=CARTESIAN_POINT('Ctrl Pts',(-12.387790426931,13.0811434342732,132.85522288076)) ;
#136371=CARTESIAN_POINT('Ctrl Pts',(-12.360228261411,13.3679217852881,132.807894792067)) ;
#136372=CARTESIAN_POINT('Ctrl Pts',(-12.3579523050129,13.6574454003315,
132.834298017918)) ;
#136373=CARTESIAN_POINT('Ctrl Pts',(-12.3801380175334,13.9304218890574,
132.932167779584)) ;
#136374=CARTESIAN_POINT('Ctrl Pts',(-12.4250230602689,14.1686008595605,
133.096583317216)) ;
#136375=CARTESIAN_POINT('Ctrl Pts',(-12.4878388913045,14.3514046814191,
133.313074404504)) ;
#136376=CARTESIAN_POINT('Ctrl Pts',(-12.5640867721586,14.4688537010489,
133.568976881112)) ;
#136377=CARTESIAN_POINT('Ctrl Pts',(-12.6473280614042,14.5110084065472,
133.845298914204)) ;
#136378=CARTESIAN_POINT('Ctrl Pts',(-12.7306234368668,14.4754271659884,
134.121689851781)) ;
#136379=CARTESIAN_POINT('Ctrl Pts',(-12.8078424891508,14.3641624802179,
134.38046802569)) ;
#136380=CARTESIAN_POINT('Ctrl Pts',(-12.8722362238059,14.1852632695012,
134.601742519835)) ;
#136381=CARTESIAN_POINT('Ctrl Pts',(-12.9184596429682,13.9526451401233,
134.769816657982)) ;
#136382=CARTESIAN_POINT('Ctrl Pts',(-12.9427606566985,13.6818447118076,
134.873904342633)) ;
#136383=CARTESIAN_POINT('Ctrl Pts',(-12.9426329031674,13.3926206452482,
134.906615051885)) ;
#136384=CARTESIAN_POINT('Ctrl Pts',(-12.9170454040847,13.1038754923078,
134.865156068369)) ;
#136385=CARTESIAN_POINT('Ctrl Pts',(-12.8675913433402,12.8403836297391,
134.753690916011)) ;
#136386=CARTESIAN_POINT('Ctrl Pts',(-12.7967823441445,12.6175434576375,
134.579955954179)) ;
#136387=CARTESIAN_POINT('Ctrl Pts',(-12.70868276548,12.4520178789147,134.355810149669)) ;
#136388=CARTESIAN_POINT('Ctrl Pts',(-12.6093449823904,12.3567780608222,
134.098765452035)) ;
#136389=CARTESIAN_POINT('Ctrl Pts',(-12.5056341234011,12.3376561109864,
133.828749759816)) ;
#136390=CARTESIAN_POINT('Ctrl Pts',(-12.402751079868,12.3963494804203,133.561441007829)) ;
#136391=CARTESIAN_POINT('Ctrl Pts',(-12.3088084112223,12.5282529228556,
133.320050046839)) ;
#136392=CARTESIAN_POINT('Ctrl Pts',(-12.2289334019483,12.7243873042916,
133.119846376778)) ;
#136393=CARTESIAN_POINT('Ctrl Pts',(-12.1683661165357,12.9708923918956,
132.976071926915)) ;
#136394=CARTESIAN_POINT('Ctrl Pts',(-12.1308341182304,13.2502126197918,
132.899629391339)) ;
#136395=CARTESIAN_POINT('Ctrl Pts',(-12.1182778756421,13.5400583828972,
132.895929792219)) ;
#136396=CARTESIAN_POINT('Ctrl Pts',(-12.1307869570981,13.8239338286533,
132.965735493257)) ;
#136397=CARTESIAN_POINT('Ctrl Pts',(-12.1668484142908,14.0777676729547,
133.104202368024)) ;
#136398=CARTESIAN_POINT('Ctrl Pts',(-12.222772912384,14.2841378500946,133.300577303525)) ;
#136399=CARTESIAN_POINT('Ctrl Pts',(-12.2942910489215,14.429815657766,133.542627629611)) ;
#136400=CARTESIAN_POINT('Ctrl Pts',(-12.3756729115768,14.5033259168077,
133.813595342621)) ;
#136401=CARTESIAN_POINT('Ctrl Pts',(-12.4597832810724,14.499135115111,134.092410952893)) ;
#136402=CARTESIAN_POINT('Ctrl Pts',(-12.5402566051309,14.4177798325381,
134.360648411857)) ;
#136403=CARTESIAN_POINT('Ctrl Pts',(-12.6102648440973,14.2657377102023,
134.59819459311)) ;
#136404=CARTESIAN_POINT('Ctrl Pts',(-12.6646057115603,14.0527574173429,
134.790109616224)) ;
#136405=CARTESIAN_POINT('Ctrl Pts',(-12.6982822917971,13.7942044324148,
134.921686113269)) ;
#136406=CARTESIAN_POINT('Ctrl Pts',(-12.7081236290535,13.509972220369,134.983521067054)) ;
#136407=CARTESIAN_POINT('Ctrl Pts',(-12.6929226435767,13.219834764377,134.972169824304)) ;
#136408=CARTESIAN_POINT('Ctrl Pts',(-12.6529041959642,12.9433154987134,
134.888419817773)) ;
#136409=CARTESIAN_POINT('Ctrl Pts',(-12.5899125810331,12.7008042356819,
134.737648548155)) ;
#136410=CARTESIAN_POINT('Ctrl Pts',(-12.5088132067507,12.5118988342583,
134.533656568728)) ;
#136411=CARTESIAN_POINT('Ctrl Pts',(-12.4134247671775,12.3867144480253,
134.288156510762)) ;
#136412=CARTESIAN_POINT('Ctrl Pts',(-12.3103723850424,12.3359851161897,
134.020244487105)) ;
#136413=CARTESIAN_POINT('Ctrl Pts',(-12.2060535029749,12.3634203970633,
133.748717660543)) ;
#136414=CARTESIAN_POINT('Ctrl Pts',(-12.1079177935451,12.4663876358086,
133.495088507556)) ;
#136415=CARTESIAN_POINT('Ctrl Pts',(-12.0212873996097,12.6389701182042,
133.275282296474)) ;
#136416=CARTESIAN_POINT('Ctrl Pts',(-11.9528459850857,12.8657474577828,
133.108290126159)) ;
#136417=CARTESIAN_POINT('Ctrl Pts',(-11.9054705654115,13.1346343436699,
133.003152675926)) ;
#136418=CARTESIAN_POINT('Ctrl Pts',(-11.8903642795437,13.3266512177486,
132.98106317886)) ;
#136419=CARTESIAN_POINT('Ctrl Pts',(-11.8869647971046,13.4226801736581,
132.982153164817)) ;
#136420=CARTESIAN_POINT('Ctrl Pts',(-33.3254395351173,13.1734341962953,
127.803113044878)) ;
#136421=CARTESIAN_POINT('Ctrl Pts',(-33.3247359866207,13.1676985117492,
127.801788763031)) ;
#136422=CARTESIAN_POINT('Ctrl Pts',(-33.3132623631218,13.0762045259503,
127.779953878293)) ;
#136423=CARTESIAN_POINT('Ctrl Pts',(-33.282285149324,12.9034782773047,127.712436580561)) ;
#136424=CARTESIAN_POINT('Ctrl Pts',(-33.2176093851333,12.6923998391673,
127.556524920366)) ;
#136425=CARTESIAN_POINT('Ctrl Pts',(-33.1366442117355,12.5327609209973,
127.353111300579)) ;
#136426=CARTESIAN_POINT('Ctrl Pts',(-33.0439865108413,12.4368205813749,
127.115708366726)) ;
#136427=CARTESIAN_POINT('Ctrl Pts',(-32.9470466339548,12.4119420222618,
126.865451857032)) ;
#136428=CARTESIAN_POINT('Ctrl Pts',(-32.8502205148306,12.4592681303251,
126.615824485106)) ;
#136429=CARTESIAN_POINT('Ctrl Pts',(-32.7609435571221,12.5756589901857,
126.388116095926)) ;
#136430=CARTESIAN_POINT('Ctrl Pts',(-32.6843652232408,12.7528353501054,
126.197555194626)) ;
#136431=CARTESIAN_POINT('Ctrl Pts',(-32.6254359841591,12.9779970726337,
126.058531505893)) ;
#136432=CARTESIAN_POINT('Ctrl Pts',(-32.5876159994447,13.2349353323575,
125.981163983675)) ;
#136433=CARTESIAN_POINT('Ctrl Pts',(-32.5727992859682,13.5051817925228,
125.970971172671)) ;
#136434=CARTESIAN_POINT('Ctrl Pts',(-32.5815223767738,13.7710455478253,
126.029743179252)) ;
#136435=CARTESIAN_POINT('Ctrl Pts',(-32.6121127150153,14.0095405119009,
126.15206688756)) ;
#136436=CARTESIAN_POINT('Ctrl Pts',(-32.6618848688714,14.207375982779,126.330592997822)) ;
#136437=CARTESIAN_POINT('Ctrl Pts',(-32.7265064202986,14.3489569036635,
126.552483435506)) ;
#136438=CARTESIAN_POINT('Ctrl Pts',(-32.8008290640631,14.4243647348289,
126.802810757179)) ;
#136439=CARTESIAN_POINT('Ctrl Pts',(-32.8783902118096,14.4276726167065,
127.062506054467)) ;
#136440=CARTESIAN_POINT('Ctrl Pts',(-32.9529895057271,14.3592846174027,
127.313499396792)) ;
#136441=CARTESIAN_POINT('Ctrl Pts',(-33.0187620925496,14.2239083327593,
127.538741069416)) ;
#136442=CARTESIAN_POINT('Ctrl Pts',(-33.0702809219999,14.0309432296264,
127.722391722539)) ;
#136443=CARTESIAN_POINT('Ctrl Pts',(-33.1029915194089,13.793723337017,127.851172033353)) ;
#136444=CARTESIAN_POINT('Ctrl Pts',(-33.1137372251236,13.531837086658,127.915541813163)) ;
#136445=CARTESIAN_POINT('Ctrl Pts',(-33.1012954087164,13.2609089527483,
127.912338104309)) ;
#136446=CARTESIAN_POINT('Ctrl Pts',(-33.0654710758441,13.0011532245151,
127.840894256415)) ;
#136447=CARTESIAN_POINT('Ctrl Pts',(-33.0086291360852,12.7729628061281,
127.707856012819)) ;
#136448=CARTESIAN_POINT('Ctrl Pts',(-32.9334589590993,12.5901802135074,
127.521462919618)) ;
#136449=CARTESIAN_POINT('Ctrl Pts',(-32.8452372911632,12.4676468179757,
127.296813129222)) ;
#136450=CARTESIAN_POINT('Ctrl Pts',(-32.74883806695,12.4133145081089,127.048434581224)) ;
#136451=CARTESIAN_POINT('Ctrl Pts',(-32.651505357267,12.4313808819739,126.797103381314)) ;
#136452=CARTESIAN_POINT('Ctrl Pts',(-32.5582583386558,12.520660304575,126.557917651661)) ;
#136453=CARTESIAN_POINT('Ctrl Pts',(-32.4760025184329,12.6744195620442,
126.350716856275)) ;
#136454=CARTESIAN_POINT('Ctrl Pts',(-32.4094362840527,12.8815892822748,
126.189358896427)) ;
#136455=CARTESIAN_POINT('Ctrl Pts',(-32.3625474664159,13.1290193057785,
126.085663140554)) ;
#136456=CARTESIAN_POINT('Ctrl Pts',(-32.3384651461866,13.3950772223713,
126.048272145446)) ;
#136457=CARTESIAN_POINT('Ctrl Pts',(-32.3375813691581,13.66434219871,126.078804798388)) ;
#136458=CARTESIAN_POINT('Ctrl Pts',(-32.3596574822361,13.9170737503532,
126.176511056621)) ;
#136459=CARTESIAN_POINT('Ctrl Pts',(-32.4021492792394,14.1334228182709,
126.333728828426)) ;
#136460=CARTESIAN_POINT('Ctrl Pts',(-32.4612401199057,14.2989215662944,
126.539406409158)) ;
#136461=CARTESIAN_POINT('Ctrl Pts',(-32.5321839761624,14.4021434485844,
126.779768376024)) ;
#136462=CARTESIAN_POINT('Ctrl Pts',(-32.6093004013496,14.4351203020035,
127.038251205167)) ;
#136463=CARTESIAN_POINT('Ctrl Pts',(-32.685749140631,14.3956460292368,127.294619936752)) ;
#136464=CARTESIAN_POINT('Ctrl Pts',(-32.7559987732593,14.2864256382767,
127.533007359851)) ;
#136465=CARTESIAN_POINT('Ctrl Pts',(-32.8139294455932,14.1149876156061,
127.735413101504)) ;
#136466=CARTESIAN_POINT('Ctrl Pts',(-32.8545469809948,13.8950778859157,
127.887084365748)) ;
#136467=CARTESIAN_POINT('Ctrl Pts',(-32.8745963697914,13.6402949383964,
127.97883429511)) ;
#136468=CARTESIAN_POINT('Ctrl Pts',(-32.8716009144099,13.3700135586503,
128.003243267968)) ;
#136469=CARTESIAN_POINT('Ctrl Pts',(-32.8451817708658,13.1040821018971,
127.959163781802)) ;
#136470=CARTESIAN_POINT('Ctrl Pts',(-32.7965610116962,12.8608604058745,
127.850228031512)) ;
#136471=CARTESIAN_POINT('Ctrl Pts',(-32.7280100000708,12.6570995861258,
127.683237242378)) ;
#136472=CARTESIAN_POINT('Ctrl Pts',(-32.6448060717616,12.5097126273575,
127.473139968475)) ;
#136473=CARTESIAN_POINT('Ctrl Pts',(-32.5510193789591,12.4266925864004,
127.23233405547)) ;
#136474=CARTESIAN_POINT('Ctrl Pts',(-32.4532256004834,12.4153566077392,
126.979772250946)) ;
#136475=CARTESIAN_POINT('Ctrl Pts',(-32.3576194837689,12.4761183331586,
126.73359550688)) ;
#136476=CARTESIAN_POINT('Ctrl Pts',(-32.2703085357419,12.6046109786899,
126.511640612033)) ;
#136477=CARTESIAN_POINT('Ctrl Pts',(-32.1966708395862,12.792032892229,126.32968693581)) ;
#136478=CARTESIAN_POINT('Ctrl Pts',(-32.141491025989,13.0246459231079,126.201630976747)) ;
#136479=CARTESIAN_POINT('Ctrl Pts',(-32.1079590635852,13.2849675496699,
126.136714360042)) ;
#136480=CARTESIAN_POINT('Ctrl Pts',(-32.0975331597763,13.5561838423073,
126.139422059227)) ;
#136481=CARTESIAN_POINT('Ctrl Pts',(-32.1105557909978,13.8182129454441,
126.210683763545)) ;
#136482=CARTESIAN_POINT('Ctrl Pts',(-32.1449979162491,14.0504673994418,
126.344307337019)) ;
#136483=CARTESIAN_POINT('Ctrl Pts',(-32.1981332617765,14.2392687956967,
126.532766020785)) ;
#136484=CARTESIAN_POINT('Ctrl Pts',(-32.2650887614462,14.3686948710642,
126.761498858709)) ;
#136485=CARTESIAN_POINT('Ctrl Pts',(-32.3399771946658,14.4303698610576,
127.013234105376)) ;
#136486=CARTESIAN_POINT('Ctrl Pts',(-32.4176418524857,14.4203874495029,
127.273299867643)) ;
#136487=CARTESIAN_POINT('Ctrl Pts',(-32.4913827908126,14.3383234433453,
127.521952665853)) ;
#136488=CARTESIAN_POINT('Ctrl Pts',(-32.5547753616378,14.1909247439309,
127.740243611178)) ;
#136489=CARTESIAN_POINT('Ctrl Pts',(-32.6027829052078,13.9894772519221,
127.913477677594)) ;
#136490=CARTESIAN_POINT('Ctrl Pts',(-32.6315787822835,13.7468083909025,
128.030718638725)) ;
#136491=CARTESIAN_POINT('Ctrl Pts',(-32.6381297055454,13.4802543553281,
128.083052077669)) ;
#136492=CARTESIAN_POINT('Ctrl Pts',(-32.621004032577,13.2092851257182,128.066265392245)) ;
#136493=CARTESIAN_POINT('Ctrl Pts',(-32.5813816261219,12.956342695595,127.983398583339)) ;
#136494=CARTESIAN_POINT('Ctrl Pts',(-32.5205209542112,12.7340443035837,
127.838851944066)) ;
#136495=CARTESIAN_POINT('Ctrl Pts',(-32.4424022518424,12.5620254475304,
127.643824006467)) ;
#136496=CARTESIAN_POINT('Ctrl Pts',(-32.3525984203938,12.45216345603,127.414440626927)) ;
#136497=CARTESIAN_POINT('Ctrl Pts',(-32.2552772387971,12.4110698281944,
127.163418282472)) ;
#136498=CARTESIAN_POINT('Ctrl Pts',(-32.1580021613722,12.4431134785041,
126.912378453322)) ;
#136499=CARTESIAN_POINT('Ctrl Pts',(-32.0668852322613,12.544720783163,126.679216971146)) ;
#136500=CARTESIAN_POINT('Ctrl Pts',(-31.9870500616397,12.7094608170751,
126.479131976701)) ;
#136501=CARTESIAN_POINT('Ctrl Pts',(-31.9237909814612,12.9261933498066,
126.32756494422)) ;
#136502=CARTESIAN_POINT('Ctrl Pts',(-31.8812909269055,13.1767718308822,
126.236400480011)) ;
#136503=CARTESIAN_POINT('Ctrl Pts',(-31.861298454265,13.4474343048381,126.211302126729)) ;
#136504=CARTESIAN_POINT('Ctrl Pts',(-31.8650124128939,13.7143157453809,
126.255202512803)) ;
#136505=CARTESIAN_POINT('Ctrl Pts',(-31.8909286602407,13.9601208806252,
126.363903867448)) ;
#136506=CARTESIAN_POINT('Ctrl Pts',(-31.9370786723428,14.1691500146303,
126.531977690957)) ;
#136507=CARTESIAN_POINT('Ctrl Pts',(-31.9987411279638,14.3234012813758,
126.74512586519)) ;
#136508=CARTESIAN_POINT('Ctrl Pts',(-32.0713879414062,14.4138714388817,
126.990519088113)) ;
#136509=CARTESIAN_POINT('Ctrl Pts',(-32.1486213371649,14.433295070235,127.249205234635)) ;
#136510=CARTESIAN_POINT('Ctrl Pts',(-32.2249233067821,14.3798377067091,
127.505417902984)) ;
#136511=CARTESIAN_POINT('Ctrl Pts',(-32.292842495317,14.2584887860387,127.736813241794)) ;
#136512=CARTESIAN_POINT('Ctrl Pts',(-32.3478706736015,14.0772215251275,
127.930687195659)) ;
#136513=CARTESIAN_POINT('Ctrl Pts',(-32.385043591268,13.847858128252,128.072541376849)) ;
#136514=CARTESIAN_POINT('Ctrl Pts',(-32.4006697912098,13.5896600373134,
128.151227440308)) ;
#136515=CARTESIAN_POINT('Ctrl Pts',(-32.3933293828918,13.3195390353182,
128.162833702852)) ;
#136516=CARTESIAN_POINT('Ctrl Pts',(-32.362503604888,13.0556171631187,128.105986435172)) ;
#136517=CARTESIAN_POINT('Ctrl Pts',(-32.3099087281082,12.8189344364704,
127.985427645554)) ;
#136518=CARTESIAN_POINT('Ctrl Pts',(-32.2383978311714,12.6251004110513,
127.809670253998)) ;
#136519=CARTESIAN_POINT('Ctrl Pts',(-32.1525576056768,12.4887479855771,
127.592000333581)) ;
#136520=CARTESIAN_POINT('Ctrl Pts',(-32.0577945487542,12.419067054962,127.348242601568)) ;
#136521=CARTESIAN_POINT('Ctrl Pts',(-31.9596036759549,12.4213699638912,
127.094633590444)) ;
#136522=CARTESIAN_POINT('Ctrl Pts',(-31.8652480188587,12.4953802031986,
126.852058359587)) ;
#136523=CARTESIAN_POINT('Ctrl Pts',(-31.7800198291274,12.6359571478174,
126.636236452674)) ;
#136524=CARTESIAN_POINT('Ctrl Pts',(-31.7096390960426,12.8329196540899,
126.463760566805)) ;
#136525=CARTESIAN_POINT('Ctrl Pts',(-31.6583487363999,13.0719648930025,
126.347032519857)) ;
#136526=CARTESIAN_POINT('Ctrl Pts',(-31.6290353321278,13.3363496355774,
126.294530496598)) ;
#136527=CARTESIAN_POINT('Ctrl Pts',(-31.6231309158897,13.6070576006529,
126.310423983356)) ;
#136528=CARTESIAN_POINT('Ctrl Pts',(-31.6403386798103,13.8644611285128,
126.393821576157)) ;
#136529=CARTESIAN_POINT('Ctrl Pts',(-31.6786205812712,14.0900772537897,
126.53875012761)) ;
#136530=CARTESIAN_POINT('Ctrl Pts',(-31.7346571079609,14.2682172289019,
126.735603420313)) ;
#136531=CARTESIAN_POINT('Ctrl Pts',(-31.803393598769,14.3854165946879,126.969447305855)) ;
#136532=CARTESIAN_POINT('Ctrl Pts',(-31.8795398028215,14.4341663213204,
127.225014629057)) ;
#136533=CARTESIAN_POINT('Ctrl Pts',(-31.9569737821743,14.4102121337139,
127.484427730781)) ;
#136534=CARTESIAN_POINT('Ctrl Pts',(-32.0289551185517,14.3156229192553,
127.727797868407)) ;
#136535=CARTESIAN_POINT('Ctrl Pts',(-32.0899457704392,14.1571117362938,
127.939092933894)) ;
#136536=CARTESIAN_POINT('Ctrl Pts',(-32.1347596628421,13.9459764077607,
128.103131375364)) ;
#136537=CARTESIAN_POINT('Ctrl Pts',(-32.1594663640903,13.6975622322246,
128.208410639942)) ;
#136538=CARTESIAN_POINT('Ctrl Pts',(-32.1615862487737,13.4293974985453,
128.247722758148)) ;
#136539=CARTESIAN_POINT('Ctrl Pts',(-32.140285070969,13.1610019357677,128.218585285993)) ;
#136540=CARTESIAN_POINT('Ctrl Pts',(-32.0961603941235,12.9105848440385,
128.12288354399)) ;
#136541=CARTESIAN_POINT('Ctrl Pts',(-32.0318978199246,12.6976134711112,
127.968256892856)) ;
#136542=CARTESIAN_POINT('Ctrl Pts',(-31.9512431314668,12.5364422844779,
127.765768139102)) ;
#136543=CARTESIAN_POINT('Ctrl Pts',(-31.8593208623527,12.4387732297296,
127.530343940325)) ;
#136544=CARTESIAN_POINT('Ctrl Pts',(-31.7616857575535,12.4116342438892,
127.278318451746)) ;
#136545=CARTESIAN_POINT('Ctrl Pts',(-31.6652363599927,12.4569142353896,
127.029622347502)) ;
#136546=CARTESIAN_POINT('Ctrl Pts',(-31.5755156798081,12.5714751747461,
126.800673437744)) ;
#136547=CARTESIAN_POINT('Ctrl Pts',(-31.4986226921134,12.7468632873084,
126.609142921284)) ;
#136548=CARTESIAN_POINT('Ctrl Pts',(-31.4391185557765,12.9706872458922,
126.468427929382)) ;
#136549=CARTESIAN_POINT('Ctrl Pts',(-31.4006101144724,13.2271704836993,
126.389077954558)) ;
#136550=CARTESIAN_POINT('Ctrl Pts',(-31.3851182967717,13.4971329274745,
126.376892427359)) ;
#136551=CARTESIAN_POINT('Ctrl Pts',(-31.3931465053214,13.7633005024016,
126.433617383089)) ;
#136552=CARTESIAN_POINT('Ctrl Pts',(-31.4230717823098,14.002826770648,126.553990439311)) ;
#136553=CARTESIAN_POINT('Ctrl Pts',(-31.4725840354185,14.2028677119568,
126.731901109757)) ;
#136554=CARTESIAN_POINT('Ctrl Pts',(-31.5366209577425,14.3455611134847,
126.951952487503)) ;
#136555=CARTESIAN_POINT('Ctrl Pts',(-31.6107344089728,14.4231516282667,
127.201672543475)) ;
#136556=CARTESIAN_POINT('Ctrl Pts',(-31.6883036036575,14.4286657485207,
127.461395249587)) ;
#136557=CARTESIAN_POINT('Ctrl Pts',(-31.7632257320844,14.3621070241951,
127.713405765765)) ;
#136558=CARTESIAN_POINT('Ctrl Pts',(-31.8292721612924,14.2287344049999,
127.939404631142)) ;
#136559=CARTESIAN_POINT('Ctrl Pts',(-31.8813900908942,14.0363062184854,
128.124936526363)) ;
#136560=CARTESIAN_POINT('Ctrl Pts',(-31.9144283378458,13.8023698285734,
128.254361978838)) ;
#136561=CARTESIAN_POINT('Ctrl Pts',(-31.9260122072278,13.538853365046,128.321462132145)) ;
#136562=CARTESIAN_POINT('Ctrl Pts',(-31.914128124353,13.2684519615159,128.319816614393)) ;
#136563=CARTESIAN_POINT('Ctrl Pts',(-31.8791690447666,13.0087998067706,
128.250796154468)) ;
#136564=CARTESIAN_POINT('Ctrl Pts',(-31.8224023910236,12.7778891535909,
128.118233618976)) ;
#136565=CARTESIAN_POINT('Ctrl Pts',(-31.7482172105361,12.5950174463895,
127.934464371389)) ;
#136566=CARTESIAN_POINT('Ctrl Pts',(-31.6598803438761,12.4700325386615,
127.709648223425)) ;
#136567=CARTESIAN_POINT('Ctrl Pts',(-31.5641604318378,12.4138573770184,
127.463058249321)) ;
#136568=CARTESIAN_POINT('Ctrl Pts',(-31.4659188821753,12.4301864135647,
127.209377342197)) ;
#136569=CARTESIAN_POINT('Ctrl Pts',(-31.3734534378068,12.5166843884807,
126.972114937016)) ;
#136570=CARTESIAN_POINT('Ctrl Pts',(-31.2902901080974,12.6693064636983,
126.762458503211)) ;
#136571=CARTESIAN_POINT('Ctrl Pts',(-31.2234519388235,12.8745470940793,
126.600193818904)) ;
#136572=CARTESIAN_POINT('Ctrl Pts',(-31.1758307675459,13.1212023426986,
126.494392150649)) ;
#136573=CARTESIAN_POINT('Ctrl Pts',(-31.1510486370885,13.3871938876445,
126.454987702193)) ;
#136574=CARTESIAN_POINT('Ctrl Pts',(-31.1495067038997,13.6567281593303,
126.483608122168)) ;
#136575=CARTESIAN_POINT('Ctrl Pts',(-31.1708676258371,13.9097854189498,
126.579158796714)) ;
#136576=CARTESIAN_POINT('Ctrl Pts',(-31.2129315448557,14.1280196349839,
126.73522563179)) ;
#136577=CARTESIAN_POINT('Ctrl Pts',(-31.2715422679824,14.2950456009744,
126.939462493752)) ;
#136578=CARTESIAN_POINT('Ctrl Pts',(-31.3426766589583,14.4005267641298,
127.180579567432)) ;
#136579=CARTESIAN_POINT('Ctrl Pts',(-31.4191922825314,14.4350836720727,
127.437076071627)) ;
#136580=CARTESIAN_POINT('Ctrl Pts',(-31.4958370560869,14.3978038966436,
127.694063116912)) ;
#136581=CARTESIAN_POINT('Ctrl Pts',(-31.5662721684202,14.290575680997,127.932952398699)) ;
#136582=CARTESIAN_POINT('Ctrl Pts',(-31.6246390663626,14.12095115065,128.136621698187)) ;
#136583=CARTESIAN_POINT('Ctrl Pts',(-31.6658960174295,13.9018371946246,
128.290224742107)) ;
#136584=CARTESIAN_POINT('Ctrl Pts',(-31.6865228260498,13.6479071600813,
128.383641361219)) ;
#136585=CARTESIAN_POINT('Ctrl Pts',(-31.6842923198617,13.3785018299636,
128.410199122277)) ;
#136586=CARTESIAN_POINT('Ctrl Pts',(-31.6583478216367,13.1105161592094,
128.36771780606)) ;
#136587=CARTESIAN_POINT('Ctrl Pts',(-31.6104959175347,12.8677237069018,
128.260861005059)) ;
#136588=CARTESIAN_POINT('Ctrl Pts',(-31.5426928619191,12.6628308000804,
128.095983031294)) ;
#136589=CARTESIAN_POINT('Ctrl Pts',(-31.4596635073516,12.5130918940735,
127.886486535544)) ;
#136590=CARTESIAN_POINT('Ctrl Pts',(-31.3658287353506,12.4280189169956,
127.645626007363)) ;
#136591=CARTESIAN_POINT('Ctrl Pts',(-31.2683509695454,12.4146728594404,
127.393890391169)) ;
#136592=CARTESIAN_POINT('Ctrl Pts',(-31.1723757083,12.4734182584077,127.146708101578)) ;
#136593=CARTESIAN_POINT('Ctrl Pts',(-31.0846573530238,12.6005220023049,
126.923613424427)) ;
#136594=CARTESIAN_POINT('Ctrl Pts',(-31.0109368887495,12.7855010880113,
126.741250268444)) ;
#136595=CARTESIAN_POINT('Ctrl Pts',(-30.955066181992,13.0169859630547,126.611193115861)) ;
#136596=CARTESIAN_POINT('Ctrl Pts',(-30.9207893580841,13.2774552371681,
126.544188371834)) ;
#136597=CARTESIAN_POINT('Ctrl Pts',(-30.9097471402995,13.5483710343065,
126.545063201967)) ;
#136598=CARTESIAN_POINT('Ctrl Pts',(-30.9219886293322,13.810085890561,126.613924362208)) ;
#136599=CARTESIAN_POINT('Ctrl Pts',(-30.9559449844738,14.0443619160834,
126.746258785875)) ;
#136600=CARTESIAN_POINT('Ctrl Pts',(-31.008405506402,14.2339605947032,126.932620299341)) ;
#136601=CARTESIAN_POINT('Ctrl Pts',(-31.0749719859752,14.3656339160498,
127.160221612215)) ;
#136602=CARTESIAN_POINT('Ctrl Pts',(-31.1500767570186,14.429668532247,127.41275139113)) ;
#136603=CARTESIAN_POINT('Ctrl Pts',(-31.2275475074464,14.4216217933316,
127.672160409701)) ;
#136604=CARTESIAN_POINT('Ctrl Pts',(-31.3012384048704,14.3422174614337,
127.920539923313)) ;
#136605=CARTESIAN_POINT('Ctrl Pts',(-31.3652787531755,14.1963613484393,
128.140837493756)) ;
#136606=CARTESIAN_POINT('Ctrl Pts',(-31.4138953869596,13.9958156934089,
128.315925248088)) ;
#136607=CARTESIAN_POINT('Ctrl Pts',(-31.4432585655663,13.7540872313105,
128.43481729489)) ;
#136608=CARTESIAN_POINT('Ctrl Pts',(-31.450475087272,13.4887318703653,128.488999277485)) ;
#136609=CARTESIAN_POINT('Ctrl Pts',(-31.43413020577,13.217649057413,128.474486119166)) ;
#136610=CARTESIAN_POINT('Ctrl Pts',(-31.3950123680558,12.9629384688392,
128.39322410481)) ;
#136611=CARTESIAN_POINT('Ctrl Pts',(-31.3345685415584,12.7394456661168,
128.249925967071)) ;
#136612=CARTESIAN_POINT('Ctrl Pts',(-31.2573511672677,12.5666312709512,
128.057344274841)) ;
#136613=CARTESIAN_POINT('Ctrl Pts',(-31.1673288730419,12.4542159420662,
127.827511121374)) ;
#136614=CARTESIAN_POINT('Ctrl Pts',(-31.070668381057,12.4113528372628,127.57822465589)) ;
#136615=CARTESIAN_POINT('Ctrl Pts',(-30.9730874968929,12.4409689748371,
127.326366763197)) ;
#136616=CARTESIAN_POINT('Ctrl Pts',(-30.8813233211208,12.5412370844769,
127.091459318539)) ;
#136617=CARTESIAN_POINT('Ctrl Pts',(-30.8013523482404,12.7041353062448,
126.890894803477)) ;
#136618=CARTESIAN_POINT('Ctrl Pts',(-30.7377485662174,12.9183855377871,
126.738165448688)) ;
#136619=CARTESIAN_POINT('Ctrl Pts',(-30.6943522476391,13.1698655592683,
126.644607861054)) ;
#136620=CARTESIAN_POINT('Ctrl Pts',(-30.673823555151,13.4380609708233,126.617664783583)) ;
#136621=CARTESIAN_POINT('Ctrl Pts',(-30.676760958467,13.7071666218626,126.659527815916)) ;
#136622=CARTESIAN_POINT('Ctrl Pts',(-30.7021921592017,13.9538087956849,
126.766828921088)) ;
#136623=CARTESIAN_POINT('Ctrl Pts',(-30.7475911892574,14.1634526907068,
126.932575600775)) ;
#136624=CARTESIAN_POINT('Ctrl Pts',(-30.8091751138635,14.3201289730171,
127.145660569958)) ;
#136625=CARTESIAN_POINT('Ctrl Pts',(-30.8812761696098,14.4121340863402,
127.389305094501)) ;
#136626=CARTESIAN_POINT('Ctrl Pts',(-30.958733820161,14.4336855953277,127.648772839054)) ;
#136627=CARTESIAN_POINT('Ctrl Pts',(-31.0346820701722,14.3827386084068,
127.90373275799)) ;
#136628=CARTESIAN_POINT('Ctrl Pts',(-31.1034133500512,14.2627494800209,
128.137724022921)) ;
#136629=CARTESIAN_POINT('Ctrl Pts',(-31.1588772991111,14.0822577525838,
128.332935808731)) ;
#136630=CARTESIAN_POINT('Ctrl Pts',(-31.1963198264823,13.8561932154224,
128.475274428315)) ;
#136631=CARTESIAN_POINT('Ctrl Pts',(-31.2127805251386,13.5974242945969,
128.556569267893)) ;
#136632=CARTESIAN_POINT('Ctrl Pts',(-31.2060956554007,13.3273252607923,
128.570089421003)) ;
#136633=CARTESIAN_POINT('Ctrl Pts',(-31.175812020864,13.0622912163539,128.514912832323)) ;
#136634=CARTESIAN_POINT('Ctrl Pts',(-31.1240000905166,12.8256130939751,
128.396503818187)) ;
#136635=CARTESIAN_POINT('Ctrl Pts',(-31.053014393086,12.6301799024571,128.222286646203)) ;
#136636=CARTESIAN_POINT('Ctrl Pts',(-30.967517721781,12.4918476681471,128.005627111809)) ;
#136637=CARTESIAN_POINT('Ctrl Pts',(-30.8725245502937,12.4199209913987,
127.761337053555)) ;
#136638=CARTESIAN_POINT('Ctrl Pts',(-30.7744792943277,12.4204245912294,
127.50810295915)) ;
#136639=CARTESIAN_POINT('Ctrl Pts',(-30.6801950959887,12.4921595921641,
127.265646464946)) ;
#136640=CARTESIAN_POINT('Ctrl Pts',(-30.5945273226143,12.6310172827489,
127.048572948748)) ;
#136641=CARTESIAN_POINT('Ctrl Pts',(-30.5237138912385,12.8262646896106,
126.87479382954)) ;
#136642=CARTESIAN_POINT('Ctrl Pts',(-30.4717477142723,13.0646913803179,
126.756146616642)) ;
#136643=CARTESIAN_POINT('Ctrl Pts',(-30.4418079793539,13.3278244086872,
126.701716231981)) ;
#136644=CARTESIAN_POINT('Ctrl Pts',(-30.4351907633276,13.5998585157466,
126.715682786109)) ;
#136645=CARTESIAN_POINT('Ctrl Pts',(-30.4517112140757,13.8569826798842,
126.79695024305)) ;
#136646=CARTESIAN_POINT('Ctrl Pts',(-30.4894856805257,14.0842218842957,
126.940467978151)) ;
#136647=CARTESIAN_POINT('Ctrl Pts',(-30.5448536574112,14.2634335835668,
127.135250757845)) ;
#136648=CARTESIAN_POINT('Ctrl Pts',(-30.61372079861,14.3833954654661,127.369690463296)) ;
#136649=CARTESIAN_POINT('Ctrl Pts',(-30.6898267170265,14.4336980433791,
127.62516189827)) ;
#136650=CARTESIAN_POINT('Ctrl Pts',(-30.7668057003665,14.4120157811793,
127.88302690415)) ;
#136651=CARTESIAN_POINT('Ctrl Pts',(-30.8392469707509,14.3192946840505,
128.127838160812)) ;
#136652=CARTESIAN_POINT('Ctrl Pts',(-30.900587536692,14.1625583197416,128.340130750955)) ;
#136653=CARTESIAN_POINT('Ctrl Pts',(-30.9460465529525,13.9521768872698,
128.506141732049)) ;
#136654=CARTESIAN_POINT('Ctrl Pts',(-30.9712728779103,13.7045477483084,
128.612931121415)) ;
#136655=CARTESIAN_POINT('Ctrl Pts',(-30.9740973294734,13.4377490370904,
128.65416965186)) ;
#136656=CARTESIAN_POINT('Ctrl Pts',(-30.9533497435813,13.1678476255433,
128.626808748527)) ;
#136657=CARTESIAN_POINT('Ctrl Pts',(-30.9100151336481,12.9176590110113,
128.533274696295)) ;
#136658=CARTESIAN_POINT('Ctrl Pts',(-30.8460093946488,12.7025601678247,
128.379540475209)) ;
#136659=CARTESIAN_POINT('Ctrl Pts',(-30.7661541649053,12.5405894739356,
128.179214757253)) ;
#136660=CARTESIAN_POINT('Ctrl Pts',(-30.6742450321208,12.4405287609816,
127.943925123088)) ;
#136661=CARTESIAN_POINT('Ctrl Pts',(-30.5767059002742,12.4114132286229,
127.69216607229)) ;
#136662=CARTESIAN_POINT('Ctrl Pts',(-30.4801944320936,12.454644377757,127.443276439968)) ;
#136663=CARTESIAN_POINT('Ctrl Pts',(-30.3903499727896,12.5668919625006,
127.213894581398)) ;
#136664=CARTESIAN_POINT('Ctrl Pts',(-30.3126378072182,12.7415275985948,
127.020134144309)) ;
#136665=CARTESIAN_POINT('Ctrl Pts',(-30.2527609211518,12.9638992642169,
126.878266781381)) ;
#136666=CARTESIAN_POINT('Ctrl Pts',(-30.2136507437356,13.2191082193463,
126.797089063546)) ;
#136667=CARTESIAN_POINT('Ctrl Pts',(-30.1974592284486,13.4893534284064,
126.782913516033)) ;
#136668=CARTESIAN_POINT('Ctrl Pts',(-30.2047500779676,13.7553188201862,
126.837397733995)) ;
#136669=CARTESIAN_POINT('Ctrl Pts',(-30.2342451153367,13.9971251061997,
126.956700334414)) ;
#136670=CARTESIAN_POINT('Ctrl Pts',(-30.2831588596257,14.1977811038748,
127.132755162612)) ;
#136671=CARTESIAN_POINT('Ctrl Pts',(-30.346836697301,14.342451043168,127.351773566812)) ;
#136672=CARTESIAN_POINT('Ctrl Pts',(-30.421041235796,14.4220642715211,127.601876667778)) ;
#136673=CARTESIAN_POINT('Ctrl Pts',(-30.4982063681556,14.4294491071756,
127.860253341172)) ;
#136674=CARTESIAN_POINT('Ctrl Pts',(-30.5732568669214,14.3652072705711,
128.112616520929)) ;
#136675=CARTESIAN_POINT('Ctrl Pts',(-30.639714705362,14.2335292315096,128.339855798)) ;
#136676=CARTESIAN_POINT('Ctrl Pts',(-30.6922904669337,14.0429180682628,
128.526684338748)) ;
#136677=CARTESIAN_POINT('Ctrl Pts',(-30.7259826319712,13.809322141679,128.658117930451)) ;
#136678=CARTESIAN_POINT('Ctrl Pts',(-30.7382344074887,13.5476219044277,
128.727006823205)) ;
#136679=CARTESIAN_POINT('Ctrl Pts',(-30.7269403534024,13.2750712862456,
128.727347582682)) ;
#136680=CARTESIAN_POINT('Ctrl Pts',(-30.6927096810356,13.0163165161328,
128.660275654036)) ;
#136681=CARTESIAN_POINT('Ctrl Pts',(-30.6367586931873,12.7846452326426,
128.530021727058)) ;
#136682=CARTESIAN_POINT('Ctrl Pts',(-30.5628122994071,12.5995256932136,
128.347061120519)) ;
#136683=CARTESIAN_POINT('Ctrl Pts',(-30.4747613342132,12.4726551815389,
128.123086887986)) ;
#136684=CARTESIAN_POINT('Ctrl Pts',(-30.3791108848396,12.4145513483266,
127.876726073933)) ;
#136685=CARTESIAN_POINT('Ctrl Pts',(-30.2813444524036,12.428469046116,127.624255078957)) ;
#136686=CARTESIAN_POINT('Ctrl Pts',(-30.1880546184578,12.5133431382162,
127.384795540324)) ;
#136687=CARTESIAN_POINT('Ctrl Pts',(-30.1045779411166,12.664436679697,127.174213781019)) ;
#136688=CARTESIAN_POINT('Ctrl Pts',(-30.0373665693582,12.8679925136389,
127.010803548602)) ;
#136689=CARTESIAN_POINT('Ctrl Pts',(-29.9891717630807,13.1131689974074,
126.903257186694)) ;
#136690=CARTESIAN_POINT('Ctrl Pts',(-29.9635947628022,13.3800002481821,
126.861679569015)) ;
#136691=CARTESIAN_POINT('Ctrl Pts',(-29.9614886970203,13.6495651471469,
126.888635732367)) ;
#136692=CARTESIAN_POINT('Ctrl Pts',(-29.9820901647901,13.9023388794203,
126.981828620855)) ;
#136693=CARTESIAN_POINT('Ctrl Pts',(-30.0237239088706,14.122657772282,127.136756156811)) ;
#136694=CARTESIAN_POINT('Ctrl Pts',(-30.0818493827078,14.2908247523975,
127.339514451375)) ;
#136695=CARTESIAN_POINT('Ctrl Pts',(-30.1523278927941,14.3981040608109,
127.578557488567)) ;
#136696=CARTESIAN_POINT('Ctrl Pts',(-30.2293017778159,14.435262692703,127.836631386951)) ;
#136697=CARTESIAN_POINT('Ctrl Pts',(-30.3061172612986,14.3995540237045,
128.094159932593)) ;
#136698=CARTESIAN_POINT('Ctrl Pts',(-30.37646616318,14.2948938625941,128.332624943181)) ;
#136699=CARTESIAN_POINT('Ctrl Pts',(-30.4355875307391,14.1259509671256,
128.538688857853)) ;
#136700=CARTESIAN_POINT('Ctrl Pts',(-30.4771902665087,13.908522649266,128.693202393505)) ;
#136701=CARTESIAN_POINT('Ctrl Pts',(-30.4984453367561,13.6557404743469,
128.788409222222)) ;
#136702=CARTESIAN_POINT('Ctrl Pts',(-30.4969183209716,13.3866405652258,
128.817008538499)) ;
#136703=CARTESIAN_POINT('Ctrl Pts',(-30.4716526944361,13.1181024502092,
128.776531708148)) ;
#136704=CARTESIAN_POINT('Ctrl Pts',(-30.4244050237175,12.8743683126388,
128.671446151271)) ;
#136705=CARTESIAN_POINT('Ctrl Pts',(-30.3571122022536,12.667995764075,128.508067284342)) ;
#136706=CARTESIAN_POINT('Ctrl Pts',(-30.2743107927955,12.5164144284275,
128.299288210376)) ;
#136707=CARTESIAN_POINT('Ctrl Pts',(-30.181040701032,12.4295970392297,128.059953712799)) ;
#136708=CARTESIAN_POINT('Ctrl Pts',(-30.0832914972491,12.4140261285354,
127.80753264675)) ;
#136709=CARTESIAN_POINT('Ctrl Pts',(-29.9873254871061,12.4707103016775,
127.560322493363)) ;
#136710=CARTESIAN_POINT('Ctrl Pts',(-29.8992941244822,12.5959067650868,
127.336315129567)) ;
#136711=CARTESIAN_POINT('Ctrl Pts',(-29.8250863434499,12.7791141929297,
127.152509042809)) ;
#136712=CARTESIAN_POINT('Ctrl Pts',(-29.7683155464233,13.0114292224114,
127.020076886844)) ;
#136713=CARTESIAN_POINT('Ctrl Pts',(-29.7337701163823,13.2689898399713,
126.951978873228)) ;
#136714=CARTESIAN_POINT('Ctrl Pts',(-29.7219200549302,13.5409256282928,
126.950629438591)) ;
#136715=CARTESIAN_POINT('Ctrl Pts',(-29.733554311949,13.8029839862651,127.017693083378)) ;
#136716=CARTESIAN_POINT('Ctrl Pts',(-29.7669729925105,14.038560788847,127.14849808743)) ;
#136717=CARTESIAN_POINT('Ctrl Pts',(-29.8189700914752,14.2294230403712,
127.333487758985)) ;
#136718=CARTESIAN_POINT('Ctrl Pts',(-29.8850962736987,14.3627051094246,
127.559749339054)) ;
#136719=CARTESIAN_POINT('Ctrl Pts',(-29.9600740109055,14.4288334049426,
127.811925871913)) ;
#136720=CARTESIAN_POINT('Ctrl Pts',(-30.0375926178455,14.4228924634038,
128.071485668505)) ;
#136721=CARTESIAN_POINT('Ctrl Pts',(-30.1116851063149,14.3451234718206,
128.321135357699)) ;
#136722=CARTESIAN_POINT('Ctrl Pts',(-30.1759653031879,14.2008973362482,
128.542101575168)) ;
#136723=CARTESIAN_POINT('Ctrl Pts',(-30.2249348888654,14.0023960855746,
128.718117429598)) ;
#136724=CARTESIAN_POINT('Ctrl Pts',(-30.2549649553424,13.7610318696562,
128.839037447966)) ;
#136725=CARTESIAN_POINT('Ctrl Pts',(-30.2627841057998,13.4967570532622,
128.894894568641)) ;
#136726=CARTESIAN_POINT('Ctrl Pts',(-30.2472089094513,13.2257686273763,
128.882599290474)) ;
#136727=CARTESIAN_POINT('Ctrl Pts',(-30.2085846766644,12.9695426801037,
128.802889416745)) ;
#136728=CARTESIAN_POINT('Ctrl Pts',(-30.1488841254311,12.7456272140063,
128.661652559478)) ;
#136729=CARTESIAN_POINT('Ctrl Pts',(-30.072111052342,12.5709695556374,128.470385081871)) ;
#136730=CARTESIAN_POINT('Ctrl Pts',(-29.9822608788723,12.4565179199043,
128.241096280183)) ;
#136731=CARTESIAN_POINT('Ctrl Pts',(-29.8856850056017,12.4114773768948,
127.992062768051)) ;
#136732=CARTESIAN_POINT('Ctrl Pts',(-29.7876800986946,12.4394645441859,
127.739096174326)) ;
#136733=CARTESIAN_POINT('Ctrl Pts',(-29.6963815648897,12.5368906975998,
127.505279670265)) ;
#136734=CARTESIAN_POINT('Ctrl Pts',(-29.6153252716396,12.6994727132711,
127.301831679422)) ;
#136735=CARTESIAN_POINT('Ctrl Pts',(-29.5516191180179,12.911284387256,127.148596694426)) ;
#136736=CARTESIAN_POINT('Ctrl Pts',(-29.5073375465469,13.1634090150243,
127.052650475059)) ;
#136737=CARTESIAN_POINT('Ctrl Pts',(-29.4863722183674,13.43009560959,127.024270357643)) ;
#136738=CARTESIAN_POINT('Ctrl Pts',(-29.4884710007012,13.6985487058695,
127.063557018195)) ;
#136739=CARTESIAN_POINT('Ctrl Pts',(-29.5134955024387,13.9480246666546,
127.169938370698)) ;
#136740=CARTESIAN_POINT('Ctrl Pts',(-29.5581845038541,14.1576527817006,
127.333424570295)) ;
#136741=CARTESIAN_POINT('Ctrl Pts',(-29.6192793503669,14.3162850148807,
127.545072239958)) ;
#136742=CARTESIAN_POINT('Ctrl Pts',(-29.6915017728377,14.4106899860489,
127.789227708375)) ;
#136743=CARTESIAN_POINT('Ctrl Pts',(-29.7689280820927,14.4339585124651,
128.048612152318)) ;
#136744=CARTESIAN_POINT('Ctrl Pts',(-29.8446720420226,14.3853107733964,
128.302830330113)) ;
#136745=CARTESIAN_POINT('Ctrl Pts',(-29.9138779062533,14.2669554463922,
128.538293583746)) ;
#136746=CARTESIAN_POINT('Ctrl Pts',(-29.9696709434551,14.0883946272744,
128.734393104411)) ;
#136747=CARTESIAN_POINT('Ctrl Pts',(-30.0077339518895,13.8631868173472,
128.878592553755)) ;
#136748=CARTESIAN_POINT('Ctrl Pts',(-30.0248332499743,13.6057121370264,
128.961669133376)) ;
#136749=CARTESIAN_POINT('Ctrl Pts',(-30.0188186236366,13.3350529276947,
128.977231035736)) ;
#136750=CARTESIAN_POINT('Ctrl Pts',(-29.9893748969538,13.070755438595,128.924351996727)) ;
#136751=CARTESIAN_POINT('Ctrl Pts',(-29.9381198967641,12.8321487482004,
128.80767194367)) ;
#136752=CARTESIAN_POINT('Ctrl Pts',(-29.8672185952709,12.6344630496442,
128.633863552684)) ;
#136753=CARTESIAN_POINT('Ctrl Pts',(-29.7824442419727,12.4951762287069,
128.419156640686)) ;
#136754=CARTESIAN_POINT('Ctrl Pts',(-29.6878398932175,12.4210996304978,
128.175941162278)) ;
#136755=CARTESIAN_POINT('Ctrl Pts',(-29.5896845117349,12.4192964067175,
127.922422995401)) ;
#136756=CARTESIAN_POINT('Ctrl Pts',(-29.4950005569696,12.4890491878224,
127.678869190978)) ;
#136757=CARTESIAN_POINT('Ctrl Pts',(-29.4087337325941,12.6268326334366,
127.460163347604)) ;
#136758=CARTESIAN_POINT('Ctrl Pts',(-29.3378740489248,12.819583008208,127.286057249325)) ;
#136759=CARTESIAN_POINT('Ctrl Pts',(-29.2851760043964,13.0571001381562,
127.165305917233)) ;
#136760=CARTESIAN_POINT('Ctrl Pts',(-29.2545650359893,13.3202804831109,
127.108978042676)) ;
#136761=CARTESIAN_POINT('Ctrl Pts',(-29.2472402862376,13.5914915741981,
127.120763375443)) ;
#136762=CARTESIAN_POINT('Ctrl Pts',(-29.2632084846412,13.8505565623955,
127.200591332072)) ;
#136763=CARTESIAN_POINT('Ctrl Pts',(-29.3002581970792,14.0777828680815,
127.341827832713)) ;
#136764=CARTESIAN_POINT('Ctrl Pts',(-29.3552517763385,14.2590885920228,
127.535591866083)) ;
#136765=CARTESIAN_POINT('Ctrl Pts',(-29.4237488183174,14.3807166711332,
127.768911763596)) ;
#136766=CARTESIAN_POINT('Ctrl Pts',(-29.4996525428167,14.433343609964,128.023765667449)) ;
#136767=CARTESIAN_POINT('Ctrl Pts',(-29.5771911863462,14.4133893696398,
128.283487783955)) ;
#136768=CARTESIAN_POINT('Ctrl Pts',(-29.6493874448515,14.322997838196,128.527374224998)) ;
#136769=CARTESIAN_POINT('Ctrl Pts',(-29.7111985626371,14.1680350352392,
128.741068674878)) ;
#136770=CARTESIAN_POINT('Ctrl Pts',(-29.7570938139527,13.9594348156913,
128.90828666285)) ;
#136771=CARTESIAN_POINT('Ctrl Pts',(-29.7830790443061,13.7128291975183,
129.017289967226)) ;
#136772=CARTESIAN_POINT('Ctrl Pts',(-29.786491574937,13.4442543437845,129.060505529858)) ;
#136773=CARTESIAN_POINT('Ctrl Pts',(-29.7666355649697,13.1766944137287,
129.03542159918)) ;
#136774=CARTESIAN_POINT('Ctrl Pts',(-29.7235723363899,12.9234094680339,
128.942988295954)) ;
#136775=CARTESIAN_POINT('Ctrl Pts',(-29.6604602934402,12.7086523131788,
128.791635677424)) ;
#136776=CARTESIAN_POINT('Ctrl Pts',(-29.5809549544293,12.5444332770708,
128.592392030058)) ;
#136777=CARTESIAN_POINT('Ctrl Pts',(-29.4889378675449,12.442265427868,128.356904521378)) ;
#136778=CARTESIAN_POINT('Ctrl Pts',(-29.3918859003814,12.4113238221151,
128.106429463482)) ;
#136779=CARTESIAN_POINT('Ctrl Pts',(-29.2951830663714,12.4521999804418,
127.857002016351)) ;
#136780=CARTESIAN_POINT('Ctrl Pts',(-29.2045584488125,12.5635389839908,
127.625544044653)) ;
#136781=CARTESIAN_POINT('Ctrl Pts',(-29.1270346002203,12.7354102486573,
127.432082992235)) ;
#136782=CARTESIAN_POINT('Ctrl Pts',(-29.0664146932763,12.9568497903179,
127.288112348408)) ;
#136783=CARTESIAN_POINT('Ctrl Pts',(-29.026628696439,13.2117694204113,127.205005677321)) ;
#136784=CARTESIAN_POINT('Ctrl Pts',(-29.009781511419,13.4825284434545,127.188995235441)) ;
#136785=CARTESIAN_POINT('Ctrl Pts',(-29.0165029066214,13.7484828360667,
127.24177102206)) ;
#136786=CARTESIAN_POINT('Ctrl Pts',(-29.0452591215666,13.990067054495,127.358763219007)) ;
#136787=CARTESIAN_POINT('Ctrl Pts',(-29.0935118085886,14.1922208547519,
127.532848793653)) ;
#136788=CARTESIAN_POINT('Ctrl Pts',(-29.1572269990264,14.3393855053723,
127.752176269274)) ;
#136789=CARTESIAN_POINT('Ctrl Pts',(-29.2305804306216,14.42040771759,127.999501211694)) ;
#136790=CARTESIAN_POINT('Ctrl Pts',(-29.3081218951313,14.4304302239803,
128.259154471138)) ;
#136791=CARTESIAN_POINT('Ctrl Pts',(-29.3835564511664,14.3678711876826,
128.512736663744)) ;
#136792=CARTESIAN_POINT('Ctrl Pts',(-29.4503619230929,14.2376928211799,
128.741022388839)) ;
#136793=CARTESIAN_POINT('Ctrl Pts',(-29.5032308391101,14.0489884118596,
128.928618678733)) ;
#136794=CARTESIAN_POINT('Ctrl Pts',(-29.5375680722681,13.8164457415788,
129.061943923346)) ;
#136795=CARTESIAN_POINT('Ctrl Pts',(-29.5503747746567,13.5541090228178,
129.132594337899)) ;
#136796=CARTESIAN_POINT('Ctrl Pts',(-29.5399467581774,13.2846773793449,
129.135075798619)) ;
#136797=CARTESIAN_POINT('Ctrl Pts',(-29.5061893697733,13.0230236388571,
129.069677559174)) ;
#136798=CARTESIAN_POINT('Ctrl Pts',(-29.4508852278089,12.7908728134741,
128.941231892332)) ;
#136799=CARTESIAN_POINT('Ctrl Pts',(-29.3772505067172,12.6038718896903,
128.75925572478)) ;
#136800=CARTESIAN_POINT('Ctrl Pts',(-29.2898362457015,12.4755978547321,
128.537018141377)) ;
#136801=CARTESIAN_POINT('Ctrl Pts',(-29.194109143763,12.4151865518673,128.290517599109)) ;
#136802=CARTESIAN_POINT('Ctrl Pts',(-29.0964293211591,12.4270410419496,
128.038256726691)) ;
#136803=CARTESIAN_POINT('Ctrl Pts',(-29.0029243016515,12.5098502218198,
127.798170594329)) ;
#136804=CARTESIAN_POINT('Ctrl Pts',(-28.9191009602141,12.6589865553575,
127.586552482933)) ;
#136805=CARTESIAN_POINT('Ctrl Pts',(-28.8512558271298,12.8615686437882,
127.421356708522)) ;
#136806=CARTESIAN_POINT('Ctrl Pts',(-28.8025728823475,13.1050265779988,
127.31227708127)) ;
#136807=CARTESIAN_POINT('Ctrl Pts',(-28.7762486857145,13.3718443264194,
127.268571741822)) ;
#136808=CARTESIAN_POINT('Ctrl Pts',(-28.7733651472645,13.6411903783996,
127.293193753917)) ;
#136809=CARTESIAN_POINT('Ctrl Pts',(-28.7936073014881,13.896863473321,127.385643006294)) ;
#136810=CARTESIAN_POINT('Ctrl Pts',(-28.8342644907742,14.1159779541294,
127.537349449591)) ;
#136811=CARTESIAN_POINT('Ctrl Pts',(-28.8923618748685,14.287325692981,127.74029379046)) ;
#136812=CARTESIAN_POINT('Ctrl Pts',(-28.9624436618844,14.3958947357892,
127.978085746243)) ;
#136813=CARTESIAN_POINT('Ctrl Pts',(-29.0390644308761,14.435126510394,128.23502978254)) ;
#136814=CARTESIAN_POINT('Ctrl Pts',(-29.1159362844718,14.4019578679091,
128.492693840916)) ;
#136815=CARTESIAN_POINT('Ctrl Pts',(-29.1870377918795,14.298265208763,128.73360610522)) ;
#136816=CARTESIAN_POINT('Ctrl Pts',(-29.2460470592508,14.1324802055206,
128.939037898302)) ;
#136817=CARTESIAN_POINT('Ctrl Pts',(-29.288497423552,13.915462828794,129.096196593093)) ;
#136818=CARTESIAN_POINT('Ctrl Pts',(-29.3103654608126,13.663371252365,129.193190377412)) ;
#136819=CARTESIAN_POINT('Ctrl Pts',(-29.3094695407686,13.3940849584222,
129.223687381527)) ;
#136820=CARTESIAN_POINT('Ctrl Pts',(-29.2850224789087,13.1263052968225,
129.185456897491)) ;
#136821=CARTESIAN_POINT('Ctrl Pts',(-29.2381611448435,12.8804158989885,
129.08167274597)) ;
#136822=CARTESIAN_POINT('Ctrl Pts',(-29.1715363437508,12.6733663230833,
128.92014851409)) ;
#136823=CARTESIAN_POINT('Ctrl Pts',(-29.0889990041124,12.5197379443073,
128.712196434406)) ;
#136824=CARTESIAN_POINT('Ctrl Pts',(-28.9959071355212,12.4310982287018,
128.473389219666)) ;
#136825=CARTESIAN_POINT('Ctrl Pts',(-28.8984687306233,12.413462824637,128.221785958842)) ;
#136826=CARTESIAN_POINT('Ctrl Pts',(-28.8022697790058,12.4679867146693,
127.973924652651)) ;
#136827=CARTESIAN_POINT('Ctrl Pts',(-28.7137196227215,12.5916525071464,
127.748478120459)) ;
#136828=CARTESIAN_POINT('Ctrl Pts',(-28.639163277288,12.773468390421,127.563641479719)) ;
#136829=CARTESIAN_POINT('Ctrl Pts',(-28.5821237966997,13.0028687582652,
127.43018831272)) ;
#136830=CARTESIAN_POINT('Ctrl Pts',(-28.5465487884164,13.2619623581497,
127.359364860779)) ;
#136831=CARTESIAN_POINT('Ctrl Pts',(-28.534169523219,13.5340191309755,127.35648469017)) ;
#136832=CARTESIAN_POINT('Ctrl Pts',(-28.5451189938016,13.7955674320649,
127.421423522418)) ;
#136833=CARTESIAN_POINT('Ctrl Pts',(-28.5779338052964,14.0322612851413,
127.550472253615)) ;
#136834=CARTESIAN_POINT('Ctrl Pts',(-28.6293739615442,14.22438976877,127.733793431735)) ;
#136835=CARTESIAN_POINT('Ctrl Pts',(-28.6952422477354,14.3598900784348,
127.959353406453)) ;
#136836=CARTESIAN_POINT('Ctrl Pts',(-28.7704037460775,14.4280176148554,
128.212213421062)) ;
#136837=CARTESIAN_POINT('Ctrl Pts',(-28.8474474420826,14.4241023882727,
128.47017427123)) ;
#136838=CARTESIAN_POINT('Ctrl Pts',(-28.9219593848284,14.3482280503466,
128.721153256107)) ;
#136839=CARTESIAN_POINT('Ctrl Pts',(-28.9864498905584,14.206072490763,128.942653447451)) ;
#136840=CARTESIAN_POINT('Ctrl Pts',(-29.035985750403,14.008680924911,129.120380524179)) ;
#136841=CARTESIAN_POINT('Ctrl Pts',(-29.0665824887295,13.7691472453329,
129.242843957834)) ;
#136842=CARTESIAN_POINT('Ctrl Pts',(-29.0751153015166,13.5031161765621,
129.301061223738)) ;
#136843=CARTESIAN_POINT('Ctrl Pts',(-29.0600884173673,13.2327334709729,
129.290277948207)) ;
#136844=CARTESIAN_POINT('Ctrl Pts',(-29.0222348119566,12.9767767271815,
129.212705748521)) ;
#136845=CARTESIAN_POINT('Ctrl Pts',(-28.9632320010006,12.7518157779669,
129.073464224787)) ;
#136846=CARTESIAN_POINT('Ctrl Pts',(-28.8865689011726,12.5749030821108,
128.882657897678)) ;
#136847=CARTESIAN_POINT('Ctrl Pts',(-28.7971500754483,12.4587258790909,
128.654567687979)) ;
#136848=CARTESIAN_POINT('Ctrl Pts',(-28.7001805984422,12.4118884075951,
128.40456104214)) ;
#136849=CARTESIAN_POINT('Ctrl Pts',(-28.6034625867503,12.4371447896242,
128.154880032499)) ;
#136850=CARTESIAN_POINT('Ctrl Pts',(-28.5108176103101,12.5335140110472,
127.917531270634)) ;
#136851=CARTESIAN_POINT('Ctrl Pts',(-28.4300750917707,12.6929505579163,
127.714687315915)) ;
#136852=CARTESIAN_POINT('Ctrl Pts',(-28.3652170696654,12.9053983605441,
127.558411095435)) ;
#136853=CARTESIAN_POINT('Ctrl Pts',(-28.320776308873,13.1539498809503,127.461624968063)) ;
#136854=CARTESIAN_POINT('Ctrl Pts',(-28.298797481994,13.4226750852024,127.430585596952)) ;
#136855=CARTESIAN_POINT('Ctrl Pts',(-28.3003278552427,13.6910891488428,
127.468168994763)) ;
#136856=CARTESIAN_POINT('Ctrl Pts',(-28.3246858188287,13.9413684449187,
127.57259757245)) ;
#136857=CARTESIAN_POINT('Ctrl Pts',(-28.3689739237031,14.1526799175884,
127.734981003135)) ;
#136858=CARTESIAN_POINT('Ctrl Pts',(-28.4295901071815,14.3125333365339,
127.945168675357)) ;
#136859=CARTESIAN_POINT('Ctrl Pts',(-28.5013420399729,14.4088194545048,
128.187852724351)) ;
#136860=CARTESIAN_POINT('Ctrl Pts',(-28.5789855165237,14.4343198922647,
128.447994052582)) ;
#136861=CARTESIAN_POINT('Ctrl Pts',(-28.6547069342175,14.3877722216923,
128.702080644945)) ;
#136862=CARTESIAN_POINT('Ctrl Pts',(-28.7242795531825,14.2711471229662,
128.938658704747)) ;
#136863=CARTESIAN_POINT('Ctrl Pts',(-28.7802793365346,14.0951743050547,
129.135196568692)) ;
#136864=CARTESIAN_POINT('Ctrl Pts',(-28.819161267005,13.870335406886,129.281932862346)) ;
#136865=CARTESIAN_POINT('Ctrl Pts',(-28.8368809389887,13.6128359937758,
129.366896771082)) ;
#136866=CARTESIAN_POINT('Ctrl Pts',(-28.8315194560845,13.3431053830175,
129.384270113394)) ;
#136867=CARTESIAN_POINT('Ctrl Pts',(-28.8028631485192,13.0784070527184,
129.333670117737)) ;
#136868=CARTESIAN_POINT('Ctrl Pts',(-28.7516974964307,12.8371326222925,
129.217513861175)) ;
#136869=CARTESIAN_POINT('Ctrl Pts',(-28.6819104589447,12.6399916348322,
129.04664441349)) ;
#136870=CARTESIAN_POINT('Ctrl Pts',(-28.5970929224664,12.4979353055065,
128.83198887352)) ;
#136871=CARTESIAN_POINT('Ctrl Pts',(-28.5024370244011,12.4220838760127,
128.588688477948)) ;
#136872=CARTESIAN_POINT('Ctrl Pts',(-28.4044917843163,12.4184701174221,
128.335717148348)) ;
#136873=CARTESIAN_POINT('Ctrl Pts',(-28.3099706653344,12.4860424298892,
128.092527425312)) ;
#136874=CARTESIAN_POINT('Ctrl Pts',(-28.223574515994,12.6212969688775,127.873340879876)) ;
#136875=CARTESIAN_POINT('Ctrl Pts',(-28.1518306616533,12.8133838986541,
127.69681361212)) ;
#136876=CARTESIAN_POINT('Ctrl Pts',(-28.0985302457413,13.0503648242526,
127.574351579876)) ;
#136877=CARTESIAN_POINT('Ctrl Pts',(-28.0673717372715,13.3123036510868,
127.516329514673)) ;
#136878=CARTESIAN_POINT('Ctrl Pts',(-28.0593362748271,13.583277796962,127.526004293595)) ;
#136879=CARTESIAN_POINT('Ctrl Pts',(-28.074579667337,13.8428842825667,127.603695842468)) ;
#136880=CARTESIAN_POINT('Ctrl Pts',(-28.1111583249458,14.0720012464851,
127.743661870436)) ;
#136881=CARTESIAN_POINT('Ctrl Pts',(-28.1656930951673,14.2546155052048,
127.936063605963)) ;
#136882=CARTESIAN_POINT('Ctrl Pts',(-28.2336890692285,14.3779471220683,
128.167835790675)) ;
#136883=CARTESIAN_POINT('Ctrl Pts',(-28.3095549362229,14.43277854508,128.422626942245)) ;
#136884=CARTESIAN_POINT('Ctrl Pts',(-28.3868885672699,14.415204860474,128.681637758062)) ;
#136885=CARTESIAN_POINT('Ctrl Pts',(-28.4596630946583,14.3266409888288,
128.927362056089)) ;
#136886=CARTESIAN_POINT('Ctrl Pts',(-28.5219364510198,14.1729215219676,
129.142467156732)) ;
#136887=CARTESIAN_POINT('Ctrl Pts',(-28.5681998414333,13.9662155734193,
129.310666589753)) ;
#136888=CARTESIAN_POINT('Ctrl Pts',(-28.5948212406952,13.7208187019913,
129.421494134839)) ;
#136889=CARTESIAN_POINT('Ctrl Pts',(-28.5989652050376,13.4521886901424,
129.466894357061)) ;
#136890=CARTESIAN_POINT('Ctrl Pts',(-28.5796745440176,13.1838897555981,
129.443530441394)) ;
#136891=CARTESIAN_POINT('Ctrl Pts',(-28.5375432029936,12.9313138708941,
129.353617345095)) ;
#136892=CARTESIAN_POINT('Ctrl Pts',(-28.4748147134164,12.7142071151624,
129.203518501486)) ;
#136893=CARTESIAN_POINT('Ctrl Pts',(-28.3955037882874,12.548182284736,129.004911407026)) ;
#136894=CARTESIAN_POINT('Ctrl Pts',(-28.3042662810769,12.4445945488069,
128.771517428537)) ;
#136895=CARTESIAN_POINT('Ctrl Pts',(-28.2072142920676,12.4110615295413,
128.521074478556)) ;
#136896=CARTESIAN_POINT('Ctrl Pts',(-28.109954279377,12.4502003407784,128.270178669755)) ;
#136897=CARTESIAN_POINT('Ctrl Pts',(-28.0196765282693,12.558798155004,128.039502633665)) ;
#136898=CARTESIAN_POINT('Ctrl Pts',(-27.9414026174185,12.7290992906361,
127.843940992415)) ;
#136899=CARTESIAN_POINT('Ctrl Pts',(-27.8799523087916,12.9505642772134,
127.697713789602)) ;
#136900=CARTESIAN_POINT('Ctrl Pts',(-27.8397310330826,13.2039533601212,
127.613220973736)) ;
#136901=CARTESIAN_POINT('Ctrl Pts',(-27.8221719989325,13.4737768024146,
127.59504291459)) ;
#136902=CARTESIAN_POINT('Ctrl Pts',(-27.828142978279,13.7408243075777,127.645702023097)) ;
#136903=CARTESIAN_POINT('Ctrl Pts',(-27.8565009523758,13.984382806197,127.761690204667)) ;
#136904=CARTESIAN_POINT('Ctrl Pts',(-27.904026451956,14.1867700036955,127.933475703758)) ;
#136905=CARTESIAN_POINT('Ctrl Pts',(-27.9674069988023,14.3360222992997,
128.151866633947)) ;
#136906=CARTESIAN_POINT('Ctrl Pts',(-28.0405654232842,14.419030482185,128.398621922666)) ;
#136907=CARTESIAN_POINT('Ctrl Pts',(-28.1180655766905,14.4311357445316,
128.658152500593)) ;
#136908=CARTESIAN_POINT('Ctrl Pts',(-28.1935404493141,14.3708888244175,
128.91179298057)) ;
#136909=CARTESIAN_POINT('Ctrl Pts',(-28.2607936473277,14.242292745065,129.141455567403)) ;
#136910=CARTESIAN_POINT('Ctrl Pts',(-28.3139374658551,14.0562620175223,
129.329683129342)) ;
#136911=CARTESIAN_POINT('Ctrl Pts',(-28.3491506733618,13.8231737937943,
129.465813554896)) ;
#136912=CARTESIAN_POINT('Ctrl Pts',(-28.3625271445841,13.5622217788933,
129.538011618253)) ;
#136913=CARTESIAN_POINT('Ctrl Pts',(-28.3527809549952,13.2923511462151,
129.542545200143)) ;
#136914=CARTESIAN_POINT('Ctrl Pts',(-28.3197908030112,13.0307857162003,
129.479299324232)) ;
#136915=CARTESIAN_POINT('Ctrl Pts',(-28.2649022282346,12.7967159869363,
129.352185243173)) ;
#136916=CARTESIAN_POINT('Ctrl Pts',(-28.1917552814469,12.6083943270826,
129.171610865605)) ;
#136917=CARTESIAN_POINT('Ctrl Pts',(-28.1045726910697,12.4782667432663,
128.950081296167)) ;
#136918=CARTESIAN_POINT('Ctrl Pts',(-28.0093162223049,12.4160107733854,
128.704845792822)) ;
#136919=CARTESIAN_POINT('Ctrl Pts',(-27.9113561678863,12.425588900326,128.451849759996)) ;
#136920=CARTESIAN_POINT('Ctrl Pts',(-27.8173088069426,12.5070742961233,
128.210311026811)) ;
#136921=CARTESIAN_POINT('Ctrl Pts',(-27.7335650904484,12.6538727227807,
127.998759420859)) ;
#136922=CARTESIAN_POINT('Ctrl Pts',(-27.6650837722555,12.8553498973186,
127.831762310882)) ;
#136923=CARTESIAN_POINT('Ctrl Pts',(-27.615801809689,13.0981033261267,127.720951140335)) ;
#136924=CARTESIAN_POINT('Ctrl Pts',(-27.58884476403,13.3649637765944,127.675446327313)) ;
#136925=CARTESIAN_POINT('Ctrl Pts',(-27.5853834682543,13.6334093866667,
127.698255596654)) ;
#136926=CARTESIAN_POINT('Ctrl Pts',(-27.6047690706477,13.8886868084012,
127.78804071139)) ;
#136927=CARTESIAN_POINT('Ctrl Pts',(-27.6450492586127,14.1104518117265,
127.938840818448)) ;
#136928=CARTESIAN_POINT('Ctrl Pts',(-27.7027415775045,14.2832226170572,
128.140591352709)) ;
#136929=CARTESIAN_POINT('Ctrl Pts',(-27.7725050879397,14.3937886197238,
128.377439933488)) ;
#136930=CARTESIAN_POINT('Ctrl Pts',(-27.8493794925505,14.4350213819736,
128.635274356798)) ;
#136931=CARTESIAN_POINT('Ctrl Pts',(-27.9259608175934,14.4038716569565,
128.891931541062)) ;
#136932=CARTESIAN_POINT('Ctrl Pts',(-27.9974403274595,14.3020574397598,
129.134001140412)) ;
#136933=CARTESIAN_POINT('Ctrl Pts',(-28.0568366490592,14.1377082667359,
129.340572157127)) ;
#136934=CARTESIAN_POINT('Ctrl Pts',(-28.0997330529527,13.922512079821,129.498952043521)) ;
#136935=CARTESIAN_POINT('Ctrl Pts',(-28.1222933683625,13.6705375109782,
129.598054557402)) ;
#136936=CARTESIAN_POINT('Ctrl Pts',(-28.1220048988863,13.4018845306058,
129.630275138781)) ;
#136937=CARTESIAN_POINT('Ctrl Pts',(-28.0983744340301,13.1344381767143,
129.594340562343)) ;
#136938=CARTESIAN_POINT('Ctrl Pts',(-28.05188015388,12.8864833216457,129.491795996965)) ;
#136939=CARTESIAN_POINT('Ctrl Pts',(-27.9861062755655,12.6791960458196,
129.332582797579)) ;
#136940=CARTESIAN_POINT('Ctrl Pts',(-27.9038435542885,12.5233811558849,
129.125499147987)) ;
#136941=CARTESIAN_POINT('Ctrl Pts',(-27.8111043969776,12.4327816680599,
128.887676707755)) ;
#136942=CARTESIAN_POINT('Ctrl Pts',(-27.7134087891038,12.412915954978,128.635426708969)) ;
#136943=CARTESIAN_POINT('Ctrl Pts',(-27.6171947184772,12.4655032606852,
128.387484215435)) ;
#136944=CARTESIAN_POINT('Ctrl Pts',(-27.528620482135,12.5866528980437,128.161850174214)) ;
#136945=CARTESIAN_POINT('Ctrl Pts',(-27.4532574084139,12.7674395130523,
127.974785517744)) ;
#136946=CARTESIAN_POINT('Ctrl Pts',(-27.3955179677537,12.996680662144,127.839402986817)) ;
#136947=CARTESIAN_POINT('Ctrl Pts',(-27.3595338870752,13.2541240952596,
127.767245304833)) ;
#136948=CARTESIAN_POINT('Ctrl Pts',(-27.3464077619685,13.5248420441081,
127.762028996665)) ;
#136949=CARTESIAN_POINT('Ctrl Pts',(-27.356666975349,13.7882270430707,127.825112744732)) ;
#136950=CARTESIAN_POINT('Ctrl Pts',(-27.3889352588637,14.026098281457,127.952588217587)) ;
#136951=CARTESIAN_POINT('Ctrl Pts',(-27.4400200252131,14.220023125983,128.134939040121)) ;
#136952=CARTESIAN_POINT('Ctrl Pts',(-27.5054425779506,14.3567721922805,
128.359124707489)) ;
#136953=CARTESIAN_POINT('Ctrl Pts',(-27.5799717340147,14.4269174319569,
128.609946622311)) ;
#136954=CARTESIAN_POINT('Ctrl Pts',(-27.6576169156365,14.4252573107259,
128.869919222744)) ;
#136955=CARTESIAN_POINT('Ctrl Pts',(-27.7321017988657,14.3512845156984,
129.120733211293)) ;
#136956=CARTESIAN_POINT('Ctrl Pts',(-27.7967359453251,14.2117350890935,
129.342525302038)) ;
#136957=CARTESIAN_POINT('Ctrl Pts',(-27.8470386906761,14.0152549017169,
129.52261496323)) ;
#136958=CARTESIAN_POINT('Ctrl Pts',(-27.8782495117232,13.7756400409677,
129.646998433737)) ;
#136959=CARTESIAN_POINT('Ctrl Pts',(-27.8873911313969,13.512293601297,129.706715524423)) ;
#136960=CARTESIAN_POINT('Ctrl Pts',(-27.8731583548882,13.24113011058,129.698336607786)) ;
#136961=CARTESIAN_POINT('Ctrl Pts',(-27.8359087024829,12.9839533998787,
129.622589483103)) ;
#136962=CARTESIAN_POINT('Ctrl Pts',(-27.7772389969083,12.757224045122,129.484428783906)) ;
#136963=CARTESIAN_POINT('Ctrl Pts',(-27.7013420867903,12.5794741736853,
129.295717193307)) ;
#136964=CARTESIAN_POINT('Ctrl Pts',(-27.61199789567,12.4611210903509,129.067932649301)) ;
#136965=CARTESIAN_POINT('Ctrl Pts',(-27.5156597037437,12.4122668276836,
128.819593542146)) ;
#136966=CARTESIAN_POINT('Ctrl Pts',(-27.4181724680739,12.4354395008957,
128.567907202221)) ;
#136967=CARTESIAN_POINT('Ctrl Pts',(-27.325352341727,12.5301694700227,128.330034016627)) ;
#136968=CARTESIAN_POINT('Ctrl Pts',(-27.2444119944152,12.6876686468163,
128.126545747607)) ;
#136969=CARTESIAN_POINT('Ctrl Pts',(-27.1791191129236,12.8982124507683,
127.968922538508)) ;
#136970=CARTESIAN_POINT('Ctrl Pts',(-27.1338326861557,13.1472879171854,
127.869844817616)) ;
#136971=CARTESIAN_POINT('Ctrl Pts',(-27.1113227512545,13.4151706330379,
127.837176477762)) ;
#136972=CARTESIAN_POINT('Ctrl Pts',(-27.1121984761234,13.6833052761831,
127.872788487339)) ;
#136973=CARTESIAN_POINT('Ctrl Pts',(-27.1357131249715,13.9335262221531,
127.97461183381)) ;
#136974=CARTESIAN_POINT('Ctrl Pts',(-27.1798239658889,14.1479664879784,
128.136760203425)) ;
#136975=CARTESIAN_POINT('Ctrl Pts',(-27.2399210422133,14.3087959148104,
128.345327481302)) ;
#136976=CARTESIAN_POINT('Ctrl Pts',(-27.3114169111032,14.4069520206095,
128.58726493726)) ;
#136977=CARTESIAN_POINT('Ctrl Pts',(-27.38862876507,14.4347039368911,128.845984629067)) ;
#136978=CARTESIAN_POINT('Ctrl Pts',(-27.4649895003704,14.3899170830749,
129.10217320422)) ;
#136979=CARTESIAN_POINT('Ctrl Pts',(-27.5344215210273,14.2758481997907,
129.338132040779)) ;
#136980=CARTESIAN_POINT('Ctrl Pts',(-27.5911283659314,14.1010294693846,
129.536862778471)) ;
#136981=CARTESIAN_POINT('Ctrl Pts',(-27.6305468417763,13.8772034754541,
129.685173590359)) ;
#136982=CARTESIAN_POINT('Ctrl Pts',(-27.6488943694278,13.6206147826081,
129.771944550201)) ;
#136983=CARTESIAN_POINT('Ctrl Pts',(-27.6442384536181,13.3509222115741,
129.791386599852)) ;
#136984=CARTESIAN_POINT('Ctrl Pts',(-27.616132866257,13.0853829719641,129.742455025968)) ;
#136985=CARTESIAN_POINT('Ctrl Pts',(-27.5659241263139,12.8445476848772,
129.628889117042)) ;
#136986=CARTESIAN_POINT('Ctrl Pts',(-27.4964177152632,12.644952930344,129.458978943419)) ;
#136987=CARTESIAN_POINT('Ctrl Pts',(-27.4119515874544,12.5012606918104,
129.245340538602)) ;
#136988=CARTESIAN_POINT('Ctrl Pts',(-27.3178276586184,12.4235056732711,
129.003484340073)) ;
#136989=CARTESIAN_POINT('Ctrl Pts',(-27.2198616603803,12.417318606479,128.750460970837)) ;
#136990=CARTESIAN_POINT('Ctrl Pts',(-27.1245890090358,12.4833714427519,
128.505283372717)) ;
#136991=CARTESIAN_POINT('Ctrl Pts',(-27.0382770555464,12.6162285125256,
128.286182494922)) ;
#136992=CARTESIAN_POINT('Ctrl Pts',(-26.9657884587366,12.8073409623945,
128.107588748283)) ;
#136993=CARTESIAN_POINT('Ctrl Pts',(-26.91197273339,13.0432164497969,127.983598029365)) ;
#136994=CARTESIAN_POINT('Ctrl Pts',(-26.8801365095611,13.3046948495717,
127.923605110898)) ;
#136995=CARTESIAN_POINT('Ctrl Pts',(-26.8714475726995,13.5764462618644,
127.931458802618)) ;
#136996=CARTESIAN_POINT('Ctrl Pts',(-26.8861390506494,13.8363549423102,
128.007514684919)) ;
#136997=CARTESIAN_POINT('Ctrl Pts',(-26.9219756410579,14.0655921172455,
128.14516922602)) ;
#136998=CARTESIAN_POINT('Ctrl Pts',(-26.9761724713165,14.2503953829721,
128.3366792907)) ;
#136999=CARTESIAN_POINT('Ctrl Pts',(-27.0441067566407,14.3757153759899,
128.568369328025)) ;
#137000=CARTESIAN_POINT('Ctrl Pts',(-27.119708134456,14.4321659861442,128.822325410149)) ;
#137001=CARTESIAN_POINT('Ctrl Pts',(-27.1968293833805,14.4167343147861,
129.08060826829)) ;
#137002=CARTESIAN_POINT('Ctrl Pts',(-27.2698051782105,14.3302900075088,
129.326910391088)) ;
#137003=CARTESIAN_POINT('Ctrl Pts',(-27.3325244628476,14.1784243814557,
129.543326387964)) ;
#137004=CARTESIAN_POINT('Ctrl Pts',(-27.3795172134242,13.971750794682,129.713846487644)) ;
#137005=CARTESIAN_POINT('Ctrl Pts',(-27.4065121003142,13.7284357059757,
129.825586303865)) ;
#137006=CARTESIAN_POINT('Ctrl Pts',(-27.411442494474,13.4606302027768,129.873232722216)) ;
#137007=CARTESIAN_POINT('Ctrl Pts',(-27.3926620627969,13.190619216966,129.851547306682)) ;
#137008=CARTESIAN_POINT('Ctrl Pts',(-27.3513990743719,12.9388679934988,
129.763965154305)) ;
#137009=CARTESIAN_POINT('Ctrl Pts',(-27.2890472382881,12.7195132188822,
129.615095019132)) ;
#137010=CARTESIAN_POINT('Ctrl Pts',(-27.2099509779105,12.5518557366653,
129.417169431718)) ;
#137011=CARTESIAN_POINT('Ctrl Pts',(-27.1194048865831,12.4467157565619,
129.185641424037)) ;
#137012=CARTESIAN_POINT('Ctrl Pts',(-27.0218870634375,12.4110145774925,
128.934027986269)) ;
#137013=CARTESIAN_POINT('Ctrl Pts',(-26.9251985270549,12.4479828352211,
128.684575244082)) ;
#137014=CARTESIAN_POINT('Ctrl Pts',(-26.8344156748515,12.5544308126574,
128.452487217202)) ;
#137015=CARTESIAN_POINT('Ctrl Pts',(-26.7552540847317,12.7245572127077,
128.254559235342)) ;
#137016=CARTESIAN_POINT('Ctrl Pts',(-26.6937193015478,12.9435039801677,
128.107866481436)) ;
#137017=CARTESIAN_POINT('Ctrl Pts',(-26.6527533456264,13.1965754196772,
128.021262076669)) ;
#137018=CARTESIAN_POINT('Ctrl Pts',(-26.6345818546693,13.4658054148295,
128.001239973814)) ;
#137019=CARTESIAN_POINT('Ctrl Pts',(-26.6398440618961,13.7328709435355,
128.049786254539)) ;
#137020=CARTESIAN_POINT('Ctrl Pts',(-26.6674841230862,13.9772572574738,
128.163645532069)) ;
#137021=CARTESIAN_POINT('Ctrl Pts',(-26.7147375930126,14.1820528886268,
128.33480544544)) ;
#137022=CARTESIAN_POINT('Ctrl Pts',(-26.7777583985121,14.3328843450188,
128.552131428521)) ;
#137023=CARTESIAN_POINT('Ctrl Pts',(-26.8509440034052,14.4178010956835,
128.799064816972)) ;
#137024=CARTESIAN_POINT('Ctrl Pts',(-26.9280312466132,14.4318123970992,
129.057219724161)) ;
#137025=CARTESIAN_POINT('Ctrl Pts',(-27.0039631337358,14.3732303174577,
129.312341756014)) ;
#137026=CARTESIAN_POINT('Ctrl Pts',(-27.0711704740135,14.246970367672,129.541698456142)) ;
#137027=CARTESIAN_POINT('Ctrl Pts',(-27.1249090976529,14.0621465768449,
129.731735704159)) ;
#137028=CARTESIAN_POINT('Ctrl Pts',(-27.1606059412427,13.8305008090445,
129.869217691575)) ;
#137029=CARTESIAN_POINT('Ctrl Pts',(-27.1746889753248,13.5704782336575,
129.943442839551)) ;
#137030=CARTESIAN_POINT('Ctrl Pts',(-27.1655792705688,13.2994607453498,
129.949975686195)) ;
#137031=CARTESIAN_POINT('Ctrl Pts',(-27.133176892415,13.0377344275702,129.888411790656)) ;
#137032=CARTESIAN_POINT('Ctrl Pts',(-27.0791944720116,12.8036246677019,
129.763785021152)) ;
#137033=CARTESIAN_POINT('Ctrl Pts',(-27.0062821178587,12.6130123925856,
129.58402121372)) ;
#137034=CARTESIAN_POINT('Ctrl Pts',(-26.9196663424445,12.4813447985494,
129.364056212953)) ;
#137035=CARTESIAN_POINT('Ctrl Pts',(-26.8242420692028,12.4167223946536,
129.118448864076)) ;
#137036=CARTESIAN_POINT('Ctrl Pts',(-26.7263952125267,12.4243655838416,
128.865737206127)) ;
#137037=CARTESIAN_POINT('Ctrl Pts',(-26.6324009307372,12.5034382504578,
128.624259769196)) ;
#137038=CARTESIAN_POINT('Ctrl Pts',(-26.5481314271763,12.6484425830615,
128.411216523542)) ;
#137039=CARTESIAN_POINT('Ctrl Pts',(-26.4789570120788,12.8490571219356,
128.242281700259)) ;
#137040=CARTESIAN_POINT('Ctrl Pts',(-26.4291671135027,13.0907448949446,
128.129961496988)) ;
#137041=CARTESIAN_POINT('Ctrl Pts',(-26.4015577929671,13.3559777711551,
128.082404456019)) ;
#137042=CARTESIAN_POINT('Ctrl Pts',(-26.3973692775735,13.6264772467065,
128.103324558719)) ;
#137043=CARTESIAN_POINT('Ctrl Pts',(-26.4161290926396,13.8815733250424,
128.191173426764)) ;
#137044=CARTESIAN_POINT('Ctrl Pts',(-26.4558018566002,14.1045282295606,
128.340192241249)) ;
#137045=CARTESIAN_POINT('Ctrl Pts',(-26.5130348991941,14.2789670310199,
128.540593076948)) ;
#137046=CARTESIAN_POINT('Ctrl Pts',(-26.5826080859745,14.3914951662386,
128.776928435221)) ;
#137047=CARTESIAN_POINT('Ctrl Pts',(-26.6590559552618,14.4348607606962,
129.033377878272)) ;
#137048=CARTESIAN_POINT('Ctrl Pts',(-26.7361279143954,14.4056890546892,
129.291651441273)) ;
#137049=CARTESIAN_POINT('Ctrl Pts',(-26.807530292351,14.3062653173801,129.533337989376)) ;
#137050=CARTESIAN_POINT('Ctrl Pts',(-26.8674978374188,14.1434405254574,
129.741649803858)) ;
#137051=CARTESIAN_POINT('Ctrl Pts',(-26.9109484293722,13.9296996080406,
129.901626502744)) ;
#137052=CARTESIAN_POINT('Ctrl Pts',(-26.9342104512912,13.6772902050266,
130.002938697121)) ;
#137053=CARTESIAN_POINT('Ctrl Pts',(-26.9345509523393,13.4099497148623,
130.036858568768)) ;
#137054=CARTESIAN_POINT('Ctrl Pts',(-26.911574948467,13.1418739584321,130.002879415227)) ;
#137055=CARTESIAN_POINT('Ctrl Pts',(-26.8659145129542,12.8939990940818,
129.90263809472)) ;
#137056=CARTESIAN_POINT('Ctrl Pts',(-26.8005350813149,12.6844791174551,
129.744684127644)) ;
#137057=CARTESIAN_POINT('Ctrl Pts',(-26.7182272801976,12.5265062887792,
129.537620729892)) ;
#137058=CARTESIAN_POINT('Ctrl Pts',(-26.6261818479671,12.4345049990361,
129.301652381516)) ;
#137059=CARTESIAN_POINT('Ctrl Pts',(-26.5282261254205,12.4124896095147,
129.04875220205)) ;
#137060=CARTESIAN_POINT('Ctrl Pts',(-26.4322917120542,12.4629154785975,
128.801487434298)) ;
#137061=CARTESIAN_POINT('Ctrl Pts',(-26.3432251854872,12.5820912201831,
128.574467292554)) ;
#137062=CARTESIAN_POINT('Ctrl Pts',(-26.2671581421373,12.7624371254393,
128.385498413564)) ;
#137063=CARTESIAN_POINT('Ctrl Pts',(-26.2094237671192,12.9881391647597,
128.249786258131)) ;
#137064=CARTESIAN_POINT('Ctrl Pts',(-26.1724245557909,13.2462582186001,
128.174853451086)) ;
#137065=CARTESIAN_POINT('Ctrl Pts',(-26.1586794395876,13.5176870879671,
128.167919605747)) ;
#137066=CARTESIAN_POINT('Ctrl Pts',(-26.1682601316726,13.7805943652363,
128.228904238184)) ;
#137067=CARTESIAN_POINT('Ctrl Pts',(-26.1998860836901,14.0195268693382,
128.35450332008)) ;
#137068=CARTESIAN_POINT('Ctrl Pts',(-26.2504691063118,14.2150384579935,
128.535393340333)) ;
#137069=CARTESIAN_POINT('Ctrl Pts',(-26.3156944845117,14.3538332405852,
128.759076824619)) ;
#137070=CARTESIAN_POINT('Ctrl Pts',(-26.3899618416788,14.4259646788893,
129.009091256447)) ;
#137071=CARTESIAN_POINT('Ctrl Pts',(-26.4678956866111,14.4260802935488,
129.270038211653)) ;
#137072=CARTESIAN_POINT('Ctrl Pts',(-26.5418878654518,14.3549351031628,
129.519100877499)) ;
#137073=CARTESIAN_POINT('Ctrl Pts',(-26.6074625898789,14.2162529727103,
129.743922519442)) ;
#137074=CARTESIAN_POINT('Ctrl Pts',(-26.6580452321054,14.0213157651239,
129.924758738153)) ;
#137075=CARTESIAN_POINT('Ctrl Pts',(-26.6898532286372,13.7835943457729,
130.050782470753)) ;
#137076=CARTESIAN_POINT('Ctrl Pts',(-26.6996483276662,13.5186609566866,
130.112664324409)) ;
#137077=CARTESIAN_POINT('Ctrl Pts',(-26.6861549241806,13.2494163240999,
130.106191722595)) ;
#137078=CARTESIAN_POINT('Ctrl Pts',(-26.6493702443734,12.9903692068144,
130.031973073397)) ;
#137079=CARTESIAN_POINT('Ctrl Pts',(-26.591620486111,12.7636901200826,129.896303906618)) ;
#137080=CARTESIAN_POINT('Ctrl Pts',(-26.5154518565401,12.5829314316244,
129.707103805501)) ;
#137081=CARTESIAN_POINT('Ctrl Pts',(-26.4273296697944,12.4640788592141,
129.482529198083)) ;
#137082=CARTESIAN_POINT('Ctrl Pts',(-26.3305930618283,12.4125693600516,
129.233221648972)) ;
#137083=CARTESIAN_POINT('Ctrl Pts',(-26.2333657019323,12.433709410136,128.982182141248)) ;
#137084=CARTESIAN_POINT('Ctrl Pts',(-26.1402024934681,12.5263145122891,
128.743340215982)) ;
#137085=CARTESIAN_POINT('Ctrl Pts',(-26.0587798870192,12.682258725893,128.538473987008)) ;
#137086=CARTESIAN_POINT('Ctrl Pts',(-25.9929595121332,12.8915625393506,
128.379320359343)) ;
#137087=CARTESIAN_POINT('Ctrl Pts',(-25.9470977802172,13.1392602988437,
128.278495272757)) ;
#137088=CARTESIAN_POINT('Ctrl Pts',(-25.923848945908,13.4076118605944,128.243769009844)) ;
#137089=CARTESIAN_POINT('Ctrl Pts',(-25.9240227025973,13.6757335665798,
128.277286286111)) ;
#137090=CARTESIAN_POINT('Ctrl Pts',(-25.9471968230485,13.9281677275871,
128.378335497117)) ;
#137091=CARTESIAN_POINT('Ctrl Pts',(-25.9901765099646,14.1410411517753,
128.536727728813)) ;
#137092=CARTESIAN_POINT('Ctrl Pts',(-26.0502174839161,14.305185990512,128.745389721773)) ;
#137093=CARTESIAN_POINT('Ctrl Pts',(-26.1214648073103,14.4050577723151,
128.98657892307)) ;
#137094=CARTESIAN_POINT('Ctrl Pts',(-26.1986808777145,14.4349188595374,
129.24534957222)) ;
#137095=CARTESIAN_POINT('Ctrl Pts',(-26.2750125302576,14.3922309403959,
129.501391075404)) ;
#137096=CARTESIAN_POINT('Ctrl Pts',(-26.3447157195158,14.2801808361509,
129.738135053733)) ;
#137097=CARTESIAN_POINT('Ctrl Pts',(-26.4019169360842,14.1070360328529,
129.938316871328)) ;
#137098=CARTESIAN_POINT('Ctrl Pts',(-26.442001427727,13.8833119932821,130.088719159854)) ;
#137099=CARTESIAN_POINT('Ctrl Pts',(-26.4608722515451,13.6288342780485,
130.176828146041)) ;
#137100=CARTESIAN_POINT('Ctrl Pts',(-26.4568988722014,13.3582466690145,
130.198396750865)) ;
#137101=CARTESIAN_POINT('Ctrl Pts',(-26.4295097212651,13.0930922580285,
130.151455564506)) ;
#137102=CARTESIAN_POINT('Ctrl Pts',(-26.3798739225849,12.8509541830077,
130.03960846532)) ;
#137103=CARTESIAN_POINT('Ctrl Pts',(-26.3109011279355,12.6500625833759,
129.871238266472)) ;
#137104=CARTESIAN_POINT('Ctrl Pts',(-26.2266721288439,12.504322047528,129.658344470603)) ;
#137105=CARTESIAN_POINT('Ctrl Pts',(-26.1325625349995,12.4246931678785,
129.41658611775)) ;
#137106=CARTESIAN_POINT('Ctrl Pts',(-26.0351158553051,12.416496187653,129.164910619629)) ;
#137107=CARTESIAN_POINT('Ctrl Pts',(-25.9396110218934,12.4802513742885,
128.919072246389)) ;
#137108=CARTESIAN_POINT('Ctrl Pts',(-25.852731120451,12.6116452281821,128.698399944407)) ;
#137109=CARTESIAN_POINT('Ctrl Pts',(-25.7798786336614,12.8011771463769,
128.518710754517)) ;
#137110=CARTESIAN_POINT('Ctrl Pts',(-25.7255934891361,13.0350449035092,
128.393230108689)) ;
#137111=CARTESIAN_POINT('Ctrl Pts',(-25.6929390835032,13.2969779492496,
128.330976980489)) ;
#137112=CARTESIAN_POINT('Ctrl Pts',(-25.6836018345808,13.5677345965553,
128.336810948533)) ;
#137113=CARTESIAN_POINT('Ctrl Pts',(-25.6975030410831,13.8283851031189,
128.410563145185)) ;
#137114=CARTESIAN_POINT('Ctrl Pts',(-25.7329373000182,14.0598713577401,
128.547204922732)) ;
#137115=CARTESIAN_POINT('Ctrl Pts',(-25.7865616994345,14.2455587170749,
128.736952477156)) ;
#137116=CARTESIAN_POINT('Ctrl Pts',(-25.8538626621655,14.3725641249717,
128.966665310634)) ;
#137117=CARTESIAN_POINT('Ctrl Pts',(-25.9295581721334,14.4315964655583,
129.221010674223)) ;
#137118=CARTESIAN_POINT('Ctrl Pts',(-26.006896602782,14.4181824327013,129.480002352547)) ;
#137119=CARTESIAN_POINT('Ctrl Pts',(-26.0800584448921,14.3336378405054,
129.726841816837)) ;
#137120=CARTESIAN_POINT('Ctrl Pts',(-26.1429821311044,14.1840091545094,
129.943759080814)) ;
#137121=CARTESIAN_POINT('Ctrl Pts',(-26.1905534207569,13.9789558731559,
130.115961872093)) ;
#137122=CARTESIAN_POINT('Ctrl Pts',(-26.2182982510239,13.7355808052625,
130.230023298186)) ;
#137123=CARTESIAN_POINT('Ctrl Pts',(-26.2237942797622,13.4678622499821,
130.279352827581)) ;
#137124=CARTESIAN_POINT('Ctrl Pts',(-26.2058494672465,13.1991328428123,
130.259921864044)) ;
#137125=CARTESIAN_POINT('Ctrl Pts',(-26.1650019081548,12.9452257319575,
130.173741107483)) ;
#137126=CARTESIAN_POINT('Ctrl Pts',(-26.1035333591206,12.7259341486132,
130.027259340735)) ;
#137127=CARTESIAN_POINT('Ctrl Pts',(-26.0247947651335,12.5559411201038,
129.830445570047)) ;
#137128=CARTESIAN_POINT('Ctrl Pts',(-25.9339940341689,12.4485460987932,
129.598349481578)) ;
#137129=CARTESIAN_POINT('Ctrl Pts',(-25.8371492819582,12.4111599413339,
129.348503860636)) ;
#137130=CARTESIAN_POINT('Ctrl Pts',(-25.7402515382401,12.4456278255399,
129.098470636215)) ;
#137131=CARTESIAN_POINT('Ctrl Pts',(-25.6485459840358,12.5514145660075,
128.863951218949)) ;
#137132=CARTESIAN_POINT('Ctrl Pts',(-25.5698638699777,12.7181519497096,
128.667054512607)) ;
#137133=CARTESIAN_POINT('Ctrl Pts',(-25.5074380429627,12.9364297066312,
128.517889419159)) ;
#137134=CARTESIAN_POINT('Ctrl Pts',(-25.4658667658109,13.1887531775189,
128.42950707232)) ;
#137135=CARTESIAN_POINT('Ctrl Pts',(-25.4469754063975,13.4580633206524,
128.407419238398)) ;
#137136=CARTESIAN_POINT('Ctrl Pts',(-25.451607744199,13.7256377650323,128.454145515707)) ;
#137137=CARTESIAN_POINT('Ctrl Pts',(-25.478575349501,13.9704139197111,128.565972664552)) ;
#137138=CARTESIAN_POINT('Ctrl Pts',(-25.5253124387396,14.1767864101741,
128.735643536007)) ;
#137139=CARTESIAN_POINT('Ctrl Pts',(-25.5879676204535,14.3292888333563,
128.951905035728)) ;
#137140=CARTESIAN_POINT('Ctrl Pts',(-25.6606881108518,14.4162418922063,
129.197374916368)) ;
#137141=CARTESIAN_POINT('Ctrl Pts',(-25.7382280461626,14.4323070636622,
129.457069048766)) ;
#137142=CARTESIAN_POINT('Ctrl Pts',(-25.8136145906716,14.3764282690484,
129.710284803776)) ;
#137143=CARTESIAN_POINT('Ctrl Pts',(-25.8816430048817,14.2515625943371,
129.942266343958)) ;
#137144=CARTESIAN_POINT('Ctrl Pts',(-25.9358089722647,14.0682229013696,
130.133536052826)) ;
#137145=CARTESIAN_POINT('Ctrl Pts',(-25.9721443127368,13.8370234728167,
130.27297416193)) ;
#137146=CARTESIAN_POINT('Ctrl Pts',(-25.9867897769764,13.5786250860868,
130.348703835847)) ;
#137147=CARTESIAN_POINT('Ctrl Pts',(-25.9784177256828,13.3076278419877,
130.357397820919)) ;
#137148=CARTESIAN_POINT('Ctrl Pts',(-25.946711000963,13.0452574114126,130.29787280956)) ;
#137149=CARTESIAN_POINT('Ctrl Pts',(-25.8930679516197,12.809151348438,130.17437735159)) ;
#137150=CARTESIAN_POINT('Ctrl Pts',(-25.820675289845,12.6175516783773,129.996081228465)) ;
#137151=CARTESIAN_POINT('Ctrl Pts',(-25.7346394044431,12.4843718423873,
129.777720227258)) ;
#137152=CARTESIAN_POINT('Ctrl Pts',(-25.6392954299083,12.417595884224,129.532379981805)) ;
#137153=CARTESIAN_POINT('Ctrl Pts',(-25.5415392329717,12.4230554793737,
129.2798939571)) ;
#137154=CARTESIAN_POINT('Ctrl Pts',(-25.44720407137,12.5002516157562,129.037475794767)) ;
#137155=CARTESIAN_POINT('Ctrl Pts',(-25.3627875475538,12.6429370956148,
128.823904379455)) ;
#137156=CARTESIAN_POINT('Ctrl Pts',(-25.2927915452869,12.8430358914049,
128.652724826988)) ;
#137157=CARTESIAN_POINT('Ctrl Pts',(-25.2425908671118,13.0829430235275,
128.539082315147)) ;
#137158=CARTESIAN_POINT('Ctrl Pts',(-25.2142446030042,13.3482625175679,
128.489444003025)) ;
#137159=CARTESIAN_POINT('Ctrl Pts',(-25.2093485809571,13.6179804749313,
128.508179789217)) ;
#137160=CARTESIAN_POINT('Ctrl Pts',(-25.2275485580834,13.8754577443227,
128.59460738022)) ;
#137161=CARTESIAN_POINT('Ctrl Pts',(-25.2668351056179,14.0994367889634,
128.742519747541)) ;
#137162=CARTESIAN_POINT('Ctrl Pts',(-25.3232457097912,14.2743408092093,
128.94029910677)) ;
#137163=CARTESIAN_POINT('Ctrl Pts',(-25.3927071649368,14.3892596649761,
129.176405541247)) ;
#137164=CARTESIAN_POINT('Ctrl Pts',(-25.4689980053617,14.4346258039945,
129.432371808498)) ;
#137165=CARTESIAN_POINT('Ctrl Pts',(-25.5463449745986,14.4074612367265,
129.691535915979)) ;
#137166=CARTESIAN_POINT('Ctrl Pts',(-25.617936621825,14.3096987873791,129.93377050553)) ;
#137167=CARTESIAN_POINT('Ctrl Pts',(-25.6780966245885,14.1493774053066,
130.142501646616)) ;
#137168=CARTESIAN_POINT('Ctrl Pts',(-25.7222855141894,13.9355628673905,
130.304835839477)) ;
#137169=CARTESIAN_POINT('Ctrl Pts',(-25.7460052192223,13.6861606086544,
130.407190418653)) ;
#137170=CARTESIAN_POINT('Ctrl Pts',(-25.7470805202155,13.4167352141788,
130.443555111418)) ;
#137171=CARTESIAN_POINT('Ctrl Pts',(-25.7247262193035,13.1492793403457,
130.411279088771)) ;
#137172=CARTESIAN_POINT('Ctrl Pts',(-25.6797214030516,12.9005268822979,
130.312955257449)) ;
#137173=CARTESIAN_POINT('Ctrl Pts',(-25.6147970669545,12.6897474327515,
130.15634284889)) ;
#137174=CARTESIAN_POINT('Ctrl Pts',(-25.5332896147307,12.5306016381553,
129.951467636062)) ;
#137175=CARTESIAN_POINT('Ctrl Pts',(-25.4410148555985,12.4360458908817,
129.71500187315)) ;
#137176=CARTESIAN_POINT('Ctrl Pts',(-25.3432666007832,12.412131814103,129.462653094517)) ;
#137177=CARTESIAN_POINT('Ctrl Pts',(-25.247007374808,12.4605357915181,129.214505440553)) ;
#137178=CARTESIAN_POINT('Ctrl Pts',(-25.1575767032805,12.5784164167772,
128.986475142405)) ;
#137179=CARTESIAN_POINT('Ctrl Pts',(-25.0816726489816,12.75548162504,128.797692124086)) ;
#137180=CARTESIAN_POINT('Ctrl Pts',(-25.0228641768447,12.9817623745855,
128.659113501594)) ;
#137181=CARTESIAN_POINT('Ctrl Pts',(-24.9854431235873,13.2381597682889,
128.58279479078)) ;
#137182=CARTESIAN_POINT('Ctrl Pts',(-24.9709442140284,13.5101991451629,
128.573753044088)) ;
#137183=CARTESIAN_POINT('Ctrl Pts',(-24.9798702789117,13.7733130624052,
128.632787335484)) ;
#137184=CARTESIAN_POINT('Ctrl Pts',(-25.0110723397697,14.0140640637462,
128.757279546855)) ;
#137185=CARTESIAN_POINT('Ctrl Pts',(-25.0609598922125,14.2098744225724,
128.935968377652)) ;
#137186=CARTESIAN_POINT('Ctrl Pts',(-25.1257461413825,14.3505801926375,
129.158347749617)) ;
#137187=CARTESIAN_POINT('Ctrl Pts',(-25.1999128259953,14.4248316495575,
129.408106389125)) ;
#137188=CARTESIAN_POINT('Ctrl Pts',(-25.2777575377082,14.4272048200234,
129.668752235258)) ;
#137189=CARTESIAN_POINT('Ctrl Pts',(-25.3521251101368,14.3577939953671,
129.919009377019)) ;
#137190=CARTESIAN_POINT('Ctrl Pts',(-25.4177703520866,14.2217458175161,
130.143874634482)) ;
#137191=CARTESIAN_POINT('Ctrl Pts',(-25.4692388352905,14.0267542055663,
130.327561274206)) ;
#137192=CARTESIAN_POINT('Ctrl Pts',(-25.5013721592421,13.7911380978429,
130.454356036342)) ;
#137193=CARTESIAN_POINT('Ctrl Pts',(-25.511924687266,13.5273991680406,130.518376373105)) ;
#137194=CARTESIAN_POINT('Ctrl Pts',(-25.4991050868109,13.2571617641776,
130.51398320948)) ;
#137195=CARTESIAN_POINT('Ctrl Pts',(-25.4629538937068,12.9974109548792,
130.441621863609)) ;
#137196=CARTESIAN_POINT('Ctrl Pts',(-25.4056927623469,12.7695380249157,
130.307406345911)) ;
#137197=CARTESIAN_POINT('Ctrl Pts',(-25.33042840628,12.5879937236174,130.120669835219)) ;
#137198=CARTESIAN_POINT('Ctrl Pts',(-25.2420766509654,12.4663339906868,
129.895635723357)) ;
#137199=CARTESIAN_POINT('Ctrl Pts',(-25.1454696806416,12.41305303315,129.64669692387)) ;
#137200=CARTESIAN_POINT('Ctrl Pts',(-25.048369544625,12.4321501041493,129.395973750274)) ;
#137201=CARTESIAN_POINT('Ctrl Pts',(-24.9551458762365,12.522410787778,129.156886231369)) ;
#137202=CARTESIAN_POINT('Ctrl Pts',(-24.8729558359052,12.677312203341,128.949927053074)) ;
#137203=CARTESIAN_POINT('Ctrl Pts',(-24.8067307250646,12.8853931735732,
128.789574538439)) ;
#137204=CARTESIAN_POINT('Ctrl Pts',(-24.7604114391819,13.1311434381669,
128.687274602819)) ;
#137205=CARTESIAN_POINT('Ctrl Pts',(-24.7363638964199,13.4000886870271,
128.650328698818)) ;
#137206=CARTESIAN_POINT('Ctrl Pts',(-24.7359629848961,13.667985481151,128.682120218875)) ;
#137207=CARTESIAN_POINT('Ctrl Pts',(-24.7581853104846,13.9198929118074,
128.780178599926)) ;
#137208=CARTESIAN_POINT('Ctrl Pts',(-24.801208903198,14.13673316727,128.939133160208)) ;
#137209=CARTESIAN_POINT('Ctrl Pts',(-24.8602641638815,14.300676131018,129.144561484622)) ;
#137210=CARTESIAN_POINT('Ctrl Pts',(-24.9316995313073,14.4034182516523,
129.386532253094)) ;
#137211=CARTESIAN_POINT('Ctrl Pts',(-25.008652081806,14.4350219439221,129.644438670051)) ;
#137212=CARTESIAN_POINT('Ctrl Pts',(-25.085177028276,14.3943912099649,129.901089775853)) ;
#137213=CARTESIAN_POINT('Ctrl Pts',(-25.1551357368836,14.2842181242634,
130.138566635532)) ;
#137214=CARTESIAN_POINT('Ctrl Pts',(-25.2127728109964,14.11233380319,130.340059721754)) ;
#137215=CARTESIAN_POINT('Ctrl Pts',(-25.2531900001201,13.8914433444145,
130.491203497753)) ;
#137216=CARTESIAN_POINT('Ctrl Pts',(-25.2728802791194,13.6364806192018,
130.581877006212)) ;
#137217=CARTESIAN_POINT('Ctrl Pts',(-25.2695691902487,13.3663281974235,
130.60534009255)) ;
#137218=CARTESIAN_POINT('Ctrl Pts',(-25.2428141688484,13.1002905199636,
130.560312718125)) ;
#137219=CARTESIAN_POINT('Ctrl Pts',(-25.1937738940479,12.8573187097229,
130.450194224165)) ;
#137220=CARTESIAN_POINT('Ctrl Pts',(-25.1252949558094,12.6550559201632,
130.28326882404)) ;
#137221=CARTESIAN_POINT('Ctrl Pts',(-25.041522175675,12.5076995201524,130.071671442903)) ;
#137222=CARTESIAN_POINT('Ctrl Pts',(-24.9476355648718,12.4260782231414,
129.830561197084)) ;
#137223=CARTESIAN_POINT('Ctrl Pts',(-24.8502501407946,12.4155414284777,
129.579046625511)) ;
#137224=CARTESIAN_POINT('Ctrl Pts',(-24.7538966162756,12.4780902528913,
129.330983042156)) ;
#137225=CARTESIAN_POINT('Ctrl Pts',(-24.6675208764697,12.6066343285888,
129.111475024232)) ;
#137226=CARTESIAN_POINT('Ctrl Pts',(-24.5938515785469,12.7952135376049,
128.9295353476)) ;
#137227=CARTESIAN_POINT('Ctrl Pts',(-24.5390606686421,13.0279818005268,
128.802553603919)) ;
#137228=CARTESIAN_POINT('Ctrl Pts',(-24.5057245134978,13.2896873731217,
128.73835017349)) ;
#137229=CARTESIAN_POINT('Ctrl Pts',(-24.4957718456139,13.5603127148141,
128.742368279822)) ;
#137230=CARTESIAN_POINT('Ctrl Pts',(-24.5089980783373,13.8211026709328,
128.814095191955)) ;
#137231=CARTESIAN_POINT('Ctrl Pts',(-24.5438612527322,14.0538031496825,
128.949086534568)) ;
#137232=CARTESIAN_POINT('Ctrl Pts',(-24.5970360172465,14.2410907162982,
129.137531563715)) ;
#137233=CARTESIAN_POINT('Ctrl Pts',(-24.6642374142229,14.3701940931664,
129.367050561935)) ;
#137234=CARTESIAN_POINT('Ctrl Pts',(-24.7397318651878,14.4308809460844,
129.62077656555)) ;
#137235=CARTESIAN_POINT('Ctrl Pts',(-24.8168605982929,14.4196139003572,
129.879052696967)) ;
#137236=CARTESIAN_POINT('Ctrl Pts',(-24.8904031542241,14.336836882695,130.127084143124)) ;
#137237=CARTESIAN_POINT('Ctrl Pts',(-24.9535128568133,14.1892311561633,
130.344459510931)) ;
#137238=CARTESIAN_POINT('Ctrl Pts',(-25.001609263022,13.9859053785223,130.518165732824)) ;
#137239=CARTESIAN_POINT('Ctrl Pts',(-25.0300402506867,13.7426112517957,
130.634341797192)) ;
#137240=CARTESIAN_POINT('Ctrl Pts',(-25.0361683447046,13.4761438814329,
130.685407728846)) ;
#137241=CARTESIAN_POINT('Ctrl Pts',(-25.0189583644701,13.2070931774866,
130.668139714786)) ;
#137242=CARTESIAN_POINT('Ctrl Pts',(-24.97869544815,12.9521503928351,130.583708331341)) ;
#137243=CARTESIAN_POINT('Ctrl Pts',(-24.9177844273565,12.7315094289201,
130.438861249866)) ;
#137244=CARTESIAN_POINT('Ctrl Pts',(-24.8391101053067,12.55952255891,130.242364324163)) ;
#137245=CARTESIAN_POINT('Ctrl Pts',(-24.7493048000512,12.4509681348577,
130.012910139936)) ;
#137246=CARTESIAN_POINT('Ctrl Pts',(-24.6517732733907,12.4111337654698,
129.761332887985)) ;
#137247=CARTESIAN_POINT('Ctrl Pts',(-24.5552548880009,12.4436883987287,
129.512247618014)) ;
#137248=CARTESIAN_POINT('Ctrl Pts',(-24.4632268332124,12.5474867410868,
129.276810629961)) ;
#137249=CARTESIAN_POINT('Ctrl Pts',(-24.3842162437121,12.7123018104689,
129.078905084089)) ;
#137250=CARTESIAN_POINT('Ctrl Pts',(-24.3210840647397,12.930070804837,128.927784936673)) ;
#137251=CARTESIAN_POINT('Ctrl Pts',(-24.2790719777108,13.1802337484168,
128.837930667053)) ;
#137252=CARTESIAN_POINT('Ctrl Pts',(-24.2593594113849,13.4510759105696,
128.813665180465)) ;
#137253=CARTESIAN_POINT('Ctrl Pts',(-24.2633748242578,13.7180592820174,
128.858471439146)) ;
#137254=CARTESIAN_POINT('Ctrl Pts',(-24.2897810253052,13.9642785857624,
128.968736525003)) ;
#137255=CARTESIAN_POINT('Ctrl Pts',(-24.3359172579478,14.1712561448263,
129.136557180843)) ;
#137256=CARTESIAN_POINT('Ctrl Pts',(-24.3979070515482,14.3253724982605,
129.350764867934)) ;
#137257=CARTESIAN_POINT('Ctrl Pts',(-24.4709758873292,14.4148742496936,
129.597512003327)) ;
#137258=CARTESIAN_POINT('Ctrl Pts',(-24.5478797311828,14.4329087927554,
129.855085425243)) ;
#137259=CARTESIAN_POINT('Ctrl Pts',(-24.6239219034766,14.3788838662948,
130.110446558237)) ;
#137260=CARTESIAN_POINT('Ctrl Pts',(-24.692012674099,14.2561020385484,130.342495417094)) ;
#137261=CARTESIAN_POINT('Ctrl Pts',(-24.7466767208365,14.0742378905462,
130.535245795861)) ;
#137262=CARTESIAN_POINT('Ctrl Pts',(-24.7834767939557,13.8451951074059,
130.675901048507)) ;
#137263=CARTESIAN_POINT('Ctrl Pts',(-24.7989416578835,13.5867436924812,
130.754122251571)) ;
#137264=CARTESIAN_POINT('Ctrl Pts',(-24.7911326203798,13.3144406104729,
130.764624304837)) ;
#137265=CARTESIAN_POINT('Ctrl Pts',(-24.760168773577,13.0528697153062,130.707111677067)) ;
#137266=CARTESIAN_POINT('Ctrl Pts',(-24.7072987550556,12.8160519673843,
130.585813252149)) ;
#137267=CARTESIAN_POINT('Ctrl Pts',(-24.6353533732366,12.6226066577663,
130.408861363044)) ;
#137268=CARTESIAN_POINT('Ctrl Pts',(-24.5494827855599,12.4871997727771,
130.1910537292)) ;
#137269=CARTESIAN_POINT('Ctrl Pts',(-24.4539509697658,12.4184347906441,
129.945282406851)) ;
#137270=CARTESIAN_POINT('Ctrl Pts',(-24.3567514327947,12.421900095689,129.694230668796)) ;
#137271=CARTESIAN_POINT('Ctrl Pts',(-24.2621043582377,12.4968773890891,
129.450935185036)) ;
#137272=CARTESIAN_POINT('Ctrl Pts',(-24.1771968895545,12.6381725134135,
129.235992950347)) ;
#137273=CARTESIAN_POINT('Ctrl Pts',(-24.1068996585392,12.8360676034159,
129.063819100228)) ;
#137274=CARTESIAN_POINT('Ctrl Pts',(-24.0558483744943,13.0762564614049,
128.947865518948)) ;
#137275=CARTESIAN_POINT('Ctrl Pts',(-24.0270075658694,13.3398739353009,
128.896618474856)) ;
#137276=CARTESIAN_POINT('Ctrl Pts',(-24.0213604180131,13.6103042607725,
128.913234992603)) ;
#137277=CARTESIAN_POINT('Ctrl Pts',(-24.0389205379422,13.8681248638129,
128.997754741653)) ;
#137278=CARTESIAN_POINT('Ctrl Pts',(-24.0775340449391,14.0932870641316,
129.14367411103)) ;
#137279=CARTESIAN_POINT('Ctrl Pts',(-24.1339243216249,14.2707836154913,
129.341616284265)) ;
#137280=CARTESIAN_POINT('Ctrl Pts',(-24.2026976504377,14.3866738270234,
129.575503449419)) ;
#137281=CARTESIAN_POINT('Ctrl Pts',(-24.2789122688586,14.4343395634598,
129.831274305498)) ;
#137282=CARTESIAN_POINT('Ctrl Pts',(-24.3561654891957,14.4093417232231,
130.090097199801)) ;
#137283=CARTESIAN_POINT('Ctrl Pts',(-24.4280593379148,14.3139583409208,
130.333211542835)) ;
#137284=CARTESIAN_POINT('Ctrl Pts',(-24.4890184297721,14.1538396198972,
130.544536166567)) ;
#137285=CARTESIAN_POINT('Ctrl Pts',(-24.5333312219411,13.9434082159672,
130.706904626891)) ;
#137286=CARTESIAN_POINT('Ctrl Pts',(-24.5579214950625,13.6926166151685,
130.812110819993)) ;
#137287=CARTESIAN_POINT('Ctrl Pts',(-24.5595818848025,13.4252309496683,
130.849953790189)) ;
#137288=CARTESIAN_POINT('Ctrl Pts',(-24.5379430220355,13.1569924841194,
130.81983442348)) ;
#137289=CARTESIAN_POINT('Ctrl Pts',(-24.4936001603481,12.907415746913,130.723430091029)) ;
#137290=CARTESIAN_POINT('Ctrl Pts',(-24.4288932095814,12.6946405642384,
130.567589996659)) ;
#137291=CARTESIAN_POINT('Ctrl Pts',(-24.3483707094481,12.5348309351463,
130.365354677471)) ;
#137292=CARTESIAN_POINT('Ctrl Pts',(-24.2557580076912,12.4376124732534,
130.128119836039)) ;
#137293=CARTESIAN_POINT('Ctrl Pts',(-24.158577834541,12.411847051202,129.877251493057)) ;
#137294=CARTESIAN_POINT('Ctrl Pts',(-24.0620294843223,12.4580456459642,
129.628319557637)) ;
#137295=CARTESIAN_POINT('Ctrl Pts',(-23.9724819407128,12.5736491008617,
129.399871559833)) ;
#137296=CARTESIAN_POINT('Ctrl Pts',(-23.8958324246764,12.7495591345061,
129.209023299466)) ;
#137297=CARTESIAN_POINT('Ctrl Pts',(-23.8363403529087,12.9753683217391,
129.06853311284)) ;
#137298=CARTESIAN_POINT('Ctrl Pts',(-23.7983705149086,13.2312289198464,
128.990617600681)) ;
#137299=CARTESIAN_POINT('Ctrl Pts',(-23.7832383935185,13.5022490913223,
128.979611461187)) ;
#137300=CARTESIAN_POINT('Ctrl Pts',(-23.7915690414023,13.7663766429706,
129.036987224607)) ;
#137301=CARTESIAN_POINT('Ctrl Pts',(-23.8218816093751,14.0063275981214,
129.158621057965)) ;
#137302=CARTESIAN_POINT('Ctrl Pts',(-23.8714125707789,14.2048735685629,
129.336436861487)) ;
#137303=CARTESIAN_POINT('Ctrl Pts',(-23.9360766035452,14.3476911545505,
129.558558579197)) ;
#137304=CARTESIAN_POINT('Ctrl Pts',(-24.0101424431012,14.4237776141336,
129.808052928934)) ;
#137305=CARTESIAN_POINT('Ctrl Pts',(-24.0877654886693,14.4280807917519,
130.067962762365)) ;
#137306=CARTESIAN_POINT('Ctrl Pts',(-24.1623469987095,14.360827921304,130.318852067325)) ;
#137307=CARTESIAN_POINT('Ctrl Pts',(-24.2285176630201,14.2256361349193,
130.545392667963)) ;
#137308=CARTESIAN_POINT('Ctrl Pts',(-24.2799186020434,14.0344801252662,
130.728492767782)) ;
#137309=CARTESIAN_POINT('Ctrl Pts',(-24.3130244781345,13.7980437562362,
130.858419713646)) ;
#137310=CARTESIAN_POINT('Ctrl Pts',(-24.3241513604221,13.53532438393,130.924036543225)) ;
#137311=CARTESIAN_POINT('Ctrl Pts',(-24.3119764531114,13.2644875678434,
130.921600659002)) ;
#137312=CARTESIAN_POINT('Ctrl Pts',(-24.276607917817,13.0050530170807,130.851402331197)) ;
#137313=CARTESIAN_POINT('Ctrl Pts',(-24.2198137245786,12.775438141039,130.718635056671)) ;
#137314=CARTESIAN_POINT('Ctrl Pts',(-24.1450871500959,12.5925960963687,
130.533426659931)) ;
#137315=CARTESIAN_POINT('Ctrl Pts',(-24.0570562303304,12.4690082469491,
130.309331812912)) ;
#137316=CARTESIAN_POINT('Ctrl Pts',(-23.9606548006948,12.4135709185057,
130.060969797119)) ;
#137317=CARTESIAN_POINT('Ctrl Pts',(-23.8633239205352,12.4306394810107,
129.809638399428)) ;
#137318=CARTESIAN_POINT('Ctrl Pts',(-23.7701586445981,12.5185474861746,
129.570614180752)) ;
#137319=CARTESIAN_POINT('Ctrl Pts',(-23.6874386169935,12.6718439913262,
129.362161787323)) ;
#137320=CARTESIAN_POINT('Ctrl Pts',(-23.6207199401336,12.8780301439606,
129.200304555462)) ;
#137321=CARTESIAN_POINT('Ctrl Pts',(-23.5734544100946,13.1252485962165,
129.095546151147)) ;
#137322=CARTESIAN_POINT('Ctrl Pts',(-23.5490275882913,13.3909665400584,
129.057124901564)) ;
#137323=CARTESIAN_POINT('Ctrl Pts',(-23.5478469452304,13.6612160877443,
129.086903188456)) ;
#137324=CARTESIAN_POINT('Ctrl Pts',(-23.5695278793464,13.9131568788034,
129.183301070422)) ;
#137325=CARTESIAN_POINT('Ctrl Pts',(-23.6117378779522,14.1304384080089,
129.339731339965)) ;
#137326=CARTESIAN_POINT('Ctrl Pts',(-23.670618868599,14.2969775137474,129.544805224008)) ;
#137327=CARTESIAN_POINT('Ctrl Pts',(-23.7419278031084,14.4015522183562,
129.786450816467)) ;
#137328=CARTESIAN_POINT('Ctrl Pts',(-23.8185327256045,14.4350500547512,
130.04322857818)) ;
#137329=CARTESIAN_POINT('Ctrl Pts',(-23.895073988246,14.396751965708,130.29988774461)) ;
#137330=CARTESIAN_POINT('Ctrl Pts',(-23.9654056990637,14.2884849239284,
130.538494109741)) ;
#137331=CARTESIAN_POINT('Ctrl Pts',(-24.0235441195686,14.1181741044495,
130.74147538802)) ;
#137332=CARTESIAN_POINT('Ctrl Pts',(-24.064579062323,13.8977533675812,130.894521933553)) ;
#137333=CARTESIAN_POINT('Ctrl Pts',(-24.0848219240481,13.6446685040666,
130.986656853548)) ;
#137334=CARTESIAN_POINT('Ctrl Pts',(-24.0822023369396,13.3734340849695,
131.012296376983)) ;
#137335=CARTESIAN_POINT('Ctrl Pts',(-24.0560179172839,13.1072277425428,
130.968914707618)) ;
#137336=CARTESIAN_POINT('Ctrl Pts',(-24.0077701366724,12.8641926256241,
130.860994227657)) ;
#137337=CARTESIAN_POINT('Ctrl Pts',(-23.9398468464116,12.6605228267135,
130.695685489353)) ;
#137338=CARTESIAN_POINT('Ctrl Pts',(-23.8566310215138,12.5114117943071,
130.485659567777)) ;
#137339=CARTESIAN_POINT('Ctrl Pts',(-23.7623999995309,12.4272142366947,
130.24373969586)) ;
#137340=CARTESIAN_POINT('Ctrl Pts',(-23.6651743173675,12.4150347895705,
129.99264727931)) ;
#137341=CARTESIAN_POINT('Ctrl Pts',(-23.5692968163676,12.4747490693336,
129.745746794804)) ;
#137342=CARTESIAN_POINT('Ctrl Pts',(-23.4818229937488,12.6023244974168,
129.523310907728)) ;
#137343=CARTESIAN_POINT('Ctrl Pts',(-23.407748924182,12.7898413054048,129.340204613242)) ;
#137344=CARTESIAN_POINT('Ctrl Pts',(-23.3526025051574,13.0206705904154,
129.212059796763)) ;
#137345=CARTESIAN_POINT('Ctrl Pts',(-23.3185827971363,13.2818516686094,
129.145867360566)) ;
#137346=CARTESIAN_POINT('Ctrl Pts',(-23.3079501436408,13.5521276503918,
129.147857520888)) ;
#137347=CARTESIAN_POINT('Ctrl Pts',(-23.320481206199,13.8139567141273,129.217605438094)) ;
#137348=CARTESIAN_POINT('Ctrl Pts',(-23.3550030243452,14.048569772894,129.351746255589)) ;
#137349=CARTESIAN_POINT('Ctrl Pts',(-23.407397020995,14.236110064849,129.537698849994)) ;
#137350=CARTESIAN_POINT('Ctrl Pts',(-23.4744514414992,14.3675383495349,
129.766892450617)) ;
#137351=CARTESIAN_POINT('Ctrl Pts',(-23.5496273539776,14.4300942129039,
130.019607525919)) ;
#137352=CARTESIAN_POINT('Ctrl Pts',(-23.6268969486743,14.4208865440108,
130.27835213759)) ;
#137353=CARTESIAN_POINT('Ctrl Pts',(-23.7004306698474,14.3405661595428,
130.526245792846)) ;
#137354=CARTESIAN_POINT('Ctrl Pts',(-23.7644224178413,14.1934623353678,
130.746473197132)) ;
#137355=CARTESIAN_POINT('Ctrl Pts',(-23.8127756419206,13.9917022900947,
130.920839890071)) ;
#137356=CARTESIAN_POINT('Ctrl Pts',(-23.8416998117934,13.7502057571416,
131.038343138081)) ;
#137357=CARTESIAN_POINT('Ctrl Pts',(-23.8485644464668,13.4844948245858,
131.091517749686)) ;
#137358=CARTESIAN_POINT('Ctrl Pts',(-23.8319362934437,13.2141841608485,
131.076089294491)) ;
#137359=CARTESIAN_POINT('Ctrl Pts',(-23.7923791092109,12.9589228600533,
130.99365805615)) ;
#137360=CARTESIAN_POINT('Ctrl Pts',(-23.7315857819428,12.7362703078518,
130.849331458812)) ;
#137361=CARTESIAN_POINT('Ctrl Pts',(-23.654489045961,12.5648475135275,130.656969361176)) ;
#137362=CARTESIAN_POINT('Ctrl Pts',(-23.5639389610065,12.452872637983,130.425740312664)) ;
#137363=CARTESIAN_POINT('Ctrl Pts',(-23.4673752556237,12.411294196787,130.176678568121)) ;
#137364=CARTESIAN_POINT('Ctrl Pts',(-23.3698780425036,12.4419882066381,
129.92505446556)) ;
#137365=CARTESIAN_POINT('Ctrl Pts',(-23.2785520721008,12.5427027858175,
129.691305126012)) ;
#137366=CARTESIAN_POINT('Ctrl Pts',(-23.1984718637741,12.706796402249,129.490533281651)) ;
#137367=CARTESIAN_POINT('Ctrl Pts',(-23.135068634506,12.9221001593752,129.338439944309)) ;
#137368=CARTESIAN_POINT('Ctrl Pts',(-23.0919954586335,13.1741319900526,
129.245841884835)) ;
#137369=CARTESIAN_POINT('Ctrl Pts',(-23.0718580306747,13.4427023276839,
129.220070404539)) ;
#137370=CARTESIAN_POINT('Ctrl Pts',(-23.0751585689848,13.7107857008536,
129.26289034347)) ;
#137371=CARTESIAN_POINT('Ctrl Pts',(-23.1008376347237,13.9568883020333,
129.370893251844)) ;
#137372=CARTESIAN_POINT('Ctrl Pts',(-23.1465403344726,14.1661036589884,
129.537562189888)) ;
#137373=CARTESIAN_POINT('Ctrl Pts',(-23.2083074256075,14.3219384877272,
129.75117659853)) ;
#137374=CARTESIAN_POINT('Ctrl Pts',(-23.2806542878813,14.4130180667709,
129.995597829584)) ;
#137375=CARTESIAN_POINT('Ctrl Pts',(-23.3580236308951,14.4335349377785,
130.254752754733)) ;
#137376=CARTESIAN_POINT('Ctrl Pts',(-23.4342369440473,14.3810414591398,
130.510644418635)) ;
#137377=CARTESIAN_POINT('Ctrl Pts',(-23.5022753810008,14.2609491563611,
130.742352348115)) ;
#137378=CARTESIAN_POINT('Ctrl Pts',(-23.5576881153806,14.0795345145358,
130.937487790807)) ;
#137379=CARTESIAN_POINT('Ctrl Pts',(-23.5948722936596,13.8529285433275,
131.079068657613)) ;
#137380=CARTESIAN_POINT('Ctrl Pts',(-23.6110592381906,13.5926909018936,
131.159708991485)) ;
#137381=CARTESIAN_POINT('Ctrl Pts',(-23.6039222248104,13.3230679904021,
131.171845507133)) ;
#137382=CARTESIAN_POINT('Ctrl Pts',(-23.5735515673625,13.0595446516906,
131.116246634271)) ;
#137383=CARTESIAN_POINT('Ctrl Pts',(-23.5210444853348,12.821409078981,130.996073210915)) ;
#137384=CARTESIAN_POINT('Ctrl Pts',(-23.4496688403902,12.6270968771254,
130.820718874116)) ;
#137385=CARTESIAN_POINT('Ctrl Pts',(-23.3644228508194,12.4904302575877,
130.604624186015)) ;
#137386=CARTESIAN_POINT('Ctrl Pts',(-23.2693883176564,12.4195264376518,
130.360202664601)) ;
#137387=CARTESIAN_POINT('Ctrl Pts',(-23.1717013390917,12.4206997747971,
130.107888702409)) ;
#137388=CARTESIAN_POINT('Ctrl Pts',(-23.07674697722,12.4940150849619,129.863744537933)) ;
#137389=CARTESIAN_POINT('Ctrl Pts',(-22.9917454792659,12.6331733496192,
129.648432936584)) ;
#137390=CARTESIAN_POINT('Ctrl Pts',(-22.9210033107914,12.8293255236082,
129.47492493208)) ;
#137391=CARTESIAN_POINT('Ctrl Pts',(-22.8693173983923,13.0683011169746,
129.357098375333)) ;
#137392=CARTESIAN_POINT('Ctrl Pts',(-22.8397009911573,13.3322965961088,
129.303691206083)) ;
#137393=CARTESIAN_POINT('Ctrl Pts',(-22.8334317380967,13.6026348428664,
129.318468394913)) ;
#137394=CARTESIAN_POINT('Ctrl Pts',(-22.8502549510441,13.8605087628932,
129.400751483274)) ;
#137395=CARTESIAN_POINT('Ctrl Pts',(-22.8883323200656,14.0871783650871,
129.545152491834)) ;
#137396=CARTESIAN_POINT('Ctrl Pts',(-22.9440423731906,14.2658343770077,
129.74099514858)) ;
#137397=CARTESIAN_POINT('Ctrl Pts',(-23.0127923157115,14.3843789391541,
129.974962574827)) ;
#137398=CARTESIAN_POINT('Ctrl Pts',(-23.0890433292092,14.4339734241572,
130.230900091451)) ;
#137399=CARTESIAN_POINT('Ctrl Pts',(-23.1661312317174,14.4110559361857,
130.489146023008)) ;
#137400=CARTESIAN_POINT('Ctrl Pts',(-23.2382006324762,14.3178925144465,
130.732739172181)) ;
#137401=CARTESIAN_POINT('Ctrl Pts',(-23.2996857722997,14.1593686690055,
130.945647915619)) ;
#137402=CARTESIAN_POINT('Ctrl Pts',(-23.3445584705906,13.9496805388889,
131.109722558938)) ;
#137403=CARTESIAN_POINT('Ctrl Pts',(-23.3696736527837,13.7013470012748,
131.216252350218)) ;
#137404=CARTESIAN_POINT('Ctrl Pts',(-23.3720920163119,13.4330164706509,
131.256471678111)) ;
#137405=CARTESIAN_POINT('Ctrl Pts',(-23.3511454215899,13.1647607659068,
131.228335735827)) ;
#137406=CARTESIAN_POINT('Ctrl Pts',(-23.3072621176942,12.9137311953691,
131.133374404822)) ;
#137407=CARTESIAN_POINT('Ctrl Pts',(-23.2434888033612,12.7007529765594,
130.980069049084)) ;
#137408=CARTESIAN_POINT('Ctrl Pts',(-23.1628787911392,12.5383275950027,
130.777785669083)) ;
#137409=CARTESIAN_POINT('Ctrl Pts',(-23.0712872888514,12.4398166155699,
130.543252817928)) ;
#137410=CARTESIAN_POINT('Ctrl Pts',(-22.9733700901106,12.4114725014285,
130.290514442298)) ;
#137411=CARTESIAN_POINT('Ctrl Pts',(-22.8769228839034,12.4557968837197,
130.041802473424)) ;
#137412=CARTESIAN_POINT('Ctrl Pts',(-22.7869968694901,12.5696290703402,
129.812287837357)) ;
#137413=CARTESIAN_POINT('Ctrl Pts',(-22.7101031050184,12.7436129145437,
129.620649242638)) ;
#137414=CARTESIAN_POINT('Ctrl Pts',(-22.6500085106509,12.9681021997866,
129.478393868049)) ;
#137415=CARTESIAN_POINT('Ctrl Pts',(-22.6113280612937,13.2239470656193,
129.398484240347)) ;
#137416=CARTESIAN_POINT('Ctrl Pts',(-22.5955724991583,13.4941632022952,
129.385572434223)) ;
#137417=CARTESIAN_POINT('Ctrl Pts',(-22.6032116810304,13.7589185594046,
129.440951942343)) ;
#137418=CARTESIAN_POINT('Ctrl Pts',(-22.6329203868012,13.999834830615,129.560819723437)) ;
#137419=CARTESIAN_POINT('Ctrl Pts',(-22.6819480888645,14.1997645777198,
129.737163915801)) ;
#137420=CARTESIAN_POINT('Ctrl Pts',(-22.7461154267965,14.3442636718176,
129.957775023844)) ;
#137421=CARTESIAN_POINT('Ctrl Pts',(-22.8201291984854,14.4224928178984,
130.207186244669)) ;
#137422=CARTESIAN_POINT('Ctrl Pts',(-22.8973493324398,14.429171124512,130.465747266348)) ;
#137423=CARTESIAN_POINT('Ctrl Pts',(-22.9726528467362,14.3636109202534,
130.718991967903)) ;
#137424=CARTESIAN_POINT('Ctrl Pts',(-23.0389194410672,14.2305642022342,
130.945696008778)) ;
#137425=CARTESIAN_POINT('Ctrl Pts',(-23.0908974390234,14.0406276478755,
131.130542175203)) ;
#137426=CARTESIAN_POINT('Ctrl Pts',(-23.1245333358198,13.8058700767644,
131.261928515044)) ;
#137427=CARTESIAN_POINT('Ctrl Pts',(-23.1363830164337,13.5427809263485,
131.329774433396)) ;
#137428=CARTESIAN_POINT('Ctrl Pts',(-23.1248575359644,13.2720606343581,
131.329212568738)) ;
#137429=CARTESIAN_POINT('Ctrl Pts',(-23.0900746108795,13.0118430008048,
131.26075620549)) ;
#137430=CARTESIAN_POINT('Ctrl Pts',(-23.0340455584365,12.7818788914411,
131.13011430412)) ;
#137431=CARTESIAN_POINT('Ctrl Pts',(-22.9596349753376,12.5968717145733,
130.945912471778)) ;
#137432=CARTESIAN_POINT('Ctrl Pts',(-22.8715122077198,12.471251749294,130.721681034181)) ;
#137433=CARTESIAN_POINT('Ctrl Pts',(-22.7757176314075,12.4142248024153,
130.474925696683)) ;
#137434=CARTESIAN_POINT('Ctrl Pts',(-22.6781851317645,12.4291610280905,
130.22306244369)) ;
#137435=CARTESIAN_POINT('Ctrl Pts',(-22.5847562522808,12.5152749264354,
129.983286515838)) ;
#137436=CARTESIAN_POINT('Ctrl Pts',(-22.5015747269694,12.6672522037425,
129.773535207759)) ;
#137437=CARTESIAN_POINT('Ctrl Pts',(-22.4346652666614,12.8714563204239,
129.610995698154)) ;
#137438=CARTESIAN_POINT('Ctrl Pts',(-22.3868994473045,13.1164156174602,
129.504613845988)) ;
#137439=CARTESIAN_POINT('Ctrl Pts',(-22.3615817594558,13.3833143441499,
129.463785300508)) ;
#137440=CARTESIAN_POINT('Ctrl Pts',(-22.3597882823452,13.6536761481919,
129.49176218256)) ;
#137441=CARTESIAN_POINT('Ctrl Pts',(-22.3807933273105,13.9063303510439,
129.58617443786)) ;
#137442=CARTESIAN_POINT('Ctrl Pts',(-22.4226906447706,14.125656517117,129.741831670047)) ;
#137443=CARTESIAN_POINT('Ctrl Pts',(-22.480992797728,14.2929703980627,129.945090280937)) ;
#137444=CARTESIAN_POINT('Ctrl Pts',(-22.5518543733382,14.3994043116304,
130.185355863779)) ;
#137445=CARTESIAN_POINT('Ctrl Pts',(-22.6285093988248,14.4351253202173,
130.442339869809)) ;
#137446=CARTESIAN_POINT('Ctrl Pts',(-22.7051973850955,14.3988243960317,
130.699449624082)) ;
#137447=CARTESIAN_POINT('Ctrl Pts',(-22.7758084986371,14.2923293352694,
130.938885575333)) ;
#137448=CARTESIAN_POINT('Ctrl Pts',(-22.8341888942695,14.1241731264117,
131.142472997224)) ;
#137449=CARTESIAN_POINT('Ctrl Pts',(-22.8758535864009,13.9051614113411,
131.297356933649)) ;
#137450=CARTESIAN_POINT('Ctrl Pts',(-22.8967675053112,13.6518311651615,
131.391575680539)) ;
#137451=CARTESIAN_POINT('Ctrl Pts',(-22.8948524255514,13.3824709073359,
131.419066522015)) ;
#137452=CARTESIAN_POINT('Ctrl Pts',(-22.8694536911301,13.1154253755206,
131.378028547348)) ;
#137453=CARTESIAN_POINT('Ctrl Pts',(-22.8216303727267,12.870532700791,131.271475250091)) ;
#137454=CARTESIAN_POINT('Ctrl Pts',(-22.7542127450307,12.6655371324335,
131.107638188433)) ;
#137455=CARTESIAN_POINT('Ctrl Pts',(-22.6711951167249,12.5146112693424,
130.898249520681)) ;
#137456=CARTESIAN_POINT('Ctrl Pts',(-22.5777454584632,12.4289102076434,
130.658411657876)) ;
#137457=CARTESIAN_POINT('Ctrl Pts',(-22.4803400259961,12.4141896647539,
130.406868783015)) ;
#137458=CARTESIAN_POINT('Ctrl Pts',(-22.3837956818218,12.4724108271044,
130.158202744766)) ;
#137459=CARTESIAN_POINT('Ctrl Pts',(-22.2964764439714,12.5978141623982,
129.936061247941)) ;
#137460=CARTESIAN_POINT('Ctrl Pts',(-22.222180894914,12.7826551138703,129.752158405497)) ;
#137461=CARTESIAN_POINT('Ctrl Pts',(-22.1661151196085,13.013381389437,129.621487955934)) ;
#137462=CARTESIAN_POINT('Ctrl Pts',(-22.1314362662289,13.2742167666549,
129.553393622124)) ;
#137463=CARTESIAN_POINT('Ctrl Pts',(-22.1201350356918,13.5450313802589,
129.553498432196)) ;
#137464=CARTESIAN_POINT('Ctrl Pts',(-22.1320713682587,13.8067210995316,
129.621436808792)) ;
#137465=CARTESIAN_POINT('Ctrl Pts',(-22.1657011419629,14.0412512155271,
129.752780861513)) ;
#137466=CARTESIAN_POINT('Ctrl Pts',(-22.2179806871803,14.2318696546287,
129.938653767515)) ;
#137467=CARTESIAN_POINT('Ctrl Pts',(-22.2845880318834,14.3645252689238,
130.16645539328)) ;
#137468=CARTESIAN_POINT('Ctrl Pts',(-22.3592798328537,14.4291513639763,
130.417628538692)) ;
#137469=CARTESIAN_POINT('Ctrl Pts',(-22.436871642398,14.4223448397237,130.677436734826)) ;
#137470=CARTESIAN_POINT('Ctrl Pts',(-22.510846648584,14.3433928726762,130.926745639385)) ;
#137471=CARTESIAN_POINT('Ctrl Pts',(-22.57467863088,14.1993298116068,131.146227665756)) ;
#137472=CARTESIAN_POINT('Ctrl Pts',(-22.6237644035119,13.9988091287191,
131.322818887298)) ;
#137473=CARTESIAN_POINT('Ctrl Pts',(-22.6533894867198,13.7578102679721,
131.442430456946)) ;
#137474=CARTESIAN_POINT('Ctrl Pts',(-22.6608850427505,13.491649195449,131.497555891874)) ;
#137475=CARTESIAN_POINT('Ctrl Pts',(-22.64500311771,13.2223244098795,131.484163859812)) ;
#137476=CARTESIAN_POINT('Ctrl Pts',(-22.6059893392227,12.96574693319,131.403407690678)) ;
#137477=CARTESIAN_POINT('Ctrl Pts',(-22.5461201352489,12.7429297081588,
131.261604090611)) ;
#137478=CARTESIAN_POINT('Ctrl Pts',(-22.4689354238792,12.5685157395234,
131.069226764808)) ;
#137479=CARTESIAN_POINT('Ctrl Pts',(-22.3786382574204,12.4549912739037,
130.83872380872)) ;
#137480=CARTESIAN_POINT('Ctrl Pts',(-22.2823846413124,12.4115665134561,
130.590501453343)) ;
#137481=CARTESIAN_POINT('Ctrl Pts',(-22.185022978805,12.439915366976,130.339196899106)) ;
#137482=CARTESIAN_POINT('Ctrl Pts',(-22.0929640431126,12.5392662703676,
130.103484375993)) ;
#137483=CARTESIAN_POINT('Ctrl Pts',(-22.0127053078525,12.7015765318143,
129.902116599291)) ;
#137484=CARTESIAN_POINT('Ctrl Pts',(-21.9489204298559,12.9151235355211,
129.748837978728)) ;
#137485=CARTESIAN_POINT('Ctrl Pts',(-21.9052335765829,13.1655123701317,
129.65434805994)) ;
#137486=CARTESIAN_POINT('Ctrl Pts',(-21.8842873311341,13.435707308921,129.626447566814)) ;
#137487=CARTESIAN_POINT('Ctrl Pts',(-21.8869481330479,13.7027427336547,
129.667228378349)) ;
#137488=CARTESIAN_POINT('Ctrl Pts',(-21.9120183916717,13.9504288164231,
129.773544414319)) ;
#137489=CARTESIAN_POINT('Ctrl Pts',(-21.9572517363974,14.1608970885181,
129.938846468588)) ;
#137490=CARTESIAN_POINT('Ctrl Pts',(-22.018507368848,14.3182076506529,130.150909064873)) ;
#137491=CARTESIAN_POINT('Ctrl Pts',(-22.0907386237567,14.4114239636762,
130.395045201029)) ;
#137492=CARTESIAN_POINT('Ctrl Pts',(-22.1678997175522,14.43387114395,130.653528180286)) ;
#137493=CARTESIAN_POINT('Ctrl Pts',(-22.2440626405903,14.3839736485786,
130.909179188166)) ;
#137494=CARTESIAN_POINT('Ctrl Pts',(-22.3128383560668,14.2649034164715,
131.143264149934)) ;
#137495=CARTESIAN_POINT('Ctrl Pts',(-22.368369781886,14.0862373803975,131.338529256948)) ;
#137496=CARTESIAN_POINT('Ctrl Pts',(-22.4063643713204,13.8593710344565,
131.482693687338)) ;
#137497=CARTESIAN_POINT('Ctrl Pts',(-22.423082781093,13.6016402973256,131.564639588124)) ;
#137498=CARTESIAN_POINT('Ctrl Pts',(-22.416710563554,13.3309242141033,131.579161001393)) ;
#137499=CARTESIAN_POINT('Ctrl Pts',(-22.3869594339498,13.0670234319289,
131.525359499281)) ;
#137500=CARTESIAN_POINT('Ctrl Pts',(-22.3352755509082,12.828626261272,131.407481838502)) ;
#137501=CARTESIAN_POINT('Ctrl Pts',(-22.2644737257156,12.6324569777035,
131.233812164351)) ;
#137502=CARTESIAN_POINT('Ctrl Pts',(-22.179026147261,12.4932134027072,131.017336188657)) ;
#137503=CARTESIAN_POINT('Ctrl Pts',(-22.0846147994345,12.4206918298189,
130.774574849433)) ;
#137504=CARTESIAN_POINT('Ctrl Pts',(-21.9866149275365,12.4196226590599,
130.521455957442)) ;
#137505=CARTESIAN_POINT('Ctrl Pts',(-21.8915517263097,12.4910154498675,
130.276970511203)) ;
#137506=CARTESIAN_POINT('Ctrl Pts',(-21.8061759252374,12.6283739089441,
130.060574403858)) ;
#137507=CARTESIAN_POINT('Ctrl Pts',(-21.734785916595,12.8237068444054,129.885261771197)) ;
#137508=CARTESIAN_POINT('Ctrl Pts',(-21.6826427874687,13.0616748025397,
129.766076185179)) ;
#137509=CARTESIAN_POINT('Ctrl Pts',(-21.6524872755057,13.3240381252934,
129.710950435826)) ;
#137510=CARTESIAN_POINT('Ctrl Pts',(-21.6454690535715,13.5952492770895,
129.723635230244)) ;
#137511=CARTESIAN_POINT('Ctrl Pts',(-21.6617842864879,13.8544594163448,
129.804532436936)) ;
#137512=CARTESIAN_POINT('Ctrl Pts',(-21.6993093477804,14.081653901287,129.947257582405)) ;
#137513=CARTESIAN_POINT('Ctrl Pts',(-21.7543881862704,14.2612879476329,
130.141148761343)) ;
#137514=CARTESIAN_POINT('Ctrl Pts',(-21.8227956619766,14.38176341734,130.374105622269)) ;
#137515=CARTESIAN_POINT('Ctrl Pts',(-21.8989363667567,14.4336477337376,
130.629729117928)) ;
#137516=CARTESIAN_POINT('Ctrl Pts',(-21.9765152606609,14.4124734002023,
130.889599388047)) ;
#137517=CARTESIAN_POINT('Ctrl Pts',(-22.0483877837567,14.3214777532126,
131.132438584826)) ;
#137518=CARTESIAN_POINT('Ctrl Pts',(-22.1102442273107,14.1652192668134,
131.34638096803)) ;
#137519=CARTESIAN_POINT('Ctrl Pts',(-22.1558537131498,13.9555650448247,
131.512795439526)) ;
#137520=CARTESIAN_POINT('Ctrl Pts',(-22.1814091769848,13.7095599731385,
131.620407563)) ;
#137521=CARTESIAN_POINT('Ctrl Pts',(-22.1846084318414,13.4405995134717,
131.66302940788)) ;
#137522=CARTESIAN_POINT('Ctrl Pts',(-22.1641410813746,13.1715077445613,
131.63637428883)) ;
#137523=CARTESIAN_POINT('Ctrl Pts',(-22.1212713726189,12.9214880531583,
131.54412153606)) ;
#137524=CARTESIAN_POINT('Ctrl Pts',(-22.0575394234642,12.7055052901806,
131.391205523699)) ;
#137525=CARTESIAN_POINT('Ctrl Pts',(-21.9777673697123,12.542519660956,131.191170277208)) ;
#137526=CARTESIAN_POINT('Ctrl Pts',(-21.8862402490834,12.4416160246637,
130.956908046475)) ;
#137527=CARTESIAN_POINT('Ctrl Pts',(-21.7883180011064,12.4112449651492,
130.704175247965)) ;
#137528=CARTESIAN_POINT('Ctrl Pts',(-21.6916915206646,12.4537097184138,
130.45497041539)) ;
#137529=CARTESIAN_POINT('Ctrl Pts',(-21.6017839340474,12.5652232692769,
130.225394633114)) ;
#137530=CARTESIAN_POINT('Ctrl Pts',(-21.5242852905658,12.7379440024603,
130.032062311546)) ;
#137531=CARTESIAN_POINT('Ctrl Pts',(-21.4638348212917,12.9603974208925,
129.888644578289)) ;
#137532=CARTESIAN_POINT('Ctrl Pts',(-21.4244019077111,13.2156634379738,
129.806566052762)) ;
#137533=CARTESIAN_POINT('Ctrl Pts',(-21.4079017130301,13.4857933225146,
129.791484741217)) ;
#137534=CARTESIAN_POINT('Ctrl Pts',(-21.4149000703604,13.7522945834018,
129.845154416319)) ;
#137535=CARTESIAN_POINT('Ctrl Pts',(-21.4441925744404,13.9943543864371,
129.96386451108)) ;
#137536=CARTESIAN_POINT('Ctrl Pts',(-21.4925040843012,14.1947045665703,
130.137957931616)) ;
#137537=CARTESIAN_POINT('Ctrl Pts',(-21.5566005957734,14.341452901732,130.358505717863)) ;
#137538=CARTESIAN_POINT('Ctrl Pts',(-21.6300619513567,14.4211242912775,
130.606132041837)) ;
#137539=CARTESIAN_POINT('Ctrl Pts',(-21.7074195269614,14.4300014441918,
130.865166461581)) ;
#137540=CARTESIAN_POINT('Ctrl Pts',(-21.782739862899,14.3664766103849,131.118399093227)) ;
#137541=CARTESIAN_POINT('Ctrl Pts',(-21.8492962143774,14.2356053057405,
131.345912604585)) ;
#137542=CARTESIAN_POINT('Ctrl Pts',(-21.9019742543641,14.0463421699273,
131.532943707079)) ;
#137543=CARTESIAN_POINT('Ctrl Pts',(-21.9360655876364,13.8127313116574,
131.665625433991)) ;
#137544=CARTESIAN_POINT('Ctrl Pts',(-21.9485792452769,13.5514862656321,
131.735251200451)) ;
#137545=CARTESIAN_POINT('Ctrl Pts',(-21.9377331317714,13.2797432937496,
131.736799208666)) ;
#137546=CARTESIAN_POINT('Ctrl Pts',(-21.9037118572088,13.0196142656872,
131.670476580031)) ;
#137547=CARTESIAN_POINT('Ctrl Pts',(-21.848095759366,12.7876902930479,131.541159383157)) ;
#137548=CARTESIAN_POINT('Ctrl Pts',(-21.774212667836,12.601531820227,131.358452186942)) ;
#137549=CARTESIAN_POINT('Ctrl Pts',(-21.6866886351043,12.4742597851615,
131.135876049528)) ;
#137550=CARTESIAN_POINT('Ctrl Pts',(-21.5909295194249,12.4148459828286,
130.889268624499)) ;
#137551=CARTESIAN_POINT('Ctrl Pts',(-21.4930969827498,12.4277167902933,
130.63661588948)) ;
#137552=CARTESIAN_POINT('Ctrl Pts',(-21.3995555315845,12.5119511239392,
130.396485892115)) ;
#137553=CARTESIAN_POINT('Ctrl Pts',(-21.3162990844251,12.6612550507726,
130.186368956131)) ;
#137554=CARTESIAN_POINT('Ctrl Pts',(-21.2483839343844,12.8654797343675,
130.021126795539)) ;
#137555=CARTESIAN_POINT('Ctrl Pts',(-21.2002270894872,13.1088715380583,
129.913494497197)) ;
#137556=CARTESIAN_POINT('Ctrl Pts',(-21.1742080824271,13.3752798477322,
129.870610368109)) ;
#137557=CARTESIAN_POINT('Ctrl Pts',(-21.1717085434086,13.6458119714847,
129.89651662008)) ;
#137558=CARTESIAN_POINT('Ctrl Pts',(-21.1921257233827,13.8994657965604,
129.989254351832)) ;
#137559=CARTESIAN_POINT('Ctrl Pts',(-21.233245209048,14.1192748903921,130.142500293083)) ;
#137560=CARTESIAN_POINT('Ctrl Pts',(-21.2914251747259,14.289180306213,130.345585373604)) ;
#137561=CARTESIAN_POINT('Ctrl Pts',(-21.3616961232879,14.3970324953059,
130.583966718822)) ;
#137562=CARTESIAN_POINT('Ctrl Pts',(-21.4384087866577,14.4351164743851,
130.841195428719)) ;
#137563=CARTESIAN_POINT('Ctrl Pts',(-21.5151210055013,14.4010787676098,
131.098338089324)) ;
#137564=CARTESIAN_POINT('Ctrl Pts',(-21.5863960251658,14.2958209234975,
131.339908880083)) ;
#137565=CARTESIAN_POINT('Ctrl Pts',(-21.6449304989321,14.1296521766069,
131.543828654143)) ;
#137566=CARTESIAN_POINT('Ctrl Pts',(-21.6871346231113,13.9121761436852,
131.700257800473)) ;
#137567=CARTESIAN_POINT('Ctrl Pts',(-21.7086771478897,13.659430364987,131.796334004922)) ;
#137568=CARTESIAN_POINT('Ctrl Pts',(-21.7075047728149,13.3906473352246,
131.825945739935)) ;
#137569=CARTESIAN_POINT('Ctrl Pts',(-21.6825267550966,13.12154860475,131.786357720267)) ;
#137570=CARTESIAN_POINT('Ctrl Pts',(-21.6355924854869,12.8774995309081,
131.682170944537)) ;
#137571=CARTESIAN_POINT('Ctrl Pts',(-21.5684160783297,12.6702279872938,
131.519185241917)) ;
#137572=CARTESIAN_POINT('Ctrl Pts',(-21.4860950112321,12.5183910771853,
131.311688639648)) ;
#137573=CARTESIAN_POINT('Ctrl Pts',(-21.3928599529137,12.4302683284587,
131.072491120113)) ;
#137574=CARTESIAN_POINT('Ctrl Pts',(-21.2947906658205,12.4138255810916,
130.819247899391)) ;
#137575=CARTESIAN_POINT('Ctrl Pts',(-21.1993133837603,12.469284941687,130.5732787841)) ;
#137576=CARTESIAN_POINT('Ctrl Pts',(-21.111045383612,12.5930867722267,130.348576358499)) ;
#137577=CARTESIAN_POINT('Ctrl Pts',(-21.0361572295438,12.7771358580158,
130.163027615693)) ;
#137578=CARTESIAN_POINT('Ctrl Pts',(-20.9797275916326,13.0059648630076,
130.031178709991)) ;
#137579=CARTESIAN_POINT('Ctrl Pts',(-20.9443527411009,13.266147051347,129.961050822874)) ;
#137580=CARTESIAN_POINT('Ctrl Pts',(-20.9323325930837,13.536990507266,129.959060513734)) ;
#137581=CARTESIAN_POINT('Ctrl Pts',(-20.9436543105165,13.7997447814263,
130.025277225395)) ;
#137582=CARTESIAN_POINT('Ctrl Pts',(-20.9766477952397,14.0350782594662,
130.154719818596)) ;
#137583=CARTESIAN_POINT('Ctrl Pts',(-21.0287127379786,14.2276700254763,
130.3400969056)) ;
#137584=CARTESIAN_POINT('Ctrl Pts',(-21.0943520323041,14.3610390583721,
130.564758598525)) ;
#137585=CARTESIAN_POINT('Ctrl Pts',(-21.1694845733918,14.4285213443226,
130.817501137148)) ;
#137586=CARTESIAN_POINT('Ctrl Pts',(-21.2469270728871,14.4233691665642,
131.076802064509)) ;
#137587=CARTESIAN_POINT('Ctrl Pts',(-21.320899695783,14.3469901017567,131.325999762253)) ;
#137588=CARTESIAN_POINT('Ctrl Pts',(-21.3855341560455,14.2034040422047,
131.548081815734)) ;
#137589=CARTESIAN_POINT('Ctrl Pts',(-21.4347256418351,14.0056848767319,
131.724728264946)) ;
#137590=CARTESIAN_POINT('Ctrl Pts',(-21.465092607587,13.7644936141034,131.846677236872)) ;
#137591=CARTESIAN_POINT('Ctrl Pts',(-21.4732444413167,13.5002464496988,
131.903523955919)) ;
#137592=CARTESIAN_POINT('Ctrl Pts',(-21.4578324144306,13.2284058869682,
131.891809873456)) ;
#137593=CARTESIAN_POINT('Ctrl Pts',(-21.4198290919617,12.9739038042497,
131.813645652512)) ;
#137594=CARTESIAN_POINT('Ctrl Pts',(-21.3602690958964,12.748470453343,131.672940766185)) ;
#137595=CARTESIAN_POINT('Ctrl Pts',(-21.2837438582424,12.5731123494061,
131.482377603287)) ;
#137596=CARTESIAN_POINT('Ctrl Pts',(-21.1936880421902,12.4573590885892,
131.252613188665)) ;
#137597=CARTESIAN_POINT('Ctrl Pts',(-21.0974470732546,12.4118025442917,
131.004458624852)) ;
#137598=CARTESIAN_POINT('Ctrl Pts',(-20.9999957475628,12.4381298230363,
130.752902669264)) ;
#137599=CARTESIAN_POINT('Ctrl Pts',(-20.9078518526991,12.5352056579817,
130.516875210043)) ;
#137600=CARTESIAN_POINT('Ctrl Pts',(-20.8269544230574,12.6963006078304,
130.313742235523)) ;
#137601=CARTESIAN_POINT('Ctrl Pts',(-20.7626803376973,12.9082756117234,
130.15899041196)) ;
#137602=CARTESIAN_POINT('Ctrl Pts',(-20.7182259000088,13.1596325354774,
130.062478814741)) ;
#137603=CARTESIAN_POINT('Ctrl Pts',(-20.6968797595826,13.4259468867853,
130.032958383663)) ;
#137604=CARTESIAN_POINT('Ctrl Pts',(-20.6987180598139,13.6953761022081,
130.071595056294)) ;
#137605=CARTESIAN_POINT('Ctrl Pts',(-20.7232215568337,13.9437170228922,
130.176233244644)) ;
#137606=CARTESIAN_POINT('Ctrl Pts',(-20.767971164486,14.1557110770192,130.340160815693)) ;
#137607=CARTESIAN_POINT('Ctrl Pts',(-20.8287309225785,14.3144000142637,
130.550712718952)) ;
#137608=CARTESIAN_POINT('Ctrl Pts',(-20.9006919276648,14.4096307818779,
130.794052371241)) ;
#137609=CARTESIAN_POINT('Ctrl Pts',(-20.9778182880555,14.4343455417677,
131.052440775311)) ;
#137610=CARTESIAN_POINT('Ctrl Pts',(-21.0544154691547,14.3860725443644,
131.309506234514)) ;
#137611=CARTESIAN_POINT('Ctrl Pts',(-21.1230945083084,14.2695097476577,
131.543118119901)) ;
#137612=CARTESIAN_POINT('Ctrl Pts',(-21.179301480217,14.0917908235827,131.740489361359)) ;
#137613=CARTESIAN_POINT('Ctrl Pts',(-21.2177234690881,13.8666927964708,
131.885799826201)) ;
#137614=CARTESIAN_POINT('Ctrl Pts',(-21.2351412575897,13.6093229660632,
131.969833893824)) ;
#137615=CARTESIAN_POINT('Ctrl Pts',(-21.2294450096949,13.3388432839998,
131.986311133137)) ;
#137616=CARTESIAN_POINT('Ctrl Pts',(-21.2003261125768,13.0740475195294,
131.934408442014)) ;
#137617=CARTESIAN_POINT('Ctrl Pts',(-21.1490766645565,12.8343947236294,
131.817855849607)) ;
#137618=CARTESIAN_POINT('Ctrl Pts',(-21.079117586523,12.6378260096104,131.646478866635)) ;
#137619=CARTESIAN_POINT('Ctrl Pts',(-20.9940307650976,12.496463053358,131.431074246898)) ;
#137620=CARTESIAN_POINT('Ctrl Pts',(-20.8995453725939,12.4217254212934,
131.188184304878)) ;
#137621=CARTESIAN_POINT('Ctrl Pts',(-20.8016533511348,12.4187226067802,
130.935348047491)) ;
#137622=CARTESIAN_POINT('Ctrl Pts',(-20.7067290384026,12.4875916105364,
130.691149701073)) ;
#137623=CARTESIAN_POINT('Ctrl Pts',(-20.6206591273952,12.6235711646796,
130.472855830561)) ;
#137624=CARTESIAN_POINT('Ctrl Pts',(-20.5490501305615,12.8167006668533,
130.296777642181)) ;
#137625=CARTESIAN_POINT('Ctrl Pts',(-20.496178051986,13.0534699877681,130.175467508203)) ;
#137626=CARTESIAN_POINT('Ctrl Pts',(-20.4652082763484,13.316652871898,130.118125632978)) ;
#137627=CARTESIAN_POINT('Ctrl Pts',(-20.4575910264854,13.5871780619914,
130.128970220053)) ;
#137628=CARTESIAN_POINT('Ctrl Pts',(-20.4730839064674,13.8461109459276,
130.207338015546)) ;
#137629=CARTESIAN_POINT('Ctrl Pts',(-20.5100737122391,14.0754122507699,
130.348613835523)) ;
#137630=CARTESIAN_POINT('Ctrl Pts',(-20.5648370930962,14.2569964936062,
130.541657854969)) ;
#137631=CARTESIAN_POINT('Ctrl Pts',(-20.6329413594287,14.3792169088182,
130.773722810003)) ;
#137632=CARTESIAN_POINT('Ctrl Pts',(-20.7087226220765,14.4330645733332,
131.028200436973)) ;
#137633=CARTESIAN_POINT('Ctrl Pts',(-20.7863398371565,14.4142942248449,
131.288175280098)) ;
#137634=CARTESIAN_POINT('Ctrl Pts',(-20.8587443892862,14.3249818846189,
131.532699501629)) ;
#137635=CARTESIAN_POINT('Ctrl Pts',(-20.9209779259209,14.170040968278,131.747774216565)) ;
#137636=CARTESIAN_POINT('Ctrl Pts',(-20.9669011427084,13.9629929132432,
131.914918567305)) ;
#137637=CARTESIAN_POINT('Ctrl Pts',(-20.9932272956991,13.716497262182,132.024969893988)) ;
#137638=CARTESIAN_POINT('Ctrl Pts',(-20.9970536036366,13.4493823964161,
132.069231580467)) ;
#137639=CARTESIAN_POINT('Ctrl Pts',(-20.9773681367216,13.1794660173532,
132.044927528063)) ;
#137640=CARTESIAN_POINT('Ctrl Pts',(-20.9348193274938,12.9274139550297,
131.953787995804)) ;
#137641=CARTESIAN_POINT('Ctrl Pts',(-20.8719669700059,12.7115777182511,
131.803243101651)) ;
#137642=CARTESIAN_POINT('Ctrl Pts',(-20.7926171746203,12.5463884321844,
131.604472050351)) ;
#137643=CARTESIAN_POINT('Ctrl Pts',(-20.7005656856551,12.4431786925169,
131.36894206665)) ;
#137644=CARTESIAN_POINT('Ctrl Pts',(-20.6037919880621,12.4112124579401,
131.119195085756)) ;
#137645=CARTESIAN_POINT('Ctrl Pts',(-20.5066772839954,12.4513454594276,
130.868694657424)) ;
#137646=CARTESIAN_POINT('Ctrl Pts',(-20.4165141092168,12.5610016830577,
130.638362595368)) ;
#137647=CARTESIAN_POINT('Ctrl Pts',(-20.3384849755394,12.7322315169158,
130.443517766448)) ;
#137648=CARTESIAN_POINT('Ctrl Pts',(-20.2774709313571,12.953682166373,130.2984736935)) ;
#137649=CARTESIAN_POINT('Ctrl Pts',(-20.2374795071584,13.207709520667,130.214695903395)) ;
#137650=CARTESIAN_POINT('Ctrl Pts',(-20.2202513164256,13.477838949959,130.19750736579)) ;
#137651=CARTESIAN_POINT('Ctrl Pts',(-20.2266080907571,13.7447249701473,
130.249306408078)) ;
#137652=CARTESIAN_POINT('Ctrl Pts',(-20.2551147268125,13.9871378811425,
130.365615989591)) ;
#137653=CARTESIAN_POINT('Ctrl Pts',(-20.3032561348622,14.1900736221216,
130.539429290487)) ;
#137654=CARTESIAN_POINT('Ctrl Pts',(-20.366375984174,14.3373317370972,130.756810802034)) ;
#137655=CARTESIAN_POINT('Ctrl Pts',(-20.4400778737823,14.4199335161434,
131.005366056279)) ;
#137656=CARTESIAN_POINT('Ctrl Pts',(-20.517398884963,14.4307824011819,131.264277739086)) ;
#137657=CARTESIAN_POINT('Ctrl Pts',(-20.593060063551,14.3690285687369,131.518596966109)) ;
#137658=CARTESIAN_POINT('Ctrl Pts',(-20.6596542407766,14.240441055026,131.746082495927)) ;
#137659=CARTESIAN_POINT('Ctrl Pts',(-20.7128484353568,14.0528077050883,
131.934627680386)) ;
#137660=CARTESIAN_POINT('Ctrl Pts',(-20.7475784142269,13.8202656328653,
132.069181756592)) ;
#137661=CARTESIAN_POINT('Ctrl Pts',(-20.7607767450837,13.5584446016604,
132.140947553018)) ;
#137662=CARTESIAN_POINT('Ctrl Pts',(-20.7505287005013,13.2871051677591,
132.144192204044)) ;
#137663=CARTESIAN_POINT('Ctrl Pts',(-20.7172718444425,13.0271137580964,
132.080012631234)) ;
#137664=CARTESIAN_POINT('Ctrl Pts',(-20.662202991394,12.7938648791111,131.952326610137)) ;
#137665=CARTESIAN_POINT('Ctrl Pts',(-20.5888877956183,12.6063348860961,
131.771239179103)) ;
#137666=CARTESIAN_POINT('Ctrl Pts',(-20.5015478328552,12.4770288288764,
131.549255832687)) ;
#137667=CARTESIAN_POINT('Ctrl Pts',(-20.4062249604456,12.4155889254397,
131.303824104185)) ;
#137668=CARTESIAN_POINT('Ctrl Pts',(-20.3079159542625,12.4264045620756,
131.049934819456)) ;
#137669=CARTESIAN_POINT('Ctrl Pts',(-20.2145031376508,12.5084012335638,
130.810058284156)) ;
#137670=CARTESIAN_POINT('Ctrl Pts',(-20.1306995642403,12.6562045204938,
130.598414583344)) ;
#137671=CARTESIAN_POINT('Ctrl Pts',(-20.0624739819763,12.8582527624523,
130.432148065107)) ;
#137672=CARTESIAN_POINT('Ctrl Pts',(-20.0133566463447,13.1022479915201,
130.321924077519)) ;
#137673=CARTESIAN_POINT('Ctrl Pts',(-19.9868280658771,13.3685510945704,
130.277573143074)) ;
#137674=CARTESIAN_POINT('Ctrl Pts',(-19.9836603277551,13.6374690116671,
130.301308492192)) ;
#137675=CARTESIAN_POINT('Ctrl Pts',(-20.0034420277648,13.8926337185126,
130.392287293504)) ;
#137676=CARTESIAN_POINT('Ctrl Pts',(-20.0439943690178,14.1134973759114,
130.543852003553)) ;
#137677=CARTESIAN_POINT('Ctrl Pts',(-20.1019010050305,14.2854804463777,
130.746225783846)) ;
#137678=CARTESIAN_POINT('Ctrl Pts',(-20.1719255332864,14.3949169663802,
130.983882406649)) ;
#137679=CARTESIAN_POINT('Ctrl Pts',(-20.248213487577,14.4350950477778,131.239727536652)) ;
#137680=CARTESIAN_POINT('Ctrl Pts',(-20.3254463492532,14.4027523557503,
131.498591864264)) ;
#137681=CARTESIAN_POINT('Ctrl Pts',(-20.396382333849,14.3004224268776,131.738877616431)) ;
#137682=CARTESIAN_POINT('Ctrl Pts',(-20.45588703209,14.1345848166218,131.945929948589)) ;
#137683=CARTESIAN_POINT('Ctrl Pts',(-20.4983986905152,13.9188292644318,
132.103144456355)) ;
#137684=CARTESIAN_POINT('Ctrl Pts',(-20.5206054593495,13.6668968300226,
132.201163345285)) ;
#137685=CARTESIAN_POINT('Ctrl Pts',(-20.5200422127212,13.3982258229591,
132.232566609447)) ;
#137686=CARTESIAN_POINT('Ctrl Pts',(-20.4959120705654,13.1299460140076,
132.195305612606)) ;
#137687=CARTESIAN_POINT('Ctrl Pts',(-20.4493854866592,12.883706046321,132.092482303726)) ;
#137688=CARTESIAN_POINT('Ctrl Pts',(-20.3827956444432,12.6755091493533,
131.931155444613)) ;
#137689=CARTESIAN_POINT('Ctrl Pts',(-20.3007023283114,12.5215778727762,
131.724390139687)) ;
#137690=CARTESIAN_POINT('Ctrl Pts',(-20.2075018171708,12.4317802296238,
131.485347148361)) ;
#137691=CARTESIAN_POINT('Ctrl Pts',(-20.1103254681884,12.4131805085562,
131.234422161529)) ;
#137692=CARTESIAN_POINT('Ctrl Pts',(-20.0139320775133,12.4668842419267,
130.986048105159)) ;
#137693=CARTESIAN_POINT('Ctrl Pts',(-19.9257741902488,12.5884449970434,
130.76151375573)) ;
#137694=CARTESIAN_POINT('Ctrl Pts',(-19.8502049393805,12.7713420307832,
130.574069477332)) ;
#137695=CARTESIAN_POINT('Ctrl Pts',(-19.793268697052,12.9988617172705,130.44070264408)) ;
#137696=CARTESIAN_POINT('Ctrl Pts',(-19.757165794996,13.2594912156624,130.368579354002)) ;
#137697=CARTESIAN_POINT('Ctrl Pts',(-19.7446008853565,13.528913215532,130.364828114744)) ;
#137698=CARTESIAN_POINT('Ctrl Pts',(-19.7551763127313,13.7920446626032,
130.428843415922)) ;
#137699=CARTESIAN_POINT('Ctrl Pts',(-19.7876094727285,14.0286822474636,
130.556687451896)) ;
#137700=CARTESIAN_POINT('Ctrl Pts',(-19.8390978347557,14.2226476411148,
130.740339467478)) ;
#137701=CARTESIAN_POINT('Ctrl Pts',(-19.9045962847081,14.3581279629795,
130.964687569436)) ;
#137702=CARTESIAN_POINT('Ctrl Pts',(-19.9791897742387,14.4275172103506,
131.215693011947)) ;
#137703=CARTESIAN_POINT('Ctrl Pts',(-20.0572472309711,14.4244373538993,
131.477053037658)) ;
#137704=CARTESIAN_POINT('Ctrl Pts',(-20.1309835390558,14.3501368659966,
131.72538106024)) ;
#137705=CARTESIAN_POINT('Ctrl Pts',(-20.1958863249354,14.2089998659338,
131.948172797202)) ;
#137706=CARTESIAN_POINT('Ctrl Pts',(-20.2457715176204,14.0121252002097,
132.126956829028)) ;
#137707=CARTESIAN_POINT('Ctrl Pts',(-20.2767468394311,13.771824837408,132.250689691059)) ;
#137708=CARTESIAN_POINT('Ctrl Pts',(-20.2855151937684,13.5078187869416,
132.309363670343)) ;
#137709=CARTESIAN_POINT('Ctrl Pts',(-20.2709382772913,13.2372790594901,
132.29991113471)) ;
#137710=CARTESIAN_POINT('Ctrl Pts',(-20.2333968985353,12.9804327969093,
132.223307498601)) ;
#137711=CARTESIAN_POINT('Ctrl Pts',(-20.1743352916517,12.7540239326364,
132.084048582146)) ;
#137712=CARTESIAN_POINT('Ctrl Pts',(-20.0983730228796,12.5774627760268,
131.895074679153)) ;
#137713=CARTESIAN_POINT('Ctrl Pts',(-20.0088178169133,12.4598743078943,
131.666703703983)) ;
#137714=CARTESIAN_POINT('Ctrl Pts',(-19.9122599860254,12.4120040784052,
131.41777242998)) ;
#137715=CARTESIAN_POINT('Ctrl Pts',(-19.8148042629863,12.4365719244432,
131.166187081806)) ;
#137716=CARTESIAN_POINT('Ctrl Pts',(-19.7227956012826,12.5311793554758,
130.930416460681)) ;
#137717=CARTESIAN_POINT('Ctrl Pts',(-19.6411874345405,12.6910252858477,
130.725320832536)) ;
#137718=CARTESIAN_POINT('Ctrl Pts',(-19.5765629416592,12.9015545976397,
130.569498377236)) ;
#137719=CARTESIAN_POINT('Ctrl Pts',(-19.5315753841879,13.1503193803916,
130.471219010104)) ;
#137720=CARTESIAN_POINT('Ctrl Pts',(-19.5093124096303,13.4198238208766,
130.439454333555)) ;
#137721=CARTESIAN_POINT('Ctrl Pts',(-19.5105321036796,13.6867201897118,
130.475929754006)) ;
#137722=CARTESIAN_POINT('Ctrl Pts',(-19.5344899978628,13.9376559886512,
130.579206334042)) ;
#137723=CARTESIAN_POINT('Ctrl Pts',(-19.5786625804763,14.15024285779,130.741353841934)) ;
#137724=CARTESIAN_POINT('Ctrl Pts',(-19.6390835815084,14.3108380618515,
130.95096108692)) ;
#137725=CARTESIAN_POINT('Ctrl Pts',(-19.710796343946,14.4079445273837,131.193561999246)) ;
#137726=CARTESIAN_POINT('Ctrl Pts',(-19.7879385451593,14.4345276708083,
131.452034692613)) ;
#137727=CARTESIAN_POINT('Ctrl Pts',(-19.8641423507794,14.3888298887491,
131.707720589177)) ;
#137728=CARTESIAN_POINT('Ctrl Pts',(-19.9334963492316,14.2738285073071,
131.943474886351)) ;
#137729=CARTESIAN_POINT('Ctrl Pts',(-19.9900753188983,14.0978368978208,
132.141892587942)) ;
#137730=CARTESIAN_POINT('Ctrl Pts',(-20.029142353165,13.873540820756,132.289148752814)) ;
#137731=CARTESIAN_POINT('Ctrl Pts',(-20.0471730607309,13.6168751421622,
132.374962241574)) ;
#137732=CARTESIAN_POINT('Ctrl Pts',(-20.0421398303126,13.3465065043273,
132.39337844358)) ;
#137733=CARTESIAN_POINT('Ctrl Pts',(-20.0137168616045,13.0815409163059,
132.343472421558)) ;
#137734=CARTESIAN_POINT('Ctrl Pts',(-19.9630818029184,12.8409648020749,
132.228711336927)) ;
#137735=CARTESIAN_POINT('Ctrl Pts',(-19.8937037272603,12.6428641094173,
132.059013597505)) ;
#137736=CARTESIAN_POINT('Ctrl Pts',(-19.8082706443675,12.4989647241715,
131.842851496796)) ;
#137737=CARTESIAN_POINT('Ctrl Pts',(-19.7148222298413,12.423107716889,131.602682335525)) ;
#137738=CARTESIAN_POINT('Ctrl Pts',(-19.6165590013728,12.4177381354183,
131.34889731826)) ;
#137739=CARTESIAN_POINT('Ctrl Pts',(-19.5215312608125,12.4847094665518,
131.104373207812)) ;
#137740=CARTESIAN_POINT('Ctrl Pts',(-19.4350279161659,12.6190666936061,
130.884854431054)) ;
#137741=CARTESIAN_POINT('Ctrl Pts',(-19.3630156634519,12.8107470171755,
130.707580165133)) ;
#137742=CARTESIAN_POINT('Ctrl Pts',(-19.3096393875782,13.046104708988,130.584743629659)) ;
#137743=CARTESIAN_POINT('Ctrl Pts',(-19.2779861809298,13.3089102809665,
130.525423125906)) ;
#137744=CARTESIAN_POINT('Ctrl Pts',(-19.2696835204742,13.5795916473862,
130.534276424891)) ;
#137745=CARTESIAN_POINT('Ctrl Pts',(-19.2846166337307,13.8398547760041,
130.611106017032)) ;
#137746=CARTESIAN_POINT('Ctrl Pts',(-19.3210881365978,14.0698648400938,
130.750835724147)) ;
#137747=CARTESIAN_POINT('Ctrl Pts',(-19.3752206498596,14.2524395531566,
130.941933848175)) ;
#137748=CARTESIAN_POINT('Ctrl Pts',(-19.443181843827,14.3767942781604,131.173660667841)) ;
#137749=CARTESIAN_POINT('Ctrl Pts',(-19.5186387491627,14.4324209526977,
131.42710546284)) ;
#137750=CARTESIAN_POINT('Ctrl Pts',(-19.5962340512703,14.4159981333991,
131.686985719429)) ;
#137751=CARTESIAN_POINT('Ctrl Pts',(-19.6690951170259,14.3283155565982,
131.93295372937)) ;
#137752=CARTESIAN_POINT('Ctrl Pts',(-19.731498600517,14.1755659528296,132.148414877089)) ;
#137753=CARTESIAN_POINT('Ctrl Pts',(-19.7780133273736,13.9699068567355,
132.317303495422)) ;
#137754=CARTESIAN_POINT('Ctrl Pts',(-19.8049862544587,13.7239840394015,
132.42928569716)) ;
#137755=CARTESIAN_POINT('Ctrl Pts',(-19.809515235663,13.4571373132025,132.475606075713)) ;
#137756=CARTESIAN_POINT('Ctrl Pts',(-19.7903204177427,13.1860385292999,
132.45286442784)) ;
#137757=CARTESIAN_POINT('Ctrl Pts',(-19.7487646879107,12.9351633483058,
132.364359945624)) ;
#137758=CARTESIAN_POINT('Ctrl Pts',(-19.6859631867643,12.7162804285951,
132.21423823404)) ;
#137759=CARTESIAN_POINT('Ctrl Pts',(-19.6073342675828,12.5504602957499,
132.017412800741)) ;
#137760=CARTESIAN_POINT('Ctrl Pts',(-19.5155082129029,12.445157177056,131.782565908142)) ;
#137761=CARTESIAN_POINT('Ctrl Pts',(-19.4189472179032,12.4110818139133,
131.533391011119)) ;
#137762=CARTESIAN_POINT('Ctrl Pts',(-19.3214401093541,12.4493848627241,
131.281852651979)) ;
#137763=CARTESIAN_POINT('Ctrl Pts',(-19.2314769431166,12.5564279113244,
131.051920666311)) ;
#137764=CARTESIAN_POINT('Ctrl Pts',(-19.1524965061616,12.7270948639173,
130.85451813902)) ;
#137765=CARTESIAN_POINT('Ctrl Pts',(-19.0911924448804,12.9467013244188,
130.708509031209)) ;
#137766=CARTESIAN_POINT('Ctrl Pts',(-19.0504665817876,13.2005745310841,
130.622663698416)) ;
#137767=CARTESIAN_POINT('Ctrl Pts',(-19.0326836209356,13.4697555759231,
130.603759575917)) ;
#137768=CARTESIAN_POINT('Ctrl Pts',(-19.0382102244379,13.7362551955502,
130.653023431916)) ;
#137769=CARTESIAN_POINT('Ctrl Pts',(-19.0663557867909,13.9814041489959,
130.76853786842)) ;
#137770=CARTESIAN_POINT('Ctrl Pts',(-19.1136199928099,14.1841666435664,
130.939526111425)) ;
#137771=CARTESIAN_POINT('Ctrl Pts',(-19.1767577967624,14.3343211623714,
131.15719018996)) ;
#137772=CARTESIAN_POINT('Ctrl Pts',(-19.2500366332053,14.418455096693,131.404394753815)) ;
#137773=CARTESIAN_POINT('Ctrl Pts',(-19.3273692986292,14.4314520041057,
131.663366130815)) ;
#137774=CARTESIAN_POINT('Ctrl Pts',(-19.4028774363666,14.3721435581282,
131.917097822485)) ;
#137775=CARTESIAN_POINT('Ctrl Pts',(-19.4700541032919,14.2453739060394,
132.146382805055)) ;
#137776=CARTESIAN_POINT('Ctrl Pts',(-19.5239307336061,14.0581567741166,
132.337084920621)) ;
#137777=CARTESIAN_POINT('Ctrl Pts',(-19.5590167477845,13.8276969055429,
132.472521311396)) ;
#137778=CARTESIAN_POINT('Ctrl Pts',(-19.5729299943671,13.5670204809412,
132.54631437139)) ;
#137779=CARTESIAN_POINT('Ctrl Pts',(-19.5634175629659,13.2953787817414,
132.551745553635)) ;
#137780=CARTESIAN_POINT('Ctrl Pts',(-19.5307814551787,13.0342215951602,
132.489449839042)) ;
#137781=CARTESIAN_POINT('Ctrl Pts',(-19.4760249872077,12.7992353621788,
132.362794033766)) ;
#137782=CARTESIAN_POINT('Ctrl Pts',(-19.4035773877406,12.6113833751158,
132.184049216232)) ;
#137783=CARTESIAN_POINT('Ctrl Pts',(-19.3165223036231,12.4798504311987,
131.962931933643)) ;
#137784=CARTESIAN_POINT('Ctrl Pts',(-19.2211653039383,12.4163978737343,
131.717463870116)) ;
#137785=CARTESIAN_POINT('Ctrl Pts',(-19.1231585738506,12.4249214769568,
131.464343284139)) ;
#137786=CARTESIAN_POINT('Ctrl Pts',(-19.0290644089191,12.5053755581291,
131.222650125226)) ;
#137787=CARTESIAN_POINT('Ctrl Pts',(-18.945316002603,12.6507858524343,131.011003544665)) ;
#137788=CARTESIAN_POINT('Ctrl Pts',(-18.8763895924228,12.8517470379754,
130.84276469136)) ;
#137789=CARTESIAN_POINT('Ctrl Pts',(-18.8267448309181,13.0945613893121,
130.730961303292)) ;
#137790=CARTESIAN_POINT('Ctrl Pts',(-18.7994718959822,13.3602125815229,
130.684409044151)) ;
#137791=CARTESIAN_POINT('Ctrl Pts',(-18.7956758360037,13.6310671509035,
130.706531095789)) ;
#137792=CARTESIAN_POINT('Ctrl Pts',(-18.8147674164781,13.8852753501133,
130.79528480511)) ;
#137793=CARTESIAN_POINT('Ctrl Pts',(-18.8547365620153,14.1076160518456,
130.945173100413)) ;
#137794=CARTESIAN_POINT('Ctrl Pts',(-18.9120865572062,14.2808806548592,
131.145853438459)) ;
#137795=CARTESIAN_POINT('Ctrl Pts',(-18.9817798655855,14.3926567066995,
131.382539424301)) ;
#137796=CARTESIAN_POINT('Ctrl Pts',(-19.0585628808164,14.4348969494453,
131.640089890739)) ;
#137797=CARTESIAN_POINT('Ctrl Pts',(-19.1351376242844,14.4049966963277,
131.896703997414)) ;
#137798=CARTESIAN_POINT('Ctrl Pts',(-19.2069795117691,14.303792887026,132.139944585753)) ;
#137799=CARTESIAN_POINT('Ctrl Pts',(-19.2664511487555,14.1405203843961,
132.346669416583)) ;
#137800=CARTESIAN_POINT('Ctrl Pts',(-19.3096417752548,13.925819103477,132.505934041616)) ;
#137801=CARTESIAN_POINT('Ctrl Pts',(-19.3325065328025,13.6747404913737,
132.605860844122)) ;
#137802=CARTESIAN_POINT('Ctrl Pts',(-19.332541849949,13.4052256729127,132.639149944979)) ;
#137803=CARTESIAN_POINT('Ctrl Pts',(-19.3092812735878,13.1384692552609,
132.604191768055)) ;
#137804=CARTESIAN_POINT('Ctrl Pts',(-19.2631063121014,12.8897551675282,
132.502613781544)) ;
#137805=CARTESIAN_POINT('Ctrl Pts',(-19.1973582392372,12.6813708112152,
132.343566871807)) ;
#137806=CARTESIAN_POINT('Ctrl Pts',(-19.1155604461688,12.5252896551219,
132.137725194002)) ;
#137807=CARTESIAN_POINT('Ctrl Pts',(-19.0228059236477,12.4335762169434,
131.899908767192)) ;
#137808=CARTESIAN_POINT('Ctrl Pts',(-18.925357266948,12.4126069646067,131.64830074567)) ;
#137809=CARTESIAN_POINT('Ctrl Pts',(-18.8285810937,12.4645413585742,131.398893890923)) ;
#137810=CARTESIAN_POINT('Ctrl Pts',(-18.740157757668,12.5845282308657,131.173590439064)) ;
#137811=CARTESIAN_POINT('Ctrl Pts',(-18.6643847827615,12.7652450506007,
130.985436414686)) ;
#137812=CARTESIAN_POINT('Ctrl Pts',(-18.6067882108563,12.9922346613826,
130.850221426745)) ;
#137813=CARTESIAN_POINT('Ctrl Pts',(-18.5702632954388,13.250181771579,130.776605389314)) ;
#137814=CARTESIAN_POINT('Ctrl Pts',(-18.5568044283898,13.5208712081626,
130.770411334257)) ;
#137815=CARTESIAN_POINT('Ctrl Pts',(-18.5668006964617,13.7852947823376,
130.832834130771)) ;
#137816=CARTESIAN_POINT('Ctrl Pts',(-18.5987394298108,14.0230293048616,
130.959264121613)) ;
#137817=CARTESIAN_POINT('Ctrl Pts',(-18.6496368762035,14.2178153725244,
131.141101449601)) ;
#137818=CARTESIAN_POINT('Ctrl Pts',(-18.7147914630156,14.3552930120595,
131.364452232031)) ;
#137819=CARTESIAN_POINT('Ctrl Pts',(-18.7895474760606,14.4265292407486,
131.616072894725)) ;
#137820=CARTESIAN_POINT('Ctrl Pts',(-18.8667133662151,14.4257522410885,
131.874439194348)) ;
#137821=CARTESIAN_POINT('Ctrl Pts',(-18.9412988303887,14.3531912390316,
132.125538928334)) ;
#137822=CARTESIAN_POINT('Ctrl Pts',(-19.006381267232,14.2139749778386,132.348774125945)) ;
#137823=CARTESIAN_POINT('Ctrl Pts',(-19.0568528029414,14.0181343967752,
132.529344981123)) ;
#137824=CARTESIAN_POINT('Ctrl Pts',(-19.0883199089333,13.7796846047307,
132.654391142837)) ;
#137825=CARTESIAN_POINT('Ctrl Pts',(-19.0978098271686,13.5155236952114,
132.715257194164)) ;
#137826=CARTESIAN_POINT('Ctrl Pts',(-19.0839141888874,13.2452127497976,
132.707751963834)) ;
#137827=CARTESIAN_POINT('Ctrl Pts',(-19.0470411501845,12.9877059092876,
132.633102744637)) ;
#137828=CARTESIAN_POINT('Ctrl Pts',(-18.9886209994034,12.7602061146998,
132.49569403547)) ;
#137829=CARTESIAN_POINT('Ctrl Pts',(-18.912954495156,12.5817513014504,132.307649978698)) ;
#137830=CARTESIAN_POINT('Ctrl Pts',(-18.823989235305,12.4625557645347,132.080895111837)) ;
#137831=CARTESIAN_POINT('Ctrl Pts',(-18.7274195905187,12.4124303731174,
131.831984343437)) ;
#137832=CARTESIAN_POINT('Ctrl Pts',(-18.6300548105444,12.4345388042572,
131.580601782827)) ;
#137833=CARTESIAN_POINT('Ctrl Pts',(-18.5370135094554,12.5283216388457,
131.342120309818)) ;
#137834=CARTESIAN_POINT('Ctrl Pts',(-18.4559097133117,12.6848122289345,
131.138130709134)) ;
#137835=CARTESIAN_POINT('Ctrl Pts',(-18.3901713005438,12.8954782844364,
130.979318768591)) ;
#137836=CARTESIAN_POINT('Ctrl Pts',(-18.3448005512406,13.1430312169486,
130.879841045138)) ;
#137837=CARTESIAN_POINT('Ctrl Pts',(-18.3218747041718,13.4109716006735,
130.845992375282)) ;
#137838=CARTESIAN_POINT('Ctrl Pts',(-18.3223625152694,13.6794257001286,
130.880484421356)) ;
#137839=CARTESIAN_POINT('Ctrl Pts',(-18.3458072065772,13.9314101129575,
130.982305968587)) ;
#137840=CARTESIAN_POINT('Ctrl Pts',(-18.3893102806117,14.1445006499188,
131.1423845234)) ;
#137841=CARTESIAN_POINT('Ctrl Pts',(-18.4492119247963,14.30675364297,131.350434987214)) ;
#137842=CARTESIAN_POINT('Ctrl Pts',(-18.5207480281994,14.4060487021468,
131.592559699906)) ;
#137843=CARTESIAN_POINT('Ctrl Pts',(-18.5978819309036,14.4348548844435,
131.851031778509)) ;
#137844=CARTESIAN_POINT('Ctrl Pts',(-18.674405910123,14.3909041683382,132.107751135057)) ;
#137845=CARTESIAN_POINT('Ctrl Pts',(-18.7437339428587,14.2783347545864,
132.343276751579)) ;
#137846=CARTESIAN_POINT('Ctrl Pts',(-18.8010355018281,14.1031935593991,
132.54396170515)) ;
#137847=CARTESIAN_POINT('Ctrl Pts',(-18.8405463694835,13.8800104934357,
132.692493251368)) ;
#137848=CARTESIAN_POINT('Ctrl Pts',(-18.859162215355,13.6249527950758,132.779899013047)) ;
#137849=CARTESIAN_POINT('Ctrl Pts',(-18.8548446588266,13.3547990721566,
132.800399354658)) ;
#137850=CARTESIAN_POINT('Ctrl Pts',(-18.827222338478,13.0897727529312,132.752776683914)) ;
#137851=CARTESIAN_POINT('Ctrl Pts',(-18.776916467683,12.8467550013015,132.639173733262)) ;
#137852=CARTESIAN_POINT('Ctrl Pts',(-18.7080316497001,12.6478124741987,
132.470872436135)) ;
#137853=CARTESIAN_POINT('Ctrl Pts',(-18.6236048883295,12.5027972402551,
132.257422574238)) ;
#137854=CARTESIAN_POINT('Ctrl Pts',(-18.5295771589345,12.4240443790735,
132.015841001444)) ;
#137855=CARTESIAN_POINT('Ctrl Pts',(-18.4312698393036,12.4170503512975,
131.761943008889)) ;
#137856=CARTESIAN_POINT('Ctrl Pts',(-18.3364462745014,12.4817913528845,
131.517890812399)) ;
#137857=CARTESIAN_POINT('Ctrl Pts',(-18.2495792781442,12.6142900077789,
131.297317545331)) ;
#137858=CARTESIAN_POINT('Ctrl Pts',(-18.1771702037882,12.8042102941726,
131.118842529841)) ;
#137859=CARTESIAN_POINT('Ctrl Pts',(-18.1230598700679,13.0388185676317,
130.993913398293)) ;
#137860=CARTESIAN_POINT('Ctrl Pts',(-18.0907140204209,13.302328429414,130.932716168419)) ;
#137861=CARTESIAN_POINT('Ctrl Pts',(-18.0818206414082,13.5713413202646,
130.939632216682)) ;
#137862=CARTESIAN_POINT('Ctrl Pts',(-18.0961078605723,13.8329961698972,
131.014678941615)) ;
#137863=CARTESIAN_POINT('Ctrl Pts',(-18.1319332307441,14.0635775985236,
131.152440731558)) ;
#137864=CARTESIAN_POINT('Ctrl Pts',(-18.1856883445983,14.2479536598407,
131.342493359132)) ;
#137865=CARTESIAN_POINT('Ctrl Pts',(-18.2530905010094,14.3739504234545,
131.572475100791)) ;
#137866=CARTESIAN_POINT('Ctrl Pts',(-18.3290310806664,14.4320428147267,
131.827608185542)) ;
#137867=CARTESIAN_POINT('Ctrl Pts',(-18.4064572253342,14.4172275166343,
132.086904527241)) ;
#137868=CARTESIAN_POINT('Ctrl Pts',(-18.4792652025405,14.3318167265824,
132.332603920243)) ;
#137869=CARTESIAN_POINT('Ctrl Pts',(-18.5420198013597,14.1811818661954,
132.549047819145)) ;
#137870=CARTESIAN_POINT('Ctrl Pts',(-18.5892218579538,13.9759968010836,
132.720084196974)) ;
#137871=CARTESIAN_POINT('Ctrl Pts',(-18.6167720804193,13.7313492742168,
132.833691346408)) ;
#137872=CARTESIAN_POINT('Ctrl Pts',(-18.6218292587465,13.4634561374574,
132.881731398093)) ;
#137873=CARTESIAN_POINT('Ctrl Pts',(-18.6036627628578,13.1958849564785,
132.861520033549)) ;
#137874=CARTESIAN_POINT('Ctrl Pts',(-18.5623283084843,12.9412337113468,
132.774062788288)) ;
#137875=CARTESIAN_POINT('Ctrl Pts',(-18.5006384449743,12.7230235201935,
132.626876709527)) ;
#137876=CARTESIAN_POINT('Ctrl Pts',(-18.4217152103521,12.5539648159992,
132.4295120841)) ;
#137877=CARTESIAN_POINT('Ctrl Pts',(-18.3311245557592,12.4477725871464,
132.19791079546)) ;
#137878=CARTESIAN_POINT('Ctrl Pts',(-18.2339496661273,12.4110238125286,
131.947200890198)) ;
#137879=CARTESIAN_POINT('Ctrl Pts',(-18.1368321085862,12.4468710259381,
131.696619131312)) ;
#137880=CARTESIAN_POINT('Ctrl Pts',(-18.0456588191261,12.5531554017273,
131.463507987167)) ;
#137881=CARTESIAN_POINT('Ctrl Pts',(-17.9669224096408,12.7211113672027,
131.26655346719)) ;
#137882=CARTESIAN_POINT('Ctrl Pts',(-17.9048518984378,12.9400020306265,
131.118407374436)) ;
#137883=CARTESIAN_POINT('Ctrl Pts',(-17.863651253699,13.1921120605742,131.031037055592)) ;
#137884=CARTESIAN_POINT('Ctrl Pts',(-17.8450388569388,13.4620045410206,
131.009824678449)) ;
#137885=CARTESIAN_POINT('Ctrl Pts',(-17.8500091814281,13.7292706250682,
131.057520791156)) ;
#137886=CARTESIAN_POINT('Ctrl Pts',(-17.877302446402,13.9738125834417,131.170328613009)) ;
#137887=CARTESIAN_POINT('Ctrl Pts',(-17.9243069985026,14.1794946936577,
131.340779996349)) ;
#137888=CARTESIAN_POINT('Ctrl Pts',(-17.9872121330728,14.3311259021016,
131.557794969855)) ;
#137889=CARTESIAN_POINT('Ctrl Pts',(-18.0598546631151,14.4169205484559,
131.802952666368)) ;
#137890=CARTESIAN_POINT('Ctrl Pts',(-18.1375957078681,14.4320030369242,
132.063314977191)) ;
#137891=CARTESIAN_POINT('Ctrl Pts',(-18.2128346595683,14.3751243958677,
132.316063847586)) ;
#137892=CARTESIAN_POINT('Ctrl Pts',(-18.2809030990878,14.2488768695212,
132.548263675906)) ;
#137893=CARTESIAN_POINT('Ctrl Pts',(-18.3346701612726,14.0648019477406,
132.738317017284)) ;
#137894=CARTESIAN_POINT('Ctrl Pts',(-18.3706065108531,13.8343789431172,
132.876418354214)) ;
#137895=CARTESIAN_POINT('Ctrl Pts',(-18.3850723877934,13.5736072409061,
132.951890561446)) ;
#137896=CARTESIAN_POINT('Ctrl Pts',(-18.3761672531653,13.3025526358433,
132.959029018342)) ;
#137897=CARTESIAN_POINT('Ctrl Pts',(-18.3442712548047,13.0417946956511,
132.898783688445)) ;
#137898=CARTESIAN_POINT('Ctrl Pts',(-18.2903655411103,12.8063141545274,
132.774510267761)) ;
#137899=CARTESIAN_POINT('Ctrl Pts',(-18.2180840269614,12.6158857625783,
132.596412350114)) ;
#137900=CARTESIAN_POINT('Ctrl Pts',(-18.1311881459215,12.4825397359329,
132.375809127955)) ;
#137901=CARTESIAN_POINT('Ctrl Pts',(-18.0362627850358,12.4173081349344,
132.131507312481)) ;
#137902=CARTESIAN_POINT('Ctrl Pts',(-17.9383440031491,12.4236049843711,
131.878609271307)) ;
#137903=CARTESIAN_POINT('Ctrl Pts',(-17.8440809897297,12.5018025571804,
131.636403802442)) ;
#137904=CARTESIAN_POINT('Ctrl Pts',(-17.7596883142505,12.6458565227928,
131.422980744586)) ;
#137905=CARTESIAN_POINT('Ctrl Pts',(-17.6903452885415,12.8453790155913,
131.25350285176)) ;
#137906=CARTESIAN_POINT('Ctrl Pts',(-17.6401750273876,13.0865651955858,
131.140080379431)) ;
#137907=CARTESIAN_POINT('Ctrl Pts',(-17.6121734948375,13.3521426916341,
131.091447534242)) ;
#137908=CARTESIAN_POINT('Ctrl Pts',(-17.6076411176606,13.6222556634887,
131.11130620512)) ;
#137909=CARTESIAN_POINT('Ctrl Pts',(-17.6260946648748,13.8783882532463,
131.198344630055)) ;
#137910=CARTESIAN_POINT('Ctrl Pts',(-17.6656422043345,14.1022120327878,
131.347061644052)) ;
#137911=CARTESIAN_POINT('Ctrl Pts',(-17.7224071623684,14.2765229338953,
131.545938908787)) ;
#137912=CARTESIAN_POINT('Ctrl Pts',(-17.7917189747294,14.3902286899454,
131.781476416858)) ;
#137913=CARTESIAN_POINT('Ctrl Pts',(-17.868504117299,14.4347769429382,132.03908049303)) ;
#137914=CARTESIAN_POINT('Ctrl Pts',(-17.945297953661,14.4066722645431,132.296405177608)) ;
#137915=CARTESIAN_POINT('Ctrl Pts',(-18.0169665014956,14.3082119147666,
132.538929595933)) ;
#137916=CARTESIAN_POINT('Ctrl Pts',(-18.0771757737706,14.1460357865502,
132.747971370351)) ;
#137917=CARTESIAN_POINT('Ctrl Pts',(-18.1208631205668,13.9328084550501,
132.908648173399)) ;
#137918=CARTESIAN_POINT('Ctrl Pts',(-18.1443765191894,13.6817741223337,
133.01057033936)) ;
#137919=CARTESIAN_POINT('Ctrl Pts',(-18.1451355362661,13.4140262375942,
133.045780899098)) ;
#137920=CARTESIAN_POINT('Ctrl Pts',(-18.1223937690385,13.1453688529206,
133.012545885146)) ;
#137921=CARTESIAN_POINT('Ctrl Pts',(-18.0772619681856,12.8977836855868,
132.913734043249)) ;
#137922=CARTESIAN_POINT('Ctrl Pts',(-18.0115583762481,12.6861562793818,
132.75510008698)) ;
#137923=CARTESIAN_POINT('Ctrl Pts',(-17.9302682655273,12.5289208756677,
132.550665981142)) ;
#137924=CARTESIAN_POINT('Ctrl Pts',(-17.8376485738812,12.4351549245617,
132.313282405298)) ;
#137925=CARTESIAN_POINT('Ctrl Pts',(-17.7404755119573,12.4122393500749,
132.06240264819)) ;
#137926=CARTESIAN_POINT('Ctrl Pts',(-17.6435763564324,12.4619213661245,
131.812631468907)) ;
#137927=CARTESIAN_POINT('Ctrl Pts',(-17.5546470358377,12.5803996271663,
131.5859316702)) ;
#137928=CARTESIAN_POINT('Ctrl Pts',(-17.4786252319612,12.7591298548141,
131.39696631873)) ;
#137929=CARTESIAN_POINT('Ctrl Pts',(-17.4203939792657,12.9850686452271,
131.259920960058)) ;
#137930=CARTESIAN_POINT('Ctrl Pts',(-17.3832212801289,13.2423776276029,
131.184410564057)) ;
#137931=CARTESIAN_POINT('Ctrl Pts',(-17.3690898070798,13.5129448157843,
131.176250191703)) ;
#137932=CARTESIAN_POINT('Ctrl Pts',(-17.3783551205516,13.77743197275,131.236478044151)) ;
#137933=CARTESIAN_POINT('Ctrl Pts',(-17.409759931989,14.0166133244865,131.361417283664)) ;
#137934=CARTESIAN_POINT('Ctrl Pts',(-17.4598438655703,14.2120829890599,
131.540706325791)) ;
#137935=CARTESIAN_POINT('Ctrl Pts',(-17.5250988063294,14.3524988741423,
131.764596500736)) ;
#137936=CARTESIAN_POINT('Ctrl Pts',(-17.5994416441049,14.4253825551606,
132.014893373193)) ;
#137937=CARTESIAN_POINT('Ctrl Pts',(-17.6767305680226,14.4267683079455,
132.273679412469)) ;
#137938=CARTESIAN_POINT('Ctrl Pts',(-17.7513139884147,14.3564920605334,
132.524684240105)) ;
#137939=CARTESIAN_POINT('Ctrl Pts',(-17.8169814369023,14.2186720033249,
132.749746015345)) ;
#137940=CARTESIAN_POINT('Ctrl Pts',(-17.8678873517568,14.024316870989,132.931562679198)) ;
#137941=CARTESIAN_POINT('Ctrl Pts',(-17.8999449624512,13.7866137007774,
133.058365103571)) ;
#137942=CARTESIAN_POINT('Ctrl Pts',(-17.9100655439473,13.5238037993467,
133.120963683801)) ;
#137943=CARTESIAN_POINT('Ctrl Pts',(-17.8968818080034,13.2527086934904,
133.115621577909)) ;
#137944=CARTESIAN_POINT('Ctrl Pts',(-17.8603976095492,12.9936531386933,
133.042239984524)) ;
#137945=CARTESIAN_POINT('Ctrl Pts',(-17.8027854988235,12.7662442453604,
132.907025673019)) ;
#137946=CARTESIAN_POINT('Ctrl Pts',(-17.727459915204,12.5858801794281,132.720034663329)) ;
#137947=CARTESIAN_POINT('Ctrl Pts',(-17.6387177576524,12.4648530906934,
132.493949883096)) ;
#137948=CARTESIAN_POINT('Ctrl Pts',(-17.5421197700846,12.4128201898405,
132.245005559525)) ;
#137949=CARTESIAN_POINT('Ctrl Pts',(-17.4450854922055,12.4330274008567,
131.994463533369)) ;
#137950=CARTESIAN_POINT('Ctrl Pts',(-17.3522227610111,12.5240123078526,
131.756341738845)) ;
#137951=CARTESIAN_POINT('Ctrl Pts',(-17.2702012517368,12.6795221093343,
131.549866414866)) ;
#137952=CARTESIAN_POINT('Ctrl Pts',(-17.2040049855668,12.8889213981569,
131.389705808723)) ;
#137953=CARTESIAN_POINT('Ctrl Pts',(-17.1579940844833,13.1354946974878,
131.288346856863)) ;
#137954=CARTESIAN_POINT('Ctrl Pts',(-17.1343661691126,13.4042911387148,
131.252587647338)) ;
#137955=CARTESIAN_POINT('Ctrl Pts',(-17.1342785297306,13.6719452303359,
131.285274315191)) ;
#137956=CARTESIAN_POINT('Ctrl Pts',(-17.1569876367207,13.9242175359662,
131.384873870538)) ;
#137957=CARTESIAN_POINT('Ctrl Pts',(-17.200011377229,14.1390288765416,131.543612046333)) ;
#137958=CARTESIAN_POINT('Ctrl Pts',(-17.2595571651154,14.3030286155002,
131.750644929818)) ;
#137959=CARTESIAN_POINT('Ctrl Pts',(-17.3308835517988,14.4041953321141,
131.992170382071)) ;
#137960=CARTESIAN_POINT('Ctrl Pts',(-17.407703870412,14.4349854776255,132.249625669667)) ;
#137961=CARTESIAN_POINT('Ctrl Pts',(-17.4843503152303,14.3934046912769,
132.506700507749)) ;
#137962=CARTESIAN_POINT('Ctrl Pts',(-17.5541977602429,14.2822103213118,
132.743866956498)) ;
#137963=CARTESIAN_POINT('Ctrl Pts',(-17.611586421142,14.1097942547729,132.944599624469)) ;
#137964=CARTESIAN_POINT('Ctrl Pts',(-17.6518405058853,13.8877667397205,
133.095350804758)) ;
#137965=CARTESIAN_POINT('Ctrl Pts',(-17.6711705177654,13.6324084843775,
133.18497005015)) ;
#137966=CARTESIAN_POINT('Ctrl Pts',(-17.667514600264,13.362418602374,133.207397716684)) ;
#137967=CARTESIAN_POINT('Ctrl Pts',(-17.6404429322753,13.0965815355502,
133.161441915775)) ;
#137968=CARTESIAN_POINT('Ctrl Pts',(-17.5910518071046,12.8540736750208,
133.050310617862)) ;
#137969=CARTESIAN_POINT('Ctrl Pts',(-17.5226154463243,12.6529924848678,
132.883394021802)) ;
#137970=CARTESIAN_POINT('Ctrl Pts',(-17.4380430797127,12.5055874669249,
132.669701279278)) ;
#137971=CARTESIAN_POINT('Ctrl Pts',(-17.3446363922236,12.4255318802945,
132.429776740736)) ;
#137972=CARTESIAN_POINT('Ctrl Pts',(-17.2467990552435,12.4160627421656,
132.17710214303)) ;
#137973=CARTESIAN_POINT('Ctrl Pts',(-17.1513349333761,12.4788298708389,
131.931338759304)) ;
#137974=CARTESIAN_POINT('Ctrl Pts',(-17.0640791511962,12.6096602147663,
131.709653385946)) ;
#137975=CARTESIAN_POINT('Ctrl Pts',(-16.9910680476231,12.7985461290531,
131.529487423907)) ;
#137976=CARTESIAN_POINT('Ctrl Pts',(-16.9365757845701,13.0317085131987,
131.403370398451)) ;
#137977=CARTESIAN_POINT('Ctrl Pts',(-16.9036356126022,13.2930834714085,
131.340246128436)) ;
#137978=CARTESIAN_POINT('Ctrl Pts',(-16.8939332084059,13.5641923615561,
131.345053455658)) ;
#137979=CARTESIAN_POINT('Ctrl Pts',(-16.9076309665478,13.825680563738,131.418292261047)) ;
#137980=CARTESIAN_POINT('Ctrl Pts',(-16.9426513295678,14.0565822354865,
131.553574700513)) ;
#137981=CARTESIAN_POINT('Ctrl Pts',(-16.9960730462588,14.2434410576494,
131.742775697406)) ;
#137982=CARTESIAN_POINT('Ctrl Pts',(-17.063462231909,14.3714533294417,131.972845687759)) ;
#137983=CARTESIAN_POINT('Ctrl Pts',(-17.1386182416936,14.4311593636965,
132.225408177244)) ;
#137984=CARTESIAN_POINT('Ctrl Pts',(-17.2162705777589,14.4188767520017,
132.485449845098)) ;
#137985=CARTESIAN_POINT('Ctrl Pts',(-17.289454458351,14.3353894135925,132.732308120181)) ;
#137986=CARTESIAN_POINT('Ctrl Pts',(-17.3527484313346,14.1858866633471,
132.950435408973)) ;
#137987=CARTESIAN_POINT('Ctrl Pts',(-17.4002649162093,13.9829323617686,
133.12224680942)) ;
#137988=CARTESIAN_POINT('Ctrl Pts',(-17.4284928876731,13.7386002363464,
133.237921480042)) ;
#137989=CARTESIAN_POINT('Ctrl Pts',(-17.4342568106554,13.4724911093289,
133.28784950881)) ;
#137990=CARTESIAN_POINT('Ctrl Pts',(-17.4166917401806,13.2027754915033,
133.269636837191)) ;
#137991=CARTESIAN_POINT('Ctrl Pts',(-17.3758922241434,12.9475729624172,
133.183729538493)) ;
#137992=CARTESIAN_POINT('Ctrl Pts',(-17.3148505174348,12.7286906957619,
133.038370433074)) ;
#137993=CARTESIAN_POINT('Ctrl Pts',(-17.2365672672713,12.5582194265839,
132.842798939928)) ;
#137994=CARTESIAN_POINT('Ctrl Pts',(-17.145755018373,12.449581474798,132.610728316885)) ;
#137995=CARTESIAN_POINT('Ctrl Pts',(-17.048869231413,12.4111325027633,132.360788548371)) ;
#137996=CARTESIAN_POINT('Ctrl Pts',(-16.9518907589334,12.4448573237376,
132.110542706646)) ;
#137997=CARTESIAN_POINT('Ctrl Pts',(-16.8606690827077,12.5485736287012,
131.877191065832)) ;
#137998=CARTESIAN_POINT('Ctrl Pts',(-16.7809677960658,12.7160675413709,
131.677651641686)) ;
#137999=CARTESIAN_POINT('Ctrl Pts',(-16.7187005371509,12.9327061605047,
131.528760508014)) ;
#138000=CARTESIAN_POINT('Ctrl Pts',(-16.6766985699532,13.1846668295447,
131.439140928805)) ;
#138001=CARTESIAN_POINT('Ctrl Pts',(-16.6574670017428,13.454422434914,131.416124014694)) ;
#138002=CARTESIAN_POINT('Ctrl Pts',(-16.661742910167,13.7215757053134,131.461733848406)) ;
#138003=CARTESIAN_POINT('Ctrl Pts',(-16.6884601779481,13.9674105502267,
131.572911655568)) ;
#138004=CARTESIAN_POINT('Ctrl Pts',(-16.7348809932181,14.1739595025082,
131.741594194927)) ;
#138005=CARTESIAN_POINT('Ctrl Pts',(-16.7971641277775,14.3272528691842,
131.95669868954)) ;
#138006=CARTESIAN_POINT('Ctrl Pts',(-16.8700735166993,14.4155297813334,
132.202859198817)) ;
#138007=CARTESIAN_POINT('Ctrl Pts',(-16.9472882019751,14.4326688958934,
132.461466810552)) ;
#138008=CARTESIAN_POINT('Ctrl Pts',(-17.0231401686984,14.3775211091171,
132.716222598503)) ;
#138009=CARTESIAN_POINT('Ctrl Pts',(-17.0910320528626,14.2540409956265,
132.947659679326)) ;
#138010=CARTESIAN_POINT('Ctrl Pts',(-17.1455765747362,14.0709649077151,
133.140134912755)) ;
#138011=CARTESIAN_POINT('Ctrl Pts',(-17.1820383867769,13.8416200756966,
133.279758830705)) ;
#138012=CARTESIAN_POINT('Ctrl Pts',(-17.1971558117406,13.5823886653328,
133.357025362899)) ;
#138013=CARTESIAN_POINT('Ctrl Pts',(-17.1890809730824,13.3112805522026,
133.366597716942)) ;
#138014=CARTESIAN_POINT('Ctrl Pts',(-17.1576142662405,13.0483998972253,
133.307814067063)) ;
#138015=CARTESIAN_POINT('Ctrl Pts',(-17.1045340611823,12.8130299251434,
133.18579186815)) ;
#138016=CARTESIAN_POINT('Ctrl Pts',(-17.0325353932624,12.6204061484624,
133.008629332675)) ;
#138017=CARTESIAN_POINT('Ctrl Pts',(-16.9460051642248,12.4854479729451,
132.789070942826)) ;
#138018=CARTESIAN_POINT('Ctrl Pts',(-16.8512268174505,12.4181326854097,
132.545207526116)) ;
#138019=CARTESIAN_POINT('Ctrl Pts',(-16.7530299629711,12.4224942327925,
132.291585045142)) ;
#138020=CARTESIAN_POINT('Ctrl Pts',(-16.6586767662889,12.4989652676932,
132.049092748305)) ;
#138021=CARTESIAN_POINT('Ctrl Pts',(-16.5742899308655,12.6405918868476,
131.835543037408)) ;
#138022=CARTESIAN_POINT('Ctrl Pts',(-16.5042089716432,12.8391592679731,
131.66400498736)) ;
#138023=CARTESIAN_POINT('Ctrl Pts',(-16.4533647225878,13.0802458850777,
131.548711680705)) ;
#138024=CARTESIAN_POINT('Ctrl Pts',(-16.4248581823331,13.3449461423443,
131.498541148238)) ;
#138025=CARTESIAN_POINT('Ctrl Pts',(-16.4196652563147,13.6142996015355,
131.516362648374)) ;
#138026=CARTESIAN_POINT('Ctrl Pts',(-16.4374352642044,13.871042063758,131.601394145467)) ;
#138027=CARTESIAN_POINT('Ctrl Pts',(-16.4763794639753,14.0962487888297,
131.748356865339)) ;
#138028=CARTESIAN_POINT('Ctrl Pts',(-16.5330749843241,14.2729913868137,
131.947221307867)) ;
#138029=CARTESIAN_POINT('Ctrl Pts',(-16.6017670425338,14.3876795373717,
132.180769530083)) ;
#138030=CARTESIAN_POINT('Ctrl Pts',(-16.6783001681769,14.4346057861214,
132.437586362415)) ;
#138031=CARTESIAN_POINT('Ctrl Pts',(-16.7555901343856,14.4082599511792,
132.696547850718)) ;
#138032=CARTESIAN_POINT('Ctrl Pts',(-16.8270546879802,14.3122705937861,
132.938272501908)) ;
#138033=CARTESIAN_POINT('Ctrl Pts',(-16.8879493008856,14.1514361884325,
133.149437664589)) ;
#138034=CARTESIAN_POINT('Ctrl Pts',(-16.9321596596727,13.938718878438,133.311723147941)) ;
#138035=CARTESIAN_POINT('Ctrl Pts',(-16.9561807399697,13.6904434101565,
133.414875985821)) ;
#138036=CARTESIAN_POINT('Ctrl Pts',(-16.9576332584604,13.4208420564826,
133.452380950427)) ;
#138037=CARTESIAN_POINT('Ctrl Pts',(-16.9356300496651,13.1534853885067,
133.421103696326)) ;
#138038=CARTESIAN_POINT('Ctrl Pts',(-16.8910845324162,12.9044050301422,
133.324087087722)) ;
#138039=CARTESIAN_POINT('Ctrl Pts',(-16.8258399516658,12.6913476051149,
133.166814351142)) ;
#138040=CARTESIAN_POINT('Ctrl Pts',(-16.7448464344601,12.5324269089272,
132.963277516479)) ;
#138041=CARTESIAN_POINT('Ctrl Pts',(-16.6527813349133,12.4369854999087,
132.727399071395)) ;
#138042=CARTESIAN_POINT('Ctrl Pts',(-16.5554635744337,12.4119049756276,
132.476169895595)) ;
#138043=CARTESIAN_POINT('Ctrl Pts',(-16.4587903747933,12.4592885776231,
132.226936038438)) ;
#138044=CARTESIAN_POINT('Ctrl Pts',(-16.369459226937,12.5757336581161,131.999091644708)) ;
#138045=CARTESIAN_POINT('Ctrl Pts',(-16.2929303792811,12.7527802479952,
131.808650847101)) ;
#138046=CARTESIAN_POINT('Ctrl Pts',(-16.233831620826,12.9786617700214,131.669233459945)) ;
#138047=CARTESIAN_POINT('Ctrl Pts',(-16.1960975343855,13.2359087639226,
131.592141252244)) ;
#138048=CARTESIAN_POINT('Ctrl Pts',(-16.1813777949376,13.5051025506678,
131.582103812986)) ;
#138049=CARTESIAN_POINT('Ctrl Pts',(-16.1900648118431,13.7711208061555,
131.640785889966)) ;
#138050=CARTESIAN_POINT('Ctrl Pts',(-16.2207641246595,14.0100002848338,
131.763493038331)) ;
#138051=CARTESIAN_POINT('Ctrl Pts',(-16.270434947496,14.2073723791963,131.941647170154)) ;
#138052=CARTESIAN_POINT('Ctrl Pts',(-16.3352409404344,14.3492225893051,
132.164164640069)) ;
#138053=CARTESIAN_POINT('Ctrl Pts',(-16.409293471862,14.4242519725476,132.413576464951)) ;
#138054=CARTESIAN_POINT('Ctrl Pts',(-16.4869103046887,14.4277364692307,
132.673460341557)) ;
#138055=CARTESIAN_POINT('Ctrl Pts',(-16.5615560359961,14.3592420521561,
132.924612133088)) ;
#138056=CARTESIAN_POINT('Ctrl Pts',(-16.6272846105789,14.2240687585133,
133.149692670284)) ;
#138057=CARTESIAN_POINT('Ctrl Pts',(-16.6788937432045,14.030558632252,133.333688881493)) ;
#138058=CARTESIAN_POINT('Ctrl Pts',(-16.711477566971,13.7945207204753,133.461937265753)) ;
#138059=CARTESIAN_POINT('Ctrl Pts',(-16.7223284172129,13.5313068874669,
133.52678750857)) ;
#138060=CARTESIAN_POINT('Ctrl Pts',(-16.7097854403445,13.2605193044374,
133.523270922987)) ;
#138061=CARTESIAN_POINT('Ctrl Pts',(-16.6741113532666,13.0015411948259,
133.452162116115)) ;
#138062=CARTESIAN_POINT('Ctrl Pts',(-16.6170671904399,12.7725524549383,
133.318651252456)) ;
#138063=CARTESIAN_POINT('Ctrl Pts',(-16.5419949518571,12.5901314518039,
133.132487335332)) ;
#138064=CARTESIAN_POINT('Ctrl Pts',(-16.4536061361104,12.4675131593939,
132.907409541441)) ;
#138065=CARTESIAN_POINT('Ctrl Pts',(-16.3575808899583,12.4133289167984,
132.659991584727)) ;
#138066=CARTESIAN_POINT('Ctrl Pts',(-16.2598099681386,12.4315113355368,
132.407532861116)) ;
#138067=CARTESIAN_POINT('Ctrl Pts',(-16.1670397257563,12.5204618518985,
132.16957309303)) ;
#138068=CARTESIAN_POINT('Ctrl Pts',(-16.0846355190378,12.6740885345687,
131.961972963439)) ;
#138069=CARTESIAN_POINT('Ctrl Pts',(-16.0179019249324,12.8820605395618,
131.800234643535)) ;
#138070=CARTESIAN_POINT('Ctrl Pts',(-15.9712426615901,13.1280848840325,
131.697024439696)) ;
#138071=CARTESIAN_POINT('Ctrl Pts',(-15.9469668397302,13.3954305340358,
131.659233485228)) ;
#138072=CARTESIAN_POINT('Ctrl Pts',(-15.9461825995179,13.6647721177767,
131.690068609628)) ;
#138073=CARTESIAN_POINT('Ctrl Pts',(-15.9681635891478,13.9166503659834,
131.787382281983)) ;
#138074=CARTESIAN_POINT('Ctrl Pts',(-16.0106798137103,14.1333087838378,
131.944714198646)) ;
#138075=CARTESIAN_POINT('Ctrl Pts',(-16.0697275923172,14.2989356853765,
132.150254382635)) ;
#138076=CARTESIAN_POINT('Ctrl Pts',(-16.1412221891328,14.4025578150193,
132.392466616012)) ;
#138077=CARTESIAN_POINT('Ctrl Pts',(-16.2177066260317,14.4350103975139,
132.648822954175)) ;
#138078=CARTESIAN_POINT('Ctrl Pts',(-16.2943852287552,14.3956728087921,
132.905961120951)) ;
#138079=CARTESIAN_POINT('Ctrl Pts',(-16.3645411469182,14.2862787628231,
133.144049835379)) ;
#138080=CARTESIAN_POINT('Ctrl Pts',(-16.4223268601029,14.1158603656016,
133.345893655305)) ;
#138081=CARTESIAN_POINT('Ctrl Pts',(-16.4633288681658,13.8934485615438,
133.499050647192)) ;
#138082=CARTESIAN_POINT('Ctrl Pts',(-16.4831146759898,13.6404741720686,
133.589770768568)) ;
#138083=CARTESIAN_POINT('Ctrl Pts',(-16.4801375304379,13.3695007769354,
133.61432799691)) ;
#138084=CARTESIAN_POINT('Ctrl Pts',(-16.4537797381838,13.1044457745781,
133.57031484177)) ;
#138085=CARTESIAN_POINT('Ctrl Pts',(-16.4050939273146,12.8607040814897,
133.461257392851)) ;
#138086=CARTESIAN_POINT('Ctrl Pts',(-16.3365614867353,12.6571155232214,
133.294299070555)) ;
#138087=CARTESIAN_POINT('Ctrl Pts',(-16.2534138250762,12.5098080882698,
133.0843480198)) ;
#138088=CARTESIAN_POINT('Ctrl Pts',(-16.1596845798564,12.4266891682411,
132.843691860747)) ;
#138089=CARTESIAN_POINT('Ctrl Pts',(-16.0616021737357,12.4154229677179,
132.590386606377)) ;
#138090=CARTESIAN_POINT('Ctrl Pts',(-15.966325957389,12.4759770344289,132.345056626352)) ;
#138091=CARTESIAN_POINT('Ctrl Pts',(-15.8787279504542,12.6048251808736,
132.12237116192)) ;
#138092=CARTESIAN_POINT('Ctrl Pts',(-15.8052016738303,12.7921644823966,
131.940705271743)) ;
#138093=CARTESIAN_POINT('Ctrl Pts',(-15.7500244795214,13.0247861234327,
131.812661169464)) ;
#138094=CARTESIAN_POINT('Ctrl Pts',(-15.7164543667027,13.2853104299406,
131.747653984486)) ;
#138095=CARTESIAN_POINT('Ctrl Pts',(-15.7061363872041,13.5574329936333,
131.750794145615)) ;
#138096=CARTESIAN_POINT('Ctrl Pts',(-15.7190145282048,13.8171020410684,
131.821326630695)) ;
#138097=CARTESIAN_POINT('Ctrl Pts',(-15.7536666697236,14.0511737874882,
131.955815273683)) ;
#138098=CARTESIAN_POINT('Ctrl Pts',(-15.8066102077267,14.2388281318634,
132.143548289998)) ;
#138099=CARTESIAN_POINT('Ctrl Pts',(-15.8734175812164,14.3685838894511,
132.371814409385)) ;
#138100=CARTESIAN_POINT('Ctrl Pts',(-15.9490084927082,14.4305511388163,
132.625903139036)) ;
#138101=CARTESIAN_POINT('Ctrl Pts',(-16.0261164552073,14.4203097552105,
132.884100960231)) ;
#138102=CARTESIAN_POINT('Ctrl Pts',(-16.0998534732104,14.3384208536168,
133.132745263409)) ;
#138103=CARTESIAN_POINT('Ctrl Pts',(-16.1631903784252,14.191573241038,133.350802092867)) ;
#138104=CARTESIAN_POINT('Ctrl Pts',(-16.2115879549403,13.9880715785311,
133.525492647251)) ;
#138105=CARTESIAN_POINT('Ctrl Pts',(-16.2400869176167,13.7471726162761,
133.641599094846)) ;
#138106=CARTESIAN_POINT('Ctrl Pts',(-16.246651218704,13.4800206998336,133.694060674702)) ;
#138107=CARTESIAN_POINT('Ctrl Pts',(-16.229778657571,13.2110031222513,133.677758671742)) ;
#138108=CARTESIAN_POINT('Ctrl Pts',(-16.1896573660202,12.9547749456752,
133.593866138619)) ;
#138109=CARTESIAN_POINT('Ctrl Pts',(-16.1291102530169,12.7344342581801,
133.449982717363)) ;
#138110=CARTESIAN_POINT('Ctrl Pts',(-16.0512258609112,12.5623453815543,
133.255586921922)) ;
#138111=CARTESIAN_POINT('Ctrl Pts',(-15.9608808173794,12.4518692126569,
133.024814380634)) ;
#138112=CARTESIAN_POINT('Ctrl Pts',(-15.8638130263969,12.4112334904619,
132.774443526975)) ;
#138113=CARTESIAN_POINT('Ctrl Pts',(-15.7668529272895,12.442749147545,132.5242072591)) ;
#138114=CARTESIAN_POINT('Ctrl Pts',(-15.6748471126679,12.5456206803201,
132.288785581323)) ;
#138115=CARTESIAN_POINT('Ctrl Pts',(-15.5957928836906,12.7091960284291,
132.090684643297)) ;
#138116=CARTESIAN_POINT('Ctrl Pts',(-15.532372609487,12.9259029795746,131.938683853535)) ;
#138117=CARTESIAN_POINT('Ctrl Pts',(-15.4898220287173,13.1770736190436,
131.847439441881)) ;
#138118=CARTESIAN_POINT('Ctrl Pts',(-15.4698955138865,13.446876823357,131.822431045904)) ;
#138119=CARTESIAN_POINT('Ctrl Pts',(-15.473510723152,13.7138795618443,131.86604868999)) ;
#138120=CARTESIAN_POINT('Ctrl Pts',(-15.4995760707828,13.9605431609207,
131.975315053857)) ;
#138121=CARTESIAN_POINT('Ctrl Pts',(-15.5454521788285,14.1686235242906,
132.142413250352)) ;
#138122=CARTESIAN_POINT('Ctrl Pts',(-15.6076569312687,14.324111246448,132.35743463947)) ;
#138123=CARTESIAN_POINT('Ctrl Pts',(-15.6799406277305,14.4138215674339,
132.60157667707)) ;
#138124=CARTESIAN_POINT('Ctrl Pts',(-15.7574038518846,14.433194510591,132.861043022859)) ;
#138125=CARTESIAN_POINT('Ctrl Pts',(-15.8331619537095,14.3801615030747,
133.115422095018)) ;
#138126=CARTESIAN_POINT('Ctrl Pts',(-15.9014613999127,14.2584943373808,
133.348094869365)) ;
#138127=CARTESIAN_POINT('Ctrl Pts',(-15.9564312114714,14.0770492595335,
133.541793626735)) ;
#138128=CARTESIAN_POINT('Ctrl Pts',(-15.9935402622882,13.8484876221982,
133.683360192996)) ;
#138129=CARTESIAN_POINT('Ctrl Pts',(-16.009247390655,13.5893551833119,133.762405373348)) ;
#138130=CARTESIAN_POINT('Ctrl Pts',(-16.0018749025918,13.3196923685202,
133.773860283275)) ;
#138131=CARTESIAN_POINT('Ctrl Pts',(-15.9711471832523,13.0561135108425,
133.717252900059)) ;
#138132=CARTESIAN_POINT('Ctrl Pts',(-15.9185145007849,12.8190742431854,
133.596625733539)) ;
#138133=CARTESIAN_POINT('Ctrl Pts',(-15.8470380014776,12.6252976951711,
133.420956165043)) ;
#138134=CARTESIAN_POINT('Ctrl Pts',(-15.7611948347474,12.4887797495905,
133.203286234919)) ;
#138135=CARTESIAN_POINT('Ctrl Pts',(-15.6662301653529,12.4190606643947,
132.959008435366)) ;
#138136=CARTESIAN_POINT('Ctrl Pts',(-15.5683946837629,12.4213023126393,
132.706315786054)) ;
#138137=CARTESIAN_POINT('Ctrl Pts',(-15.4738004702747,12.4953371872364,
132.463124320861)) ;
#138138=CARTESIAN_POINT('Ctrl Pts',(-15.388635753643,12.6358732180601,132.247464766846)) ;
#138139=CARTESIAN_POINT('Ctrl Pts',(-15.3182966935884,12.8325868641011,
132.075082447187)) ;
#138140=CARTESIAN_POINT('Ctrl Pts',(-15.2669461693639,13.0715961519443,
131.958183075629)) ;
#138141=CARTESIAN_POINT('Ctrl Pts',(-15.2375683477149,13.3366927750057,
131.905581597702)) ;
#138142=CARTESIAN_POINT('Ctrl Pts',(-15.2316989598249,13.606785296831,131.921501350001)) ;
#138143=CARTESIAN_POINT('Ctrl Pts',(-15.2488554240905,13.8640946124835,
132.004734373222)) ;
#138144=CARTESIAN_POINT('Ctrl Pts',(-15.2871043553366,14.0898396891215,
132.149570187172)) ;
#138145=CARTESIAN_POINT('Ctrl Pts',(-15.3432768304583,14.2683601358406,
132.346899303774)) ;
#138146=CARTESIAN_POINT('Ctrl Pts',(-15.4119474860211,14.3854877046267,
132.58051583122)) ;
#138147=CARTESIAN_POINT('Ctrl Pts',(-15.4884424926978,14.4341894572121,
132.837252051673)) ;
#138148=CARTESIAN_POINT('Ctrl Pts',(-15.5653738474254,14.4102459921106,
133.094979330122)) ;
#138149=CARTESIAN_POINT('Ctrl Pts',(-15.6374786298125,14.3157190634071,
133.33876207548)) ;
#138150=CARTESIAN_POINT('Ctrl Pts',(-15.6984108184879,14.1574303068782,
133.549845061473)) ;
#138151=CARTESIAN_POINT('Ctrl Pts',(-15.7433567069142,13.9458829151207,
133.714346199498)) ;
#138152=CARTESIAN_POINT('Ctrl Pts',(-15.7680544461719,13.6969896292084,
133.819651524776)) ;
#138153=CARTESIAN_POINT('Ctrl Pts',(-15.7701128925175,13.4292803760991,
133.858728163607)) ;
#138154=CARTESIAN_POINT('Ctrl Pts',(-15.7489102637766,13.161309101516,133.829820281867)) ;
#138155=CARTESIAN_POINT('Ctrl Pts',(-15.7044987762573,12.9096301866455,
133.733459274238)) ;
#138156=CARTESIAN_POINT('Ctrl Pts',(-15.6404646327747,12.6977069175332,
133.579353143141)) ;
#138157=CARTESIAN_POINT('Ctrl Pts',(-15.559648556402,12.5361591830993,133.376465293707)) ;
#138158=CARTESIAN_POINT('Ctrl Pts',(-15.4678292234998,12.4388403169488,
133.141295158116)) ;
#138159=CARTESIAN_POINT('Ctrl Pts',(-15.3704747732284,12.4115721832676,
132.889995995841)) ;
#138160=CARTESIAN_POINT('Ctrl Pts',(-15.2736312055909,12.457029405049,132.640284459813)) ;
#138161=CARTESIAN_POINT('Ctrl Pts',(-15.184195197508,12.5713337324556,132.412066033633)) ;
#138162=CARTESIAN_POINT('Ctrl Pts',(-15.1071501777741,12.7468028195077,
132.220136803515)) ;
#138163=CARTESIAN_POINT('Ctrl Pts',(-15.047509486281,12.9715572514285,132.079139887293)) ;
#138164=CARTESIAN_POINT('Ctrl Pts',(-15.0091484797696,13.2272670730613,
132.000111495129)) ;
#138165=CARTESIAN_POINT('Ctrl Pts',(-14.9936966441721,13.4980618104753,
131.988152202933)) ;
#138166=CARTESIAN_POINT('Ctrl Pts',(-15.001604720738,13.7620973804226,132.044245602663)) ;
#138167=CARTESIAN_POINT('Ctrl Pts',(-15.0317823075058,14.0037248374368,
132.165654919109)) ;
#138168=CARTESIAN_POINT('Ctrl Pts',(-15.0809769621606,14.2023999767799,
132.342402115779)) ;
#138169=CARTESIAN_POINT('Ctrl Pts',(-15.1456099214344,14.3463072474208,
132.564505013179)) ;
#138170=CARTESIAN_POINT('Ctrl Pts',(-15.2191783755769,14.422940695718,132.812364240475)) ;
#138171=CARTESIAN_POINT('Ctrl Pts',(-15.2967860408574,14.4287087327574,
133.072227594889)) ;
#138172=CARTESIAN_POINT('Ctrl Pts',(-15.3716376729965,14.3623692114808,
133.323987574419)) ;
#138173=CARTESIAN_POINT('Ctrl Pts',(-15.4379695538221,14.2283780368313,
133.550970447247)) ;
#138174=CARTESIAN_POINT('Ctrl Pts',(-15.4899134645702,14.0364257268117,
133.735894159578)) ;
#138175=CARTESIAN_POINT('Ctrl Pts',(-15.5230141171127,13.8020945875402,
133.865562324939)) ;
#138176=CARTESIAN_POINT('Ctrl Pts',(-15.5345523813327,13.5391614868317,
133.932453214591)) ;
#138177=CARTESIAN_POINT('Ctrl Pts',(-15.5227285394594,13.2686187848472,
133.930998203796)) ;
#138178=CARTESIAN_POINT('Ctrl Pts',(-15.4876456278164,13.0086420125285,
133.861671450079)) ;
#138179=CARTESIAN_POINT('Ctrl Pts',(-15.4313828702978,12.7791081292504,
133.730344592057)) ;
#138180=CARTESIAN_POINT('Ctrl Pts',(-15.3564307908051,12.5942977815412,
133.544687034302)) ;
#138181=CARTESIAN_POINT('Ctrl Pts',(-15.2686565651916,12.470297081659,133.321282306556)) ;
#138182=CARTESIAN_POINT('Ctrl Pts',(-15.1725820175887,12.4139049910115,
133.073791862213)) ;
#138183=CARTESIAN_POINT('Ctrl Pts',(-15.0751009055877,12.4297924178913,
132.822062245848)) ;
#138184=CARTESIAN_POINT('Ctrl Pts',(-14.9814943161782,12.5172147153485,
132.581873444977)) ;
#138185=CARTESIAN_POINT('Ctrl Pts',(-14.8987521018085,12.6696685432672,
132.373307698593)) ;
#138186=CARTESIAN_POINT('Ctrl Pts',(-14.8319357526133,12.8748935660195,
132.211108712332)) ;
#138187=CARTESIAN_POINT('Ctrl Pts',(-14.7844724177792,13.1206629009233,
132.105647075877)) ;
#138188=CARTESIAN_POINT('Ctrl Pts',(-14.7595563487713,13.3874986726008,
132.06596134526)) ;
#138189=CARTESIAN_POINT('Ctrl Pts',(-14.758095005719,13.6577700342002,132.094905614256)) ;
#138190=CARTESIAN_POINT('Ctrl Pts',(-14.7795395109122,13.9102263509794,
132.190647313271)) ;
#138191=CARTESIAN_POINT('Ctrl Pts',(-14.8212877176841,14.1273421319092,
132.345592371695)) ;
#138192=CARTESIAN_POINT('Ctrl Pts',(-14.8803004027794,14.2954362033895,
132.5512322011)) ;
#138193=CARTESIAN_POINT('Ctrl Pts',(-14.9508986266852,14.4001990487277,
132.790525926894)) ;
#138194=CARTESIAN_POINT('Ctrl Pts',(-15.0280123654046,14.4351706370755,
133.049038822137)) ;
#138195=CARTESIAN_POINT('Ctrl Pts',(-15.1043517226695,14.3977719552174,
133.304998580299)) ;
#138196=CARTESIAN_POINT('Ctrl Pts',(-15.1749382989597,14.2904204351337,
133.544401657337)) ;
#138197=CARTESIAN_POINT('Ctrl Pts',(-15.2332991479685,14.1205426319521,
133.748067460587)) ;
#138198=CARTESIAN_POINT('Ctrl Pts',(-15.2744570161202,13.9015880459834,
133.901346174034)) ;
#138199=CARTESIAN_POINT('Ctrl Pts',(-15.2950942480665,13.6483197880018,
133.994710398155)) ;
#138200=CARTESIAN_POINT('Ctrl Pts',(-15.2927791762567,13.3774460440173,
134.021204705381)) ;
#138201=CARTESIAN_POINT('Ctrl Pts',(-15.2670274488561,13.1115164567619,
133.979025907644)) ;
#138202=CARTESIAN_POINT('Ctrl Pts',(-15.2190484647999,12.8676277943346,
133.871940072646)) ;
#138203=CARTESIAN_POINT('Ctrl Pts',(-15.151375622549,12.6630942095761,133.70737402675)) ;
#138204=CARTESIAN_POINT('Ctrl Pts',(-15.0680214022309,12.5128296966432,
133.497060151253)) ;
#138205=CARTESIAN_POINT('Ctrl Pts',(-14.9744932694045,12.42805223675,133.256979709909)) ;
#138206=CARTESIAN_POINT('Ctrl Pts',(-14.8766121383161,12.4147676661353,
133.004208092286)) ;
#138207=CARTESIAN_POINT('Ctrl Pts',(-14.7811668098369,12.4732051898518,
132.75838587031)) ;
#138208=CARTESIAN_POINT('Ctrl Pts',(-14.6929706084526,12.6008829742714,
132.534073690074)) ;
#138209=CARTESIAN_POINT('Ctrl Pts',(-14.6193920014731,12.7859099614939,
132.352088247255)) ;
#138210=CARTESIAN_POINT('Ctrl Pts',(-14.5636050471311,13.0171549052487,
132.222240809291)) ;
#138211=CARTESIAN_POINT('Ctrl Pts',(-14.5293360875052,13.277402309204,132.155230612714)) ;
#138212=CARTESIAN_POINT('Ctrl Pts',(-14.5182996919213,13.5492090907174,
132.156231309037)) ;
#138213=CARTESIAN_POINT('Ctrl Pts',(-14.5305857227298,13.8101281640257,
132.225131951709)) ;
#138214=CARTESIAN_POINT('Ctrl Pts',(-14.5644345612442,14.0442615498891,
132.35711154665)) ;
#138215=CARTESIAN_POINT('Ctrl Pts',(-14.6173143320161,14.2348996277818,
132.54492092966)) ;
#138216=CARTESIAN_POINT('Ctrl Pts',(-14.6834945620548,14.365488247491,132.771175660337)) ;
#138217=CARTESIAN_POINT('Ctrl Pts',(-14.7587206634414,14.429722906614,133.024124517551)) ;
#138218=CARTESIAN_POINT('Ctrl Pts',(-14.8361154517203,14.4216680373145,
133.283271314569)) ;
#138219=CARTESIAN_POINT('Ctrl Pts',(-14.9100777170694,14.3417421595957,
133.532580346532)) ;
#138220=CARTESIAN_POINT('Ctrl Pts',(-14.9737927629375,14.1964292169101,
133.751768065663)) ;
#138221=CARTESIAN_POINT('Ctrl Pts',(-15.0224985277877,13.9955519637573,
133.927180888922)) ;
#138222=CARTESIAN_POINT('Ctrl Pts',(-15.0518421016778,13.7541465447125,
134.045965793673)) ;
#138223=CARTESIAN_POINT('Ctrl Pts',(-15.058983051814,13.4873871522708,134.100101961475)) ;
#138224=CARTESIAN_POINT('Ctrl Pts',(-15.0427889947955,13.2187119669683,
134.085726725674)) ;
#138225=CARTESIAN_POINT('Ctrl Pts',(-15.0034481865866,12.9622340924051,
134.004045221197)) ;
#138226=CARTESIAN_POINT('Ctrl Pts',(-14.9431938775443,12.7396655368573,
133.861166062646)) ;
#138227=CARTESIAN_POINT('Ctrl Pts',(-14.8657108599282,12.5663130362906,
133.667926321551)) ;
#138228=CARTESIAN_POINT('Ctrl Pts',(-14.7760398095514,12.4542929852172,
133.438984177008)) ;
#138229=CARTESIAN_POINT('Ctrl Pts',(-14.678743994539,12.4113060985389,133.188061925005)) ;
#138230=CARTESIAN_POINT('Ctrl Pts',(-14.5818778745094,12.440972973662,132.938049002869)) ;
#138231=CARTESIAN_POINT('Ctrl Pts',(-14.4900849893319,12.5408195803972,
132.703054608506)) ;
#138232=CARTESIAN_POINT('Ctrl Pts',(-14.4096989960112,12.7045177215447,
132.501438908251)) ;
#138233=CARTESIAN_POINT('Ctrl Pts',(-14.346132189806,12.9194126862855,132.348873857722)) ;
#138234=CARTESIAN_POINT('Ctrl Pts',(-14.3030031795231,13.1689179469772,
132.255840036165)) ;
#138235=CARTESIAN_POINT('Ctrl Pts',(-14.2823169602156,13.4397285772897,
132.228764995968)) ;
#138236=CARTESIAN_POINT('Ctrl Pts',(-14.2853193282304,13.7064270482981,
132.270516703463)) ;
#138237=CARTESIAN_POINT('Ctrl Pts',(-14.3107446190627,13.9538862841149,
132.377905843498)) ;
#138238=CARTESIAN_POINT('Ctrl Pts',(-14.3560623753014,14.1631927449857,
132.543351061516)) ;
#138239=CARTESIAN_POINT('Ctrl Pts',(-14.4179193623701,14.3205261030357,
132.757382303374)) ;
#138240=CARTESIAN_POINT('Ctrl Pts',(-14.4898754019086,14.4121066368491,
133.00052214106)) ;
#138241=CARTESIAN_POINT('Ctrl Pts',(-14.5673432317612,14.4337042758691,
133.260027216362)) ;
#138242=CARTESIAN_POINT('Ctrl Pts',(-14.6433126851901,14.3826278342729,
133.515059598052)) ;
#138243=CARTESIAN_POINT('Ctrl Pts',(-14.711870574383,14.2628852897391,133.748467202197)) ;
#138244=CARTESIAN_POINT('Ctrl Pts',(-14.767308001138,14.0829262304897,133.943544580163)) ;
#138245=CARTESIAN_POINT('Ctrl Pts',(-14.804958064437,13.8556922728628,134.08666212542)) ;
#138246=CARTESIAN_POINT('Ctrl Pts',(-14.821309401496,13.5972599907668,134.167584085587)) ;
#138247=CARTESIAN_POINT('Ctrl Pts',(-14.8147006723657,13.3277680057125,
134.181252611574)) ;
#138248=CARTESIAN_POINT('Ctrl Pts',(-14.7842864021737,13.0618110658261,
134.125814803658)) ;
#138249=CARTESIAN_POINT('Ctrl Pts',(-14.7326708515057,12.8260390349159,
134.007850477343)) ;
#138250=CARTESIAN_POINT('Ctrl Pts',(-14.6614620611927,12.6298697180506,
133.833098581207)) ;
#138251=CARTESIAN_POINT('Ctrl Pts',(-14.575982707112,12.4917687928696,133.616467821938)) ;
#138252=CARTESIAN_POINT('Ctrl Pts',(-14.4810796906638,12.4199839443985,
133.372411393608)) ;
#138253=CARTESIAN_POINT('Ctrl Pts',(-14.383292851168,12.4203084099031,133.119842779795)) ;
#138254=CARTESIAN_POINT('Ctrl Pts',(-14.2886705183159,12.4922084263286,
132.876515661936)) ;
#138255=CARTESIAN_POINT('Ctrl Pts',(-14.203107613883,12.6309968831691,132.659710749856)) ;
#138256=CARTESIAN_POINT('Ctrl Pts',(-14.1322473538398,12.8263310850707,
132.485816844473)) ;
#138257=CARTESIAN_POINT('Ctrl Pts',(-14.0801877023912,13.0651227719104,
132.366942948258)) ;
#138258=CARTESIAN_POINT('Ctrl Pts',(-14.0502840451506,13.3295667495973,
132.312773352509)) ;
#138259=CARTESIAN_POINT('Ctrl Pts',(-14.0437510939769,13.5989123639349,
132.326651696683)) ;
#138260=CARTESIAN_POINT('Ctrl Pts',(-14.0603102617504,13.8574710596154,
132.408219676378)) ;
#138261=CARTESIAN_POINT('Ctrl Pts',(-14.0979300090043,14.0837078972677,
132.551132179434)) ;
#138262=CARTESIAN_POINT('Ctrl Pts',(-14.1535518862661,14.2638191910291,
132.746822281892)) ;
#138263=CARTESIAN_POINT('Ctrl Pts',(-14.2221618886066,14.3831695722174,
132.980371817265)) ;
#138264=CARTESIAN_POINT('Ctrl Pts',(-14.2982848293422,14.4337176680091,
133.235911108826)) ;
#138265=CARTESIAN_POINT('Ctrl Pts',(-14.3753145515019,14.4120588735212,
133.493942054439)) ;
#138266=CARTESIAN_POINT('Ctrl Pts',(-14.4477414803192,14.3193773095664,
133.738707356022)) ;
#138267=CARTESIAN_POINT('Ctrl Pts',(-14.5091083465657,14.1628171058123,
133.951066133343)) ;
#138268=CARTESIAN_POINT('Ctrl Pts',(-14.5546602501446,13.9515916314902,
134.117466746109)) ;
#138269=CARTESIAN_POINT('Ctrl Pts',(-14.5798144029916,13.705523326728,134.223839172995)) ;
#138270=CARTESIAN_POINT('Ctrl Pts',(-14.5825811444736,13.4359481915904,
134.265260316511)) ;
#138271=CARTESIAN_POINT('Ctrl Pts',(-14.5620507546937,13.169026252587,134.238153095214)) ;
#138272=CARTESIAN_POINT('Ctrl Pts',(-14.5182618166179,12.916272819337,134.143645987583)) ;
#138273=CARTESIAN_POINT('Ctrl Pts',(-14.4549186809599,12.7036779649805,
133.99146914691)) ;
#138274=CARTESIAN_POINT('Ctrl Pts',(-14.374687848165,12.5403117624792,133.790249344614)) ;
#138275=CARTESIAN_POINT('Ctrl Pts',(-14.2824989348909,12.4404489594076,
133.554219478518)) ;
#138276=CARTESIAN_POINT('Ctrl Pts',(-14.1856763731449,12.4114485635984,
133.304313177069)) ;
#138277=CARTESIAN_POINT('Ctrl Pts',(-14.0887755516816,12.4544846359496,
133.054413939327)) ;
#138278=CARTESIAN_POINT('Ctrl Pts',(-13.998682567479,12.5672617568272,132.824403407284)) ;
#138279=CARTESIAN_POINT('Ctrl Pts',(-13.9211585063749,12.7417744672769,
132.631137059237)) ;
#138280=CARTESIAN_POINT('Ctrl Pts',(-13.8614037350289,12.9633750466865,
132.489527799616)) ;
#138281=CARTESIAN_POINT('Ctrl Pts',(-13.8220394457413,13.2203111282886,
132.40782907511)) ;
#138282=CARTESIAN_POINT('Ctrl Pts',(-13.8060358886469,13.4905143177326,
132.394191857521)) ;
#138283=CARTESIAN_POINT('Ctrl Pts',(-13.8133099943821,13.755021596538,132.448448822965)) ;
#138284=CARTESIAN_POINT('Ctrl Pts',(-13.8427459453627,13.9967495673617,
132.567564010889)) ;
#138285=CARTESIAN_POINT('Ctrl Pts',(-13.8915602482871,14.1974242169902,
132.743295638543)) ;
#138286=CARTESIAN_POINT('Ctrl Pts',(-13.9555090185762,14.3425139654286,
132.963240650371)) ;
#138287=CARTESIAN_POINT('Ctrl Pts',(-14.0290714695679,14.4218015795288,
133.21118520583)) ;
#138288=CARTESIAN_POINT('Ctrl Pts',(-14.1070493874014,14.4294553596466,
133.472292177633)) ;
#138289=CARTESIAN_POINT('Ctrl Pts',(-14.181690309578,14.3652618643662,133.723279219976)) ;
#138290=CARTESIAN_POINT('Ctrl Pts',(-14.2482705789536,14.2335997278837,
133.950926411238)) ;
#138291=CARTESIAN_POINT('Ctrl Pts',(-14.3008003166485,14.043065952539,134.137599115662)) ;
#138292=CARTESIAN_POINT('Ctrl Pts',(-14.334600453399,13.8093139342674,134.269381140691)) ;
#138293=CARTESIAN_POINT('Ctrl Pts',(-14.3467469914,13.5459140316558,134.338166616757)) ;
#138294=CARTESIAN_POINT('Ctrl Pts',(-14.3356273569063,13.2769104618193,
134.338576916924)) ;
#138295=CARTESIAN_POINT('Ctrl Pts',(-14.3012529645766,13.0160047166174,
134.271353792998)) ;
#138296=CARTESIAN_POINT('Ctrl Pts',(-14.2454215258121,12.7850162006338,
134.141350290204)) ;
#138297=CARTESIAN_POINT('Ctrl Pts',(-14.1712185020009,12.5991696538989,
133.957766591908)) ;
#138298=CARTESIAN_POINT('Ctrl Pts',(-14.083300535675,12.4727066988936,133.734115733787)) ;
#138299=CARTESIAN_POINT('Ctrl Pts',(-13.9878279907723,12.4146340125785,
133.488219860348)) ;
#138300=CARTESIAN_POINT('Ctrl Pts',(-13.8900938776437,12.4282724622725,
133.235826128764)) ;
#138301=CARTESIAN_POINT('Ctrl Pts',(-13.7963885477012,12.5136821957653,
132.995310230063)) ;
#138302=CARTESIAN_POINT('Ctrl Pts',(-13.7132720195936,12.6640313593757,
132.785624145284)) ;
#138303=CARTESIAN_POINT('Ctrl Pts',(-13.645547905693,12.8694014058608,132.620995535521)) ;
#138304=CARTESIAN_POINT('Ctrl Pts',(-13.5978347475723,13.1128473164404,
132.514595028059)) ;
#138305=CARTESIAN_POINT('Ctrl Pts',(-13.5721656264375,13.3794713552814,
132.472736688106)) ;
#138306=CARTESIAN_POINT('Ctrl Pts',(-13.5700232955001,13.6493875459495,
132.499624261885)) ;
#138307=CARTESIAN_POINT('Ctrl Pts',(-13.5906979487209,13.9027716733404,
132.593113973492)) ;
#138308=CARTESIAN_POINT('Ctrl Pts',(-13.6323003089401,14.1226003916879,
132.747892074304)) ;
#138309=CARTESIAN_POINT('Ctrl Pts',(-13.6903176396252,14.2907614910249,
132.950296656493)) ;
#138310=CARTESIAN_POINT('Ctrl Pts',(-13.76127060048,14.3985142710539,133.190934634915)) ;
#138311=CARTESIAN_POINT('Ctrl Pts',(-13.8377932896785,14.4350393250775,
133.447491800336)) ;
#138312=CARTESIAN_POINT('Ctrl Pts',(-13.9143676794725,14.400035592365,133.704198098061)) ;
#138313=CARTESIAN_POINT('Ctrl Pts',(-13.9854510810604,14.2940192580209,
133.945170020293)) ;
#138314=CARTESIAN_POINT('Ctrl Pts',(-14.0439573923053,14.1264036829356,
134.149121613712)) ;
#138315=CARTESIAN_POINT('Ctrl Pts',(-14.0857782181044,13.9087136150407,
134.304358215958)) ;
#138316=CARTESIAN_POINT('Ctrl Pts',(-14.1070694486661,13.6545233565068,
134.399835876429)) ;
#138317=CARTESIAN_POINT('Ctrl Pts',(-14.1053844366646,13.3858501360358,
134.427920015331)) ;
#138318=CARTESIAN_POINT('Ctrl Pts',(-14.0803367946603,13.11900556216,134.387865314787)) ;
#138319=CARTESIAN_POINT('Ctrl Pts',(-14.0328788178783,12.8738785752154,
134.282346772143)) ;
#138320=CARTESIAN_POINT('Ctrl Pts',(-13.9655106265573,12.6676054071639,
134.118751181152)) ;
#138321=CARTESIAN_POINT('Ctrl Pts',(-13.8825856552335,12.516077131837,133.909646349396)) ;
#138322=CARTESIAN_POINT('Ctrl Pts',(-13.7897110779122,12.4297444851197,
133.671323006778)) ;
#138323=CARTESIAN_POINT('Ctrl Pts',(-13.6919754716078,12.4139325771417,
133.418938373948)) ;
#138324=CARTESIAN_POINT('Ctrl Pts',(-13.5958285338883,12.4708186129552,
133.171266520997)) ;
#138325=CARTESIAN_POINT('Ctrl Pts',(-13.5080655357658,12.5954480986012,
132.94792799004)) ;
#138326=CARTESIAN_POINT('Ctrl Pts',(-13.4335244933812,12.7795462403225,
132.763308241075)) ;
#138327=CARTESIAN_POINT('Ctrl Pts',(-13.3770299436409,13.0105017874409,
132.631490811353)) ;
#138328=CARTESIAN_POINT('Ctrl Pts',(-13.3421556868852,13.2704658553687,
132.562743301802)) ;
#138329=CARTESIAN_POINT('Ctrl Pts',(-13.3305220477458,13.5415024018121,
132.561910660489)) ;
#138330=CARTESIAN_POINT('Ctrl Pts',(-13.3421066509126,13.8030869084645,
132.628769487748)) ;
#138331=CARTESIAN_POINT('Ctrl Pts',(-13.3756345993665,14.0389746831751,
132.759952112845)) ;
#138332=CARTESIAN_POINT('Ctrl Pts',(-13.4273915726418,14.2290323686529,
132.944092286592)) ;
#138333=CARTESIAN_POINT('Ctrl Pts',(-13.4937472681949,14.3629000991712,
133.17115070044)) ;
#138334=CARTESIAN_POINT('Ctrl Pts',(-13.5686675780257,14.4288302625026,
133.423124913234)) ;
#138335=CARTESIAN_POINT('Ctrl Pts',(-13.6462332083306,14.422836536164,133.682844745829)) ;
#138336=CARTESIAN_POINT('Ctrl Pts',(-13.7201301396068,14.3452102750607,
133.931839588516)) ;
#138337=CARTESIAN_POINT('Ctrl Pts',(-13.7843830850645,14.2014203774082,
134.152682847936)) ;
#138338=CARTESIAN_POINT('Ctrl Pts',(-13.8335217961475,14.002164262405,134.329317533484)) ;
#138339=CARTESIAN_POINT('Ctrl Pts',(-13.8634889037809,13.7617532002817,
134.449925964223)) ;
#138340=CARTESIAN_POINT('Ctrl Pts',(-13.8713352949717,13.4956080912223,
134.506099255839)) ;
#138341=CARTESIAN_POINT('Ctrl Pts',(-13.8557782269919,13.2262846444733,
134.493650674134)) ;
#138342=CARTESIAN_POINT('Ctrl Pts',(-13.8172322300386,12.9698877409975,
134.414183738046)) ;
#138343=CARTESIAN_POINT('Ctrl Pts',(-13.7574812944028,12.7457364397051,
134.272830100964)) ;
#138344=CARTESIAN_POINT('Ctrl Pts',(-13.6806317994049,12.5708017682082,
134.081378097011)) ;
#138345=CARTESIAN_POINT('Ctrl Pts',(-13.5903919715778,12.456149717707,133.851080417193)) ;
#138346=CARTESIAN_POINT('Ctrl Pts',(-13.4942558602785,12.4116404870963,
133.603177645582)) ;
#138347=CARTESIAN_POINT('Ctrl Pts',(-13.3965419126512,12.4391729305521,
133.350956099842)) ;
#138348=CARTESIAN_POINT('Ctrl Pts',(-13.3047832313469,12.5371797605548,
133.115969475029)) ;
#138349=CARTESIAN_POINT('Ctrl Pts',(-13.224224637073,12.6985743465351,132.913751244712)) ;
#138350=CARTESIAN_POINT('Ctrl Pts',(-13.1600523063441,12.9117741381151,
132.75938813857)) ;
#138351=CARTESIAN_POINT('Ctrl Pts',(-13.1160389583248,13.1624013185224,
132.664019628854)) ;
#138352=CARTESIAN_POINT('Ctrl Pts',(-13.0948693964311,13.430527916598,132.635227970366)) ;
#138353=CARTESIAN_POINT('Ctrl Pts',(-13.0970891229502,13.6988963503242,
132.674862389402)) ;
#138354=CARTESIAN_POINT('Ctrl Pts',(-13.1219243680964,13.9472005331235,
132.780524168488)) ;
#138355=CARTESIAN_POINT('Ctrl Pts',(-13.1668095584822,14.1580510542122,
132.944759839031)) ;
#138356=CARTESIAN_POINT('Ctrl Pts',(-13.2279893075256,14.3165352263592,
133.156667794039)) ;
#138357=CARTESIAN_POINT('Ctrl Pts',(-13.300074213206,14.4105996600904,133.400356897989)) ;
#138358=CARTESIAN_POINT('Ctrl Pts',(-13.3772745227853,14.4340684661328,
133.65898364802)) ;
#138359=CARTESIAN_POINT('Ctrl Pts',(-13.4534960317781,14.3850544028617,
133.914807927191)) ;
#138360=CARTESIAN_POINT('Ctrl Pts',(-13.5223409843892,14.2669952592305,
134.149060765162)) ;
#138361=CARTESIAN_POINT('Ctrl Pts',(-13.5780776236805,14.08911548236,134.344922101581)) ;
#138362=CARTESIAN_POINT('Ctrl Pts',(-13.6163713098489,13.8629229464963,
134.489949169064)) ;
#138363=CARTESIAN_POINT('Ctrl Pts',(-13.6334000812586,13.604494449949,134.572926457528)) ;
#138364=CARTESIAN_POINT('Ctrl Pts',(-13.6273628390361,13.3352196406284,
134.588252141428)) ;
#138365=CARTESIAN_POINT('Ctrl Pts',(-13.5979289468704,13.0705830393377,
134.535442159946)) ;
#138366=CARTESIAN_POINT('Ctrl Pts',(-13.5465441539597,12.8316693122143,
134.418434168296)) ;
#138367=CARTESIAN_POINT('Ctrl Pts',(-13.4756744662724,12.6342706901117,
134.244688087508)) ;
#138368=CARTESIAN_POINT('Ctrl Pts',(-13.3908617467319,12.4949548455415,
134.029880371869)) ;
#138369=CARTESIAN_POINT('Ctrl Pts',(-13.2961267998515,12.421067631229,133.786322706496)) ;
#138370=CARTESIAN_POINT('Ctrl Pts',(-13.1984664907621,12.4192534681359,
133.53408220403)) ;
#138371=CARTESIAN_POINT('Ctrl Pts',(-13.1034923930835,12.4890550596445,
133.28977926538)) ;
#138372=CARTESIAN_POINT('Ctrl Pts',(-13.017265404549,12.6269264793826,133.071181056084)) ;
#138373=CARTESIAN_POINT('Ctrl Pts',(-12.9463889263436,12.8196494832229,
132.897028166528)) ;
#138374=CARTESIAN_POINT('Ctrl Pts',(-12.8935445665423,13.0580835296679,
132.775965890197)) ;
#138375=CARTESIAN_POINT('Ctrl Pts',(-12.8630605529485,13.321466149626,132.720020527257)) ;
#138376=CARTESIAN_POINT('Ctrl Pts',(-12.8558430268871,13.5912986837364,
132.731956034601)) ;
#138377=CARTESIAN_POINT('Ctrl Pts',(-12.8716409242927,13.8497218506693,
132.811188161045)) ;
#138378=CARTESIAN_POINT('Ctrl Pts',(-12.9090128451689,14.0789422009193,
132.953652047894)) ;
#138379=CARTESIAN_POINT('Ctrl Pts',(-12.9641549217213,14.2597600748466,
133.147850764733)) ;
#138380=CARTESIAN_POINT('Ctrl Pts',(-13.0322170994182,14.3805241466999,
133.379686428977)) ;
#138381=CARTESIAN_POINT('Ctrl Pts',(-13.1081075369044,14.4333051039602,
133.634503568026)) ;
#138382=CARTESIAN_POINT('Ctrl Pts',(-13.1855018681886,14.4135763254968,
133.893739522478)) ;
#138383=CARTESIAN_POINT('Ctrl Pts',(-13.2580501555575,14.3230160042054,
134.138797856071)) ;
#138384=CARTESIAN_POINT('Ctrl Pts',(-13.3200141919047,14.1669880886898,
134.353077810686)) ;
#138385=CARTESIAN_POINT('Ctrl Pts',(-13.3655273041903,13.9601855279978,
134.518891328518)) ;
#138386=CARTESIAN_POINT('Ctrl Pts',(-13.39166667475,13.7121979850729,134.628542890827)) ;
#138387=CARTESIAN_POINT('Ctrl Pts',(-13.3950941590884,13.44532544281,134.671581655692)) ;
#138388=CARTESIAN_POINT('Ctrl Pts',(-13.3750645278574,13.1756579344581,
134.646260957203)) ;
#138389=CARTESIAN_POINT('Ctrl Pts',(-13.3324016363677,12.9248371120238,
134.554668453737)) ;
#138390=CARTESIAN_POINT('Ctrl Pts',(-13.2691521870421,12.7087904185415,
134.403066738095)) ;
#138391=CARTESIAN_POINT('Ctrl Pts',(-13.189355166933,12.5441839960965,134.203071426488)) ;
#138392=CARTESIAN_POINT('Ctrl Pts',(-13.0974574702678,12.4422953635853,
133.967886639172)) ;
#138393=CARTESIAN_POINT('Ctrl Pts',(-13.0004980461265,12.4112745925655,
133.717648882006)) ;
#138394=CARTESIAN_POINT('Ctrl Pts',(-12.9036891883039,12.4523611217467,
133.467956597446)) ;
#138395=CARTESIAN_POINT('Ctrl Pts',(-12.8135499305002,12.5627156193445,
133.237713892736)) ;
#138396=CARTESIAN_POINT('Ctrl Pts',(-12.7352975800842,12.736203215032,133.04244250152)) ;
#138397=CARTESIAN_POINT('Ctrl Pts',(-12.6751129170403,12.9562236735918,
132.899511681536)) ;
#138398=CARTESIAN_POINT('Ctrl Pts',(-12.6350705235841,13.212763202245,132.81587545549)) ;
#138399=CARTESIAN_POINT('Ctrl Pts',(-12.618415408845,13.4814739437606,132.800169250016)) ;
#138400=CARTESIAN_POINT('Ctrl Pts',(-12.624949611358,13.747602021364,132.852409321137)) ;
#138401=CARTESIAN_POINT('Ctrl Pts',(-12.6539126495085,13.9907502143909,
132.970218060048)) ;
#138402=CARTESIAN_POINT('Ctrl Pts',(-12.7021026429137,14.192126827699,133.144029351541)) ;
#138403=CARTESIAN_POINT('Ctrl Pts',(-12.765596611934,14.3392030081547,133.362624554204)) ;
#138404=CARTESIAN_POINT('Ctrl Pts',(-12.8395683339224,14.420750007367,133.612027485091)) ;
#138405=CARTESIAN_POINT('Ctrl Pts',(-12.9167981216665,14.4302362672735,
133.870632857131)) ;
#138406=CARTESIAN_POINT('Ctrl Pts',(-12.992010059953,14.3680283061645,134.123465509195)) ;
#138407=CARTESIAN_POINT('Ctrl Pts',(-13.0589983401631,14.237554410734,134.352370279363)) ;
#138408=CARTESIAN_POINT('Ctrl Pts',(-13.1118284099058,14.0487160493496,
134.539853291678)) ;
#138409=CARTESIAN_POINT('Ctrl Pts',(-13.146070298649,13.8167884864147,134.672814185713)) ;
#138410=CARTESIAN_POINT('Ctrl Pts',(-13.158940600161,13.5548285940714,134.743611055561)) ;
#138411=CARTESIAN_POINT('Ctrl Pts',(-13.1485141240606,13.2844751401064,
134.74620797937)) ;
#138412=CARTESIAN_POINT('Ctrl Pts',(-13.1146632560627,13.0226684871857,
134.680563192847)) ;
#138413=CARTESIAN_POINT('Ctrl Pts',(-13.0595530042838,12.7913020649599,
134.552571784859)) ;
#138414=CARTESIAN_POINT('Ctrl Pts',(-12.9859254140349,12.6040508049077,
134.370634704252)) ;
#138415=CARTESIAN_POINT('Ctrl Pts',(-12.8984068250737,12.4756114262356,
134.148131473393)) ;
#138416=CARTESIAN_POINT('Ctrl Pts',(-12.8027801955588,12.4152434956171,
133.901891080666)) ;
#138417=CARTESIAN_POINT('Ctrl Pts',(-12.7050832331602,12.4269403592131,
133.649583880182)) ;
#138418=CARTESIAN_POINT('Ctrl Pts',(-12.6113870773195,12.5099952735333,
133.409010819848)) ;
#138419=CARTESIAN_POINT('Ctrl Pts',(-12.5277681815658,12.6587328614396,
133.19790502644)) ;
#138420=CARTESIAN_POINT('Ctrl Pts',(-12.4597036669732,12.8618951640278,
133.03216961154)) ;
#138421=CARTESIAN_POINT('Ctrl Pts',(-12.4110853088982,13.1054069389763,
132.923273357885)) ;
#138422=CARTESIAN_POINT('Ctrl Pts',(-12.3847729703008,13.3721986649784,
132.879596342574)) ;
#138423=CARTESIAN_POINT('Ctrl Pts',(-12.3819859406308,13.6415133850086,
132.904506589099)) ;
#138424=CARTESIAN_POINT('Ctrl Pts',(-12.4019516425332,13.8954057097587,
132.995891115908)) ;
#138425=CARTESIAN_POINT('Ctrl Pts',(-12.4430233781849,14.1169004603375,
133.149166980611)) ;
#138426=CARTESIAN_POINT('Ctrl Pts',(-12.5007743421724,14.286862322143,133.350862259024)) ;
#138427=CARTESIAN_POINT('Ctrl Pts',(-12.5710080643675,14.3960130352986,
133.589195796255)) ;
#138428=CARTESIAN_POINT('Ctrl Pts',(-12.6477378354541,14.435114922765,133.846495972005)) ;
#138429=CARTESIAN_POINT('Ctrl Pts',(-12.7245100764212,14.4019052021935,
134.103831117832)) ;
#138430=CARTESIAN_POINT('Ctrl Pts',(-12.7956173758933,14.2983009170395,
134.344755254071)) ;
#138431=CARTESIAN_POINT('Ctrl Pts',(-12.8547869888769,14.1317969214597,
134.550768714552)) ;
#138432=CARTESIAN_POINT('Ctrl Pts',(-12.8970503379981,13.915343377283,134.707274446338)) ;
#138433=CARTESIAN_POINT('Ctrl Pts',(-12.9189151717186,13.6633971798664,
134.804245408245)) ;
#138434=CARTESIAN_POINT('Ctrl Pts',(-12.9180538654643,13.3943409624926,
134.83481321692)) ;
#138435=CARTESIAN_POINT('Ctrl Pts',(-12.8935049395089,13.1257595222001,
134.796388178548)) ;
#138436=CARTESIAN_POINT('Ctrl Pts',(-12.846763798285,12.880696500419,134.692848177627)) ;
#138437=CARTESIAN_POINT('Ctrl Pts',(-12.7801601096525,12.6734734022958,
134.531398034018)) ;
#138438=CARTESIAN_POINT('Ctrl Pts',(-12.697476922483,12.5195858406816,134.323074933688)) ;
#138439=CARTESIAN_POINT('Ctrl Pts',(-12.6043494730584,12.4310932858069,
134.084172254176)) ;
#138440=CARTESIAN_POINT('Ctrl Pts',(-12.5071674014279,12.4134132661188,
133.833228867129)) ;
#138441=CARTESIAN_POINT('Ctrl Pts',(-12.4107585325106,12.468118840117,133.584832882078)) ;
#138442=CARTESIAN_POINT('Ctrl Pts',(-12.322679446483,12.5909169061166,133.360570988226)) ;
#138443=CARTESIAN_POINT('Ctrl Pts',(-12.2476924053518,12.773448841542,133.174646358778)) ;
#138444=CARTESIAN_POINT('Ctrl Pts',(-12.1906716921723,13.0028153371377,
133.041232379228)) ;
#138445=CARTESIAN_POINT('Ctrl Pts',(-12.1550824724469,13.2626811935882,
132.970465210837)) ;
#138446=CARTESIAN_POINT('Ctrl Pts',(-12.1427326514074,13.5323090949329,
132.967368623297)) ;
#138447=CARTESIAN_POINT('Ctrl Pts',(-12.1536928653571,13.7963542441069,
133.032649674846)) ;
#138448=CARTESIAN_POINT('Ctrl Pts',(-12.186561825762,14.0324257207359,133.161790426664)) ;
#138449=CARTESIAN_POINT('Ctrl Pts',(-12.237904814768,14.2243211070582,133.344781568927)) ;
#138450=CARTESIAN_POINT('Ctrl Pts',(-12.3037435818566,14.3597396565784,
133.570240962877)) ;
#138451=CARTESIAN_POINT('Ctrl Pts',(-12.3787469038738,14.4280132025405,
133.822575280817)) ;
#138452=CARTESIAN_POINT('Ctrl Pts',(-12.4562812799884,14.424002708898,134.082180684632)) ;
#138453=CARTESIAN_POINT('Ctrl Pts',(-12.5304216950177,14.3482149181964,
134.331918050498)) ;
#138454=CARTESIAN_POINT('Ctrl Pts',(-12.5948207053285,14.2066839719766,
134.553078199398)) ;
#138455=CARTESIAN_POINT('Ctrl Pts',(-12.6446347356738,14.0084845387879,
134.731769140596)) ;
#138456=CARTESIAN_POINT('Ctrl Pts',(-12.675219666801,13.7679164068615,134.854314117452)) ;
#138457=CARTESIAN_POINT('Ctrl Pts',(-12.6836312574652,13.5034894092934,
134.911972405466)) ;
#138458=CARTESIAN_POINT('Ctrl Pts',(-12.6687474515576,13.2335994760701,
134.901547727802)) ;
#138459=CARTESIAN_POINT('Ctrl Pts',(-12.6307771287539,12.9764076821957,
134.823780832756)) ;
#138460=CARTESIAN_POINT('Ctrl Pts',(-12.5714387747411,12.7508792714819,
134.683681699463)) ;
#138461=CARTESIAN_POINT('Ctrl Pts',(-12.495269711498,12.5752390770026,134.494092455625)) ;
#138462=CARTESIAN_POINT('Ctrl Pts',(-12.4058116411776,12.4588915032614,
134.265916566441)) ;
#138463=CARTESIAN_POINT('Ctrl Pts',(-12.3092343034192,12.4118138319928,
134.016919850756)) ;
#138464=CARTESIAN_POINT('Ctrl Pts',(-12.2114871975486,12.4374481797596,
133.764590911581)) ;
#138465=CARTESIAN_POINT('Ctrl Pts',(-12.1195045200242,12.5333386342992,
133.528936382898)) ;
#138466=CARTESIAN_POINT('Ctrl Pts',(-12.0382298417102,12.693967439573,133.324775627438)) ;
#138467=CARTESIAN_POINT('Ctrl Pts',(-11.9738864832373,12.9050030598073,
133.169754954227)) ;
#138468=CARTESIAN_POINT('Ctrl Pts',(-11.9291410370529,13.1551457617761,
133.072300353404)) ;
#138469=CARTESIAN_POINT('Ctrl Pts',(-11.9146402414172,13.3338156180663,
133.051979646352)) ;
#138470=CARTESIAN_POINT('Ctrl Pts',(-11.9112544450943,13.4231220139207,
133.053109614684)) ;
#138471=CARTESIAN_POINT('Ctrl Pts',(-33.254172394553,13.1734341962953,127.827509047315)) ;
#138472=CARTESIAN_POINT('Ctrl Pts',(-33.2534688468502,13.1676985193225,
127.826184767787)) ;
#138473=CARTESIAN_POINT('Ctrl Pts',(-33.2419952032343,13.0762043638356,
127.804349824282)) ;
#138474=CARTESIAN_POINT('Ctrl Pts',(-33.211018017341,12.9034783486566,127.736832608067)) ;
#138475=CARTESIAN_POINT('Ctrl Pts',(-33.1463422411098,12.6923998158235,
127.580920912699)) ;
#138476=CARTESIAN_POINT('Ctrl Pts',(-33.065377068761,12.5327609203509,127.377507295976)) ;
#138477=CARTESIAN_POINT('Ctrl Pts',(-32.9727193640174,12.4368205750072,
127.140104350878)) ;
#138478=CARTESIAN_POINT('Ctrl Pts',(-32.8757794851729,12.4119420230158,
126.889847835464)) ;
#138479=CARTESIAN_POINT('Ctrl Pts',(-32.7789533634292,12.4592681400663,
126.640220455885)) ;
#138480=CARTESIAN_POINT('Ctrl Pts',(-32.6896764047084,12.5756590132109,
126.412512063749)) ;
#138481=CARTESIAN_POINT('Ctrl Pts',(-32.6130980713007,12.7528353886377,
126.221951163832)) ;
#138482=CARTESIAN_POINT('Ctrl Pts',(-32.5541688347234,12.9779971268721,
126.082927482414)) ;
#138483=CARTESIAN_POINT('Ctrl Pts',(-32.516348854518,13.2349353999384,126.005559973369)) ;
#138484=CARTESIAN_POINT('Ctrl Pts',(-32.5015321471705,13.505181868833,125.99536718027)) ;
#138485=CARTESIAN_POINT('Ctrl Pts',(-32.510255245493,13.7710456278858,126.054139208809)) ;
#138486=CARTESIAN_POINT('Ctrl Pts',(-32.5408455912521,14.0095405856191,
126.176462939078)) ;
#138487=CARTESIAN_POINT('Ctrl Pts',(-32.590617752256,14.2073760437107,126.354989070221)) ;
#138488=CARTESIAN_POINT('Ctrl Pts',(-32.6552393094493,14.348956944597,126.576879524749)) ;
#138489=CARTESIAN_POINT('Ctrl Pts',(-32.7295619569501,14.4243647503837,
126.827206857336)) ;
#138490=CARTESIAN_POINT('Ctrl Pts',(-32.8071231055973,14.4276726038888,
127.086902157256)) ;
#138491=CARTESIAN_POINT('Ctrl Pts',(-32.8817223975628,14.359284576391,127.337895493878)) ;
#138492=CARTESIAN_POINT('Ctrl Pts',(-32.9474949797647,14.2239082664501,
127.563137153005)) ;
#138493=CARTESIAN_POINT('Ctrl Pts',(-32.999013802318,14.0309431435162,127.74678778598)) ;
#138494=CARTESIAN_POINT('Ctrl Pts',(-33.0317243912484,13.7937232390813,
127.875568072026)) ;
#138495=CARTESIAN_POINT('Ctrl Pts',(-33.0424700880379,13.531836984712,127.939937825762)) ;
#138496=CARTESIAN_POINT('Ctrl Pts',(-33.0300282628962,13.2609088557136,
127.936734091393)) ;
#138497=CARTESIAN_POINT('Ctrl Pts',(-32.994203922637,13.0011531405438,127.865290221919)) ;
#138498=CARTESIAN_POINT('Ctrl Pts',(-32.9373619772109,12.7729627395585,
127.732251961769)) ;
#138499=CARTESIAN_POINT('Ctrl Pts',(-32.8621917971211,12.590180168645,127.545858859501)) ;
#138500=CARTESIAN_POINT('Ctrl Pts',(-32.7739701282575,12.4676467946536,
127.321209066395)) ;
#138501=CARTESIAN_POINT('Ctrl Pts',(-32.6775709057836,12.4133145045735,
127.072830523477)) ;
#138502=CARTESIAN_POINT('Ctrl Pts',(-32.5802381988428,12.4313808939379,
126.821499331578)) ;
#138503=CARTESIAN_POINT('Ctrl Pts',(-32.4869911846938,12.5206603265203,
126.58231361496)) ;
#138504=CARTESIAN_POINT('Ctrl Pts',(-32.4047353688031,12.6744195884329,
126.37511283223)) ;
#138505=CARTESIAN_POINT('Ctrl Pts',(-32.338169138496,12.8815893082003,126.21375488428)) ;
#138506=CARTESIAN_POINT('Ctrl Pts',(-32.2912803241275,13.1290193256912,
126.110059137956)) ;
#138507=CARTESIAN_POINT('Ctrl Pts',(-32.267198005655,13.3950772370959,126.072668147979)) ;
#138508=CARTESIAN_POINT('Ctrl Pts',(-32.2663142294123,13.664342206485,126.103200803217)) ;
#138509=CARTESIAN_POINT('Ctrl Pts',(-32.2883903421483,13.9170737521182,
126.200907060451)) ;
#138510=CARTESIAN_POINT('Ctrl Pts',(-32.3308821384472,14.1334228172292,
126.358124830198)) ;
#138511=CARTESIAN_POINT('Ctrl Pts',(-32.3899729784829,14.2989215646412,
126.563802409089)) ;
#138512=CARTESIAN_POINT('Ctrl Pts',(-32.4609168345964,14.402143447902,126.804164375536)) ;
#138513=CARTESIAN_POINT('Ctrl Pts',(-32.5380332606012,14.4351203022994,
127.062647207067)) ;
#138514=CARTESIAN_POINT('Ctrl Pts',(-32.6144820010754,14.3956460287634,
127.319015942137)) ;
#138515=CARTESIAN_POINT('Ctrl Pts',(-32.6847316352454,14.2864256341772,
127.557403369739)) ;
#138516=CARTESIAN_POINT('Ctrl Pts',(-32.7426623087253,14.1149876043022,
127.75980911474)) ;
#138517=CARTESIAN_POINT('Ctrl Pts',(-32.7832798440404,13.8950778661998,
127.911480378731)) ;
#138518=CARTESIAN_POINT('Ctrl Pts',(-32.8033292316642,13.6402949079638,
128.003230304667)) ;
#138519=CARTESIAN_POINT('Ctrl Pts',(-32.8003337734113,13.3700135183461,
128.027639269137)) ;
#138520=CARTESIAN_POINT('Ctrl Pts',(-32.773914625545,13.1040820554216,127.983559770344)) ;
#138521=CARTESIAN_POINT('Ctrl Pts',(-32.7252938610734,12.8608603578453,
127.874624004567)) ;
#138522=CARTESIAN_POINT('Ctrl Pts',(-32.6567428432369,12.6570995418072,
127.707633197288)) ;
#138523=CARTESIAN_POINT('Ctrl Pts',(-32.5735389098173,12.5097125952048,
127.497535908456)) ;
#138524=CARTESIAN_POINT('Ctrl Pts',(-32.4797522125056,12.4266925714705,
127.256729982278)) ;
#138525=CARTESIAN_POINT('Ctrl Pts',(-32.3819584315157,12.4153566152999,
127.00416817041)) ;
#138526=CARTESIAN_POINT('Ctrl Pts',(-32.2863523147031,12.4761183658278,
126.757991426057)) ;
#138527=CARTESIAN_POINT('Ctrl Pts',(-32.1990413692234,12.604611036471,126.536036538651)) ;
#138528=CARTESIAN_POINT('Ctrl Pts',(-32.1254036781347,12.7920329725734,
126.35408287723)) ;
#138529=CARTESIAN_POINT('Ctrl Pts',(-32.0702238718563,13.0246460204259,
126.226026939548)) ;
#138530=CARTESIAN_POINT('Ctrl Pts',(-32.0366919182254,13.2849676562724,
126.161110348471)) ;
#138531=CARTESIAN_POINT('Ctrl Pts',(-32.026266023829,13.5561839498762,126.163818075152)) ;
#138532=CARTESIAN_POINT('Ctrl Pts',(-32.0392886640995,13.8182130447303,
126.235079805905)) ;
#138533=CARTESIAN_POINT('Ctrl Pts',(-32.0737307971117,14.0504674828932,
126.36870340205)) ;
#138534=CARTESIAN_POINT('Ctrl Pts',(-32.1268661482956,14.2392688566164,
126.55716210234)) ;
#138535=CARTESIAN_POINT('Ctrl Pts',(-32.1938216509952,14.3686949061628,
126.785894949115)) ;
#138536=CARTESIAN_POINT('Ctrl Pts',(-32.2687100849035,14.4303698699092,
127.037630197794)) ;
#138537=CARTESIAN_POINT('Ctrl Pts',(-32.3463747404381,14.4203874335836,
127.297695953386)) ;
#138538=CARTESIAN_POINT('Ctrl Pts',(-32.4201156741376,14.3383234077631,
127.546348738078)) ;
#138539=CARTESIAN_POINT('Ctrl Pts',(-32.4835082392893,14.1909246948651,
127.764639666828)) ;
#138540=CARTESIAN_POINT('Ctrl Pts',(-32.5315157767965,13.9894771952072,
127.937873715533)) ;
#138541=CARTESIAN_POINT('Ctrl Pts',(-32.5603116476677,13.746808334038,128.05511465854)) ;
#138542=CARTESIAN_POINT('Ctrl Pts',(-32.5668625656013,13.4802543050363,
128.107448081919)) ;
#138543=CARTESIAN_POINT('Ctrl Pts',(-32.5497368890375,13.2092850864011,
128.090661385991)) ;
#138544=CARTESIAN_POINT('Ctrl Pts',(-32.510114480248,12.9563426654799,128.007794570266)) ;
#138545=CARTESIAN_POINT('Ctrl Pts',(-32.4492538079865,12.7340442860679,
127.863247929968)) ;
#138546=CARTESIAN_POINT('Ctrl Pts',(-32.3711351066077,12.5620254392794,
127.668219995262)) ;
#138547=CARTESIAN_POINT('Ctrl Pts',(-32.281331276348,12.4521634534599,127.438836619194)) ;
#138548=CARTESIAN_POINT('Ctrl Pts',(-32.1840100969233,12.411069828673,127.187814281084)) ;
#138549=CARTESIAN_POINT('Ctrl Pts',(-32.0867350208807,12.4431134787165,
126.936774455973)) ;
#138550=CARTESIAN_POINT('Ctrl Pts',(-31.9956180924333,12.544720782059,126.703612975735)) ;
#138551=CARTESIAN_POINT('Ctrl Pts',(-31.9157829218615,12.7094608145556,
126.503527981435)) ;
#138552=CARTESIAN_POINT('Ctrl Pts',(-31.8525238410862,12.9261933483464,
126.351960947211)) ;
#138553=CARTESIAN_POINT('Ctrl Pts',(-31.8100237861107,13.176771832056,126.260796481775)) ;
#138554=CARTESIAN_POINT('Ctrl Pts',(-31.7900313135677,13.4474343122789,
126.235698128778)) ;
#138555=CARTESIAN_POINT('Ctrl Pts',(-31.7937452734304,13.7143157583518,
126.279598518457)) ;
#138556=CARTESIAN_POINT('Ctrl Pts',(-31.8196615228194,13.9601208974721,
126.388299879067)) ;
#138557=CARTESIAN_POINT('Ctrl Pts',(-31.865811538458,14.1691500345588,126.556373712908)) ;
#138558=CARTESIAN_POINT('Ctrl Pts',(-31.9274739976856,14.3234012984993,
126.769521897676)) ;
#138559=CARTESIAN_POINT('Ctrl Pts',(-32.0001208151247,14.4138714488527,
127.014915132275)) ;
#138560=CARTESIAN_POINT('Ctrl Pts',(-32.0773542138778,14.4332950677581,
127.273601287544)) ;
#138561=CARTESIAN_POINT('Ctrl Pts',(-32.1536561858525,14.3798376866145,
127.529813962779)) ;
#138562=CARTESIAN_POINT('Ctrl Pts',(-32.2215753737412,14.2584887466458,
127.761209299702)) ;
#138563=CARTESIAN_POINT('Ctrl Pts',(-32.2766035496271,14.0772214658074,
127.95508324656)) ;
#138564=CARTESIAN_POINT('Ctrl Pts',(-32.3137764626411,13.8478580499734,
128.096937414159)) ;
#138565=CARTESIAN_POINT('Ctrl Pts',(-32.329402655682,13.5896599466639,128.175623457458)) ;
#138566=CARTESIAN_POINT('Ctrl Pts',(-32.3220622392593,13.3195389388511,
128.187229696327)) ;
#138567=CARTESIAN_POINT('Ctrl Pts',(-32.2912364524646,13.0556170681804,
128.130382402966)) ;
#138568=CARTESIAN_POINT('Ctrl Pts',(-32.2386415673211,12.818934352168,128.009823588916)) ;
#138569=CARTESIAN_POINT('Ctrl Pts',(-32.1671306632537,12.6251003449816,
127.834066176529)) ;
#138570=CARTESIAN_POINT('Ctrl Pts',(-32.0812904327446,12.4887479439426,
127.616396241464)) ;
#138571=CARTESIAN_POINT('Ctrl Pts',(-31.9865273733683,12.4190670413713,
127.372638502282)) ;
#138572=CARTESIAN_POINT('Ctrl Pts',(-31.8883365010758,12.4213699793115,
127.119029492639)) ;
#138573=CARTESIAN_POINT('Ctrl Pts',(-31.7939808471855,12.4953802453317,
126.876454271148)) ;
#138574=CARTESIAN_POINT('Ctrl Pts',(-31.7087526630847,12.6359572118525,
126.660632380682)) ;
#138575=CARTESIAN_POINT('Ctrl Pts',(-31.638371937277,12.8329197331058,126.488156516072)) ;
#138576=CARTESIAN_POINT('Ctrl Pts',(-31.587081585685,13.0719649791817,126.371428492643)) ;
#138577=CARTESIAN_POINT('Ctrl Pts',(-31.5577681893857,13.3363497207088,
126.318926492673)) ;
#138578=CARTESIAN_POINT('Ctrl Pts',(-31.5518637801405,13.6070576774105,
126.33481999986)) ;
#138579=CARTESIAN_POINT('Ctrl Pts',(-31.5690715493904,13.8644611915849,
126.418217608229)) ;
#138580=CARTESIAN_POINT('Ctrl Pts',(-31.6073534542258,14.0900773002825,
126.56314616954)) ;
#138581=CARTESIAN_POINT('Ctrl Pts',(-31.6633899820247,14.2682172577694,
126.759999465483)) ;
#138582=CARTESIAN_POINT('Ctrl Pts',(-31.7321264723496,14.385416608164,126.993843349614)) ;
#138583=CARTESIAN_POINT('Ctrl Pts',(-31.8082726742393,14.4341663222017,
127.249410666497)) ;
#138584=CARTESIAN_POINT('Ctrl Pts',(-31.8857066502997,14.4102121268538,
127.508823758604)) ;
#138585=CARTESIAN_POINT('Ctrl Pts',(-31.957687983606,14.3156229092393,127.752193887258)) ;
#138586=CARTESIAN_POINT('Ctrl Pts',(-32.0186786327333,14.157111727064,127.963488944682)) ;
#138587=CARTESIAN_POINT('Ctrl Pts',(-32.0634925232266,13.9459764019392,
128.127527380573)) ;
#138588=CARTESIAN_POINT('Ctrl Pts',(-32.0881992235517,13.6975622305703,
128.232806642455)) ;
#138589=CARTESIAN_POINT('Ctrl Pts',(-32.0903191081306,13.4293975003276,
128.272118760355)) ;
#138590=CARTESIAN_POINT('Ctrl Pts',(-32.0690179306767,13.1610019390536,
128.242981289226)) ;
#138591=CARTESIAN_POINT('Ctrl Pts',(-32.0248932540369,12.910584846224,128.147279547823)) ;
#138592=CARTESIAN_POINT('Ctrl Pts',(-31.960630679398,12.6976134707592,127.992652895403)) ;
#138593=CARTESIAN_POINT('Ctrl Pts',(-31.8799759896631,12.536442281865,127.790164137919)) ;
#138594=CARTESIAN_POINT('Ctrl Pts',(-31.788053718589,12.4387732267397,127.554739933416)) ;
#138595=CARTESIAN_POINT('Ctrl Pts',(-31.6904186112103,12.4116342438423,
127.302714437302)) ;
#138596=CARTESIAN_POINT('Ctrl Pts',(-31.5939692116319,12.4569142421678,
127.054018327164)) ;
#138597=CARTESIAN_POINT('Ctrl Pts',(-31.5042485299717,12.5714751922183,
126.825069413096)) ;
#138598=CARTESIAN_POINT('Ctrl Pts',(-31.4273555423138,12.7468633179545,
126.633538896743)) ;
#138599=CARTESIAN_POINT('Ctrl Pts',(-31.367851407675,12.9706872906827,126.492823909801)) ;
#138600=CARTESIAN_POINT('Ctrl Pts',(-31.3293429699657,13.2271705417113,
126.413473945479)) ;
#138601=CARTESIAN_POINT('Ctrl Pts',(-31.3138511575412,13.4971329945125,
126.401288433693)) ;
#138602=CARTESIAN_POINT('Ctrl Pts',(-31.3218793728741,13.7633005745665,
126.458013409239)) ;
#138603=CARTESIAN_POINT('Ctrl Pts',(-31.3518046568443,14.0028268383939,
126.578386485857)) ;
#138604=CARTESIAN_POINT('Ctrl Pts',(-31.4013169171817,14.2028677697453,
126.756297177419)) ;
#138605=CARTESIAN_POINT('Ctrl Pts',(-31.4653538450798,14.3455611528234,
126.976348571448)) ;
#138606=CARTESIAN_POINT('Ctrl Pts',(-31.5394673004167,14.4231516441217,
127.226068639417)) ;
#138607=CARTESIAN_POINT('Ctrl Pts',(-31.6170364965111,14.428665737009,127.485791349647)) ;
#138608=CARTESIAN_POINT('Ctrl Pts',(-31.6919586235444,14.3621069846461,
127.737801861754)) ;
#138609=CARTESIAN_POINT('Ctrl Pts',(-31.7580050485926,14.2287343396627,
127.963800714979)) ;
#138610=CARTESIAN_POINT('Ctrl Pts',(-31.8101229715983,14.0363061322534,
128.149332590931)) ;
#138611=CARTESIAN_POINT('Ctrl Pts',(-31.8431612103325,13.8023697285695,
128.2787580194)) ;
#138612=CARTESIAN_POINT('Ctrl Pts',(-31.8547450705058,13.5388532599518,
128.345858145807)) ;
#138613=CARTESIAN_POINT('Ctrl Pts',(-31.842860978612,13.2684518599204,128.344212601708)) ;
#138614=CARTESIAN_POINT('Ctrl Pts',(-31.8079018909361,13.0087997166185,
128.275192118151)) ;
#138615=CARTESIAN_POINT('Ctrl Pts',(-31.751135231145,12.7778890822412,128.142629564991)) ;
#138616=CARTESIAN_POINT('Ctrl Pts',(-31.67695004648,12.5950173960976,127.958860305201)) ;
#138617=CARTESIAN_POINT('Ctrl Pts',(-31.5886131786522,12.4700325121189,
127.734044153826)) ;
#138618=CARTESIAN_POINT('Ctrl Pts',(-31.4928932673828,12.4138573722268,
127.487454181968)) ;
#138619=CARTESIAN_POINT('Ctrl Pts',(-31.3946517212827,12.4301864266095,
127.23377328525)) ;
#138620=CARTESIAN_POINT('Ctrl Pts',(-31.302186280418,12.5166844150512,126.996510890305)) ;
#138621=CARTESIAN_POINT('Ctrl Pts',(-31.2190229561058,12.6693064963876,
126.786854472266)) ;
#138622=CARTESIAN_POINT('Ctrl Pts',(-31.1521847913265,12.8745471287187,
126.62458980109)) ;
#138623=CARTESIAN_POINT('Ctrl Pts',(-31.1045636243091,13.1212023718215,
126.51878814528)) ;
#138624=CARTESIAN_POINT('Ctrl Pts',(-31.0797814964469,13.3871939110425,
126.479383704405)) ;
#138625=CARTESIAN_POINT('Ctrl Pts',(-31.0782395647314,13.6567281745513,
126.508004128684)) ;
#138626=CARTESIAN_POINT('Ctrl Pts',(-31.0996004868119,13.9097854264049,
126.603554803648)) ;
#138627=CARTESIAN_POINT('Ctrl Pts',(-31.1416644050721,14.1280196368697,
126.759621636509)) ;
#138628=CARTESIAN_POINT('Ctrl Pts',(-31.2002751272883,14.2950456004005,
126.96385849581)) ;
#138629=CARTESIAN_POINT('Ctrl Pts',(-31.2714095173753,14.4005267631623,
127.204975566894)) ;
#138630=CARTESIAN_POINT('Ctrl Pts',(-31.3479251409683,14.4350836721885,
127.461472071147)) ;
#138631=CARTESIAN_POINT('Ctrl Pts',(-31.4245699151336,14.397803897227,127.718459118213)) ;
#138632=CARTESIAN_POINT('Ctrl Pts',(-31.4950050286166,14.2905756800978,
127.957348403359)) ;
#138633=CARTESIAN_POINT('Ctrl Pts',(-31.5533719277229,14.1209511451637,
128.161017706247)) ;
#138634=CARTESIAN_POINT('Ctrl Pts',(-31.5946288792335,13.9018371823522,
128.314620751464)) ;
#138635=CARTESIAN_POINT('Ctrl Pts',(-31.6152556872759,13.6479071387663,
128.408037368887)) ;
#138636=CARTESIAN_POINT('Ctrl Pts',(-31.6130251791501,13.378501800303,128.434595124285)) ;
#138637=CARTESIAN_POINT('Ctrl Pts',(-31.5870806772977,13.1105161208594,
128.392113797471)) ;
#138638=CARTESIAN_POINT('Ctrl Pts',(-31.5392287688349,12.8677236673919,
128.285256983731)) ;
#138639=CARTESIAN_POINT('Ctrl Pts',(-31.4714257078563,12.662830762423,128.120378994299)) ;
#138640=CARTESIAN_POINT('Ctrl Pts',(-31.3883963482576,12.513091865374,127.910882483852)) ;
#138641=CARTESIAN_POINT('Ctrl Pts',(-31.2945615714775,12.4280189029097,
127.670021941709)) ;
#138642=CARTESIAN_POINT('Ctrl Pts',(-31.1970838031679,12.4146728655739,
127.418286318199)) ;
#138643=CARTESIAN_POINT('Ctrl Pts',(-31.1011085411165,12.473418288016,127.171104026254)) ;
#138644=CARTESIAN_POINT('Ctrl Pts',(-31.0133901877585,12.6005220564223,
126.948009354706)) ;
#138645=CARTESIAN_POINT('Ctrl Pts',(-30.9396697281207,12.7855011637684,
126.765646212268)) ;
#138646=CARTESIAN_POINT('Ctrl Pts',(-30.8837990280299,13.0169860566136,
126.63558907916)) ;
#138647=CARTESIAN_POINT('Ctrl Pts',(-30.849522212533,13.2774553414867,126.568584359704)) ;
#138648=CARTESIAN_POINT('Ctrl Pts',(-30.8384800040019,13.5483711409958,
126.569459216869)) ;
#138649=CARTESIAN_POINT('Ctrl Pts',(-30.8507215021823,13.8100859907312,
126.638320403832)) ;
#138650=CARTESIAN_POINT('Ctrl Pts',(-30.8846778654308,14.0443620014337,
126.770654851182)) ;
#138651=CARTESIAN_POINT('Ctrl Pts',(-30.9371383935864,14.2339606584883,
126.95701638284)) ;
#138652=CARTESIAN_POINT('Ctrl Pts',(-31.0037048768907,14.3656339537851,
127.184617706613)) ;
#138653=CARTESIAN_POINT('Ctrl Pts',(-31.0788096488771,14.4296685423803,
127.437147488283)) ;
#138654=CARTESIAN_POINT('Ctrl Pts',(-31.1562803975842,14.4216217772437,
127.696556501827)) ;
#138655=CARTESIAN_POINT('Ctrl Pts',(-31.2299712909159,14.3422174229119,
127.944936003485)) ;
#138656=CARTESIAN_POINT('Ctrl Pts',(-31.294011633153,14.1963612940614,128.165233556202)) ;
#138657=CARTESIAN_POINT('Ctrl Pts',(-31.342628260302,13.9958156297376,128.340321291151)) ;
#138658=CARTESIAN_POINT('Ctrl Pts',(-31.3719914321145,13.7540871657713,
128.459213318105)) ;
#138659=CARTESIAN_POINT('Ctrl Pts',(-31.379207947723,13.4887318093835,128.513395282888)) ;
#138660=CARTESIAN_POINT('Ctrl Pts',(-31.3628630615942,13.2176490073036,
128.498882111054)) ;
#138661=CARTESIAN_POINT('Ctrl Pts',(-31.32374522082,12.9629384302475,128.417620087759)) ;
#138662=CARTESIAN_POINT('Ctrl Pts',(-31.2633013934625,12.739445641898,128.274321947507)) ;
#138663=CARTESIAN_POINT('Ctrl Pts',(-31.1860840193193,12.5666312573546,
128.081740255708)) ;
#138664=CARTESIAN_POINT('Ctrl Pts',(-31.0960617266757,12.4542159373709,
127.851907106863)) ;
#138665=CARTESIAN_POINT('Ctrl Pts',(-30.9994012366927,12.4113528375642,
127.602620647228)) ;
#138666=CARTESIAN_POINT('Ctrl Pts',(-30.9018203547689,12.4409689765868,
127.350762761079)) ;
#138667=CARTESIAN_POINT('Ctrl Pts',(-30.8100561805039,12.5412370849313,
127.115855320823)) ;
#138668=CARTESIAN_POINT('Ctrl Pts',(-30.7300852082415,12.7041353047709,
126.915290807566)) ;
#138669=CARTESIAN_POINT('Ctrl Pts',(-30.6664814262111,12.9183855347654,
126.762561452756)) ;
#138670=CARTESIAN_POINT('Ctrl Pts',(-30.6230851071898,13.1698655571926,
126.669003863828)) ;
#138671=CARTESIAN_POINT('Ctrl Pts',(-30.6025564144617,13.4380609714907,
126.642060785656)) ;
#138672=CARTESIAN_POINT('Ctrl Pts',(-30.6054938183217,13.7071666281258,
126.683923819577)) ;
#138673=CARTESIAN_POINT('Ctrl Pts',(-30.630925020495,13.95380880599,126.791224928952)) ;
#138674=CARTESIAN_POINT('Ctrl Pts',(-30.6763240529893,14.1634527040787,
126.956971615764)) ;
#138675=CARTESIAN_POINT('Ctrl Pts',(-30.737907981033,14.3201289862677,127.170056594989)) ;
#138676=CARTESIAN_POINT('Ctrl Pts',(-30.8100090399554,14.4121340944115,
127.413701128809)) ;
#138677=CARTESIAN_POINT('Ctrl Pts',(-30.8874666938385,14.4336855937072,
127.673168883096)) ;
#138678=CARTESIAN_POINT('Ctrl Pts',(-30.9634149457897,14.3827385924792,
127.928128807699)) ;
#138679=CARTESIAN_POINT('Ctrl Pts',(-31.0321462262809,14.2627494461532,
128.162120074418)) ;
#138680=CARTESIAN_POINT('Ctrl Pts',(-31.0876101736151,14.0822576993362,
128.357331855187)) ;
#138681=CARTESIAN_POINT('Ctrl Pts',(-31.1250526967628,13.856193146146,128.499670462433)) ;
#138682=CARTESIAN_POINT('Ctrl Pts',(-31.1415133894991,13.5974242111817,
128.580965284718)) ;
#138683=CARTESIAN_POINT('Ctrl Pts',(-31.1348285122354,13.3273251704849,
128.594485415842)) ;
#138684=CARTESIAN_POINT('Ctrl Pts',(-31.1045448692166,13.062291125414,128.539308802384)) ;
#138685=CARTESIAN_POINT('Ctrl Pts',(-31.0527329307778,12.8256130125541,
128.420899764611)) ;
#138686=CARTESIAN_POINT('Ctrl Pts',(-30.98174722609,12.6301798373562,128.246682571427)) ;
#138687=CARTESIAN_POINT('Ctrl Pts',(-30.8962505494071,12.4918476261695,
128.030023021322)) ;
#138688=CARTESIAN_POINT('Ctrl Pts',(-30.8012573749623,12.4199209769537,
127.785732954429)) ;
#138689=CARTESIAN_POINT('Ctrl Pts',(-30.703212119019,12.4204246059211,127.53249886009)) ;
#138690=CARTESIAN_POINT('Ctrl Pts',(-30.6089279234257,12.492159634428,127.290042373906)) ;
#138691=CARTESIAN_POINT('Ctrl Pts',(-30.5232601554124,12.6310173484571,
127.072968873371)) ;
#138692=CARTESIAN_POINT('Ctrl Pts',(-30.4524467312471,12.8262647723397,
126.899189775226)) ;
#138693=CARTESIAN_POINT('Ctrl Pts',(-30.4004805626087,13.0646914718589,
126.780542586656)) ;
#138694=CARTESIAN_POINT('Ctrl Pts',(-30.3705408361266,13.3278245014775,
126.72611222664)) ;
#138695=CARTESIAN_POINT('Ctrl Pts',(-30.3639236278037,13.5998586000628,
126.740078803271)) ;
#138696=CARTESIAN_POINT('Ctrl Pts',(-30.3804440847528,13.8569827516154,
126.821346278327)) ;
#138697=CARTESIAN_POINT('Ctrl Pts',(-30.4182185553018,14.0842219381739,
126.964864025402)) ;
#138698=CARTESIAN_POINT('Ctrl Pts',(-30.4735865343095,14.2634336188574,
127.159646811296)) ;
#138699=CARTESIAN_POINT('Ctrl Pts',(-30.5424536748966,14.3833954818559,
127.39408651496)) ;
#138700=CARTESIAN_POINT('Ctrl Pts',(-30.6185595912135,14.433698045123,127.6495579438)) ;
#138701=CARTESIAN_POINT('Ctrl Pts',(-30.6955385718699,14.412015772317,127.90742294184)) ;
#138702=CARTESIAN_POINT('Ctrl Pts',(-30.7679798384188,14.319294669833,128.152234187299)) ;
#138703=CARTESIAN_POINT('Ctrl Pts',(-30.829320400999,14.16255830471,128.364526767623)) ;
#138704=CARTESIAN_POINT('Ctrl Pts',(-30.8747794144243,13.9521768757504,
128.530537740434)) ;
#138705=CARTESIAN_POINT('Ctrl Pts',(-30.9000057378481,13.7045477413862,
128.637327125319)) ;
#138706=CARTESIAN_POINT('Ctrl Pts',(-30.9028301887914,13.4377490344594,
128.678565653954)) ;
#138707=CARTESIAN_POINT('Ctrl Pts',(-30.8820826030584,13.1678476271901,
128.651204751086)) ;
#138708=CARTESIAN_POINT('Ctrl Pts',(-30.8387479936137,12.917659013908,128.55767070028)) ;
#138709=CARTESIAN_POINT('Ctrl Pts',(-30.7747422547336,12.7025601696351,
128.403936479543)) ;
#138710=CARTESIAN_POINT('Ctrl Pts',(-30.6948870245618,12.5405894739967,
128.203610760336)) ;
#138711=CARTESIAN_POINT('Ctrl Pts',(-30.6029778904066,12.4405287595892,
127.968321122167)) ;
#138712=CARTESIAN_POINT('Ctrl Pts',(-30.5054387564785,12.4114132283242,
127.716562065288)) ;
#138713=CARTESIAN_POINT('Ctrl Pts',(-30.4089272864758,12.4546443819082,
127.467672427643)) ;
#138714=CARTESIAN_POINT('Ctrl Pts',(-30.3190828257142,12.5668919742526,
127.238290564815)) ;
#138715=CARTESIAN_POINT('Ctrl Pts',(-30.241370659299,12.7415276223377,127.044530125261)) ;
#138716=CARTESIAN_POINT('Ctrl Pts',(-30.1814937744117,12.963899300171,126.902662765778)) ;
#138717=CARTESIAN_POINT('Ctrl Pts',(-30.1423835997439,13.2191082670462,
126.821485055972)) ;
#138718=CARTESIAN_POINT('Ctrl Pts',(-30.1261920888456,13.4893534858843,
126.807309521278)) ;
#138719=CARTESIAN_POINT('Ctrl Pts',(-30.1334829442477,13.7553188833262,
126.861793756427)) ;
#138720=CARTESIAN_POINT('Ctrl Pts',(-30.1629779883077,13.9971251681561,
126.981096376392)) ;
#138721=CARTESIAN_POINT('Ctrl Pts',(-30.2118917393662,14.1977811573069,
127.157151224366)) ;
#138722=CARTESIAN_POINT('Ctrl Pts',(-30.2755695825853,14.3424510805747,
127.37616964476)) ;
#138723=CARTESIAN_POINT('Ctrl Pts',(-30.3497741256928,14.4220642873528,
127.6262727592)) ;
#138724=CARTESIAN_POINT('Ctrl Pts',(-30.4269392595461,14.429449097017,127.884649436958)) ;
#138725=CARTESIAN_POINT('Ctrl Pts',(-30.5019897574921,14.3652072331767,
128.137012614321)) ;
#138726=CARTESIAN_POINT('Ctrl Pts',(-30.5684475923327,14.2335291681656,
128.364251880874)) ;
#138727=CARTESIAN_POINT('Ctrl Pts',(-30.6210233478071,14.0429179829767,
128.551080403811)) ;
#138728=CARTESIAN_POINT('Ctrl Pts',(-30.6547155048059,13.8093220415122,
128.682513972031)) ;
#138729=CARTESIAN_POINT('Ctrl Pts',(-30.6669672711903,13.5476217971459,
128.751402838105)) ;
#138730=CARTESIAN_POINT('Ctrl Pts',(-30.655673207762,13.2750711815888,128.751743570291)) ;
#138731=CARTESIAN_POINT('Ctrl Pts',(-30.6214425269047,13.0163164213971,
128.684671616842)) ;
#138732=CARTESIAN_POINT('Ctrl Pts',(-30.5654915322016,12.7846451556795,
128.554417669839)) ;
#138733=CARTESIAN_POINT('Ctrl Pts',(-30.4915451337098,12.5995256384001,
128.371457049536)) ;
#138734=CARTESIAN_POINT('Ctrl Pts',(-30.4034941667108,12.4726551517152,
128.14748281173)) ;
#138735=CARTESIAN_POINT('Ctrl Pts',(-30.3078437177502,12.4145513421249,
127.901121998884)) ;
#138736=CARTESIAN_POINT('Ctrl Pts',(-30.210077288083,12.4284690605263,127.648651011996)) ;
#138737=CARTESIAN_POINT('Ctrl Pts',(-30.1167874583968,12.5133431684666,
127.409191485807)) ;
#138738=CARTESIAN_POINT('Ctrl Pts',(-30.0333107867574,12.6644367182662,
127.198609743159)) ;
#138739=CARTESIAN_POINT('Ctrl Pts',(-29.9660994199644,12.8679925564765,
127.035199525246)) ;
#138740=CARTESIAN_POINT('Ctrl Pts',(-29.9179046187407,13.1131690365504,
126.927653178102)) ;
#138741=CARTESIAN_POINT('Ctrl Pts',(-29.8923276220366,13.3800002802051,
126.886075570865)) ;
#138742=CARTESIAN_POINT('Ctrl Pts',(-29.890221558393,13.6495651704166,126.913031740464)) ;
#138743=CARTESIAN_POINT('Ctrl Pts',(-29.9108230270758,13.9023388943094,
127.006224631618)) ;
#138744=CARTESIAN_POINT('Ctrl Pts',(-29.9524567704631,14.1226577783971,
127.161152165549)) ;
#138745=CARTESIAN_POINT('Ctrl Pts',(-30.0105822434621,14.2908247544057,
127.363910457664)) ;
#138746=CARTESIAN_POINT('Ctrl Pts',(-30.0810607522141,14.3981040604,127.602953490958)) ;
#138747=CARTESIAN_POINT('Ctrl Pts',(-30.1580346362768,14.4352626925802,
127.861027386541)) ;
#138748=CARTESIAN_POINT('Ctrl Pts',(-30.2348501197493,14.3995540245642,
128.118555932153)) ;
#138749=CARTESIAN_POINT('Ctrl Pts',(-30.3051990221144,14.2948938638273,
128.357020944154)) ;
#138750=CARTESIAN_POINT('Ctrl Pts',(-30.3643203908641,14.125950965529,128.563084862304)) ;
#138751=CARTESIAN_POINT('Ctrl Pts',(-30.4059231271862,13.9085226432365,
128.717598399571)) ;
#138752=CARTESIAN_POINT('Ctrl Pts',(-30.4271781973549,13.655740461518,128.812805228058)) ;
#138753=CARTESIAN_POINT('Ctrl Pts',(-30.425651180432,13.3866405451627,128.841404541009)) ;
#138754=CARTESIAN_POINT('Ctrl Pts',(-30.400385551166,13.1181024213027,128.800927702681)) ;
#138755=CARTESIAN_POINT('Ctrl Pts',(-30.3531378768886,12.8743682814219,
128.695842135408)) ;
#138756=CARTESIAN_POINT('Ctrl Pts',(-30.2858450507144,12.6679957327003,
128.532463254719)) ;
#138757=CARTESIAN_POINT('Ctrl Pts',(-30.2030436364601,12.5164144034558,
128.323684166742)) ;
#138758=CARTESIAN_POINT('Ctrl Pts',(-30.1097735403851,12.4295970264179,
128.08434965657)) ;
#138759=CARTESIAN_POINT('Ctrl Pts',(-30.0120243335714,12.4140261333183,
127.831928581667)) ;
#138760=CARTESIAN_POINT('Ctrl Pts',(-29.9160583223097,12.4707103278581,
127.584718425012)) ;
#138761=CARTESIAN_POINT('Ctrl Pts',(-29.8280269609598,12.5959068144279,
127.360711064938)) ;
#138762=CARTESIAN_POINT('Ctrl Pts',(-29.7538191838626,12.7791142632462,
127.176904989675)) ;
#138763=CARTESIAN_POINT('Ctrl Pts',(-29.6970483927431,13.0114293123004,
127.044472850966)) ;
#138764=CARTESIAN_POINT('Ctrl Pts',(-29.6625029707419,13.2689899400059,
126.976374860837)) ;
#138765=CARTESIAN_POINT('Ctrl Pts',(-29.6506529182366,13.5409257328685,
126.975025452337)) ;
#138766=CARTESIAN_POINT('Ctrl Pts',(-29.6622871843877,13.8029840857302,
127.0420891238)) ;
#138767=CARTESIAN_POINT('Ctrl Pts',(-29.6957058732804,14.0385608749257,
127.17289415219)) ;
#138768=CARTESIAN_POINT('Ctrl Pts',(-29.7477029788471,14.2294231057281,
127.357883843032)) ;
#138769=CARTESIAN_POINT('Ctrl Pts',(-29.8138291653475,14.3627051490732,
127.584145435595)) ;
#138770=CARTESIAN_POINT('Ctrl Pts',(-29.8888069040326,14.428833416405,127.836321972772)) ;
#138771=CARTESIAN_POINT('Ctrl Pts',(-29.9663255096702,14.4228924472986,
128.095881765559)) ;
#138772=CARTESIAN_POINT('Ctrl Pts',(-30.0404179941072,14.3451234315922,
128.345531442974)) ;
#138773=CARTESIAN_POINT('Ctrl Pts',(-30.1046981850006,14.2008972781255,
128.566497642975)) ;
#138774=CARTESIAN_POINT('Ctrl Pts',(-30.1536677639362,14.0023960154245,
128.742513477709)) ;
#138775=CARTESIAN_POINT('Ctrl Pts',(-30.1836978229632,13.761031796391,128.863433474315)) ;
#138776=CARTESIAN_POINT('Ctrl Pts',(-30.1915169666826,13.4967569826491,
128.919290575306)) ;
#138777=CARTESIAN_POINT('Ctrl Pts',(-30.1759417647318,13.2257685669237,
128.906995280774)) ;
#138778=CARTESIAN_POINT('Ctrl Pts',(-30.1373175281481,12.9695426329055,
128.827285395953)) ;
#138779=CARTESIAN_POINT('Ctrl Pts',(-30.0776169751352,12.7456271817385,
128.686048533487)) ;
#138780=CARTESIAN_POINT('Ctrl Pts',(-30.0008439016691,12.5709695365104,
128.494781054778)) ;
#138781=CARTESIAN_POINT('Ctrl Pts',(-29.9109937297079,12.4565179124428,
128.265492257497)) ;
#138782=CARTESIAN_POINT('Ctrl Pts',(-29.8144178586128,12.411477377022,128.016458751721)) ;
#138783=CARTESIAN_POINT('Ctrl Pts',(-29.7164129546977,12.4394645473503,
127.763492166737)) ;
#138784=CARTESIAN_POINT('Ctrl Pts',(-29.625114422541,12.5368907011572,127.52967566749)) ;
#138785=CARTESIAN_POINT('Ctrl Pts',(-29.5440581310289,12.6994727139768,
127.326227681724)) ;
#138786=CARTESIAN_POINT('Ctrl Pts',(-29.4803519777916,12.9112843857967,
127.172992697851)) ;
#138787=CARTESIAN_POINT('Ctrl Pts',(-29.4360704062874,13.1634090116609,
127.077046478387)) ;
#138788=CARTESIAN_POINT('Ctrl Pts',(-29.4151050777489,13.4300956070728,
127.048666359922)) ;
#138789=CARTESIAN_POINT('Ctrl Pts',(-29.4172038600174,13.698548706025,127.087953020284)) ;
#138790=CARTESIAN_POINT('Ctrl Pts',(-29.4422283626999,13.948024671753,127.194334375548)) ;
#138791=CARTESIAN_POINT('Ctrl Pts',(-29.4869173656092,14.1576527891806,
127.357820579509)) ;
#138792=CARTESIAN_POINT('Ctrl Pts',(-29.54801221472,14.3162850237807,127.569468256761)) ;
#138793=CARTESIAN_POINT('Ctrl Pts',(-29.6202346404057,14.4106899925297,
127.813623734569)) ;
#138794=CARTESIAN_POINT('Ctrl Pts',(-29.6976609528792,14.4339585114454,
128.073008187915)) ;
#138795=CARTESIAN_POINT('Ctrl Pts',(-29.7734049144381,14.3853107611265,
128.327226370468)) ;
#138796=CARTESIAN_POINT('Ctrl Pts',(-29.8426107800081,14.2669554182004,
128.562689628014)) ;
#138797=CARTESIAN_POINT('Ctrl Pts',(-29.8984038160143,14.0883945818005,
128.758789145186)) ;
#138798=CARTESIAN_POINT('Ctrl Pts',(-29.9364668210969,13.8631867563802,
128.902988584739)) ;
#138799=CARTESIAN_POINT('Ctrl Pts',(-29.9535661140654,13.6057120624757,
128.986065149413)) ;
#138800=CARTESIAN_POINT('Ctrl Pts',(-29.9475514809259,13.3350528446723,
129.001627031904)) ;
#138801=CARTESIAN_POINT('Ctrl Pts',(-29.9181077464122,13.0707553542234,
128.948747970018)) ;
#138802=CARTESIAN_POINT('Ctrl Pts',(-29.8668527383469,12.8321486706852,
128.832067893954)) ;
#138803=CARTESIAN_POINT('Ctrl Pts',(-29.7959514293353,12.634462986152,128.658259481005)) ;
#138804=CARTESIAN_POINT('Ctrl Pts',(-29.7111770706639,12.4951761871636,
128.443552553311)) ;
#138805=CARTESIAN_POINT('Ctrl Pts',(-29.6165727185072,12.4210996152358,
128.200337064967)) ;
#138806=CARTESIAN_POINT('Ctrl Pts',(-29.5184173364358,12.4192964203799,
127.946818896369)) ;
#138807=CARTESIAN_POINT('Ctrl Pts',(-29.4237333839853,12.4890492296412,
127.703265098707)) ;
#138808=CARTESIAN_POINT('Ctrl Pts',(-29.3374665646916,12.6268326997912,
127.48455927018)) ;
#138809=CARTESIAN_POINT('Ctrl Pts',(-29.2666068879605,12.8195830933143,
127.310453192169)) ;
#138810=CARTESIAN_POINT('Ctrl Pts',(-29.2139088518931,13.0571002340723,
127.189701884794)) ;
#138811=CARTESIAN_POINT('Ctrl Pts',(-29.1832978923029,13.3202805814274,
127.133374035993)) ;
#138812=CARTESIAN_POINT('Ctrl Pts',(-29.1759731508813,13.5914916661993,
127.145159393094)) ;
#138813=CARTESIAN_POINT('Ctrl Pts',(-29.1919413561174,13.850556640903,127.224987369683)) ;
#138814=CARTESIAN_POINT('Ctrl Pts',(-29.2289910736229,14.0777829295082,
127.366223885127)) ;
#138815=CARTESIAN_POINT('Ctrl Pts',(-29.2839846556262,14.2590886329476,
127.559987926514)) ;
#138816=CARTESIAN_POINT('Ctrl Pts',(-29.3524816976542,14.3807166913486,
127.79330782417)) ;
#138817=CARTESIAN_POINT('Ctrl Pts',(-29.4283854204452,14.433343612586,128.048161723033)) ;
#138818=CARTESIAN_POINT('Ctrl Pts',(-29.5059240605093,14.4133893592863,
128.307883829415)) ;
#138819=CARTESIAN_POINT('Ctrl Pts',(-29.5781203155356,14.3229978195751,
128.551770260296)) ;
#138820=CARTESIAN_POINT('Ctrl Pts',(-29.6399314292429,14.1680350137977,
128.765464698261)) ;
#138821=CARTESIAN_POINT('Ctrl Pts',(-29.685826677058,13.9594347962821,128.932682676008)) ;
#138822=CARTESIAN_POINT('Ctrl Pts',(-29.7118119049308,13.7128291828127,
129.041685973137)) ;
#138823=CARTESIAN_POINT('Ctrl Pts',(-29.7152244342629,13.4442543360426,
129.084901531975)) ;
#138824=CARTESIAN_POINT('Ctrl Pts',(-29.6953684239956,13.1766944104108,
129.059817600421)) ;
#138825=CARTESIAN_POINT('Ctrl Pts',(-29.6523051959867,12.9234094695572,
128.967384298863)) ;
#138826=CARTESIAN_POINT('Ctrl Pts',(-29.5891931535503,12.7086523153548,
128.816031681833)) ;
#138827=CARTESIAN_POINT('Ctrl Pts',(-29.5096878148105,12.5444332786266,
128.616788035257)) ;
#138828=CARTESIAN_POINT('Ctrl Pts',(-29.4176707271872,12.4422654276919,
128.381300524419)) ;
#138829=CARTESIAN_POINT('Ctrl Pts',(-29.3206187587525,12.4113238218205,
128.13082546281)) ;
#138830=CARTESIAN_POINT('Ctrl Pts',(-29.2239159231989,12.4521999821779,
127.881398011169)) ;
#138831=CARTESIAN_POINT('Ctrl Pts',(-29.1332913036832,12.5635389919688,
127.649940033755)) ;
#138832=CARTESIAN_POINT('Ctrl Pts',(-29.0557674545012,12.7354102649258,
127.456478979614)) ;
#138833=CARTESIAN_POINT('Ctrl Pts',(-28.9951475479058,12.9568498172893,
127.312508336806)) ;
#138834=CARTESIAN_POINT('Ctrl Pts',(-28.9553615529616,13.2117694586679,
127.229401671249)) ;
#138835=CARTESIAN_POINT('Ctrl Pts',(-28.9385143715075,13.4825284922973,
127.213391239786)) ;
#138836=CARTESIAN_POINT('Ctrl Pts',(-28.9452357718578,13.7484828909248,
127.266167041443)) ;
#138837=CARTESIAN_POINT('Ctrl Pts',(-28.973991992575,13.9900671084782,127.383159255252)) ;
#138838=CARTESIAN_POINT('Ctrl Pts',(-29.0222446858003,14.1922209027102,
127.557244848018)) ;
#138839=CARTESIAN_POINT('Ctrl Pts',(-29.0859598821377,14.3393855403521,
127.776572340874)) ;
#138840=CARTESIAN_POINT('Ctrl Pts',(-29.1593133178373,14.4204077329138,
128.023897295284)) ;
#138841=CARTESIAN_POINT('Ctrl Pts',(-29.23685478466,14.4304302154213,128.283550561485)) ;
#138842=CARTESIAN_POINT('Ctrl Pts',(-29.312289340566,14.367871152587,128.537132753714)) ;
#138843=CARTESIAN_POINT('Ctrl Pts',(-29.3790948094322,14.2376927603017,
128.765418469869)) ;
#138844=CARTESIAN_POINT('Ctrl Pts',(-29.4319637198198,14.0489883287211,
128.953014743318)) ;
#138845=CARTESIAN_POINT('Ctrl Pts',(-29.4663009452838,13.8164456424353,
129.086339965454)) ;
#138846=CARTESIAN_POINT('Ctrl Pts',(-29.4791076386463,13.5541089152985,
129.156990353639)) ;
#138847=CARTESIAN_POINT('Ctrl Pts',(-29.4686796127963,13.2846772722545,
129.159471786986)) ;
#138848=CARTESIAN_POINT('Ctrl Pts',(-29.4349222155091,13.0230235410346,
129.094073521591)) ;
#138849=CARTESIAN_POINT('Ctrl Pts',(-29.3796180661493,12.790872732509,128.965627833144)) ;
#138850=CARTESIAN_POINT('Ctrl Pts',(-29.3059833398163,12.603871831162,128.783651650281)) ;
#138851=CARTESIAN_POINT('Ctrl Pts',(-29.2185690761389,12.4755978216217,
128.561414059103)) ;
#138852=CARTESIAN_POINT('Ctrl Pts',(-29.122841974274,12.4151865443115,128.31491351705)) ;
#138853=CARTESIAN_POINT('Ctrl Pts',(-29.0251621540499,12.4270410572104,
128.062652651585)) ;
#138854=CARTESIAN_POINT('Ctrl Pts',(-28.9316571387812,12.5098502555296,
127.822566531605)) ;
#138855=CARTESIAN_POINT('Ctrl Pts',(-28.847833803276,12.6589866002263,127.610948437538)) ;
#138856=CARTESIAN_POINT('Ctrl Pts',(-28.7799886758662,12.8615686944882,
127.445752679704)) ;
#138857=CARTESIAN_POINT('Ctrl Pts',(-28.7313057367753,13.1050266274507,
127.336673069078)) ;
#138858=CARTESIAN_POINT('Ctrl Pts',(-28.7049815446916,13.3718443687466,
127.292967742919)) ;
#138859=CARTESIAN_POINT('Ctrl Pts',(-28.7020980093711,13.6411904118671,
127.317589764157)) ;
#138860=CARTESIAN_POINT('Ctrl Pts',(-28.7223401648118,13.8968634944342,
127.41003902009)) ;
#138861=CARTESIAN_POINT('Ctrl Pts',(-28.7629973543961,14.1159779670334,
127.561745464258)) ;
#138862=CARTESIAN_POINT('Ctrl Pts',(-28.8210947372898,14.287325697854,127.764689801619)) ;
#138863=CARTESIAN_POINT('Ctrl Pts',(-28.8911765229029,14.3958947367542,
128.002481753305)) ;
#138864=CARTESIAN_POINT('Ctrl Pts',(-28.9677972904603,14.4351265100489,
128.259425785411)) ;
#138865=CARTESIAN_POINT('Ctrl Pts',(-29.0446691431128,14.401957868372,128.517089841033)) ;
#138866=CARTESIAN_POINT('Ctrl Pts',(-29.1157706503648,14.2982652104899,
128.758002104881)) ;
#138867=CARTESIAN_POINT('Ctrl Pts',(-29.174779918269,14.132480207139,128.96343389952)) ;
#138868=CARTESIAN_POINT('Ctrl Pts',(-29.2172302832933,13.915462827869,129.120592596423)) ;
#138869=CARTESIAN_POINT('Ctrl Pts',(-29.2390983208705,13.6633712465324,
129.217586381667)) ;
#138870=CARTESIAN_POINT('Ctrl Pts',(-29.2382024002942,13.3940849462189,
129.248083384228)) ;
#138871=CARTESIAN_POINT('Ctrl Pts',(-29.2137553366703,13.1263052775463,
129.209852895038)) ;
#138872=CARTESIAN_POINT('Ctrl Pts',(-29.1668939996439,12.8804158751522,
129.106068734867)) ;
#138873=CARTESIAN_POINT('Ctrl Pts',(-29.1002691947144,12.6733662983206,
128.944544491779)) ;
#138874=CARTESIAN_POINT('Ctrl Pts',(-29.0177318506309,12.5197379232373,
128.736592399109)) ;
#138875=CARTESIAN_POINT('Ctrl Pts',(-28.9246399778716,12.4310982173194,
128.497785172193)) ;
#138876=CARTESIAN_POINT('Ctrl Pts',(-28.8272015701286,12.4134628281618,
128.246181903058)) ;
#138877=CARTESIAN_POINT('Ctrl Pts',(-28.7310026168688,12.4679867371616,
127.998320592069)) ;
#138878=CARTESIAN_POINT('Ctrl Pts',(-28.6424524610437,12.5916525516401,
127.772874061218)) ;
#138879=CARTESIAN_POINT('Ctrl Pts',(-28.5678961190025,12.7734684549556,
127.588037430388)) ;
#138880=CARTESIAN_POINT('Ctrl Pts',(-28.5108566436919,13.0028688411228,
127.454584278807)) ;
#138881=CARTESIAN_POINT('Ctrl Pts',(-28.475281642713,13.2619624535534,127.383760848204)) ;
#138882=CARTESIAN_POINT('Ctrl Pts',(-28.4629023861597,13.5340192322936,
127.380880702846)) ;
#138883=CARTESIAN_POINT('Ctrl Pts',(-28.4738518656341,13.7955675293532,
127.44581956107)) ;
#138884=CARTESIAN_POINT('Ctrl Pts',(-28.5066666855688,14.0322613707932,
127.574868316922)) ;
#138885=CARTESIAN_POINT('Ctrl Pts',(-28.5581068487113,14.224389834904,127.758189515183)) ;
#138886=CARTESIAN_POINT('Ctrl Pts',(-28.623975139686,14.3598901194567,127.983749503875)) ;
#138887=CARTESIAN_POINT('Ctrl Pts',(-28.6991366399092,14.4280176273918,
128.236609523979)) ;
#138888=CARTESIAN_POINT('Ctrl Pts',(-28.7761803352426,14.4241023725172,
128.494570372186)) ;
#138889=CARTESIAN_POINT('Ctrl Pts',(-28.8506922742166,14.3482280088461,
128.745549346044)) ;
#138890=CARTESIAN_POINT('Ctrl Pts',(-28.91518277418,14.2060724290961,128.967049520542)) ;
#138891=CARTESIAN_POINT('Ctrl Pts',(-28.9647186270019,14.0086808494732,
129.144776576755)) ;
#138892=CARTESIAN_POINT('Ctrl Pts',(-28.995315357535,13.7691471639152,129.267239987643)) ;
#138893=CARTESIAN_POINT('Ctrl Pts',(-29.003848162705,13.5031160987729,129.325457231296)) ;
#138894=CARTESIAN_POINT('Ctrl Pts',(-28.9888212723258,13.2327334020777,
129.314673937566)) ;
#138895=CARTESIAN_POINT('Ctrl Pts',(-28.9509676621617,12.9767766707072,
129.237101723994)) ;
#138896=CARTESIAN_POINT('Ctrl Pts',(-28.891964848477,12.7518157375075,129.097860192288)) ;
#138897=CARTESIAN_POINT('Ctrl Pts',(-28.8153017480323,12.5749030577416,
128.907053863378)) ;
#138898=CARTESIAN_POINT('Ctrl Pts',(-28.7258829233603,12.458725868686,128.678963656753)) ;
#138899=CARTESIAN_POINT('Ctrl Pts',(-28.6289134490532,12.4118884071783,
128.428957018799)) ;
#138900=CARTESIAN_POINT('Ctrl Pts',(-28.5321954393679,12.4371447951342,
128.179276015019)) ;
#138901=CARTESIAN_POINT('Ctrl Pts',(-28.4395504661701,12.5335140178268,
127.941927262626)) ;
#138902=CARTESIAN_POINT('Ctrl Pts',(-28.358807949602,12.6929505633227,127.739083313665)) ;
#138903=CARTESIAN_POINT('Ctrl Pts',(-28.2939499289173,12.9053983623053,
127.582807097336)) ;
#138904=CARTESIAN_POINT('Ctrl Pts',(-28.2495091684995,13.1539498796381,
127.486020971058)) ;
#138905=CARTESIAN_POINT('Ctrl Pts',(-28.2275303414602,13.4226750818637,
127.454981599478)) ;
#138906=CARTESIAN_POINT('Ctrl Pts',(-28.2290607143686,13.6910891460654,
127.492564996296)) ;
#138907=CARTESIAN_POINT('Ctrl Pts',(-28.2534186782273,13.9413684453662,
127.59699357478)) ;
#138908=CARTESIAN_POINT('Ctrl Pts',(-28.2977067840336,14.1526799208371,
127.759377008187)) ;
#138909=CARTESIAN_POINT('Ctrl Pts',(-28.3583229693319,14.3125333416555,
127.969564685725)) ;
#138910=CARTESIAN_POINT('Ctrl Pts',(-28.430074904473,14.4088194589569,128.212248741583)) ;
#138911=CARTESIAN_POINT('Ctrl Pts',(-28.507718384322,14.4343198918705,128.472390079449)) ;
#138912=CARTESIAN_POINT('Ctrl Pts',(-28.5834398035334,14.3877722127897,
128.726476676245)) ;
#138913=CARTESIAN_POINT('Ctrl Pts',(-28.6530124243077,14.2711471004472,
128.963054741333)) ;
#138914=CARTESIAN_POINT('Ctrl Pts',(-28.7090122067586,14.0951742684999,
129.159592602646)) ;
#138915=CARTESIAN_POINT('Ctrl Pts',(-28.7478941350473,13.870335354891,129.306328889926)) ;
#138916=CARTESIAN_POINT('Ctrl Pts',(-28.7656138027504,13.612835927565,129.391292786156)) ;
#138917=CARTESIAN_POINT('Ctrl Pts',(-28.760252313802,13.3431053086278,129.408666110812)) ;
#138918=CARTESIAN_POINT('Ctrl Pts',(-28.7315959991371,13.0784069754049,
129.358066094416)) ;
#138919=CARTESIAN_POINT('Ctrl Pts',(-28.6804303391378,12.8371325485697,
129.241909814744)) ;
#138920=CARTESIAN_POINT('Ctrl Pts',(-28.6106432947035,12.6399915744991,
129.071040346761)) ;
#138921=CARTESIAN_POINT('Ctrl Pts',(-28.5258257524472,12.4979352646964,
128.856384789912)) ;
#138922=CARTESIAN_POINT('Ctrl Pts',(-28.4311698505634,12.4220838603556,
128.613084383185)) ;
#138923=CARTESIAN_POINT('Ctrl Pts',(-28.3332246094965,12.4184701300548,
128.360113050716)) ;
#138924=CARTESIAN_POINT('Ctrl Pts',(-28.2387034924304,12.4860424705287,
128.116923333277)) ;
#138925=CARTESIAN_POINT('Ctrl Pts',(-28.1523073475974,12.6212970350437,
127.897736801008)) ;
#138926=CARTESIAN_POINT('Ctrl Pts',(-28.0805635000624,12.8133839848722,
127.721209553133)) ;
#138927=CARTESIAN_POINT('Ctrl Pts',(-28.0272630926043,13.050364922785,127.598747545585)) ;
#138928=CARTESIAN_POINT('Ctrl Pts',(-27.9961045931269,13.3123037538977,
127.540725506652)) ;
#138929=CARTESIAN_POINT('Ctrl Pts',(-27.988069139493,13.5832778951352,127.550400311311)) ;
#138930=CARTESIAN_POINT('Ctrl Pts',(-28.0033125395844,13.8428843681781,
127.628091882332)) ;
#138931=CARTESIAN_POINT('Ctrl Pts',(-28.0398912028952,14.0720013140808,
127.768057926957)) ;
#138932=CARTESIAN_POINT('Ctrl Pts',(-28.0944259765686,14.2546155515289,
127.960459672568)) ;
#138933=CARTESIAN_POINT('Ctrl Pts',(-28.1624219515475,14.3779471461467,
128.192231859961)) ;
#138934=CARTESIAN_POINT('Ctrl Pts',(-28.2382878170761,14.4327785489293,
128.447023007249)) ;
#138935=CARTESIAN_POINT('Ctrl Pts',(-28.3156214450991,14.4152048482771,
128.706033814232)) ;
#138936=CARTESIAN_POINT('Ctrl Pts',(-28.3883959682431,14.3266409658442,
128.95175809986)) ;
#138937=CARTESIAN_POINT('Ctrl Pts',(-28.4506693198691,14.1729214945641,
129.16686318667)) ;
#138938=CARTESIAN_POINT('Ctrl Pts',(-28.4969327062817,13.9662155459552,
129.335062608003)) ;
#138939=CARTESIAN_POINT('Ctrl Pts',(-28.5235541022144,13.7208186783693,
129.445890143364)) ;
#138940=CARTESIAN_POINT('Ctrl Pts',(-28.5276980643996,13.4521886748155,
129.491290359284)) ;
#138941=CARTESIAN_POINT('Ctrl Pts',(-28.5084074025572,13.1838897462868,
129.467926441214)) ;
#138942=CARTESIAN_POINT('Ctrl Pts',(-28.4662760617063,12.9313138678917,
129.378013345421)) ;
#138943=CARTESIAN_POINT('Ctrl Pts',(-28.4035475729084,12.7142071157524,
129.227914504089)) ;
#138944=CARTESIAN_POINT('Ctrl Pts',(-28.3242366485113,12.5481822862925,
129.029307411766)) ;
#138945=CARTESIAN_POINT('Ctrl Pts',(-28.2329991415399,12.4445945495957,
128.795913433975)) ;
#138946=CARTESIAN_POINT('Ctrl Pts',(-28.1359471520329,12.4110615292549,
128.54547048254)) ;
#138947=CARTESIAN_POINT('Ctrl Pts',(-28.0386871379967,12.4502003410622,
128.294574669809)) ;
#138948=CARTESIAN_POINT('Ctrl Pts',(-27.9484093855994,12.5587981584367,
128.063898629952)) ;
#138949=CARTESIAN_POINT('Ctrl Pts',(-27.8701354737038,12.7290992999271,
127.86833698565)) ;
#138950=CARTESIAN_POINT('Ctrl Pts',(-27.8086851646448,12.9505642966122,
127.722109781574)) ;
#138951=CARTESIAN_POINT('Ctrl Pts',(-27.7684638902634,13.2039533885785,
127.637616969587)) ;
#138952=CARTESIAN_POINT('Ctrl Pts',(-27.7509048587101,13.4737768400672,
127.619438918027)) ;
#138953=CARTESIAN_POINT('Ctrl Pts',(-27.7568758422641,13.7408243528461,
127.670098038824)) ;
#138954=CARTESIAN_POINT('Ctrl Pts',(-27.7852338217469,13.9843828533781,
127.786086236129)) ;
#138955=CARTESIAN_POINT('Ctrl Pts',(-27.8327593266423,14.1867700455966,
127.957871750746)) ;
#138956=CARTESIAN_POINT('Ctrl Pts',(-27.896139879253,14.3360223311849,128.176262697775)) ;
#138957=CARTESIAN_POINT('Ctrl Pts',(-27.9692983079035,14.4190304968155,
128.423017998671)) ;
#138958=CARTESIAN_POINT('Ctrl Pts',(-28.0467984639361,14.4311357374112,
128.682548584271)) ;
#138959=CARTESIAN_POINT('Ctrl Pts',(-28.1222733369049,14.3708887924222,
128.936189065257)) ;
#138960=CARTESIAN_POINT('Ctrl Pts',(-28.1895265325835,14.2422926877059,
129.165851645267)) ;
#138961=CARTESIAN_POINT('Ctrl Pts',(-28.2426703459913,14.0562619383273,
129.354079192252)) ;
#138962=CARTESIAN_POINT('Ctrl Pts',(-28.2778835463942,13.8231736969123,
129.490209597053)) ;
#138963=CARTESIAN_POINT('Ctrl Pts',(-28.2912600088371,13.5622216724448,
129.562407634763)) ;
#138964=CARTESIAN_POINT('Ctrl Pts',(-28.2815138099123,13.2923510388066,
129.56694118938)) ;
#138965=CARTESIAN_POINT('Ctrl Pts',(-28.2485236488303,13.0307856163929,
129.503695286891)) ;
#138966=CARTESIAN_POINT('Ctrl Pts',(-28.1936350662213,12.7967159031727,
129.376581182953)) ;
#138967=CARTESIAN_POINT('Ctrl Pts',(-28.1204881136384,12.6083942654361,
129.196006788455)) ;
#138968=CARTESIAN_POINT('Ctrl Pts',(-28.033305520065,12.4782667075604,128.97447720968)) ;
#138969=CARTESIAN_POINT('Ctrl Pts',(-27.9380490506444,12.4160107642981,
128.72924170442)) ;
#138970=CARTESIAN_POINT('Ctrl Pts',(-27.840088998415,12.425588916255,128.476245677989)) ;
#138971=CARTESIAN_POINT('Ctrl Pts',(-27.7460416419619,12.5070743322311,
128.234706957922)) ;
#138972=CARTESIAN_POINT('Ctrl Pts',(-27.6622979311355,12.6538727730597,
128.023155368527)) ;
#138973=CARTESIAN_POINT('Ctrl Pts',(-27.5938166192311,12.8553499552797,
127.85615827692)) ;
#138974=CARTESIAN_POINT('Ctrl Pts',(-27.5445346630511,13.098103384175,127.74534712503)) ;
#138975=CARTESIAN_POINT('Ctrl Pts',(-27.5175776227433,13.3649638276871,
127.69984232764)) ;
#138976=CARTESIAN_POINT('Ctrl Pts',(-27.5141163308945,13.6334094300958,
127.722651608453)) ;
#138977=CARTESIAN_POINT('Ctrl Pts',(-27.5335019356169,13.8886868396263,
127.812436729992)) ;
#138978=CARTESIAN_POINT('Ctrl Pts',(-27.5737821241816,14.1104518310445,
127.963236838802)) ;
#138979=CARTESIAN_POINT('Ctrl Pts',(-27.6314744421073,14.2832226261628,
128.164987370241)) ;
#138980=CARTESIAN_POINT('Ctrl Pts',(-27.7012379510992,14.3937886224781,
128.401835946804)) ;
#138981=CARTESIAN_POINT('Ctrl Pts',(-27.7781123535692,14.4350213815805,
128.65967036386)) ;
#138982=CARTESIAN_POINT('Ctrl Pts',(-27.8546936773711,14.4038716563582,
128.916327544499)) ;
#138983=CARTESIAN_POINT('Ctrl Pts',(-27.9261731861543,14.302057440806,129.158397140685)) ;
#138984=CARTESIAN_POINT('Ctrl Pts',(-27.9855695077338,14.1377082691097,
129.364968157342)) ;
#138985=CARTESIAN_POINT('Ctrl Pts',(-28.0284659120487,13.9225120820519,
129.523348044967)) ;
#138986=CARTESIAN_POINT('Ctrl Pts',(-28.0510262279841,13.6705375102117,
129.622450560383)) ;
#138987=CARTESIAN_POINT('Ctrl Pts',(-28.0507377584204,13.401884525291,129.654671141506)) ;
#138988=CARTESIAN_POINT('Ctrl Pts',(-28.027107292662,13.1344381659713,129.618736562433)) ;
#138989=CARTESIAN_POINT('Ctrl Pts',(-27.9806130101491,12.8864833048174,
129.516191990152)) ;
#138990=CARTESIAN_POINT('Ctrl Pts',(-27.9148391290743,12.6791960280418,
129.356978782703)) ;
#138991=CARTESIAN_POINT('Ctrl Pts',(-27.8325764038185,12.5233811391943,
129.149895121488)) ;
#138992=CARTESIAN_POINT('Ctrl Pts',(-27.7398372427668,12.4327816584244,
128.912072670328)) ;
#138993=CARTESIAN_POINT('Ctrl Pts',(-27.6421416316699,12.4129159573699,
128.659822662127)) ;
#138994=CARTESIAN_POINT('Ctrl Pts',(-27.5459275592162,12.4655032796393,
128.411880163255)) ;
#138995=CARTESIAN_POINT('Ctrl Pts',(-27.4573533230035,12.5866529362795,
128.186246122412)) ;
#138996=CARTESIAN_POINT('Ctrl Pts',(-27.3819902516143,12.7674395708452,
127.999181472755)) ;
#138997=CARTESIAN_POINT('Ctrl Pts',(-27.3242508154076,12.9966807390071,
127.863798954836)) ;
#138998=CARTESIAN_POINT('Ctrl Pts',(-27.2882667414954,13.2541241840609,
127.79164129262)) ;
#138999=CARTESIAN_POINT('Ctrl Pts',(-27.2751406243702,13.5248421394856,
127.786425007767)) ;
#139000=CARTESIAN_POINT('Ctrl Pts',(-27.2853998464079,13.7882271369091,
127.849508781125)) ;
#139001=CARTESIAN_POINT('Ctrl Pts',(-27.3176681383781,14.0260983655197,
127.97698427868)) ;
#139002=CARTESIAN_POINT('Ctrl Pts',(-27.3687529118647,14.2200231919602,
128.159335122063)) ;
#139003=CARTESIAN_POINT('Ctrl Pts',(-27.4341754696823,14.356772234067,128.383520804271)) ;
#139004=CARTESIAN_POINT('Ctrl Pts',(-27.5087046282768,14.4269174457709,
128.634342726485)) ;
#139005=CARTESIAN_POINT('Ctrl Pts',(-27.5863498095606,14.4252572954794,
128.894315325931)) ;
#139006=CARTESIAN_POINT('Ctrl Pts',(-27.6608346895068,14.3512844735739,
129.14512930489)) ;
#139007=CARTESIAN_POINT('Ctrl Pts',(-27.7254688305769,14.2117350246389,
129.366921379891)) ;
#139008=CARTESIAN_POINT('Ctrl Pts',(-27.7757715686293,14.0152548216542,
129.547011019762)) ;
#139009=CARTESIAN_POINT('Ctrl Pts',(-27.8069823814624,13.7756399540023,
129.671394466275)) ;
#139010=CARTESIAN_POINT('Ctrl Pts',(-27.8161239931437,13.5122935142519,
129.731111533612)) ;
#139011=CARTESIAN_POINT('Ctrl Pts',(-27.8018912094678,13.241130032097,129.722732596038)) ;
#139012=CARTESIAN_POINT('Ctrl Pts',(-27.7646415514717,12.9839533345939,
129.646985455023)) ;
#139013=CARTESIAN_POINT('Ctrl Pts',(-27.705971842593,12.7572239976212,129.508824746173)) ;
#139014=CARTESIAN_POINT('Ctrl Pts',(-27.6300749308619,12.5794741431288,
129.320113150862)) ;
#139015=CARTESIAN_POINT('Ctrl Pts',(-27.5407307406086,12.4611210765961,
129.092328609389)) ;
#139016=CARTESIAN_POINT('Ctrl Pts',(-27.4443925507261,12.4122668265322,
128.843989508204)) ;
#139017=CARTESIAN_POINT('Ctrl Pts',(-27.3469053180412,12.4354395083141,
128.592303176999)) ;
#139018=CARTESIAN_POINT('Ctrl Pts',(-27.2540851953818,12.5301694803305,
128.354430002177)) ;
#139019=CARTESIAN_POINT('Ctrl Pts',(-27.1731448505004,12.6876686572945,
128.150941740257)) ;
#139020=CARTESIAN_POINT('Ctrl Pts',(-27.1078519711564,12.8982124580512,
127.993318537432)) ;
#139021=CARTESIAN_POINT('Ctrl Pts',(-27.062565545524,13.1472879194742,127.894240819857)) ;
#139022=CARTESIAN_POINT('Ctrl Pts',(-27.0400556107669,13.4151706318018,
127.861572480424)) ;
#139023=CARTESIAN_POINT('Ctrl Pts',(-27.0409313353343,13.6833052731468,
127.89718448912)) ;
#139024=CARTESIAN_POINT('Ctrl Pts',(-27.0644459838438,13.9335262194554,
127.999007834601)) ;
#139025=CARTESIAN_POINT('Ctrl Pts',(-27.1085568252031,14.1479664880633,
128.161156205508)) ;
#139026=CARTESIAN_POINT('Ctrl Pts',(-27.1686539025929,14.3087959168501,
128.369723486497)) ;
#139027=CARTESIAN_POINT('Ctrl Pts',(-27.2401497732243,14.4069520231813,
128.611660947542)) ;
#139028=CARTESIAN_POINT('Ctrl Pts',(-27.3173616295847,14.4347039370495,
128.870380646342)) ;
#139029=CARTESIAN_POINT('Ctrl Pts',(-27.3937223670572,14.3899170768859,
129.12656922784)) ;
#139030=CARTESIAN_POINT('Ctrl Pts',(-27.463154389175,14.2758481834518,129.362528068667)) ;
#139031=CARTESIAN_POINT('Ctrl Pts',(-27.5198612341215,14.1010294405417,
129.561258806483)) ;
#139032=CARTESIAN_POINT('Ctrl Pts',(-27.5592797085226,13.8772034323747,
129.709569614153)) ;
#139033=CARTESIAN_POINT('Ctrl Pts',(-27.5776272327468,13.6206147260663,
129.796340563983)) ;
#139034=CARTESIAN_POINT('Ctrl Pts',(-27.5729713117708,13.3509221462812,
129.815782598542)) ;
#139035=CARTESIAN_POINT('Ctrl Pts',(-27.544865717924,13.0853829020601,129.766851005711)) ;
#139036=CARTESIAN_POINT('Ctrl Pts',(-27.494656970879,12.8445476179022,129.653285076039)) ;
#139037=CARTESIAN_POINT('Ctrl Pts',(-27.42515055289,12.6449528736105,129.483374882147)) ;
#139038=CARTESIAN_POINT('Ctrl Pts',(-27.3406844192613,12.501260652652,129.269736460329)) ;
#139039=CARTESIAN_POINT('Ctrl Pts',(-27.2465604864716,12.423505657414,129.02788025025)) ;
#139040=CARTESIAN_POINT('Ctrl Pts',(-27.1485944866452,12.4173186176401,
128.774856876374)) ;
#139041=CARTESIAN_POINT('Ctrl Pts',(-27.0533218365845,12.4833714818954,
128.529679282004)) ;
#139042=CARTESIAN_POINT('Ctrl Pts',(-26.9670098871684,12.6162285773946,
128.310578416108)) ;
#139043=CARTESIAN_POINT('Ctrl Pts',(-26.8945212967897,12.8073410485065,
128.131984688256)) ;
#139044=CARTESIAN_POINT('Ctrl Pts',(-26.8407055797364,13.0432165498209,
128.007993993565)) ;
#139045=CARTESIAN_POINT('Ctrl Pts',(-26.8088693650207,13.3046949553566,
127.94800110172)) ;
#139046=CARTESIAN_POINT('Ctrl Pts',(-26.8001804373194,13.5764463640802,
127.9558548202)) ;
#139047=CARTESIAN_POINT('Ctrl Pts',(-26.8148719233268,13.8363550328947,
128.031910726039)) ;
#139048=CARTESIAN_POINT('Ctrl Pts',(-26.8507085202357,14.0655921907836,
128.169565286129)) ;
#139049=CARTESIAN_POINT('Ctrl Pts',(-26.9049053545545,14.2503954340108,
128.36107536267)) ;
#139050=CARTESIAN_POINT('Ctrl Pts',(-26.9728396411132,14.3757154030236,
128.592765403602)) ;
#139051=CARTESIAN_POINT('Ctrl Pts',(-27.048441018008,14.4321659912553,128.846721483037)) ;
#139052=CARTESIAN_POINT('Ctrl Pts',(-27.1255622643999,14.4167343012476,
129.10500433378)) ;
#139053=CARTESIAN_POINT('Ctrl Pts',(-27.198538054879,14.3302899803119,129.351306443868)) ;
#139054=CARTESIAN_POINT('Ctrl Pts',(-27.2612573342443,14.1784243472653,
129.567722425343)) ;
#139055=CARTESIAN_POINT('Ctrl Pts',(-27.3082500797653,13.9717507603948,
129.738242510254)) ;
#139056=CARTESIAN_POINT('Ctrl Pts',(-27.3352449628971,13.7284356730931,
129.849982315497)) ;
#139057=CARTESIAN_POINT('Ctrl Pts',(-27.3401753539222,13.4606301780327,
129.897628724691)) ;
#139058=CARTESIAN_POINT('Ctrl Pts',(-27.3213949208222,13.1906192009326,
129.875943304999)) ;
#139059=CARTESIAN_POINT('Ctrl Pts',(-27.2801319319356,12.9388679840775,
129.788361151274)) ;
#139060=CARTESIAN_POINT('Ctrl Pts',(-27.2177800966894,12.7195132163599,
129.639491018548)) ;
#139061=CARTESIAN_POINT('Ctrl Pts',(-27.1386838373461,12.5518557369755,
129.441565434155)) ;
#139062=CARTESIAN_POINT('Ctrl Pts',(-27.0481377468026,12.4467157573859,
129.210037428764)) ;
#139063=CARTESIAN_POINT('Ctrl Pts',(-26.950619923967,12.4110145774445,128.958423991903)) ;
#139064=CARTESIAN_POINT('Ctrl Pts',(-26.8539313870607,12.4479828345384,
128.708971248185)) ;
#139065=CARTESIAN_POINT('Ctrl Pts',(-26.7631485338844,12.5544308128886,
128.476883218463)) ;
#139066=CARTESIAN_POINT('Ctrl Pts',(-26.6839869423467,12.7245572177545,
128.278955232461)) ;
#139067=CARTESIAN_POINT('Ctrl Pts',(-26.622452158733,12.9435039918997,128.1322624773)) ;
#139068=CARTESIAN_POINT('Ctrl Pts',(-26.5814862033874,13.1965754394182,
128.045658074214)) ;
#139069=CARTESIAN_POINT('Ctrl Pts',(-26.5633147142469,13.465805442607,128.025635976667)) ;
#139070=CARTESIAN_POINT('Ctrl Pts',(-26.5685769247246,13.7328709787398,
128.074182266888)) ;
#139071=CARTESIAN_POINT('Ctrl Pts',(-26.5962169903584,13.9772572958127,
128.188041557399)) ;
#139072=CARTESIAN_POINT('Ctrl Pts',(-26.6434704653874,14.1820529249742,
128.359201485676)) ;
#139073=CARTESIAN_POINT('Ctrl Pts',(-26.7064912763497,14.3328843736513,
128.576527484716)) ;
#139074=CARTESIAN_POINT('Ctrl Pts',(-26.779676885671,14.417801109475,128.823460886102)) ;
#139075=CARTESIAN_POINT('Ctrl Pts',(-26.8567641312626,14.4318123913692,
129.081615800254)) ;
#139076=CARTESIAN_POINT('Ctrl Pts',(-26.932696019571,14.373230288219,129.336737835572)) ;
#139077=CARTESIAN_POINT('Ctrl Pts',(-26.9999033577708,14.2469703146016,
129.56609452963)) ;
#139078=CARTESIAN_POINT('Ctrl Pts',(-27.0536419770243,14.062146501963,129.756131764833)) ;
#139079=CARTESIAN_POINT('Ctrl Pts',(-27.089338814048,13.8305007160398,129.893613733069)) ;
#139080=CARTESIAN_POINT('Ctrl Pts',(-27.1034218397827,13.5704781299009,
129.967838856659)) ;
#139081=CARTESIAN_POINT('Ctrl Pts',(-27.0943121258094,13.299460638904,129.974371676377)) ;
#139082=CARTESIAN_POINT('Ctrl Pts',(-27.061909738513,13.0377343274411,129.91280775413)) ;
#139083=CARTESIAN_POINT('Ctrl Pts',(-27.0079273099502,12.8036245820339,
129.78818096079)) ;
#139084=CARTESIAN_POINT('Ctrl Pts',(-26.9350149495085,12.6130123285287,
129.608417134988)) ;
#139085=CARTESIAN_POINT('Ctrl Pts',(-26.8483991702399,12.4813447603753,
129.388452122961)) ;
#139086=CARTESIAN_POINT('Ctrl Pts',(-26.7529748959595,12.4167223842582,
129.14284477105)) ;
#139087=CARTESIAN_POINT('Ctrl Pts',(-26.6551280409943,12.42436559993,128.890133118099)) ;
#139088=CARTESIAN_POINT('Ctrl Pts',(-26.5611337632536,12.5034382891946,
128.648655692995)) ;
#139089=CARTESIAN_POINT('Ctrl Pts',(-26.4768642655678,12.6484426384731,
128.435612464504)) ;
#139090=CARTESIAN_POINT('Ctrl Pts',(-26.4076898573312,12.8490571867036,
128.266677661264)) ;
#139091=CARTESIAN_POINT('Ctrl Pts',(-26.3578999656574,13.0907449616811,
128.154357478156)) ;
#139092=CARTESIAN_POINT('Ctrl Pts',(-26.3302906513053,13.3559778335449,
128.106800455251)) ;
#139093=CARTESIAN_POINT('Ctrl Pts',(-26.3261021407339,13.626477299062,128.127720572037)) ;
#139094=CARTESIAN_POINT('Ctrl Pts',(-26.344861958985,13.8815733654641,128.215569449386)) ;
#139095=CARTESIAN_POINT('Ctrl Pts',(-26.3845347243026,14.1045282563564,
128.364588267836)) ;
#139096=CARTESIAN_POINT('Ctrl Pts',(-26.4417677663433,14.2789670451528,
128.564989101919)) ;
#139097=CARTESIAN_POINT('Ctrl Pts',(-26.5113409516761,14.3914951714323,
128.801324455963)) ;
#139098=CARTESIAN_POINT('Ctrl Pts',(-26.5877888188324,14.434860760417,129.057773892789)) ;
#139099=CARTESIAN_POINT('Ctrl Pts',(-26.6648607758356,14.4056890526457,
129.316047449567)) ;
#139100=CARTESIAN_POINT('Ctrl Pts',(-26.7362631521833,14.3062653162723,
129.557733992972)) ;
#139101=CARTESIAN_POINT('Ctrl Pts',(-26.7962306963923,14.1434405265247,
129.766045804946)) ;
#139102=CARTESIAN_POINT('Ctrl Pts',(-26.8396812882404,13.9296996110321,
129.926022503524)) ;
#139103=CARTESIAN_POINT('Ctrl Pts',(-26.8629433105894,13.6772902073351,
130.027334699158)) ;
#139104=CARTESIAN_POINT('Ctrl Pts',(-26.8632838118661,13.4099497148246,
130.061254571472)) ;
#139105=CARTESIAN_POINT('Ctrl Pts',(-26.8403078076667,13.1418739541198,
130.027275416975)) ;
#139106=CARTESIAN_POINT('Ctrl Pts',(-26.7946473707701,12.8939990849847,
129.927034092426)) ;
#139107=CARTESIAN_POINT('Ctrl Pts',(-26.7292679370309,12.6844791056233,
129.769080119216)) ;
#139108=CARTESIAN_POINT('Ctrl Pts',(-26.6469601321073,12.5265062757821,
129.562016710345)) ;
#139109=CARTESIAN_POINT('Ctrl Pts',(-26.5549146970139,12.4345049912951,
129.326048353605)) ;
#139110=CARTESIAN_POINT('Ctrl Pts',(-26.4569589709664,12.4124896110262,
129.073148163912)) ;
#139111=CARTESIAN_POINT('Ctrl Pts',(-26.3610245559965,12.4629154938197,
128.825883391475)) ;
#139112=CARTESIAN_POINT('Ctrl Pts',(-26.271958028802,12.582091252431,128.598863247898)) ;
#139113=CARTESIAN_POINT('Ctrl Pts',(-26.1958909868628,12.7624371771161,
128.409894373029)) ;
#139114=CARTESIAN_POINT('Ctrl Pts',(-26.1381566159572,12.9881392321824,
128.27418222961)) ;
#139115=CARTESIAN_POINT('Ctrl Pts',(-26.1011574103229,13.2462582998136,
128.199249439198)) ;
#139116=CARTESIAN_POINT('Ctrl Pts',(-26.0874123015779,13.5176871774874,
128.192315615647)) ;
#139117=CARTESIAN_POINT('Ctrl Pts',(-26.0969930018115,13.7805944540118,
128.253300271888)) ;
#139118=CARTESIAN_POINT('Ctrl Pts',(-26.1286189621167,14.0195269504541,
128.378899377995)) ;
#139119=CARTESIAN_POINT('Ctrl Pts',(-26.1792019920037,14.2150385228552,
128.559789419472)) ;
#139120=CARTESIAN_POINT('Ctrl Pts',(-26.2444273756428,14.3538332825844,
128.783472919647)) ;
#139121=CARTESIAN_POINT('Ctrl Pts',(-26.3186947357783,14.425964693576,129.033487360147)) ;
#139122=CARTESIAN_POINT('Ctrl Pts',(-26.396628580836,14.4260802790596,129.294434315719)) ;
#139123=CARTESIAN_POINT('Ctrl Pts',(-26.4706207570241,14.3549350609901,
129.543496973816)) ;
#139124=CARTESIAN_POINT('Ctrl Pts',(-26.5361954761091,14.2162529068252,
129.768318600153)) ;
#139125=CARTESIAN_POINT('Ctrl Pts',(-26.5867781111596,14.0213156820109,
129.949154797901)) ;
#139126=CARTESIAN_POINT('Ctrl Pts',(-26.618586099352,13.7835942530776,130.07517850614)) ;
#139127=CARTESIAN_POINT('Ctrl Pts',(-26.6283811897984,13.5186608640693,
130.137060334724)) ;
#139128=CARTESIAN_POINT('Ctrl Pts',(-26.6148877785356,13.2494162372405,
130.13058771019)) ;
#139129=CARTESIAN_POINT('Ctrl Pts',(-26.5781030924617,12.9903691341897,
130.056369042685)) ;
#139130=CARTESIAN_POINT('Ctrl Pts',(-26.5203533297591,12.7636900645103,
129.920699862936)) ;
#139131=CARTESIAN_POINT('Ctrl Pts',(-26.4441846986195,12.58293139644,129.731499757236)) ;
#139132=CARTESIAN_POINT('Ctrl Pts',(-26.3560625112512,12.464078841243,129.506925147999)) ;
#139133=CARTESIAN_POINT('Ctrl Pts',(-26.2593259056977,12.4125693581943,
129.257617605936)) ;
#139134=CARTESIAN_POINT('Ctrl Pts',(-26.1620985485317,12.4337094194749,
129.006578106188)) ;
#139135=CARTESIAN_POINT('Ctrl Pts',(-26.0689353443424,12.5263145270348,
128.76773619341)) ;
#139136=CARTESIAN_POINT('Ctrl Pts',(-25.9875127410395,12.6822587422614,
128.562869973626)) ;
#139137=CARTESIAN_POINT('Ctrl Pts',(-25.9216923690682,12.8915625531578,
128.403716354475)) ;
#139138=CARTESIAN_POINT('Ctrl Pts',(-25.8758306390324,13.1392603074742,
128.302891273382)) ;
#139139=CARTESIAN_POINT('Ctrl Pts',(-25.8525818054641,13.4076118636345,
128.268165012633)) ;
#139140=CARTESIAN_POINT('Ctrl Pts',(-25.8527555620702,13.6757335658836,
128.301682288657)) ;
#139141=CARTESIAN_POINT('Ctrl Pts',(-25.8759296819954,13.9281677247044,
128.402731498127)) ;
#139142=CARTESIAN_POINT('Ctrl Pts',(-25.9189093686323,14.1410411495776,
128.561123729007)) ;
#139143=CARTESIAN_POINT('Ctrl Pts',(-25.9789503429921,14.3051859901722,
128.76978572316)) ;
#139144=CARTESIAN_POINT('Ctrl Pts',(-26.0501976675012,14.4050577733478,
129.010974927713)) ;
#139145=CARTESIAN_POINT('Ctrl Pts',(-26.1274137398456,14.4349188598701,
129.269745582532)) ;
#139146=CARTESIAN_POINT('Ctrl Pts',(-26.2037453942148,14.3922309368258,
129.52578709105)) ;
#139147=CARTESIAN_POINT('Ctrl Pts',(-26.2734485850338,14.2801808251174,
129.762531073939)) ;
#139148=CARTESIAN_POINT('Ctrl Pts',(-26.3306498021722,14.1070360117015,
129.962712893199)) ;
#139149=CARTESIAN_POINT('Ctrl Pts',(-26.3707342932592,13.8833119581465,
130.113115180101)) ;
#139150=CARTESIAN_POINT('Ctrl Pts',(-26.389605114305,13.6288342320535,130.20122415819)) ;
#139151=CARTESIAN_POINT('Ctrl Pts',(-26.3856317307219,13.3582466127621,
130.222792750629)) ;
#139152=CARTESIAN_POINT('Ctrl Pts',(-26.3582425741299,13.0930921970462,
130.175851547749)) ;
#139153=CARTESIAN_POINT('Ctrl Pts',(-26.3086067689133,12.8509541226963,
130.064004429468)) ;
#139154=CARTESIAN_POINT('Ctrl Pts',(-26.2396339676843,12.650062531176,129.895634211399)) ;
#139155=CARTESIAN_POINT('Ctrl Pts',(-26.1554049626922,12.504322010349,129.682740398293)) ;
#139156=CARTESIAN_POINT('Ctrl Pts',(-26.0612953645753,12.424693152161,129.440982032959)) ;
#139157=CARTESIAN_POINT('Ctrl Pts',(-25.9638486832033,12.4164961973712,
129.189306529937)) ;
#139158=CARTESIAN_POINT('Ctrl Pts',(-25.8683438504238,12.4802514111472,
128.943468158545)) ;
#139159=CARTESIAN_POINT('Ctrl Pts',(-25.7814639524611,12.6116452910191,
128.722795866727)) ;
#139160=CARTESIAN_POINT('Ctrl Pts',(-25.7086114716684,12.8011772311019,
128.543106694356)) ;
#139161=CARTESIAN_POINT('Ctrl Pts',(-25.6543263351022,13.0350450036084,
128.417626071778)) ;
#139162=CARTESIAN_POINT('Ctrl Pts',(-25.6216719385945,13.2969780565828,
128.355372970236)) ;
#139163=CARTESIAN_POINT('Ctrl Pts',(-25.6123346990145,13.5677347022496,
128.36120696557)) ;
#139164=CARTESIAN_POINT('Ctrl Pts',(-25.6262359141222,13.8283851985519,
128.434959187361)) ;
#139165=CARTESIAN_POINT('Ctrl Pts',(-25.6616701800478,14.0598714357244,
128.57160098533)) ;
#139166=CARTESIAN_POINT('Ctrl Pts',(-25.7152945842557,14.2455587727683,
128.761348553752)) ;
#139167=CARTESIAN_POINT('Ctrl Pts',(-25.7825955492344,14.3725641558704,
128.991061393796)) ;
#139168=CARTESIAN_POINT('Ctrl Pts',(-25.8582910585464,14.4315964719956,
129.245406755469)) ;
#139169=CARTESIAN_POINT('Ctrl Pts',(-25.9356294866348,14.4181824180769,
129.504398426313)) ;
#139170=CARTESIAN_POINT('Ctrl Pts',(-26.0087913243708,14.3336378097198,
129.751237877826)) ;
#139171=CARTESIAN_POINT('Ctrl Pts',(-26.0717150052296,14.1840091136267,
129.968155126164)) ;
#139172=CARTESIAN_POINT('Ctrl Pts',(-26.1192862891209,13.9789558298509,
130.140357900612)) ;
#139173=CARTESIAN_POINT('Ctrl Pts',(-26.1470311145863,13.735580763414,130.254419312679)) ;
#139174=CARTESIAN_POINT('Ctrl Pts',(-26.1525271394237,13.4678622164134,
130.303748830678)) ;
#139175=CARTESIAN_POINT('Ctrl Pts',(-26.1345823245785,13.1991328170732,
130.284317860337)) ;
#139176=CARTESIAN_POINT('Ctrl Pts',(-26.0937347645656,12.9452257159657,
130.198137101084)) ;
#139177=CARTESIAN_POINT('Ctrl Pts',(-26.0322662158017,12.7259341405257,
130.051655335126)) ;
#139178=CARTESIAN_POINT('Ctrl Pts',(-25.9535276230655,12.5559411179341,
129.854841568092)) ;
#139179=CARTESIAN_POINT('Ctrl Pts',(-25.8627268934651,12.4485460989971,
129.622745483608)) ;
#139180=CARTESIAN_POINT('Ctrl Pts',(-25.7658821421245,12.411159941536,129.372899865208)) ;
#139181=CARTESIAN_POINT('Ctrl Pts',(-25.6689843987872,12.4456278245902,
129.122866641899)) ;
#139182=CARTESIAN_POINT('Ctrl Pts',(-25.5772788439363,12.5514145649144,
128.888347222745)) ;
#139183=CARTESIAN_POINT('Ctrl Pts',(-25.4985967290999,12.7181519501975,
128.691450514129)) ;
#139184=CARTESIAN_POINT('Ctrl Pts',(-25.4361709012921,12.9364297118054,
128.542285418365)) ;
#139185=CARTESIAN_POINT('Ctrl Pts',(-25.3945996241829,13.1887531889945,
128.45390307165)) ;
#139186=CARTESIAN_POINT('Ctrl Pts',(-25.3757082658116,13.4580633394379,
128.431815240773)) ;
#139187=CARTESIAN_POINT('Ctrl Pts',(-25.3803406060574,13.7256377913563,
128.478541525222)) ;
#139188=CARTESIAN_POINT('Ctrl Pts',(-25.4073082148746,13.9704139495142,
128.590368684336)) ;
#139189=CARTESIAN_POINT('Ctrl Pts',(-25.4540453085521,14.1767864400758,
128.760039568759)) ;
#139190=CARTESIAN_POINT('Ctrl Pts',(-25.5167004953322,14.3292888579234,
128.976301083279)) ;
#139191=CARTESIAN_POINT('Ctrl Pts',(-25.5894209897251,14.4162419047305,
129.221770975587)) ;
#139192=CARTESIAN_POINT('Ctrl Pts',(-25.6669609282362,14.4323070590761,
129.481465117335)) ;
#139193=CARTESIAN_POINT('Ctrl Pts',(-25.7423474735605,14.3764282439281,
129.734680874727)) ;
#139194=CARTESIAN_POINT('Ctrl Pts',(-25.8103758869325,14.2515625460975,
129.96666241246)) ;
#139195=CARTESIAN_POINT('Ctrl Pts',(-25.8645418505469,14.0682228318719,
130.157932110319)) ;
#139196=CARTESIAN_POINT('Ctrl Pts',(-25.9008771851767,13.8370233843303,
130.297370202357)) ;
#139197=CARTESIAN_POINT('Ctrl Pts',(-25.9155226415146,13.5786249866576,
130.37309985319)) ;
#139198=CARTESIAN_POINT('Ctrl Pts',(-25.907150581353,13.3076277382397,130.381793812356)) ;
#139199=CARTESIAN_POINT('Ctrl Pts',(-25.8754438475342,13.0452573122607,
130.322268774417)) ;
#139200=CARTESIAN_POINT('Ctrl Pts',(-25.8218007897925,12.8091512622852,
130.198773291913)) ;
#139201=CARTESIAN_POINT('Ctrl Pts',(-25.7494081213582,12.617551612867,130.020477149333)) ;
#139202=CARTESIAN_POINT('Ctrl Pts',(-25.6633722315796,12.4843718023618,
129.802116135341)) ;
#139203=CARTESIAN_POINT('Ctrl Pts',(-25.5680282554624,12.4175958724791,
129.556775885265)) ;
#139204=CARTESIAN_POINT('Ctrl Pts',(-25.4702720597222,12.4230554954089,
129.304289864055)) ;
#139205=CARTESIAN_POINT('Ctrl Pts',(-25.3759369019875,12.5002516562104,
129.061871713019)) ;
#139206=CARTESIAN_POINT('Ctrl Pts',(-25.2915203838476,12.6429371553798,
128.848300314289)) ;
#139207=CARTESIAN_POINT('Ctrl Pts',(-25.2215243889668,12.8430359620073,
128.677120783399)) ;
#139208=CARTESIAN_POINT('Ctrl Pts',(-25.1713237180579,13.0829430987805,
128.563478292785)) ;
#139209=CARTESIAN_POINT('Ctrl Pts',(-25.1429774609377,13.348262589156,128.513840001074)) ;
#139210=CARTESIAN_POINT('Ctrl Pts',(-25.1380814446493,13.617980538018,128.532575804089)) ;
#139211=CARTESIAN_POINT('Ctrl Pts',(-25.1562814256738,13.8754577927148,
128.61900340648)) ;
#139212=CARTESIAN_POINT('Ctrl Pts',(-25.1955679750799,14.0994368224178,
128.766915779269)) ;
#139213=CARTESIAN_POINT('Ctrl Pts',(-25.2519785797865,14.2743408293056,
128.964695140055)) ;
#139214=CARTESIAN_POINT('Ctrl Pts',(-25.3214400334483,14.3892596729095,
129.200801570197)) ;
#139215=CARTESIAN_POINT('Ctrl Pts',(-25.3977308716843,14.4346258040112,
129.456767831054)) ;
#139216=CARTESIAN_POINT('Ctrl Pts',(-25.4750778381126,14.4074612330324,
129.715931930331)) ;
#139217=CARTESIAN_POINT('Ctrl Pts',(-25.5466694832016,14.3096987835835,
129.958166513638)) ;
#139218=CARTESIAN_POINT('Ctrl Pts',(-25.6068294845438,14.1493774031888,
130.166897650572)) ;
#139219=CARTESIAN_POINT('Ctrl Pts',(-25.6510183732772,13.935562868649,130.329231840898)) ;
#139220=CARTESIAN_POINT('Ctrl Pts',(-25.6747380783682,13.6861606118435,
130.431586420245)) ;
#139221=CARTESIAN_POINT('Ctrl Pts',(-25.6758133796976,13.4167352169348,
130.467951113991)) ;
#139222=CARTESIAN_POINT('Ctrl Pts',(-25.653459078872,13.1492793406519,130.435675091596)) ;
#139223=CARTESIAN_POINT('Ctrl Pts',(-25.6084542619497,12.9005268787558,
130.337351258316)) ;
#139224=CARTESIAN_POINT('Ctrl Pts',(-25.5435299244083,12.6897474261303,
130.180738845539)) ;
#139225=CARTESIAN_POINT('Ctrl Pts',(-25.4620224695308,12.5306016297354,
129.975863624958)) ;
#139226=CARTESIAN_POINT('Ctrl Pts',(-25.3697477074986,12.4360458848473,
129.739397853574)) ;
#139227=CARTESIAN_POINT('Ctrl Pts',(-25.2719994495299,12.412131814889,129.48704906573)) ;
#139228=CARTESIAN_POINT('Ctrl Pts',(-25.175740221563,12.4605358033904,129.238901405947)) ;
#139229=CARTESIAN_POINT('Ctrl Pts',(-25.0863095489117,12.5784164440372,
129.010871104516)) ;
#139230=CARTESIAN_POINT('Ctrl Pts',(-25.0104054959568,12.7554816677878,
128.822088090123)) ;
#139231=CARTESIAN_POINT('Ctrl Pts',(-24.9515970266411,12.981762434369,128.683509475873)) ;
#139232=CARTESIAN_POINT('Ctrl Pts',(-24.9141759784363,13.2381598405705,
128.607190779819)) ;
#139233=CARTESIAN_POINT('Ctrl Pts',(-24.8996770755616,13.5101992275675,
128.598149052653)) ;
#139234=CARTESIAN_POINT('Ctrl Pts',(-24.9086031480491,13.7733131452284,
128.657183366263)) ;
#139235=CARTESIAN_POINT('Ctrl Pts',(-24.9398052171064,14.0140641414936,
128.781675601586)) ;
#139236=CARTESIAN_POINT('Ctrl Pts',(-24.9896927765608,14.2098744851872,
128.960364452866)) ;
#139237=CARTESIAN_POINT('Ctrl Pts',(-25.0544790313913,14.350580234219,129.182743841367)) ;
#139238=CARTESIAN_POINT('Ctrl Pts',(-25.1286457194053,14.424831664933,129.432502490811)) ;
#139239=CARTESIAN_POINT('Ctrl Pts',(-25.206490431836,14.4272048065726,129.69314833904)) ;
#139240=CARTESIAN_POINT('Ctrl Pts',(-25.2808580019925,14.3577939538396,
129.943405474164)) ;
#139241=CARTESIAN_POINT('Ctrl Pts',(-25.3465032391174,14.2217457510102,
130.168270717532)) ;
#139242=CARTESIAN_POINT('Ctrl Pts',(-25.3979717151172,14.0267541205093,
130.35195733621)) ;
#139243=CARTESIAN_POINT('Ctrl Pts',(-25.4301050307948,13.7911380012518,
130.478752074177)) ;
#139244=CARTESIAN_POINT('Ctrl Pts',(-25.4406575499018,13.5273990690374,
130.542772384891)) ;
#139245=CARTESIAN_POINT('Ctrl Pts',(-25.427837941042,13.2571616705375,130.538379196713)) ;
#139246=CARTESIAN_POINT('Ctrl Pts',(-25.3916867409364,12.9974108749585,
130.466017830389)) ;
#139247=CARTESIAN_POINT('Ctrl Pts',(-25.3344256044563,12.7695379625925,
130.331802297734)) ;
#139248=CARTESIAN_POINT('Ctrl Pts',(-25.2591612456238,12.5879936819102,
130.145065778963)) ;
#139249=CARTESIAN_POINT('Ctrl Pts',(-25.1708094896904,12.4663339694794,
129.920031665293)) ;
#139250=CARTESIAN_POINT('Ctrl Pts',(-25.0742025214906,12.4130530302768,
129.671092872011)) ;
#139251=CARTESIAN_POINT('Ctrl Pts',(-24.9771023880055,12.4321501151392,
129.420369705811)) ;
#139252=CARTESIAN_POINT('Ctrl Pts',(-24.8838787240354,12.5224108071959,
129.181282199813)) ;
#139253=CARTESIAN_POINT('Ctrl Pts',(-24.8016886878617,12.6773122255345,
128.974323033663)) ;
#139254=CARTESIAN_POINT('Ctrl Pts',(-24.7354635805379,12.8853931942508,
128.813970529302)) ;
#139255=CARTESIAN_POINT('Ctrl Pts',(-24.6891442972207,13.1311434549155,
128.711670601176)) ;
#139256=CARTESIAN_POINT('Ctrl Pts',(-24.6650967559786,13.4000886960601,
128.674724701615)) ;
#139257=CARTESIAN_POINT('Ctrl Pts',(-24.6646958448049,13.6679854854521,
128.706516222695)) ;
#139258=CARTESIAN_POINT('Ctrl Pts',(-24.6869181699987,13.9198929114768,
128.804574602593)) ;
#139259=CARTESIAN_POINT('Ctrl Pts',(-24.7299417619901,14.1367331650745,
128.963529160766)) ;
#139260=CARTESIAN_POINT('Ctrl Pts',(-24.78899702236,14.3006761293965,129.168957484263)) ;
#139261=CARTESIAN_POINT('Ctrl Pts',(-24.8604323902462,14.4034182515294,
129.410928254081)) ;
#139262=CARTESIAN_POINT('Ctrl Pts',(-24.9373849419803,14.4350219442823,
129.668834674646)) ;
#139263=CARTESIAN_POINT('Ctrl Pts',(-25.0139098900193,14.3943912084008,
129.925485785032)) ;
#139264=CARTESIAN_POINT('Ctrl Pts',(-25.0838686001623,14.2842181176635,
130.162962649196)) ;
#139265=CARTESIAN_POINT('Ctrl Pts',(-25.141505675191,14.1123337883522,130.364455738094)) ;
#139266=CARTESIAN_POINT('Ctrl Pts',(-25.1819228640214,13.8914433195642,
130.515599513236)) ;
#139267=CARTESIAN_POINT('Ctrl Pts',(-25.201613141345,13.6364805830374,130.606273016799)) ;
#139268=CARTESIAN_POINT('Ctrl Pts',(-25.1983020491001,13.3663281514523,
130.629736093281)) ;
#139269=CARTESIAN_POINT('Ctrl Pts',(-25.1715470228642,13.1002904677936,
130.58470870473)) ;
#139270=CARTESIAN_POINT('Ctrl Pts',(-25.1225067421903,12.857318656671,130.474590193612)) ;
#139271=CARTESIAN_POINT('Ctrl Pts',(-25.0540277977989,12.6550558730351,
130.307664775512)) ;
#139272=CARTESIAN_POINT('Ctrl Pts',(-24.9702550119896,12.5076994857307,
130.096067377798)) ;
#139273=CARTESIAN_POINT('Ctrl Pts',(-24.8763683967754,12.4260782078646,
129.854957119094)) ;
#139274=CARTESIAN_POINT('Ctrl Pts',(-24.7789829706749,12.415541436623,129.60344254161)) ;
#139275=CARTESIAN_POINT('Ctrl Pts',(-24.6826294458462,12.4780902877727,
129.35537895735)) ;
#139276=CARTESIAN_POINT('Ctrl Pts',(-24.5962537093982,12.6066343882026,
129.135870949235)) ;
#139277=CARTESIAN_POINT('Ctrl Pts',(-24.5225844167585,12.7952136199714,
128.953931288036)) ;
#139278=CARTESIAN_POINT('Ctrl Pts',(-24.4677935144789,13.027981899229,128.826949566631)) ;
#139279=CARTESIAN_POINT('Ctrl Pts',(-24.43445736829,13.289687480561,128.762746162363)) ;
#139280=CARTESIAN_POINT('Ctrl Pts',(-24.4245047098199,13.5603128220289,
128.766764296195)) ;
#139281=CARTESIAN_POINT('Ctrl Pts',(-24.4377309514563,13.8211027693198,
128.838491234365)) ;
#139282=CARTESIAN_POINT('Ctrl Pts',(-24.4725941333539,14.0538032313773,
128.973482598895)) ;
#139283=CARTESIAN_POINT('Ctrl Pts',(-24.5257689032639,14.241090775664,129.161927643805)) ;
#139284=CARTESIAN_POINT('Ctrl Pts',(-24.5929703029174,14.3701941266746,
129.391446649845)) ;
#139285=CARTESIAN_POINT('Ctrl Pts',(-24.6684647537559,14.4308809538835,
129.645172653091)) ;
#139286=CARTESIAN_POINT('Ctrl Pts',(-24.7455934848516,14.419613884929,129.903448778638)) ;
#139287=CARTESIAN_POINT('Ctrl Pts',(-24.8191360362311,14.336836848792,130.151480211498)) ;
#139288=CARTESIAN_POINT('Ctrl Pts',(-24.8822457334504,14.1892311094166,
130.368855563618)) ;
#139289=CARTESIAN_POINT('Ctrl Pts',(-24.9303421333715,13.9859053267194,
130.542561767144)) ;
#139290=CARTESIAN_POINT('Ctrl Pts',(-24.958773115316,13.742611201067,130.658737814802)) ;
#139291=CARTESIAN_POINT('Ctrl Pts',(-24.9649012046553,13.4761438373695,
130.709803732788)) ;
#139292=CARTESIAN_POINT('Ctrl Pts',(-24.9476912211436,13.2070931418873,
130.692535709155)) ;
#139293=CARTESIAN_POINT('Ctrl Pts',(-24.9074283032168,12.9521503687759,
130.608104321017)) ;
#139294=CARTESIAN_POINT('Ctrl Pts',(-24.8465172822224,12.7315094149766,
130.463257238954)) ;
#139295=CARTESIAN_POINT('Ctrl Pts',(-24.7678429615914,12.5595225536488,
130.266760317396)) ;
#139296=CARTESIAN_POINT('Ctrl Pts',(-24.6780376574106,12.4509681334738,
130.037306136309)) ;
#139297=CARTESIAN_POINT('Ctrl Pts',(-24.5805061326321,12.4111337658692,
129.785728889855)) ;
#139298=CARTESIAN_POINT('Ctrl Pts',(-24.4839877480091,12.4436883984276,
129.536643622124)) ;
#139299=CARTESIAN_POINT('Ctrl Pts',(-24.3919596936368,12.547486739405,129.301206635287)) ;
#139300=CARTESIAN_POINT('Ctrl Pts',(-24.3129491036762,12.7123018084608,
129.103301088071)) ;
#139301=CARTESIAN_POINT('Ctrl Pts',(-24.2498169239358,12.9300708055824,
128.952180938411)) ;
#139302=CARTESIAN_POINT('Ctrl Pts',(-24.2078048366664,13.1802337524753,
128.862326668088)) ;
#139303=CARTESIAN_POINT('Ctrl Pts',(-24.1880922707095,13.4510759220384,
128.838061182578)) ;
#139304=CARTESIAN_POINT('Ctrl Pts',(-24.1921076852184,13.7180592996578,
128.882867446039)) ;
#139305=CARTESIAN_POINT('Ctrl Pts',(-24.2185138890603,13.964278608138,128.993132540059)) ;
#139306=CARTESIAN_POINT('Ctrl Pts',(-24.2646501252742,14.1712561679291,
129.160953206331)) ;
#139307=CARTESIAN_POINT('Ctrl Pts',(-24.3266399230232,14.325372518196,129.375160905542)) ;
#139308=CARTESIAN_POINT('Ctrl Pts',(-24.3997087634312,14.4148742609065,
129.621908054451)) ;
#139309=CARTESIAN_POINT('Ctrl Pts',(-24.4766126097422,14.4329087895001,
129.879481483547)) ;
#139310=CARTESIAN_POINT('Ctrl Pts',(-24.5526547839398,14.3788838445396,
130.134842622102)) ;
#139311=CARTESIAN_POINT('Ctrl Pts',(-24.6207455540188,14.2561019956526,
130.366891479371)) ;
#139312=CARTESIAN_POINT('Ctrl Pts',(-24.6754095977467,14.0742378272797,
130.559641849346)) ;
#139313=CARTESIAN_POINT('Ctrl Pts',(-24.7122096656787,13.8451950259534,
130.700297086839)) ;
#139314=CARTESIAN_POINT('Ctrl Pts',(-24.727674522459,13.5867435987056,130.778518269024)) ;
#139315=CARTESIAN_POINT('Ctrl Pts',(-24.7198654764314,13.3144405101765,
130.789020297388)) ;
#139316=CARTESIAN_POINT('Ctrl Pts',(-24.6889016208014,13.0528696187883,
130.731507643832)) ;
#139317=CARTESIAN_POINT('Ctrl Pts',(-24.6360315938546,12.8160518820106,
130.610209194301)) ;
#139318=CARTESIAN_POINT('Ctrl Pts',(-24.5640862049924,12.6226065915497,
130.433257284621)) ;
#139319=CARTESIAN_POINT('Ctrl Pts',(-24.4782156125006,12.4871997315169,
130.215449636711)) ;
#139320=CARTESIAN_POINT('Ctrl Pts',(-24.3826837946767,12.4184347778258,
129.969678308433)) ;
#139321=CARTESIAN_POINT('Ctrl Pts',(-24.285484258313,12.4219001112793,129.718626572152)) ;
#139322=CARTESIAN_POINT('Ctrl Pts',(-24.1908371872593,12.4968774308013,
129.475331098626)) ;
#139323=CARTESIAN_POINT('Ctrl Pts',(-24.1059297242578,12.6381725760813,
129.260388880534)) ;
#139324=CARTESIAN_POINT('Ctrl Pts',(-24.0356325005768,12.836067679816,129.088215051841)) ;
#139325=CARTESIAN_POINT('Ctrl Pts',(-23.9845812244526,13.0762565431926,
128.9722614937)) ;
#139326=CARTESIAN_POINT('Ctrl Pts',(-23.9557404233227,13.3398740160854,
128.921014471502)) ;
#139327=CARTESIAN_POINT('Ctrl Pts',(-23.9500932821032,13.6103043330608,
128.937631008638)) ;
#139328=CARTESIAN_POINT('Ctrl Pts',(-23.9676534068118,13.8681249215715,
129.02215077165)) ;
#139329=CARTESIAN_POINT('Ctrl Pts',(-24.0062669166322,14.093287105724,129.168070149275)) ;
#139330=CARTESIAN_POINT('Ctrl Pts',(-24.0626571938418,14.2707836403436,
129.36601232404)) ;
#139331=CARTESIAN_POINT('Ctrl Pts',(-24.1314305220899,14.3866738384329,
129.599899487544)) ;
#139332=CARTESIAN_POINT('Ctrl Pts',(-24.2076451382746,14.4343395639672,
129.855670337091)) ;
#139333=CARTESIAN_POINT('Ctrl Pts',(-24.2848983556719,14.4093417175208,
130.114493222806)) ;
#139334=CARTESIAN_POINT('Ctrl Pts',(-24.3567922015602,14.3139583331245,
130.35760755757)) ;
#139335=CARTESIAN_POINT('Ctrl Pts',(-24.4177512909038,14.1538396141847,
130.568932173959)) ;
#139336=CARTESIAN_POINT('Ctrl Pts',(-24.4620640818478,13.9434082127298,
130.731300630705)) ;
#139337=CARTESIAN_POINT('Ctrl Pts',(-24.4866543542614,13.6926166165872,
130.836506821739)) ;
#139338=CARTESIAN_POINT('Ctrl Pts',(-24.4883147442223,13.425230952717,130.874349792581)) ;
#139339=CARTESIAN_POINT('Ctrl Pts',(-24.4666758817606,13.1569924871447,
130.844230426763)) ;
#139340=CARTESIAN_POINT('Ctrl Pts',(-24.4223330200419,12.9074157476161,
130.747826094221)) ;
#139341=CARTESIAN_POINT('Ctrl Pts',(-24.3576260683162,12.6946405616374,
130.591985997049)) ;
#139342=CARTESIAN_POINT('Ctrl Pts',(-24.2771035667315,12.5348309308551,
130.389750673622)) ;
#139343=CARTESIAN_POINT('Ctrl Pts',(-24.1844908621363,12.4376124689349,
130.152515823898)) ;
#139344=CARTESIAN_POINT('Ctrl Pts',(-24.0873106866223,12.4118470514465,
129.90164747401)) ;
#139345=CARTESIAN_POINT('Ctrl Pts',(-23.9907623342062,12.4580456544619,
129.652715532171)) ;
#139346=CARTESIAN_POINT('Ctrl Pts',(-23.9012147893026,12.5736491216982,
129.424267530587)) ;
#139347=CARTESIAN_POINT('Ctrl Pts',(-23.8245652736496,12.7495591694402,
129.23341927134)) ;
#139348=CARTESIAN_POINT('Ctrl Pts',(-23.7650732037928,12.9753683734727,
129.092929090297)) ;
#139349=CARTESIAN_POINT('Ctrl Pts',(-23.7271033701168,13.2312289838448,
129.015013590769)) ;
#139350=CARTESIAN_POINT('Ctrl Pts',(-23.7119712545994,13.5022491651901,
129.004007468431)) ;
#139351=CARTESIAN_POINT('Ctrl Pts',(-23.7203019095383,13.7663767191028,
129.061383252461)) ;
#139352=CARTESIAN_POINT('Ctrl Pts',(-23.7506144849391,14.0063276697149,
129.183017107517)) ;
#139353=CARTESIAN_POINT('Ctrl Pts',(-23.8001454534432,14.2048736282249,
129.360832931781)) ;
#139354=CARTESIAN_POINT('Ctrl Pts',(-23.8648094922,14.347691195203,129.582954666991)) ;
#139355=CARTESIAN_POINT('Ctrl Pts',(-23.9388753354998,14.4237776298714,
129.832449027665)) ;
#139356=CARTESIAN_POINT('Ctrl Pts',(-24.0164983821894,14.4280807794616,
130.092358864372)) ;
#139357=CARTESIAN_POINT('Ctrl Pts',(-24.0910798904586,14.3608278808949,
130.343248164158)) ;
#139358=CARTESIAN_POINT('Ctrl Pts',(-24.1572505503088,14.2256360688744,
130.569788751767)) ;
#139359=CARTESIAN_POINT('Ctrl Pts',(-24.2086514826109,14.0344800390557,
130.752888831951)) ;
#139360=CARTESIAN_POINT('Ctrl Pts',(-24.2417573503002,13.7980436571723,
130.882815753271)) ;
#139361=CARTESIAN_POINT('Ctrl Pts',(-24.2528842234986,13.5353242806262,
130.948432556299)) ;
#139362=CARTESIAN_POINT('Ctrl Pts',(-24.2407093073429,13.2644874689488,
130.945996646237)) ;
#139363=CARTESIAN_POINT('Ctrl Pts',(-24.2053407643436,13.0050529303368,
130.875798295924)) ;
#139364=CARTESIAN_POINT('Ctrl Pts',(-24.1485465653022,12.7754380725172,
130.743031004446)) ;
#139365=CARTESIAN_POINT('Ctrl Pts',(-24.0738199872738,12.5925960491714,
130.557822597348)) ;
#139366=CARTESIAN_POINT('Ctrl Pts',(-23.9857890662773,12.4690082220502,
130.333727746733)) ;
#139367=CARTESIAN_POINT('Ctrl Pts',(-23.8893876382777,12.4135709144517,
130.085365735719)) ;
#139368=CARTESIAN_POINT('Ctrl Pts',(-23.7920567607928,12.4306394934732,
129.834034345841)) ;
#139369=CARTESIAN_POINT('Ctrl Pts',(-23.6988914891641,12.518547510187,129.595010139751)) ;
#139370=CARTESIAN_POINT('Ctrl Pts',(-23.6161714664072,12.6718440202401,
129.386557760484)) ;
#139371=CARTESIAN_POINT('Ctrl Pts',(-23.549452793789,12.8780301734486,129.224700541014)) ;
#139372=CARTESIAN_POINT('Ctrl Pts',(-23.5021872674409,13.1252486196316,
129.119942147481)) ;
#139373=CARTESIAN_POINT('Ctrl Pts',(-23.4777604477291,13.3909665583226,
129.081520904008)) ;
#139374=CARTESIAN_POINT('Ctrl Pts',(-23.4765798056597,13.6612160977101,
129.111299193796)) ;
#139375=CARTESIAN_POINT('Ctrl Pts',(-23.4982607396798,13.9131568829426,
129.207697075482)) ;
#139376=CARTESIAN_POINT('Ctrl Pts',(-23.5404707375718,14.1304384080909,
129.36412734294)) ;
#139377=CARTESIAN_POINT('Ctrl Pts',(-23.5993517273674,14.2969775123332,
129.569201224497)) ;
#139378=CARTESIAN_POINT('Ctrl Pts',(-23.6706606614751,14.4015522175217,
129.810846815782)) ;
#139379=CARTESIAN_POINT('Ctrl Pts',(-23.7472655844458,14.4350500549688,
130.067624578881)) ;
#139380=CARTESIAN_POINT('Ctrl Pts',(-23.8238068480449,14.3967519657553,
130.324283748109)) ;
#139381=CARTESIAN_POINT('Ctrl Pts',(-23.8941385602596,14.288484921225,130.56289011732)) ;
#139382=CARTESIAN_POINT('Ctrl Pts',(-23.9522769819151,14.1181740958946,
130.76587139896)) ;
#139383=CARTESIAN_POINT('Ctrl Pts',(-23.99331192498,13.897753350153,130.918917945401)) ;
#139384=CARTESIAN_POINT('Ctrl Pts',(-24.0135547856214,13.6446684780805,
131.01105286223)) ;
#139385=CARTESIAN_POINT('Ctrl Pts',(-24.0109351960766,13.3734340480479,
131.036692378548)) ;
#139386=CARTESIAN_POINT('Ctrl Pts',(-23.984750772328,13.1072276991085,130.993310697227)) ;
#139387=CARTESIAN_POINT('Ctrl Pts',(-23.9365029867963,12.8641925809132,
130.885390202893)) ;
#139388=CARTESIAN_POINT('Ctrl Pts',(-23.8685796909686,12.660522785721,130.720081448326)) ;
#139389=CARTESIAN_POINT('Ctrl Pts',(-23.7853638608259,12.511411763425,130.510055511429)) ;
#139390=CARTESIAN_POINT('Ctrl Pts',(-23.6911328337757,12.4272142219304,
130.268135624709)) ;
#139391=CARTESIAN_POINT('Ctrl Pts',(-23.5939071495122,12.4150347964973,
130.017043202023)) ;
#139392=CARTESIAN_POINT('Ctrl Pts',(-23.4980296480192,12.4747491007078,
129.770142716077)) ;
#139393=CARTESIAN_POINT('Ctrl Pts',(-23.4105558276953,12.6023245536218,
129.547706835705)) ;
#139394=CARTESIAN_POINT('Ctrl Pts',(-23.336481762881,12.7898413846695,129.364600555102)) ;
#139395=CARTESIAN_POINT('Ctrl Pts',(-23.2813353510646,13.0206706862551,
129.23645575968)) ;
#139396=CARTESIAN_POINT('Ctrl Pts',(-23.2473156516746,13.2818517746603,
129.170263348697)) ;
#139397=CARTESIAN_POINT('Ctrl Pts',(-23.2366830075241,13.5521277577084,
129.172253536318)) ;
#139398=CARTESIAN_POINT('Ctrl Pts',(-23.2492140792166,13.813956814144,129.242001480208)) ;
#139399=CARTESIAN_POINT('Ctrl Pts',(-23.2837359052188,14.0485698568868,
129.376142320652)) ;
#139400=CARTESIAN_POINT('Ctrl Pts',(-23.3361299078761,14.2361101273789,
129.562094932607)) ;
#139401=CARTESIAN_POINT('Ctrl Pts',(-23.403184331613,14.3675383856298,129.791288542673)) ;
#139402=CARTESIAN_POINT('Ctrl Pts',(-23.4783602446362,14.4300942221494,
130.044003619567)) ;
#139403=CARTESIAN_POINT('Ctrl Pts',(-23.5556298375246,14.4208865281834,
130.302748225955)) ;
#139404=CARTESIAN_POINT('Ctrl Pts',(-23.6291635545595,14.3405661224656,
130.550641869123)) ;
#139405=CARTESIAN_POINT('Ctrl Pts',(-23.6931552963386,14.1934622842168,
130.770869255254)) ;
#139406=CARTESIAN_POINT('Ctrl Pts',(-23.7415085139769,13.9917022316215,
130.945235929377)) ;
#139407=CARTESIAN_POINT('Ctrl Pts',(-23.7704326776443,13.7502056970642,
131.06273915926)) ;
#139408=CARTESIAN_POINT('Ctrl Pts',(-23.7772973067199,13.4844947698669,
131.115913754511)) ;
#139409=CARTESIAN_POINT('Ctrl Pts',(-23.7606691495744,13.2141841161546,
131.100485287274)) ;
#139410=CARTESIAN_POINT('Ctrl Pts',(-23.7211119628859,12.9589228275276,
131.018054041759)) ;
#139411=CARTESIAN_POINT('Ctrl Pts',(-23.6603186352369,12.736270288281,130.873727443309)) ;
#139412=CARTESIAN_POINT('Ctrl Pts',(-23.5832218993153,12.5648475025287,
130.681365345848)) ;
#139413=CARTESIAN_POINT('Ctrl Pts',(-23.4926718163616,12.452872634964,130.450136303181)) ;
#139414=CARTESIAN_POINT('Ctrl Pts',(-23.3961081126866,12.4112941971035,
130.201074563628)) ;
#139415=CARTESIAN_POINT('Ctrl Pts',(-23.2986109014059,12.4419882074806,
129.949450466439)) ;
#139416=CARTESIAN_POINT('Ctrl Pts',(-23.2072849319717,12.5427027853094,
129.715701129722)) ;
#139417=CARTESIAN_POINT('Ctrl Pts',(-23.1272047239973,12.7067963999461,
129.514929286389)) ;
#139418=CARTESIAN_POINT('Ctrl Pts',(-23.0638014943553,12.9221001567719,
129.362835947955)) ;
#139419=CARTESIAN_POINT('Ctrl Pts',(-23.0207283179547,13.1741319901515,
129.270237886939)) ;
#139420=CARTESIAN_POINT('Ctrl Pts',(-23.0005908899832,13.44270233198,129.244466406606)) ;
#139421=CARTESIAN_POINT('Ctrl Pts',(-23.0038914292178,13.7107857110311,
129.287286348237)) ;
#139422=CARTESIAN_POINT('Ctrl Pts',(-23.0295704967675,13.9568883161136,
129.395289261901)) ;
#139423=CARTESIAN_POINT('Ctrl Pts',(-23.0752731994709,14.1661036759461,
129.561958208576)) ;
#139424=CARTESIAN_POINT('Ctrl Pts',(-23.1370402944096,14.3219385035442,
129.77557262833)) ;
#139425=CARTESIAN_POINT('Ctrl Pts',(-23.2093871602734,14.4130180760167,
130.019993869871)) ;
#139426=CARTESIAN_POINT('Ctrl Pts',(-23.2867565065069,14.4335349357277,
130.279148804425)) ;
#139427=CARTESIAN_POINT('Ctrl Pts',(-23.3629698219185,14.3810414404785,
130.535040474928)) ;
#139428=CARTESIAN_POINT('Ctrl Pts',(-23.4310082584103,14.2609491196068,
130.766748403059)) ;
#139429=CARTESIAN_POINT('Ctrl Pts',(-23.4864209908859,14.0795344573349,
130.961883840188)) ;
#139430=CARTESIAN_POINT('Ctrl Pts',(-23.5236051645126,13.8529284696564,
131.103464693403)) ;
#139431=CARTESIAN_POINT('Ctrl Pts',(-23.5397921027113,13.5926908131845,
131.184105008777)) ;
#139432=CARTESIAN_POINT('Ctrl Pts',(-23.5326550813306,13.3230678960584,
131.196241501053)) ;
#139433=CARTESIAN_POINT('Ctrl Pts',(-23.5022844153317,13.0595445585026,
131.140642603212)) ;
#139434=CARTESIAN_POINT('Ctrl Pts',(-23.4497773248406,12.8214089952354,
131.020469155132)) ;
#139435=CARTESIAN_POINT('Ctrl Pts',(-23.3784016727207,12.6270968112276,
130.845114797372)) ;
#139436=CARTESIAN_POINT('Ctrl Pts',(-23.293155678087,12.4904302156697,130.629020094481)) ;
#139437=CARTESIAN_POINT('Ctrl Pts',(-23.1981211422612,12.4195264236209,
130.384598565288)) ;
#139438=CARTESIAN_POINT('Ctrl Pts',(-23.1004341639123,12.4206997898043,
130.132284603727)) ;
#139439=CARTESIAN_POINT('Ctrl Pts',(-23.0054798051943,12.4940151271389,
129.888140448463)) ;
#139440=CARTESIAN_POINT('Ctrl Pts',(-22.9204783126155,12.6331734144625,
129.672828862818)) ;
#139441=CARTESIAN_POINT('Ctrl Pts',(-22.8497361514307,12.829325604419,129.499320879608)) ;
#139442=CARTESIAN_POINT('Ctrl Pts',(-22.798050247268,13.0683012054675,129.381494346922)) ;
#139443=CARTESIAN_POINT('Ctrl Pts',(-22.7684338481907,13.332296684324,129.328087201503)) ;
#139444=CARTESIAN_POINT('Ctrl Pts',(-22.7621646024436,13.6026349235875,
129.342864411698)) ;
#139445=CARTESIAN_POINT('Ctrl Pts',(-22.7789878211364,13.8605088298962,
129.425147516842)) ;
#139446=CARTESIAN_POINT('Ctrl Pts',(-22.8170651937567,14.0871784145907,
129.569548535915)) ;
#139447=CARTESIAN_POINT('Ctrl Pts',(-22.8727752484208,14.2658344085649,
129.765391197157)) ;
#139448=CARTESIAN_POINT('Ctrl Pts',(-22.9415251904135,14.3843789538156,
129.999358621862)) ;
#139449=CARTESIAN_POINT('Ctrl Pts',(-23.0177762015768,14.4339734253515,
130.255296131666)) ;
#139450=CARTESIAN_POINT('Ctrl Pts',(-23.0948641012711,14.4110559285979,
130.513542055004)) ;
#139451=CARTESIAN_POINT('Ctrl Pts',(-23.1669334987967,14.3178925023023,
130.757135194731)) ;
#139452=CARTESIAN_POINT('Ctrl Pts',(-23.228418635195,14.159368658012,130.970043928164)) ;
#139453=CARTESIAN_POINT('Ctrl Pts',(-23.2732913315262,13.9496805303502,
131.134118565758)) ;
#139454=CARTESIAN_POINT('Ctrl Pts',(-23.2984065123964,13.7013469975745,
131.240648353173)) ;
#139455=CARTESIAN_POINT('Ctrl Pts',(-23.3008248756517,13.433016471187,131.280867680268)) ;
#139456=CARTESIAN_POINT('Ctrl Pts',(-23.2798782812281,13.1647607687427,
131.252731738856)) ;
#139457=CARTESIAN_POINT('Ctrl Pts',(-23.2359949776677,12.9137311981176,
131.157770408831)) ;
#139458=CARTESIAN_POINT('Ctrl Pts',(-23.1722216632218,12.7007529774686,
131.004465052763)) ;
#139459=CARTESIAN_POINT('Ctrl Pts',(-23.0916116499635,12.5383275935417,
130.802181669735)) ;
#139460=CARTESIAN_POINT('Ctrl Pts',(-23.0000201461418,12.4398166133593,
130.567648814099)) ;
#139461=CARTESIAN_POINT('Ctrl Pts',(-22.9021029447549,12.4114725012227,
130.314910430739)) ;
#139462=CARTESIAN_POINT('Ctrl Pts',(-22.8056557366078,12.4557968893907,
130.066198456197)) ;
#139463=CARTESIAN_POINT('Ctrl Pts',(-22.7157297205741,12.5696290859636,
129.836683815397)) ;
#139464=CARTESIAN_POINT('Ctrl Pts',(-22.638835956155,12.7436129416571,129.645045220832)) ;
#139465=CARTESIAN_POINT('Ctrl Pts',(-22.5787413628733,12.9681022420836,
129.502789849415)) ;
#139466=CARTESIAN_POINT('Ctrl Pts',(-22.5400609169273,13.2239471204996,
129.422880231678)) ;
#139467=CARTESIAN_POINT('Ctrl Pts',(-22.5243053598294,13.4941632666535,
129.40996844027)) ;
#139468=CARTESIAN_POINT('Ctrl Pts',(-22.5319445480063,13.7589186275191,
129.465347966808)) ;
#139469=CARTESIAN_POINT('Ctrl Pts',(-22.561653260686,13.9998348960523,129.585215768084)) ;
#139470=CARTESIAN_POINT('Ctrl Pts',(-22.6106809695864,14.1997646334102,
129.761559980421)) ;
#139471=CARTESIAN_POINT('Ctrl Pts',(-22.6748483134623,14.3442637107108,
129.982171105828)) ;
#139472=CARTESIAN_POINT('Ctrl Pts',(-22.7488620893119,14.4224928337565,
130.231582338807)) ;
#139473=CARTESIAN_POINT('Ctrl Pts',(-22.826082224651,14.4291711137562,130.490143364531)) ;
#139474=CARTESIAN_POINT('Ctrl Pts',(-22.901385737979,14.3636108814792,130.743388063258)) ;
#139475=CARTESIAN_POINT('Ctrl Pts',(-22.9676523282968,14.2305641375214,
130.970092092409)) ;
#139476=CARTESIAN_POINT('Ctrl Pts',(-23.0196303198745,14.0406275620916,
131.154938240201)) ;
#139477=CARTESIAN_POINT('Ctrl Pts',(-23.0532662084991,13.8058699764793,
131.286324556169)) ;
#139478=CARTESIAN_POINT('Ctrl Pts',(-23.0651158799014,13.5427808202944,
131.354170447612)) ;
#139479=CARTESIAN_POINT('Ctrl Pts',(-23.0535903902688,13.2720605312769,
131.353608556185)) ;
#139480=CARTESIAN_POINT('Ctrl Pts',(-23.0188074569815,13.0118429090763,
131.285152168977)) ;
#139481=CARTESIAN_POINT('Ctrl Pts',(-22.9627783979762,12.7818788170933,
131.154510248436)) ;
#139482=CARTESIAN_POINT('Ctrl Pts',(-22.8883678106929,12.5968716626886,
130.97030840387)) ;
#139483=CARTESIAN_POINT('Ctrl Pts',(-22.8002450416258,12.4712517214802,
130.74607696204)) ;
#139484=CARTESIAN_POINT('Ctrl Pts',(-22.7044504660725,12.4142247969978,
130.499321626759)) ;
#139485=CARTESIAN_POINT('Ctrl Pts',(-22.6069179691138,12.4291610418386,
130.247458381608)) ;
#139486=CARTESIAN_POINT('Ctrl Pts',(-22.513489094124,12.5152749541959,130.007682466883)) ;
#139487=CARTESIAN_POINT('Ctrl Pts',(-22.4303075741883,12.6672522382755,
129.797931174508)) ;
#139488=CARTESIAN_POINT('Ctrl Pts',(-22.3633981184116,12.8714563581182,
129.63539167814)) ;
#139489=CARTESIAN_POINT('Ctrl Pts',(-22.315632303497,13.1164156516164,129.529009838952)) ;
#139490=CARTESIAN_POINT('Ctrl Pts',(-22.2903146188003,13.3833143712004,
129.48818130268)) ;
#139491=CARTESIAN_POINT('Ctrl Pts',(-22.2885211433467,13.6536761659143,
129.516158189572)) ;
#139492=CARTESIAN_POINT('Ctrl Pts',(-22.309526188747,13.9063303611245,129.610570446142)) ;
#139493=CARTESIAN_POINT('Ctrl Pts',(-22.3514235054152,14.1256565202968,
129.766227676016)) ;
#139494=CARTESIAN_POINT('Ctrl Pts',(-22.4097256575423,14.2929703983871,
129.969486284481)) ;
#139495=CARTESIAN_POINT('Ctrl Pts',(-22.4805872320115,14.3994043107509,
130.20975186399)) ;
#139496=CARTESIAN_POINT('Ctrl Pts',(-22.5572422571753,14.4351253202345,
130.466735869076)) ;
#139497=CARTESIAN_POINT('Ctrl Pts',(-22.6339302437926,14.3988243968592,
130.723845624362)) ;
#139498=CARTESIAN_POINT('Ctrl Pts',(-22.7045413583506,14.2923293351463,
130.963281578582)) ;
#139499=CARTESIAN_POINT('Ctrl Pts',(-22.7629217549356,14.1241731231248,
131.166869003256)) ;
#139500=CARTESIAN_POINT('Ctrl Pts',(-22.8045864477495,13.9051614017352,
131.321752941675)) ;
#139501=CARTESIAN_POINT('Ctrl Pts',(-22.8255003662911,13.6518311474299,
131.415971687488)) ;
#139502=CARTESIAN_POINT('Ctrl Pts',(-22.8235852848836,13.3824708815404,
131.44346252415)) ;
#139503=CARTESIAN_POINT('Ctrl Pts',(-22.7981865474188,13.1154253424266,
131.402424540592)) ;
#139504=CARTESIAN_POINT('Ctrl Pts',(-22.7503632246924,12.870532663978,131.295871230707)) ;
#139505=CARTESIAN_POINT('Ctrl Pts',(-22.6829455920271,12.6655370974074,
131.132034154533)) ;
#139506=CARTESIAN_POINT('Ctrl Pts',(-22.5999279586424,12.5146112418993,
130.922645471943)) ;
#139507=CARTESIAN_POINT('Ctrl Pts',(-22.5064782959341,12.4289101941166,
130.682807596149)) ;
#139508=CARTESIAN_POINT('Ctrl Pts',(-22.4090728608906,12.414189670065,130.431264713762)) ;
#139509=CARTESIAN_POINT('Ctrl Pts',(-22.312528515273,12.4724108557129,130.182598671296)) ;
#139510=CARTESIAN_POINT('Ctrl Pts',(-22.225209279529,12.5978142142,129.960457180624)) ;
#139511=CARTESIAN_POINT('Ctrl Pts',(-22.1509137345901,12.7826551877608,
129.776554350212)) ;
#139512=CARTESIAN_POINT('Ctrl Pts',(-22.0948479657602,13.0133814811485,
129.645883919566)) ;
#139513=CARTESIAN_POINT('Ctrl Pts',(-22.0601691205954,13.2742168699271,
129.577789609753)) ;
#139514=CARTESIAN_POINT('Ctrl Pts',(-22.0488678992467,13.5450314863386,
129.577894446666)) ;
#139515=CARTESIAN_POINT('Ctrl Pts',(-22.0608042409464,13.8067211996107,
129.645832849942)) ;
#139516=CARTESIAN_POINT('Ctrl Pts',(-22.094434022848,14.041251301363,129.77717692661)) ;
#139517=CARTESIAN_POINT('Ctrl Pts',(-22.1467135744848,14.2318697191873,
129.963049851365)) ;
#139518=CARTESIAN_POINT('Ctrl Pts',(-22.2133209230258,14.3645253073145,
130.190851488341)) ;
#139519=CARTESIAN_POINT('Ctrl Pts',(-22.2880127253032,14.4291513748126,
130.442024637572)) ;
#139520=CARTESIAN_POINT('Ctrl Pts',(-22.3656045332651,14.4223448235858,
130.701832829083)) ;
#139521=CARTESIAN_POINT('Ctrl Pts',(-22.4395795352273,14.3433928337176,
130.951141721303)) ;
#139522=CARTESIAN_POINT('Ctrl Pts',(-22.5034115118926,14.1993297551337,
131.170623731226)) ;
#139523=CARTESIAN_POINT('Ctrl Pts',(-22.5524972774972,13.9988090626419,
131.347214932239)) ;
#139524=CARTESIAN_POINT('Ctrl Pts',(-22.5821223537297,13.7578101990109,
131.46682648151)) ;
#139525=CARTESIAN_POINT('Ctrl Pts',(-22.5896179033506,13.4916491318397,
131.521951897713)) ;
#139526=CARTESIAN_POINT('Ctrl Pts',(-22.5737359732877,13.2223243547225,
131.50855985098)) ;
#139527=CARTESIAN_POINT('Ctrl Pts',(-22.5347221915636,12.9657468918016,
131.42780367239)) ;
#139528=CARTESIAN_POINT('Ctrl Pts',(-22.4748529861467,12.7429296801426,
131.286000068107)) ;
#139529=CARTESIAN_POINT('Ctrl Pts',(-22.3976682749232,12.5685157240841,
131.093622742732)) ;
#139530=CARTESIAN_POINT('Ctrl Pts',(-22.3073711104087,12.4549912685616,
130.863119792323)) ;
#139531=CARTESIAN_POINT('Ctrl Pts',(-22.2111174959793,12.4115665135432,
130.61489744185)) ;
#139532=CARTESIAN_POINT('Ctrl Pts',(-22.1137558357218,12.4399153694957,
130.363592894185)) ;
#139533=CARTESIAN_POINT('Ctrl Pts',(-22.0216969019763,12.539266271838,130.12788037676)) ;
#139534=CARTESIAN_POINT('Ctrl Pts',(-21.9414381676257,12.7015765311082,
129.926512602715)) ;
#139535=CARTESIAN_POINT('Ctrl Pts',(-21.8776532898284,12.9151235328842,
129.773233982734)) ;
#139536=CARTESIAN_POINT('Ctrl Pts',(-21.8339664362384,13.1655123669942,
129.67874406302)) ;
#139537=CARTESIAN_POINT('Ctrl Pts',(-21.8130201904645,13.4357073087156,
129.650843568944)) ;
#139538=CARTESIAN_POINT('Ctrl Pts',(-21.8156809926834,13.7027427371582,
129.69162438137)) ;
#139539=CARTESIAN_POINT('Ctrl Pts',(-21.8407512524161,13.9504288241065,
129.79794042058)) ;
#139540=CARTESIAN_POINT('Ctrl Pts',(-21.8859845993865,14.1608970997243,
129.963242481406)) ;
#139541=CARTESIAN_POINT('Ctrl Pts',(-21.9472402348266,14.3182076621176,
130.175305086424)) ;
#139542=CARTESIAN_POINT('Ctrl Pts',(-22.0194714930934,14.4114239711584,
130.41944123239)) ;
#139543=CARTESIAN_POINT('Ctrl Pts',(-22.0966325897837,14.4338711426872,
130.677924220104)) ;
#139544=CARTESIAN_POINT('Ctrl Pts',(-22.1727955150631,14.3839736341,130.933575234531)) ;
#139545=CARTESIAN_POINT('Ctrl Pts',(-22.2415712312017,14.2649033849915,
131.167660198233)) ;
#139546=CARTESIAN_POINT('Ctrl Pts',(-22.2971026553746,14.0862373314476,
131.362925300438)) ;
#139547=CARTESIAN_POINT('Ctrl Pts',(-22.3350972412815,13.8593709680806,
131.507089720524)) ;
#139548=CARTESIAN_POINT('Ctrl Pts',(-22.3518156453636,13.6016402175067,
131.589035604686)) ;
#139549=CARTESIAN_POINT('Ctrl Pts',(-22.3454434205743,13.3309241263673,
131.603556996775)) ;
#139550=CARTESIAN_POINT('Ctrl Pts',(-22.3156922828301,13.0670233439019,
131.549755470883)) ;
#139551=CARTESIAN_POINT('Ctrl Pts',(-22.2640083916553,12.8286261810775,
131.431877786345)) ;
#139552=CARTESIAN_POINT('Ctrl Pts',(-22.1932065591499,12.6324569131355,
131.258208090831)) ;
#139553=CARTESIAN_POINT('Ctrl Pts',(-22.1077589751913,12.4932133607205,
131.041732099059)) ;
#139554=CARTESIAN_POINT('Ctrl Pts',(-22.0133476243497,12.4206918149119,
130.798970751027)) ;
#139555=CARTESIAN_POINT('Ctrl Pts',(-21.9153477521299,12.4196226732146,
130.545851858096)) ;
#139556=CARTESIAN_POINT('Ctrl Pts',(-21.8202845535771,12.4910154919702,
130.301366419668)) ;
#139557=CARTESIAN_POINT('Ctrl Pts',(-21.7349087576259,12.6283739750249,
130.084970327283)) ;
#139558=CARTESIAN_POINT('Ctrl Pts',(-21.6635187562755,12.8237069279728,
129.909657715924)) ;
#139559=CARTESIAN_POINT('Ctrl Pts',(-21.6113756355089,13.0616748954868,
129.790472154327)) ;
#139560=CARTESIAN_POINT('Ctrl Pts',(-21.5812201320458,13.3240382203917,
129.735346429805)) ;
#139561=CARTESIAN_POINT('Ctrl Pts',(-21.5742019181363,13.5952493651547,
129.748031247665)) ;
#139562=CARTESIAN_POINT('Ctrl Pts',(-21.5905171574251,13.8544594901405,
129.828928472972)) ;
#139563=CARTESIAN_POINT('Ctrl Pts',(-21.6280422230899,14.0816539575776,
129.971653631214)) ;
#139564=CARTESIAN_POINT('Ctrl Pts',(-21.6831210640629,14.2612879852104,
130.165544817405)) ;
#139565=CARTESIAN_POINT('Ctrl Pts',(-21.7515285398232,14.3817634357603,
130.39850167849)) ;
#139566=CARTESIAN_POINT('Ctrl Pts',(-21.8276692424797,14.4336477356996,
130.654125167946)) ;
#139567=CARTESIAN_POINT('Ctrl Pts',(-21.9052481328329,14.4124733910525,
130.913995427691)) ;
#139568=CARTESIAN_POINT('Ctrl Pts',(-21.9771206529507,14.3214777368465,
131.15683461577)) ;
#139569=CARTESIAN_POINT('Ctrl Pts',(-22.0389770924245,14.1652192493521,
131.370776987055)) ;
#139570=CARTESIAN_POINT('Ctrl Pts',(-22.0845865752622,13.9555650304119,
131.537191449783)) ;
#139571=CARTESIAN_POINT('Ctrl Pts',(-22.110142037256,13.7095599623908,131.644803567879)) ;
#139572=CARTESIAN_POINT('Ctrl Pts',(-22.1133412911239,13.4405995094296,
131.68742540987)) ;
#139573=CARTESIAN_POINT('Ctrl Pts',(-22.0928739407392,13.1715077447804,
131.660770291061)) ;
#139574=CARTESIAN_POINT('Ctrl Pts',(-22.0500042324198,12.9214880554527,
131.568517539565)) ;
#139575=CARTESIAN_POINT('Ctrl Pts',(-21.986272283684,12.7055052925361,131.415601528427)) ;
#139576=CARTESIAN_POINT('Ctrl Pts',(-21.9065002297074,12.5425196617187,
131.21556628128)) ;
#139577=CARTESIAN_POINT('Ctrl Pts',(-21.8149731081815,12.4416160239473,
130.981304047927)) ;
#139578=CARTESIAN_POINT('Ctrl Pts',(-21.717050858099,12.4112449647392,130.728571243266)) ;
#139579=CARTESIAN_POINT('Ctrl Pts',(-21.6204243758217,12.4537097217899,
130.479366405329)) ;
#139580=CARTESIAN_POINT('Ctrl Pts',(-21.5305167877764,12.5652232795711,
130.249790618881)) ;
#139581=CARTESIAN_POINT('Ctrl Pts',(-21.4530181437376,12.7379440224027,
130.056458295685)) ;
#139582=CARTESIAN_POINT('Ctrl Pts',(-21.3925676750595,12.960397453185,129.91304056417)) ;
#139583=CARTESIAN_POINT('Ctrl Pts',(-21.3531347639013,13.2156634821883,
129.830962045719)) ;
#139584=CARTESIAN_POINT('Ctrl Pts',(-21.336634573283,13.4857933764674,129.815880746042)) ;
#139585=CARTESIAN_POINT('Ctrl Pts',(-21.343632936242,13.7522946438347,129.869550437587)) ;
#139586=CARTESIAN_POINT('Ctrl Pts',(-21.372925446852,13.9943544460531,129.988260551423)) ;
#139587=CARTESIAN_POINT('Ctrl Pts',(-21.4212369628702,14.1947046175958,
130.162353989947)) ;
#139588=CARTESIAN_POINT('Ctrl Pts',(-21.4853334805668,14.3414529387325,
130.382901794377)) ;
#139589=CARTESIAN_POINT('Ctrl Pts',(-21.5587948401416,14.4211243068953,
130.630528130011)) ;
#139590=CARTESIAN_POINT('Ctrl Pts',(-21.6361524176439,14.4300014348132,
130.889562555299)) ;
#139591=CARTESIAN_POINT('Ctrl Pts',(-21.7114727530929,14.3664765738552,
131.142795185518)) ;
#139592=CARTESIAN_POINT('Ctrl Pts',(-21.778029101135,14.235605243378,131.370308686837)) ;
#139593=CARTESIAN_POINT('Ctrl Pts',(-21.8307071352233,14.0463420855303,
131.5573397721)) ;
#139594=CARTESIAN_POINT('Ctrl Pts',(-21.8647984605866,13.8127312117544,
131.690021475908)) ;
#139595=CARTESIAN_POINT('Ctrl Pts',(-21.8773121091469,13.5514861581268,
131.759647215842)) ;
#139596=CARTESIAN_POINT('Ctrl Pts',(-21.8664659862452,13.2797431877816,
131.761195196609)) ;
#139597=CARTESIAN_POINT('Ctrl Pts',(-21.8324447030282,13.0196141695931,
131.694872542692)) ;
#139598=CARTESIAN_POINT('Ctrl Pts',(-21.7768285980867,12.7876902143184,
131.565555325081)) ;
#139599=CARTESIAN_POINT('Ctrl Pts',(-21.7029455016982,12.6015317639528,
131.382848114673)) ;
#139600=CARTESIAN_POINT('Ctrl Pts',(-21.6154214666389,12.4742597537388,
131.160271970459)) ;
#139601=CARTESIAN_POINT('Ctrl Pts',(-21.5196623512914,12.4148459760243,
130.913664546399)) ;
#139602=CARTESIAN_POINT('Ctrl Pts',(-21.4218298173218,12.4277168050886,
130.661011819284)) ;
#139603=CARTESIAN_POINT('Ctrl Pts',(-21.3282883705838,12.5119511552026,
130.420881834853)) ;
#139604=CARTESIAN_POINT('Ctrl Pts',(-21.2450319287907,12.6612550924709,
130.210764914545)) ;
#139605=CARTESIAN_POINT('Ctrl Pts',(-21.1771167844571,12.8654797795072,
130.045522770625)) ;
#139606=CARTESIAN_POINT('Ctrl Pts',(-21.1289599445452,13.1088715817203,
129.937890486847)) ;
#139607=CARTESIAN_POINT('Ctrl Pts',(-21.1029409415662,13.3752798847283,
129.89500636968)) ;
#139608=CARTESIAN_POINT('Ctrl Pts',(-21.100441405058,13.6458119983222,129.920912628984)) ;
#139609=CARTESIAN_POINT('Ctrl Pts',(-21.1208585860571,13.899465813918,130.013650363731)) ;
#139610=CARTESIAN_POINT('Ctrl Pts',(-21.1619780714701,14.1192748992269,
130.166896304245)) ;
#139611=CARTESIAN_POINT('Ctrl Pts',(-21.2201580360466,14.2891803091472,
130.369981381548)) ;
#139612=CARTESIAN_POINT('Ctrl Pts',(-21.2904289832578,14.3970324953894,
130.60836272282)) ;
#139613=CARTESIAN_POINT('Ctrl Pts',(-21.3671416455221,14.4351164741298,
130.865591429488)) ;
#139614=CARTESIAN_POINT('Ctrl Pts',(-21.4438538638505,14.4010787684845,
131.122734088588)) ;
#139615=CARTESIAN_POINT('Ctrl Pts',(-21.5151288839755,14.2958209248288,
131.364304880692)) ;
#139616=CARTESIAN_POINT('Ctrl Pts',(-21.5736633584408,14.129652176779,131.568224656794)) ;
#139617=CARTESIAN_POINT('Ctrl Pts',(-21.6158674833682,13.912176140122,131.72465380531)) ;
#139618=CARTESIAN_POINT('Ctrl Pts',(-21.6374100082649,13.6594303550192,
131.820730010105)) ;
#139619=CARTESIAN_POINT('Ctrl Pts',(-21.6362376323324,13.3906473187371,
131.850341742612)) ;
#139620=CARTESIAN_POINT('Ctrl Pts',(-21.6112596121911,13.1215485791247,
131.810753715866)) ;
#139621=CARTESIAN_POINT('Ctrl Pts',(-21.5643253393536,12.877499502744,131.706566930706)) ;
#139622=CARTESIAN_POINT('Ctrl Pts',(-21.4971489276021,12.6702279580221,
131.543581214665)) ;
#139623=CARTESIAN_POINT('Ctrl Pts',(-21.4148278562299,12.5183910541011,
131.336084599909)) ;
#139624=CARTESIAN_POINT('Ctrl Pts',(-21.321592793567,12.4302683160369,131.096887067683)) ;
#139625=CARTESIAN_POINT('Ctrl Pts',(-21.2235235030194,12.4138255854832,
130.84364383687)) ;
#139626=CARTESIAN_POINT('Ctrl Pts',(-21.1280462202582,12.4692849661908,
130.59767471953)) ;
#139627=CARTESIAN_POINT('Ctrl Pts',(-21.0397782209746,12.5930868189149,
130.372972296455)) ;
#139628=CARTESIAN_POINT('Ctrl Pts',(-20.9648900702745,12.7771359268665,
130.187423563488)) ;
#139629=CARTESIAN_POINT('Ctrl Pts',(-20.9084604382932,13.0059649491312,
130.055574675109)) ;
#139630=CARTESIAN_POINT('Ctrl Pts',(-20.8730855953741,13.2661471501604,
129.98544681023)) ;
#139631=CARTESIAN_POINT('Ctrl Pts',(-20.8610654562158,13.536990610461,129.983456526969)) ;
#139632=CARTESIAN_POINT('Ctrl Pts',(-20.8723871827311,13.7997448803438,
130.049673265163)) ;
#139633=CARTESIAN_POINT('Ctrl Pts',(-20.90538067581,14.0350783455638,130.179115882773)) ;
#139634=CARTESIAN_POINT('Ctrl Pts',(-20.9574456253222,14.2276700912271,
130.364492989564)) ;
#139635=CARTESIAN_POINT('Ctrl Pts',(-21.0230849241156,14.3610390987627,
130.589154695541)) ;
#139636=CARTESIAN_POINT('Ctrl Pts',(-21.0982174668606,14.4285213562849,
130.841897239005)) ;
#139637=CARTESIAN_POINT('Ctrl Pts',(-21.1756599652311,14.4233691506753,
131.10119816308)) ;
#139638=CARTESIAN_POINT('Ctrl Pts',(-21.2496325844285,14.3469900608794,
131.35039585002)) ;
#139639=CARTESIAN_POINT('Ctrl Pts',(-21.3142670386072,14.2034039826352,
131.572477885729)) ;
#139640=CARTESIAN_POINT('Ctrl Pts',(-21.3634585175808,14.0056848042437,
131.749124315029)) ;
#139641=CARTESIAN_POINT('Ctrl Pts',(-21.3938254756421,13.7644935379873,
131.87107326449)) ;
#139642=CARTESIAN_POINT('Ctrl Pts',(-21.4019773023267,13.5002463759362,
131.927919962956)) ;
#139643=CARTESIAN_POINT('Ctrl Pts',(-21.3865652696606,13.2284058241885,
131.916205863608)) ;
#139644=CARTESIAN_POINT('Ctrl Pts',(-21.3485619428079,12.9739037522761,
131.838041629857)) ;
#139645=CARTESIAN_POINT('Ctrl Pts',(-21.2890019447558,12.7484704180283,
131.697336737727)) ;
#139646=CARTESIAN_POINT('Ctrl Pts',(-21.212476706466,12.5731123279677,131.506773572971)) ;
#139647=CARTESIAN_POINT('Ctrl Pts',(-21.1224208921965,12.45735908031,131.277009163557)) ;
#139648=CARTESIAN_POINT('Ctrl Pts',(-21.0261799251125,12.4118025440313,
131.028854605153)) ;
#139649=CARTESIAN_POINT('Ctrl Pts',(-20.9287286020676,12.4381298273325,
130.777298657297)) ;
#139650=CARTESIAN_POINT('Ctrl Pts',(-20.8365847097189,12.5352056627263,
130.541271205423)) ;
#139651=CARTESIAN_POINT('Ctrl Pts',(-20.7556872818817,12.696300610242,130.338138236175)) ;
#139652=CARTESIAN_POINT('Ctrl Pts',(-20.6914131973187,12.9082756113126,
130.183386414941)) ;
#139653=CARTESIAN_POINT('Ctrl Pts',(-20.6469587597595,13.1596325323724,
130.086874818099)) ;
#139654=CARTESIAN_POINT('Ctrl Pts',(-20.6256126189791,13.4259468835544,
130.057354385986)) ;
#139655=CARTESIAN_POINT('Ctrl Pts',(-20.6274509190732,13.6953761011822,
130.095991058217)) ;
#139656=CARTESIAN_POINT('Ctrl Pts',(-20.6519544165665,13.9437170252716,
130.20062924795)) ;
#139657=CARTESIAN_POINT('Ctrl Pts',(-20.6967040257505,14.155711083142,130.364556823473)) ;
#139658=CARTESIAN_POINT('Ctrl Pts',(-20.7574637860279,14.3144000216169,
130.575108733115)) ;
#139659=CARTESIAN_POINT('Ctrl Pts',(-20.8294247939273,14.4096307873655,
130.818448393621)) ;
#139660=CARTESIAN_POINT('Ctrl Pts',(-20.9065511570391,14.4343455413494,
131.076836805641)) ;
#139661=CARTESIAN_POINT('Ctrl Pts',(-20.9831483409494,14.3860725328483,
131.333902273055)) ;
#139662=CARTESIAN_POINT('Ctrl Pts',(-21.0518273806318,14.2695097224109,
131.567514159987)) ;
#139663=CARTESIAN_POINT('Ctrl Pts',(-21.1080343518942,14.0917907818256,
131.764885399557)) ;
#139664=CARTESIAN_POINT('Ctrl Pts',(-21.1464563378518,13.8666927390169,
131.910195855888)) ;
#139665=CARTESIAN_POINT('Ctrl Pts',(-21.1638741215799,13.6093228948058,
131.994229909567)) ;
#139666=CARTESIAN_POINT('Ctrl Pts',(-21.1581778671763,13.3388432041032,
132.010707129866)) ;
#139667=CARTESIAN_POINT('Ctrl Pts',(-21.1290589624462,13.0740474373603,
131.958804416506)) ;
#139668=CARTESIAN_POINT('Ctrl Pts',(-21.0778095064892,12.8343946472962,
131.842251800914)) ;
#139669=CARTESIAN_POINT('Ctrl Pts',(-21.0078504214422,12.6378259475901,
131.670874797454)) ;
#139670=CARTESIAN_POINT('Ctrl Pts',(-20.9227635942453,12.4964630119009,
131.455470160856)) ;
#139671=CARTESIAN_POINT('Ctrl Pts',(-20.8282781982489,12.421725405798,131.212580208633)) ;
#139672=CARTESIAN_POINT('Ctrl Pts',(-20.7303861760134,12.4187226198539,
130.959743948979)) ;
#139673=CARTESIAN_POINT('Ctrl Pts',(-20.635461865384,12.4875916518615,130.715545608703)) ;
#139674=CARTESIAN_POINT('Ctrl Pts',(-20.5493919591687,12.6235712310503,
130.49725175219)) ;
#139675=CARTESIAN_POINT('Ctrl Pts',(-20.4777829693133,12.8167007524725,
130.321173584195)) ;
#139676=CARTESIAN_POINT('Ctrl Pts',(-20.424910899171,13.053470084932,130.199863474853)) ;
#139677=CARTESIAN_POINT('Ctrl Pts',(-20.3939411324719,13.3166529719994,
130.14252162574)) ;
#139678=CARTESIAN_POINT('Ctrl Pts',(-20.3863238911027,13.5871781568045,
130.153366237627)) ;
#139679=CARTESIAN_POINT('Ctrl Pts',(-20.4018167783541,13.8461110281262,
130.231734054356)) ;
#139680=CARTESIAN_POINT('Ctrl Pts',(-20.4388065892668,14.0754123142472,
130.373009889351)) ;
#139681=CARTESIAN_POINT('Ctrl Pts',(-20.49356997314,14.2569965366052,130.566053917608)) ;
#139682=CARTESIAN_POINT('Ctrl Pts',(-20.5616742400838,14.3792169308405,
130.798118874428)) ;
#139683=CARTESIAN_POINT('Ctrl Pts',(-20.6374555012612,14.4330645765252,
131.052596497103)) ;
#139684=CARTESIAN_POINT('Ctrl Pts',(-20.7150727128244,14.4142942137405,
131.312571329954)) ;
#139685=CARTESIAN_POINT('Ctrl Pts',(-20.7874772612268,14.3249818640555,
131.557095540597)) ;
#139686=CARTESIAN_POINT('Ctrl Pts',(-20.8497107932074,14.1700409450456,
131.772170241937)) ;
#139687=CARTESIAN_POINT('Ctrl Pts',(-20.8956340065545,13.9629928904563,
131.939314582627)) ;
#139688=CARTESIAN_POINT('Ctrl Pts',(-20.9219601566609,13.716497244272,132.049365900883)) ;
#139689=CARTESIAN_POINT('Ctrl Pts',(-20.9257864629784,13.449382384683,132.093627582631)) ;
#139690=CARTESIAN_POINT('Ctrl Pts',(-20.9061009955916,13.179466012535,132.069323528848)) ;
#139691=CARTESIAN_POINT('Ctrl Pts',(-20.8635521867842,12.9274139548691,
131.978183997817)) ;
#139692=CARTESIAN_POINT('Ctrl Pts',(-20.8006998299117,12.7115777199899,
131.827639105462)) ;
#139693=CARTESIAN_POINT('Ctrl Pts',(-20.7213500350591,12.5463884339408,
131.628868055719)) ;
#139694=CARTESIAN_POINT('Ctrl Pts',(-20.6292985456697,12.4431786927595,
131.393338070779)) ;
#139695=CARTESIAN_POINT('Ctrl Pts',(-20.5325248471645,12.4112124576001,
131.14359108722)) ;
#139696=CARTESIAN_POINT('Ctrl Pts',(-20.4354101414637,12.4513454606681,
130.893090654114)) ;
#139697=CARTESIAN_POINT('Ctrl Pts',(-20.3452469652715,12.5610016888449,
130.662758587929)) ;
#139698=CARTESIAN_POINT('Ctrl Pts',(-20.2672178306558,12.7322315301459,
130.467913756268)) ;
#139699=CARTESIAN_POINT('Ctrl Pts',(-20.2062037864739,12.9536821902703,
130.322869683321)) ;
#139700=CARTESIAN_POINT('Ctrl Pts',(-20.1662123639624,13.2077095547012,
130.239091898145)) ;
#139701=CARTESIAN_POINT('Ctrl Pts',(-20.1489841763445,13.4778389937593,
130.221903369639)) ;
#139702=CARTESIAN_POINT('Ctrl Pts',(-20.1553409554788,13.7447250212435,
130.273702425957)) ;
#139703=CARTESIAN_POINT('Ctrl Pts',(-20.1838475971167,13.9871379324524,
130.390012023778)) ;
#139704=CARTESIAN_POINT('Ctrl Pts',(-20.2319890113485,14.1900736683291,
130.563825342734)) ;
#139705=CARTESIAN_POINT('Ctrl Pts',(-20.2951088659413,14.3373317705726,
130.781206869708)) ;
#139706=CARTESIAN_POINT('Ctrl Pts',(-20.3688107602542,14.4199335314477,
131.029762137696)) ;
#139707=CARTESIAN_POINT('Ctrl Pts',(-20.446131773642,14.4307823932299,131.288673826951)) ;
#139708=CARTESIAN_POINT('Ctrl Pts',(-20.5217929524515,14.3690285346023,
131.542993054621)) ;
#139709=CARTESIAN_POINT('Ctrl Pts',(-20.5883871265995,14.2404409958973,
131.770478575448)) ;
#139710=CARTESIAN_POINT('Ctrl Pts',(-20.6415813159015,14.0528076235366,
131.959023744489)) ;
#139711=CARTESIAN_POINT('Ctrl Pts',(-20.6763112872876,13.8202655346865,
132.093577798832)) ;
#139712=CARTESIAN_POINT('Ctrl Pts',(-20.6895096092303,13.5584444943241,
132.165343569218)) ;
#139713=CARTESIAN_POINT('Ctrl Pts',(-20.6792615552115,13.2871050604655,
132.168588192677)) ;
#139714=CARTESIAN_POINT('Ctrl Pts',(-20.6460046902205,13.0271136592546,
132.104408593774)) ;
#139715=CARTESIAN_POINT('Ctrl Pts',(-20.590935829574,12.7938647968009,131.976722550481)) ;
#139716=CARTESIAN_POINT('Ctrl Pts',(-20.517620628279,12.6063348260336,131.795635103324)) ;
#139717=CARTESIAN_POINT('Ctrl Pts',(-20.4302806626542,12.4770287945195,
131.573651748548)) ;
#139718=CARTESIAN_POINT('Ctrl Pts',(-20.3349577898321,12.4155889171301,
131.328220018841)) ;
#139719=CARTESIAN_POINT('Ctrl Pts',(-20.2366487863863,12.4264045775595,
131.074330742108)) ;
#139720=CARTESIAN_POINT('Ctrl Pts',(-20.1432359738446,12.5084012682064,
130.834454218698)) ;
#139721=CARTESIAN_POINT('Ctrl Pts',(-20.0594324062122,12.6562045678091,
130.622810534766)) ;
#139722=CARTESIAN_POINT('Ctrl Pts',(-19.9912068299662,12.8582528163381,
130.456544034109)) ;
#139723=CARTESIAN_POINT('Ctrl Pts',(-19.9420895004565,13.1022480435351,
130.346320064404)) ;
#139724=CARTESIAN_POINT('Ctrl Pts',(-19.9155609247342,13.3685511401161,
130.301969143821)) ;
#139725=CARTESIAN_POINT('Ctrl Pts',(-19.9123931900497,13.6374690489365,
130.325704502981)) ;
#139726=CARTESIAN_POINT('Ctrl Pts',(-19.9321748917974,13.8926337439443,
130.416683309371)) ;
#139727=CARTESIAN_POINT('Ctrl Pts',(-19.9727272333172,14.1134973909665,
130.568248020198)) ;
#139728=CARTESIAN_POINT('Ctrl Pts',(-20.030633868195,14.2854804526752,130.770621797177)) ;
#139729=CARTESIAN_POINT('Ctrl Pts',(-20.1006583949635,14.3949169679371,
131.008278415634)) ;
#139730=CARTESIAN_POINT('Ctrl Pts',(-20.1769463478651,14.4350950474159,
131.26412354158)) ;
#139731=CARTESIAN_POINT('Ctrl Pts',(-20.2541792081547,14.4027523558799,
131.522987865141)) ;
#139732=CARTESIAN_POINT('Ctrl Pts',(-20.3251151923492,14.3004224284984,
131.763273616136)) ;
#139733=CARTESIAN_POINT('Ctrl Pts',(-20.3846198909271,14.1345848186711,
131.970325949278)) ;
#139734=CARTESIAN_POINT('Ctrl Pts',(-20.4271315499746,13.9188292649382,
132.127540458863)) ;
#139735=CARTESIAN_POINT('Ctrl Pts',(-20.4493383192168,13.6668968263447,
132.225559348984)) ;
#139736=CARTESIAN_POINT('Ctrl Pts',(-20.4487750722731,13.3982258139503,
132.256962612225)) ;
#139737=CARTESIAN_POINT('Ctrl Pts',(-20.424644928654,13.1299459979309,132.219701611108)) ;
#139738=CARTESIAN_POINT('Ctrl Pts',(-20.3781183421514,12.8837060255956,
132.116878294644)) ;
#139739=CARTESIAN_POINT('Ctrl Pts',(-20.3115284961441,12.6755091265604,
131.955551424455)) ;
#139740=CARTESIAN_POINT('Ctrl Pts',(-20.2294351760645,12.5215778534682,
131.748786107997)) ;
#139741=CARTESIAN_POINT('Ctrl Pts',(-20.1362346606042,12.4317802187368,
131.509743104052)) ;
#139742=CARTESIAN_POINT('Ctrl Pts',(-20.0390583090231,12.4131805115513,
131.258818109629)) ;
#139743=CARTESIAN_POINT('Ctrl Pts',(-19.9426649164388,12.4668842631246,
131.010444047681)) ;
#139744=CARTESIAN_POINT('Ctrl Pts',(-19.8545070298818,12.5884450381112,
130.785909700319)) ;
#139745=CARTESIAN_POINT('Ctrl Pts',(-19.7789377814184,12.7713420936062,
130.598465428946)) ;
#139746=CARTESIAN_POINT('Ctrl Pts',(-19.7220015443685,12.9988617969997,
130.465098611114)) ;
#139747=CARTESIAN_POINT('Ctrl Pts',(-19.6858986492706,13.2594913097142,
130.392975341362)) ;
#139748=CARTESIAN_POINT('Ctrl Pts',(-19.6733337480537,13.5289133142041,
130.38922412671)) ;
#139749=CARTESIAN_POINT('Ctrl Pts',(-19.6839091842483,13.7920447587741,
130.453239453652)) ;
#139750=CARTESIAN_POINT('Ctrl Pts',(-19.7163423526536,14.028682332542,130.581083514188)) ;
#139751=CARTESIAN_POINT('Ctrl Pts',(-19.7678307217928,14.2226477073875,
130.764735550547)) ;
#139752=CARTESIAN_POINT('Ctrl Pts',(-19.8333291765721,14.358128004445,130.989083666605)) ;
#139753=CARTESIAN_POINT('Ctrl Pts',(-19.9079226684156,14.427517223623,131.240089115873)) ;
#139754=CARTESIAN_POINT('Ctrl Pts',(-19.9859801243066,14.4244373383238,
131.501449139126)) ;
#139755=CARTESIAN_POINT('Ctrl Pts',(-20.0597164291861,14.3501368241958,
131.749777152345)) ;
#139756=CARTESIAN_POINT('Ctrl Pts',(-20.1246192093162,14.2089998029508,
131.972568872511)) ;
#139757=CARTESIAN_POINT('Ctrl Pts',(-20.1745043948321,14.0121251226583,
132.151352883394)) ;
#139758=CARTESIAN_POINT('Ctrl Pts',(-20.205479708551,13.7718247542597,132.275085721787)) ;
#139759=CARTESIAN_POINT('Ctrl Pts',(-20.2142480552375,13.5078187050463,
132.333759678721)) ;
#139760=CARTESIAN_POINT('Ctrl Pts',(-20.1996711320823,13.2372789861246,
132.324307123579)) ;
#139761=CARTESIAN_POINT('Ctrl Pts',(-20.1621297481922,12.9804327366812,
132.247703472472)) ;
#139762=CARTESIAN_POINT('Ctrl Pts',(-20.103068138609,12.7540238900059,132.108444548132)) ;
#139763=CARTESIAN_POINT('Ctrl Pts',(-20.0271058684499,12.577462748724,131.919470641086)) ;
#139764=CARTESIAN_POINT('Ctrl Pts',(-19.9375506636755,12.4598742961996,
131.691099669398)) ;
#139765=CARTESIAN_POINT('Ctrl Pts',(-19.8409928350901,12.4120040777539,
131.442168402122)) ;
#139766=CARTESIAN_POINT('Ctrl Pts',(-19.7435371148839,12.4365719304023,
131.190583062223)) ;
#139767=CARTESIAN_POINT('Ctrl Pts',(-19.6515284558936,12.5311793642618,
130.954812449025)) ;
#139768=CARTESIAN_POINT('Ctrl Pts',(-19.5699202919936,12.6910252925006,
130.749716829182)) ;
#139769=CARTESIAN_POINT('Ctrl Pts',(-19.5052958004438,12.901554601713,130.593894377772)) ;
#139770=CARTESIAN_POINT('Ctrl Pts',(-19.4603082437547,13.1503193803292,
130.495615012924)) ;
#139771=CARTESIAN_POINT('Ctrl Pts',(-19.4380452691141,13.4198238179189,
130.463850336133)) ;
#139772=CARTESIAN_POINT('Ctrl Pts',(-19.4392649628103,13.6867201864748,
130.500325755553)) ;
#139773=CARTESIAN_POINT('Ctrl Pts',(-19.4632228569756,13.9376559874792,
130.603602335536)) ;
#139774=CARTESIAN_POINT('Ctrl Pts',(-19.5073954403515,14.1502428596578,
130.765749845655)) ;
#139775=CARTESIAN_POINT('Ctrl Pts',(-19.5678164429334,14.3108380657866,
130.975357095169)) ;
#139776=CARTESIAN_POINT('Ctrl Pts',(-19.63952920761,14.4079445311136,131.217958014036)) ;
#139777=CARTESIAN_POINT('Ctrl Pts',(-19.7166714113582,14.4345276707165,
131.476430714807)) ;
#139778=CARTESIAN_POINT('Ctrl Pts',(-19.7928752190649,14.3888298809399,
131.732116617467)) ;
#139779=CARTESIAN_POINT('Ctrl Pts',(-19.862229218925,14.2738284878411,131.967870918754)) ;
#139780=CARTESIAN_POINT('Ctrl Pts',(-19.9188081884538,14.0978368640531,
132.166288619942)) ;
#139781=CARTESIAN_POINT('Ctrl Pts',(-19.9578752207231,13.8735407720446,
132.31354477898)) ;
#139782=CARTESIAN_POINT('Ctrl Pts',(-19.9759059243398,13.616875079998,132.399358256203)) ;
#139783=CARTESIAN_POINT('Ctrl Pts',(-19.9708726882155,13.3465064329097,
132.41777444154)) ;
#139784=CARTESIAN_POINT('Ctrl Pts',(-19.9424497125854,13.0815408414728,
132.367868399297)) ;
#139785=CARTESIAN_POINT('Ctrl Pts',(-19.8918146463953,12.8409647311381,
132.253107292745)) ;
#139786=CARTESIAN_POINT('Ctrl Pts',(-19.8224365639408,12.642864050615,132.083409533469)) ;
#139787=CARTESIAN_POINT('Ctrl Pts',(-19.7370034747035,12.498964683589,131.867247414225)) ;
#139788=CARTESIAN_POINT('Ctrl Pts',(-19.6435550568839,12.4231077011215,
131.627078243334)) ;
#139789=CARTESIAN_POINT('Ctrl Pts',(-19.5452918269363,12.4177381472718,
131.373293221748)) ;
#139790=CARTESIAN_POINT('Ctrl Pts',(-19.4502640880226,12.4847095066073,
131.12876911611)) ;
#139791=CARTESIAN_POINT('Ctrl Pts',(-19.3637607477036,12.6190667593984,
130.909250351995)) ;
#139792=CARTESIAN_POINT('Ctrl Pts',(-19.2917485016945,12.8107471033722,
130.73197610566)) ;
#139793=CARTESIAN_POINT('Ctrl Pts',(-19.2383722341429,13.0461048084143,
130.609139594497)) ;
#139794=CARTESIAN_POINT('Ctrl Pts',(-19.2067190366217,13.3089103849839,
130.549819117407)) ;
#139795=CARTESIAN_POINT('Ctrl Pts',(-19.1984163850956,13.5795917474079,
130.558672442477)) ;
#139796=CARTESIAN_POINT('Ctrl Pts',(-19.2133495061686,13.839854863598,130.635502057452)) ;
#139797=CARTESIAN_POINT('Ctrl Pts',(-19.2498210148366,14.069864909241,130.775231781513)) ;
#139798=CARTESIAN_POINT('Ctrl Pts',(-19.303953532,14.2524396014981,130.966329916939)) ;
#139799=CARTESIAN_POINT('Ctrl Pts',(-19.3719147269832,14.3767943035019,
131.198056739573)) ;
#139800=CARTESIAN_POINT('Ctrl Pts',(-19.4473716314663,14.4324209572319,
131.451501532081)) ;
#139801=CARTESIAN_POINT('Ctrl Pts',(-19.5249669302885,14.4159981206257,
131.711381779073)) ;
#139802=CARTESIAN_POINT('Ctrl Pts',(-19.597827991755,14.3283155320889,131.957349776484)) ;
#139803=CARTESIAN_POINT('Ctrl Pts',(-19.6602314704124,14.1755659228116,
132.172810910082)) ;
#139804=CARTESIAN_POINT('Ctrl Pts',(-19.7067461930134,13.969906825541,132.341699515984)) ;
#139805=CARTESIAN_POINT('Ctrl Pts',(-19.733719116319,13.7239840128541,132.45368170668)) ;
#139806=CARTESIAN_POINT('Ctrl Pts',(-19.7382480950635,13.4571372933653,
132.500002078048)) ;
#139807=CARTESIAN_POINT('Ctrl Pts',(-19.7190532761567,13.1860385186985,
132.477260427293)) ;
#139808=CARTESIAN_POINT('Ctrl Pts',(-19.6774975461961,12.9351633427926,
132.388755944701)) ;
#139809=CARTESIAN_POINT('Ctrl Pts',(-19.6146960459712,12.716280428453,132.238634235809)) ;
#139810=CARTESIAN_POINT('Ctrl Pts',(-19.5360671274921,12.5504602967878,
132.041808804563)) ;
#139811=CARTESIAN_POINT('Ctrl Pts',(-19.4442410734227,12.4451571780271,
131.806961913747)) ;
#139812=CARTESIAN_POINT('Ctrl Pts',(-19.3476800781724,12.4110818136484,
131.557787015992)) ;
#139813=CARTESIAN_POINT('Ctrl Pts',(-19.2501729684496,12.4493848627275,
131.306248653423)) ;
#139814=CARTESIAN_POINT('Ctrl Pts',(-19.1602098012831,12.556427913144,131.076316665042)) ;
#139815=CARTESIAN_POINT('Ctrl Pts',(-19.0812293628911,12.7270948717805,
130.878914133552)) ;
#139816=CARTESIAN_POINT('Ctrl Pts',(-19.0199253013521,12.9467013402175,
130.732905024988)) ;
#139817=CARTESIAN_POINT('Ctrl Pts',(-18.9791994391495,13.2005745563337,
130.647059694796)) ;
#139818=CARTESIAN_POINT('Ctrl Pts',(-18.961416480655,13.4697556094875,130.628155579184)) ;
#139819=CARTESIAN_POINT('Ctrl Pts',(-18.9669430878151,13.7362552359381,
130.677419445868)) ;
#139820=CARTESIAN_POINT('Ctrl Pts',(-18.9950886554368,13.9814041933257,
130.792933897764)) ;
#139821=CARTESIAN_POINT('Ctrl Pts',(-19.0423528665076,14.1841666830384,
130.963922155526)) ;
#139822=CARTESIAN_POINT('Ctrl Pts',(-19.1054906760443,14.3343211929266,
131.181586250373)) ;
#139823=CARTESIAN_POINT('Ctrl Pts',(-19.1787695169468,14.4184551111194,
131.428790827256)) ;
#139824=CARTESIAN_POINT('Ctrl Pts',(-19.2561021849108,14.4314519975607,
131.687762211676)) ;
#139825=CARTESIAN_POINT('Ctrl Pts',(-19.3316103231487,14.3721435273992,
131.941493904809)) ;
#139826=CARTESIAN_POINT('Ctrl Pts',(-19.3987869878459,14.2453738509882,
132.17077888087)) ;
#139827=CARTESIAN_POINT('Ctrl Pts',(-19.4526636136295,14.0581566958374,
132.361480983201)) ;
#139828=CARTESIAN_POINT('Ctrl Pts',(-19.4877496207034,13.8276968106527,
132.496917353222)) ;
#139829=CARTESIAN_POINT('Ctrl Pts',(-19.5016628587778,13.5670203755234,
132.570710388361)) ;
#139830=CARTESIAN_POINT('Ctrl Pts',(-19.4921504180094,13.2953786744785,
132.576141543242)) ;
#139831=CARTESIAN_POINT('Ctrl Pts',(-19.4595143011011,13.0342214950179,
132.513845802004)) ;
#139832=CARTESIAN_POINT('Ctrl Pts',(-19.404757825179,12.7992352777049,132.3871899735)) ;
#139833=CARTESIAN_POINT('Ctrl Pts',(-19.3323102196323,12.6113833120471,
132.208445138207)) ;
#139834=CARTESIAN_POINT('Ctrl Pts',(-19.245255132006,12.4798503942449,131.987327845367)) ;
#139835=CARTESIAN_POINT('Ctrl Pts',(-19.1498981315355,12.416397864002,131.741859779545)) ;
#139836=CARTESIAN_POINT('Ctrl Pts',(-19.0518914034853,12.4249214929509,
131.48873919952)) ;
#139837=CARTESIAN_POINT('Ctrl Pts',(-18.9577972429175,12.5053755952326,
131.247046053355)) ;
#139838=CARTESIAN_POINT('Ctrl Pts',(-18.8740488421285,12.6507859052006,
131.03539948894)) ;
#139839=CARTESIAN_POINT('Ctrl Pts',(-18.8051224385857,12.8517470992337,
130.867160655025)) ;
#139840=CARTESIAN_POINT('Ctrl Pts',(-18.755477683788,13.0945614507412,130.755357286549)) ;
#139841=CARTESIAN_POINT('Ctrl Pts',(-18.7282047545516,13.3602126376938,
130.708805044059)) ;
#139842=CARTESIAN_POINT('Ctrl Pts',(-18.7244086987787,13.6310671963869,
130.730927107982)) ;
#139843=CARTESIAN_POINT('Ctrl Pts',(-18.743500281934,13.8852753848623,130.819680825134)) ;
#139844=CARTESIAN_POINT('Ctrl Pts',(-18.7834694283885,14.1076160740045,
130.969569123117)) ;
#139845=CARTESIAN_POINT('Ctrl Pts',(-18.8408194229245,14.2808806662079,
131.17024945925)) ;
#139846=CARTESIAN_POINT('Ctrl Pts',(-18.9105127297827,14.3926567103846,
131.406935440649)) ;
#139847=CARTESIAN_POINT('Ctrl Pts',(-18.9872957427596,14.4348969491125,
131.664485900502)) ;
#139848=CARTESIAN_POINT('Ctrl Pts',(-19.0638704847947,14.4049966950683,
131.921100002991)) ;
#139849=CARTESIAN_POINT('Ctrl Pts',(-19.1357123707124,14.3037928875116,
132.164340586752)) ;
#139850=CARTESIAN_POINT('Ctrl Pts',(-19.1951840074815,14.1405203865162,
132.371065416947)) ;
#139851=CARTESIAN_POINT('Ctrl Pts',(-19.2383746342019,13.9258191062473,
132.530330042627)) ;
#139852=CARTESIAN_POINT('Ctrl Pts',(-19.2612393922595,13.6747404924344,
132.630256846622)) ;
#139853=CARTESIAN_POINT('Ctrl Pts',(-19.2612747094853,13.4052256695436,
132.663545947711)) ;
#139854=CARTESIAN_POINT('Ctrl Pts',(-19.2380141324854,13.1384692475265,
132.628587768921)) ;
#139855=CARTESIAN_POINT('Ctrl Pts',(-19.1918391689992,12.8897551535746,
132.527009776568)) ;
#139856=CARTESIAN_POINT('Ctrl Pts',(-19.126091093419,12.6813707953234,132.367962858897)) ;
#139857=CARTESIAN_POINT('Ctrl Pts',(-19.0442932969066,12.5252896402636,
132.162121171031)) ;
#139858=CARTESIAN_POINT('Ctrl Pts',(-18.9515387706438,12.4335762079788,
131.92430473329)) ;
#139859=CARTESIAN_POINT('Ctrl Pts',(-18.8540901109851,12.4126069664436,
131.672696703125)) ;
#139860=CARTESIAN_POINT('Ctrl Pts',(-18.7573139352387,12.4645413764585,
131.423289841079)) ;
#139861=CARTESIAN_POINT('Ctrl Pts',(-18.6688905994528,12.5845282668637,
131.197986389939)) ;
#139862=CARTESIAN_POINT('Ctrl Pts',(-18.5931176264357,12.7652451064021,
131.00983237108)) ;
#139863=CARTESIAN_POINT('Ctrl Pts',(-18.5355210589981,12.9922347341953,
130.87461739619)) ;
#139864=CARTESIAN_POINT('Ctrl Pts',(-18.4989961498704,13.2501818574091,
130.801001377133)) ;
#139865=CARTESIAN_POINT('Ctrl Pts',(-18.4855372905734,13.5208713010695,
130.794807344722)) ;
#139866=CARTESIAN_POINT('Ctrl Pts',(-18.4955335672346,13.7852948748941,
130.857230166328)) ;
#139867=CARTESIAN_POINT('Ctrl Pts',(-18.5274723089381,14.0230293879869,
130.983660181575)) ;
#139868=CARTESIAN_POINT('Ctrl Pts',(-18.5783697625451,14.2178154382897,
131.165497530638)) ;
#139869=CARTESIAN_POINT('Ctrl Pts',(-18.643524354548,14.3552930540828,131.388848328232)) ;
#139870=CARTESIAN_POINT('Ctrl Pts',(-18.7182803703141,14.4265292549101,
131.640468998874)) ;
#139871=CARTESIAN_POINT('Ctrl Pts',(-18.7954462603385,14.425752226316,131.898835298117)) ;
#139872=CARTESIAN_POINT('Ctrl Pts',(-18.8700317215188,14.3531911968223,
132.149935023359)) ;
#139873=CARTESIAN_POINT('Ctrl Pts',(-18.9351141529095,14.2139749127786,
132.373170205042)) ;
#139874=CARTESIAN_POINT('Ctrl Pts',(-18.9855856813573,14.0181343155111,
132.553741039007)) ;
#139875=CARTESIAN_POINT('Ctrl Pts',(-19.0170527791197,13.7796845152241,
132.67878717668)) ;
#139876=CARTESIAN_POINT('Ctrl Pts',(-19.0265426890785,13.5155236059082,
132.73965320383)) ;
#139877=CARTESIAN_POINT('Ctrl Pts',(-19.0126470434056,13.245212667821,132.732147951906)) ;
#139878=CARTESIAN_POINT('Ctrl Pts',(-18.9757739987236,12.987705840382,132.657498715243)) ;
#139879=CARTESIAN_POINT('Ctrl Pts',(-18.917353844323,12.7602060641004,132.520089995502)) ;
#139880=CARTESIAN_POINT('Ctrl Pts',(-18.8416873381816,12.5817512683668,
132.332045933198)) ;
#139881=CARTESIAN_POINT('Ctrl Pts',(-18.7527220787295,12.4625557490256,
132.105291067502)) ;
#139882=CARTESIAN_POINT('Ctrl Pts',(-18.6561524362465,12.4124303716615,
131.85638030583)) ;
#139883=CARTESIAN_POINT('Ctrl Pts',(-18.5587876591386,12.4345388124725,
131.604997753593)) ;
#139884=CARTESIAN_POINT('Ctrl Pts',(-18.4657463620496,12.5283216508309,
131.366516292269)) ;
#139885=CARTESIAN_POINT('Ctrl Pts',(-18.3846425685644,12.6848122418478,
131.162526699351)) ;
#139886=CARTESIAN_POINT('Ctrl Pts',(-18.3189041583985,12.8954782936503,
131.003714766411)) ;
#139887=CARTESIAN_POINT('Ctrl Pts',(-18.2735334103624,13.1430312218348,
130.904237046659)) ;
#139888=CARTESIAN_POINT('Ctrl Pts',(-18.2506075637187,13.4109716011332,
130.870388378044)) ;
#139889=CARTESIAN_POINT('Ctrl Pts',(-18.2510953745575,13.6794256976715,
130.904880423363)) ;
#139890=CARTESIAN_POINT('Ctrl Pts',(-18.2745400654485,13.9314101100325,
131.006701969376)) ;
#139891=CARTESIAN_POINT('Ctrl Pts',(-18.3180431395774,14.1445006487741,
131.166780524465)) ;
#139892=CARTESIAN_POINT('Ctrl Pts',(-18.3779447844779,14.3067536437968,
131.374830990371)) ;
#139893=CARTESIAN_POINT('Ctrl Pts',(-18.4494808894986,14.406048704081,131.616955707788)) ;
#139894=CARTESIAN_POINT('Ctrl Pts',(-18.5266147943566,14.4348548847552,
131.875427792683)) ;
#139895=CARTESIAN_POINT('Ctrl Pts',(-18.6031387758285,14.3909041630567,
132.13214715581)) ;
#139896=CARTESIAN_POINT('Ctrl Pts',(-18.672466809759,14.2783347408893,132.367672775823)) ;
#139897=CARTESIAN_POINT('Ctrl Pts',(-18.729768369512,14.1031935326512,132.568357731683)) ;
#139898=CARTESIAN_POINT('Ctrl Pts',(-18.7692792357669,13.8800104531449,
132.716889273809)) ;
#139899=CARTESIAN_POINT('Ctrl Pts',(-18.7878950784534,13.6249527431351,
132.804295026184)) ;
#139900=CARTESIAN_POINT('Ctrl Pts',(-18.7835775171384,13.3547990106838,
132.824795353813)) ;
#139901=CARTESIAN_POINT('Ctrl Pts',(-18.7559551907665,13.0897726871477,
132.777172665473)) ;
#139902=CARTESIAN_POINT('Ctrl Pts',(-18.7056493126971,12.8467549358408,
132.663569693571)) ;
#139903=CARTESIAN_POINT('Ctrl Pts',(-18.6367644882602,12.6478124194814,
132.495268377589)) ;
#139904=CARTESIAN_POINT('Ctrl Pts',(-18.5523377209398,12.5027972017395,
132.281818498312)) ;
#139905=CARTESIAN_POINT('Ctrl Pts',(-18.4583099874776,12.4240443631204,
132.040236913636)) ;
#139906=CARTESIAN_POINT('Ctrl Pts',(-18.3600026659222,12.4170503620235,
131.78633891546)) ;
#139907=CARTESIAN_POINT('Ctrl Pts',(-18.2651791024171,12.4817913910706,
131.542286722758)) ;
#139908=CARTESIAN_POINT('Ctrl Pts',(-18.1783121098205,12.6142900720352,
131.321713466676)) ;
#139909=CARTESIAN_POINT('Ctrl Pts',(-18.1059030417794,12.8042103797361,
131.143238469633)) ;
#139910=CARTESIAN_POINT('Ctrl Pts',(-18.0517927161876,13.0388186679886,
131.018309361831)) ;
#139911=CARTESIAN_POINT('Ctrl Pts',(-18.0194468757643,13.3023285356057,
130.957112158902)) ;
#139912=CARTESIAN_POINT('Ctrl Pts',(-18.010553505915,13.5713414244093,130.964028233933)) ;
#139913=CARTESIAN_POINT('Ctrl Pts',(-18.0248407334206,13.8329962624196,
131.039074983234)) ;
#139914=CARTESIAN_POINT('Ctrl Pts',(-18.0606661101291,14.0635776732595,
131.176836792273)) ;
#139915=CARTESIAN_POINT('Ctrl Pts',(-18.1144212284498,14.2479537129057,
131.366889432895)) ;
#139916=CARTESIAN_POINT('Ctrl Pts',(-18.181823386805,14.3739504524616,131.596871180233)) ;
#139917=CARTESIAN_POINT('Ctrl Pts',(-18.2577639652939,14.4320428202114,
131.852004261572)) ;
#139918=CARTESIAN_POINT('Ctrl Pts',(-18.335190107087,14.4172275028747,132.111300594873)) ;
#139919=CARTESIAN_POINT('Ctrl Pts',(-18.4079980802751,14.3318166981341,
132.356999976137)) ;
#139920=CARTESIAN_POINT('Ctrl Pts',(-18.4707526739101,14.1811818293068,
132.573443859894)) ;
#139921=CARTESIAN_POINT('Ctrl Pts',(-18.5179547252937,13.9759967622757,
132.744480222502)) ;
#139922=CARTESIAN_POINT('Ctrl Pts',(-18.5455049432356,13.7313492386451,
132.858087358722)) ;
#139923=CARTESIAN_POINT('Ctrl Pts',(-18.5505621183255,13.4634561102099,
132.90612740095)) ;
#139924=CARTESIAN_POINT('Ctrl Pts',(-18.5323956205154,13.195884935421,132.885916030793)) ;
#139925=CARTESIAN_POINT('Ctrl Pts',(-18.4910611657277,12.9412337002998,
132.798458784321)) ;
#139926=CARTESIAN_POINT('Ctrl Pts',(-18.4293713026605,12.7230235152343,
132.651272706854)) ;
#139927=CARTESIAN_POINT('Ctrl Pts',(-18.3504480692178,12.5539648154296,
132.453908084872)) ;
#139928=CARTESIAN_POINT('Ctrl Pts',(-18.2598574156189,12.4477725877379,
132.222306799137)) ;
#139929=CARTESIAN_POINT('Ctrl Pts',(-18.1626825266472,12.4110238126212,
131.971596895803)) ;
#139930=CARTESIAN_POINT('Ctrl Pts',(-18.0655649689106,12.4468710250015,
131.721015136346)) ;
#139931=CARTESIAN_POINT('Ctrl Pts',(-17.9743916784582,12.553155401547,131.487903989302)) ;
#139932=CARTESIAN_POINT('Ctrl Pts',(-17.8956552680024,12.7211113699614,
131.29094946649)) ;
#139933=CARTESIAN_POINT('Ctrl Pts',(-17.8335847561052,12.9400020395614,
131.142803371709)) ;
#139934=CARTESIAN_POINT('Ctrl Pts',(-17.792384111752,13.1921120762229,131.055433053991)) ;
#139935=CARTESIAN_POINT('Ctrl Pts',(-17.7737717164207,13.4620045651565,
131.034220681022)) ;
#139936=CARTESIAN_POINT('Ctrl Pts',(-17.7787420438599,13.7292706567068,
131.081916802346)) ;
#139937=CARTESIAN_POINT('Ctrl Pts',(-17.8060353128766,13.9738126182776,
131.194724636009)) ;
#139938=CARTESIAN_POINT('Ctrl Pts',(-17.853039869841,14.1794947275424,131.365176033557)) ;
#139939=CARTESIAN_POINT('Ctrl Pts',(-17.9159450098139,14.3311259291818,
131.582191022847)) ;
#139940=CARTESIAN_POINT('Ctrl Pts',(-17.9885875436753,14.4169205617397,
131.827348730516)) ;
#139941=CARTESIAN_POINT('Ctrl Pts',(-18.0663285917671,14.4320030315974,
132.087711051093)) ;
#139942=CARTESIAN_POINT('Ctrl Pts',(-18.1415675439527,14.3751243687379,
132.340459922905)) ;
#139943=CARTESIAN_POINT('Ctrl Pts',(-18.2096359824422,14.2488768179311,
132.572659748216)) ;
#139944=CARTESIAN_POINT('Ctrl Pts',(-18.2634030402634,14.0648018746923,
132.762713076847)) ;
#139945=CARTESIAN_POINT('Ctrl Pts',(-18.2993393835354,13.8343788522074,
132.900814395349)) ;
#139946=CARTESIAN_POINT('Ctrl Pts',(-18.3138052523307,13.5736071381831,
132.976286578787)) ;
#139947=CARTESIAN_POINT('Ctrl Pts',(-18.304900108542,13.3025525300613,132.983425008922)) ;
#139948=CARTESIAN_POINT('Ctrl Pts',(-18.2730041011089,13.0417945957582,
132.923179652522)) ;
#139949=CARTESIAN_POINT('Ctrl Pts',(-18.2190983791431,12.8063140685278,
132.798906207675)) ;
#139950=CARTESIAN_POINT('Ctrl Pts',(-18.1468168584937,12.6158856975737,
132.620808271038)) ;
#139951=CARTESIAN_POINT('Ctrl Pts',(-18.0599209734576,12.4825396970198,
132.400205037205)) ;
#139952=CARTESIAN_POINT('Ctrl Pts',(-17.9649956111779,12.4173081237828,
132.155903217659)) ;
#139953=CARTESIAN_POINT('Ctrl Pts',(-17.8670768307849,12.423605000428,131.903005180849)) ;
#139954=CARTESIAN_POINT('Ctrl Pts',(-17.7728138214266,12.5018025966581,
131.660799723848)) ;
#139955=CARTESIAN_POINT('Ctrl Pts',(-17.6884211517769,12.6458565798938,
131.44737668302)) ;
#139956=CARTESIAN_POINT('Ctrl Pts',(-17.6190781329538,12.8453790833706,
131.27789881031)) ;
#139957=CARTESIAN_POINT('Ctrl Pts',(-17.5689078790036,13.0865652662194,
131.164476359025)) ;
#139958=CARTESIAN_POINT('Ctrl Pts',(-17.5409063530065,13.3521427577607,
131.11584353298)) ;
#139959=CARTESIAN_POINT('Ctrl Pts',(-17.5363739810292,13.6222557202932,
131.135702219047)) ;
#139960=CARTESIAN_POINT('Ctrl Pts',(-17.5548275317412,13.8783882969557,
131.2227406542)) ;
#139961=CARTESIAN_POINT('Ctrl Pts',(-17.5943750726365,14.1022120618795,
131.37145767239)) ;
#139962=CARTESIAN_POINT('Ctrl Pts',(-17.6511400306937,14.2765229506337,
131.570334937194)) ;
#139963=CARTESIAN_POINT('Ctrl Pts',(-17.7204518418135,14.3902286964009,
131.805872441639)) ;
#139964=CARTESIAN_POINT('Ctrl Pts',(-17.7972369816987,14.4347769427253,
132.063476509969)) ;
#139965=CARTESIAN_POINT('Ctrl Pts',(-17.8740308161132,14.4066722617846,
132.320801188858)) ;
#139966=CARTESIAN_POINT('Ctrl Pts',(-17.9456993619042,14.3082119125381,
132.563325601213)) ;
#139967=CARTESIAN_POINT('Ctrl Pts',(-18.0059086330157,14.1460357867196,
132.772367372232)) ;
#139968=CARTESIAN_POINT('Ctrl Pts',(-18.0495959794959,13.9328084574968,
132.933044174357)) ;
#139969=CARTESIAN_POINT('Ctrl Pts',(-18.0731093783754,13.681774125451,133.034966341069)) ;
#139970=CARTESIAN_POINT('Ctrl Pts',(-18.0738683957939,13.414026239165,133.070176901805)) ;
#139971=CARTESIAN_POINT('Ctrl Pts',(-18.0511266283768,13.1453688505525,
133.036941887299)) ;
#139972=CARTESIAN_POINT('Ctrl Pts',(-18.0059948266115,12.8977836793382,
132.938130042737)) ;
#139973=CARTESIAN_POINT('Ctrl Pts',(-17.9402912323445,12.6861562687701,
132.779496079662)) ;
#139974=CARTESIAN_POINT('Ctrl Pts',(-17.8590011189062,12.5289208649723,
132.575061965886)) ;
#139975=CARTESIAN_POINT('Ctrl Pts',(-17.7663814238346,12.4351549173609,
132.337678380036)) ;
#139976=CARTESIAN_POINT('Ctrl Pts',(-17.6692083593153,12.41223935111,132.086798615346)) ;
#139977=CARTESIAN_POINT('Ctrl Pts',(-17.5723092010791,12.4619213802628,
131.837027428142)) ;
#139978=CARTESIAN_POINT('Ctrl Pts',(-17.4833798800122,12.5803996576492,
131.610327628056)) ;
#139979=CARTESIAN_POINT('Ctrl Pts',(-17.4073580775245,12.7591299029993,
131.421362280643)) ;
#139980=CARTESIAN_POINT('Ctrl Pts',(-17.3491268284245,12.9850687098392,
131.284316932474)) ;
#139981=CARTESIAN_POINT('Ctrl Pts',(-17.3119541347841,13.2423777054139,
131.20880655253)) ;
#139982=CARTESIAN_POINT('Ctrl Pts',(-17.2978226688005,13.5129449016412,
131.200646200816)) ;
#139983=CARTESIAN_POINT('Ctrl Pts',(-17.3070879903219,13.7774320597186,
131.260874076779)) ;
#139984=CARTESIAN_POINT('Ctrl Pts',(-17.3384928099776,14.0166134042629,
131.385813340299)) ;
#139985=CARTESIAN_POINT('Ctrl Pts',(-17.3885767506353,14.2120830530507,
131.565102403099)) ;
#139986=CARTESIAN_POINT('Ctrl Pts',(-17.4538316971294,14.352498916215,131.788992594797)) ;
#139987=CARTESIAN_POINT('Ctrl Pts',(-17.5281745380114,14.4253825701344,
132.039289476329)) ;
#139988=CARTESIAN_POINT('Ctrl Pts',(-17.6054634622487,14.426768294094,132.298075516539)) ;
#139989=CARTESIAN_POINT('Ctrl Pts',(-17.6800468801876,14.3564920185828,
132.549080337008)) ;
#139990=CARTESIAN_POINT('Ctrl Pts',(-17.7457143234865,14.2186719371757,
132.774142097091)) ;
#139991=CARTESIAN_POINT('Ctrl Pts',(-17.7966202311834,14.024316786925,132.955958740035)) ;
#139992=CARTESIAN_POINT('Ctrl Pts',(-17.8286778334795,13.7866136068205,
133.082761139873)) ;
#139993=CARTESIAN_POINT('Ctrl Pts',(-17.8387984063553,13.5238037033397,
133.145359694921)) ;
#139994=CARTESIAN_POINT('Ctrl Pts',(-17.8256146623074,13.2527086042196,
133.140017565356)) ;
#139995=CARTESIAN_POINT('Ctrl Pts',(-17.7891304573137,12.9936530632693,
133.066635952867)) ;
#139996=CARTESIAN_POINT('Ctrl Pts',(-17.7315183419931,12.7662441874236,
132.93142162794)) ;
#139997=CARTESIAN_POINT('Ctrl Pts',(-17.6561927558797,12.5858801409006,
132.744430610963)) ;
#139998=CARTESIAN_POINT('Ctrl Pts',(-17.5674505982938,12.4648530718858,
132.518345830631)) ;
#139999=CARTESIAN_POINT('Ctrl Pts',(-17.4708526129738,12.4128201875619,
132.269401513626)) ;
#140000=CARTESIAN_POINT('Ctrl Pts',(-17.3738183375729,12.4330274107103,
132.018859494709)) ;
#140001=CARTESIAN_POINT('Ctrl Pts',(-17.2809556103288,12.524012324909,131.780737711725)) ;
#140002=CARTESIAN_POINT('Ctrl Pts',(-17.1989341049103,12.6795221282536,
131.57426239901)) ;
#140003=CARTESIAN_POINT('Ctrl Pts',(-17.1327378420487,12.8889214141028,
131.414101802532)) ;
#140004=CARTESIAN_POINT('Ctrl Pts',(-17.0867269430234,13.1354947089828,
131.312742856685)) ;
#140005=CARTESIAN_POINT('Ctrl Pts',(-17.0630990286742,13.4042911436029,
131.276983650143)) ;
#140006=CARTESIAN_POINT('Ctrl Pts',(-17.0630113893596,13.6719452313923,
131.309670318193)) ;
#140007=CARTESIAN_POINT('Ctrl Pts',(-17.0857204958191,13.9242175336792,
131.409269871991)) ;
#140008=CARTESIAN_POINT('Ctrl Pts',(-17.1287442358938,14.1390288741834,
131.568008046519)) ;
#140009=CARTESIAN_POINT('Ctrl Pts',(-17.1882900238395,14.3030286144717,
131.775040930177)) ;
#140010=CARTESIAN_POINT('Ctrl Pts',(-17.2596164114591,14.4041953326341,
132.016566385165)) ;
#140011=CARTESIAN_POINT('Ctrl Pts',(-17.3364367314704,14.4349854779899,
132.274021676845)) ;
#140012=CARTESIAN_POINT('Ctrl Pts',(-17.4130831782189,14.3934046886661,
132.531096520565)) ;
#140013=CARTESIAN_POINT('Ctrl Pts',(-17.4829306248326,14.2822103121525,
132.768262973992)) ;
#140014=CARTESIAN_POINT('Ctrl Pts',(-17.5403192864147,14.1097942363152,
132.968995643959)) ;
#140015=CARTESIAN_POINT('Ctrl Pts',(-17.5805733706792,13.8877667094565,
133.119746822849)) ;
#140016=CARTESIAN_POINT('Ctrl Pts',(-17.5999033803559,13.6324084420419,
133.209366061804)) ;
#140017=CARTESIAN_POINT('Ctrl Pts',(-17.596247458933,13.3624185504467,133.231793716882)) ;
#140018=CARTESIAN_POINT('Ctrl Pts',(-17.5691757856173,13.0965814778885,
133.185837900411)) ;
#140019=CARTESIAN_POINT('Ctrl Pts',(-17.5197846541153,12.8540736174815,
133.074706584003)) ;
#140020=CARTESIAN_POINT('Ctrl Pts',(-17.451348287198,12.652992435015,132.907789970015)) ;
#140021=CARTESIAN_POINT('Ctrl Pts',(-17.3667759142286,12.5055874303856,
132.694097208918)) ;
#140022=CARTESIAN_POINT('Ctrl Pts',(-17.2733692229142,12.4255318647486,
132.454172659202)) ;
#140023=CARTESIAN_POINT('Ctrl Pts',(-17.1755318837841,12.4160627512278,
132.201498055215)) ;
#140024=CARTESIAN_POINT('Ctrl Pts',(-17.0800677624105,12.4788299066414,
131.955734672931)) ;
#140025=CARTESIAN_POINT('Ctrl Pts',(-16.9928119833877,12.6096602766835,
131.734049308796)) ;
#140026=CARTESIAN_POINT('Ctrl Pts',(-16.9198008856656,12.7985462130252,
131.553883363849)) ;
#140027=CARTESIAN_POINT('Ctrl Pts',(-16.8653086304422,13.031708612879,131.427766361266)) ;
#140028=CARTESIAN_POINT('Ctrl Pts',(-16.8323684675315,13.293083578928,131.364642117709)) ;
#140029=CARTESIAN_POINT('Ctrl Pts',(-16.8226660727472,13.5641924680593,
131.369449472426)) ;
#140030=CARTESIAN_POINT('Ctrl Pts',(-16.8363638395971,13.8256806601297,
131.442688303253)) ;
#140031=CARTESIAN_POINT('Ctrl Pts',(-16.8713842098541,14.0565823152587,
131.577970763861)) ;
#140032=CARTESIAN_POINT('Ctrl Pts',(-16.9248059316069,14.2434411149003,
131.76717177554)) ;
#140033=CARTESIAN_POINT('Ctrl Pts',(-16.9921951195004,14.3714533613372,
131.997241772447)) ;
#140034=CARTESIAN_POINT('Ctrl Pts',(-17.0673511293183,14.4311593709141,
132.249804262029)) ;
#140035=CARTESIAN_POINT('Ctrl Pts',(-17.1450034626173,14.4188767370812,
132.509845921802)) ;
#140036=CARTESIAN_POINT('Ctrl Pts',(-17.2181873389402,14.3353893813971,
132.756704184413)) ;
#140037=CARTESIAN_POINT('Ctrl Pts',(-17.2814813061672,14.1858866209329,
132.974831456389)) ;
#140038=CARTESIAN_POINT('Ctrl Pts',(-17.3289977855556,13.9829323143578,
133.14664284081)) ;
#140039=CARTESIAN_POINT('Ctrl Pts',(-17.3572257515771,13.7386001915966,
133.262317495533)) ;
#140040=CARTESIAN_POINT('Ctrl Pts',(-17.3629896704757,13.472491070878,133.312245512371)) ;
#140041=CARTESIAN_POINT('Ctrl Pts',(-17.3454245972226,13.2027754622607,
133.294032832636)) ;
#140042=CARTESIAN_POINT('Ctrl Pts',(-17.3046250802462,12.9475729445581,
133.208125531195)) ;
#140043=CARTESIAN_POINT('Ctrl Pts',(-17.2435833734801,12.7286906854066,
133.062766425607)) ;
#140044=CARTESIAN_POINT('Ctrl Pts',(-17.1653001243494,12.5582194228626,
132.867194935478)) ;
#140045=CARTESIAN_POINT('Ctrl Pts',(-17.0744878770675,12.4495814745878,
132.635124317158)) ;
#140046=CARTESIAN_POINT('Ctrl Pts',(-16.977602091249,12.4111325030014,132.385184551978)) ;
#140047=CARTESIAN_POINT('Ctrl Pts',(-16.8806236193526,12.4448573230465,
132.134938711957)) ;
#140048=CARTESIAN_POINT('Ctrl Pts',(-16.7894019430177,12.5485736269638,
131.901587070824)) ;
#140049=CARTESIAN_POINT('Ctrl Pts',(-16.7097006554741,12.7160675409956,
131.702047644044)) ;
#140050=CARTESIAN_POINT('Ctrl Pts',(-16.6474333959251,12.9327061634172,
131.55315650852)) ;
#140051=CARTESIAN_POINT('Ctrl Pts',(-16.6054314285535,13.1846668378338,
131.463536928802)) ;
#140052=CARTESIAN_POINT('Ctrl Pts',(-16.5861998611225,13.4544224505961,
131.440520016968)) ;
#140053=CARTESIAN_POINT('Ctrl Pts',(-16.5904757716003,13.7215757277082,
131.486129856679)) ;
#140054=CARTESIAN_POINT('Ctrl Pts',(-16.6171930426673,13.9674105771419,
131.597307673441)) ;
#140055=CARTESIAN_POINT('Ctrl Pts',(-16.6636138619868,14.173959529566,131.765990224629)) ;
#140056=CARTESIAN_POINT('Ctrl Pts',(-16.7258970011584,14.3272528917974,
131.981094732715)) ;
#140057=CARTESIAN_POINT('Ctrl Pts',(-16.7988063944434,14.4155297933765,
132.227255254739)) ;
#140058=CARTESIAN_POINT('Ctrl Pts',(-16.8760210825582,14.4326688919931,
132.485862874767)) ;
#140059=CARTESIAN_POINT('Ctrl Pts',(-16.951873050781,14.3775210851954,132.740618667098)) ;
#140060=CARTESIAN_POINT('Ctrl Pts',(-17.0197649340033,14.2540409497735,
132.97205574517)) ;
#140061=CARTESIAN_POINT('Ctrl Pts',(-17.0743094525665,14.0709648404294,
133.164530968928)) ;
#140062=CARTESIAN_POINT('Ctrl Pts',(-17.1107712589207,13.8416199904244,
133.304154870266)) ;
#140063=CARTESIAN_POINT('Ctrl Pts',(-17.1258886763416,13.582388567831,133.381421380426)) ;
#140064=CARTESIAN_POINT('Ctrl Pts',(-17.1178138289345,13.3112804497714,
133.390993708911)) ;
#140065=CARTESIAN_POINT('Ctrl Pts',(-17.0863471130288,13.0483997987315,
133.332210032555)) ;
#140066=CARTESIAN_POINT('Ctrl Pts',(-17.0332668996353,12.8130298392026,
133.210187809291)) ;
#140067=CARTESIAN_POINT('Ctrl Pts',(-16.9612682248294,12.6204060823588,
133.033025253701)) ;
#140068=CARTESIAN_POINT('Ctrl Pts',(-16.8747379912783,12.4854479324355,
132.813466850666)) ;
#140069=CARTESIAN_POINT('Ctrl Pts',(-16.7799596426297,12.4181326730335,
132.569603428481)) ;
#140070=CARTESIAN_POINT('Ctrl Pts',(-16.6817627892976,12.4224942487035,
132.315980950859)) ;
#140071=CARTESIAN_POINT('Ctrl Pts',(-16.5874095963749,12.4989653084942,
132.073488665005)) ;
#140072=CARTESIAN_POINT('Ctrl Pts',(-16.5030227664661,12.6405919477357,
131.859938970218)) ;
#140073=CARTESIAN_POINT('Ctrl Pts',(-16.4329418145269,12.8391593414189,
131.688400941445)) ;
#140074=CARTESIAN_POINT('Ctrl Pts',(-16.3820975732448,13.080245962358,131.573107657497)) ;
#140075=CARTESIAN_POINT('Ctrl Pts',(-16.3535910400909,13.3449462168028,
131.522937145774)) ;
#140076=CARTESIAN_POINT('Ctrl Pts',(-16.3483981201149,13.6142996681917,
131.540758663562)) ;
#140077=CARTESIAN_POINT('Ctrl Pts',(-16.3661681324322,13.8710421169928,
131.625790173589)) ;
#140078=CARTESIAN_POINT('Ctrl Pts',(-16.4051123344729,14.0962488257935,
131.772752900092)) ;
#140079=CARTESIAN_POINT('Ctrl Pts',(-16.4618078548578,14.2729914081674,
131.971617342725)) ;
#140080=CARTESIAN_POINT('Ctrl Pts',(-16.5304999126162,14.38767954712,132.205165563622)) ;
#140081=CARTESIAN_POINT('Ctrl Pts',(-16.6070330356264,14.4346057861831,
132.461982388263)) ;
#140082=CARTESIAN_POINT('Ctrl Pts',(-16.6843229990153,14.4082599468392,
132.720943868329)) ;
#140083=CARTESIAN_POINT('Ctrl Pts',(-16.7557875504688,14.3122705880149,
132.962668513264)) ;
#140084=CARTESIAN_POINT('Ctrl Pts',(-16.8166821611392,14.151436185241,133.173833669416)) ;
#140085=CARTESIAN_POINT('Ctrl Pts',(-16.8608925190079,13.9387188784377,
133.336119150085)) ;
#140086=CARTESIAN_POINT('Ctrl Pts',(-16.8849135991378,13.6904434125759,
133.439271987478)) ;
#140087=CARTESIAN_POINT('Ctrl Pts',(-16.8863661179106,13.4208420598601,
133.476776952907)) ;
#140088=CARTESIAN_POINT('Ctrl Pts',(-16.8643629093214,13.1534853902676,
133.445499699409)) ;
#140089=CARTESIAN_POINT('Ctrl Pts',(-16.8198173917774,12.9044050288982,
133.348483089943)) ;
#140090=CARTESIAN_POINT('Ctrl Pts',(-16.7545728094688,12.6913475994885,
133.19121034881)) ;
#140091=CARTESIAN_POINT('Ctrl Pts',(-16.6735792900983,12.5324269019675,
132.987673507823)) ;
#140092=CARTESIAN_POINT('Ctrl Pts',(-16.5815141879572,12.4369854947191,
132.751795055161)) ;
#140093=CARTESIAN_POINT('Ctrl Pts',(-16.484196424873,12.4119049760396,132.500565871752)) ;
#140094=CARTESIAN_POINT('Ctrl Pts',(-16.3875232228243,12.459288588066,132.25133200756)) ;
#140095=CARTESIAN_POINT('Ctrl Pts',(-16.2981920739487,12.5757336822765,
132.023487610852)) ;
#140096=CARTESIAN_POINT('Ctrl Pts',(-16.221663226933,12.7527802879128,131.833046815115)) ;
#140097=CARTESIAN_POINT('Ctrl Pts',(-16.1625644709713,12.9786618268138,
131.693629435243)) ;
#140098=CARTESIAN_POINT('Ctrl Pts',(-16.1248303893333,13.2359088344013,
131.616537241571)) ;
#140099=CARTESIAN_POINT('Ctrl Pts',(-16.1101106562054,13.5051026285248,
131.606499820776)) ;
#140100=CARTESIAN_POINT('Ctrl Pts',(-16.1187976807236,13.7711208876962,
131.665181919994)) ;
#140101=CARTESIAN_POINT('Ctrl Pts',(-16.1494970012602,14.0100003599807,
131.787889090912)) ;
#140102=CARTESIAN_POINT('Ctrl Pts',(-16.1991678311649,14.2073724408212,
131.966043243383)) ;
#140103=CARTESIAN_POINT('Ctrl Pts',(-16.2639738299788,14.3492226306733,
132.188560730462)) ;
#140104=CARTESIAN_POINT('Ctrl Pts',(-16.3380263648965,14.4242519881516,
132.43797256554)) ;
#140105=CARTESIAN_POINT('Ctrl Pts',(-16.4156431986028,14.4277364563771,
132.697856444715)) ;
#140106=CARTESIAN_POINT('Ctrl Pts',(-16.490288927873,14.3592420110673,132.949008230295)) ;
#140107=CARTESIAN_POINT('Ctrl Pts',(-16.5560174977799,14.2240686922171,
133.174088753831)) ;
#140108=CARTESIAN_POINT('Ctrl Pts',(-16.6076266234123,14.0305585465179,
133.358084944611)) ;
#140109=CARTESIAN_POINT('Ctrl Pts',(-16.6402104387998,13.7945206228156,
133.486333304394)) ;
#140110=CARTESIAN_POINT('Ctrl Pts',(-16.651061280046,13.5313067865741,133.551183520933)) ;
#140111=CARTESIAN_POINT('Ctrl Pts',(-16.6385182945988,13.2605192088026,
133.547666910289)) ;
#140112=CARTESIAN_POINT('Ctrl Pts',(-16.6028442001819,13.0015411116714,
133.476558081978)) ;
#140113=CARTESIAN_POINT('Ctrl Pts',(-16.5458000319494,12.7725523899085,
133.343047202527)) ;
#140114=CARTESIAN_POINT('Ctrl Pts',(-16.4707277903299,12.5901314079498,
133.156883276531)) ;
#140115=CARTESIAN_POINT('Ctrl Pts',(-16.3823389739391,12.4675131368497,
132.931805480759)) ;
#140116=CARTESIAN_POINT('Ctrl Pts',(-16.286313729189,12.4133289133512,132.684387528141)) ;
#140117=CARTESIAN_POINT('Ctrl Pts',(-16.1885428106146,12.4315113469885,
132.43192881401)) ;
#140118=CARTESIAN_POINT('Ctrl Pts',(-16.0957725720943,12.5204618731953,
132.193969057206)) ;
#140119=CARTESIAN_POINT('Ctrl Pts',(-16.0133683697875,12.6740885600686,
131.986368940502)) ;
#140120=CARTESIAN_POINT('Ctrl Pts',(-15.9466347797837,12.8820605633652,
131.82463063258)) ;
#140121=CARTESIAN_POINT('Ctrl Pts',(-15.8999755193379,13.1280849033747,
131.721420437203)) ;
#140122=CARTESIAN_POINT('Ctrl Pts',(-15.8756996992524,13.3954305468035,
131.683629487919)) ;
#140123=CARTESIAN_POINT('Ctrl Pts',(-15.8749154596136,13.6647721239679,
131.714464613994)) ;
#140124=CARTESIAN_POINT('Ctrl Pts',(-15.8968964489419,13.9166503672092,
131.811778285468)) ;
#140125=CARTESIAN_POINT('Ctrl Pts',(-15.9394126728008,14.1333087824096,
131.969110200075)) ;
#140126=CARTESIAN_POINT('Ctrl Pts',(-15.9984604507846,14.2989356836214,
132.174650382244)) ;
#140127=CARTESIAN_POINT('Ctrl Pts',(-16.069955047821,14.4025578145927,132.416862616266)) ;
#140128=CARTESIAN_POINT('Ctrl Pts',(-16.1464394854795,14.435010397795,132.673218956648)) ;
#140129=CARTESIAN_POINT('Ctrl Pts',(-16.2231180895877,14.3956728080676,
132.930357127469)) ;
#140130=CARTESIAN_POINT('Ctrl Pts',(-16.2932740093016,14.2862787578303,
133.168445846428)) ;
#140131=CARTESIAN_POINT('Ctrl Pts',(-16.3510597233741,14.1158603541274,
133.370289668947)) ;
#140132=CARTESIAN_POINT('Ctrl Pts',(-16.392061731818,13.8934485383183,133.523446661948)) ;
#140133=CARTESIAN_POINT('Ctrl Pts',(-16.4118475379423,13.6404741399982,
133.614166778358)) ;
#140134=CARTESIAN_POINT('Ctrl Pts',(-16.4088703893971,13.3695007340468,
133.638723997956)) ;
#140135=CARTESIAN_POINT('Ctrl Pts',(-16.382512592704,13.1044457267252,133.594710829848)) ;
#140136=CARTESIAN_POINT('Ctrl Pts',(-16.3338267763214,12.860704031683,133.485653364823)) ;
#140137=CARTESIAN_POINT('Ctrl Pts',(-16.2652943294484,12.6571154777524,
133.318695024141)) ;
#140138=CARTESIAN_POINT('Ctrl Pts',(-16.1821466626859,12.5098080554844,
133.108743958478)) ;
#140139=CARTESIAN_POINT('Ctrl Pts',(-16.0884174129943,12.4266891530237,
132.868087786362)) ;
#140140=CARTESIAN_POINT('Ctrl Pts',(-15.9903350041764,12.4154229755217,
132.614782524112)) ;
#140141=CARTESIAN_POINT('Ctrl Pts',(-15.8950587880633,12.4759770673935,
132.36945254477)) ;
#140142=CARTESIAN_POINT('Ctrl Pts',(-15.8074607836014,12.6048252394354,
132.146767087562)) ;
#140143=CARTESIAN_POINT('Ctrl Pts',(-15.7339345122349,12.7921645634063,
131.965101212743)) ;
#140144=CARTESIAN_POINT('Ctrl Pts',(-15.6787573253253,13.0247862212583,
131.83705713208)) ;
#140145=CARTESIAN_POINT('Ctrl Pts',(-15.6451872213494,13.2853105369572,
131.772049972934)) ;
#140146=CARTESIAN_POINT('Ctrl Pts',(-15.6348692512998,13.5574331010645,
131.775190161666)) ;
#140147=CARTESIAN_POINT('Ctrl Pts',(-15.6477474012688,13.8171021403353,
131.845722672944)) ;
#140148=CARTESIAN_POINT('Ctrl Pts',(-15.6823995504724,14.0511738702826,
131.980211338381)) ;
#140149=CARTESIAN_POINT('Ctrl Pts',(-15.7353430940617,14.2388281925165,
132.167944371015)) ;
#140150=CARTESIAN_POINT('Ctrl Pts',(-15.8021504706626,14.3685839243643,
132.396210499492)) ;
#140151=CARTESIAN_POINT('Ctrl Pts',(-15.8777413821372,14.430551147229,132.650299229092)) ;
#140152=CARTESIAN_POINT('Ctrl Pts',(-15.9548493427787,14.4203097396042,
132.908497044861)) ;
#140153=CARTESIAN_POINT('Ctrl Pts',(-16.0285863561776,14.3384208186475,
133.157141334588)) ;
#140154=CARTESIAN_POINT('Ctrl Pts',(-16.0919232558738,14.191573192343,133.375198147925)) ;
#140155=CARTESIAN_POINT('Ctrl Pts',(-16.1403208257874,13.9880715249732,
133.549888683024)) ;
#140156=CARTESIAN_POINT('Ctrl Pts',(-16.1688197828895,13.74717256078,133.665995114336)) ;
#140157=CARTESIAN_POINT('Ctrl Pts',(-16.1753840787558,13.4800206517718,
133.71845667894)) ;
#140158=CARTESIAN_POINT('Ctrl Pts',(-16.1585115139942,13.2110030826081,
133.70215466538)) ;
#140159=CARTESIAN_POINT('Ctrl Pts',(-16.1183902206883,12.9547749192264,
133.61826212713)) ;
#140160=CARTESIAN_POINT('Ctrl Pts',(-16.0578431071565,12.7344342414435,
133.474378704329)) ;
#140161=CARTESIAN_POINT('Ctrl Pts',(-15.9799587158776,12.56234537382,133.279982911303)) ;
#140162=CARTESIAN_POINT('Ctrl Pts',(-15.8896136740205,12.4518692107331,
133.049210374909)) ;
#140163=CARTESIAN_POINT('Ctrl Pts',(-15.7925458848479,12.4112334908308,
132.798839526536)) ;
#140164=CARTESIAN_POINT('Ctrl Pts',(-15.6955857869506,12.4427491476605,
132.548603262196)) ;
#140165=CARTESIAN_POINT('Ctrl Pts',(-15.6035799730376,12.5456206788136,
132.313181586489)) ;
#140166=CARTESIAN_POINT('Ctrl Pts',(-15.5245257438388,12.7091960260598,
132.115080647817)) ;
#140167=CARTESIAN_POINT('Ctrl Pts',(-15.4611054690331,12.9259029784642,
131.963079856296)) ;
#140168=CARTESIAN_POINT('Ctrl Pts',(-15.4185548878178,13.1770736213742,
131.871835443339)) ;
#140169=CARTESIAN_POINT('Ctrl Pts',(-15.398628373212,13.4468768316793,131.846827048019)) ;
#140170=CARTESIAN_POINT('Ctrl Pts',(-15.4022435837397,13.7138795758086,
131.890444695793)) ;
#140171=CARTESIAN_POINT('Ctrl Pts',(-15.4283089337862,13.9605431797111,
131.999711066717)) ;
#140172=CARTESIAN_POINT('Ctrl Pts',(-15.4741850451082,14.1686235448508,
132.166809272783)) ;
#140173=CARTESIAN_POINT('Ctrl Pts',(-15.536389802078,14.324111265305,132.381830675133)) ;
#140174=CARTESIAN_POINT('Ctrl Pts',(-15.6086735020593,14.4138215777412,
132.625972723014)) ;
#140175=CARTESIAN_POINT('Ctrl Pts',(-15.6861367295395,14.4331945078177,
132.88543907852)) ;
#140176=CARTESIAN_POINT('Ctrl Pts',(-15.7618948329016,14.3801614828431,
133.13981815517)) ;
#140177=CARTESIAN_POINT('Ctrl Pts',(-15.8301942788936,14.2584942969663,
133.3724909289)) ;
#140178=CARTESIAN_POINT('Ctrl Pts',(-15.8851640878315,14.0770491987957,
133.566189678613)) ;
#140179=CARTESIAN_POINT('Ctrl Pts',(-15.922273133789,13.848487543227,133.707756230679)) ;
#140180=CARTESIAN_POINT('Ctrl Pts',(-15.9379802552091,13.5893550911286,
133.786801390738)) ;
#140181=CARTESIAN_POINT('Ctrl Pts',(-15.9306077589097,13.3196922711331,
133.798256276605)) ;
#140182=CARTESIAN_POINT('Ctrl Pts',(-15.8998800307797,13.0561134153821,
133.74164886771)) ;
#140183=CARTESIAN_POINT('Ctrl Pts',(-15.8472473398955,12.8190741584449,
133.621021676602)) ;
#140184=CARTESIAN_POINT('Ctrl Pts',(-15.7757708334939,12.6252976289265,
133.445352087381)) ;
#140185=CARTESIAN_POINT('Ctrl Pts',(-15.689927661777,12.4887797079064,133.22768214269)) ;
#140186=CARTESIAN_POINT('Ctrl Pts',(-15.594962990031,12.4190606508798,132.983404336267)) ;
#140187=CARTESIAN_POINT('Ctrl Pts',(-15.4971275089631,12.4213023279721,
132.730711688481)) ;
#140188=CARTESIAN_POINT('Ctrl Pts',(-15.4025332987901,12.4953372291496,
132.487520232972)) ;
#140189=CARTESIAN_POINT('Ctrl Pts',(-15.3173685878029,12.6358732815743,
132.271860695447)) ;
#140190=CARTESIAN_POINT('Ctrl Pts',(-15.2470295349631,12.8325869424309,
132.099478396863)) ;
#140191=CARTESIAN_POINT('Ctrl Pts',(-15.1956790187667,13.0715962372375,
131.982579048758)) ;
#140192=CARTESIAN_POINT('Ctrl Pts',(-15.1663012050405,13.3366928582969,
131.929977593975)) ;
#140193=CARTESIAN_POINT('Ctrl Pts',(-15.1604318239741,13.6067853722367,
131.945897366208)) ;
#140194=CARTESIAN_POINT('Ctrl Pts',(-15.1775882934779,13.8640946743987,
132.029130404731)) ;
#140195=CARTESIAN_POINT('Ctrl Pts',(-15.2158372279991,14.0898397345162,
132.173966228249)) ;
#140196=CARTESIAN_POINT('Ctrl Pts',(-15.2720097039108,14.268360163449,132.371295347158)) ;
#140197=CARTESIAN_POINT('Ctrl Pts',(-15.3406803590063,14.3854877174078,
132.60491187324)) ;
#140198=CARTESIAN_POINT('Ctrl Pts',(-15.4171753630051,14.4341894579408,
132.861648085869)) ;
#140199=CARTESIAN_POINT('Ctrl Pts',(-15.4941067151991,14.4102459856392,
133.119375356917)) ;
#140200=CARTESIAN_POINT('Ctrl Pts',(-15.5662114944303,14.3157190540823,
133.363158093056)) ;
#140201=CARTESIAN_POINT('Ctrl Pts',(-15.6271436805455,14.1574302983803,
133.57424107157)) ;
#140202=CARTESIAN_POINT('Ctrl Pts',(-15.6720895670541,13.9458829104796,
133.738742203992)) ;
#140203=CARTESIAN_POINT('Ctrl Pts',(-15.6967873055417,13.6969896287775,
133.844047527021)) ;
#140204=CARTESIAN_POINT('Ctrl Pts',(-15.698845751887,13.429280378355,133.883124165852)) ;
#140205=CARTESIAN_POINT('Ctrl Pts',(-15.6776431235188,13.1613091049485,
133.8542162852)) ;
#140206=CARTESIAN_POINT('Ctrl Pts',(-15.6332316360466,12.9096301880815,
133.757855277709)) ;
#140207=CARTESIAN_POINT('Ctrl Pts',(-15.5691974920527,12.6977069165648,
133.603749145118)) ;
#140208=CARTESIAN_POINT('Ctrl Pts',(-15.488381414163,12.5361591796786,133.400861291253)) ;
#140209=CARTESIAN_POINT('Ctrl Pts',(-15.3965620792199,12.4388403136538,
133.165691149699)) ;
#140210=CARTESIAN_POINT('Ctrl Pts',(-15.2992076265801,12.4115721831835,
132.914391980506)) ;
#140211=CARTESIAN_POINT('Ctrl Pts',(-15.2023640564988,12.457029412505,132.664680437339)) ;
#140212=CARTESIAN_POINT('Ctrl Pts',(-15.1129280472859,12.5713337507617,
132.436462007858)) ;
#140213=CARTESIAN_POINT('Ctrl Pts',(-15.0358830275159,12.7468028515201,
132.244532777634)) ;
#140214=CARTESIAN_POINT('Ctrl Pts',(-14.9762423377458,12.9715572990884,
132.103535866445)) ;
#140215=CARTESIAN_POINT('Ctrl Pts',(-14.937881335131,13.2272671330663,132.024507485665)) ;
#140216=CARTESIAN_POINT('Ctrl Pts',(-14.9224295050719,13.498061880378,132.012548209648)) ;
#140217=CARTESIAN_POINT('Ctrl Pts',(-14.9303375882874,13.762097452862,132.068641628803)) ;
#140218=CARTESIAN_POINT('Ctrl Pts',(-14.9605151825436,14.0037249073099,
132.190050967125)) ;
#140219=CARTESIAN_POINT('Ctrl Pts',(-15.0097098440868,14.2024000350369,
132.366798183917)) ;
#140220=CARTESIAN_POINT('Ctrl Pts',(-15.0743428095158,14.3463072876563,
132.588901099298)) ;
#140221=CARTESIAN_POINT('Ctrl Pts',(-15.1479112672098,14.4229407115658,
132.836760336969)) ;
#140222=CARTESIAN_POINT('Ctrl Pts',(-15.2255189338972,14.428708721228,133.096623695493)) ;
#140223=CARTESIAN_POINT('Ctrl Pts',(-15.3003705645565,14.3623691718519,
133.348383670699)) ;
#140224=CARTESIAN_POINT('Ctrl Pts',(-15.3667024411799,14.2283779712588,
133.575366531252)) ;
#140225=CARTESIAN_POINT('Ctrl Pts',(-15.4186463452488,14.036425640657,133.760290224072)) ;
#140226=CARTESIAN_POINT('Ctrl Pts',(-15.4517469895417,13.8020944878478,
133.889958365334)) ;
#140227=CARTESIAN_POINT('Ctrl Pts',(-15.463285244604,13.539161382227,133.956849228233)) ;
#140228=CARTESIAN_POINT('Ctrl Pts',(-15.4514613937325,13.2686186839106,
133.955394191152)) ;
#140229=CARTESIAN_POINT('Ctrl Pts',(-15.4163784741773,13.008641923509,133.886067414322)) ;
#140230=CARTESIAN_POINT('Ctrl Pts',(-15.3601157103994,12.7791080577395,
133.754740538015)) ;
#140231=CARTESIAN_POINT('Ctrl Pts',(-15.2851636273898,12.594297732826,133.569082969986)) ;
#140232=CARTESIAN_POINT('Ctrl Pts',(-15.1973894002634,12.4702970553751,
133.34567823782)) ;
#140233=CARTESIAN_POINT('Ctrl Pts',(-15.1013148538407,12.4139049863059,
133.098187796925)) ;
#140234=CARTESIAN_POINT('Ctrl Pts',(-15.0038337445877,12.4297924309748,
132.846458188587)) ;
#140235=CARTESIAN_POINT('Ctrl Pts',(-14.9102271599336,12.5172147404821,
132.606269401608)) ;
#140236=CARTESIAN_POINT('Ctrl Pts',(-14.8274849504,12.6696685741938,132.397703669352)) ;
#140237=CARTESIAN_POINT('Ctrl Pts',(-14.7606686055306,12.8748935986054,
132.235504695728)) ;
#140238=CARTESIAN_POINT('Ctrl Pts',(-14.713205274637,13.1206629289391,132.130043070784)) ;
#140239=CARTESIAN_POINT('Ctrl Pts',(-14.6882892081952,13.3874986938653,
132.090357347663)) ;
#140240=CARTESIAN_POINT('Ctrl Pts',(-14.6868278663472,13.6577700467963,
132.119301620178)) ;
#140241=CARTESIAN_POINT('Ctrl Pts',(-14.7082723715754,13.9102263569756,
132.215043319294)) ;
#140242=CARTESIAN_POINT('Ctrl Pts',(-14.7500205778049,14.1273421335156,
132.369988376134)) ;
#140243=CARTESIAN_POINT('Ctrl Pts',(-14.8090332618092,14.2954362023137,
132.575628202352)) ;
#140244=CARTESIAN_POINT('Ctrl Pts',(-14.8796314850833,14.4001990478318,
132.8149219263)) ;
#140245=CARTESIAN_POINT('Ctrl Pts',(-14.9567452239667,14.4351706372086,
133.073434822023)) ;
#140246=CARTESIAN_POINT('Ctrl Pts',(-15.0330845819348,14.3977719556556,
133.329394582239)) ;
#140247=CARTESIAN_POINT('Ctrl Pts',(-15.1036711595281,14.2904204336126,
133.568797663084)) ;
#140248=CARTESIAN_POINT('Ctrl Pts',(-15.1620320097608,14.1205426251184,
133.772463469909)) ;
#140249=CARTESIAN_POINT('Ctrl Pts',(-15.2031898781849,13.9015880320261,
133.925742184152)) ;
#140250=CARTESIAN_POINT('Ctrl Pts',(-15.2238271094252,13.6483197654843,
134.019106406211)) ;
#140251=CARTESIAN_POINT('Ctrl Pts',(-15.2215120354708,13.3774460111694,
134.045600707171)) ;
#140252=CARTESIAN_POINT('Ctrl Pts',(-15.1957603044427,13.1115164178379,
134.003421898838)) ;
#140253=CARTESIAN_POINT('Ctrl Pts',(-15.1477813157542,12.8676277530858,
133.896336050308)) ;
#140254=CARTESIAN_POINT('Ctrl Pts',(-15.0801084681596,12.6630941709717,
133.731769988801)) ;
#140255=CARTESIAN_POINT('Ctrl Pts',(-14.9967542423809,12.5128296668561,
133.521456097352)) ;
#140256=CARTESIAN_POINT('Ctrl Pts',(-14.9032261050874,12.4280522223888,
133.281375642958)) ;
#140257=CARTESIAN_POINT('Ctrl Pts',(-14.8053449711548,12.4147676725694,
133.028604017027)) ;
#140258=CARTESIAN_POINT('Ctrl Pts',(-14.7098996424149,12.4732052197203,
132.782781794289)) ;
#140259=CARTESIAN_POINT('Ctrl Pts',(-14.6217034426985,12.6008830294735,
132.558469618926)) ;
#140260=CARTESIAN_POINT('Ctrl Pts',(-14.5481248406048,12.7859100383565,
132.376484190379)) ;
#140261=CARTESIAN_POINT('Ctrl Pts',(-14.4923378930718,13.0171549996097,
132.246636772306)) ;
#140262=CARTESIAN_POINT('Ctrl Pts',(-14.4580689419293,13.277402414091,132.179626600512)) ;
#140263=CARTESIAN_POINT('Ctrl Pts',(-14.4470325556808,13.549209197848,132.180627324106)) ;
#140264=CARTESIAN_POINT('Ctrl Pts',(-14.4593185955846,13.8101282641669,
132.249527993347)) ;
#140265=CARTESIAN_POINT('Ctrl Pts',(-14.4931674421932,14.0442616351561,
132.381507611934)) ;
#140266=CARTESIAN_POINT('Ctrl Pts',(-14.54604721898,14.234899690822,132.569317012515)) ;
#140267=CARTESIAN_POINT('Ctrl Pts',(-14.6122274527619,14.3654882849947,
132.795571754127)) ;
#140268=CARTESIAN_POINT('Ctrl Pts',(-14.6874535549381,14.4297229165876,
133.048520613647)) ;
#140269=CARTESIAN_POINT('Ctrl Pts',(-14.7648483414879,14.4216680213317,
133.307667405615)) ;
#140270=CARTESIAN_POINT('Ctrl Pts',(-14.8388106024003,14.3417421219821,
133.556976424616)) ;
#140271=CARTESIAN_POINT('Ctrl Pts',(-14.902525642574,14.1964291634702,133.776164127113)) ;
#140272=CARTESIAN_POINT('Ctrl Pts',(-14.9512314007499,13.9955519017587,
133.951576930874)) ;
#140273=CARTESIAN_POINT('Ctrl Pts',(-14.9805749680013,13.7541464807844,
134.070361816232)) ;
#140274=CARTESIAN_POINT('Ctrl Pts',(-14.9877159121976,13.4873870948836,
134.124497966682)) ;
#140275=CARTESIAN_POINT('Ctrl Pts',(-14.971521850687,13.2187119173844,134.110122717758)) ;
#140276=CARTESIAN_POINT('Ctrl Pts',(-14.9321810397444,12.9622340564561,
134.028441205295)) ;
#140277=CARTESIAN_POINT('Ctrl Pts',(-14.8719267297993,12.7396655137431,
133.885562044107)) ;
#140278=CARTESIAN_POINT('Ctrl Pts',(-14.7944437126708,12.5663130240366,
133.692322304437)) ;
#140279=CARTESIAN_POINT('Ctrl Pts',(-14.7047726635642,12.4542929808878,
133.463380163604)) ;
#140280=CARTESIAN_POINT('Ctrl Pts',(-14.607476851049,12.4113060989113,133.212457918896)) ;
#140281=CARTESIAN_POINT('Ctrl Pts',(-14.5106107325521,12.4409729751149,
132.962445001237)) ;
#140282=CARTESIAN_POINT('Ctrl Pts',(-14.4188178488728,12.5408195806537,
132.727450611251)) ;
#140283=CARTESIAN_POINT('Ctrl Pts',(-14.3384318561653,12.7045177195062,
132.525834912788)) ;
#140284=CARTESIAN_POINT('Ctrl Pts',(-14.2748650497426,12.9194126835292,
132.373269861623)) ;
#140285=CARTESIAN_POINT('Ctrl Pts',(-14.2317360390318,13.1689179450109,
132.280236038816)) ;
#140286=CARTESIAN_POINT('Ctrl Pts',(-14.2110498195284,13.4397285799231,
132.253160998047)) ;
#140287=CARTESIAN_POINT('Ctrl Pts',(-14.2140521881657,13.706427055275,132.294912707361)) ;
#140288=CARTESIAN_POINT('Ctrl Pts',(-14.2394774806085,13.953886295735,132.4023018521)) ;
#140289=CARTESIAN_POINT('Ctrl Pts',(-14.2847952393077,14.1631927592464,
132.567747077305)) ;
#140290=CARTESIAN_POINT('Ctrl Pts',(-14.3466522303324,14.3205261176051,
132.78177833072)) ;
#140291=CARTESIAN_POINT('Ctrl Pts',(-14.4186082729192,14.4121066452954,
133.024918177311)) ;
#140292=CARTESIAN_POINT('Ctrl Pts',(-14.4960761061432,14.4337042741575,
133.284423262461)) ;
#140293=CARTESIAN_POINT('Ctrl Pts',(-14.572045561504,14.3826278175705,133.539455649795)) ;
#140294=CARTESIAN_POINT('Ctrl Pts',(-14.6406034509692,14.2628852550259,
133.772863254736)) ;
#140295=CARTESIAN_POINT('Ctrl Pts',(-14.6960408758465,14.08292617671,133.967940627217)) ;
#140296=CARTESIAN_POINT('Ctrl Pts',(-14.7336909350444,13.8556922014923,
134.111058160493)) ;
#140297=CARTESIAN_POINT('Ctrl Pts',(-14.7500422659047,13.597259905774,134.191980102552)) ;
#140298=CARTESIAN_POINT('Ctrl Pts',(-14.7434335291913,13.3277679144463,
134.205648606387)) ;
#140299=CARTESIAN_POINT('Ctrl Pts',(-14.7130192503405,13.0618109735796,
134.150210773176)) ;
#140300=CARTESIAN_POINT('Ctrl Pts',(-14.6614036916594,12.826038953014,134.032246423453)) ;
#140301=CARTESIAN_POINT('Ctrl Pts',(-14.5901948939726,12.6298696524396,
133.857494505776)) ;
#140302=CARTESIAN_POINT('Ctrl Pts',(-14.5047155345941,12.4917687507878,
133.640863731031)) ;
#140303=CARTESIAN_POINT('Ctrl Pts',(-14.4098125153078,12.4199839299598,
133.39680729441)) ;
#140304=CARTESIAN_POINT('Ctrl Pts',(-14.3120256758759,12.4203084245316,
133.144238680783)) ;
#140305=CARTESIAN_POINT('Ctrl Pts',(-14.2174033458745,12.4922084684858,
132.900911571252)) ;
#140306=CARTESIAN_POINT('Ctrl Pts',(-14.1318404468406,12.6309969485081,
132.684106674944)) ;
#140307=CARTESIAN_POINT('Ctrl Pts',(-14.060980194024,12.8263311670906,132.510212790672)) ;
#140308=CARTESIAN_POINT('Ctrl Pts',(-14.0089205509473,13.0651228622206,
132.391338918913)) ;
#140309=CARTESIAN_POINT('Ctrl Pts',(-13.9790169020332,13.3295668395412,
132.337169347488)) ;
#140310=CARTESIAN_POINT('Ctrl Pts',(-13.9724839583839,13.5989124476963,
132.351047713643)) ;
#140311=CARTESIAN_POINT('Ctrl Pts',(-13.9890431321451,13.8574711293399,
132.432615710829)) ;
#140312=CARTESIAN_POINT('Ctrl Pts',(-14.0266628835637,14.0837079504238,
132.575528226051)) ;
#140313=CARTESIAN_POINT('Ctrl Pts',(-14.0822847624689,14.2638192247761,
132.77121833331)) ;
#140314=CARTESIAN_POINT('Ctrl Pts',(-14.1508947644669,14.3831695883009,
133.004767867683)) ;
#140315=CARTESIAN_POINT('Ctrl Pts',(-14.2270177030481,14.4337176696405,
133.260307152951)) ;
#140316=CARTESIAN_POINT('Ctrl Pts',(-14.3040474224697,14.4120588650256,
133.518338090565)) ;
#140317=CARTESIAN_POINT('Ctrl Pts',(-14.376474347551,14.3193772960994,133.763103381234)) ;
#140318=CARTESIAN_POINT('Ctrl Pts',(-14.4378412105215,14.162817091715,133.975462148985)) ;
#140319=CARTESIAN_POINT('Ctrl Pts',(-14.4833931112873,13.9515916217657,
134.141862753533)) ;
#140320=CARTESIAN_POINT('Ctrl Pts',(-14.5085472628772,13.7055233203187,
134.248235176747)) ;
#140321=CARTESIAN_POINT('Ctrl Pts',(-14.5113140037808,13.4359481909895,
134.289656318574)) ;
#140322=CARTESIAN_POINT('Ctrl Pts',(-14.4907836142237,13.1690262543573,
134.262549097928)) ;
#140323=CARTESIAN_POINT('Ctrl Pts',(-14.4469946766069,12.9162728223831,
134.168041991638)) ;
#140324=CARTESIAN_POINT('Ctrl Pts',(-14.3836515410097,12.7036779666449,
134.015865151141)) ;
#140325=CARTESIAN_POINT('Ctrl Pts',(-14.3034207076497,12.5403117621087,
133.814645347195)) ;
#140326=CARTESIAN_POINT('Ctrl Pts',(-14.2112317925761,12.4404489575973,
133.578615475842)) ;
#140327=CARTESIAN_POINT('Ctrl Pts',(-14.1144092292276,12.4114485633587,
133.328709169712)) ;
#140328=CARTESIAN_POINT('Ctrl Pts',(-14.0175084056,12.4544846403687,133.078809925647)) ;
#140329=CARTESIAN_POINT('Ctrl Pts',(-13.9274154196742,12.5672617699685,
132.84879938857)) ;
#140330=CARTESIAN_POINT('Ctrl Pts',(-13.8498913580063,12.7417744927464,
132.655533038876)) ;
#140331=CARTESIAN_POINT('Ctrl Pts',(-13.7901365880796,12.9633750836739,
132.513923783402)) ;
#140332=CARTESIAN_POINT('Ctrl Pts',(-13.7507723014847,13.2203111794704,
132.432225066762)) ;
#140333=CARTESIAN_POINT('Ctrl Pts',(-13.7347687491892,13.4905143785451,
132.418587863191)) ;
#140334=CARTESIAN_POINT('Ctrl Pts',(-13.7420428608409,13.7550216610133,
132.472844845919)) ;
#140335=CARTESIAN_POINT('Ctrl Pts',(-13.7714788185508,13.996749630301,132.591960053501)) ;
#140336=CARTESIAN_POINT('Ctrl Pts',(-13.8202931282288,14.1974242710986,
132.767691700884)) ;
#140337=CARTESIAN_POINT('Ctrl Pts',(-13.8842419043715,14.342514003419,132.987636729813)) ;
#140338=CARTESIAN_POINT('Ctrl Pts',(-13.957804359372,14.4218015954934,133.235581296981)) ;
#140339=CARTESIAN_POINT('Ctrl Pts',(-14.0357822793224,14.4294553492896,
133.496688274969)) ;
#140340=CARTESIAN_POINT('Ctrl Pts',(-14.1104232002843,14.3652618267525,
133.747675313763)) ;
#140341=CARTESIAN_POINT('Ctrl Pts',(-14.1770034660584,14.2335996642439,
133.975322494504)) ;
#140342=CARTESIAN_POINT('Ctrl Pts',(-14.2295331975556,14.0430658671341,
134.161995180824)) ;
#140343=CARTESIAN_POINT('Ctrl Pts',(-14.263333326228,13.8093138339715,134.293777182255)) ;
#140344=CARTESIAN_POINT('Ctrl Pts',(-14.2754798550196,13.5459139250659,
134.362562631417)) ;
#140345=CARTESIAN_POINT('Ctrl Pts',(-14.2643602113247,13.2769103570782,
134.362972904705)) ;
#140346=CARTESIAN_POINT('Ctrl Pts',(-14.2299858105317,13.0160046226691,
134.295749756055)) ;
#140347=CARTESIAN_POINT('Ctrl Pts',(-14.1741543649749,12.7850161242088,
134.165746233419)) ;
#140348=CARTESIAN_POINT('Ctrl Pts',(-14.0999513367095,12.5991696001074,
133.982162522111)) ;
#140349=CARTESIAN_POINT('Ctrl Pts',(-14.0120333686313,12.4727066695535,
133.758511658872)) ;
#140350=CARTESIAN_POINT('Ctrl Pts',(-13.9165608240464,12.4146340063818,
133.512615786361)) ;
#140351=CARTESIAN_POINT('Ctrl Pts',(-13.8188267136632,12.428272476576,133.260222062798)) ;
#140352=CARTESIAN_POINT('Ctrl Pts',(-13.725121388422,12.5136822248399,133.019706177829)) ;
#140353=CARTESIAN_POINT('Ctrl Pts',(-13.6420048655474,12.6640313971838,
132.810020108338)) ;
#140354=CARTESIAN_POINT('Ctrl Pts',(-13.5742807570679,12.8694014453016,
132.645391514411)) ;
#140355=CARTESIAN_POINT('Ctrl Pts',(-13.5265676033014,13.1128473541502,
132.538991019669)) ;
#140356=CARTESIAN_POINT('Ctrl Pts',(-13.5008984856995,13.3794713860966,
132.497132690037)) ;
#140357=CARTESIAN_POINT('Ctrl Pts',(-13.498756156776,13.6493875676937,132.524020269698)) ;
#140358=CARTESIAN_POINT('Ctrl Pts',(-13.5194308106777,13.9027716863457,
132.617509983294)) ;
#140359=CARTESIAN_POINT('Ctrl Pts',(-13.5610331702241,14.1226003969304,
132.772288082141)) ;
#140360=CARTESIAN_POINT('Ctrl Pts',(-13.6190505001098,14.2907614924808,
132.974692661995)) ;
#140361=CARTESIAN_POINT('Ctrl Pts',(-13.6900034594533,14.3985142703266,
133.215330636002)) ;
#140362=CARTESIAN_POINT('Ctrl Pts',(-13.766526148139,14.4350393250072,133.471887799925)) ;
#140363=CARTESIAN_POINT('Ctrl Pts',(-13.8431005378829,14.4000355933247,
133.728594097503)) ;
#140364=CARTESIAN_POINT('Ctrl Pts',(-13.9141839403901,14.294019258596,133.969566022421)) ;
#140365=CARTESIAN_POINT('Ctrl Pts',(-13.9726902525623,14.1264036808229,
134.173517618549)) ;
#140366=CARTESIAN_POINT('Ctrl Pts',(-14.01451107899,13.9087136081249,134.328754222631)) ;
#140367=CARTESIAN_POINT('Ctrl Pts',(-14.0358023095098,13.6545233409047,
134.42423188298)) ;
#140368=CARTESIAN_POINT('Ctrl Pts',(-14.03411729603,13.3858501132774,134.452316017563)) ;
#140369=CARTESIAN_POINT('Ctrl Pts',(-14.0090696513313,13.1190055325829,
134.412261309148)) ;
#140370=CARTESIAN_POINT('Ctrl Pts',(-13.9616116706279,12.8738785417747,
134.30674275505)) ;
#140371=CARTESIAN_POINT('Ctrl Pts',(-13.8942434743611,12.6676053740016,
134.14314714961)) ;
#140372=CARTESIAN_POINT('Ctrl Pts',(-13.8113184980164,12.5160771056389,
133.934042303186)) ;
#140373=CARTESIAN_POINT('Ctrl Pts',(-13.7184439168081,12.4297444721253,
133.695718949214)) ;
#140374=CARTESIAN_POINT('Ctrl Pts',(-13.6207083074889,12.4139325819383,
133.443334307576)) ;
#140375=CARTESIAN_POINT('Ctrl Pts',(-13.5245613685599,12.4708186398046,
133.195662451093)) ;
#140376=CARTESIAN_POINT('Ctrl Pts',(-13.4367983720263,12.5954481483175,
132.972323924776)) ;
#140377=CARTESIAN_POINT('Ctrl Pts',(-13.3622573334654,12.7795463119932,
132.787704186982)) ;
#140378=CARTESIAN_POINT('Ctrl Pts',(-13.3057627898852,13.0105018776207,
132.655886775255)) ;
#140379=CARTESIAN_POINT('Ctrl Pts',(-13.2708885411926,13.270465957133,132.587139289259)) ;
#140380=CARTESIAN_POINT('Ctrl Pts',(-13.2592549111302,13.5415025070648,
132.586306674461)) ;
#140381=CARTESIAN_POINT('Ctrl Pts',(-13.2708395234052,13.8030870082756,
132.653165528328)) ;
#140382=CARTESIAN_POINT('Ctrl Pts',(-13.304367480166,14.0389747692379,132.784348177691)) ;
#140383=CARTESIAN_POINT('Ctrl Pts',(-13.3561244599786,14.2290324339817,
132.968488370536)) ;
#140384=CARTESIAN_POINT('Ctrl Pts',(-13.4224801597023,14.36290013857,133.195546796567)) ;
#140385=CARTESIAN_POINT('Ctrl Pts',(-13.4974004709148,14.4288302738408,
133.447521013397)) ;
#140386=CARTESIAN_POINT('Ctrl Pts',(-13.5749660998,14.4228365201876,133.707240841845)) ;
#140387=CARTESIAN_POINT('Ctrl Pts',(-13.6488630271482,14.3452102352826,
133.956235673057)) ;
#140388=CARTESIAN_POINT('Ctrl Pts',(-13.7131159667098,14.2014203196955,
134.177078915254)) ;
#140389=CARTESIAN_POINT('Ctrl Pts',(-13.7622546708898,14.0021641937243,
134.353713580636)) ;
#140390=CARTESIAN_POINT('Ctrl Pts',(-13.7922217713026,13.761753127779,134.474321990283)) ;
#140391=CARTESIAN_POINT('Ctrl Pts',(-13.8000681557409,13.4956080237515,
134.530495262172)) ;
#140392=CARTESIAN_POINT('Ctrl Pts',(-13.7845110824094,13.2262845852455,
134.518046664834)) ;
#140393=CARTESIAN_POINT('Ctrl Pts',(-13.7459650817114,12.9698876950621,
134.438579717807)) ;
#140394=CARTESIAN_POINT('Ctrl Pts',(-13.6862141444836,12.7457364087332,
134.297226076074)) ;
#140395=CARTESIAN_POINT('Ctrl Pts',(-13.6093646492958,12.5708017503329,
134.105774071566)) ;
#140396=CARTESIAN_POINT('Ctrl Pts',(-13.519124823432,12.4561497112336,133.875476397484)) ;
#140397=CARTESIAN_POINT('Ctrl Pts',(-13.422988713799,12.4116404870858,133.62757363074)) ;
#140398=CARTESIAN_POINT('Ctrl Pts',(-13.3252747688584,12.4391729336107,
133.375352092848)) ;
#140399=CARTESIAN_POINT('Ctrl Pts',(-13.2335160894411,12.5371797633224,
133.140365473548)) ;
#140400=CARTESIAN_POINT('Ctrl Pts',(-13.1529574964824,12.6985743471033,
132.938147247073)) ;
#140401=CARTESIAN_POINT('Ctrl Pts',(-13.0887851662366,12.9117741360547,
132.783784142342)) ;
#140402=CARTESIAN_POINT('Ctrl Pts',(-13.0447718180386,13.1624013152274,
132.688415632104)) ;
#140403=CARTESIAN_POINT('Ctrl Pts',(-13.0236022557923,13.4305279145417,
132.659623972586)) ;
#140404=CARTESIAN_POINT('Ctrl Pts',(-13.0258219823811,13.6988963516455,
132.699258391825)) ;
#140405=CARTESIAN_POINT('Ctrl Pts',(-13.0506572284253,13.9472005386101,
132.804920173535)) ;
#140406=CARTESIAN_POINT('Ctrl Pts',(-13.0955424206449,14.1580510630495,
132.969155849435)) ;
#140407=CARTESIAN_POINT('Ctrl Pts',(-13.1567221725549,14.3165352363587,
133.181063812817)) ;
#140408=CARTESIAN_POINT('Ctrl Pts',(-13.228807081375,14.4105996668628,133.424752925939)) ;
#140409=CARTESIAN_POINT('Ctrl Pts',(-13.306007393883,14.4340684651961,133.683379684526)) ;
#140410=CARTESIAN_POINT('Ctrl Pts',(-13.382228905179,14.3850543896185,133.939203970425)) ;
#140411=CARTESIAN_POINT('Ctrl Pts',(-13.4510738585261,14.2669952300402,
134.173456810545)) ;
#140412=CARTESIAN_POINT('Ctrl Pts',(-13.506810496423,14.0891154364107,134.369318142891)) ;
#140413=CARTESIAN_POINT('Ctrl Pts',(-13.5451041794166,13.8629228835357,
134.5143452011)) ;
#140414=CARTESIAN_POINT('Ctrl Pts',(-13.5621329454697,13.6044943724102,
134.597322473916)) ;
#140415=CARTESIAN_POINT('Ctrl Pts',(-13.5560956962621,13.3352195562946,
134.612648137411)) ;
#140416=CARTESIAN_POINT('Ctrl Pts',(-13.5266617961689,13.0705829535361,
134.559838132771)) ;
#140417=CARTESIAN_POINT('Ctrl Pts',(-13.475276995217,12.8316692334543,134.44283011763)) ;
#140418=CARTESIAN_POINT('Ctrl Pts',(-13.4044073000562,12.6342706260099,
134.26908401501)) ;
#140419=CARTESIAN_POINT('Ctrl Pts',(-13.3195945751411,12.4949548036794,
134.05427628367)) ;
#140420=CARTESIAN_POINT('Ctrl Pts',(-13.2248596249454,12.4210676160077,
133.810718608612)) ;
#140421=CARTESIAN_POINT('Ctrl Pts',(-13.1271993154374,12.4192534817676,
133.558478104923)) ;
#140422=CARTESIAN_POINT('Ctrl Pts',(-13.0322252201144,12.4890551014873,
133.314175173155)) ;
#140423=CARTESIAN_POINT('Ctrl Pts',(-12.9459982367621,12.626926545497,133.095576978998)) ;
#140424=CARTESIAN_POINT('Ctrl Pts',(-12.8751217655022,12.8196495679067,
132.921424109731)) ;
#140425=CARTESIAN_POINT('Ctrl Pts',(-12.8222774142593,13.0580836243581,
132.800361858401)) ;
#140426=CARTESIAN_POINT('Ctrl Pts',(-12.7917934093607,13.3214662460235,
132.744416520862)) ;
#140427=CARTESIAN_POINT('Ctrl Pts',(-12.7845758914213,13.5912987745739,
132.756352051933)) ;
#140428=CARTESIAN_POINT('Ctrl Pts',(-12.8003737957129,13.8497219287496,
132.835584198493)) ;
#140429=CARTESIAN_POINT('Ctrl Pts',(-12.8377457211529,14.0789422598233,
132.978048098674)) ;
#140430=CARTESIAN_POINT('Ctrl Pts',(-12.8928878000828,14.2597601138698,
133.172246822458)) ;
#140431=CARTESIAN_POINT('Ctrl Pts',(-12.960949978305,14.3805241665643,133.404082488237)) ;
#140432=CARTESIAN_POINT('Ctrl Pts',(-13.036840414061,14.4333051065353,133.658899622232)) ;
#140433=CARTESIAN_POINT('Ctrl Pts',(-13.1142347421023,14.4135763153339,
133.91813556721)) ;
#140434=CARTESIAN_POINT('Ctrl Pts',(-13.1867830255326,14.3230159864486,
134.163193889297)) ;
#140435=CARTESIAN_POINT('Ctrl Pts',(-13.2487470576845,14.1669880697449,
134.377473831657)) ;
#140436=CARTESIAN_POINT('Ctrl Pts',(-13.2942601671939,13.9601855092309,
134.543287341378)) ;
#140437=CARTESIAN_POINT('Ctrl Pts',(-13.3203995351673,13.7121979724763,
134.652938896133)) ;
#140438=CARTESIAN_POINT('Ctrl Pts',(-13.3238270184238,13.4453254354835,
134.695977657837)) ;
#140439=CARTESIAN_POINT('Ctrl Pts',(-13.3037973870205,13.1756579328103,
134.670656958844)) ;
#140440=CARTESIAN_POINT('Ctrl Pts',(-13.2611344959684,12.9248371133689,
134.579064456657)) ;
#140441=CARTESIAN_POINT('Ctrl Pts',(-13.1978850472197,12.7087904209721,
134.427462742701)) ;
#140442=CARTESIAN_POINT('Ctrl Pts',(-13.1180880272232,12.5441839973877,
134.227467431422)) ;
#140443=CARTESIAN_POINT('Ctrl Pts',(-13.0261903296275,12.4422953631874,
133.992282641388)) ;
#140444=CARTESIAN_POINT('Ctrl Pts',(-12.9292309041857,12.4112745922159,
133.742044880422)) ;
#140445=CARTESIAN_POINT('Ctrl Pts',(-12.8324220446461,12.4523611240387,
133.492352590847)) ;
#140446=CARTESIAN_POINT('Ctrl Pts',(-12.7422827853316,12.5627156272335,
133.262109881724)) ;
#140447=CARTESIAN_POINT('Ctrl Pts',(-12.6640304336884,12.7362032335438,
133.066838486923)) ;
#140448=CARTESIAN_POINT('Ctrl Pts',(-12.6038457715157,12.9562237014372,
132.923907669484)) ;
#140449=CARTESIAN_POINT('Ctrl Pts',(-12.5638033798923,13.2127632436766,
132.840271448791)) ;
#140450=CARTESIAN_POINT('Ctrl Pts',(-12.5471482690012,13.4814739931662,
132.824565254559)) ;
#140451=CARTESIAN_POINT('Ctrl Pts',(-12.55368247659,13.7476020769462,132.876805340507)) ;
#140452=CARTESIAN_POINT('Ctrl Pts',(-12.5826455210226,13.9907502707064,
132.99461409777)) ;
#140453=CARTESIAN_POINT('Ctrl Pts',(-12.6308355205781,14.1921268766281,
133.168425407229)) ;
#140454=CARTESIAN_POINT('Ctrl Pts',(-12.6943294952942,14.3392030436754,
133.387020626531)) ;
#140455=CARTESIAN_POINT('Ctrl Pts',(-12.7683012220631,14.4207500230976,
133.636423571384)) ;
#140456=CARTESIAN_POINT('Ctrl Pts',(-12.8455310116652,14.4302362583739,
133.895028948852)) ;
#140457=CARTESIAN_POINT('Ctrl Pts',(-12.9207429495786,14.368028270843,134.147861599825)) ;
#140458=CARTESIAN_POINT('Ctrl Pts',(-12.9877312267405,14.2375543492764,
134.376766361089)) ;
#140459=CARTESIAN_POINT('Ctrl Pts',(-13.040561290709,14.0487159657188,134.564249356536)) ;
#140460=CARTESIAN_POINT('Ctrl Pts',(-13.0748031716909,13.8167883871292,
134.697210227898)) ;
#140461=CARTESIAN_POINT('Ctrl Pts',(-13.0876734641736,13.5548284865375,
134.768007071369)) ;
#140462=CARTESIAN_POINT('Ctrl Pts',(-13.0772469786685,13.2844750332118,
134.770603967705)) ;
#140463=CARTESIAN_POINT('Ctrl Pts',(-13.0433961018683,13.0226683900031,
134.704959155467)) ;
#140464=CARTESIAN_POINT('Ctrl Pts',(-12.9882858427434,12.7913019843532,
134.57696772602)) ;
#140465=CARTESIAN_POINT('Ctrl Pts',(-12.9146582473163,12.6040507467942,
134.395030630286)) ;
#140466=CARTESIAN_POINT('Ctrl Pts',(-12.8271396558594,12.4756113935465,
134.172527392137)) ;
#140467=CARTESIAN_POINT('Ctrl Pts',(-12.7315130264268,12.415243488117,133.92628699965)) ;
#140468=CARTESIAN_POINT('Ctrl Pts',(-12.6338160664484,12.4269403743014,
133.673979806236)) ;
#140469=CARTESIAN_POINT('Ctrl Pts',(-12.5401199150452,12.5099953063745,
133.433406758865)) ;
#140470=CARTESIAN_POINT('Ctrl Pts',(-12.4565010249555,12.6587329054093,
133.222300982003)) ;
#140471=CARTESIAN_POINT('Ctrl Pts',(-12.3884365161738,12.8618952127667,
133.056565584079)) ;
#140472=CARTESIAN_POINT('Ctrl Pts',(-12.3398181635713,13.1054069861002,
132.94766934641)) ;
#140473=CARTESIAN_POINT('Ctrl Pts',(-12.3135058293376,13.3721987049067,
132.903992343846)) ;
#140474=CARTESIAN_POINT('Ctrl Pts',(-12.3107188025145,13.6415134162569,
132.928902598688)) ;
#140475=CARTESIAN_POINT('Ctrl Pts',(-12.3306845058955,13.8954057310282,
133.020287129816)) ;
#140476=CARTESIAN_POINT('Ctrl Pts',(-12.3717562411778,14.1169004710299,
133.173562993441)) ;
#140477=CARTESIAN_POINT('Ctrl Pts',(-12.4295072043719,14.2868623267828,
133.375258269535)) ;
#140478=CARTESIAN_POINT('Ctrl Pts',(-12.4997409250019,14.396013035847,133.613591802194)) ;
#140479=CARTESIAN_POINT('Ctrl Pts',(-12.5764706947144,14.4351149224746,
133.870891973931)) ;
#140480=CARTESIAN_POINT('Ctrl Pts',(-12.6532429349451,14.4019052027925,
134.128227117607)) ;
#140481=CARTESIAN_POINT('Ctrl Pts',(-12.7243502344129,14.2983009187854,
134.369151253832)) ;
#140482=CARTESIAN_POINT('Ctrl Pts',(-12.7835198481276,14.1317969224175,
134.575164716449)) ;
#140483=CARTESIAN_POINT('Ctrl Pts',(-12.8257831979134,13.91534337541,134.731670450177)) ;
#140484=CARTESIAN_POINT('Ctrl Pts',(-12.8476480318692,13.6633971728162,
134.828641412771)) ;
#140485=CARTESIAN_POINT('Ctrl Pts',(-12.8467867250038,13.3943409490525,
134.859209219661)) ;
#140486=CARTESIAN_POINT('Ctrl Pts',(-12.8222377970458,13.125759500651,134.820784175439)) ;
#140487=CARTESIAN_POINT('Ctrl Pts',(-12.7754966528095,12.8806964753524,
134.717244165718)) ;
#140488=CARTESIAN_POINT('Ctrl Pts',(-12.7088929602356,12.6734733763792,
134.555794010594)) ;
#140489=CARTESIAN_POINT('Ctrl Pts',(-12.626209768345,12.5195858185458,134.347470896474)) ;
#140490=CARTESIAN_POINT('Ctrl Pts',(-12.5330823146692,12.4310932740595,
134.108568204543)) ;
#140491=CARTESIAN_POINT('Ctrl Pts',(-12.4359002404825,12.4134132696985,
133.857624810028)) ;
#140492=CARTESIAN_POINT('Ctrl Pts',(-12.3394913697739,12.4681188633571,
133.609228819744)) ;
#140493=CARTESIAN_POINT('Ctrl Pts',(-12.2514122847404,12.5909169506631,
133.384966928797)) ;
#140494=CARTESIAN_POINT('Ctrl Pts',(-12.1764252467238,12.7734489072163,
133.199042308447)) ;
#140495=CARTESIAN_POINT('Ctrl Pts',(-12.1194045389883,13.0028154211787,
133.0656283448)) ;
#140496=CARTESIAN_POINT('Ctrl Pts',(-12.0838153267167,13.2626812904981,
132.994861198184)) ;
#140497=CARTESIAN_POINT('Ctrl Pts',(-12.0714655142961,13.5323091961428,
132.991764635821)) ;
#140498=CARTESIAN_POINT('Ctrl Pts',(-12.0824257373207,13.7963543423531,
133.057045713881)) ;
#140499=CARTESIAN_POINT('Ctrl Pts',(-12.1152947061301,14.0324258066149,
133.186186490251)) ;
#140500=CARTESIAN_POINT('Ctrl Pts',(-12.1666377019664,14.2243211732623,
133.369177652466)) ;
#140501=CARTESIAN_POINT('Ctrl Pts',(-12.232476473759,14.3597396975641,133.594637060158)) ;
#140502=CARTESIAN_POINT('Ctrl Pts',(-12.3074797976533,14.4280132150894,
133.846971383581)) ;
#140503=CARTESIAN_POINT('Ctrl Pts',(-12.3850141728136,14.4240026931505,
134.106576784609)) ;
#140504=CARTESIAN_POINT('Ctrl Pts',(-12.4591545841739,14.348214877112,134.356314139757)) ;
#140505=CARTESIAN_POINT('Ctrl Pts',(-12.5235535888618,14.2066839106137,
134.577474272231)) ;
#140506=CARTESIAN_POINT('Ctrl Pts',(-12.5733676119359,14.0084844644838,
134.756165192188)) ;
#140507=CARTESIAN_POINT('Ctrl Pts',(-12.6039525352688,13.76791632806,134.878710146275)) ;
#140508=CARTESIAN_POINT('Ctrl Pts',(-12.612364118678,13.5034893328133,134.936368413095)) ;
#140509=CARTESIAN_POINT('Ctrl Pts',(-12.5974803065642,13.2335994078643,
134.925943717301)) ;
#140510=CARTESIAN_POINT('Ctrl Pts',(-12.5595099792057,12.976407627843,134.84817680895)) ;
#140511=CARTESIAN_POINT('Ctrl Pts',(-12.5001716230381,12.7508792337382,
134.708077669362)) ;
#140512=CARTESIAN_POINT('Ctrl Pts',(-12.4240025586213,12.5752390532541,
134.518488422095)) ;
#140513=CARTESIAN_POINT('Ctrl Pts',(-12.3345444898954,12.4588914929926,
134.290312537568)) ;
#140514=CARTESIAN_POINT('Ctrl Pts',(-12.2379671531426,12.4118138328558,
134.041315824821)) ;
#140515=CARTESIAN_POINT('Ctrl Pts',(-12.1402200536129,12.4374481799832,
133.78898690417)) ;
#140516=CARTESIAN_POINT('Ctrl Pts',(-12.0482373710984,12.5333386552095,
133.553332360909)) ;
#140517=CARTESIAN_POINT('Ctrl Pts',(-11.9669627091784,12.6939674039094,
133.349171653341)) ;
#140518=CARTESIAN_POINT('Ctrl Pts',(-11.902619330109,12.9050031482846,133.194150919962)) ;
#140519=CARTESIAN_POINT('Ctrl Pts',(-11.857873910087,13.1551455919413,133.096696395566)) ;
#140520=CARTESIAN_POINT('Ctrl Pts',(-11.8433730930553,13.3338157805737,
133.076375626011)) ;
#140521=CARTESIAN_POINT('Ctrl Pts',(-11.83998730453,13.4231220893089,133.077505617122)) ;
#140522=CARTESIAN_POINT('Ctrl Pts',(-33.1829052539887,13.1734341962953,
127.851905049753)) ;
#140523=CARTESIAN_POINT('Ctrl Pts',(-33.1822017070797,13.1676985268958,
127.850580772544)) ;
#140524=CARTESIAN_POINT('Ctrl Pts',(-33.1707280433469,13.076204201721,127.828745770272)) ;
#140525=CARTESIAN_POINT('Ctrl Pts',(-33.1397508853579,12.9034784200084,
127.761228635573)) ;
#140526=CARTESIAN_POINT('Ctrl Pts',(-33.0750750970862,12.6923997924798,
127.605316905031)) ;
#140527=CARTESIAN_POINT('Ctrl Pts',(-32.9941099257864,12.5327609197045,
127.401903291373)) ;
#140528=CARTESIAN_POINT('Ctrl Pts',(-32.9014522171935,12.4368205686394,
127.16450033503)) ;
#140529=CARTESIAN_POINT('Ctrl Pts',(-32.8045123363909,12.4119420237697,
126.914243813896)) ;
#140530=CARTESIAN_POINT('Ctrl Pts',(-32.7076862120277,12.4592681498074,
126.664616426665)) ;
#140531=CARTESIAN_POINT('Ctrl Pts',(-32.6184092522946,12.575659036236,126.436908031571)) ;
#140532=CARTESIAN_POINT('Ctrl Pts',(-32.5418309193606,12.75283542717,126.246347133038)) ;
#140533=CARTESIAN_POINT('Ctrl Pts',(-32.4829016852876,12.9779971811105,
126.107323458936)) ;
#140534=CARTESIAN_POINT('Ctrl Pts',(-32.4450817095912,13.2349354675193,
126.029955963063)) ;
#140535=CARTESIAN_POINT('Ctrl Pts',(-32.4302650083729,13.5051819451432,
126.019763187868)) ;
#140536=CARTESIAN_POINT('Ctrl Pts',(-32.4389881142122,13.7710457079463,
126.078535238366)) ;
#140537=CARTESIAN_POINT('Ctrl Pts',(-32.4695784674888,14.0095406593372,
126.200858990596)) ;
#140538=CARTESIAN_POINT('Ctrl Pts',(-32.5193506356405,14.2073761046424,
126.379385142619)) ;
#140539=CARTESIAN_POINT('Ctrl Pts',(-32.5839721986,14.3489569855306,126.601275613991)) ;
#140540=CARTESIAN_POINT('Ctrl Pts',(-32.6582948498371,14.4243647659385,
126.851602957494)) ;
#140541=CARTESIAN_POINT('Ctrl Pts',(-32.735855999385,14.427672591071,127.111298260045)) ;
#140542=CARTESIAN_POINT('Ctrl Pts',(-32.8104552893985,14.3592845353793,
127.362291590965)) ;
#140543=CARTESIAN_POINT('Ctrl Pts',(-32.8762278669798,14.2239082001409,
127.587533236593)) ;
#140544=CARTESIAN_POINT('Ctrl Pts',(-32.927746682636,14.0309430574059,127.77118384942)) ;
#140545=CARTESIAN_POINT('Ctrl Pts',(-32.960457263088,13.7937231411456,127.899964110698)) ;
#140546=CARTESIAN_POINT('Ctrl Pts',(-32.9712029509523,13.5318368827659,
127.964333838362)) ;
#140547=CARTESIAN_POINT('Ctrl Pts',(-32.9587611170759,13.260908758679,127.961130078476)) ;
#140548=CARTESIAN_POINT('Ctrl Pts',(-32.9229367694298,13.0011530565724,
127.889686187424)) ;
#140549=CARTESIAN_POINT('Ctrl Pts',(-32.8660948183366,12.7729626729889,
127.756647910718)) ;
#140550=CARTESIAN_POINT('Ctrl Pts',(-32.790924635143,12.5901801237826,127.570254799383)) ;
#140551=CARTESIAN_POINT('Ctrl Pts',(-32.7027029653519,12.4676467713314,
127.345605003568)) ;
#140552=CARTESIAN_POINT('Ctrl Pts',(-32.6063037446173,12.413314501038,127.097226465731)) ;
#140553=CARTESIAN_POINT('Ctrl Pts',(-32.5089710404186,12.4313809059018,
126.845895281843)) ;
#140554=CARTESIAN_POINT('Ctrl Pts',(-32.4157240307319,12.5206603484656,
126.60670957826)) ;
#140555=CARTESIAN_POINT('Ctrl Pts',(-32.3334682191733,12.6744196148216,
126.399508808185)) ;
#140556=CARTESIAN_POINT('Ctrl Pts',(-32.2669019929393,12.8815893341258,
126.238150872134)) ;
#140557=CARTESIAN_POINT('Ctrl Pts',(-32.2200131818392,13.1290193456038,
126.134455135357)) ;
#140558=CARTESIAN_POINT('Ctrl Pts',(-32.1959308651233,13.3950772518204,
126.097064150513)) ;
#140559=CARTESIAN_POINT('Ctrl Pts',(-32.1950470896664,13.6643422142601,
126.127596808045)) ;
#140560=CARTESIAN_POINT('Ctrl Pts',(-32.2171232020604,13.9170737538833,
126.22530306428)) ;
#140561=CARTESIAN_POINT('Ctrl Pts',(-32.2596149976549,14.1334228161875,
126.38252083197)) ;
#140562=CARTESIAN_POINT('Ctrl Pts',(-32.3187058370602,14.2989215629879,
126.588198409019)) ;
#140563=CARTESIAN_POINT('Ctrl Pts',(-32.3896496930304,14.4021434472197,
126.828560375048)) ;
#140564=CARTESIAN_POINT('Ctrl Pts',(-32.4667661198528,14.4351203025954,
127.087043208967)) ;
#140565=CARTESIAN_POINT('Ctrl Pts',(-32.5432148615198,14.3956460282901,
127.343411947521)) ;
#140566=CARTESIAN_POINT('Ctrl Pts',(-32.6134644972313,14.2864256300776,
127.581799379627)) ;
#140567=CARTESIAN_POINT('Ctrl Pts',(-32.6713951718574,14.1149875929984,
127.784205127976)) ;
#140568=CARTESIAN_POINT('Ctrl Pts',(-32.7120127070859,13.8950778464839,
127.935876391714)) ;
#140569=CARTESIAN_POINT('Ctrl Pts',(-32.7320620935371,13.6402948775312,
128.027626314225)) ;
#140570=CARTESIAN_POINT('Ctrl Pts',(-32.7290666324127,13.3700134780419,
128.052035270306)) ;
#140571=CARTESIAN_POINT('Ctrl Pts',(-32.7026474802242,13.1040820089462,
128.007955758887)) ;
#140572=CARTESIAN_POINT('Ctrl Pts',(-32.6540267104507,12.8608603098162,
127.899019977621)) ;
#140573=CARTESIAN_POINT('Ctrl Pts',(-32.5854756864029,12.6570994974887,
127.732029152198)) ;
#140574=CARTESIAN_POINT('Ctrl Pts',(-32.5022717478729,12.509712563052,127.521931848437)) ;
#140575=CARTESIAN_POINT('Ctrl Pts',(-32.4084850460521,12.4266925565407,
127.281125909087)) ;
#140576=CARTESIAN_POINT('Ctrl Pts',(-32.310691262548,12.4153566228605,127.028564089873)) ;
#140577=CARTESIAN_POINT('Ctrl Pts',(-32.2150851456372,12.476118398497,126.782387345234)) ;
#140578=CARTESIAN_POINT('Ctrl Pts',(-32.127774202705,12.6046110942521,126.56043246527)) ;
#140579=CARTESIAN_POINT('Ctrl Pts',(-32.0541365166832,12.7920330529179,
126.378478818651)) ;
#140580=CARTESIAN_POINT('Ctrl Pts',(-31.9989567177235,13.024646117744,126.250422902348)) ;
#140581=CARTESIAN_POINT('Ctrl Pts',(-31.9654247728656,13.2849677628749,
126.1855063369)) ;
#140582=CARTESIAN_POINT('Ctrl Pts',(-31.9549988878817,13.5561840574451,
126.188214091077)) ;
#140583=CARTESIAN_POINT('Ctrl Pts',(-31.9680215372011,13.8182131440166,
126.259475848264)) ;
#140584=CARTESIAN_POINT('Ctrl Pts',(-32.0024636779742,14.0504675663447,
126.393099467081)) ;
#140585=CARTESIAN_POINT('Ctrl Pts',(-32.0555990348147,14.2392689175362,
126.581558183895)) ;
#140586=CARTESIAN_POINT('Ctrl Pts',(-32.1225545405442,14.3686949412613,
126.810291039521)) ;
#140587=CARTESIAN_POINT('Ctrl Pts',(-32.1974429751412,14.4303698787607,
127.062026290213)) ;
#140588=CARTESIAN_POINT('Ctrl Pts',(-32.2751076283904,14.4203874176643,
127.322092039128)) ;
#140589=CARTESIAN_POINT('Ctrl Pts',(-32.3488485574625,14.3383233721809,
127.570744810303)) ;
#140590=CARTESIAN_POINT('Ctrl Pts',(-32.4122411169408,14.1909246457993,
127.789035722479)) ;
#140591=CARTESIAN_POINT('Ctrl Pts',(-32.4602486483851,13.9894771384923,
127.962269753473)) ;
#140592=CARTESIAN_POINT('Ctrl Pts',(-32.4890445130519,13.7468082771736,
128.079510678355)) ;
#140593=CARTESIAN_POINT('Ctrl Pts',(-32.4955954256572,13.4802542547444,
128.131844086168)) ;
#140594=CARTESIAN_POINT('Ctrl Pts',(-32.478469745498,13.2092850470841,128.115057379737)) ;
#140595=CARTESIAN_POINT('Ctrl Pts',(-32.4388473343741,12.9563426353649,
128.032190557193)) ;
#140596=CARTESIAN_POINT('Ctrl Pts',(-32.3779866617617,12.7340442685521,
127.887643915871)) ;
#140597=CARTESIAN_POINT('Ctrl Pts',(-32.299867961373,12.5620254310283,127.692615984056)) ;
#140598=CARTESIAN_POINT('Ctrl Pts',(-32.2100641323022,12.4521634508898,
127.463232611462)) ;
#140599=CARTESIAN_POINT('Ctrl Pts',(-32.1127429550496,12.4110698291516,
127.212210279697)) ;
#140600=CARTESIAN_POINT('Ctrl Pts',(-32.0154678803892,12.4431134789288,
126.961170458623)) ;
#140601=CARTESIAN_POINT('Ctrl Pts',(-31.9243509526054,12.544720780955,126.728008980324)) ;
#140602=CARTESIAN_POINT('Ctrl Pts',(-31.8445157820833,12.709460812036,126.527923986169)) ;
#140603=CARTESIAN_POINT('Ctrl Pts',(-31.7812567007112,12.9261933468861,
126.376356950201)) ;
#140604=CARTESIAN_POINT('Ctrl Pts',(-31.7387566453158,13.1767718332297,
126.285192483539)) ;
#140605=CARTESIAN_POINT('Ctrl Pts',(-31.7187641728704,13.4474343197197,
126.260094130827)) ;
#140606=CARTESIAN_POINT('Ctrl Pts',(-31.722478133967,13.7143157713228,126.30399452411)) ;
#140607=CARTESIAN_POINT('Ctrl Pts',(-31.7483943853981,13.960120914319,126.412695890686)) ;
#140608=CARTESIAN_POINT('Ctrl Pts',(-31.7945444045731,14.1691500544874,
126.580769734858)) ;
#140609=CARTESIAN_POINT('Ctrl Pts',(-31.8562068674074,14.3234013156229,
126.793917930162)) ;
#140610=CARTESIAN_POINT('Ctrl Pts',(-31.9288536888432,14.4138714588237,
127.039311176437)) ;
#140611=CARTESIAN_POINT('Ctrl Pts',(-32.0060870905907,14.4332950652812,
127.297997340453)) ;
#140612=CARTESIAN_POINT('Ctrl Pts',(-32.0823890649229,14.37983766652,127.554210022575)) ;
#140613=CARTESIAN_POINT('Ctrl Pts',(-32.1503082521653,14.2584887072528,
127.78560535761)) ;
#140614=CARTESIAN_POINT('Ctrl Pts',(-32.2053364256527,14.0772214064872,
127.979479297461)) ;
#140615=CARTESIAN_POINT('Ctrl Pts',(-32.2425093340143,13.8478579716949,
128.12133345147)) ;
#140616=CARTESIAN_POINT('Ctrl Pts',(-32.2581355201543,13.5896598560144,
128.200019474609)) ;
#140617=CARTESIAN_POINT('Ctrl Pts',(-32.2507950956267,13.3195388423839,
128.211625689801)) ;
#140618=CARTESIAN_POINT('Ctrl Pts',(-32.2199693000412,13.0556169732422,
128.15477837076)) ;
#140619=CARTESIAN_POINT('Ctrl Pts',(-32.1673744065339,12.8189342678657,
128.034219532277)) ;
#140620=CARTESIAN_POINT('Ctrl Pts',(-32.0958634953359,12.625100278912,127.85846209906)) ;
#140621=CARTESIAN_POINT('Ctrl Pts',(-32.0100232598123,12.4887479023081,
127.640792149346)) ;
#140622=CARTESIAN_POINT('Ctrl Pts',(-31.9152601979825,12.4190670277806,
127.397034402997)) ;
#140623=CARTESIAN_POINT('Ctrl Pts',(-31.8170693261966,12.4213699947317,
127.143425394833)) ;
#140624=CARTESIAN_POINT('Ctrl Pts',(-31.7227136755124,12.4953802874648,
126.900850182708)) ;
#140625=CARTESIAN_POINT('Ctrl Pts',(-31.6374854970419,12.6359572758876,
126.685028308691)) ;
#140626=CARTESIAN_POINT('Ctrl Pts',(-31.5671047785113,12.8329198121217,
126.512552465339)) ;
#140627=CARTESIAN_POINT('Ctrl Pts',(-31.5158144349701,13.0719650653609,
126.395824465428)) ;
#140628=CARTESIAN_POINT('Ctrl Pts',(-31.4865010466435,13.3363498058402,
126.343322488749)) ;
#140629=CARTESIAN_POINT('Ctrl Pts',(-31.4805966443912,13.6070577541681,
126.359216016363)) ;
#140630=CARTESIAN_POINT('Ctrl Pts',(-31.4978044189705,13.8644612546569,
126.442613640301)) ;
#140631=CARTESIAN_POINT('Ctrl Pts',(-31.5360863271803,14.0900773467752,
126.58754221147)) ;
#140632=CARTESIAN_POINT('Ctrl Pts',(-31.5921228560885,14.2682172866369,
126.784395510653)) ;
#140633=CARTESIAN_POINT('Ctrl Pts',(-31.6608593459301,14.38541662164,127.018239393372)) ;
#140634=CARTESIAN_POINT('Ctrl Pts',(-31.7370055456571,14.4341663230829,
127.273806703938)) ;
#140635=CARTESIAN_POINT('Ctrl Pts',(-31.8144395184252,14.4102121199937,
127.533219786427)) ;
#140636=CARTESIAN_POINT('Ctrl Pts',(-31.8864208486602,14.3156228992233,
127.776589906109)) ;
#140637=CARTESIAN_POINT('Ctrl Pts',(-31.9474114950274,14.1571117178342,
127.98788495547)) ;
#140638=CARTESIAN_POINT('Ctrl Pts',(-31.992225383611,13.9459763961177,128.151923385783)) ;
#140639=CARTESIAN_POINT('Ctrl Pts',(-32.016932083013,13.697562228916,128.257202644968)) ;
#140640=CARTESIAN_POINT('Ctrl Pts',(-32.0190519674874,13.4293975021098,
128.296514762563)) ;
#140641=CARTESIAN_POINT('Ctrl Pts',(-31.9977507903844,13.1610019423395,
128.267377292458)) ;
#140642=CARTESIAN_POINT('Ctrl Pts',(-31.9536261139503,12.9105848484096,
128.171675551657)) ;
#140643=CARTESIAN_POINT('Ctrl Pts',(-31.8893635388713,12.6976134704073,
128.017048897951)) ;
#140644=CARTESIAN_POINT('Ctrl Pts',(-31.8087088478594,12.536442279252,127.814560136736)) ;
#140645=CARTESIAN_POINT('Ctrl Pts',(-31.7167865748252,12.4387732237497,
127.579135926508)) ;
#140646=CARTESIAN_POINT('Ctrl Pts',(-31.6191514648672,12.4116342437955,
127.327110422858)) ;
#140647=CARTESIAN_POINT('Ctrl Pts',(-31.5227020632712,12.4569142489461,
127.078414306826)) ;
#140648=CARTESIAN_POINT('Ctrl Pts',(-31.4329813801353,12.5714752096904,
126.849465388448)) ;
#140649=CARTESIAN_POINT('Ctrl Pts',(-31.3560883925141,12.7468633486005,
126.657934872202)) ;
#140650=CARTESIAN_POINT('Ctrl Pts',(-31.2965842595734,12.9706873354731,
126.517219890221)) ;
#140651=CARTESIAN_POINT('Ctrl Pts',(-31.258075825459,13.2271705997234,126.4378699364)) ;
#140652=CARTESIAN_POINT('Ctrl Pts',(-31.2425840183107,13.4971330615505,
126.425684440027)) ;
#140653=CARTESIAN_POINT('Ctrl Pts',(-31.2506122404268,13.7633006467314,
126.482409435389)) ;
#140654=CARTESIAN_POINT('Ctrl Pts',(-31.2805375313788,14.0028269061398,
126.602782532402)) ;
#140655=CARTESIAN_POINT('Ctrl Pts',(-31.330049798945,14.2028678275338,126.780693245081)) ;
#140656=CARTESIAN_POINT('Ctrl Pts',(-31.3940867324171,14.3455611921622,
127.000744655394)) ;
#140657=CARTESIAN_POINT('Ctrl Pts',(-31.4682001918605,14.4231516599767,
127.250464735358)) ;
#140658=CARTESIAN_POINT('Ctrl Pts',(-31.5457693893647,14.4286657254974,
127.510187449708)) ;
#140659=CARTESIAN_POINT('Ctrl Pts',(-31.6206915150044,14.3621069450972,
127.762197957743)) ;
#140660=CARTESIAN_POINT('Ctrl Pts',(-31.6867379358927,14.2287342743254,
127.988196798816)) ;
#140661=CARTESIAN_POINT('Ctrl Pts',(-31.7388558523025,14.0363060460215,
128.1737286555)) ;
#140662=CARTESIAN_POINT('Ctrl Pts',(-31.7718940828191,13.8023696285656,
128.303154059963)) ;
#140663=CARTESIAN_POINT('Ctrl Pts',(-31.7834779337839,13.5388531548576,
128.370254159469)) ;
#140664=CARTESIAN_POINT('Ctrl Pts',(-31.771593832871,13.268451758325,128.368608589023)) ;
#140665=CARTESIAN_POINT('Ctrl Pts',(-31.7366347371057,13.0087996264663,
128.299588081835)) ;
#140666=CARTESIAN_POINT('Ctrl Pts',(-31.6798680712665,12.7778890108915,
128.167025511007)) ;
#140667=CARTESIAN_POINT('Ctrl Pts',(-31.6056828824239,12.5950173458057,
127.983256239013)) ;
#140668=CARTESIAN_POINT('Ctrl Pts',(-31.5173460134283,12.4700324855763,
127.758440084226)) ;
#140669=CARTESIAN_POINT('Ctrl Pts',(-31.4216261029277,12.4138573674352,
127.511850114614)) ;
#140670=CARTESIAN_POINT('Ctrl Pts',(-31.32338456039,12.4301864396543,127.258169228303)) ;
#140671=CARTESIAN_POINT('Ctrl Pts',(-31.2309191230293,12.5166844416216,
127.020906843594)) ;
#140672=CARTESIAN_POINT('Ctrl Pts',(-31.1477558041141,12.6693065290769,
126.811250441322)) ;
#140673=CARTESIAN_POINT('Ctrl Pts',(-31.0809176438295,12.8745471633582,
126.648985783275)) ;
#140674=CARTESIAN_POINT('Ctrl Pts',(-31.0332964810723,13.1212024009445,
126.54318413991)) ;
#140675=CARTESIAN_POINT('Ctrl Pts',(-31.0085143558054,13.3871939344405,
126.503779706618)) ;
#140676=CARTESIAN_POINT('Ctrl Pts',(-31.006972425563,13.6567281897723,126.532400135199)) ;
#140677=CARTESIAN_POINT('Ctrl Pts',(-31.0283333477867,13.90978543386,126.627950810582)) ;
#140678=CARTESIAN_POINT('Ctrl Pts',(-31.0703972652886,14.1280196387556,
126.784017641227)) ;
#140679=CARTESIAN_POINT('Ctrl Pts',(-31.1290079865942,14.2950455998267,
126.988254497869)) ;
#140680=CARTESIAN_POINT('Ctrl Pts',(-31.2001423757924,14.4005267621949,
127.229371566356)) ;
#140681=CARTESIAN_POINT('Ctrl Pts',(-31.2766579994051,14.4350836723043,
127.485868070667)) ;
#140682=CARTESIAN_POINT('Ctrl Pts',(-31.3533027741803,14.3978038978104,
127.742855119514)) ;
#140683=CARTESIAN_POINT('Ctrl Pts',(-31.4237378888131,14.2905756791986,
127.981744408019)) ;
#140684=CARTESIAN_POINT('Ctrl Pts',(-31.4821047890832,14.1209511396773,
128.185413714307)) ;
#140685=CARTESIAN_POINT('Ctrl Pts',(-31.5233617410375,13.9018371700798,
128.33901676082)) ;
#140686=CARTESIAN_POINT('Ctrl Pts',(-31.543988548502,13.6479071174512,128.432433376555)) ;
#140687=CARTESIAN_POINT('Ctrl Pts',(-31.5417580384384,13.3785017706424,
128.458991126292)) ;
#140688=CARTESIAN_POINT('Ctrl Pts',(-31.5158135329586,13.1105160825095,
128.416509788881)) ;
#140689=CARTESIAN_POINT('Ctrl Pts',(-31.467961620135,12.867723627882,128.309652962403)) ;
#140690=CARTESIAN_POINT('Ctrl Pts',(-31.4001585537936,12.6628307247657,
128.144774957304)) ;
#140691=CARTESIAN_POINT('Ctrl Pts',(-31.3171291891636,12.5130918366744,
127.935278432159)) ;
#140692=CARTESIAN_POINT('Ctrl Pts',(-31.2232944076044,12.4280188888238,
127.694417876056)) ;
#140693=CARTESIAN_POINT('Ctrl Pts',(-31.1258166367903,12.4146728717073,
127.442682245229)) ;
#140694=CARTESIAN_POINT('Ctrl Pts',(-31.0298413739331,12.4734183176243,
127.19549995093)) ;
#140695=CARTESIAN_POINT('Ctrl Pts',(-30.9421230224932,12.6005221105397,
126.972405284986)) ;
#140696=CARTESIAN_POINT('Ctrl Pts',(-30.8684025674919,12.7855012395254,
126.790042156092)) ;
#140697=CARTESIAN_POINT('Ctrl Pts',(-30.8125318740678,13.0169861501724,
126.659985042459)) ;
#140698=CARTESIAN_POINT('Ctrl Pts',(-30.778255066982,13.2774554458054,126.592980347573)) ;
#140699=CARTESIAN_POINT('Ctrl Pts',(-30.7672128677042,13.548371247685,126.59385523177)) ;
#140700=CARTESIAN_POINT('Ctrl Pts',(-30.7794543750323,13.8100860909014,
126.662716445457)) ;
#140701=CARTESIAN_POINT('Ctrl Pts',(-30.8134107463879,14.0443620867839,
126.795050916489)) ;
#140702=CARTESIAN_POINT('Ctrl Pts',(-30.8658712807709,14.2339607222734,
126.981412466339)) ;
#140703=CARTESIAN_POINT('Ctrl Pts',(-30.9324377678062,14.3656339915205,
127.209013801012)) ;
#140704=CARTESIAN_POINT('Ctrl Pts',(-31.0075425407356,14.4296685525136,
127.461543585436)) ;
#140705=CARTESIAN_POINT('Ctrl Pts',(-31.085013287722,14.4216217611559,127.720952593954)) ;
#140706=CARTESIAN_POINT('Ctrl Pts',(-31.1587041769614,14.3422173843901,
127.969332083657)) ;
#140707=CARTESIAN_POINT('Ctrl Pts',(-31.2227445131305,14.1963612396834,
128.189629618647)) ;
#140708=CARTESIAN_POINT('Ctrl Pts',(-31.2713611336444,13.9958155660663,
128.364717334213)) ;
#140709=CARTESIAN_POINT('Ctrl Pts',(-31.3007242986626,13.754087100232,128.48360934132)) ;
#140710=CARTESIAN_POINT('Ctrl Pts',(-31.307940808174,13.4887317484018,128.537791288292)) ;
#140711=CARTESIAN_POINT('Ctrl Pts',(-31.2915959174183,13.2176489571942,
128.523278102941)) ;
#140712=CARTESIAN_POINT('Ctrl Pts',(-31.2524780735841,12.9629383916558,
128.442016070707)) ;
#140713=CARTESIAN_POINT('Ctrl Pts',(-31.1920342453667,12.7394456176792,
128.298717927943)) ;
#140714=CARTESIAN_POINT('Ctrl Pts',(-31.114816871371,12.5666312437579,128.106136236575)) ;
#140715=CARTESIAN_POINT('Ctrl Pts',(-31.0247945803096,12.4542159326756,
127.876303092352)) ;
#140716=CARTESIAN_POINT('Ctrl Pts',(-30.9281340923285,12.4113528378657,
127.627016638565)) ;
#140717=CARTESIAN_POINT('Ctrl Pts',(-30.8305532126448,12.4409689783365,
127.37515875896)) ;
#140718=CARTESIAN_POINT('Ctrl Pts',(-30.7387890398871,12.5412370853856,
127.140251323107)) ;
#140719=CARTESIAN_POINT('Ctrl Pts',(-30.6588180682426,12.7041353032971,
126.939686811656)) ;
#140720=CARTESIAN_POINT('Ctrl Pts',(-30.5952142862048,12.9183855317437,
126.786957456823)) ;
#140721=CARTESIAN_POINT('Ctrl Pts',(-30.5518179667405,13.1698655551169,
126.693399866601)) ;
#140722=CARTESIAN_POINT('Ctrl Pts',(-30.5312892737723,13.4380609721582,
126.666456787728)) ;
#140723=CARTESIAN_POINT('Ctrl Pts',(-30.5342266781763,13.707166634389,126.708319823239)) ;
#140724=CARTESIAN_POINT('Ctrl Pts',(-30.5596578817882,13.9538088162951,
126.815620936816)) ;
#140725=CARTESIAN_POINT('Ctrl Pts',(-30.6050569167213,14.1634527174507,
126.981367630752)) ;
#140726=CARTESIAN_POINT('Ctrl Pts',(-30.6666408482026,14.3201289995184,
127.194452620019)) ;
#140727=CARTESIAN_POINT('Ctrl Pts',(-30.738741910301,14.4121341024828,127.438097163118)) ;
#140728=CARTESIAN_POINT('Ctrl Pts',(-30.8161995675161,14.4336855920868,
127.697564927138)) ;
#140729=CARTESIAN_POINT('Ctrl Pts',(-30.8921478214072,14.3827385765516,
127.952524857408)) ;
#140730=CARTESIAN_POINT('Ctrl Pts',(-30.9608791025106,14.2627494122855,
128.186516125915)) ;
#140731=CARTESIAN_POINT('Ctrl Pts',(-31.0163430481192,14.0822576460886,
128.381727901644)) ;
#140732=CARTESIAN_POINT('Ctrl Pts',(-31.0537855670433,13.8561930768697,
128.524066496551)) ;
#140733=CARTESIAN_POINT('Ctrl Pts',(-31.0702462538596,13.5974241277666,
128.605361301542)) ;
#140734=CARTESIAN_POINT('Ctrl Pts',(-31.06356136907,13.3273250801774,128.618881410681)) ;
#140735=CARTESIAN_POINT('Ctrl Pts',(-31.0332777175692,13.0622910344741,
128.563704772445)) ;
#140736=CARTESIAN_POINT('Ctrl Pts',(-30.9814657710391,12.8256129311331,
128.445295711035)) ;
#140737=CARTESIAN_POINT('Ctrl Pts',(-30.910480059094,12.6301797722552,128.271078496651)) ;
#140738=CARTESIAN_POINT('Ctrl Pts',(-30.8249833770331,12.491847584192,128.054418930835)) ;
#140739=CARTESIAN_POINT('Ctrl Pts',(-30.7299901996309,12.4199209625087,
127.810128855303)) ;
#140740=CARTESIAN_POINT('Ctrl Pts',(-30.6319449437103,12.4204246206127,
127.55689476103)) ;
#140741=CARTESIAN_POINT('Ctrl Pts',(-30.5376607508626,12.4921596766918,
127.314438282867)) ;
#140742=CARTESIAN_POINT('Ctrl Pts',(-30.4519929882104,12.6310174141653,
127.097364797993)) ;
#140743=CARTESIAN_POINT('Ctrl Pts',(-30.3811795712557,12.8262648550687,
126.923585720912)) ;
#140744=CARTESIAN_POINT('Ctrl Pts',(-30.3292134109451,13.0646915634,126.804938556669)) ;
#140745=CARTESIAN_POINT('Ctrl Pts',(-30.2992736928993,13.3278245942677,
126.750508221298)) ;
#140746=CARTESIAN_POINT('Ctrl Pts',(-30.2926564922798,13.599858684379,126.764474820433)) ;
#140747=CARTESIAN_POINT('Ctrl Pts',(-30.30917695543,13.8569828233467,126.845742313604)) ;
#140748=CARTESIAN_POINT('Ctrl Pts',(-30.3469514300778,14.0842219920521,
126.989260072652)) ;
#140749=CARTESIAN_POINT('Ctrl Pts',(-30.4023194112078,14.263433654148,127.184042864747)) ;
#140750=CARTESIAN_POINT('Ctrl Pts',(-30.4711865511833,14.3833954982456,
127.418482566623)) ;
#140751=CARTESIAN_POINT('Ctrl Pts',(-30.5472924654005,14.4336980468668,
127.67395398933)) ;
#140752=CARTESIAN_POINT('Ctrl Pts',(-30.6242714433732,14.4120157634547,
127.931818979531)) ;
#140753=CARTESIAN_POINT('Ctrl Pts',(-30.6967127060867,14.3192946556154,
128.176630213785)) ;
#140754=CARTESIAN_POINT('Ctrl Pts',(-30.758053265306,14.1625582896785,128.388922784291)) ;
#140755=CARTESIAN_POINT('Ctrl Pts',(-30.8035122758961,13.9521768642311,
128.55493374882)) ;
#140756=CARTESIAN_POINT('Ctrl Pts',(-30.8287385977858,13.7045477344639,
128.661723129224)) ;
#140757=CARTESIAN_POINT('Ctrl Pts',(-30.8315630481093,13.4377490318283,
128.702961656048)) ;
#140758=CARTESIAN_POINT('Ctrl Pts',(-30.8108154625355,13.1678476288368,
128.675600753644)) ;
#140759=CARTESIAN_POINT('Ctrl Pts',(-30.7674808535793,12.9176590168047,
128.582066704266)) ;
#140760=CARTESIAN_POINT('Ctrl Pts',(-30.7034751148183,12.7025601714455,
128.428332483877)) ;
#140761=CARTESIAN_POINT('Ctrl Pts',(-30.6236198842184,12.5405894740577,
128.228006763419)) ;
#140762=CARTESIAN_POINT('Ctrl Pts',(-30.5317107486925,12.4405287581968,
127.992717121245)) ;
#140763=CARTESIAN_POINT('Ctrl Pts',(-30.4341716126828,12.4114132280254,
127.740958058286)) ;
#140764=CARTESIAN_POINT('Ctrl Pts',(-30.3376601408581,12.4546443860593,
127.492068415319)) ;
#140765=CARTESIAN_POINT('Ctrl Pts',(-30.2478156786388,12.5668919860046,
127.262686548233)) ;
#140766=CARTESIAN_POINT('Ctrl Pts',(-30.1701035113798,12.7415276460806,
127.068926106213)) ;
#140767=CARTESIAN_POINT('Ctrl Pts',(-30.1102266276716,12.9638993361252,
126.927058750175)) ;
#140768=CARTESIAN_POINT('Ctrl Pts',(-30.0711164557523,13.2191083147461,
126.845881048397)) ;
#140769=CARTESIAN_POINT('Ctrl Pts',(-30.0549249492426,13.4893535433623,
126.831705526524)) ;
#140770=CARTESIAN_POINT('Ctrl Pts',(-30.0622158105278,13.7553189464662,
126.886189778859)) ;
#140771=CARTESIAN_POINT('Ctrl Pts',(-30.0917108612786,13.9971252301126,
127.00549241837)) ;
#140772=CARTESIAN_POINT('Ctrl Pts',(-30.1406246191067,14.197781210739,127.181547286119)) ;
#140773=CARTESIAN_POINT('Ctrl Pts',(-30.2043024678696,14.3424511179814,
127.400565722708)) ;
#140774=CARTESIAN_POINT('Ctrl Pts',(-30.2785070155895,14.4220643031845,
127.650668850622)) ;
#140775=CARTESIAN_POINT('Ctrl Pts',(-30.3556721509366,14.4294490868584,
127.909045532744)) ;
#140776=CARTESIAN_POINT('Ctrl Pts',(-30.4307226480629,14.3652071957823,
128.161408707712)) ;
#140777=CARTESIAN_POINT('Ctrl Pts',(-30.4971804793035,14.2335291048216,
128.388647963749)) ;
#140778=CARTESIAN_POINT('Ctrl Pts',(-30.5497562286805,14.0429178976906,
128.575476468873)) ;
#140779=CARTESIAN_POINT('Ctrl Pts',(-30.5834483776407,13.8093219413454,
128.706910013611)) ;
#140780=CARTESIAN_POINT('Ctrl Pts',(-30.595700134892,13.547621689864,128.775798853004)) ;
#140781=CARTESIAN_POINT('Ctrl Pts',(-30.5844060621216,13.275071076932,128.7761395579)) ;
#140782=CARTESIAN_POINT('Ctrl Pts',(-30.5501753727738,13.0163163266613,
128.709067579648)) ;
#140783=CARTESIAN_POINT('Ctrl Pts',(-30.4942243712158,12.7846450787164,
128.578813612621)) ;
#140784=CARTESIAN_POINT('Ctrl Pts',(-30.4202779680125,12.5995255835865,
128.395852978554)) ;
#140785=CARTESIAN_POINT('Ctrl Pts',(-30.3322269992084,12.4726551218916,
128.171878735475)) ;
#140786=CARTESIAN_POINT('Ctrl Pts',(-30.2365765506608,12.4145513359232,
127.925517923835)) ;
#140787=CARTESIAN_POINT('Ctrl Pts',(-30.1388101237624,12.4284690749365,
127.673046945035)) ;
#140788=CARTESIAN_POINT('Ctrl Pts',(-30.0455202983357,12.513343198717,127.43358743129)) ;
#140789=CARTESIAN_POINT('Ctrl Pts',(-29.9620436323982,12.6644367568353,
127.223005705298)) ;
#140790=CARTESIAN_POINT('Ctrl Pts',(-29.8948322705706,12.8679925993142,
127.059595501891)) ;
#140791=CARTESIAN_POINT('Ctrl Pts',(-29.8466374744008,13.1131690756933,
126.95204916951)) ;
#140792=CARTESIAN_POINT('Ctrl Pts',(-29.8210604812711,13.380000312228,126.910471572715)) ;
#140793=CARTESIAN_POINT('Ctrl Pts',(-29.8189544197658,13.6495651936862,
126.93742774856)) ;
#140794=CARTESIAN_POINT('Ctrl Pts',(-29.8395558893614,13.9023389091985,
127.030620642381)) ;
#140795=CARTESIAN_POINT('Ctrl Pts',(-29.8811896320557,14.1226577845122,
127.185548174288)) ;
#140796=CARTESIAN_POINT('Ctrl Pts',(-29.9393151042164,14.2908247564139,
127.388306463954)) ;
#140797=CARTESIAN_POINT('Ctrl Pts',(-30.0097936116339,14.398104059989,127.62734949335)) ;
#140798=CARTESIAN_POINT('Ctrl Pts',(-30.0867674947376,14.4352626924574,
127.885423386131)) ;
#140799=CARTESIAN_POINT('Ctrl Pts',(-30.1635829782001,14.3995540254238,
128.142951931714)) ;
#140800=CARTESIAN_POINT('Ctrl Pts',(-30.2339318810488,14.2948938650605,
128.381416945128)) ;
#140801=CARTESIAN_POINT('Ctrl Pts',(-30.2930532509891,14.1259509639325,
128.587480866756)) ;
#140802=CARTESIAN_POINT('Ctrl Pts',(-30.3346559878636,13.9085226372069,
128.741994405636)) ;
#140803=CARTESIAN_POINT('Ctrl Pts',(-30.3559110579538,13.6557404486892,
128.837201233893)) ;
#140804=CARTESIAN_POINT('Ctrl Pts',(-30.3543840398925,13.3866405250996,
128.865800543519)) ;
#140805=CARTESIAN_POINT('Ctrl Pts',(-30.3291184078958,13.1181023923962,
128.825323697214)) ;
#140806=CARTESIAN_POINT('Ctrl Pts',(-30.2818707300597,12.8743682502049,
128.720238119545)) ;
#140807=CARTESIAN_POINT('Ctrl Pts',(-30.2145778991752,12.6679957013257,
128.556859225096)) ;
#140808=CARTESIAN_POINT('Ctrl Pts',(-30.1317764801247,12.5164143784842,
128.348080123108)) ;
#140809=CARTESIAN_POINT('Ctrl Pts',(-30.0385063797381,12.4295970136061,
128.108745600341)) ;
#140810=CARTESIAN_POINT('Ctrl Pts',(-29.9407571698938,12.4140261381013,
127.856324516585)) ;
#140811=CARTESIAN_POINT('Ctrl Pts',(-29.8447911575134,12.4707103540387,
127.609114356662)) ;
#140812=CARTESIAN_POINT('Ctrl Pts',(-29.7567597974375,12.595906863769,127.385107000309)) ;
#140813=CARTESIAN_POINT('Ctrl Pts',(-29.6825520242752,12.7791143335627,
127.201300936542)) ;
#140814=CARTESIAN_POINT('Ctrl Pts',(-29.6257812390629,13.0114294021893,
127.068868815089)) ;
#140815=CARTESIAN_POINT('Ctrl Pts',(-29.5912358251014,13.2689900400404,
127.000770848446)) ;
#140816=CARTESIAN_POINT('Ctrl Pts',(-29.5793857815431,13.5409258374442,
126.999421466082)) ;
#140817=CARTESIAN_POINT('Ctrl Pts',(-29.5910200568263,13.8029841851952,
127.066485164223)) ;
#140818=CARTESIAN_POINT('Ctrl Pts',(-29.6244387540503,14.0385609610044,
127.197290216951)) ;
#140819=CARTESIAN_POINT('Ctrl Pts',(-29.676435866219,14.229423171085,127.382279927079)) ;
#140820=CARTESIAN_POINT('Ctrl Pts',(-29.7425620569963,14.3627051887218,
127.608541532135)) ;
#140821=CARTESIAN_POINT('Ctrl Pts',(-29.8175397971597,14.4288334278673,
127.860718073631)) ;
#140822=CARTESIAN_POINT('Ctrl Pts',(-29.8950584014949,14.4228924311934,
128.120277862613)) ;
#140823=CARTESIAN_POINT('Ctrl Pts',(-29.9691508818996,14.3451233913639,
128.369927528249)) ;
#140824=CARTESIAN_POINT('Ctrl Pts',(-30.0334310668133,14.2008972200028,
128.590893710781)) ;
#140825=CARTESIAN_POINT('Ctrl Pts',(-30.0824006390069,14.0023959452744,
128.766909525821)) ;
#140826=CARTESIAN_POINT('Ctrl Pts',(-30.112430690584,13.7610317231258,128.887829500663)) ;
#140827=CARTESIAN_POINT('Ctrl Pts',(-30.1202498275654,13.496756912036,128.943686581971)) ;
#140828=CARTESIAN_POINT('Ctrl Pts',(-30.1046746200123,13.2257685064712,
128.931391271073)) ;
#140829=CARTESIAN_POINT('Ctrl Pts',(-30.0660503796317,12.9695425857073,
128.85168137516)) ;
#140830=CARTESIAN_POINT('Ctrl Pts',(-30.0063498248392,12.7456271494707,
128.710444507496)) ;
#140831=CARTESIAN_POINT('Ctrl Pts',(-29.9295767509961,12.5709695173834,
128.519177027686)) ;
#140832=CARTESIAN_POINT('Ctrl Pts',(-29.8397265805435,12.4565179049814,
128.289888234812)) ;
#140833=CARTESIAN_POINT('Ctrl Pts',(-29.743150711624,12.4114773771493,128.040854735391)) ;
#140834=CARTESIAN_POINT('Ctrl Pts',(-29.6451458107009,12.4394645505146,
127.787888159147)) ;
#140835=CARTESIAN_POINT('Ctrl Pts',(-29.5538472801924,12.5368907047146,
127.554071664716)) ;
#140836=CARTESIAN_POINT('Ctrl Pts',(-29.4727909904181,12.6994727146824,
127.350623684027)) ;
#140837=CARTESIAN_POINT('Ctrl Pts',(-29.4090848375654,12.9112843843373,
127.197388701276)) ;
#140838=CARTESIAN_POINT('Ctrl Pts',(-29.3648032660279,13.1634090082974,
127.101442481715)) ;
#140839=CARTESIAN_POINT('Ctrl Pts',(-29.3438379371304,13.4300956045555,
127.073062362202)) ;
#140840=CARTESIAN_POINT('Ctrl Pts',(-29.3459367193337,13.6985487061805,
127.112349022373)) ;
#140841=CARTESIAN_POINT('Ctrl Pts',(-29.3709612229612,13.9480246768514,
127.218730380397)) ;
#140842=CARTESIAN_POINT('Ctrl Pts',(-29.4156502273643,14.1576527966606,
127.382216588722)) ;
#140843=CARTESIAN_POINT('Ctrl Pts',(-29.4767450790731,14.3162850326807,
127.593864273564)) ;
#140844=CARTESIAN_POINT('Ctrl Pts',(-29.5489675079737,14.4106899990105,
127.838019760763)) ;
#140845=CARTESIAN_POINT('Ctrl Pts',(-29.6263938236657,14.4339585104257,
128.097404223511)) ;
#140846=CARTESIAN_POINT('Ctrl Pts',(-29.7021377868535,14.3853107488566,
128.351622410823)) ;
#140847=CARTESIAN_POINT('Ctrl Pts',(-29.771343653763,14.2669553900087,128.587085672282)) ;
#140848=CARTESIAN_POINT('Ctrl Pts',(-29.8271366885734,14.0883945363266,
128.78318518596)) ;
#140849=CARTESIAN_POINT('Ctrl Pts',(-29.8651996903043,13.8631866954131,
128.927384615722)) ;
#140850=CARTESIAN_POINT('Ctrl Pts',(-29.8822989781565,13.6057119879249,
129.01046116545)) ;
#140851=CARTESIAN_POINT('Ctrl Pts',(-29.8762843382152,13.3350527616499,
129.026023028071)) ;
#140852=CARTESIAN_POINT('Ctrl Pts',(-29.8468405958706,13.0707552698518,
128.973143943309)) ;
#140853=CARTESIAN_POINT('Ctrl Pts',(-29.7955855799297,12.8321485931701,
128.856463844239)) ;
#140854=CARTESIAN_POINT('Ctrl Pts',(-29.7246842633997,12.6344629226598,
128.682655409326)) ;
#140855=CARTESIAN_POINT('Ctrl Pts',(-29.6399098993552,12.4951761456202,
128.467948465936)) ;
#140856=CARTESIAN_POINT('Ctrl Pts',(-29.545305543797,12.4210995999737,128.224732967655)) ;
#140857=CARTESIAN_POINT('Ctrl Pts',(-29.4471501611367,12.4192964340424,
127.971214797337)) ;
#140858=CARTESIAN_POINT('Ctrl Pts',(-29.3524662110009,12.4890492714601,
127.727661006437)) ;
#140859=CARTESIAN_POINT('Ctrl Pts',(-29.2661993967892,12.6268327661457,
127.508955192755)) ;
#140860=CARTESIAN_POINT('Ctrl Pts',(-29.1953397269962,12.8195831784206,
127.334849135012)) ;
#140861=CARTESIAN_POINT('Ctrl Pts',(-29.1426416993899,13.0571003299884,
127.214097852355)) ;
#140862=CARTESIAN_POINT('Ctrl Pts',(-29.1120307486165,13.320280679744,127.15777002931)) ;
#140863=CARTESIAN_POINT('Ctrl Pts',(-29.1047060155249,13.5914917582005,
127.169555410746)) ;
#140864=CARTESIAN_POINT('Ctrl Pts',(-29.1206742275936,13.8505567194106,
127.249383407295)) ;
#140865=CARTESIAN_POINT('Ctrl Pts',(-29.1577239501666,14.0777829909349,
127.390619937542)) ;
#140866=CARTESIAN_POINT('Ctrl Pts',(-29.212717534914,14.2590886738723,127.584383986945)) ;
#140867=CARTESIAN_POINT('Ctrl Pts',(-29.2812145769909,14.3807167115641,
127.817703884744)) ;
#140868=CARTESIAN_POINT('Ctrl Pts',(-29.3571182980737,14.433343615208,128.072557778617)) ;
#140869=CARTESIAN_POINT('Ctrl Pts',(-29.4346569346725,14.4133893489329,
128.332279874876)) ;
#140870=CARTESIAN_POINT('Ctrl Pts',(-29.5068531862197,14.3229978009541,
128.576166295593)) ;
#140871=CARTESIAN_POINT('Ctrl Pts',(-29.5686642958486,14.1680349923561,
128.789860721644)) ;
#140872=CARTESIAN_POINT('Ctrl Pts',(-29.6145595401633,13.959434776873,128.957078689166)) ;
#140873=CARTESIAN_POINT('Ctrl Pts',(-29.6405447655555,13.712829168107,129.066081979048)) ;
#140874=CARTESIAN_POINT('Ctrl Pts',(-29.6439572935887,13.4442543283008,
129.109297534092)) ;
#140875=CARTESIAN_POINT('Ctrl Pts',(-29.6241012830215,13.176694407093,129.084213601662)) ;
#140876=CARTESIAN_POINT('Ctrl Pts',(-29.5810380555836,12.9234094710806,
128.991780301771)) ;
#140877=CARTESIAN_POINT('Ctrl Pts',(-29.5179260136605,12.7086523175308,
128.840427686241)) ;
#140878=CARTESIAN_POINT('Ctrl Pts',(-29.4384206751917,12.5444332801825,
128.641184040457)) ;
#140879=CARTESIAN_POINT('Ctrl Pts',(-29.3464035868294,12.4422654275157,
128.40569652746)) ;
#140880=CARTESIAN_POINT('Ctrl Pts',(-29.2493516171235,12.4113238215259,
128.155221462137)) ;
#140881=CARTESIAN_POINT('Ctrl Pts',(-29.1526487800264,12.452199983914,127.905794005988)) ;
#140882=CARTESIAN_POINT('Ctrl Pts',(-29.0620241585539,12.5635389999469,
127.674336022858)) ;
#140883=CARTESIAN_POINT('Ctrl Pts',(-28.9845003087822,12.7354102811942,
127.480874966993)) ;
#140884=CARTESIAN_POINT('Ctrl Pts',(-28.9238804025353,12.9568498442606,
127.336904325203)) ;
#140885=CARTESIAN_POINT('Ctrl Pts',(-28.8840944094843,13.2117694969246,
127.253797665177)) ;
#140886=CARTESIAN_POINT('Ctrl Pts',(-28.867247231596,13.48252854114,127.23778724413)) ;
#140887=CARTESIAN_POINT('Ctrl Pts',(-28.8739686370942,13.748482945783,127.290563060827)) ;
#140888=CARTESIAN_POINT('Ctrl Pts',(-28.9027248635833,13.9900671624614,
127.407555291496)) ;
#140889=CARTESIAN_POINT('Ctrl Pts',(-28.9509775630119,14.1922209506685,
127.581640902384)) ;
#140890=CARTESIAN_POINT('Ctrl Pts',(-29.014692765249,14.3393855753319,127.800968412475)) ;
#140891=CARTESIAN_POINT('Ctrl Pts',(-29.0880462050529,14.4204077482377,
128.048293378874)) ;
#140892=CARTESIAN_POINT('Ctrl Pts',(-29.1655876741887,14.4304302068623,
128.307946651833)) ;
#140893=CARTESIAN_POINT('Ctrl Pts',(-29.2410222299655,14.3678711174913,
128.561528843684)) ;
#140894=CARTESIAN_POINT('Ctrl Pts',(-29.3078276957715,14.2376926994235,
128.789814550899)) ;
#140895=CARTESIAN_POINT('Ctrl Pts',(-29.3606966005294,14.0489882455827,
128.977410807902)) ;
#140896=CARTESIAN_POINT('Ctrl Pts',(-29.3950338182995,13.8164455432918,
129.110736007563)) ;
#140897=CARTESIAN_POINT('Ctrl Pts',(-29.4078405026359,13.5541088077793,
129.18138636938)) ;
#140898=CARTESIAN_POINT('Ctrl Pts',(-29.3974124674152,13.2846771651641,
129.183867775352)) ;
#140899=CARTESIAN_POINT('Ctrl Pts',(-29.3636550612449,13.0230234432121,
129.118469484008)) ;
#140900=CARTESIAN_POINT('Ctrl Pts',(-29.3083509044896,12.7908726515439,
128.990023773957)) ;
#140901=CARTESIAN_POINT('Ctrl Pts',(-29.2347161729155,12.6038717726337,
128.808047575783)) ;
#140902=CARTESIAN_POINT('Ctrl Pts',(-29.1473019065763,12.4755977885113,
128.585809976829)) ;
#140903=CARTESIAN_POINT('Ctrl Pts',(-29.051574804785,12.4151865367556,128.339309434992)) ;
#140904=CARTESIAN_POINT('Ctrl Pts',(-28.9538949869407,12.4270410724712,
128.087048576477)) ;
#140905=CARTESIAN_POINT('Ctrl Pts',(-28.8603899759108,12.5098502892393,
127.846962468881)) ;
#140906=CARTESIAN_POINT('Ctrl Pts',(-28.7765666463378,12.6589866450951,
127.635344392143)) ;
#140907=CARTESIAN_POINT('Ctrl Pts',(-28.7087215246026,12.8615687451882,
127.470148650886)) ;
#140908=CARTESIAN_POINT('Ctrl Pts',(-28.6600385912031,13.1050266769027,
127.361069056887)) ;
#140909=CARTESIAN_POINT('Ctrl Pts',(-28.6337144036686,13.3718444110737,
127.317363744017)) ;
#140910=CARTESIAN_POINT('Ctrl Pts',(-28.6308308714776,13.6411904453346,
127.341985774397)) ;
#140911=CARTESIAN_POINT('Ctrl Pts',(-28.6510730281356,13.8968635155474,
127.434435033886)) ;
#140912=CARTESIAN_POINT('Ctrl Pts',(-28.6917302180179,14.1159779799374,
127.586141478924)) ;
#140913=CARTESIAN_POINT('Ctrl Pts',(-28.7498275997111,14.2873257027271,
127.789085812779)) ;
#140914=CARTESIAN_POINT('Ctrl Pts',(-28.8199093839214,14.3958947377193,
128.026877760367)) ;
#140915=CARTESIAN_POINT('Ctrl Pts',(-28.8965301500445,14.4351265097039,
128.283821788283)) ;
#140916=CARTESIAN_POINT('Ctrl Pts',(-28.9734020017538,14.401957868835,128.541485841149)) ;
#140917=CARTESIAN_POINT('Ctrl Pts',(-29.04450350885,14.2982652122168,128.782398104542)) ;
#140918=CARTESIAN_POINT('Ctrl Pts',(-29.1035127772872,14.1324802087574,
128.987829900738)) ;
#140919=CARTESIAN_POINT('Ctrl Pts',(-29.1459631430346,13.9154628269439,
129.144988599754)) ;
#140920=CARTESIAN_POINT('Ctrl Pts',(-29.1678311809284,13.6633712406997,
129.241982385923)) ;
#140921=CARTESIAN_POINT('Ctrl Pts',(-29.1669352598198,13.3940849340156,
129.272479386928)) ;
#140922=CARTESIAN_POINT('Ctrl Pts',(-29.1424881944319,13.1263052582701,
129.234248892586)) ;
#140923=CARTESIAN_POINT('Ctrl Pts',(-29.0956268544443,12.8804158513159,
129.130464723764)) ;
#140924=CARTESIAN_POINT('Ctrl Pts',(-29.0290020456781,12.6733662735578,
128.968940469468)) ;
#140925=CARTESIAN_POINT('Ctrl Pts',(-28.9464646971493,12.5197379021673,
128.760988363812)) ;
#140926=CARTESIAN_POINT('Ctrl Pts',(-28.853372820222,12.4310982059369,128.52218112472)) ;
#140927=CARTESIAN_POINT('Ctrl Pts',(-28.7559344096338,12.4134628316865,
128.270577847274)) ;
#140928=CARTESIAN_POINT('Ctrl Pts',(-28.6597354547319,12.4679867596538,
128.022716531487)) ;
#140929=CARTESIAN_POINT('Ctrl Pts',(-28.5711852993659,12.5916525961337,
127.797270001978)) ;
#140930=CARTESIAN_POINT('Ctrl Pts',(-28.496628960717,12.7734685194903,127.612433381058)) ;
#140931=CARTESIAN_POINT('Ctrl Pts',(-28.4395894906841,13.0028689239805,
127.478980244894)) ;
#140932=CARTESIAN_POINT('Ctrl Pts',(-28.4040144970096,13.261962548957,127.408156835628)) ;
#140933=CARTESIAN_POINT('Ctrl Pts',(-28.3916352491005,13.5340193336117,
127.405276715523)) ;
#140934=CARTESIAN_POINT('Ctrl Pts',(-28.4025847374665,13.7955676266414,
127.470215599722)) ;
#140935=CARTESIAN_POINT('Ctrl Pts',(-28.4353995658411,14.0322614564451,
127.599264380229)) ;
#140936=CARTESIAN_POINT('Ctrl Pts',(-28.4868397358784,14.2243899010379,
127.782585598631)) ;
#140937=CARTESIAN_POINT('Ctrl Pts',(-28.5527080316366,14.3598901604785,
128.008145601297)) ;
#140938=CARTESIAN_POINT('Ctrl Pts',(-28.6278695337408,14.4280176399282,
128.261005626896)) ;
#140939=CARTESIAN_POINT('Ctrl Pts',(-28.7049132284027,14.4241023567618,
128.518966473141)) ;
#140940=CARTESIAN_POINT('Ctrl Pts',(-28.7794251636048,14.3482279673457,
128.76994543598)) ;
#140941=CARTESIAN_POINT('Ctrl Pts',(-28.8439156578016,14.2060723674291,
128.991445593633)) ;
#140942=CARTESIAN_POINT('Ctrl Pts',(-28.8934515036008,14.0086807740354,
129.169172629331)) ;
#140943=CARTESIAN_POINT('Ctrl Pts',(-28.9240482263405,13.7691470824975,
129.291636017452)) ;
#140944=CARTESIAN_POINT('Ctrl Pts',(-28.9325810238934,13.5031160209837,
129.349853238854)) ;
#140945=CARTESIAN_POINT('Ctrl Pts',(-28.9175541272843,13.2327333331826,
129.339069926924)) ;
#140946=CARTESIAN_POINT('Ctrl Pts',(-28.8797005123668,12.976776614233,129.261497699467)) ;
#140947=CARTESIAN_POINT('Ctrl Pts',(-28.8206976959534,12.7518156970481,
129.12225615979)) ;
#140948=CARTESIAN_POINT('Ctrl Pts',(-28.744034594892,12.5749030333723,128.931449829078)) ;
#140949=CARTESIAN_POINT('Ctrl Pts',(-28.6546157712723,12.4587258582811,
128.703359625527)) ;
#140950=CARTESIAN_POINT('Ctrl Pts',(-28.5576462996642,12.4118884067616,
128.453352995457)) ;
#140951=CARTESIAN_POINT('Ctrl Pts',(-28.4609282919855,12.4371448006442,
128.203671997539)) ;
#140952=CARTESIAN_POINT('Ctrl Pts',(-28.3682833220301,12.5335140246063,
127.966323254618)) ;
#140953=CARTESIAN_POINT('Ctrl Pts',(-28.2875408074332,12.6929505687292,
127.763479311416)) ;
#140954=CARTESIAN_POINT('Ctrl Pts',(-28.2226827881692,12.9053983640665,
127.607203099237)) ;
#140955=CARTESIAN_POINT('Ctrl Pts',(-28.1782420281259,13.1539498783259,
127.510416974053)) ;
#140956=CARTESIAN_POINT('Ctrl Pts',(-28.1562632009264,13.422675078525,127.479377602005)) ;
#140957=CARTESIAN_POINT('Ctrl Pts',(-28.1577935734945,13.691089143288,127.516960997828)) ;
#140958=CARTESIAN_POINT('Ctrl Pts',(-28.1821515376259,13.9413684458137,
127.621389577109)) ;
#140959=CARTESIAN_POINT('Ctrl Pts',(-28.226439644364,14.1526799240858,127.783773013239)) ;
#140960=CARTESIAN_POINT('Ctrl Pts',(-28.2870558314823,14.3125333467772,
127.993960696093)) ;
#140961=CARTESIAN_POINT('Ctrl Pts',(-28.3588077689731,14.408819463409,128.236644758816)) ;
#140962=CARTESIAN_POINT('Ctrl Pts',(-28.4364512521204,14.4343198914763,
128.496786106316)) ;
#140963=CARTESIAN_POINT('Ctrl Pts',(-28.5121726728494,14.3877722038871,
128.750872707546)) ;
#140964=CARTESIAN_POINT('Ctrl Pts',(-28.5817452954328,14.2711470779282,
128.987450777919)) ;
#140965=CARTESIAN_POINT('Ctrl Pts',(-28.6377450769826,14.0951742319451,
129.183988636599)) ;
#140966=CARTESIAN_POINT('Ctrl Pts',(-28.6766270030896,13.870335302896,129.330724917506)) ;
#140967=CARTESIAN_POINT('Ctrl Pts',(-28.6943466665121,13.6128358613542,
129.415688801231)) ;
#140968=CARTESIAN_POINT('Ctrl Pts',(-28.6889851715194,13.3431052342381,
129.43306210823)) ;
#140969=CARTESIAN_POINT('Ctrl Pts',(-28.660328849755,13.0784068980914,129.382462071094)) ;
#140970=CARTESIAN_POINT('Ctrl Pts',(-28.6091631818449,12.8371324748468,
129.266305768313)) ;
#140971=CARTESIAN_POINT('Ctrl Pts',(-28.5393761304624,12.639991514166,129.095436280033)) ;
#140972=CARTESIAN_POINT('Ctrl Pts',(-28.454558582428,12.4979352238862,128.880780706304)) ;
#140973=CARTESIAN_POINT('Ctrl Pts',(-28.3599026767257,12.4220838446985,
128.637480288422)) ;
#140974=CARTESIAN_POINT('Ctrl Pts',(-28.2619574346768,12.4184701426874,
128.384508953084)) ;
#140975=CARTESIAN_POINT('Ctrl Pts',(-28.1674363195264,12.4860425111682,
128.141319241242)) ;
#140976=CARTESIAN_POINT('Ctrl Pts',(-28.0810401792008,12.62129710121,127.92213272214)) ;
#140977=CARTESIAN_POINT('Ctrl Pts',(-28.0092963384714,12.8133840710904,
127.745605494146)) ;
#140978=CARTESIAN_POINT('Ctrl Pts',(-27.9559959394673,13.0503650213175,
127.623143511295)) ;
#140979=CARTESIAN_POINT('Ctrl Pts',(-27.9248374489822,13.3123038567085,
127.56512149863)) ;
#140980=CARTESIAN_POINT('Ctrl Pts',(-27.9168020041589,13.5832779933084,
127.574796329027)) ;
#140981=CARTESIAN_POINT('Ctrl Pts',(-27.9320454118317,13.8428844537896,
127.652487922196)) ;
#140982=CARTESIAN_POINT('Ctrl Pts',(-27.9686240808447,14.0720013816764,
127.792453983478)) ;
#140983=CARTESIAN_POINT('Ctrl Pts',(-28.02315885797,14.2546155978529,127.984855739173)) ;
#140984=CARTESIAN_POINT('Ctrl Pts',(-28.0911548338665,14.3779471702252,
128.216627929247)) ;
#140985=CARTESIAN_POINT('Ctrl Pts',(-28.1670206979292,14.4327785527786,
128.471419072253)) ;
#140986=CARTESIAN_POINT('Ctrl Pts',(-28.2443543229282,14.4152048360803,
128.730429870402)) ;
#140987=CARTESIAN_POINT('Ctrl Pts',(-28.3171288418279,14.3266409428597,
128.976154143631)) ;
#140988=CARTESIAN_POINT('Ctrl Pts',(-28.3794021887183,14.1729214671605,
129.191259216607)) ;
#140989=CARTESIAN_POINT('Ctrl Pts',(-28.4256655711301,13.9662155184911,
129.359458626253)) ;
#140990=CARTESIAN_POINT('Ctrl Pts',(-28.4522869637337,13.7208186547473,
129.470286151888)) ;
#140991=CARTESIAN_POINT('Ctrl Pts',(-28.4564309237617,13.4521886594885,
129.515686361507)) ;
#140992=CARTESIAN_POINT('Ctrl Pts',(-28.4371402610968,13.1838897369756,
129.492322441034)) ;
#140993=CARTESIAN_POINT('Ctrl Pts',(-28.395008920419,12.9313138648893,129.402409345746)) ;
#140994=CARTESIAN_POINT('Ctrl Pts',(-28.3322804324004,12.7142071163423,
129.252310506691)) ;
#140995=CARTESIAN_POINT('Ctrl Pts',(-28.2529695087352,12.5481822878489,
129.053703416506)) ;
#140996=CARTESIAN_POINT('Ctrl Pts',(-28.1617320020028,12.4445945503844,
128.820309439414)) ;
#140997=CARTESIAN_POINT('Ctrl Pts',(-28.0646800119981,12.4110615289685,
128.569866486525)) ;
#140998=CARTESIAN_POINT('Ctrl Pts',(-27.9674199966164,12.4502003413461,
128.318970669863)) ;
#140999=CARTESIAN_POINT('Ctrl Pts',(-27.8771422429295,12.5587981618695,
128.088294626238)) ;
#141000=CARTESIAN_POINT('Ctrl Pts',(-27.798868329989,12.7290993092181,127.892732978884)) ;
#141001=CARTESIAN_POINT('Ctrl Pts',(-27.737418020498,12.950564316011,127.746505773547)) ;
#141002=CARTESIAN_POINT('Ctrl Pts',(-27.6971967474441,13.2039534170359,
127.662012965437)) ;
#141003=CARTESIAN_POINT('Ctrl Pts',(-27.6796377184877,13.4737768777198,
127.643834921464)) ;
#141004=CARTESIAN_POINT('Ctrl Pts',(-27.6856087062491,13.7408243981145,
127.694494054552)) ;
#141005=CARTESIAN_POINT('Ctrl Pts',(-27.713966691118,13.9843829005592,127.81048226759)) ;
#141006=CARTESIAN_POINT('Ctrl Pts',(-27.7614922013285,14.1867700874977,
127.982267797735)) ;
#141007=CARTESIAN_POINT('Ctrl Pts',(-27.8248727597038,14.3360223630702,
128.200658761603)) ;
#141008=CARTESIAN_POINT('Ctrl Pts',(-27.8980311925229,14.4190305114461,
128.447414074677)) ;
#141009=CARTESIAN_POINT('Ctrl Pts',(-27.9755313511817,14.4311357302908,
128.706944667949)) ;
#141010=CARTESIAN_POINT('Ctrl Pts',(-28.0510062244958,14.3708887604269,
128.960585149943)) ;
#141011=CARTESIAN_POINT('Ctrl Pts',(-28.1182594178393,14.2422926303469,
129.190247723132)) ;
#141012=CARTESIAN_POINT('Ctrl Pts',(-28.1714032261274,14.0562618591324,
129.378475255161)) ;
#141013=CARTESIAN_POINT('Ctrl Pts',(-28.2066164194266,13.8231736000303,
129.51460563921)) ;
#141014=CARTESIAN_POINT('Ctrl Pts',(-28.2199928730901,13.5622215659962,
129.586803651273)) ;
#141015=CARTESIAN_POINT('Ctrl Pts',(-28.2102466648294,13.2923509313982,
129.591337178618)) ;
#141016=CARTESIAN_POINT('Ctrl Pts',(-28.1772564946493,13.0307855165856,
129.528091249551)) ;
#141017=CARTESIAN_POINT('Ctrl Pts',(-28.1223679042081,12.796715819409,129.400977122732)) ;
#141018=CARTESIAN_POINT('Ctrl Pts',(-28.0492209458298,12.6083942037896,
129.220402711305)) ;
#141019=CARTESIAN_POINT('Ctrl Pts',(-27.9620383490602,12.4782666718545,
128.998873123193)) ;
#141020=CARTESIAN_POINT('Ctrl Pts',(-27.8667818789838,12.4160107552107,
128.753637616017)) ;
#141021=CARTESIAN_POINT('Ctrl Pts',(-27.7688218289437,12.4255889321841,
128.500641595981)) ;
#141022=CARTESIAN_POINT('Ctrl Pts',(-27.6747744769812,12.5070743683389,
128.259102889033)) ;
#141023=CARTESIAN_POINT('Ctrl Pts',(-27.5910307718227,12.6538728233386,
128.047551316195)) ;
#141024=CARTESIAN_POINT('Ctrl Pts',(-27.5225494662066,12.8553500132408,
127.880554242958)) ;
#141025=CARTESIAN_POINT('Ctrl Pts',(-27.4732675164133,13.0981034422233,
127.769743109725)) ;
#141026=CARTESIAN_POINT('Ctrl Pts',(-27.4463104814565,13.3649638787798,
127.724238327967)) ;
#141027=CARTESIAN_POINT('Ctrl Pts',(-27.4428491935347,13.633409473525,127.747047620251)) ;
#141028=CARTESIAN_POINT('Ctrl Pts',(-27.4622348005861,13.8886868708514,
127.836832748595)) ;
#141029=CARTESIAN_POINT('Ctrl Pts',(-27.5025149897505,14.1104518503625,
127.987632859157)) ;
#141030=CARTESIAN_POINT('Ctrl Pts',(-27.5602073067102,14.2832226352683,
128.189383387774)) ;
#141031=CARTESIAN_POINT('Ctrl Pts',(-27.6299708142586,14.3937886252325,
128.426231960119)) ;
#141032=CARTESIAN_POINT('Ctrl Pts',(-27.7068452145878,14.4350213811874,
128.684066370922)) ;
#141033=CARTESIAN_POINT('Ctrl Pts',(-27.7834265371489,14.4038716557598,
128.940723547936)) ;
#141034=CARTESIAN_POINT('Ctrl Pts',(-27.8549060448491,14.3020574418522,
129.182793140959)) ;
#141035=CARTESIAN_POINT('Ctrl Pts',(-27.9143023664084,14.1377082714835,
129.389364157556)) ;
#141036=CARTESIAN_POINT('Ctrl Pts',(-27.9571987711447,13.9225120842828,
129.547744046412)) ;
#141037=CARTESIAN_POINT('Ctrl Pts',(-27.9797590876057,13.6705375094453,
129.646846563363)) ;
#141038=CARTESIAN_POINT('Ctrl Pts',(-27.9794706179545,13.4018845199762,
129.679067144231)) ;
#141039=CARTESIAN_POINT('Ctrl Pts',(-27.9558401512939,13.1344381552283,
129.643132562523)) ;
#141040=CARTESIAN_POINT('Ctrl Pts',(-27.9093458664183,12.8864832879891,
129.540587983339)) ;
#141041=CARTESIAN_POINT('Ctrl Pts',(-27.8435719825832,12.679196010264,129.381374767827)) ;
#141042=CARTESIAN_POINT('Ctrl Pts',(-27.7613092533485,12.5233811225036,
129.174291094988)) ;
#141043=CARTESIAN_POINT('Ctrl Pts',(-27.6685700885561,12.4327816487888,
128.936468632901)) ;
#141044=CARTESIAN_POINT('Ctrl Pts',(-27.5708744742361,12.4129159597619,
128.684218615284)) ;
#141045=CARTESIAN_POINT('Ctrl Pts',(-27.4746603999551,12.4655032985934,
128.436276111074)) ;
#141046=CARTESIAN_POINT('Ctrl Pts',(-27.386086163872,12.5866529745153,128.21064207061)) ;
#141047=CARTESIAN_POINT('Ctrl Pts',(-27.3107230948148,12.767439628638,128.023577427765)) ;
#141048=CARTESIAN_POINT('Ctrl Pts',(-27.2529836630615,12.9966808158701,
127.888194922856)) ;
#141049=CARTESIAN_POINT('Ctrl Pts',(-27.2169995959156,13.2541242728622,
127.816037280406)) ;
#141050=CARTESIAN_POINT('Ctrl Pts',(-27.2038734867719,13.524842234863,127.810821018869)) ;
#141051=CARTESIAN_POINT('Ctrl Pts',(-27.2141327174669,13.7882272307475,
127.873904817517)) ;
#141052=CARTESIAN_POINT('Ctrl Pts',(-27.2464010178925,14.0260984495824,
128.001380339773)) ;
#141053=CARTESIAN_POINT('Ctrl Pts',(-27.2974857985163,14.2200232579374,
128.183731204006)) ;
#141054=CARTESIAN_POINT('Ctrl Pts',(-27.362908361414,14.3567722758536,128.407916901054)) ;
#141055=CARTESIAN_POINT('Ctrl Pts',(-27.4374375225388,14.4269174595849,
128.65873883066)) ;
#141056=CARTESIAN_POINT('Ctrl Pts',(-27.5150827034848,14.4252572802329,
128.918711429118)) ;
#141057=CARTESIAN_POINT('Ctrl Pts',(-27.5895675801479,14.3512844314495,
129.169525398487)) ;
#141058=CARTESIAN_POINT('Ctrl Pts',(-27.6542017158287,14.2117349601844,
129.391317457744)) ;
#141059=CARTESIAN_POINT('Ctrl Pts',(-27.7045044465824,14.0152547415916,
129.571407076294)) ;
#141060=CARTESIAN_POINT('Ctrl Pts',(-27.7357152512017,13.7756398670369,
129.695790498812)) ;
#141061=CARTESIAN_POINT('Ctrl Pts',(-27.7448568548906,13.5122934272068,
129.755507542801)) ;
#141062=CARTESIAN_POINT('Ctrl Pts',(-27.7306240640475,13.2411299536141,
129.74712858429)) ;
#141063=CARTESIAN_POINT('Ctrl Pts',(-27.6933744004606,12.9839532693091,
129.671381426942)) ;
#141064=CARTESIAN_POINT('Ctrl Pts',(-27.6347046882777,12.7572239501203,
129.533220708441)) ;
#141065=CARTESIAN_POINT('Ctrl Pts',(-27.5588077749335,12.5794741125724,
129.344509108417)) ;
#141066=CARTESIAN_POINT('Ctrl Pts',(-27.4694635855471,12.4611210628414,
129.116724569477)) ;
#141067=CARTESIAN_POINT('Ctrl Pts',(-27.3731253977084,12.4122668253808,
128.868385474263)) ;
#141068=CARTESIAN_POINT('Ctrl Pts',(-27.2756381680084,12.4354395157324,
128.616699151777)) ;
#141069=CARTESIAN_POINT('Ctrl Pts',(-27.1828180490366,12.5301694906382,
128.378825987728)) ;
#141070=CARTESIAN_POINT('Ctrl Pts',(-27.1018777065855,12.6876686677728,
128.175337732907)) ;
#141071=CARTESIAN_POINT('Ctrl Pts',(-27.0365848293891,12.898212465334,128.017714536355)) ;
#141072=CARTESIAN_POINT('Ctrl Pts',(-26.9912984048923,13.1472879217631,
127.918636822097)) ;
#141073=CARTESIAN_POINT('Ctrl Pts',(-26.9687884702793,13.4151706305656,
127.885968483086)) ;
#141074=CARTESIAN_POINT('Ctrl Pts',(-26.9696641945452,13.6833052701105,
127.921580490902)) ;
#141075=CARTESIAN_POINT('Ctrl Pts',(-26.993178842716,13.9335262167577,128.023403835393)) ;
#141076=CARTESIAN_POINT('Ctrl Pts',(-27.0372896845173,14.1479664881483,
128.185552207591)) ;
#141077=CARTESIAN_POINT('Ctrl Pts',(-27.0973867629725,14.3087959188899,
128.394119491692)) ;
#141078=CARTESIAN_POINT('Ctrl Pts',(-27.1688826353453,14.4069520257531,
128.636056957824)) ;
#141079=CARTESIAN_POINT('Ctrl Pts',(-27.2460944940994,14.434703937208,128.894776663616)) ;
#141080=CARTESIAN_POINT('Ctrl Pts',(-27.322455233744,14.3899170706969,129.15096525146)) ;
#141081=CARTESIAN_POINT('Ctrl Pts',(-27.3918872573227,14.275848167113,129.386924096555)) ;
#141082=CARTESIAN_POINT('Ctrl Pts',(-27.4485941023117,14.1010294116989,
129.585654834495)) ;
#141083=CARTESIAN_POINT('Ctrl Pts',(-27.4880125752689,13.8772033892953,
129.733965637947)) ;
#141084=CARTESIAN_POINT('Ctrl Pts',(-27.5063600960657,13.6206146695245,
129.820736577765)) ;
#141085=CARTESIAN_POINT('Ctrl Pts',(-27.5017041699236,13.3509220809883,
129.840178597232)) ;
#141086=CARTESIAN_POINT('Ctrl Pts',(-27.473598569591,13.0853828321562,129.791246985454)) ;
#141087=CARTESIAN_POINT('Ctrl Pts',(-27.4233898154442,12.8445475509271,
129.677681035035)) ;
#141088=CARTESIAN_POINT('Ctrl Pts',(-27.3538833905169,12.6449528168769,
129.507770820876)) ;
#141089=CARTESIAN_POINT('Ctrl Pts',(-27.2694172510683,12.5012606134937,
129.294132382056)) ;
#141090=CARTESIAN_POINT('Ctrl Pts',(-27.1752933143249,12.4235056415569,
129.052276160427)) ;
#141091=CARTESIAN_POINT('Ctrl Pts',(-27.0773273129102,12.4173186288012,
128.799252781911)) ;
#141092=CARTESIAN_POINT('Ctrl Pts',(-26.9820546641332,12.4833715210388,
128.554075191291)) ;
#141093=CARTESIAN_POINT('Ctrl Pts',(-26.8957427187905,12.6162286422635,
128.334974337295)) ;
#141094=CARTESIAN_POINT('Ctrl Pts',(-26.8232541348428,12.8073411346184,
128.156380628229)) ;
#141095=CARTESIAN_POINT('Ctrl Pts',(-26.7694384260827,13.0432166498449,
128.032389957765)) ;
#141096=CARTESIAN_POINT('Ctrl Pts',(-26.7376022204803,13.3046950611415,
127.972397092543)) ;
#141097=CARTESIAN_POINT('Ctrl Pts',(-26.7289133019392,13.5764464662961,
127.980250837782)) ;
#141098=CARTESIAN_POINT('Ctrl Pts',(-26.7436047960042,13.8363551234792,
128.05630676716)) ;
#141099=CARTESIAN_POINT('Ctrl Pts',(-26.7794413994135,14.0655922643217,
128.193961346238)) ;
#141100=CARTESIAN_POINT('Ctrl Pts',(-26.8336382377925,14.2503954850495,
128.38547143464)) ;
#141101=CARTESIAN_POINT('Ctrl Pts',(-26.9015725255857,14.3757154300573,
128.617161479179)) ;
#141102=CARTESIAN_POINT('Ctrl Pts',(-26.97717390156,14.4321659963664,128.871117555925)) ;
#141103=CARTESIAN_POINT('Ctrl Pts',(-27.0542951454193,14.416734287709,129.129400399269)) ;
#141104=CARTESIAN_POINT('Ctrl Pts',(-27.1272709315475,14.330289953115,129.375702496647)) ;
#141105=CARTESIAN_POINT('Ctrl Pts',(-27.189990205641,14.1784243130749,129.592118462722)) ;
#141106=CARTESIAN_POINT('Ctrl Pts',(-27.2369829461064,13.9717507261075,
129.762638532864)) ;
#141107=CARTESIAN_POINT('Ctrl Pts',(-27.2639778254799,13.7284356402105,
129.874378327128)) ;
#141108=CARTESIAN_POINT('Ctrl Pts',(-27.2689082133704,13.4606301532886,
129.922024727165)) ;
#141109=CARTESIAN_POINT('Ctrl Pts',(-27.2501277788475,13.1906191848992,
129.900339303317)) ;
#141110=CARTESIAN_POINT('Ctrl Pts',(-27.2088647894994,12.9388679746563,
129.812757148243)) ;
#141111=CARTESIAN_POINT('Ctrl Pts',(-27.1465129550907,12.7195132138376,
129.663887017964)) ;
#141112=CARTESIAN_POINT('Ctrl Pts',(-27.0674166967818,12.5518557372857,
129.465961436593)) ;
#141113=CARTESIAN_POINT('Ctrl Pts',(-26.9768706070221,12.4467157582098,
129.234433433492)) ;
#141114=CARTESIAN_POINT('Ctrl Pts',(-26.8793527844966,12.4110145773966,
128.982819997536)) ;
#141115=CARTESIAN_POINT('Ctrl Pts',(-26.7826642470665,12.4479828338558,
128.733367252288)) ;
#141116=CARTESIAN_POINT('Ctrl Pts',(-26.6918813929173,12.5544308131199,
128.501279219724)) ;
#141117=CARTESIAN_POINT('Ctrl Pts',(-26.6127197999617,12.7245572228014,
128.30335122958)) ;
#141118=CARTESIAN_POINT('Ctrl Pts',(-26.5511850159183,12.9435040036317,
128.156658473163)) ;
#141119=CARTESIAN_POINT('Ctrl Pts',(-26.5102190611483,13.1965754591591,
128.07005407176)) ;
#141120=CARTESIAN_POINT('Ctrl Pts',(-26.4920475738245,13.4658054703846,
128.050031979519)) ;
#141121=CARTESIAN_POINT('Ctrl Pts',(-26.4973097875531,13.732871013944,128.098578279237)) ;
#141122=CARTESIAN_POINT('Ctrl Pts',(-26.5249498576305,13.9772573341515,
128.212437582729)) ;
#141123=CARTESIAN_POINT('Ctrl Pts',(-26.5722033377622,14.1820529613216,
128.383597525912)) ;
#141124=CARTESIAN_POINT('Ctrl Pts',(-26.6352241541874,14.3328844022839,
128.60092354091)) ;
#141125=CARTESIAN_POINT('Ctrl Pts',(-26.7084097679367,14.4178011232664,
128.847856955232)) ;
#141126=CARTESIAN_POINT('Ctrl Pts',(-26.7854970159119,14.4318123856393,
129.106011876347)) ;
#141127=CARTESIAN_POINT('Ctrl Pts',(-26.8614289054063,14.3732302589804,
129.36113391513)) ;
#141128=CARTESIAN_POINT('Ctrl Pts',(-26.9286362415281,14.2469702615313,
129.590490603117)) ;
#141129=CARTESIAN_POINT('Ctrl Pts',(-26.9823748563956,14.062146427081,129.780527825508)) ;
#141130=CARTESIAN_POINT('Ctrl Pts',(-27.0180716868534,13.8305006230351,
129.918009774563)) ;
#141131=CARTESIAN_POINT('Ctrl Pts',(-27.0321547042406,13.5704780261443,
129.992234873768)) ;
#141132=CARTESIAN_POINT('Ctrl Pts',(-27.02304498105,13.2994605324582,129.99876766656)) ;
#141133=CARTESIAN_POINT('Ctrl Pts',(-26.990642584611,13.037734227312,129.937203717605)) ;
#141134=CARTESIAN_POINT('Ctrl Pts',(-26.9366601478888,12.803624496366,129.812576900429)) ;
#141135=CARTESIAN_POINT('Ctrl Pts',(-26.8637477811583,12.6130122644718,
129.632813056256)) ;
#141136=CARTESIAN_POINT('Ctrl Pts',(-26.7771319980352,12.4813447222013,
129.412848032968)) ;
#141137=CARTESIAN_POINT('Ctrl Pts',(-26.6817077227162,12.4167223738628,
129.167240678023)) ;
#141138=CARTESIAN_POINT('Ctrl Pts',(-26.5838608694619,12.4243656160183,
128.91452903007)) ;
#141139=CARTESIAN_POINT('Ctrl Pts',(-26.4898665957701,12.5034383279314,
128.673051616794)) ;
#141140=CARTESIAN_POINT('Ctrl Pts',(-26.4055971039593,12.6484426938847,
128.460008405466)) ;
#141141=CARTESIAN_POINT('Ctrl Pts',(-26.3364227025837,12.8490572514717,
128.291073622268)) ;
#141142=CARTESIAN_POINT('Ctrl Pts',(-26.286632817812,13.0907450284177,128.178753459324)) ;
#141143=CARTESIAN_POINT('Ctrl Pts',(-26.2590235096436,13.3559778959346,
128.131196454483)) ;
#141144=CARTESIAN_POINT('Ctrl Pts',(-26.2548350038944,13.6264773514175,
128.152116585356)) ;
#141145=CARTESIAN_POINT('Ctrl Pts',(-26.2735948253303,13.8815734058857,
128.239965472009)) ;
#141146=CARTESIAN_POINT('Ctrl Pts',(-26.3132675920051,14.1045282831523,
128.388984294423)) ;
#141147=CARTESIAN_POINT('Ctrl Pts',(-26.3705006334924,14.2789670592856,
128.58938512689)) ;
#141148=CARTESIAN_POINT('Ctrl Pts',(-26.4400738173777,14.391495176626,128.825720476705)) ;
#141149=CARTESIAN_POINT('Ctrl Pts',(-26.516521682403,14.4348607601378,129.082169907306)) ;
#141150=CARTESIAN_POINT('Ctrl Pts',(-26.5935936372758,14.4056890506022,
129.34044345786)) ;
#141151=CARTESIAN_POINT('Ctrl Pts',(-26.6649960120157,14.3062653151645,
129.582129996569)) ;
#141152=CARTESIAN_POINT('Ctrl Pts',(-26.7249635553657,14.143440527592,129.790441806033)) ;
#141153=CARTESIAN_POINT('Ctrl Pts',(-26.7684141471086,13.9296996140236,
129.950418504304)) ;
#141154=CARTESIAN_POINT('Ctrl Pts',(-26.7916761698876,13.6772902096435,
130.051730701194)) ;
#141155=CARTESIAN_POINT('Ctrl Pts',(-26.7920166713928,13.409949714787,130.085650574175)) ;
#141156=CARTESIAN_POINT('Ctrl Pts',(-26.7690406668665,13.1418739498075,
130.051671418724)) ;
#141157=CARTESIAN_POINT('Ctrl Pts',(-26.723380228586,12.8939990758876,129.951430090132)) ;
#141158=CARTESIAN_POINT('Ctrl Pts',(-26.6580007927469,12.6844790937915,
129.793476110788)) ;
#141159=CARTESIAN_POINT('Ctrl Pts',(-26.5756929840171,12.5265062627849,
129.586412690797)) ;
#141160=CARTESIAN_POINT('Ctrl Pts',(-26.4836475460607,12.4345049835541,
129.350444325695)) ;
#141161=CARTESIAN_POINT('Ctrl Pts',(-26.3856918165124,12.4124896125378,
129.097544125775)) ;
#141162=CARTESIAN_POINT('Ctrl Pts',(-26.2897573999388,12.4629155090419,
128.850279348653)) ;
#141163=CARTESIAN_POINT('Ctrl Pts',(-26.2006908721167,12.5820912846789,
128.623259203242)) ;
#141164=CARTESIAN_POINT('Ctrl Pts',(-26.1246238315882,12.762437228793,128.434290332495)) ;
#141165=CARTESIAN_POINT('Ctrl Pts',(-26.0668894647953,12.9881392996051,
128.298578201089)) ;
#141166=CARTESIAN_POINT('Ctrl Pts',(-26.0298902648549,13.2462583810271,
128.223645427311)) ;
#141167=CARTESIAN_POINT('Ctrl Pts',(-26.0161451635682,13.5176872670076,
128.216711625548)) ;
#141168=CARTESIAN_POINT('Ctrl Pts',(-26.0257258719504,13.7805945427873,
128.277696305593)) ;
#141169=CARTESIAN_POINT('Ctrl Pts',(-26.0573518405434,14.0195270315699,
128.403295435911)) ;
#141170=CARTESIAN_POINT('Ctrl Pts',(-26.1079348776956,14.215038587717,128.58418549861)) ;
#141171=CARTESIAN_POINT('Ctrl Pts',(-26.1731602667738,14.3538333245836,
128.807869014675)) ;
#141172=CARTESIAN_POINT('Ctrl Pts',(-26.2474276298777,14.4259647082628,
129.057883463846)) ;
#141173=CARTESIAN_POINT('Ctrl Pts',(-26.3253614750608,14.4260802645705,
129.318830419785)) ;
#141174=CARTESIAN_POINT('Ctrl Pts',(-26.3993536485964,14.3549350188174,
129.567893070133)) ;
#141175=CARTESIAN_POINT('Ctrl Pts',(-26.4649283623393,14.2162528409401,
129.792714680865)) ;
#141176=CARTESIAN_POINT('Ctrl Pts',(-26.5155109902137,14.0213155988979,
129.97355085765)) ;
#141177=CARTESIAN_POINT('Ctrl Pts',(-26.5473189700669,13.7835941603823,
130.099574541527)) ;
#141178=CARTESIAN_POINT('Ctrl Pts',(-26.5571140519307,13.5186607714519,
130.161456345039)) ;
#141179=CARTESIAN_POINT('Ctrl Pts',(-26.5436206328906,13.2494161503812,
130.154983697786)) ;
#141180=CARTESIAN_POINT('Ctrl Pts',(-26.50683594055,12.990369061565,130.080765011974)) ;
#141181=CARTESIAN_POINT('Ctrl Pts',(-26.4490861734073,12.763690008938,129.945095819254)) ;
#141182=CARTESIAN_POINT('Ctrl Pts',(-26.3729175406989,12.5829313612557,
129.755895708972)) ;
#141183=CARTESIAN_POINT('Ctrl Pts',(-26.2847953527081,12.4640788232719,
129.531321097916)) ;
#141184=CARTESIAN_POINT('Ctrl Pts',(-26.1880587495672,12.4125693563369,
129.282013562901)) ;
#141185=CARTESIAN_POINT('Ctrl Pts',(-26.0908313951311,12.4337094288139,
129.030974071127)) ;
#141186=CARTESIAN_POINT('Ctrl Pts',(-25.9976681952167,12.5263145417804,
128.792132170837)) ;
#141187=CARTESIAN_POINT('Ctrl Pts',(-25.9162455950597,12.6822587586298,
128.587265960244)) ;
#141188=CARTESIAN_POINT('Ctrl Pts',(-25.8504252260032,12.891562566965,128.428112349608)) ;
#141189=CARTESIAN_POINT('Ctrl Pts',(-25.8045634978476,13.1392603161048,
128.327287274008)) ;
#141190=CARTESIAN_POINT('Ctrl Pts',(-25.7813146650202,13.4076118666746,
128.292561015423)) ;
#141191=CARTESIAN_POINT('Ctrl Pts',(-25.7814884215431,13.6757335651874,
128.326078291203)) ;
#141192=CARTESIAN_POINT('Ctrl Pts',(-25.8046625409424,13.9281677218218,
128.427127499137)) ;
#141193=CARTESIAN_POINT('Ctrl Pts',(-25.8476422273,14.1410411473799,128.585519729201)) ;
#141194=CARTESIAN_POINT('Ctrl Pts',(-25.907683202068,14.3051859898324,128.794181724547)) ;
#141195=CARTESIAN_POINT('Ctrl Pts',(-25.978930527692,14.4050577743806,129.035370932357)) ;
#141196=CARTESIAN_POINT('Ctrl Pts',(-26.0561466019767,14.4349188602028,
129.294141592844)) ;
#141197=CARTESIAN_POINT('Ctrl Pts',(-26.132478258172,14.3922309332557,129.550183106697)) ;
#141198=CARTESIAN_POINT('Ctrl Pts',(-26.2021814505518,14.280180814084,129.786927094144)) ;
#141199=CARTESIAN_POINT('Ctrl Pts',(-26.2593826682603,14.1070359905501,
129.98710891507)) ;
#141200=CARTESIAN_POINT('Ctrl Pts',(-26.2994671587914,13.8833119230109,
130.137511200348)) ;
#141201=CARTESIAN_POINT('Ctrl Pts',(-26.318337977065,13.6288341860585,130.225620170339)) ;
#141202=CARTESIAN_POINT('Ctrl Pts',(-26.3143645892423,13.3582465565096,
130.247188750393)) ;
#141203=CARTESIAN_POINT('Ctrl Pts',(-26.2869754269948,13.0930921360638,
130.200247530991)) ;
#141204=CARTESIAN_POINT('Ctrl Pts',(-26.2373396152418,12.8509540623848,
130.088400393616)) ;
#141205=CARTESIAN_POINT('Ctrl Pts',(-26.1683668074332,12.6500624789761,
129.920030156326)) ;
#141206=CARTESIAN_POINT('Ctrl Pts',(-26.0841377965404,12.5043219731701,
129.707136325983)) ;
#141207=CARTESIAN_POINT('Ctrl Pts',(-25.9900281941511,12.4246931364435,
129.465377948168)) ;
#141208=CARTESIAN_POINT('Ctrl Pts',(-25.8925815111015,12.4164962070895,
129.213702440245)) ;
#141209=CARTESIAN_POINT('Ctrl Pts',(-25.7970766789543,12.480251448006,128.9678640707)) ;
#141210=CARTESIAN_POINT('Ctrl Pts',(-25.7101967844713,12.6116453538561,
128.747191789048)) ;
#141211=CARTESIAN_POINT('Ctrl Pts',(-25.6373443096755,12.8011773158268,
128.567502634195)) ;
#141212=CARTESIAN_POINT('Ctrl Pts',(-25.5830591810682,13.0350451037076,
128.442022034867)) ;
#141213=CARTESIAN_POINT('Ctrl Pts',(-25.5504047936859,13.296978163916,128.379768959982)) ;
#141214=CARTESIAN_POINT('Ctrl Pts',(-25.5410675634481,13.567734807944,128.385602982608)) ;
#141215=CARTESIAN_POINT('Ctrl Pts',(-25.5549687871613,13.8283852939848,
128.459355229538)) ;
#141216=CARTESIAN_POINT('Ctrl Pts',(-25.5904030600774,14.0598715137087,
128.595997047928)) ;
#141217=CARTESIAN_POINT('Ctrl Pts',(-25.6440274690769,14.2455588284616,
128.785744630347)) ;
#141218=CARTESIAN_POINT('Ctrl Pts',(-25.7113284363032,14.372564186769,129.015457476957)) ;
#141219=CARTESIAN_POINT('Ctrl Pts',(-25.7870239449595,14.4315964784329,
129.269802836714)) ;
#141220=CARTESIAN_POINT('Ctrl Pts',(-25.8643623704875,14.4181824034525,
129.528794500079)) ;
#141221=CARTESIAN_POINT('Ctrl Pts',(-25.9375242038495,14.3336377789342,
129.775633938815)) ;
#141222=CARTESIAN_POINT('Ctrl Pts',(-26.0004478793548,14.1840090727439,
129.992551171513)) ;
#141223=CARTESIAN_POINT('Ctrl Pts',(-26.0480191574849,13.9789557865459,
130.164753929132)) ;
#141224=CARTESIAN_POINT('Ctrl Pts',(-26.0757639781487,13.7355807215654,
130.278815327172)) ;
#141225=CARTESIAN_POINT('Ctrl Pts',(-26.0812599990852,13.4678621828446,
130.328144833775)) ;
#141226=CARTESIAN_POINT('Ctrl Pts',(-26.0633151819106,13.1991327913341,
130.308713856629)) ;
#141227=CARTESIAN_POINT('Ctrl Pts',(-26.0224676209765,12.945225699974,130.222533094685)) ;
#141228=CARTESIAN_POINT('Ctrl Pts',(-25.9609990724827,12.7259341324381,
130.076051329516)) ;
#141229=CARTESIAN_POINT('Ctrl Pts',(-25.8822604809974,12.5559411157644,
129.879237566137)) ;
#141230=CARTESIAN_POINT('Ctrl Pts',(-25.7914597527613,12.448546099201,129.647141485638)) ;
#141231=CARTESIAN_POINT('Ctrl Pts',(-25.6946150022909,12.4111599417381,
129.39729586978)) ;
#141232=CARTESIAN_POINT('Ctrl Pts',(-25.5977172593343,12.4456278236405,
129.147262647583)) ;
#141233=CARTESIAN_POINT('Ctrl Pts',(-25.5060117038367,12.5514145638213,
128.91274322654)) ;
#141234=CARTESIAN_POINT('Ctrl Pts',(-25.4273295882221,12.7181519506854,
128.715846515651)) ;
#141235=CARTESIAN_POINT('Ctrl Pts',(-25.3649037596215,12.9364297169796,
128.566681417571)) ;
#141236=CARTESIAN_POINT('Ctrl Pts',(-25.323332482555,13.18875320047,128.478299070981)) ;
#141237=CARTESIAN_POINT('Ctrl Pts',(-25.3044411252258,13.4580633582235,
128.456211243148)) ;
#141238=CARTESIAN_POINT('Ctrl Pts',(-25.3090734679159,13.7256378176803,
128.502937534738)) ;
#141239=CARTESIAN_POINT('Ctrl Pts',(-25.3360410802481,13.9704139793173,
128.61476470412)) ;
#141240=CARTESIAN_POINT('Ctrl Pts',(-25.3827781783647,14.1767864699774,
128.78443560151)) ;
#141241=CARTESIAN_POINT('Ctrl Pts',(-25.4454333702109,14.3292888824905,
129.00069713083)) ;
#141242=CARTESIAN_POINT('Ctrl Pts',(-25.5181538685983,14.4162419172546,
129.246167034807)) ;
#141243=CARTESIAN_POINT('Ctrl Pts',(-25.5956938103097,14.4323070544899,
129.505861185904)) ;
#141244=CARTESIAN_POINT('Ctrl Pts',(-25.6710803564494,14.3764282188079,
129.759076945677)) ;
#141245=CARTESIAN_POINT('Ctrl Pts',(-25.7391087689832,14.2515624978579,
129.991058480962)) ;
#141246=CARTESIAN_POINT('Ctrl Pts',(-25.7932747288291,14.0682227623741,
130.182328167812)) ;
#141247=CARTESIAN_POINT('Ctrl Pts',(-25.8296100576166,13.8370232958438,
130.321766242783)) ;
#141248=CARTESIAN_POINT('Ctrl Pts',(-25.8442555060527,13.5786248872284,
130.397495870533)) ;
#141249=CARTESIAN_POINT('Ctrl Pts',(-25.8358834370233,13.3076276344917,
130.406189803794)) ;
#141250=CARTESIAN_POINT('Ctrl Pts',(-25.8041766941054,13.0452572131087,
130.346664739274)) ;
#141251=CARTESIAN_POINT('Ctrl Pts',(-25.7505336279653,12.8091511761324,
130.223169232237)) ;
#141252=CARTESIAN_POINT('Ctrl Pts',(-25.6781409528713,12.6175515473568,
130.044873070202)) ;
#141253=CARTESIAN_POINT('Ctrl Pts',(-25.592105058716,12.4843717623364,129.826512043424)) ;
#141254=CARTESIAN_POINT('Ctrl Pts',(-25.4967610810165,12.4175958607342,
129.581171788726)) ;
#141255=CARTESIAN_POINT('Ctrl Pts',(-25.3990048864728,12.423055511444,129.328685771011)) ;
#141256=CARTESIAN_POINT('Ctrl Pts',(-25.304669732605,12.5002516966647,129.086267631271)) ;
#141257=CARTESIAN_POINT('Ctrl Pts',(-25.2202532201414,12.6429372151447,
128.872696249123)) ;
#141258=CARTESIAN_POINT('Ctrl Pts',(-25.1502572326467,12.8430360326097,
128.70151673981)) ;
#141259=CARTESIAN_POINT('Ctrl Pts',(-25.100056569004,13.0829431740334,128.587874270422)) ;
#141260=CARTESIAN_POINT('Ctrl Pts',(-25.0717103188712,13.3482626607442,
128.538235999123)) ;
#141261=CARTESIAN_POINT('Ctrl Pts',(-25.0668143083415,13.6179806011048,
128.556971818961)) ;
#141262=CARTESIAN_POINT('Ctrl Pts',(-25.0850142932641,13.875457841107,128.64339943274)) ;
#141263=CARTESIAN_POINT('Ctrl Pts',(-25.124300844542,14.0994368558722,128.791311810996)) ;
#141264=CARTESIAN_POINT('Ctrl Pts',(-25.1807114497818,14.2743408494019,
128.989091173341)) ;
#141265=CARTESIAN_POINT('Ctrl Pts',(-25.2501729019598,14.3892596808428,
129.225197599148)) ;
#141266=CARTESIAN_POINT('Ctrl Pts',(-25.3264637380068,14.4346258040279,
129.481163853611)) ;
#141267=CARTESIAN_POINT('Ctrl Pts',(-25.4038107016267,14.4074612293383,
129.740327944683)) ;
#141268=CARTESIAN_POINT('Ctrl Pts',(-25.4754023445781,14.309698779788,129.982562521745)) ;
#141269=CARTESIAN_POINT('Ctrl Pts',(-25.5355623444991,14.149377401071,130.191293654527)) ;
#141270=CARTESIAN_POINT('Ctrl Pts',(-25.579751232365,13.9355628699076,130.35362784232)) ;
#141271=CARTESIAN_POINT('Ctrl Pts',(-25.6034709375141,13.6861606150325,
130.455982421836)) ;
#141272=CARTESIAN_POINT('Ctrl Pts',(-25.6045462391797,13.4167352196909,
130.492347116565)) ;
#141273=CARTESIAN_POINT('Ctrl Pts',(-25.5821919384405,13.1492793409581,
130.460071094422)) ;
#141274=CARTESIAN_POINT('Ctrl Pts',(-25.5371871208477,12.9005268752137,
130.361747259184)) ;
#141275=CARTESIAN_POINT('Ctrl Pts',(-25.4722627818621,12.6897474195092,
130.205134842187)) ;
#141276=CARTESIAN_POINT('Ctrl Pts',(-25.390755324331,12.5306016213155,130.000259613854)) ;
#141277=CARTESIAN_POINT('Ctrl Pts',(-25.2984805593987,12.4360458788129,
129.763793833998)) ;
#141278=CARTESIAN_POINT('Ctrl Pts',(-25.2007322982766,12.412131815675,129.511445036942)) ;
#141279=CARTESIAN_POINT('Ctrl Pts',(-25.104473068318,12.4605358152628,129.263297371341)) ;
#141280=CARTESIAN_POINT('Ctrl Pts',(-25.015042394543,12.5784164712972,129.035267066627)) ;
#141281=CARTESIAN_POINT('Ctrl Pts',(-24.939138342932,12.7554817105356,128.84648405616)) ;
#141282=CARTESIAN_POINT('Ctrl Pts',(-24.8803298764375,12.9817624941524,
128.707905450152)) ;
#141283=CARTESIAN_POINT('Ctrl Pts',(-24.8429088332853,13.238159912852,128.631586768857)) ;
#141284=CARTESIAN_POINT('Ctrl Pts',(-24.8284099370948,13.5101993099721,
128.622545061218)) ;
#141285=CARTESIAN_POINT('Ctrl Pts',(-24.8373360171865,13.7733132280516,
128.681579397042)) ;
#141286=CARTESIAN_POINT('Ctrl Pts',(-24.8685380944431,14.014064219241,128.806071656317)) ;
#141287=CARTESIAN_POINT('Ctrl Pts',(-24.9184256609091,14.209874547802,128.98476052808)) ;
#141288=CARTESIAN_POINT('Ctrl Pts',(-24.9832119214002,14.3505802758006,
129.207139933116)) ;
#141289=CARTESIAN_POINT('Ctrl Pts',(-25.0573786128153,14.4248316803085,
129.456898592496)) ;
#141290=CARTESIAN_POINT('Ctrl Pts',(-25.1352233259638,14.4272047931218,
129.717544442823)) ;
#141291=CARTESIAN_POINT('Ctrl Pts',(-25.2095908938482,14.3577939123121,
129.967801571309)) ;
#141292=CARTESIAN_POINT('Ctrl Pts',(-25.2752361261482,14.2217456845042,
130.192666800583)) ;
#141293=CARTESIAN_POINT('Ctrl Pts',(-25.3267045949438,14.0267540354523,
130.376353398215)) ;
#141294=CARTESIAN_POINT('Ctrl Pts',(-25.3588379023475,13.7911379046606,
130.503148112011)) ;
#141295=CARTESIAN_POINT('Ctrl Pts',(-25.3693904125377,13.5273989700341,
130.567168396677)) ;
#141296=CARTESIAN_POINT('Ctrl Pts',(-25.356570795273,13.2571615768974,130.562775183947)) ;
#141297=CARTESIAN_POINT('Ctrl Pts',(-25.3204195881661,12.9974107950377,
130.49041379717)) ;
#141298=CARTESIAN_POINT('Ctrl Pts',(-25.2631584465656,12.7695379002692,
130.356198249557)) ;
#141299=CARTESIAN_POINT('Ctrl Pts',(-25.1878940849675,12.5879936402029,
130.169461722707)) ;
#141300=CARTESIAN_POINT('Ctrl Pts',(-25.0995423284155,12.4663339482719,
129.94442760723)) ;
#141301=CARTESIAN_POINT('Ctrl Pts',(-25.0029353623396,12.4130530274037,
129.695488820152)) ;
#141302=CARTESIAN_POINT('Ctrl Pts',(-24.9058352313859,12.4321501261291,
129.444765661347)) ;
#141303=CARTESIAN_POINT('Ctrl Pts',(-24.8126115718343,12.5224108266138,
129.205678168256)) ;
#141304=CARTESIAN_POINT('Ctrl Pts',(-24.7304215398182,12.677312247728,128.998719014252)) ;
#141305=CARTESIAN_POINT('Ctrl Pts',(-24.6641964360112,12.8853932149283,
128.838366520164)) ;
#141306=CARTESIAN_POINT('Ctrl Pts',(-24.6178771552594,13.1311434716641,
128.736066599532)) ;
#141307=CARTESIAN_POINT('Ctrl Pts',(-24.5938296155373,13.400088705093,128.699120704413)) ;
#141308=CARTESIAN_POINT('Ctrl Pts',(-24.5934287047137,13.6679854897532,
128.730912226515)) ;
#141309=CARTESIAN_POINT('Ctrl Pts',(-24.6156510295128,13.9198929111463,
128.82897060526)) ;
#141310=CARTESIAN_POINT('Ctrl Pts',(-24.6586746207821,14.1367331628791,
128.987925161323)) ;
#141311=CARTESIAN_POINT('Ctrl Pts',(-24.7177298808385,14.300676127775,129.193353483904)) ;
#141312=CARTESIAN_POINT('Ctrl Pts',(-24.7891652491851,14.4034182514066,
129.435324255067)) ;
#141313=CARTESIAN_POINT('Ctrl Pts',(-24.8661178021545,14.4350219446425,
129.693230679241)) ;
#141314=CARTESIAN_POINT('Ctrl Pts',(-24.9426427517626,14.3943912068368,
129.949881794211)) ;
#141315=CARTESIAN_POINT('Ctrl Pts',(-25.0126014634411,14.2842181110636,
130.187358662861)) ;
#141316=CARTESIAN_POINT('Ctrl Pts',(-25.0702385393857,14.1123337735145,
130.388851754434)) ;
#141317=CARTESIAN_POINT('Ctrl Pts',(-25.1106557279227,13.8914432947139,
130.539995528719)) ;
#141318=CARTESIAN_POINT('Ctrl Pts',(-25.1303460035706,13.6364805468731,
130.630669027387)) ;
#141319=CARTESIAN_POINT('Ctrl Pts',(-25.1270349079514,13.3663281054811,
130.654132094012)) ;
#141320=CARTESIAN_POINT('Ctrl Pts',(-25.10027987688,13.1002904156236,130.609104691335)) ;
#141321=CARTESIAN_POINT('Ctrl Pts',(-25.0512395903328,12.8573186036191,
130.498986163059)) ;
#141322=CARTESIAN_POINT('Ctrl Pts',(-24.9827606397883,12.655055825907,130.332060726985)) ;
#141323=CARTESIAN_POINT('Ctrl Pts',(-24.8989878483042,12.5076994513089,
130.120463312692)) ;
#141324=CARTESIAN_POINT('Ctrl Pts',(-24.8051012286791,12.4260781925878,
129.879353041103)) ;
#141325=CARTESIAN_POINT('Ctrl Pts',(-24.7077158005553,12.4155414447684,
129.627838457708)) ;
#141326=CARTESIAN_POINT('Ctrl Pts',(-24.6113622754169,12.478090322654,129.379774872544)) ;
#141327=CARTESIAN_POINT('Ctrl Pts',(-24.5249865423267,12.6066344478164,
129.160266874238)) ;
#141328=CARTESIAN_POINT('Ctrl Pts',(-24.4513172549699,12.7952137023379,
128.978327228472)) ;
#141329=CARTESIAN_POINT('Ctrl Pts',(-24.3965263603158,13.0279819979312,
128.851345529342)) ;
#141330=CARTESIAN_POINT('Ctrl Pts',(-24.3631902230821,13.2896875880003,
128.787142151235)) ;
#141331=CARTESIAN_POINT('Ctrl Pts',(-24.353237574026,13.5603129292438,128.791160312568)) ;
#141332=CARTESIAN_POINT('Ctrl Pts',(-24.3664638245753,13.8211028677067,
128.862887276775)) ;
#141333=CARTESIAN_POINT('Ctrl Pts',(-24.4013270139757,14.053803313072,128.997878663223)) ;
#141334=CARTESIAN_POINT('Ctrl Pts',(-24.4545017892813,14.2410908350298,
129.186323723895)) ;
#141335=CARTESIAN_POINT('Ctrl Pts',(-24.5217031916119,14.3701941601828,
129.415842737755)) ;
#141336=CARTESIAN_POINT('Ctrl Pts',(-24.597197642324,14.4308809616827,129.669568740632)) ;
#141337=CARTESIAN_POINT('Ctrl Pts',(-24.6743263714102,14.4196138695008,
129.927844860309)) ;
#141338=CARTESIAN_POINT('Ctrl Pts',(-24.7478689182381,14.3368368148889,
130.175876279872)) ;
#141339=CARTESIAN_POINT('Ctrl Pts',(-24.8109786100875,14.1892310626699,
130.393251616306)) ;
#141340=CARTESIAN_POINT('Ctrl Pts',(-24.8590750037211,13.9859052749166,
130.566957801464)) ;
#141341=CARTESIAN_POINT('Ctrl Pts',(-24.8875059799453,13.7426111503383,
130.683133832411)) ;
#141342=CARTESIAN_POINT('Ctrl Pts',(-24.893634064606,13.4761437933061,130.734199736731)) ;
#141343=CARTESIAN_POINT('Ctrl Pts',(-24.876424077817,13.207093106288,130.716931703523)) ;
#141344=CARTESIAN_POINT('Ctrl Pts',(-24.8361611582837,12.9521503447167,
130.632500310692)) ;
#141345=CARTESIAN_POINT('Ctrl Pts',(-24.7752501370882,12.7315094010331,
130.487653228042)) ;
#141346=CARTESIAN_POINT('Ctrl Pts',(-24.6965758178761,12.5595225483876,
130.291156310629)) ;
#141347=CARTESIAN_POINT('Ctrl Pts',(-24.6067705147701,12.4509681320899,
130.061702132681)) ;
#141348=CARTESIAN_POINT('Ctrl Pts',(-24.5092389918735,12.4111337662686,
129.810124891726)) ;
#141349=CARTESIAN_POINT('Ctrl Pts',(-24.4127206080174,12.4436883981266,
129.561039626234)) ;
#141350=CARTESIAN_POINT('Ctrl Pts',(-24.3206925540612,12.5474867377232,
129.325602640613)) ;
#141351=CARTESIAN_POINT('Ctrl Pts',(-24.2416819636404,12.7123018064528,
129.127697092053)) ;
#141352=CARTESIAN_POINT('Ctrl Pts',(-24.1785497831319,12.9300708063277,
128.976576940149)) ;
#141353=CARTESIAN_POINT('Ctrl Pts',(-24.1365376956219,13.1802337565337,
128.886722669123)) ;
#141354=CARTESIAN_POINT('Ctrl Pts',(-24.1168251300341,13.4510759335073,
128.862457184691)) ;
#141355=CARTESIAN_POINT('Ctrl Pts',(-24.120840546179,13.7180593172982,128.907263452931)) ;
#141356=CARTESIAN_POINT('Ctrl Pts',(-24.1472467528154,13.9642786305136,
129.017528555115)) ;
#141357=CARTESIAN_POINT('Ctrl Pts',(-24.1933829926006,14.1712561910319,
129.18534923182)) ;
#141358=CARTESIAN_POINT('Ctrl Pts',(-24.2553727944982,14.3253725381315,
129.399556943149)) ;
#141359=CARTESIAN_POINT('Ctrl Pts',(-24.3284416395332,14.4148742721194,
129.646304105575)) ;
#141360=CARTESIAN_POINT('Ctrl Pts',(-24.4053454883016,14.4329087862449,
129.90387754185)) ;
#141361=CARTESIAN_POINT('Ctrl Pts',(-24.481387664403,14.3788838227845,130.159238685966)) ;
#141362=CARTESIAN_POINT('Ctrl Pts',(-24.5494784339386,14.2561019527568,
130.391287541648)) ;
#141363=CARTESIAN_POINT('Ctrl Pts',(-24.6041424746569,14.0742377640131,
130.584037902831)) ;
#141364=CARTESIAN_POINT('Ctrl Pts',(-24.6409425374017,13.8451949445008,
130.724693125171)) ;
#141365=CARTESIAN_POINT('Ctrl Pts',(-24.6564073870346,13.58674350493,130.802914286476)) ;
#141366=CARTESIAN_POINT('Ctrl Pts',(-24.648598332483,13.3144404098801,130.81341628994)) ;
#141367=CARTESIAN_POINT('Ctrl Pts',(-24.6176344680258,13.0528695222705,
130.755903610597)) ;
#141368=CARTESIAN_POINT('Ctrl Pts',(-24.5647644326536,12.8160517966369,
130.634605136453)) ;
#141369=CARTESIAN_POINT('Ctrl Pts',(-24.4928190367482,12.6226065253332,
130.457653206199)) ;
#141370=CARTESIAN_POINT('Ctrl Pts',(-24.4069484394412,12.4871996902566,
130.239845544222)) ;
#141371=CARTESIAN_POINT('Ctrl Pts',(-24.3114166195875,12.4184347650075,
129.994074210014)) ;
#141372=CARTESIAN_POINT('Ctrl Pts',(-24.2142170838312,12.4219001268695,
129.743022475508)) ;
#141373=CARTESIAN_POINT('Ctrl Pts',(-24.1195700162809,12.4968774725135,
129.499727012216)) ;
#141374=CARTESIAN_POINT('Ctrl Pts',(-24.0346625589609,12.6381726387492,
129.284784810722)) ;
#141375=CARTESIAN_POINT('Ctrl Pts',(-23.9643653426145,12.8360677562161,
129.112611003455)) ;
#141376=CARTESIAN_POINT('Ctrl Pts',(-23.9133140744109,13.0762566249802,
128.996657468451)) ;
#141377=CARTESIAN_POINT('Ctrl Pts',(-23.8844732807761,13.3398740968699,
128.945410468149)) ;
#141378=CARTESIAN_POINT('Ctrl Pts',(-23.8788261461933,13.6103044053491,
128.962027024672)) ;
#141379=CARTESIAN_POINT('Ctrl Pts',(-23.8963862756814,13.86812497933,129.046546801647)) ;
#141380=CARTESIAN_POINT('Ctrl Pts',(-23.9349997883254,14.0932871473164,
129.19246618752)) ;
#141381=CARTESIAN_POINT('Ctrl Pts',(-23.9913900660586,14.2707836651958,
129.390408363815)) ;
#141382=CARTESIAN_POINT('Ctrl Pts',(-24.060163393742,14.3866738498425,129.62429552567)) ;
#141383=CARTESIAN_POINT('Ctrl Pts',(-24.1363780076905,14.4343395644747,
129.880066368684)) ;
#141384=CARTESIAN_POINT('Ctrl Pts',(-24.2136312221482,14.4093417118186,
130.138889245811)) ;
#141385=CARTESIAN_POINT('Ctrl Pts',(-24.2855250652056,14.3139583253282,
130.382003572305)) ;
#141386=CARTESIAN_POINT('Ctrl Pts',(-24.3464841520355,14.1538396084722,
130.593328181351)) ;
#141387=CARTESIAN_POINT('Ctrl Pts',(-24.3907969417544,13.9434082094923,
130.755696634518)) ;
#141388=CARTESIAN_POINT('Ctrl Pts',(-24.4153872134604,13.6926166180059,
130.860902823485)) ;
#141389=CARTESIAN_POINT('Ctrl Pts',(-24.4170476036422,13.4252309557657,
130.898745794972)) ;
#141390=CARTESIAN_POINT('Ctrl Pts',(-24.3954087414857,13.15699249017,130.868626430046)) ;
#141391=CARTESIAN_POINT('Ctrl Pts',(-24.3510658797357,12.9074157483193,
130.772222097412)) ;
#141392=CARTESIAN_POINT('Ctrl Pts',(-24.2863589270511,12.6946405590363,
130.61638199744)) ;
#141393=CARTESIAN_POINT('Ctrl Pts',(-24.2058364240148,12.5348309265639,
130.414146669772)) ;
#141394=CARTESIAN_POINT('Ctrl Pts',(-24.1132237165813,12.4376124646164,
130.176911811757)) ;
#141395=CARTESIAN_POINT('Ctrl Pts',(-24.0160435387035,12.411847051691,129.926043454964)) ;
#141396=CARTESIAN_POINT('Ctrl Pts',(-23.9194951840902,12.4580456629596,
129.677111506706)) ;
#141397=CARTESIAN_POINT('Ctrl Pts',(-23.8299476378923,12.5736491425348,
129.44866350134)) ;
#141398=CARTESIAN_POINT('Ctrl Pts',(-23.7532981226229,12.7495592043743,
129.257815243214)) ;
#141399=CARTESIAN_POINT('Ctrl Pts',(-23.6938060546769,12.9753684252062,
129.117325067753)) ;
#141400=CARTESIAN_POINT('Ctrl Pts',(-23.655836225325,13.2312290478431,129.039409580857)) ;
#141401=CARTESIAN_POINT('Ctrl Pts',(-23.6407041156802,13.5022492390578,
129.028403475674)) ;
#141402=CARTESIAN_POINT('Ctrl Pts',(-23.6490347776743,13.766376795235,129.085779280314)) ;
#141403=CARTESIAN_POINT('Ctrl Pts',(-23.679347360503,14.0063277413084,129.20741315707)) ;
#141404=CARTESIAN_POINT('Ctrl Pts',(-23.7288783361076,14.2048736878869,
129.385229002076)) ;
#141405=CARTESIAN_POINT('Ctrl Pts',(-23.7935423808548,14.3476912358554,
129.607350754785)) ;
#141406=CARTESIAN_POINT('Ctrl Pts',(-23.8676082278984,14.4237776456092,
129.856845126396)) ;
#141407=CARTESIAN_POINT('Ctrl Pts',(-23.9452312757094,14.4280807671714,
130.116754966379)) ;
#141408=CARTESIAN_POINT('Ctrl Pts',(-24.0198127822077,14.3608278404858,
130.367644260992)) ;
#141409=CARTESIAN_POINT('Ctrl Pts',(-24.0859834375975,14.2256360028295,
130.59418483557)) ;
#141410=CARTESIAN_POINT('Ctrl Pts',(-24.1373843631784,14.0344799528452,
130.77728489612)) ;
#141411=CARTESIAN_POINT('Ctrl Pts',(-24.1704902224659,13.7980435581084,
130.907211792896)) ;
#141412=CARTESIAN_POINT('Ctrl Pts',(-24.181617086575,13.5353241773225,130.972828569372)) ;
#141413=CARTESIAN_POINT('Ctrl Pts',(-24.1694421615744,13.2644873700543,
130.970392633471)) ;
#141414=CARTESIAN_POINT('Ctrl Pts',(-24.1340736108702,13.0050528435928,
130.900194260651)) ;
#141415=CARTESIAN_POINT('Ctrl Pts',(-24.0772794060259,12.7754380039954,
130.767426952221)) ;
#141416=CARTESIAN_POINT('Ctrl Pts',(-24.0025528244517,12.592596001974,130.582218534765)) ;
#141417=CARTESIAN_POINT('Ctrl Pts',(-23.9145219022242,12.4690081971512,
130.358123680554)) ;
#141418=CARTESIAN_POINT('Ctrl Pts',(-23.8181204758606,12.4135709103977,
130.109761674319)) ;
#141419=CARTESIAN_POINT('Ctrl Pts',(-23.7207896010503,12.4306395059357,
129.858430292254)) ;
#141420=CARTESIAN_POINT('Ctrl Pts',(-23.6276243337301,12.5185475341995,
129.619406098751)) ;
#141421=CARTESIAN_POINT('Ctrl Pts',(-23.5449043158209,12.671844049154,129.410953733645)) ;
#141422=CARTESIAN_POINT('Ctrl Pts',(-23.4781856474444,12.8780302029366,
129.249096526566)) ;
#141423=CARTESIAN_POINT('Ctrl Pts',(-23.4309201247871,13.1252486430467,
129.144338143815)) ;
#141424=CARTESIAN_POINT('Ctrl Pts',(-23.406493307167,13.3909665765868,129.105916906452)) ;
#141425=CARTESIAN_POINT('Ctrl Pts',(-23.405312666089,13.6612161076759,129.135695199137)) ;
#141426=CARTESIAN_POINT('Ctrl Pts',(-23.4269936000131,13.9131568870817,
129.232093080542)) ;
#141427=CARTESIAN_POINT('Ctrl Pts',(-23.4692035971914,14.130438408173,129.388523345915)) ;
#141428=CARTESIAN_POINT('Ctrl Pts',(-23.5280845861359,14.2969775109189,
129.593597224986)) ;
#141429=CARTESIAN_POINT('Ctrl Pts',(-23.5993935198417,14.4015522166871,
129.835242815097)) ;
#141430=CARTESIAN_POINT('Ctrl Pts',(-23.675998443287,14.4350500551864,130.092020579583)) ;
#141431=CARTESIAN_POINT('Ctrl Pts',(-23.7525397078438,14.3967519658026,
130.348679751607)) ;
#141432=CARTESIAN_POINT('Ctrl Pts',(-23.8228714214555,14.2884849185217,
130.5872861249)) ;
#141433=CARTESIAN_POINT('Ctrl Pts',(-23.8810098442615,14.1181740873397,
130.790267409901)) ;
#141434=CARTESIAN_POINT('Ctrl Pts',(-23.922044787637,13.8977533327247,130.943313957249)) ;
#141435=CARTESIAN_POINT('Ctrl Pts',(-23.9422876471947,13.6446684520944,
131.035448870912)) ;
#141436=CARTESIAN_POINT('Ctrl Pts',(-23.9396680552135,13.3734340111263,
131.061088380113)) ;
#141437=CARTESIAN_POINT('Ctrl Pts',(-23.9134836273722,13.1072276556743,
131.017706686836)) ;
#141438=CARTESIAN_POINT('Ctrl Pts',(-23.8652358369202,12.8641925362022,
130.909786178128)) ;
#141439=CARTESIAN_POINT('Ctrl Pts',(-23.7973125355255,12.6605227447286,
130.744477407299)) ;
#141440=CARTESIAN_POINT('Ctrl Pts',(-23.7140967001381,12.511411732543,130.534451455081)) ;
#141441=CARTESIAN_POINT('Ctrl Pts',(-23.6198656680205,12.4272142071662,
130.292531553557)) ;
#141442=CARTESIAN_POINT('Ctrl Pts',(-23.522639981657,12.415034803424,130.041439124737)) ;
#141443=CARTESIAN_POINT('Ctrl Pts',(-23.4267624796708,12.474749132082,129.79453863735)) ;
#141444=CARTESIAN_POINT('Ctrl Pts',(-23.3392886616417,12.6023246098268,
129.572102763682)) ;
#141445=CARTESIAN_POINT('Ctrl Pts',(-23.26521460158,12.7898414639342,129.388996496963)) ;
#141446=CARTESIAN_POINT('Ctrl Pts',(-23.2100681969718,13.0206707820948,
129.260851722597)) ;
#141447=CARTESIAN_POINT('Ctrl Pts',(-23.1760485062128,13.2818518807112,
129.194659336828)) ;
#141448=CARTESIAN_POINT('Ctrl Pts',(-23.1654158714073,13.552127865025,129.196649551748)) ;
#141449=CARTESIAN_POINT('Ctrl Pts',(-23.1779469522343,13.8139569141608,
129.266397522322)) ;
#141450=CARTESIAN_POINT('Ctrl Pts',(-23.2124687860924,14.0485699408796,
129.400538385715)) ;
#141451=CARTESIAN_POINT('Ctrl Pts',(-23.2648627947572,14.2361101899088,
129.58649101522)) ;
#141452=CARTESIAN_POINT('Ctrl Pts',(-23.3319172217269,14.3675384217247,
129.81568463473)) ;
#141453=CARTESIAN_POINT('Ctrl Pts',(-23.4070931352948,14.4300942313948,
130.068399713215)) ;
#141454=CARTESIAN_POINT('Ctrl Pts',(-23.4843627263749,14.420886512356,130.327144314321)) ;
#141455=CARTESIAN_POINT('Ctrl Pts',(-23.5578964392717,14.3405660853883,
130.575037945399)) ;
#141456=CARTESIAN_POINT('Ctrl Pts',(-23.6218881748358,14.1934622330658,
130.795265313375)) ;
#141457=CARTESIAN_POINT('Ctrl Pts',(-23.6702413860333,13.9917021731483,
130.969631968682)) ;
#141458=CARTESIAN_POINT('Ctrl Pts',(-23.6991655434952,13.7502056369867,
131.087135180438)) ;
#141459=CARTESIAN_POINT('Ctrl Pts',(-23.706030166973,13.4844947151479,131.140309759337)) ;
#141460=CARTESIAN_POINT('Ctrl Pts',(-23.6894020057051,13.2141840714607,
131.124881280057)) ;
#141461=CARTESIAN_POINT('Ctrl Pts',(-23.6498448165609,12.958922795002,131.042450027368)) ;
#141462=CARTESIAN_POINT('Ctrl Pts',(-23.589051488531,12.7362702687102,130.898123427805)) ;
#141463=CARTESIAN_POINT('Ctrl Pts',(-23.5119547526697,12.5648474915298,
130.705761330521)) ;
#141464=CARTESIAN_POINT('Ctrl Pts',(-23.4214046717168,12.452872631945,130.474532293699)) ;
#141465=CARTESIAN_POINT('Ctrl Pts',(-23.3248409697496,12.41129419742,130.225470559134)) ;
#141466=CARTESIAN_POINT('Ctrl Pts',(-23.2273437603083,12.4419882083232,
129.973846467319)) ;
#141467=CARTESIAN_POINT('Ctrl Pts',(-23.1360177918426,12.5427027848013,
129.740097133431)) ;
#141468=CARTESIAN_POINT('Ctrl Pts',(-23.0559375842205,12.7067963976432,
129.539325291128)) ;
#141469=CARTESIAN_POINT('Ctrl Pts',(-22.9925343542045,12.9221001541686,
129.387231951601)) ;
#141470=CARTESIAN_POINT('Ctrl Pts',(-22.9494611772759,13.1741319902504,
129.294633889042)) ;
#141471=CARTESIAN_POINT('Ctrl Pts',(-22.9293237492918,13.4427023362762,
129.268862408672)) ;
#141472=CARTESIAN_POINT('Ctrl Pts',(-22.9326242894509,13.7107857212086,
129.311682353004)) ;
#141473=CARTESIAN_POINT('Ctrl Pts',(-22.9583033588113,13.956888330194,129.419685271958)) ;
#141474=CARTESIAN_POINT('Ctrl Pts',(-23.0040060644692,14.1661036929037,
129.586354227263)) ;
#141475=CARTESIAN_POINT('Ctrl Pts',(-23.0657731632118,14.3219385193613,
129.79996865813)) ;
#141476=CARTESIAN_POINT('Ctrl Pts',(-23.1381200326655,14.4130180852625,
130.044389910157)) ;
#141477=CARTESIAN_POINT('Ctrl Pts',(-23.2154893821187,14.4335349336769,
130.303544854118)) ;
#141478=CARTESIAN_POINT('Ctrl Pts',(-23.2917026997898,14.3810414218173,
130.559436531221)) ;
#141479=CARTESIAN_POINT('Ctrl Pts',(-23.3597411358198,14.2609490828525,
130.791144458003)) ;
#141480=CARTESIAN_POINT('Ctrl Pts',(-23.4151538663912,14.079534400134,130.986279889569)) ;
#141481=CARTESIAN_POINT('Ctrl Pts',(-23.4523380353655,13.8529283959852,
131.127860729194)) ;
#141482=CARTESIAN_POINT('Ctrl Pts',(-23.468524967232,13.5926907244754,131.208501026069)) ;
#141483=CARTESIAN_POINT('Ctrl Pts',(-23.4613879378508,13.3230678017147,
131.220637494974)) ;
#141484=CARTESIAN_POINT('Ctrl Pts',(-23.4310172633009,13.0595444653147,
131.165038572153)) ;
#141485=CARTESIAN_POINT('Ctrl Pts',(-23.3785101643465,12.8214089114898,
131.044865099349)) ;
#141486=CARTESIAN_POINT('Ctrl Pts',(-23.3071345050513,12.6270967453298,
130.869510720629)) ;
#141487=CARTESIAN_POINT('Ctrl Pts',(-23.2218885053547,12.4904301737517,
130.653416002948)) ;
#141488=CARTESIAN_POINT('Ctrl Pts',(-23.1268539668659,12.41952640959,130.408994465976)) ;
#141489=CARTESIAN_POINT('Ctrl Pts',(-23.0291669887329,12.4206998048116,
130.156680505045)) ;
#141490=CARTESIAN_POINT('Ctrl Pts',(-22.9342126331685,12.4940151693159,
129.912536358994)) ;
#141491=CARTESIAN_POINT('Ctrl Pts',(-22.8492111459651,12.6331734793058,
129.697224789051)) ;
#141492=CARTESIAN_POINT('Ctrl Pts',(-22.7784689920698,12.8293256852298,
129.523716827136)) ;
#141493=CARTESIAN_POINT('Ctrl Pts',(-22.7267830961436,13.0683012939604,
129.405890318511)) ;
#141494=CARTESIAN_POINT('Ctrl Pts',(-22.6971667052242,13.3322967725392,
129.352483196923)) ;
#141495=CARTESIAN_POINT('Ctrl Pts',(-22.6908974667905,13.6026350043085,
129.367260428482)) ;
#141496=CARTESIAN_POINT('Ctrl Pts',(-22.7077206912287,13.8605088968992,
129.44954355041)) ;
#141497=CARTESIAN_POINT('Ctrl Pts',(-22.7457980674478,14.0871784640944,
129.593944579997)) ;
#141498=CARTESIAN_POINT('Ctrl Pts',(-22.8015081236511,14.265834440122,129.789787245735)) ;
#141499=CARTESIAN_POINT('Ctrl Pts',(-22.8702580651156,14.3843789684771,
130.023754668897)) ;
#141500=CARTESIAN_POINT('Ctrl Pts',(-22.9465090739444,14.4339734265458,
130.279692171881)) ;
#141501=CARTESIAN_POINT('Ctrl Pts',(-23.0235969708249,14.4110559210102,
130.537938086999)) ;
#141502=CARTESIAN_POINT('Ctrl Pts',(-23.0956663651172,14.3178924901581,
130.781531217281)) ;
#141503=CARTESIAN_POINT('Ctrl Pts',(-23.1571514980903,14.1593686470185,
130.994439940708)) ;
#141504=CARTESIAN_POINT('Ctrl Pts',(-23.2020241924619,13.9496805218115,
131.158514572577)) ;
#141505=CARTESIAN_POINT('Ctrl Pts',(-23.2271393720092,13.7013469938743,
131.265044356128)) ;
#141506=CARTESIAN_POINT('Ctrl Pts',(-23.2295577349915,13.4330164717232,
131.305263682426)) ;
#141507=CARTESIAN_POINT('Ctrl Pts',(-23.2086111408663,13.1647607715786,
131.277127741886)) ;
#141508=CARTESIAN_POINT('Ctrl Pts',(-23.1647278376412,12.9137312008662,
131.18216641284)) ;
#141509=CARTESIAN_POINT('Ctrl Pts',(-23.1009545230825,12.7007529783777,
131.028861056442)) ;
#141510=CARTESIAN_POINT('Ctrl Pts',(-23.0203445087878,12.5383275920807,
130.826577670387)) ;
#141511=CARTESIAN_POINT('Ctrl Pts',(-22.9287530034321,12.4398166111486,
130.59204481027)) ;
#141512=CARTESIAN_POINT('Ctrl Pts',(-22.8308357993991,12.4114725010168,
130.339306419179)) ;
#141513=CARTESIAN_POINT('Ctrl Pts',(-22.7343885893122,12.4557968950616,
130.090594438971)) ;
#141514=CARTESIAN_POINT('Ctrl Pts',(-22.644462571658,12.569629101587,129.861079793437)) ;
#141515=CARTESIAN_POINT('Ctrl Pts',(-22.5675688072916,12.7436129687706,
129.669441199026)) ;
#141516=CARTESIAN_POINT('Ctrl Pts',(-22.5074742150958,12.9681022843807,
129.527185830781)) ;
#141517=CARTESIAN_POINT('Ctrl Pts',(-22.468793772561,13.2239471753799,129.447276223009)) ;
#141518=CARTESIAN_POINT('Ctrl Pts',(-22.4530382205004,13.4941633310118,
129.434364446316)) ;
#141519=CARTESIAN_POINT('Ctrl Pts',(-22.4606774149823,13.7589186956337,
129.489743991273)) ;
#141520=CARTESIAN_POINT('Ctrl Pts',(-22.4903861345707,13.9998349614895,
129.609611812731)) ;
#141521=CARTESIAN_POINT('Ctrl Pts',(-22.5394138503083,14.1997646891006,
129.785956045042)) ;
#141522=CARTESIAN_POINT('Ctrl Pts',(-22.6035812001282,14.344263749604,130.006567187812)) ;
#141523=CARTESIAN_POINT('Ctrl Pts',(-22.6775949801385,14.4224928496146,
130.255978432946)) ;
#141524=CARTESIAN_POINT('Ctrl Pts',(-22.7548151168621,14.4291711030004,
130.514539462714)) ;
#141525=CARTESIAN_POINT('Ctrl Pts',(-22.8301186292218,14.3636108427049,
130.767784158612)) ;
#141526=CARTESIAN_POINT('Ctrl Pts',(-22.8963852155264,14.2305640728087,
130.994488176039)) ;
#141527=CARTESIAN_POINT('Ctrl Pts',(-22.9483632007256,14.0406274763076,
131.179334305198)) ;
#141528=CARTESIAN_POINT('Ctrl Pts',(-22.9819990811783,13.8058698761943,
131.310720597295)) ;
#141529=CARTESIAN_POINT('Ctrl Pts',(-22.9938487433692,13.5427807142404,
131.378566461829)) ;
#141530=CARTESIAN_POINT('Ctrl Pts',(-22.9823232445732,13.2720604281958,
131.378004543633)) ;
#141531=CARTESIAN_POINT('Ctrl Pts',(-22.9475403030834,13.0118428173477,
131.309548132463)) ;
#141532=CARTESIAN_POINT('Ctrl Pts',(-22.8915112375159,12.7818787427455,
131.178906192752)) ;
#141533=CARTESIAN_POINT('Ctrl Pts',(-22.8171006460482,12.5968716108038,
130.994704335963)) ;
#141534=CARTESIAN_POINT('Ctrl Pts',(-22.7289778755317,12.4712516936664,
130.770472889898)) ;
#141535=CARTESIAN_POINT('Ctrl Pts',(-22.6331833007374,12.4142247915804,
130.523717556835)) ;
#141536=CARTESIAN_POINT('Ctrl Pts',(-22.5356508064631,12.4291610555867,
130.271854319525)) ;
#141537=CARTESIAN_POINT('Ctrl Pts',(-22.4422219359673,12.5152749819563,
130.032078417929)) ;
#141538=CARTESIAN_POINT('Ctrl Pts',(-22.3590404214073,12.6672522728085,
129.822327141258)) ;
#141539=CARTESIAN_POINT('Ctrl Pts',(-22.2921309701618,12.8714563958125,
129.659787658127)) ;
#141540=CARTESIAN_POINT('Ctrl Pts',(-22.2443651596895,13.1164156857726,
129.553405831915)) ;
#141541=CARTESIAN_POINT('Ctrl Pts',(-22.2190474781447,13.3833143982509,
129.512577304851)) ;
#141542=CARTESIAN_POINT('Ctrl Pts',(-22.2172540043482,13.6536761836367,
129.540554196584)) ;
#141543=CARTESIAN_POINT('Ctrl Pts',(-22.2382590501835,13.9063303712051,
129.634966454425)) ;
#141544=CARTESIAN_POINT('Ctrl Pts',(-22.2801563660598,14.1256565234766,
129.790623681986)) ;
#141545=CARTESIAN_POINT('Ctrl Pts',(-22.3384585173566,14.2929703987116,
129.993882288025)) ;
#141546=CARTESIAN_POINT('Ctrl Pts',(-22.4093200906847,14.3994043098715,
130.2341478642)) ;
#141547=CARTESIAN_POINT('Ctrl Pts',(-22.4859751155258,14.4351253202518,
130.491131868344)) ;
#141548=CARTESIAN_POINT('Ctrl Pts',(-22.5626631024897,14.3988243976867,
130.748241624642)) ;
#141549=CARTESIAN_POINT('Ctrl Pts',(-22.6332742180642,14.2923293350233,
130.987677581832)) ;
#141550=CARTESIAN_POINT('Ctrl Pts',(-22.6916546156017,14.1241731198379,
131.191265009288)) ;
#141551=CARTESIAN_POINT('Ctrl Pts',(-22.7333193090981,13.9051613921294,
131.346148949701)) ;
#141552=CARTESIAN_POINT('Ctrl Pts',(-22.754233227271,13.6518311296983,131.440367694437)) ;
#141553=CARTESIAN_POINT('Ctrl Pts',(-22.7523181442158,13.382470855745,131.467858526285)) ;
#141554=CARTESIAN_POINT('Ctrl Pts',(-22.7269194037075,13.1154253093326,
131.426820533837)) ;
#141555=CARTESIAN_POINT('Ctrl Pts',(-22.6790960766581,12.870532627165,131.320267211323)) ;
#141556=CARTESIAN_POINT('Ctrl Pts',(-22.6116784390235,12.6655370623813,
131.156430120632)) ;
#141557=CARTESIAN_POINT('Ctrl Pts',(-22.52866080056,12.5146112144562,130.947041423206)) ;
#141558=CARTESIAN_POINT('Ctrl Pts',(-22.4352111334049,12.4289101805898,
130.707203534422)) ;
#141559=CARTESIAN_POINT('Ctrl Pts',(-22.337805695785,12.414189675376,130.455660644508)) ;
#141560=CARTESIAN_POINT('Ctrl Pts',(-22.2412613487243,12.4724108843215,
130.206994597826)) ;
#141561=CARTESIAN_POINT('Ctrl Pts',(-22.1539421150866,12.5978142660017,
129.984853113308)) ;
#141562=CARTESIAN_POINT('Ctrl Pts',(-22.0796465742663,12.7826552616513,
129.800950294926)) ;
#141563=CARTESIAN_POINT('Ctrl Pts',(-22.023580811912,13.0133815728599,129.670279883198)) ;
#141564=CARTESIAN_POINT('Ctrl Pts',(-21.9889019749618,13.2742169731993,
129.602185597382)) ;
#141565=CARTESIAN_POINT('Ctrl Pts',(-21.9776007628016,13.5450315924184,
129.602290461137)) ;
#141566=CARTESIAN_POINT('Ctrl Pts',(-21.9895371136341,13.8067212996898,
129.670228891093)) ;
#141567=CARTESIAN_POINT('Ctrl Pts',(-22.0231669037331,14.041251387199,129.801572991707)) ;
#141568=CARTESIAN_POINT('Ctrl Pts',(-22.0754464617893,14.2318697837458,
129.987445935215)) ;
#141569=CARTESIAN_POINT('Ctrl Pts',(-22.1420538141681,14.3645253457052,
130.215247583402)) ;
#141570=CARTESIAN_POINT('Ctrl Pts',(-22.2167456177527,14.4291513856489,
130.466420736451)) ;
#141571=CARTESIAN_POINT('Ctrl Pts',(-22.2943374241322,14.4223448074479,
130.72622892334)) ;
#141572=CARTESIAN_POINT('Ctrl Pts',(-22.3683124218705,14.3433927947591,
130.975537803221)) ;
#141573=CARTESIAN_POINT('Ctrl Pts',(-22.4321443929052,14.1993296986607,
131.195019796695)) ;
#141574=CARTESIAN_POINT('Ctrl Pts',(-22.4812301514825,13.9988089965648,
131.37161097718)) ;
#141575=CARTESIAN_POINT('Ctrl Pts',(-22.5108552207397,13.7578101300497,
131.491222506074)) ;
#141576=CARTESIAN_POINT('Ctrl Pts',(-22.5183507639506,13.4916490682303,
131.546347903552)) ;
#141577=CARTESIAN_POINT('Ctrl Pts',(-22.5024688288655,13.2223242995655,
131.532955842147)) ;
#141578=CARTESIAN_POINT('Ctrl Pts',(-22.4634550439045,12.9657468504133,
131.452199654102)) ;
#141579=CARTESIAN_POINT('Ctrl Pts',(-22.4035858370445,12.7429296521264,
131.310396045604)) ;
#141580=CARTESIAN_POINT('Ctrl Pts',(-22.3264011259672,12.5685157086448,
131.118018720655)) ;
#141581=CARTESIAN_POINT('Ctrl Pts',(-22.2361039633969,12.4549912632195,
130.887515775926)) ;
#141582=CARTESIAN_POINT('Ctrl Pts',(-22.1398503506461,12.4115665136302,
130.639293430357)) ;
#141583=CARTESIAN_POINT('Ctrl Pts',(-22.0424886926386,12.4399153720153,
130.387988889265)) ;
#141584=CARTESIAN_POINT('Ctrl Pts',(-21.9504297608399,12.5392662733084,
130.152276377526)) ;
#141585=CARTESIAN_POINT('Ctrl Pts',(-21.8701710273988,12.7015765304021,
129.950908606138)) ;
#141586=CARTESIAN_POINT('Ctrl Pts',(-21.8063861498009,12.9151235302472,
129.79762998674)) ;
#141587=CARTESIAN_POINT('Ctrl Pts',(-21.7626992958939,13.1655123638567,
129.7031400661)) ;
#141588=CARTESIAN_POINT('Ctrl Pts',(-21.7417530497949,13.4357073085102,
129.675239571074)) ;
#141589=CARTESIAN_POINT('Ctrl Pts',(-21.7444138523188,13.7027427406616,
129.716020384392)) ;
#141590=CARTESIAN_POINT('Ctrl Pts',(-21.7694841131605,13.9504288317899,
129.822336426841)) ;
#141591=CARTESIAN_POINT('Ctrl Pts',(-21.8147174623756,14.1608971109305,
129.987638494224)) ;
#141592=CARTESIAN_POINT('Ctrl Pts',(-21.8759731008052,14.3182076735822,
130.199701107976)) ;
#141593=CARTESIAN_POINT('Ctrl Pts',(-21.94820436243,14.4114239786406,130.443837263751)) ;
#141594=CARTESIAN_POINT('Ctrl Pts',(-22.0253654620152,14.4338711414245,
130.702320259921)) ;
#141595=CARTESIAN_POINT('Ctrl Pts',(-22.101528389536,14.3839736196214,130.957971280896)) ;
#141596=CARTESIAN_POINT('Ctrl Pts',(-22.1703041063366,14.2649033535115,
131.192056246532)) ;
#141597=CARTESIAN_POINT('Ctrl Pts',(-22.2258355288632,14.0862372824977,
131.387321343928)) ;
#141598=CARTESIAN_POINT('Ctrl Pts',(-22.2638301112426,13.8593709017047,
131.531485753709)) ;
#141599=CARTESIAN_POINT('Ctrl Pts',(-22.2805485096342,13.6016401376878,
131.613431621248)) ;
#141600=CARTESIAN_POINT('Ctrl Pts',(-22.2741762775947,13.3309240386314,
131.627952992157)) ;
#141601=CARTESIAN_POINT('Ctrl Pts',(-22.2444251317103,13.0670232558749,
131.574151442485)) ;
#141602=CARTESIAN_POINT('Ctrl Pts',(-22.1927412324025,12.828626100883,131.456273734189)) ;
#141603=CARTESIAN_POINT('Ctrl Pts',(-22.1219393925841,12.6324568485675,
131.282604017312)) ;
#141604=CARTESIAN_POINT('Ctrl Pts',(-22.0364918031217,12.4932133187338,
131.066128009462)) ;
#141605=CARTESIAN_POINT('Ctrl Pts',(-21.9420804492648,12.4206918000049,
130.823366652621)) ;
#141606=CARTESIAN_POINT('Ctrl Pts',(-21.8440805767233,12.4196226873693,
130.57024775875)) ;
#141607=CARTESIAN_POINT('Ctrl Pts',(-21.7490173808445,12.491015534073,130.325762328134)) ;
#141608=CARTESIAN_POINT('Ctrl Pts',(-21.6636415900144,12.6283740411058,
130.109366250709)) ;
#141609=CARTESIAN_POINT('Ctrl Pts',(-21.5922515959559,12.8237070115403,
129.934053660651)) ;
#141610=CARTESIAN_POINT('Ctrl Pts',(-21.5401084835492,13.061674988434,129.814868123476)) ;
#141611=CARTESIAN_POINT('Ctrl Pts',(-21.509952988586,13.32403831549,129.759742423784)) ;
#141612=CARTESIAN_POINT('Ctrl Pts',(-21.5029347827011,13.5952494532198,
129.772427265086)) ;
#141613=CARTESIAN_POINT('Ctrl Pts',(-21.5192500283624,13.8544595639362,
129.853324509009)) ;
#141614=CARTESIAN_POINT('Ctrl Pts',(-21.5567750983994,14.0816540138682,
129.996049680023)) ;
#141615=CARTESIAN_POINT('Ctrl Pts',(-21.6118539418553,14.2612880227879,
130.189940873468)) ;
#141616=CARTESIAN_POINT('Ctrl Pts',(-21.6802614176699,14.3817634541805,
130.422897734711)) ;
#141617=CARTESIAN_POINT('Ctrl Pts',(-21.7564021182027,14.4336477376616,
130.678521217963)) ;
#141618=CARTESIAN_POINT('Ctrl Pts',(-21.8339810050049,14.4124733819028,
130.938391467335)) ;
#141619=CARTESIAN_POINT('Ctrl Pts',(-21.9058535221447,14.3214777204803,
131.181230646715)) ;
#141620=CARTESIAN_POINT('Ctrl Pts',(-21.9677099575383,14.1652192318908,
131.39517300608)) ;
#141621=CARTESIAN_POINT('Ctrl Pts',(-22.0133194373746,13.955565015999,131.56158746004)) ;
#141622=CARTESIAN_POINT('Ctrl Pts',(-22.0388748975272,13.709559951643,131.669199572757)) ;
#141623=CARTESIAN_POINT('Ctrl Pts',(-22.0420741504065,13.4405995053874,
131.711821411861)) ;
#141624=CARTESIAN_POINT('Ctrl Pts',(-22.0216068001038,13.1715077449996,
131.685166293291)) ;
#141625=CARTESIAN_POINT('Ctrl Pts',(-21.9787370922207,12.9214880577471,
131.592913543069)) ;
#141626=CARTESIAN_POINT('Ctrl Pts',(-21.9150051439039,12.7055052948916,
131.439997533155)) ;
#141627=CARTESIAN_POINT('Ctrl Pts',(-21.8352330897024,12.5425196624815,
131.239962285351)) ;
#141628=CARTESIAN_POINT('Ctrl Pts',(-21.7437059672795,12.4416160232308,
131.005700049378)) ;
#141629=CARTESIAN_POINT('Ctrl Pts',(-21.6457837150915,12.4112449643292,
130.752967238567)) ;
#141630=CARTESIAN_POINT('Ctrl Pts',(-21.5491572309789,12.4537097251659,
130.503762395268)) ;
#141631=CARTESIAN_POINT('Ctrl Pts',(-21.4592496415054,12.5652232898652,
130.274186604649)) ;
#141632=CARTESIAN_POINT('Ctrl Pts',(-21.3817509969093,12.7379440423451,
130.080854279824)) ;
#141633=CARTESIAN_POINT('Ctrl Pts',(-21.3213005288273,12.9603974854775,
129.93743655005)) ;
#141634=CARTESIAN_POINT('Ctrl Pts',(-21.2818676200916,13.2156635264027,
129.855358038676)) ;
#141635=CARTESIAN_POINT('Ctrl Pts',(-21.2653674335359,13.4857934304202,
129.840276750867)) ;
#141636=CARTESIAN_POINT('Ctrl Pts',(-21.2723658021236,13.7522947042676,
129.893946458855)) ;
#141637=CARTESIAN_POINT('Ctrl Pts',(-21.3016583192635,13.9943545056691,
130.012656591767)) ;
#141638=CARTESIAN_POINT('Ctrl Pts',(-21.3499698414391,14.1947046686213,
130.186750048278)) ;
#141639=CARTESIAN_POINT('Ctrl Pts',(-21.4140663653601,14.341452975733,130.407297870891)) ;
#141640=CARTESIAN_POINT('Ctrl Pts',(-21.4875277289265,14.4211243225131,
130.654924218185)) ;
#141641=CARTESIAN_POINT('Ctrl Pts',(-21.5648853083263,14.4300014254347,
130.913958649016)) ;
#141642=CARTESIAN_POINT('Ctrl Pts',(-21.6402056432869,14.3664765373256,
131.167191277808)) ;
#141643=CARTESIAN_POINT('Ctrl Pts',(-21.7067619878926,14.2356051810154,
131.394704769089)) ;
#141644=CARTESIAN_POINT('Ctrl Pts',(-21.7594400160825,14.0463420011333,
131.581735837121)) ;
#141645=CARTESIAN_POINT('Ctrl Pts',(-21.7935313335368,13.8127311118514,
131.714417517825)) ;
#141646=CARTESIAN_POINT('Ctrl Pts',(-21.8060449730169,13.5514860506215,
131.784043231233)) ;
#141647=CARTESIAN_POINT('Ctrl Pts',(-21.7951988407191,13.2797430818136,
131.785591184551)) ;
#141648=CARTESIAN_POINT('Ctrl Pts',(-21.7611775488476,13.0196140734991,
131.719268505353)) ;
#141649=CARTESIAN_POINT('Ctrl Pts',(-21.7055614368075,12.7876901355889,
131.589951267005)) ;
#141650=CARTESIAN_POINT('Ctrl Pts',(-21.6316783355603,12.6015317076786,
131.407244042403)) ;
#141651=CARTESIAN_POINT('Ctrl Pts',(-21.5441542981735,12.474259722316,131.18466789139)) ;
#141652=CARTESIAN_POINT('Ctrl Pts',(-21.4483951831579,12.41484596922,130.9380604683)) ;
#141653=CARTESIAN_POINT('Ctrl Pts',(-21.3505626518937,12.4277168198839,
130.685407749088)) ;
#141654=CARTESIAN_POINT('Ctrl Pts',(-21.257021209583,12.511951186466,130.44527777759)) ;
#141655=CARTESIAN_POINT('Ctrl Pts',(-21.1737647731563,12.6612551341691,
130.235160872959)) ;
#141656=CARTESIAN_POINT('Ctrl Pts',(-21.1058496345299,12.8654798246469,
130.069918745711)) ;
#141657=CARTESIAN_POINT('Ctrl Pts',(-21.0576927996032,13.1088716253824,
129.962286476496)) ;
#141658=CARTESIAN_POINT('Ctrl Pts',(-21.0316738007053,13.3752799217244,
129.919402371251)) ;
#141659=CARTESIAN_POINT('Ctrl Pts',(-21.0291742667073,13.6458120251598,
129.945308637888)) ;
#141660=CARTESIAN_POINT('Ctrl Pts',(-21.0495914487314,13.8994658312756,
130.03804637563)) ;
#141661=CARTESIAN_POINT('Ctrl Pts',(-21.0907109338922,14.1192749080617,
130.191292315407)) ;
#141662=CARTESIAN_POINT('Ctrl Pts',(-21.1488908973672,14.2891803120814,
130.394377389492)) ;
#141663=CARTESIAN_POINT('Ctrl Pts',(-21.2191618432277,14.3970324954729,
130.632758726818)) ;
#141664=CARTESIAN_POINT('Ctrl Pts',(-21.2958745043866,14.4351164738745,
130.889987430257)) ;
#141665=CARTESIAN_POINT('Ctrl Pts',(-21.3725867221997,14.4010787693592,
131.147130087852)) ;
#141666=CARTESIAN_POINT('Ctrl Pts',(-21.4438617427851,14.2958209261601,
131.388700881301)) ;
#141667=CARTESIAN_POINT('Ctrl Pts',(-21.5023962179495,14.1296521769512,
131.592620659444)) ;
#141668=CARTESIAN_POINT('Ctrl Pts',(-21.5446003436252,13.9121761365587,
131.749049810147)) ;
#141669=CARTESIAN_POINT('Ctrl Pts',(-21.5661428686401,13.6594303450515,
131.845126015287)) ;
#141670=CARTESIAN_POINT('Ctrl Pts',(-21.56497049185,13.3906473022496,131.874737745289)) ;
#141671=CARTESIAN_POINT('Ctrl Pts',(-21.5399924692855,13.1215485534994,
131.835149711464)) ;
#141672=CARTESIAN_POINT('Ctrl Pts',(-21.4930581932203,12.8774994745799,
131.730962916876)) ;
#141673=CARTESIAN_POINT('Ctrl Pts',(-21.4258817768746,12.6702279287505,
131.567977187413)) ;
#141674=CARTESIAN_POINT('Ctrl Pts',(-21.3435607012276,12.5183910310168,
131.360480560169)) ;
#141675=CARTESIAN_POINT('Ctrl Pts',(-21.2503256342203,12.4302683036152,
131.121283015252)) ;
#141676=CARTESIAN_POINT('Ctrl Pts',(-21.1522563402183,12.4138255898749,
130.868039774348)) ;
#141677=CARTESIAN_POINT('Ctrl Pts',(-21.0567790567561,12.4692849906945,
130.622070654961)) ;
#141678=CARTESIAN_POINT('Ctrl Pts',(-20.9685110583371,12.593086865603,130.397368234412)) ;
#141679=CARTESIAN_POINT('Ctrl Pts',(-20.8936229110052,12.7771359957172,
130.211819511284)) ;
#141680=CARTESIAN_POINT('Ctrl Pts',(-20.8371932849537,13.0059650352549,
130.079970640227)) ;
#141681=CARTESIAN_POINT('Ctrl Pts',(-20.8018184496472,13.2661472489738,
130.009842797586)) ;
#141682=CARTESIAN_POINT('Ctrl Pts',(-20.7897983193479,13.5369907136561,
130.007852540205)) ;
#141683=CARTESIAN_POINT('Ctrl Pts',(-20.8011200549456,13.7997449792612,
130.074069304931)) ;
#141684=CARTESIAN_POINT('Ctrl Pts',(-20.8341135563802,14.0350784316614,
130.20351194695)) ;
#141685=CARTESIAN_POINT('Ctrl Pts',(-20.8861785126658,14.2276701569779,
130.388889073528)) ;
#141686=CARTESIAN_POINT('Ctrl Pts',(-20.9518178159271,14.3610391391533,
130.613550792557)) ;
#141687=CARTESIAN_POINT('Ctrl Pts',(-21.0269503603294,14.4285213682471,
130.866293340862)) ;
#141688=CARTESIAN_POINT('Ctrl Pts',(-21.1043928575752,14.4233691347863,
131.125594261652)) ;
#141689=CARTESIAN_POINT('Ctrl Pts',(-21.1783654730741,14.3469900200021,
131.374791937787)) ;
#141690=CARTESIAN_POINT('Ctrl Pts',(-21.2429999211689,14.2034039230656,
131.596873955724)) ;
#141691=CARTESIAN_POINT('Ctrl Pts',(-21.2921913933265,14.0056847317555,
131.773520365113)) ;
#141692=CARTESIAN_POINT('Ctrl Pts',(-21.3225583436973,13.7644934618712,
131.895469292107)) ;
#141693=CARTESIAN_POINT('Ctrl Pts',(-21.3307101633366,13.5002463021735,
131.952315969993)) ;
#141694=CARTESIAN_POINT('Ctrl Pts',(-21.3152981248906,13.2284057614088,
131.940601853759)) ;
#141695=CARTESIAN_POINT('Ctrl Pts',(-21.2772947936541,12.9739037003026,
131.862437607203)) ;
#141696=CARTESIAN_POINT('Ctrl Pts',(-21.2177347936152,12.7484703827135,
131.721732709268)) ;
#141697=CARTESIAN_POINT('Ctrl Pts',(-21.1412095546896,12.5731123065293,
131.531169542656)) ;
#141698=CARTESIAN_POINT('Ctrl Pts',(-21.0511537422027,12.4573590720307,
131.301405138449)) ;
#141699=CARTESIAN_POINT('Ctrl Pts',(-20.9549127769704,12.4118025437708,
131.053250585454)) ;
#141700=CARTESIAN_POINT('Ctrl Pts',(-20.8574614565724,12.4381298316287,
130.80169464533)) ;
#141701=CARTESIAN_POINT('Ctrl Pts',(-20.7653175667387,12.5352056674708,
130.565667200803)) ;
#141702=CARTESIAN_POINT('Ctrl Pts',(-20.6844201407059,12.6963006126537,
130.362534236826)) ;
#141703=CARTESIAN_POINT('Ctrl Pts',(-20.6201460569402,12.9082756109017,
130.207782417921)) ;
#141704=CARTESIAN_POINT('Ctrl Pts',(-20.5756916195102,13.1596325292673,
130.111270821457)) ;
#141705=CARTESIAN_POINT('Ctrl Pts',(-20.5543454783755,13.4259468803236,
130.08175038831)) ;
#141706=CARTESIAN_POINT('Ctrl Pts',(-20.5561837783325,13.6953761001562,
130.120387060139)) ;
#141707=CARTESIAN_POINT('Ctrl Pts',(-20.5806872762992,13.943717027651,130.225025251255)) ;
#141708=CARTESIAN_POINT('Ctrl Pts',(-20.625436887015,14.1557110892649,130.388952831254)) ;
#141709=CARTESIAN_POINT('Ctrl Pts',(-20.6861966494772,14.3144000289701,
130.599504747278)) ;
#141710=CARTESIAN_POINT('Ctrl Pts',(-20.7581576601897,14.4096307928531,
130.842844416002)) ;
#141711=CARTESIAN_POINT('Ctrl Pts',(-20.8352840260227,14.4343455409311,
131.10123283597)) ;
#141712=CARTESIAN_POINT('Ctrl Pts',(-20.9118812127441,14.3860725213322,
131.358298311597)) ;
#141713=CARTESIAN_POINT('Ctrl Pts',(-20.9805602529552,14.269509697164,131.591910200073)) ;
#141714=CARTESIAN_POINT('Ctrl Pts',(-21.0367672235713,14.0917907400684,
131.789281437755)) ;
#141715=CARTESIAN_POINT('Ctrl Pts',(-21.0751892066154,13.8666926815631,
131.934591885575)) ;
#141716=CARTESIAN_POINT('Ctrl Pts',(-21.0926069855701,13.6093228235484,
132.01862592531)) ;
#141717=CARTESIAN_POINT('Ctrl Pts',(-21.0869107246577,13.3388431242067,
132.035103126594)) ;
#141718=CARTESIAN_POINT('Ctrl Pts',(-21.0577918123157,13.0740473551912,
131.983200390998)) ;
#141719=CARTESIAN_POINT('Ctrl Pts',(-21.0065423484218,12.834394570963,131.86664775222)) ;
#141720=CARTESIAN_POINT('Ctrl Pts',(-20.9365832563614,12.6378258855697,
131.695270728272)) ;
#141721=CARTESIAN_POINT('Ctrl Pts',(-20.851496423393,12.4964629704439,131.479866074815)) ;
#141722=CARTESIAN_POINT('Ctrl Pts',(-20.7570110239039,12.4217253903026,
131.236976112388)) ;
#141723=CARTESIAN_POINT('Ctrl Pts',(-20.6591190008919,12.4187226329277,
130.984139850466)) ;
#141724=CARTESIAN_POINT('Ctrl Pts',(-20.5641946923653,12.4875916931866,
130.739941516333)) ;
#141725=CARTESIAN_POINT('Ctrl Pts',(-20.4781247909421,12.6235712974209,
130.521647673819)) ;
#141726=CARTESIAN_POINT('Ctrl Pts',(-20.4065158080652,12.8167008380917,
130.34556952621)) ;
#141727=CARTESIAN_POINT('Ctrl Pts',(-20.353643746356,13.053470182096,130.224259441503)) ;
#141728=CARTESIAN_POINT('Ctrl Pts',(-20.3226739885955,13.3166530721009,
130.166917618502)) ;
#141729=CARTESIAN_POINT('Ctrl Pts',(-20.31505675572,13.5871782516177,130.177762255202)) ;
#141730=CARTESIAN_POINT('Ctrl Pts',(-20.3305496502409,13.8461111103248,
130.256130093167)) ;
#141731=CARTESIAN_POINT('Ctrl Pts',(-20.3675394662945,14.0754123777246,
130.39740594318)) ;
#141732=CARTESIAN_POINT('Ctrl Pts',(-20.4223028531838,14.2569965796042,
130.590449980248)) ;
#141733=CARTESIAN_POINT('Ctrl Pts',(-20.4904071207389,14.3792169528627,
130.822514938853)) ;
#141734=CARTESIAN_POINT('Ctrl Pts',(-20.566188380446,14.4330645797171,131.076992557233)) ;
#141735=CARTESIAN_POINT('Ctrl Pts',(-20.6438055884923,14.4142942026361,
131.33696737981)) ;
#141736=CARTESIAN_POINT('Ctrl Pts',(-20.7162101331673,14.3249818434921,
131.581491579565)) ;
#141737=CARTESIAN_POINT('Ctrl Pts',(-20.7784436604938,14.1700409218133,
131.796566267309)) ;
#141738=CARTESIAN_POINT('Ctrl Pts',(-20.8243668704006,13.9629928676694,
131.963710597949)) ;
#141739=CARTESIAN_POINT('Ctrl Pts',(-20.8506930176227,13.7164972263621,
132.073761907779)) ;
#141740=CARTESIAN_POINT('Ctrl Pts',(-20.8545193223202,13.4493823729498,
132.118023584794)) ;
#141741=CARTESIAN_POINT('Ctrl Pts',(-20.8348338544616,13.1794660077169,
132.093719529633)) ;
#141742=CARTESIAN_POINT('Ctrl Pts',(-20.7922850460746,12.9274139547086,
132.002579999831)) ;
#141743=CARTESIAN_POINT('Ctrl Pts',(-20.7294326898175,12.7115777217288,
131.852035109273)) ;
#141744=CARTESIAN_POINT('Ctrl Pts',(-20.6500828954979,12.5463884356972,
131.653264061087)) ;
#141745=CARTESIAN_POINT('Ctrl Pts',(-20.5580314056843,12.443178693002,131.417734074908)) ;
#141746=CARTESIAN_POINT('Ctrl Pts',(-20.4612577062668,12.4112124572602,
131.167987088684)) ;
#141747=CARTESIAN_POINT('Ctrl Pts',(-20.3641429989321,12.4513454619086,
130.917486650805)) ;
#141748=CARTESIAN_POINT('Ctrl Pts',(-20.2739798213262,12.5610016946322,
130.68715458049)) ;
#141749=CARTESIAN_POINT('Ctrl Pts',(-20.1959506857722,12.732231543376,130.492309746088)) ;
#141750=CARTESIAN_POINT('Ctrl Pts',(-20.1349366415907,12.9536822141676,
130.347265673142)) ;
#141751=CARTESIAN_POINT('Ctrl Pts',(-20.0949452207664,13.2077095887355,
130.263487892895)) ;
#141752=CARTESIAN_POINT('Ctrl Pts',(-20.0777170362633,13.4778390375596,
130.246299373488)) ;
#141753=CARTESIAN_POINT('Ctrl Pts',(-20.0840738202005,13.7447250723396,
130.298098443837)) ;
#141754=CARTESIAN_POINT('Ctrl Pts',(-20.1125804674209,13.9871379837623,
130.414408057966)) ;
#141755=CARTESIAN_POINT('Ctrl Pts',(-20.1607218878349,14.1900737145365,
130.588221394981)) ;
#141756=CARTESIAN_POINT('Ctrl Pts',(-20.2238417477086,14.3373318040479,
130.805602937382)) ;
#141757=CARTESIAN_POINT('Ctrl Pts',(-20.2975436467262,14.419933546752,131.054158219114)) ;
#141758=CARTESIAN_POINT('Ctrl Pts',(-20.3748646623211,14.4307823852778,
131.313069914816)) ;
#141759=CARTESIAN_POINT('Ctrl Pts',(-20.4505258413519,14.3690285004678,
131.567389143133)) ;
#141760=CARTESIAN_POINT('Ctrl Pts',(-20.5171200124224,14.2404409367686,
131.794874654969)) ;
#141761=CARTESIAN_POINT('Ctrl Pts',(-20.5703141964463,14.0528075419849,
131.983419808591)) ;
#141762=CARTESIAN_POINT('Ctrl Pts',(-20.6050441603483,13.8202654365076,
132.117973841072)) ;
#141763=CARTESIAN_POINT('Ctrl Pts',(-20.618242473377,13.5584443869878,132.189739585417)) ;
#141764=CARTESIAN_POINT('Ctrl Pts',(-20.6079944099217,13.2871049531719,
132.19298418131)) ;
#141765=CARTESIAN_POINT('Ctrl Pts',(-20.5747375359983,13.0271135604128,
132.128804556313)) ;
#141766=CARTESIAN_POINT('Ctrl Pts',(-20.519668667754,12.7938647144907,132.001118490825)) ;
#141767=CARTESIAN_POINT('Ctrl Pts',(-20.4463534609398,12.6063347659711,
131.820031027545)) ;
#141768=CARTESIAN_POINT('Ctrl Pts',(-20.3590134924532,12.4770287601625,
131.598047664409)) ;
#141769=CARTESIAN_POINT('Ctrl Pts',(-20.2636906192186,12.4155889088205,
131.352615933497)) ;
#141770=CARTESIAN_POINT('Ctrl Pts',(-20.16538161851,12.4264045930434,131.098726664761)) ;
#141771=CARTESIAN_POINT('Ctrl Pts',(-20.0719688100384,12.5084013028489,
130.85885015324)) ;
#141772=CARTESIAN_POINT('Ctrl Pts',(-19.9881652481842,12.6562046151244,
130.647206486187)) ;
#141773=CARTESIAN_POINT('Ctrl Pts',(-19.9199396779561,12.8582528702238,
130.48094000311)) ;
#141774=CARTESIAN_POINT('Ctrl Pts',(-19.8708223545684,13.10224809555,130.370716051289)) ;
#141775=CARTESIAN_POINT('Ctrl Pts',(-19.8442937835913,13.3685511856617,
130.326365144569)) ;
#141776=CARTESIAN_POINT('Ctrl Pts',(-19.8411260523443,13.6374690862059,
130.350100513771)) ;
#141777=CARTESIAN_POINT('Ctrl Pts',(-19.86090775583,13.8926337693761,130.441079325237)) ;
#141778=CARTESIAN_POINT('Ctrl Pts',(-19.9014600976165,14.1134974060216,
130.592644036844)) ;
#141779=CARTESIAN_POINT('Ctrl Pts',(-19.9593667313595,14.2854804589728,
130.795017810507)) ;
#141780=CARTESIAN_POINT('Ctrl Pts',(-20.0293912566406,14.394916969494,131.03267442462)) ;
#141781=CARTESIAN_POINT('Ctrl Pts',(-20.1056792081533,14.435095047054,131.288519546508)) ;
#141782=CARTESIAN_POINT('Ctrl Pts',(-20.1829120670562,14.4027523560096,
131.547383866018)) ;
#141783=CARTESIAN_POINT('Ctrl Pts',(-20.2538480508494,14.3004224301193,
131.787669615841)) ;
#141784=CARTESIAN_POINT('Ctrl Pts',(-20.3133527497641,14.1345848207203,
131.994721949967)) ;
#141785=CARTESIAN_POINT('Ctrl Pts',(-20.355864409434,13.9188292654447,132.15193646137)) ;
#141786=CARTESIAN_POINT('Ctrl Pts',(-20.378071179084,13.6668968226668,132.249955352682)) ;
#141787=CARTESIAN_POINT('Ctrl Pts',(-20.3775079318251,13.3982258049414,
132.281358615002)) ;
#141788=CARTESIAN_POINT('Ctrl Pts',(-20.3533777867425,13.1299459818543,
132.24409760961)) ;
#141789=CARTESIAN_POINT('Ctrl Pts',(-20.3068511976437,12.8837060048702,
132.141274285562)) ;
#141790=CARTESIAN_POINT('Ctrl Pts',(-20.240261347845,12.6755091037675,131.979947404298)) ;
#141791=CARTESIAN_POINT('Ctrl Pts',(-20.1581680238177,12.5215778341602,
131.773182076307)) ;
#141792=CARTESIAN_POINT('Ctrl Pts',(-20.0649675040375,12.4317802078497,
131.534139059742)) ;
#141793=CARTESIAN_POINT('Ctrl Pts',(-19.9677911498579,12.4131805145463,
131.283214057728)) ;
#141794=CARTESIAN_POINT('Ctrl Pts',(-19.8713977553643,12.4668842843224,
131.034839990203)) ;
#141795=CARTESIAN_POINT('Ctrl Pts',(-19.7832398695149,12.5884450791791,
130.810305644908)) ;
#141796=CARTESIAN_POINT('Ctrl Pts',(-19.7076706234563,12.7713421564293,
130.62286138056)) ;
#141797=CARTESIAN_POINT('Ctrl Pts',(-19.650734391685,12.9988618767288,130.489494578148)) ;
#141798=CARTESIAN_POINT('Ctrl Pts',(-19.6146315035451,13.259491403766,130.417371328723)) ;
#141799=CARTESIAN_POINT('Ctrl Pts',(-19.602066610751,13.5289134128762,130.413620138675)) ;
#141800=CARTESIAN_POINT('Ctrl Pts',(-19.6126420557654,13.792044854945,130.477635491383)) ;
#141801=CARTESIAN_POINT('Ctrl Pts',(-19.6450752325787,14.0286824176204,
130.605479576481)) ;
#141802=CARTESIAN_POINT('Ctrl Pts',(-19.6965636088298,14.2226477736602,
130.789131633615)) ;
#141803=CARTESIAN_POINT('Ctrl Pts',(-19.7620620684361,14.3581280459106,
131.013479763775)) ;
#141804=CARTESIAN_POINT('Ctrl Pts',(-19.8366555625925,14.4275172368953,
131.264485219799)) ;
#141805=CARTESIAN_POINT('Ctrl Pts',(-19.914713017642,14.4244373227483,131.525845240593)) ;
#141806=CARTESIAN_POINT('Ctrl Pts',(-19.9884493193164,14.3501367823951,
131.77417324445)) ;
#141807=CARTESIAN_POINT('Ctrl Pts',(-20.0533520936969,14.2089997399679,
131.99696494782)) ;
#141808=CARTESIAN_POINT('Ctrl Pts',(-20.1032372720437,14.0121250451069,
132.17574893776)) ;
#141809=CARTESIAN_POINT('Ctrl Pts',(-20.1342125776709,13.7718246711113,
132.299481752515)) ;
#141810=CARTESIAN_POINT('Ctrl Pts',(-20.1429809167067,13.5078186231509,
132.358155687099)) ;
#141811=CARTESIAN_POINT('Ctrl Pts',(-20.1284039868733,13.2372789127591,
132.348703112449)) ;
#141812=CARTESIAN_POINT('Ctrl Pts',(-20.0908625978491,12.980432676453,132.272099446344)) ;
#141813=CARTESIAN_POINT('Ctrl Pts',(-20.0318009855664,12.7540238473754,
132.132840514117)) ;
#141814=CARTESIAN_POINT('Ctrl Pts',(-19.9558387140201,12.5774627214212,
131.943866603019)) ;
#141815=CARTESIAN_POINT('Ctrl Pts',(-19.8662835104376,12.4598742845048,
131.715495634813)) ;
#141816=CARTESIAN_POINT('Ctrl Pts',(-19.7697256841548,12.4120040771025,
131.466564374263)) ;
#141817=CARTESIAN_POINT('Ctrl Pts',(-19.6722699667815,12.4365719363613,
131.21497904264)) ;
#141818=CARTESIAN_POINT('Ctrl Pts',(-19.5802613105046,12.5311793730478,
130.979208437368)) ;
#141819=CARTESIAN_POINT('Ctrl Pts',(-19.4986531494467,12.6910252991536,
130.774112825828)) ;
#141820=CARTESIAN_POINT('Ctrl Pts',(-19.4340286592284,12.9015546057863,
130.618290378308)) ;
#141821=CARTESIAN_POINT('Ctrl Pts',(-19.3890411033215,13.1503193802668,
130.520011015745)) ;
#141822=CARTESIAN_POINT('Ctrl Pts',(-19.3667781285979,13.4198238149612,
130.488246338711)) ;
#141823=CARTESIAN_POINT('Ctrl Pts',(-19.3679978219409,13.6867201832379,
130.524721757099)) ;
#141824=CARTESIAN_POINT('Ctrl Pts',(-19.3919557160883,13.9376559863072,
130.62799833703)) ;
#141825=CARTESIAN_POINT('Ctrl Pts',(-19.4361283002266,14.1502428615257,
130.790145849377)) ;
#141826=CARTESIAN_POINT('Ctrl Pts',(-19.4965493043583,14.3108380697217,
130.999753103418)) ;
#141827=CARTESIAN_POINT('Ctrl Pts',(-19.568262071274,14.4079445348436,131.242354028825)) ;
#141828=CARTESIAN_POINT('Ctrl Pts',(-19.6454042775569,14.4345276706247,
131.500826737002)) ;
#141829=CARTESIAN_POINT('Ctrl Pts',(-19.7216080873504,14.3888298731307,
131.756512645757)) ;
#141830=CARTESIAN_POINT('Ctrl Pts',(-19.7909620886184,14.273828468375,131.992266951157)) ;
#141831=CARTESIAN_POINT('Ctrl Pts',(-19.8475410580093,14.0978368302853,
132.190684651942)) ;
#141832=CARTESIAN_POINT('Ctrl Pts',(-19.8866080882812,13.8735407233332,
132.337940805145)) ;
#141833=CARTESIAN_POINT('Ctrl Pts',(-19.9046387879488,13.6168750178338,
132.423754270832)) ;
#141834=CARTESIAN_POINT('Ctrl Pts',(-19.8996055461185,13.346506361492,132.4421704395)) ;
#141835=CARTESIAN_POINT('Ctrl Pts',(-19.8711825635662,13.0815407666398,
132.392264377035)) ;
#141836=CARTESIAN_POINT('Ctrl Pts',(-19.8205474898722,12.8409646602013,
132.277503248563)) ;
#141837=CARTESIAN_POINT('Ctrl Pts',(-19.7511694006213,12.6428639918128,
132.107805469433)) ;
#141838=CARTESIAN_POINT('Ctrl Pts',(-19.6657363050394,12.4989646430065,
131.891643331655)) ;
#141839=CARTESIAN_POINT('Ctrl Pts',(-19.5722878839265,12.4231076853541,
131.651474151143)) ;
#141840=CARTESIAN_POINT('Ctrl Pts',(-19.4740246524998,12.4177381591252,
131.397689125236)) ;
#141841=CARTESIAN_POINT('Ctrl Pts',(-19.3789969152326,12.4847095466627,
131.153165024408)) ;
#141842=CARTESIAN_POINT('Ctrl Pts',(-19.2924935792413,12.6190668251906,
130.933646272935)) ;
#141843=CARTESIAN_POINT('Ctrl Pts',(-19.2204813399372,12.8107471895688,
130.756372046187)) ;
#141844=CARTESIAN_POINT('Ctrl Pts',(-19.1671050807076,13.0461049078406,
130.633535559335)) ;
#141845=CARTESIAN_POINT('Ctrl Pts',(-19.1354518923136,13.3089104890012,
130.574215108908)) ;
#141846=CARTESIAN_POINT('Ctrl Pts',(-19.1271492497169,13.5795918474296,
130.583068460063)) ;
#141847=CARTESIAN_POINT('Ctrl Pts',(-19.1420823786064,13.8398549511919,
130.659898097872)) ;
#141848=CARTESIAN_POINT('Ctrl Pts',(-19.1785538930754,14.0698649783882,
130.79962783888)) ;
#141849=CARTESIAN_POINT('Ctrl Pts',(-19.2326864141405,14.2524396498396,
130.990725985703)) ;
#141850=CARTESIAN_POINT('Ctrl Pts',(-19.3006476101395,14.3767943288433,
131.222452811304)) ;
#141851=CARTESIAN_POINT('Ctrl Pts',(-19.37610451377,14.4324209617662,131.475897601322)) ;
#141852=CARTESIAN_POINT('Ctrl Pts',(-19.4536998093068,14.4159981078524,
131.735777838716)) ;
#141853=CARTESIAN_POINT('Ctrl Pts',(-19.5265608664841,14.3283155075796,
131.981745823597)) ;
#141854=CARTESIAN_POINT('Ctrl Pts',(-19.5889643403077,14.1755658927935,
132.197206943075)) ;
#141855=CARTESIAN_POINT('Ctrl Pts',(-19.6354790586532,13.9699067943466,
132.366095536546)) ;
#141856=CARTESIAN_POINT('Ctrl Pts',(-19.6624519781793,13.7239839863066,
132.478077716201)) ;
#141857=CARTESIAN_POINT('Ctrl Pts',(-19.666980954464,13.4571372735282,132.524398080383)) ;
#141858=CARTESIAN_POINT('Ctrl Pts',(-19.6477861345708,13.1860385080971,
132.501656426746)) ;
#141859=CARTESIAN_POINT('Ctrl Pts',(-19.6062304044814,12.9351633372793,
132.413151943778)) ;
#141860=CARTESIAN_POINT('Ctrl Pts',(-19.5434289051781,12.7162804283108,
132.263030237578)) ;
#141861=CARTESIAN_POINT('Ctrl Pts',(-19.4647999874014,12.5504602978257,
132.066204808384)) ;
#141862=CARTESIAN_POINT('Ctrl Pts',(-19.3729739339425,12.4451571789981,
131.831357919352)) ;
#141863=CARTESIAN_POINT('Ctrl Pts',(-19.2764129384417,12.4110818133835,
131.582183020865)) ;
#141864=CARTESIAN_POINT('Ctrl Pts',(-19.1789058275452,12.4493848627309,
131.330644654867)) ;
#141865=CARTESIAN_POINT('Ctrl Pts',(-19.0889426594496,12.5564279149636,
131.100712663772)) ;
#141866=CARTESIAN_POINT('Ctrl Pts',(-19.0099622196206,12.7270948796437,
130.903310128084)) ;
#141867=CARTESIAN_POINT('Ctrl Pts',(-18.9486581578239,12.9467013560163,
130.757301018768)) ;
#141868=CARTESIAN_POINT('Ctrl Pts',(-18.9079322965114,13.2005745815833,
130.671455691176)) ;
#141869=CARTESIAN_POINT('Ctrl Pts',(-18.8901493403744,13.4697556430519,
130.652551582451)) ;
#141870=CARTESIAN_POINT('Ctrl Pts',(-18.8956759511923,13.736255276326,130.70181545982)) ;
#141871=CARTESIAN_POINT('Ctrl Pts',(-18.9238215240828,13.9814042376555,
130.817329927107)) ;
#141872=CARTESIAN_POINT('Ctrl Pts',(-18.9710857402053,14.1841667225104,
130.988318199626)) ;
#141873=CARTESIAN_POINT('Ctrl Pts',(-19.0342235553262,14.3343212234818,
131.205982310787)) ;
#141874=CARTESIAN_POINT('Ctrl Pts',(-19.1075024006883,14.4184551255459,
131.453186900697)) ;
#141875=CARTESIAN_POINT('Ctrl Pts',(-19.1848350711925,14.4314519910157,
131.712158292538)) ;
#141876=CARTESIAN_POINT('Ctrl Pts',(-19.260343209931,14.3721434966701,131.965889987133)) ;
#141877=CARTESIAN_POINT('Ctrl Pts',(-19.3275198723999,14.245373795937,132.195174956684)) ;
#141878=CARTESIAN_POINT('Ctrl Pts',(-19.381396493653,14.0581566175582,132.38587704578)) ;
#141879=CARTESIAN_POINT('Ctrl Pts',(-19.4164824936223,13.8276967157625,
132.521313395047)) ;
#141880=CARTESIAN_POINT('Ctrl Pts',(-19.4303957231885,13.5670202701056,
132.595106405332)) ;
#141881=CARTESIAN_POINT('Ctrl Pts',(-19.4208832730529,13.2953785672156,
132.600537532849)) ;
#141882=CARTESIAN_POINT('Ctrl Pts',(-19.3882471470235,13.0342213948757,
132.538241764966)) ;
#141883=CARTESIAN_POINT('Ctrl Pts',(-19.3334906631503,12.799235193231,132.411585913234)) ;
#141884=CARTESIAN_POINT('Ctrl Pts',(-19.261043051524,12.6113832489784,132.232841060181)) ;
#141885=CARTESIAN_POINT('Ctrl Pts',(-19.1739879603888,12.4798503572911,
132.011723757091)) ;
#141886=CARTESIAN_POINT('Ctrl Pts',(-19.0786309591327,12.4163978542697,
131.766255688974)) ;
#141887=CARTESIAN_POINT('Ctrl Pts',(-18.98062423312,12.4249215089451,131.513135114901)) ;
#141888=CARTESIAN_POINT('Ctrl Pts',(-18.8865300769159,12.505375632336,131.271441981484)) ;
#141889=CARTESIAN_POINT('Ctrl Pts',(-18.8027816816541,12.6507859579669,
131.059795433215)) ;
#141890=CARTESIAN_POINT('Ctrl Pts',(-18.7338552847486,12.8517471604921,
130.891556618689)) ;
#141891=CARTESIAN_POINT('Ctrl Pts',(-18.6842105366579,13.0945615121704,
130.779753269807)) ;
#141892=CARTESIAN_POINT('Ctrl Pts',(-18.6569376131211,13.3602126938648,
130.733201043966)) ;
#141893=CARTESIAN_POINT('Ctrl Pts',(-18.6531415615538,13.6310672418703,
130.755323120175)) ;
#141894=CARTESIAN_POINT('Ctrl Pts',(-18.6722331473898,13.8852754196112,
130.844076845159)) ;
#141895=CARTESIAN_POINT('Ctrl Pts',(-18.7122022947617,14.1076160961634,
130.993965145821)) ;
#141896=CARTESIAN_POINT('Ctrl Pts',(-18.7695522886427,14.2808806775566,
131.194645480041)) ;
#141897=CARTESIAN_POINT('Ctrl Pts',(-18.83924559398,14.3926567140697,131.431331456996)) ;
#141898=CARTESIAN_POINT('Ctrl Pts',(-18.9160286047029,14.4348969487797,
131.688881910265)) ;
#141899=CARTESIAN_POINT('Ctrl Pts',(-18.9926033453051,14.4049966938089,
131.945496008568)) ;
#141900=CARTESIAN_POINT('Ctrl Pts',(-19.0644452296558,14.3037928879971,
132.188736587752)) ;
#141901=CARTESIAN_POINT('Ctrl Pts',(-19.1239168662076,14.1405203886364,
132.395461417312)) ;
#141902=CARTESIAN_POINT('Ctrl Pts',(-19.167107493149,13.9258191090176,132.554726043637)) ;
#141903=CARTESIAN_POINT('Ctrl Pts',(-19.1899722517165,13.6747404934951,
132.654652849122)) ;
#141904=CARTESIAN_POINT('Ctrl Pts',(-19.1900075690217,13.4052256661744,
132.687941950443)) ;
#141905=CARTESIAN_POINT('Ctrl Pts',(-19.166746991383,13.138469239792,132.652983769787)) ;
#141906=CARTESIAN_POINT('Ctrl Pts',(-19.1205720258971,12.8897551396211,
132.551405771592)) ;
#141907=CARTESIAN_POINT('Ctrl Pts',(-19.0548239476007,12.6813707794316,
132.392358845986)) ;
#141908=CARTESIAN_POINT('Ctrl Pts',(-18.9730261476444,12.5252896254052,
132.18651714806)) ;
#141909=CARTESIAN_POINT('Ctrl Pts',(-18.8802716176398,12.4335761990142,
131.948700699389)) ;
#141910=CARTESIAN_POINT('Ctrl Pts',(-18.7828229550223,12.4126069682806,
131.697092660579)) ;
#141911=CARTESIAN_POINT('Ctrl Pts',(-18.6860467767773,12.4645413943428,
131.447685791234)) ;
#141912=CARTESIAN_POINT('Ctrl Pts',(-18.5976234412375,12.5845283028617,
131.222382340814)) ;
#141913=CARTESIAN_POINT('Ctrl Pts',(-18.5218504701098,12.7652451622035,
131.034228327474)) ;
#141914=CARTESIAN_POINT('Ctrl Pts',(-18.4642539071398,12.9922348070079,
130.899013365635)) ;
#141915=CARTESIAN_POINT('Ctrl Pts',(-18.4277290043019,13.2501819432392,
130.825397364952)) ;
#141916=CARTESIAN_POINT('Ctrl Pts',(-18.414270152757,13.5208713939763,130.819203355187)) ;
#141917=CARTESIAN_POINT('Ctrl Pts',(-18.4242664380075,13.7852949674506,
130.881626201884)) ;
#141918=CARTESIAN_POINT('Ctrl Pts',(-18.4562051880654,14.0230294711121,
131.008056241537)) ;
#141919=CARTESIAN_POINT('Ctrl Pts',(-18.5071026488867,14.217815504055,131.189893611675)) ;
#141920=CARTESIAN_POINT('Ctrl Pts',(-18.5722572460804,14.355293096106,131.413244424432)) ;
#141921=CARTESIAN_POINT('Ctrl Pts',(-18.6470132645676,14.4265292690715,
131.664865103024)) ;
#141922=CARTESIAN_POINT('Ctrl Pts',(-18.7241791544619,14.4257522115435,
131.923231401887)) ;
#141923=CARTESIAN_POINT('Ctrl Pts',(-18.798764612649,14.353191154613,132.174331118384)) ;
#141924=CARTESIAN_POINT('Ctrl Pts',(-18.863847038587,14.2139748477186,132.397566284138)) ;
#141925=CARTESIAN_POINT('Ctrl Pts',(-18.9143185597732,14.0181342342469,
132.57813709689)) ;
#141926=CARTESIAN_POINT('Ctrl Pts',(-18.945785649306,13.7796844257176,132.703183210523)) ;
#141927=CARTESIAN_POINT('Ctrl Pts',(-18.9552755509885,13.515523516605,132.764049213495)) ;
#141928=CARTESIAN_POINT('Ctrl Pts',(-18.9413798979237,13.2452125858444,
132.756543939979)) ;
#141929=CARTESIAN_POINT('Ctrl Pts',(-18.9045068472628,12.9877057714763,
132.681894685849)) ;
#141930=CARTESIAN_POINT('Ctrl Pts',(-18.8460866892425,12.760206013501,132.544485955534)) ;
#141931=CARTESIAN_POINT('Ctrl Pts',(-18.7704201812073,12.5817512352831,
132.356441887698)) ;
#141932=CARTESIAN_POINT('Ctrl Pts',(-18.6814549221541,12.4625557335165,
132.129687023167)) ;
#141933=CARTESIAN_POINT('Ctrl Pts',(-18.5848852819742,12.4124303702056,
131.880776268223)) ;
#141934=CARTESIAN_POINT('Ctrl Pts',(-18.4875205077328,12.4345388206878,
131.62939372436)) ;
#141935=CARTESIAN_POINT('Ctrl Pts',(-18.3944792146438,12.5283216628162,
131.390912274721)) ;
#141936=CARTESIAN_POINT('Ctrl Pts',(-18.313375423817,12.6848122547612,131.186922689569)) ;
#141937=CARTESIAN_POINT('Ctrl Pts',(-18.2476370162531,12.8954783028643,
131.02811076423)) ;
#141938=CARTESIAN_POINT('Ctrl Pts',(-18.2022662694842,13.143031226721,130.92863304818)) ;
#141939=CARTESIAN_POINT('Ctrl Pts',(-18.1793404232656,13.4109716015929,
130.894784380807)) ;
#141940=CARTESIAN_POINT('Ctrl Pts',(-18.1798282338456,13.6794256952143,
130.929276425369)) ;
#141941=CARTESIAN_POINT('Ctrl Pts',(-18.2032729243198,13.9314101071075,
131.031097970165)) ;
#141942=CARTESIAN_POINT('Ctrl Pts',(-18.2467759985431,14.1445006476294,
131.19117652553)) ;
#141943=CARTESIAN_POINT('Ctrl Pts',(-18.3066776441594,14.3067536446236,
131.399226993527)) ;
#141944=CARTESIAN_POINT('Ctrl Pts',(-18.3782137507977,14.4060487060152,
131.641351715669)) ;
#141945=CARTESIAN_POINT('Ctrl Pts',(-18.4553476578096,14.4348548850669,
131.899823806856)) ;
#141946=CARTESIAN_POINT('Ctrl Pts',(-18.5318716415341,14.3909041577753,
132.156543176564)) ;
#141947=CARTESIAN_POINT('Ctrl Pts',(-18.6011996766594,14.2783347271922,
132.392068800067)) ;
#141948=CARTESIAN_POINT('Ctrl Pts',(-18.6585012371958,14.1031935059032,
132.592753758215)) ;
#141949=CARTESIAN_POINT('Ctrl Pts',(-18.6980121020502,13.880010412854,132.741285296251)) ;
#141950=CARTESIAN_POINT('Ctrl Pts',(-18.7166279415518,13.6249526911944,
132.828691039322)) ;
#141951=CARTESIAN_POINT('Ctrl Pts',(-18.7123103754502,13.354798949211,132.849191352967)) ;
#141952=CARTESIAN_POINT('Ctrl Pts',(-18.6846880430549,13.0897726213642,
132.801568647031)) ;
#141953=CARTESIAN_POINT('Ctrl Pts',(-18.6343821577113,12.8467548703801,
132.687965653879)) ;
#141954=CARTESIAN_POINT('Ctrl Pts',(-18.5654973268203,12.6478123647641,
132.519664319044)) ;
#141955=CARTESIAN_POINT('Ctrl Pts',(-18.48107055355,12.5027971632239,132.306214422385)) ;
#141956=CARTESIAN_POINT('Ctrl Pts',(-18.3870428160206,12.4240443471672,
132.064632825828)) ;
#141957=CARTESIAN_POINT('Ctrl Pts',(-18.2887354925409,12.4170503727496,
131.81073482203)) ;
#141958=CARTESIAN_POINT('Ctrl Pts',(-18.1939119303328,12.4817914292567,
131.566682633117)) ;
#141959=CARTESIAN_POINT('Ctrl Pts',(-18.1070449414969,12.6142901362916,
131.346109388021)) ;
#141960=CARTESIAN_POINT('Ctrl Pts',(-18.0346358797705,12.8042104652996,
131.167634409426)) ;
#141961=CARTESIAN_POINT('Ctrl Pts',(-17.9805255623072,13.0388187683455,
131.042705325369)) ;
#141962=CARTESIAN_POINT('Ctrl Pts',(-17.9481797311077,13.3023286417973,
130.981508149385)) ;
#141963=CARTESIAN_POINT('Ctrl Pts',(-17.9392863704219,13.571341528554,130.988424251185)) ;
#141964=CARTESIAN_POINT('Ctrl Pts',(-17.953573606269,13.8329963549421,131.063471024854)) ;
#141965=CARTESIAN_POINT('Ctrl Pts',(-17.9893989895141,14.0635777479953,
131.201232852988)) ;
#141966=CARTESIAN_POINT('Ctrl Pts',(-18.0431541123013,14.2479537659708,
131.391285506657)) ;
#141967=CARTESIAN_POINT('Ctrl Pts',(-18.1105562726005,14.3739504814687,
131.621267259674)) ;
#141968=CARTESIAN_POINT('Ctrl Pts',(-18.1864968499214,14.4320428256961,
131.876400337601)) ;
#141969=CARTESIAN_POINT('Ctrl Pts',(-18.2639229888398,14.417227489115,132.135696662505)) ;
#141970=CARTESIAN_POINT('Ctrl Pts',(-18.3367309580096,14.3318166696858,
132.38139603203)) ;
#141971=CARTESIAN_POINT('Ctrl Pts',(-18.3994855464605,14.1811817924182,
132.597839900643)) ;
#141972=CARTESIAN_POINT('Ctrl Pts',(-18.4466875926336,13.9759967234678,
132.76887624803)) ;
#141973=CARTESIAN_POINT('Ctrl Pts',(-18.4742378060519,13.7313492030733,
132.882483371035)) ;
#141974=CARTESIAN_POINT('Ctrl Pts',(-18.4792949779045,13.4634560829624,
132.930523403806)) ;
#141975=CARTESIAN_POINT('Ctrl Pts',(-18.461128478173,13.1958849143636,132.910312028036)) ;
#141976=CARTESIAN_POINT('Ctrl Pts',(-18.4197940229711,12.9412336892527,
132.822854780355)) ;
#141977=CARTESIAN_POINT('Ctrl Pts',(-18.3581041603467,12.7230235102752,
132.675668704181)) ;
#141978=CARTESIAN_POINT('Ctrl Pts',(-18.2791809280835,12.5539648148601,
132.478304085645)) ;
#141979=CARTESIAN_POINT('Ctrl Pts',(-18.1885902754786,12.4477725883293,
132.246702802813)) ;
#141980=CARTESIAN_POINT('Ctrl Pts',(-18.0914153871671,12.4110238127138,
131.995992901408)) ;
#141981=CARTESIAN_POINT('Ctrl Pts',(-17.994297829235,12.4468710240649,131.74541114138)) ;
#141982=CARTESIAN_POINT('Ctrl Pts',(-17.9031245377903,12.5531554013667,
131.512299991437)) ;
#141983=CARTESIAN_POINT('Ctrl Pts',(-17.8243881263639,12.7211113727201,
131.31534546579)) ;
#141984=CARTESIAN_POINT('Ctrl Pts',(-17.7623176137726,12.9400020484962,
131.167199368981)) ;
#141985=CARTESIAN_POINT('Ctrl Pts',(-17.721116969805,13.1921120918715,131.07982905239)) ;
#141986=CARTESIAN_POINT('Ctrl Pts',(-17.7025045759027,13.4620045892925,
131.058616683595)) ;
#141987=CARTESIAN_POINT('Ctrl Pts',(-17.7074749062916,13.7292706883455,
131.106312813536)) ;
#141988=CARTESIAN_POINT('Ctrl Pts',(-17.7347681793512,13.9738126531135,
131.219120659009)) ;
#141989=CARTESIAN_POINT('Ctrl Pts',(-17.7817727411794,14.179494761427,131.389572070766)) ;
#141990=CARTESIAN_POINT('Ctrl Pts',(-17.844677886555,14.3311259562621,131.606587075838)) ;
#141991=CARTESIAN_POINT('Ctrl Pts',(-17.9173204242354,14.4169205750236,
131.851744794664)) ;
#141992=CARTESIAN_POINT('Ctrl Pts',(-17.995061475666,14.4320030262707,132.112107124994)) ;
#141993=CARTESIAN_POINT('Ctrl Pts',(-18.0703004283371,14.3751243416082,
132.364855998224)) ;
#141994=CARTESIAN_POINT('Ctrl Pts',(-18.1383688657966,14.2488767663409,
132.597055820527)) ;
#141995=CARTESIAN_POINT('Ctrl Pts',(-18.1921359192542,14.0648018016439,
132.78710913641)) ;
#141996=CARTESIAN_POINT('Ctrl Pts',(-18.2280722562178,13.8343787612975,
132.925210436483)) ;
#141997=CARTESIAN_POINT('Ctrl Pts',(-18.242538116868,13.57360703546,133.000682596127)) ;
#141998=CARTESIAN_POINT('Ctrl Pts',(-18.2336329639187,13.3025524242793,
133.007820999502)) ;
#141999=CARTESIAN_POINT('Ctrl Pts',(-18.2017369474132,13.0417944958654,
132.947575616599)) ;
#142000=CARTESIAN_POINT('Ctrl Pts',(-18.1478312171758,12.8063139825281,
132.823302147589)) ;
#142001=CARTESIAN_POINT('Ctrl Pts',(-18.0755496900259,12.6158856325691,
132.645204191962)) ;
#142002=CARTESIAN_POINT('Ctrl Pts',(-17.9886538009937,12.4825396581066,
132.424600946456)) ;
#142003=CARTESIAN_POINT('Ctrl Pts',(-17.8937284373199,12.4173081126312,
132.180299122837)) ;
#142004=CARTESIAN_POINT('Ctrl Pts',(-17.7958096584206,12.4236050164849,
131.92740109039)) ;
#142005=CARTESIAN_POINT('Ctrl Pts',(-17.7015466531236,12.5018026361359,
131.685195645254)) ;
#142006=CARTESIAN_POINT('Ctrl Pts',(-17.6171539893032,12.6458566369947,
131.471772621455)) ;
#142007=CARTESIAN_POINT('Ctrl Pts',(-17.5478109773661,12.8453791511498,
131.302294768861)) ;
#142008=CARTESIAN_POINT('Ctrl Pts',(-17.4976407306197,13.0865653368531,
131.18887233862)) ;
#142009=CARTESIAN_POINT('Ctrl Pts',(-17.4696392111755,13.3521428238873,
131.140239531717)) ;
#142010=CARTESIAN_POINT('Ctrl Pts',(-17.4651068443978,13.6222557770976,
131.160098232974)) ;
#142011=CARTESIAN_POINT('Ctrl Pts',(-17.4835603986076,13.878388340665,131.247136678345)) ;
#142012=CARTESIAN_POINT('Ctrl Pts',(-17.5231079409385,14.1022120909712,
131.395853700729)) ;
#142013=CARTESIAN_POINT('Ctrl Pts',(-17.5798728990191,14.2765229673721,
131.594730965601)) ;
#142014=CARTESIAN_POINT('Ctrl Pts',(-17.6491847088976,14.3902287028563,
131.830268466419)) ;
#142015=CARTESIAN_POINT('Ctrl Pts',(-17.7259698460983,14.4347769425123,
132.087872526908)) ;
#142016=CARTESIAN_POINT('Ctrl Pts',(-17.8027636785654,14.406672259026,132.345197200108)) ;
#142017=CARTESIAN_POINT('Ctrl Pts',(-17.8744322223128,14.3082119103095,
132.587721606493)) ;
#142018=CARTESIAN_POINT('Ctrl Pts',(-17.9346414922608,14.146035786889,132.796763374113)) ;
#142019=CARTESIAN_POINT('Ctrl Pts',(-17.978328838425,13.9328084599434,132.957440175315)) ;
#142020=CARTESIAN_POINT('Ctrl Pts',(-18.0018422375615,13.6817741285683,
133.059362342777)) ;
#142021=CARTESIAN_POINT('Ctrl Pts',(-18.0026012553216,13.4140262407359,
133.094572904511)) ;
#142022=CARTESIAN_POINT('Ctrl Pts',(-17.9798594877152,13.1453688481844,
133.061337889453)) ;
#142023=CARTESIAN_POINT('Ctrl Pts',(-17.9347276850374,12.8977836730895,
132.962526042225)) ;
#142024=CARTESIAN_POINT('Ctrl Pts',(-17.8690240884409,12.6861562581584,
132.803892072345)) ;
#142025=CARTESIAN_POINT('Ctrl Pts',(-17.7877339722851,12.5289208542769,
132.599457950631)) ;
#142026=CARTESIAN_POINT('Ctrl Pts',(-17.6951142737879,12.43515491016,132.362074354773)) ;
#142027=CARTESIAN_POINT('Ctrl Pts',(-17.5979412066733,12.4122393521451,
132.111194582501)) ;
#142028=CARTESIAN_POINT('Ctrl Pts',(-17.5010420457257,12.461921394401,131.861423387377)) ;
#142029=CARTESIAN_POINT('Ctrl Pts',(-17.4121127241867,12.5803996881322,
131.634723585912)) ;
#142030=CARTESIAN_POINT('Ctrl Pts',(-17.3360909230878,12.7591299511845,
131.445758242556)) ;
#142031=CARTESIAN_POINT('Ctrl Pts',(-17.2778596775834,12.9850687744513,
131.30871290489)) ;
#142032=CARTESIAN_POINT('Ctrl Pts',(-17.2406869894393,13.2423777832249,
131.233202541002)) ;
#142033=CARTESIAN_POINT('Ctrl Pts',(-17.2265555305213,13.5129449874981,
131.225042209929)) ;
#142034=CARTESIAN_POINT('Ctrl Pts',(-17.2358208600922,13.7774321466873,
131.285270109407)) ;
#142035=CARTESIAN_POINT('Ctrl Pts',(-17.2672256879663,14.0166134840393,
131.410209396935)) ;
#142036=CARTESIAN_POINT('Ctrl Pts',(-17.3173096357002,14.2120831170415,
131.589498480406)) ;
#142037=CARTESIAN_POINT('Ctrl Pts',(-17.3825645879294,14.3524989582878,
131.813388688858)) ;
#142038=CARTESIAN_POINT('Ctrl Pts',(-17.4569074319178,14.4253825851082,
132.063685579465)) ;
#142039=CARTESIAN_POINT('Ctrl Pts',(-17.5341963564748,14.4267682802424,
132.322471620608)) ;
#142040=CARTESIAN_POINT('Ctrl Pts',(-17.6087797719604,14.3564919766321,
132.573476433911)) ;
#142041=CARTESIAN_POINT('Ctrl Pts',(-17.6744472100706,14.2186718710266,
132.798538178836)) ;
#142042=CARTESIAN_POINT('Ctrl Pts',(-17.72535311061,14.024316702861,132.980354800871)) ;
#142043=CARTESIAN_POINT('Ctrl Pts',(-17.7574107045078,13.7866135128635,
133.107157176176)) ;
#142044=CARTESIAN_POINT('Ctrl Pts',(-17.7675312687633,13.5238036073327,
133.169755706042)) ;
#142045=CARTESIAN_POINT('Ctrl Pts',(-17.7543475166113,13.2527085149488,
133.164413552802)) ;
#142046=CARTESIAN_POINT('Ctrl Pts',(-17.7178633050782,12.9936529878453,
133.09103192121)) ;
#142047=CARTESIAN_POINT('Ctrl Pts',(-17.6602511851627,12.7662441294868,
132.95581758286)) ;
#142048=CARTESIAN_POINT('Ctrl Pts',(-17.5849255965554,12.5858801023732,
132.768826558598)) ;
#142049=CARTESIAN_POINT('Ctrl Pts',(-17.4961834389353,12.4648530530782,
132.542741778166)) ;
#142050=CARTESIAN_POINT('Ctrl Pts',(-17.3995854558629,12.4128201852834,
132.293797467727)) ;
#142051=CARTESIAN_POINT('Ctrl Pts',(-17.3025511829403,12.4330274205639,
132.04325545605)) ;
#142052=CARTESIAN_POINT('Ctrl Pts',(-17.2096884596466,12.5240123419654,
131.805133684606)) ;
#142053=CARTESIAN_POINT('Ctrl Pts',(-17.1276669580838,12.6795221471728,
131.598658383154)) ;
#142054=CARTESIAN_POINT('Ctrl Pts',(-17.0614706985305,12.8889214300487,
131.438497796341)) ;
#142055=CARTESIAN_POINT('Ctrl Pts',(-17.0154598015636,13.1354947204779,
131.337138856507)) ;
#142056=CARTESIAN_POINT('Ctrl Pts',(-16.9918318882357,13.4042911484909,
131.301379652949)) ;
#142057=CARTESIAN_POINT('Ctrl Pts',(-16.9917442489886,13.6719452324486,
131.334066321195)) ;
#142058=CARTESIAN_POINT('Ctrl Pts',(-17.0144533549174,13.9242175313922,
131.433665873443)) ;
#142059=CARTESIAN_POINT('Ctrl Pts',(-17.0574770945585,14.1390288718251,
131.592404046704)) ;
#142060=CARTESIAN_POINT('Ctrl Pts',(-17.1170228825635,14.3030286134432,
131.799436930536)) ;
#142061=CARTESIAN_POINT('Ctrl Pts',(-17.1883492711194,14.404195333154,132.040962388259)) ;
#142062=CARTESIAN_POINT('Ctrl Pts',(-17.2651695925288,14.4349854783543,
132.298417684023)) ;
#142063=CARTESIAN_POINT('Ctrl Pts',(-17.3418160412074,14.3934046860553,
132.555492533382)) ;
#142064=CARTESIAN_POINT('Ctrl Pts',(-17.4116634894223,14.2822103029933,
132.792658991486)) ;
#142065=CARTESIAN_POINT('Ctrl Pts',(-17.4690521516874,14.1097942178576,
132.993391663448)) ;
#142066=CARTESIAN_POINT('Ctrl Pts',(-17.5093062354731,13.8877666791924,
133.144142840939)) ;
#142067=CARTESIAN_POINT('Ctrl Pts',(-17.5286362429465,13.6324083997063,
133.233762073457)) ;
#142068=CARTESIAN_POINT('Ctrl Pts',(-17.5249803176019,13.3624184985193,
133.25618971708)) ;
#142069=CARTESIAN_POINT('Ctrl Pts',(-17.4979086389593,13.0965814202268,
133.210233885048)) ;
#142070=CARTESIAN_POINT('Ctrl Pts',(-17.448517501126,12.8540735599423,133.099102550144)) ;
#142071=CARTESIAN_POINT('Ctrl Pts',(-17.3800811280718,12.6529923851621,
132.932185918228)) ;
#142072=CARTESIAN_POINT('Ctrl Pts',(-17.2955087487444,12.5055873938463,
132.718493138558)) ;
#142073=CARTESIAN_POINT('Ctrl Pts',(-17.2021020536049,12.4255318492028,
132.478568577667)) ;
#142074=CARTESIAN_POINT('Ctrl Pts',(-17.1042647123247,12.41606276029,132.2258939674)) ;
#142075=CARTESIAN_POINT('Ctrl Pts',(-17.0088005914449,12.478829942444,131.980130586559)) ;
#142076=CARTESIAN_POINT('Ctrl Pts',(-16.9215448155793,12.6096603386007,
131.758445231646)) ;
#142077=CARTESIAN_POINT('Ctrl Pts',(-16.848533723708,12.7985462969973,131.578279303791)) ;
#142078=CARTESIAN_POINT('Ctrl Pts',(-16.7940414763144,13.0317087125592,
131.452162324081)) ;
#142079=CARTESIAN_POINT('Ctrl Pts',(-16.7611013224607,13.2930836864475,
131.389038106982)) ;
#142080=CARTESIAN_POINT('Ctrl Pts',(-16.7513989370885,13.5641925745626,
131.393845489194)) ;
#142081=CARTESIAN_POINT('Ctrl Pts',(-16.7650967126463,13.8256807565213,
131.46708434546)) ;
#142082=CARTESIAN_POINT('Ctrl Pts',(-16.8001170901404,14.0565823950309,
131.602366827208)) ;
#142083=CARTESIAN_POINT('Ctrl Pts',(-16.853538816955,14.2434411721512,131.791567853675)) ;
#142084=CARTESIAN_POINT('Ctrl Pts',(-16.9209280070917,14.3714533932326,
132.021637857135)) ;
#142085=CARTESIAN_POINT('Ctrl Pts',(-16.9960840169429,14.4311593781317,
132.274200346814)) ;
#142086=CARTESIAN_POINT('Ctrl Pts',(-17.0737363474756,14.4188767221607,
132.534241998506)) ;
#142087=CARTESIAN_POINT('Ctrl Pts',(-17.1469202195293,14.3353893492018,
132.781100248646)) ;
#142088=CARTESIAN_POINT('Ctrl Pts',(-17.2102141809998,14.1858865785186,
132.999227503805)) ;
#142089=CARTESIAN_POINT('Ctrl Pts',(-17.257730654902,13.982932266947,133.171038872199)) ;
#142090=CARTESIAN_POINT('Ctrl Pts',(-17.2859586154811,13.7386001468469,
133.286713511024)) ;
#142091=CARTESIAN_POINT('Ctrl Pts',(-17.291722530296,13.472491032427,133.336641515932)) ;
#142092=CARTESIAN_POINT('Ctrl Pts',(-17.2741574542646,13.2027754330182,
133.318428828081)) ;
#142093=CARTESIAN_POINT('Ctrl Pts',(-17.233357936349,12.947572926699,133.232521523896)) ;
#142094=CARTESIAN_POINT('Ctrl Pts',(-17.1723162295254,12.7286906750514,
133.08716241814)) ;
#142095=CARTESIAN_POINT('Ctrl Pts',(-17.0940329814276,12.5582194191414,
132.891590931029)) ;
#142096=CARTESIAN_POINT('Ctrl Pts',(-17.003220735762,12.4495814743775,132.65952031743)) ;
#142097=CARTESIAN_POINT('Ctrl Pts',(-16.9063349510849,12.4111325032394,
132.409580555585)) ;
#142098=CARTESIAN_POINT('Ctrl Pts',(-16.8093564797719,12.4448573223553,
132.159334717268)) ;
#142099=CARTESIAN_POINT('Ctrl Pts',(-16.7181348033276,12.5485736252265,
131.925983075815)) ;
#142100=CARTESIAN_POINT('Ctrl Pts',(-16.6384335148824,12.7160675406203,
131.726443646401)) ;
#142101=CARTESIAN_POINT('Ctrl Pts',(-16.5761662546992,12.9327061663297,
131.577552509025)) ;
#142102=CARTESIAN_POINT('Ctrl Pts',(-16.5341642871538,13.1846668461228,
131.4879329288)) ;
#142103=CARTESIAN_POINT('Ctrl Pts',(-16.5149327205021,13.4544224662781,
131.464916019242)) ;
#142104=CARTESIAN_POINT('Ctrl Pts',(-16.5192086330336,13.7215757501031,
131.510525864953)) ;
#142105=CARTESIAN_POINT('Ctrl Pts',(-16.5459259073865,13.9674106040572,
131.621703691313)) ;
#142106=CARTESIAN_POINT('Ctrl Pts',(-16.5923467307556,14.1739595566239,
131.790386254332)) ;
#142107=CARTESIAN_POINT('Ctrl Pts',(-16.6546298745393,14.3272529144105,
132.00549077589)) ;
#142108=CARTESIAN_POINT('Ctrl Pts',(-16.7275392721876,14.4155298054197,
132.25165131066)) ;
#142109=CARTESIAN_POINT('Ctrl Pts',(-16.8047539631414,14.4326688880929,
132.510258938982)) ;
#142110=CARTESIAN_POINT('Ctrl Pts',(-16.8806059328636,14.3775210612736,
132.765014735693)) ;
#142111=CARTESIAN_POINT('Ctrl Pts',(-16.948497815144,14.2540409039206,132.996451811014)) ;
#142112=CARTESIAN_POINT('Ctrl Pts',(-17.0030423303969,14.0709647731437,
133.188927025101)) ;
#142113=CARTESIAN_POINT('Ctrl Pts',(-17.0395041310645,13.8416199051522,
133.328550909828)) ;
#142114=CARTESIAN_POINT('Ctrl Pts',(-17.0546215409426,13.5823884703292,
133.405817397953)) ;
#142115=CARTESIAN_POINT('Ctrl Pts',(-17.0465466847866,13.3112803473401,
133.41538970088)) ;
#142116=CARTESIAN_POINT('Ctrl Pts',(-17.0150799598172,13.0483997002377,
133.356605998046)) ;
#142117=CARTESIAN_POINT('Ctrl Pts',(-16.9619997380882,12.8130297532618,
133.234583750432)) ;
#142118=CARTESIAN_POINT('Ctrl Pts',(-16.8900010563963,12.6204060162552,
133.057421174726)) ;
#142119=CARTESIAN_POINT('Ctrl Pts',(-16.8034708183318,12.4854478919258,
132.837862758507)) ;
#142120=CARTESIAN_POINT('Ctrl Pts',(-16.7086924678089,12.4181326606572,
132.593999330846)) ;
#142121=CARTESIAN_POINT('Ctrl Pts',(-16.6104956156241,12.4224942646145,
132.340376856576)) ;
#142122=CARTESIAN_POINT('Ctrl Pts',(-16.5161424264609,12.4989653492952,
132.097884581704)) ;
#142123=CARTESIAN_POINT('Ctrl Pts',(-16.4317556020667,12.6405920086238,
131.884334903027)) ;
#142124=CARTESIAN_POINT('Ctrl Pts',(-16.3616746574105,12.8391594148647,
131.71279689553)) ;
#142125=CARTESIAN_POINT('Ctrl Pts',(-16.3108304239017,13.0802460396382,
131.59750363429)) ;
#142126=CARTESIAN_POINT('Ctrl Pts',(-16.2823238978487,13.3449462912613,
131.54733314331)) ;
#142127=CARTESIAN_POINT('Ctrl Pts',(-16.2771309839151,13.614299734848,131.565154678749)) ;
#142128=CARTESIAN_POINT('Ctrl Pts',(-16.2949010006599,13.8710421702277,
131.65018620171)) ;
#142129=CARTESIAN_POINT('Ctrl Pts',(-16.3338452049706,14.0962488627573,
131.797148934845)) ;
#142130=CARTESIAN_POINT('Ctrl Pts',(-16.3905407253916,14.272991429521,131.996013377583)) ;
#142131=CARTESIAN_POINT('Ctrl Pts',(-16.4592327826985,14.3876795568682,
132.229561597162)) ;
#142132=CARTESIAN_POINT('Ctrl Pts',(-16.5357659030759,14.4346057862448,
132.486378414112)) ;
#142133=CARTESIAN_POINT('Ctrl Pts',(-16.613055863645,14.4082599424993,132.74533988594)) ;
#142134=CARTESIAN_POINT('Ctrl Pts',(-16.6845204129575,14.3122705822436,
132.98706452462)) ;
#142135=CARTESIAN_POINT('Ctrl Pts',(-16.7454150213927,14.1514361820495,
133.198229674243)) ;
#142136=CARTESIAN_POINT('Ctrl Pts',(-16.7896253783432,13.9387188784373,
133.36051515223)) ;
#142137=CARTESIAN_POINT('Ctrl Pts',(-16.8136464583059,13.6904434149952,
133.463667989134)) ;
#142138=CARTESIAN_POINT('Ctrl Pts',(-16.8150989773608,13.4208420632377,
133.501172955387)) ;
#142139=CARTESIAN_POINT('Ctrl Pts',(-16.7930957689776,13.1534853920285,
133.469895702491)) ;
#142140=CARTESIAN_POINT('Ctrl Pts',(-16.7485502511386,12.9044050276542,
133.372879092163)) ;
#142141=CARTESIAN_POINT('Ctrl Pts',(-16.6833056672716,12.691347593862,133.215606346478)) ;
#142142=CARTESIAN_POINT('Ctrl Pts',(-16.6023121457365,12.5324268950077,
133.012069499167)) ;
#142143=CARTESIAN_POINT('Ctrl Pts',(-16.510247041001,12.4369854895294,132.776191038926)) ;
#142144=CARTESIAN_POINT('Ctrl Pts',(-16.4129292753124,12.4119049764517,
132.52496184791)) ;
#142145=CARTESIAN_POINT('Ctrl Pts',(-16.3162560708554,12.4592885985088,
132.275727976682)) ;
#142146=CARTESIAN_POINT('Ctrl Pts',(-16.2269249209603,12.575733706437,132.047883576996)) ;
#142147=CARTESIAN_POINT('Ctrl Pts',(-16.1503960745848,12.7527803278304,
131.857442783129)) ;
#142148=CARTESIAN_POINT('Ctrl Pts',(-16.0912973211166,12.9786618836061,
131.718025410541)) ;
#142149=CARTESIAN_POINT('Ctrl Pts',(-16.053563244281,13.2359089048801,131.640933230899)) ;
#142150=CARTESIAN_POINT('Ctrl Pts',(-16.0388435174732,13.5051027063819,
131.630895828566)) ;
#142151=CARTESIAN_POINT('Ctrl Pts',(-16.047530549604,13.771120969237,131.689577950022)) ;
#142152=CARTESIAN_POINT('Ctrl Pts',(-16.078229877861,14.0100004351276,131.812285143493)) ;
#142153=CARTESIAN_POINT('Ctrl Pts',(-16.1279007148338,14.2073725024461,
131.990439316612)) ;
#142154=CARTESIAN_POINT('Ctrl Pts',(-16.1927067195232,14.3492226720416,
132.212956820855)) ;
#142155=CARTESIAN_POINT('Ctrl Pts',(-16.2667592579309,14.4242520037555,
132.462368666128)) ;
#142156=CARTESIAN_POINT('Ctrl Pts',(-16.3443760925168,14.4277364435235,
132.722252547872)) ;
#142157=CARTESIAN_POINT('Ctrl Pts',(-16.4190218197498,14.3592419699784,
132.973404327502)) ;
#142158=CARTESIAN_POINT('Ctrl Pts',(-16.4847503849809,14.2240686259208,
133.198484837379)) ;
#142159=CARTESIAN_POINT('Ctrl Pts',(-16.5363595036201,14.0305584607837,
133.38248100773)) ;
#142160=CARTESIAN_POINT('Ctrl Pts',(-16.5689433106285,13.7945205251559,
133.510729343035)) ;
#142161=CARTESIAN_POINT('Ctrl Pts',(-16.5797941428791,13.5313066856814,
133.575579533295)) ;
#142162=CARTESIAN_POINT('Ctrl Pts',(-16.567251148853,13.2605191131678,133.57206289759)) ;
#142163=CARTESIAN_POINT('Ctrl Pts',(-16.5315770470974,13.0015410285169,
133.50095404784)) ;
#142164=CARTESIAN_POINT('Ctrl Pts',(-16.4745328734589,12.7725523248786,
133.367443152597)) ;
#142165=CARTESIAN_POINT('Ctrl Pts',(-16.3994606288027,12.5901313640957,
133.181279217731)) ;
#142166=CARTESIAN_POINT('Ctrl Pts',(-16.3110718117679,12.4675131143056,
132.956201420078)) ;
#142167=CARTESIAN_POINT('Ctrl Pts',(-16.2150465684198,12.4133289099041,
132.708783471555)) ;
#142168=CARTESIAN_POINT('Ctrl Pts',(-16.1172756530906,12.4315113584402,
132.456324766904)) ;
#142169=CARTESIAN_POINT('Ctrl Pts',(-16.0245054184323,12.5204618944922,
132.218365021381)) ;
#142170=CARTESIAN_POINT('Ctrl Pts',(-15.9421012205372,12.6740885855686,
132.010764917566)) ;
#142171=CARTESIAN_POINT('Ctrl Pts',(-15.875367634635,12.8820605871686,131.849026621626)) ;
#142172=CARTESIAN_POINT('Ctrl Pts',(-15.8287083770857,13.1280849227168,
131.74581643471)) ;
#142173=CARTESIAN_POINT('Ctrl Pts',(-15.8044325587747,13.3954305595711,
131.70802549061)) ;
#142174=CARTESIAN_POINT('Ctrl Pts',(-15.8036483197092,13.664772130159,131.738860618359)) ;
#142175=CARTESIAN_POINT('Ctrl Pts',(-15.825629308736,13.916650368435,131.836174288953)) ;
#142176=CARTESIAN_POINT('Ctrl Pts',(-15.8681455318913,14.1333087809813,
131.993506201505)) ;
#142177=CARTESIAN_POINT('Ctrl Pts',(-15.927193309252,14.2989356818664,132.199046381853)) ;
#142178=CARTESIAN_POINT('Ctrl Pts',(-15.9986879065092,14.4025578141661,
132.44125861652)) ;
#142179=CARTESIAN_POINT('Ctrl Pts',(-16.0751723449273,14.4350103980761,
132.697614959121)) ;
#142180=CARTESIAN_POINT('Ctrl Pts',(-16.1518509504202,14.3956728073431,
132.954753133988)) ;
#142181=CARTESIAN_POINT('Ctrl Pts',(-16.2220068716851,14.2862787528374,
133.192841857477)) ;
#142182=CARTESIAN_POINT('Ctrl Pts',(-16.2797925866452,14.1158603426533,
133.394685682589)) ;
#142183=CARTESIAN_POINT('Ctrl Pts',(-16.3207945954701,13.8934485150928,
133.547842676703)) ;
#142184=CARTESIAN_POINT('Ctrl Pts',(-16.3405803998949,13.6404741079279,
133.638562788148)) ;
#142185=CARTESIAN_POINT('Ctrl Pts',(-16.3376032483563,13.3695006911583,
133.663119999001)) ;
#142186=CARTESIAN_POINT('Ctrl Pts',(-16.3112454472243,13.1044456788723,
133.619106817927)) ;
#142187=CARTESIAN_POINT('Ctrl Pts',(-16.2625596253282,12.8607039818763,
133.510049336795)) ;
#142188=CARTESIAN_POINT('Ctrl Pts',(-16.1940271721615,12.6571154322834,
133.343090977728)) ;
#142189=CARTESIAN_POINT('Ctrl Pts',(-16.1108795002955,12.509808022699,133.133139897156)) ;
#142190=CARTESIAN_POINT('Ctrl Pts',(-16.0171502461323,12.4266891378063,
132.892483711977)) ;
#142191=CARTESIAN_POINT('Ctrl Pts',(-15.919067834617,12.4154229833254,132.639178441848)) ;
#142192=CARTESIAN_POINT('Ctrl Pts',(-15.8237916187375,12.4759771003581,
132.393848463188)) ;
#142193=CARTESIAN_POINT('Ctrl Pts',(-15.7361936167486,12.6048252979973,
132.171163013204)) ;
#142194=CARTESIAN_POINT('Ctrl Pts',(-15.6626673506394,12.792164644416,131.989497153743)) ;
#142195=CARTESIAN_POINT('Ctrl Pts',(-15.6074901711292,13.0247863190839,
131.861453094695)) ;
#142196=CARTESIAN_POINT('Ctrl Pts',(-15.5739200759961,13.2853106439738,
131.796445961381)) ;
#142197=CARTESIAN_POINT('Ctrl Pts',(-15.5636021153955,13.5574332084958,
131.799586177716)) ;
#142198=CARTESIAN_POINT('Ctrl Pts',(-15.5764802743328,13.8171022396022,
131.870118715194)) ;
#142199=CARTESIAN_POINT('Ctrl Pts',(-15.611132431221,14.051173953077,132.004607403079)) ;
#142200=CARTESIAN_POINT('Ctrl Pts',(-15.6640759803966,14.2388282531697,
132.192340452033)) ;
#142201=CARTESIAN_POINT('Ctrl Pts',(-15.7308833601088,14.3685839592775,
132.420606589598)) ;
#142202=CARTESIAN_POINT('Ctrl Pts',(-15.8064742715662,14.4305511556418,
132.674695319148)) ;
#142203=CARTESIAN_POINT('Ctrl Pts',(-15.8835822303502,14.4203097239978,
132.93289312949)) ;
#142204=CARTESIAN_POINT('Ctrl Pts',(-15.9573192391447,14.3384207836783,
133.181537405768)) ;
#142205=CARTESIAN_POINT('Ctrl Pts',(-16.0206561333224,14.1915731436481,
133.399594202983)) ;
#142206=CARTESIAN_POINT('Ctrl Pts',(-16.0690536966344,13.9880714714153,
133.574284718797)) ;
#142207=CARTESIAN_POINT('Ctrl Pts',(-16.0975526481624,13.7471725052838,
133.690391133825)) ;
#142208=CARTESIAN_POINT('Ctrl Pts',(-16.1041169388077,13.4800206037099,
133.742852683177)) ;
#142209=CARTESIAN_POINT('Ctrl Pts',(-16.0872443704174,13.2110030429649,
133.726550659017)) ;
#142210=CARTESIAN_POINT('Ctrl Pts',(-16.0471230753564,12.9547748927777,
133.64265811564)) ;
#142211=CARTESIAN_POINT('Ctrl Pts',(-15.9865759612961,12.7344342247069,
133.498774691296)) ;
#142212=CARTESIAN_POINT('Ctrl Pts',(-15.9086915708439,12.5623453660856,
133.304378900685)) ;
#142213=CARTESIAN_POINT('Ctrl Pts',(-15.8183465306617,12.4518692088092,
133.073606369183)) ;
#142214=CARTESIAN_POINT('Ctrl Pts',(-15.7212787432989,12.4112334911996,
132.823235526097)) ;
#142215=CARTESIAN_POINT('Ctrl Pts',(-15.6243186466118,12.442749147776,132.572999265293)) ;
#142216=CARTESIAN_POINT('Ctrl Pts',(-15.5323128334074,12.5456206773071,
132.337577591656)) ;
#142217=CARTESIAN_POINT('Ctrl Pts',(-15.453258603987,12.7091960236905,132.139476652336)) ;
#142218=CARTESIAN_POINT('Ctrl Pts',(-15.3898383285792,12.9259029773537,
131.987475859056)) ;
#142219=CARTESIAN_POINT('Ctrl Pts',(-15.3472877469184,13.1770736237047,
131.896231444798)) ;
#142220=CARTESIAN_POINT('Ctrl Pts',(-15.3273612325374,13.4468768400015,
131.871223050135)) ;
#142221=CARTESIAN_POINT('Ctrl Pts',(-15.3309764443274,13.7138795897728,
131.914840701596)) ;
#142222=CARTESIAN_POINT('Ctrl Pts',(-15.3570417967896,13.9605431985016,
132.024107079577)) ;
#142223=CARTESIAN_POINT('Ctrl Pts',(-15.4029179113879,14.1686235654109,
132.191205295214)) ;
#142224=CARTESIAN_POINT('Ctrl Pts',(-15.4651226728873,14.324111284162,132.406226710796)) ;
#142225=CARTESIAN_POINT('Ctrl Pts',(-15.5374063763882,14.4138215880485,
132.650368768959)) ;
#142226=CARTESIAN_POINT('Ctrl Pts',(-15.6148696071944,14.4331945050443,
132.909835134181)) ;
#142227=CARTESIAN_POINT('Ctrl Pts',(-15.6906277120936,14.3801614626116,
133.164214215321)) ;
#142228=CARTESIAN_POINT('Ctrl Pts',(-15.7589271578745,14.2584942565519,
133.396886988434)) ;
#142229=CARTESIAN_POINT('Ctrl Pts',(-15.8138969641916,14.0770491380578,
133.590585730492)) ;
#142230=CARTESIAN_POINT('Ctrl Pts',(-15.8510060052898,13.8484874642558,
133.732152268361)) ;
#142231=CARTESIAN_POINT('Ctrl Pts',(-15.8667131197633,13.5893549989453,
133.811197408128)) ;
#142232=CARTESIAN_POINT('Ctrl Pts',(-15.8593406152276,13.319692173746,133.822652269934)) ;
#142233=CARTESIAN_POINT('Ctrl Pts',(-15.8286128783071,13.0561133199218,
133.76604483536)) ;
#142234=CARTESIAN_POINT('Ctrl Pts',(-15.7759801790062,12.8190740737043,
133.645417619665)) ;
#142235=CARTESIAN_POINT('Ctrl Pts',(-15.7045036655101,12.6252975626819,
133.469748009719)) ;
#142236=CARTESIAN_POINT('Ctrl Pts',(-15.6186604888065,12.4887796662223,
133.252078050461)) ;
#142237=CARTESIAN_POINT('Ctrl Pts',(-15.5236958147091,12.4190606373648,
133.007800237169)) ;
#142238=CARTESIAN_POINT('Ctrl Pts',(-15.4258603341632,12.4213023433048,
132.755107590907)) ;
#142239=CARTESIAN_POINT('Ctrl Pts',(-15.3312661273055,12.4953372710628,
132.511916145083)) ;
#142240=CARTESIAN_POINT('Ctrl Pts',(-15.2461014219628,12.6358733450884,
132.296256624047)) ;
#142241=CARTESIAN_POINT('Ctrl Pts',(-15.1757623763379,12.8325870207608,
132.12387434654)) ;
#142242=CARTESIAN_POINT('Ctrl Pts',(-15.1244118681695,13.0715963225307,
132.006975021887)) ;
#142243=CARTESIAN_POINT('Ctrl Pts',(-15.0950340623661,13.336692941588,131.954373590249)) ;
#142244=CARTESIAN_POINT('Ctrl Pts',(-15.0891646881233,13.6067854476423,
131.970293382415)) ;
#142245=CARTESIAN_POINT('Ctrl Pts',(-15.1063211628653,13.8640947363139,
132.05352643624)) ;
#142246=CARTESIAN_POINT('Ctrl Pts',(-15.1445701006616,14.089839779911,132.198362269326)) ;
#142247=CARTESIAN_POINT('Ctrl Pts',(-15.2007425773632,14.2683601910573,
132.395691390543)) ;
#142248=CARTESIAN_POINT('Ctrl Pts',(-15.2694132319916,14.385487730189,132.629307915259)) ;
#142249=CARTESIAN_POINT('Ctrl Pts',(-15.3459082333124,14.4341894586694,
132.886044120066)) ;
#142250=CARTESIAN_POINT('Ctrl Pts',(-15.4228395829729,14.4102459791679,
133.143771383713)) ;
#142251=CARTESIAN_POINT('Ctrl Pts',(-15.494944359048,14.3157190447574,133.387554110632)) ;
#142252=CARTESIAN_POINT('Ctrl Pts',(-15.5558765426031,14.1574302898824,
133.598637081667)) ;
#142253=CARTESIAN_POINT('Ctrl Pts',(-15.6008224271939,13.9458829058386,
133.763138208487)) ;
#142254=CARTESIAN_POINT('Ctrl Pts',(-15.6255201649115,13.6969896283466,
133.868443529266)) ;
#142255=CARTESIAN_POINT('Ctrl Pts',(-15.6275786112566,13.4292803806108,
133.907520168097)) ;
#142256=CARTESIAN_POINT('Ctrl Pts',(-15.6063759832611,13.1613091083809,
133.878612288534)) ;
#142257=CARTESIAN_POINT('Ctrl Pts',(-15.5619644958359,12.9096301895175,
133.78225128118)) ;
#142258=CARTESIAN_POINT('Ctrl Pts',(-15.4979303513307,12.6977069155964,
133.628145147095)) ;
#142259=CARTESIAN_POINT('Ctrl Pts',(-15.417114271924,12.536159176258,133.425257288799)) ;
#142260=CARTESIAN_POINT('Ctrl Pts',(-15.3252949349401,12.4388403103588,
133.190087141283)) ;
#142261=CARTESIAN_POINT('Ctrl Pts',(-15.2279404799318,12.4115721830993,
132.93878796517)) ;
#142262=CARTESIAN_POINT('Ctrl Pts',(-15.1310969074068,12.457029419961,132.689076414865)) ;
#142263=CARTESIAN_POINT('Ctrl Pts',(-15.0416608970638,12.5713337690677,
132.460857982082)) ;
#142264=CARTESIAN_POINT('Ctrl Pts',(-14.9646158772577,12.7468028835324,
132.268928751753)) ;
#142265=CARTESIAN_POINT('Ctrl Pts',(-14.9049751892106,12.9715573467482,
132.127931845598)) ;
#142266=CARTESIAN_POINT('Ctrl Pts',(-14.8666141904923,13.2272671930713,
132.0489034762)) ;
#142267=CARTESIAN_POINT('Ctrl Pts',(-14.8511623659717,13.4980619502807,
132.036944216363)) ;
#142268=CARTESIAN_POINT('Ctrl Pts',(-14.8590704558367,13.7620975253013,
132.093037654942)) ;
#142269=CARTESIAN_POINT('Ctrl Pts',(-14.8892480575814,14.0037249771829,
132.21444701514)) ;
#142270=CARTESIAN_POINT('Ctrl Pts',(-14.9384427260129,14.202400093294,132.391194252055)) ;
#142271=CARTESIAN_POINT('Ctrl Pts',(-15.0030756975973,14.3463073278919,
132.613297185418)) ;
#142272=CARTESIAN_POINT('Ctrl Pts',(-15.0766441588427,14.4229407274136,
132.861156433463)) ;
#142273=CARTESIAN_POINT('Ctrl Pts',(-15.1542518269372,14.4287087096985,
133.121019796098)) ;
#142274=CARTESIAN_POINT('Ctrl Pts',(-15.2291034561164,14.3623691322231,
133.37277976698)) ;
#142275=CARTESIAN_POINT('Ctrl Pts',(-15.2954353285377,14.2283779056864,
133.599762615258)) ;
#142276=CARTESIAN_POINT('Ctrl Pts',(-15.3473792259273,14.0364255545022,
133.784686288565)) ;
#142277=CARTESIAN_POINT('Ctrl Pts',(-15.3804798619707,13.8020943881553,
133.914354405728)) ;
#142278=CARTESIAN_POINT('Ctrl Pts',(-15.3920181078753,13.5391612776222,
133.981245241876)) ;
#142279=CARTESIAN_POINT('Ctrl Pts',(-15.3801942480057,13.268618582974,133.979790178508)) ;
#142280=CARTESIAN_POINT('Ctrl Pts',(-15.3451113205383,13.0086418344895,
133.910463378564)) ;
#142281=CARTESIAN_POINT('Ctrl Pts',(-15.2888485505009,12.7791079862287,
133.779136483972)) ;
#142282=CARTESIAN_POINT('Ctrl Pts',(-15.2138964639745,12.5942976841109,
133.59347890567)) ;
#142283=CARTESIAN_POINT('Ctrl Pts',(-15.1261222353351,12.4702970290912,
133.370074169085)) ;
#142284=CARTESIAN_POINT('Ctrl Pts',(-15.0300476900928,12.4139049816003,
133.122583731637)) ;
#142285=CARTESIAN_POINT('Ctrl Pts',(-14.9325665835877,12.4297924440583,
132.870854131327)) ;
#142286=CARTESIAN_POINT('Ctrl Pts',(-14.838960003689,12.5172147656158,132.63066535824)) ;
#142287=CARTESIAN_POINT('Ctrl Pts',(-14.7562177989916,12.6696686051205,
132.422099640111)) ;
#142288=CARTESIAN_POINT('Ctrl Pts',(-14.6894014584479,12.8748936311913,
132.259900679124)) ;
#142289=CARTESIAN_POINT('Ctrl Pts',(-14.6419381314949,13.1206629569548,
132.154439065691)) ;
#142290=CARTESIAN_POINT('Ctrl Pts',(-14.617022067619,13.3874987151297,132.114753350066)) ;
#142291=CARTESIAN_POINT('Ctrl Pts',(-14.6155607269755,13.6577700593923,
132.143697626099)) ;
#142292=CARTESIAN_POINT('Ctrl Pts',(-14.6370052322387,13.9102263629719,
132.239439325318)) ;
#142293=CARTESIAN_POINT('Ctrl Pts',(-14.6787534379256,14.127342135122,132.394384380573)) ;
#142294=CARTESIAN_POINT('Ctrl Pts',(-14.737766120839,14.2954362012379,132.600024203604)) ;
#142295=CARTESIAN_POINT('Ctrl Pts',(-14.8083643434813,14.400199046936,132.839317925707)) ;
#142296=CARTESIAN_POINT('Ctrl Pts',(-14.8854780825288,14.4351706373417,
133.097830821909)) ;
#142297=CARTESIAN_POINT('Ctrl Pts',(-14.9618174412002,14.3977719560938,
133.35379058418)) ;
#142298=CARTESIAN_POINT('Ctrl Pts',(-15.0324040200964,14.2904204320916,
133.59319366883)) ;
#142299=CARTESIAN_POINT('Ctrl Pts',(-15.090764871553,14.1205426182846,133.796859479231)) ;
#142300=CARTESIAN_POINT('Ctrl Pts',(-15.1319227402497,13.9015880180689,
133.95013819427)) ;
#142301=CARTESIAN_POINT('Ctrl Pts',(-15.1525599707839,13.6483197429669,
134.043502414266)) ;
#142302=CARTESIAN_POINT('Ctrl Pts',(-15.1502448946848,13.3774459783215,
134.069996708961)) ;
#142303=CARTESIAN_POINT('Ctrl Pts',(-15.1244931600293,13.1115163789139,
134.027817890031)) ;
#142304=CARTESIAN_POINT('Ctrl Pts',(-15.0765141667085,12.867627711837,133.920732027969)) ;
#142305=CARTESIAN_POINT('Ctrl Pts',(-15.0088413137702,12.6630941323673,
133.756165950852)) ;
#142306=CARTESIAN_POINT('Ctrl Pts',(-14.9254870825308,12.5128296370691,
133.545852043451)) ;
#142307=CARTESIAN_POINT('Ctrl Pts',(-14.8319589407702,12.4280522080275,
133.305771576008)) ;
#142308=CARTESIAN_POINT('Ctrl Pts',(-14.7340778039936,12.4147676790035,
133.052999941768)) ;
#142309=CARTESIAN_POINT('Ctrl Pts',(-14.6386324749928,12.4732052495888,
132.807177718268)) ;
#142310=CARTESIAN_POINT('Ctrl Pts',(-14.5504362769443,12.6008830846757,
132.582865547777)) ;
#142311=CARTESIAN_POINT('Ctrl Pts',(-14.4768576797366,12.7859101152191,
132.400880133504)) ;
#142312=CARTESIAN_POINT('Ctrl Pts',(-14.4210707390125,13.0171550939707,
132.271032735321)) ;
#142313=CARTESIAN_POINT('Ctrl Pts',(-14.3868017963535,13.2774025189781,
132.204022588309)) ;
#142314=CARTESIAN_POINT('Ctrl Pts',(-14.3757654194404,13.5492093049786,
132.205023339175)) ;
#142315=CARTESIAN_POINT('Ctrl Pts',(-14.3880514684394,13.8101283643081,
132.273924034985)) ;
#142316=CARTESIAN_POINT('Ctrl Pts',(-14.4219003231422,14.0442617204232,
132.405903677218)) ;
#142317=CARTESIAN_POINT('Ctrl Pts',(-14.4747801059438,14.2348997538622,
132.593713095369)) ;
#142318=CARTESIAN_POINT('Ctrl Pts',(-14.5409603434691,14.3654883224984,
132.819967847917)) ;
#142319=CARTESIAN_POINT('Ctrl Pts',(-14.6161864464348,14.4297229265612,
133.072916709743)) ;
#142320=CARTESIAN_POINT('Ctrl Pts',(-14.6935812312555,14.421668005349,133.33206349666)) ;
#142321=CARTESIAN_POINT('Ctrl Pts',(-14.7675434877312,14.3417420843685,
133.5813725027)) ;
#142322=CARTESIAN_POINT('Ctrl Pts',(-14.8312585222105,14.1964291100303,
133.800560188562)) ;
#142323=CARTESIAN_POINT('Ctrl Pts',(-14.8799642737121,13.9955518397601,
133.975972972826)) ;
#142324=CARTESIAN_POINT('Ctrl Pts',(-14.9093078343249,13.7541464168563,
134.094757838791)) ;
#142325=CARTESIAN_POINT('Ctrl Pts',(-14.9164487725813,13.4873870374965,
134.148893971889)) ;
#142326=CARTESIAN_POINT('Ctrl Pts',(-14.9002547065785,13.2187118678006,
134.134518709842)) ;
#142327=CARTESIAN_POINT('Ctrl Pts',(-14.8609138929022,12.9622340205071,
134.052837189393)) ;
#142328=CARTESIAN_POINT('Ctrl Pts',(-14.8006595820543,12.7396654906289,
133.909958025568)) ;
#142329=CARTESIAN_POINT('Ctrl Pts',(-14.7231765654135,12.5663130117826,
133.716718287322)) ;
#142330=CARTESIAN_POINT('Ctrl Pts',(-14.6335055175769,12.4542929765583,
133.487776150199)) ;
#142331=CARTESIAN_POINT('Ctrl Pts',(-14.536209707559,12.4113060992836,133.236853912787)) ;
#142332=CARTESIAN_POINT('Ctrl Pts',(-14.4393435905948,12.4409729765678,
132.986840999606)) ;
#142333=CARTESIAN_POINT('Ctrl Pts',(-14.3475507084136,12.5408195809103,
132.751846613996)) ;
#142334=CARTESIAN_POINT('Ctrl Pts',(-14.2671647163194,12.7045177174677,
132.550230917324)) ;
#142335=CARTESIAN_POINT('Ctrl Pts',(-14.2035979096792,12.919412680773,132.397665865524)) ;
#142336=CARTESIAN_POINT('Ctrl Pts',(-14.1604688985404,13.1689179430447,
132.304632041467)) ;
#142337=CARTESIAN_POINT('Ctrl Pts',(-14.139782678841,13.4397285825566,132.277557000125)) ;
#142338=CARTESIAN_POINT('Ctrl Pts',(-14.142785048101,13.7064270622518,132.319308711258)) ;
#142339=CARTESIAN_POINT('Ctrl Pts',(-14.1682103421544,13.9538863073551,
132.426697860702)) ;
#142340=CARTESIAN_POINT('Ctrl Pts',(-14.2135281033141,14.163192773507,132.592143093095)) ;
#142341=CARTESIAN_POINT('Ctrl Pts',(-14.2753850982946,14.3205261321744,
132.806174358066)) ;
#142342=CARTESIAN_POINT('Ctrl Pts',(-14.3473411439298,14.4121066537417,
133.049314213563)) ;
#142343=CARTESIAN_POINT('Ctrl Pts',(-14.4248089805252,14.433704272446,133.308819308561)) ;
#142344=CARTESIAN_POINT('Ctrl Pts',(-14.5007784378179,14.3826278008681,
133.563851701539)) ;
#142345=CARTESIAN_POINT('Ctrl Pts',(-14.5693363275554,14.2628852203127,
133.797259307275)) ;
#142346=CARTESIAN_POINT('Ctrl Pts',(-14.6247737505551,14.0829261229302,
133.992336674271)) ;
#142347=CARTESIAN_POINT('Ctrl Pts',(-14.6624238056517,13.8556921301219,
134.135454195566)) ;
#142348=CARTESIAN_POINT('Ctrl Pts',(-14.6787751303134,13.5972598207812,
134.216376119518)) ;
#142349=CARTESIAN_POINT('Ctrl Pts',(-14.6721663860168,13.3277678231801,
134.230044601199)) ;
#142350=CARTESIAN_POINT('Ctrl Pts',(-14.6417520985073,13.061810881333,134.174606742694)) ;
#142351=CARTESIAN_POINT('Ctrl Pts',(-14.5901365318131,12.8260388711121,
134.056642369562)) ;
#142352=CARTESIAN_POINT('Ctrl Pts',(-14.5189277267524,12.6298695868286,
133.881890430345)) ;
#142353=CARTESIAN_POINT('Ctrl Pts',(-14.4334483620761,12.491768708706,133.665259640123)) ;
#142354=CARTESIAN_POINT('Ctrl Pts',(-14.3385453399518,12.4199839155212,
133.421203195212)) ;
#142355=CARTESIAN_POINT('Ctrl Pts',(-14.2407585005838,12.4203084391601,
133.168634581772)) ;
#142356=CARTESIAN_POINT('Ctrl Pts',(-14.1461361734331,12.492208510643,132.925307480569)) ;
#142357=CARTESIAN_POINT('Ctrl Pts',(-14.0605732797982,12.630997013847,132.708502600032)) ;
#142358=CARTESIAN_POINT('Ctrl Pts',(-13.9897130342082,12.8263312491105,
132.53460873687)) ;
#142359=CARTESIAN_POINT('Ctrl Pts',(-13.9376533995034,13.0651229525308,
132.415734889569)) ;
#142360=CARTESIAN_POINT('Ctrl Pts',(-13.9077497589157,13.3295669294852,
132.361565342467)) ;
#142361=CARTESIAN_POINT('Ctrl Pts',(-13.901216822791,13.5989125314577,132.375443730603)) ;
#142362=CARTESIAN_POINT('Ctrl Pts',(-13.9177760025398,13.8574711990645,
132.457011745281)) ;
#142363=CARTESIAN_POINT('Ctrl Pts',(-13.9553957581231,14.08370800358,132.599924272669)) ;
#142364=CARTESIAN_POINT('Ctrl Pts',(-14.0110176386716,14.2638192585231,
132.795614384729)) ;
#142365=CARTESIAN_POINT('Ctrl Pts',(-14.0796276403271,14.3831696043844,
133.029163918101)) ;
#142366=CARTESIAN_POINT('Ctrl Pts',(-14.1557505767541,14.4337176712718,
133.284703197076)) ;
#142367=CARTESIAN_POINT('Ctrl Pts',(-14.2327802934375,14.4120588565301,
133.542734126691)) ;
#142368=CARTESIAN_POINT('Ctrl Pts',(-14.3052072147828,14.3193772826324,
133.787499406446)) ;
#142369=CARTESIAN_POINT('Ctrl Pts',(-14.3665740744773,14.1628170776178,
133.999858164627)) ;
#142370=CARTESIAN_POINT('Ctrl Pts',(-14.4121259724299,13.9515916120412,
134.166258760957)) ;
#142371=CARTESIAN_POINT('Ctrl Pts',(-14.4372801227629,13.7055233139094,
134.272631180499)) ;
#142372=CARTESIAN_POINT('Ctrl Pts',(-14.440046863088,13.4359481903885,134.314052320636)) ;
#142373=CARTESIAN_POINT('Ctrl Pts',(-14.4195164737538,13.1690262561277,
134.286945100641)) ;
#142374=CARTESIAN_POINT('Ctrl Pts',(-14.375727536596,12.9162728254293,134.192437995692)) ;
#142375=CARTESIAN_POINT('Ctrl Pts',(-14.3123844010594,12.7036779683092,
134.040261155373)) ;
#142376=CARTESIAN_POINT('Ctrl Pts',(-14.2321535671344,12.5403117617381,
133.839041349776)) ;
#142377=CARTESIAN_POINT('Ctrl Pts',(-14.1399646502613,12.4404489557871,
133.603011473166)) ;
#142378=CARTESIAN_POINT('Ctrl Pts',(-14.0431420853103,12.4114485631191,
133.353105162355)) ;
#142379=CARTESIAN_POINT('Ctrl Pts',(-13.9462412595183,12.4544846447878,
133.103205911968)) ;
#142380=CARTESIAN_POINT('Ctrl Pts',(-13.8561482718694,12.5672617831098,
132.873195369857)) ;
#142381=CARTESIAN_POINT('Ctrl Pts',(-13.7786242096377,12.741774518216,132.679929018516)) ;
#142382=CARTESIAN_POINT('Ctrl Pts',(-13.7188694411303,12.9633751206612,
132.538319767188)) ;
#142383=CARTESIAN_POINT('Ctrl Pts',(-13.6795051572281,13.2203112306522,
132.456621058414)) ;
#142384=CARTESIAN_POINT('Ctrl Pts',(-13.6635016097314,13.4905144393576,
132.442983868862)) ;
#142385=CARTESIAN_POINT('Ctrl Pts',(-13.6707757272997,13.7550217254887,
132.497240868873)) ;
#142386=CARTESIAN_POINT('Ctrl Pts',(-13.7002116917388,13.9967496932403,
132.616356096113)) ;
#142387=CARTESIAN_POINT('Ctrl Pts',(-13.7490260081706,14.1974243252069,
132.792087763225)) ;
#142388=CARTESIAN_POINT('Ctrl Pts',(-13.8129747901669,14.3425140414095,
133.012032809254)) ;
#142389=CARTESIAN_POINT('Ctrl Pts',(-13.8865372491761,14.4218016114581,
133.259977388133)) ;
#142390=CARTESIAN_POINT('Ctrl Pts',(-13.9645151712435,14.4294553389326,
133.521084372305)) ;
#142391=CARTESIAN_POINT('Ctrl Pts',(-14.0391560909907,14.3652617891387,
133.772071407551)) ;
#142392=CARTESIAN_POINT('Ctrl Pts',(-14.1057363531632,14.2335996006041,
133.999718577771)) ;
#142393=CARTESIAN_POINT('Ctrl Pts',(-14.1582660784627,14.0430657817291,
134.186391245985)) ;
#142394=CARTESIAN_POINT('Ctrl Pts',(-14.1920661990571,13.8093137336756,
134.318173223818)) ;
#142395=CARTESIAN_POINT('Ctrl Pts',(-14.2042127186391,13.5459138184761,
134.386958646077)) ;
#142396=CARTESIAN_POINT('Ctrl Pts',(-14.1930930657431,13.2769102523372,
134.387368892485)) ;
#142397=CARTESIAN_POINT('Ctrl Pts',(-14.1587186564867,13.0160045287208,
134.320145719112)) ;
#142398=CARTESIAN_POINT('Ctrl Pts',(-14.1028872041378,12.7850160477838,
134.190142176635)) ;
#142399=CARTESIAN_POINT('Ctrl Pts',(-14.028684171418,12.5991695463159,134.006558452314)) ;
#142400=CARTESIAN_POINT('Ctrl Pts',(-13.9407662015876,12.4727066402134,
133.782907583956)) ;
#142401=CARTESIAN_POINT('Ctrl Pts',(-13.8452936573205,12.414634000185,133.537011712374)) ;
#142402=CARTESIAN_POINT('Ctrl Pts',(-13.7475595496828,12.4282724908794,
133.28461799683)) ;
#142403=CARTESIAN_POINT('Ctrl Pts',(-13.6538542291428,12.5136822539145,
133.044102125595)) ;
#142404=CARTESIAN_POINT('Ctrl Pts',(-13.5707377115012,12.6640314349918,
132.834416071391)) ;
#142405=CARTESIAN_POINT('Ctrl Pts',(-13.5030136084428,12.8694014847424,
132.669787493301)) ;
#142406=CARTESIAN_POINT('Ctrl Pts',(-13.4553004590304,13.11284739186,132.563387011279)) ;
#142407=CARTESIAN_POINT('Ctrl Pts',(-13.4296313449615,13.3794714169119,
132.521528691967)) ;
#142408=CARTESIAN_POINT('Ctrl Pts',(-13.4274890180519,13.649387589438,132.548416277511)) ;
#142409=CARTESIAN_POINT('Ctrl Pts',(-13.4481636726345,13.9027716993511,
132.641905993097)) ;
#142410=CARTESIAN_POINT('Ctrl Pts',(-13.489766031508,14.1226004021729,132.796684089978)) ;
#142411=CARTESIAN_POINT('Ctrl Pts',(-13.5477833605945,14.2907614939367,
132.999088667497)) ;
#142412=CARTESIAN_POINT('Ctrl Pts',(-13.6187363184265,14.3985142695992,
133.239726637088)) ;
#142413=CARTESIAN_POINT('Ctrl Pts',(-13.6952590065994,14.4350393249369,
133.496283799514)) ;
#142414=CARTESIAN_POINT('Ctrl Pts',(-13.7718333962932,14.4000355942845,
133.752990096946)) ;
#142415=CARTESIAN_POINT('Ctrl Pts',(-13.8429167997199,14.294019259171,133.99396202455)) ;
#142416=CARTESIAN_POINT('Ctrl Pts',(-13.9014231128193,14.1264036787102,
134.197913623386)) ;
#142417=CARTESIAN_POINT('Ctrl Pts',(-13.9432439398755,13.908713601209,134.353150229304)) ;
#142418=CARTESIAN_POINT('Ctrl Pts',(-13.9645351703535,13.6545233253026,
134.448627889531)) ;
#142419=CARTESIAN_POINT('Ctrl Pts',(-13.9628501553954,13.385850090519,134.476712019796)) ;
#142420=CARTESIAN_POINT('Ctrl Pts',(-13.9378025080024,13.1190055030057,
134.43665730351)) ;
#142421=CARTESIAN_POINT('Ctrl Pts',(-13.8903445233776,12.8738785083339,
134.331138737956)) ;
#142422=CARTESIAN_POINT('Ctrl Pts',(-13.822976322165,12.6676053408392,134.167543118068)) ;
#142423=CARTESIAN_POINT('Ctrl Pts',(-13.7400513407993,12.5160770794409,
133.958438256977)) ;
#142424=CARTESIAN_POINT('Ctrl Pts',(-13.6471767557041,12.429744459131,133.72011489165)) ;
#142425=CARTESIAN_POINT('Ctrl Pts',(-13.5494411433701,12.4139325867349,
133.467730241205)) ;
#142426=CARTESIAN_POINT('Ctrl Pts',(-13.4532942032315,12.470818666654,133.220058381188)) ;
#142427=CARTESIAN_POINT('Ctrl Pts',(-13.3655312082867,12.5954481980338,
132.996719859513)) ;
#142428=CARTESIAN_POINT('Ctrl Pts',(-13.2909901735497,12.7795463836638,
132.812100132889)) ;
#142429=CARTESIAN_POINT('Ctrl Pts',(-13.2344956361294,13.0105019678005,
132.680282739157)) ;
#142430=CARTESIAN_POINT('Ctrl Pts',(-13.1996213955,13.2704660588973,132.611535276715)) ;
#142431=CARTESIAN_POINT('Ctrl Pts',(-13.1879877745145,13.5415026123175,
132.610702688434)) ;
#142432=CARTESIAN_POINT('Ctrl Pts',(-13.1995723958978,13.8030871080867,
132.677561568908)) ;
#142433=CARTESIAN_POINT('Ctrl Pts',(-13.2331003609654,14.0389748553007,
132.808744242538)) ;
#142434=CARTESIAN_POINT('Ctrl Pts',(-13.2848573473153,14.2290324993106,
132.992884454479)) ;
#142435=CARTESIAN_POINT('Ctrl Pts',(-13.3512130512097,14.3629001779689,
133.219942892695)) ;
#142436=CARTESIAN_POINT('Ctrl Pts',(-13.4261333638039,14.428830285179,133.471917113561)) ;
#142437=CARTESIAN_POINT('Ctrl Pts',(-13.5036989912694,14.4228365042112,
133.731636937861)) ;
#142438=CARTESIAN_POINT('Ctrl Pts',(-13.5775959146896,14.3452101955046,
133.980631757599)) ;
#142439=CARTESIAN_POINT('Ctrl Pts',(-13.641848848355,14.2014202619827,134.201474982571)) ;
#142440=CARTESIAN_POINT('Ctrl Pts',(-13.6909875456321,14.0021641250436,
134.378109627788)) ;
#142441=CARTESIAN_POINT('Ctrl Pts',(-13.7209546388244,13.7617530552763,
134.498718016342)) ;
#142442=CARTESIAN_POINT('Ctrl Pts',(-13.7288010165101,13.4956079562807,
134.554891268505)) ;
#142443=CARTESIAN_POINT('Ctrl Pts',(-13.7132439378269,13.2262845260177,
134.542442655534)) ;
#142444=CARTESIAN_POINT('Ctrl Pts',(-13.6746979333842,12.9698876491267,
134.462975697567)) ;
#142445=CARTESIAN_POINT('Ctrl Pts',(-13.6149469945644,12.7457363777613,
134.321622051184)) ;
#142446=CARTESIAN_POINT('Ctrl Pts',(-13.5380974991867,12.5708017324576,
134.130170046121)) ;
#142447=CARTESIAN_POINT('Ctrl Pts',(-13.4478576752863,12.4561497047602,
133.899872377774)) ;
#142448=CARTESIAN_POINT('Ctrl Pts',(-13.3517215673195,12.4116404870753,
133.651969615898)) ;
#142449=CARTESIAN_POINT('Ctrl Pts',(-13.2540076250656,12.4391729366694,
133.399748085855)) ;
#142450=CARTESIAN_POINT('Ctrl Pts',(-13.1622489475353,12.53717976609,133.164761472067)) ;
#142451=CARTESIAN_POINT('Ctrl Pts',(-13.0816903558919,12.6985743476714,
132.962543249434)) ;
#142452=CARTESIAN_POINT('Ctrl Pts',(-13.0175180261292,12.9117741339943,
132.808180146115)) ;
#142453=CARTESIAN_POINT('Ctrl Pts',(-12.9735046777524,13.1624013119324,
132.712811635355)) ;
#142454=CARTESIAN_POINT('Ctrl Pts',(-12.9523351151535,13.4305279124855,
132.684019974806)) ;
#142455=CARTESIAN_POINT('Ctrl Pts',(-12.9545548418119,13.6988963529668,
132.723654394249)) ;
#142456=CARTESIAN_POINT('Ctrl Pts',(-12.9793900887543,13.9472005440968,
132.829316178582)) ;
#142457=CARTESIAN_POINT('Ctrl Pts',(-13.0242752828077,14.1580510718868,
132.993551859839)) ;
#142458=CARTESIAN_POINT('Ctrl Pts',(-13.0854550375843,14.3165352463583,
133.205459831595)) ;
#142459=CARTESIAN_POINT('Ctrl Pts',(-13.157539949544,14.4105996736352,133.449148953889)) ;
#142460=CARTESIAN_POINT('Ctrl Pts',(-13.2347402649807,14.4340684642594,
133.707775721031)) ;
#142461=CARTESIAN_POINT('Ctrl Pts',(-13.3109617785798,14.3850543763753,
133.963600013658)) ;
#142462=CARTESIAN_POINT('Ctrl Pts',(-13.3798067326629,14.2669952008499,
134.197852855929)) ;
#142463=CARTESIAN_POINT('Ctrl Pts',(-13.4355433691654,14.0891153904615,
134.393714184201)) ;
#142464=CARTESIAN_POINT('Ctrl Pts',(-13.4738370489843,13.862922820575,134.538741233136)) ;
#142465=CARTESIAN_POINT('Ctrl Pts',(-13.4908658096809,13.6044942948714,
134.621718490304)) ;
#142466=CARTESIAN_POINT('Ctrl Pts',(-13.4848285534881,13.3352194719608,
134.637044133393)) ;
#142467=CARTESIAN_POINT('Ctrl Pts',(-13.4553946454675,13.0705828677346,
134.584234105595)) ;
#142468=CARTESIAN_POINT('Ctrl Pts',(-13.4040098364742,12.8316691546943,
134.467226066963)) ;
#142469=CARTESIAN_POINT('Ctrl Pts',(-13.33314013384,12.6342705619082,134.293479942512)) ;
#142470=CARTESIAN_POINT('Ctrl Pts',(-13.2483274035502,12.4949547618174,
134.078672195471)) ;
#142471=CARTESIAN_POINT('Ctrl Pts',(-13.1535924500394,12.4210676007864,
133.835114510728)) ;
#142472=CARTESIAN_POINT('Ctrl Pts',(-13.0559321401126,12.4192534953992,
133.582874005816)) ;
#142473=CARTESIAN_POINT('Ctrl Pts',(-12.9609580471452,12.4890551433301,
133.338571080929)) ;
#142474=CARTESIAN_POINT('Ctrl Pts',(-12.8747310689753,12.6269266116115,
133.119972901911)) ;
#142475=CARTESIAN_POINT('Ctrl Pts',(-12.8038546046608,12.8196496525906,
132.945820052933)) ;
#142476=CARTESIAN_POINT('Ctrl Pts',(-12.7510102619763,13.0580837190484,
132.824757826606)) ;
#142477=CARTESIAN_POINT('Ctrl Pts',(-12.7205262657728,13.3214663424209,
132.768812514467)) ;
#142478=CARTESIAN_POINT('Ctrl Pts',(-12.7133087559554,13.5912988654113,
132.780748069265)) ;
#142479=CARTESIAN_POINT('Ctrl Pts',(-12.729106667133,13.8497220068298,132.85998023594)) ;
#142480=CARTESIAN_POINT('Ctrl Pts',(-12.7664785971369,14.0789423187272,
133.002444149453)) ;
#142481=CARTESIAN_POINT('Ctrl Pts',(-12.8216206784442,14.259760152893,133.196642880183)) ;
#142482=CARTESIAN_POINT('Ctrl Pts',(-12.8896828571919,14.3805241864287,
133.428478547497)) ;
#142483=CARTESIAN_POINT('Ctrl Pts',(-12.9655732912177,14.4333051091104,
133.683295676437)) ;
#142484=CARTESIAN_POINT('Ctrl Pts',(-13.042967616016,14.4135763051709,133.942531611941)) ;
#142485=CARTESIAN_POINT('Ctrl Pts',(-13.1155158955077,14.3230159686918,
134.187589922523)) ;
#142486=CARTESIAN_POINT('Ctrl Pts',(-13.1774799234643,14.1669880508,134.401869852628)) ;
#142487=CARTESIAN_POINT('Ctrl Pts',(-13.2229930301975,13.960185490464,134.567683354239)) ;
#142488=CARTESIAN_POINT('Ctrl Pts',(-13.2491323955846,13.7121979598798,
134.677334901438)) ;
#142489=CARTESIAN_POINT('Ctrl Pts',(-13.2525598777593,13.445325428157,134.720373659982)) ;
#142490=CARTESIAN_POINT('Ctrl Pts',(-13.2325302461836,13.1756579311624,
134.695052960486)) ;
#142491=CARTESIAN_POINT('Ctrl Pts',(-13.1898673555691,12.9248371147139,
134.603460459577)) ;
#142492=CARTESIAN_POINT('Ctrl Pts',(-13.1266179073973,12.7087904234027,
134.451858747306)) ;
#142493=CARTESIAN_POINT('Ctrl Pts',(-13.0468208875135,12.5441839986788,
134.251863436356)) ;
#142494=CARTESIAN_POINT('Ctrl Pts',(-12.9549231889871,12.4422953627895,
134.016678643604)) ;
#142495=CARTESIAN_POINT('Ctrl Pts',(-12.8579637622449,12.4112745918663,
133.766440878839)) ;
#142496=CARTESIAN_POINT('Ctrl Pts',(-12.7611549009883,12.4523611263307,
133.516748584247)) ;
#142497=CARTESIAN_POINT('Ctrl Pts',(-12.6710156401631,12.5627156351226,
133.286505870711)) ;
#142498=CARTESIAN_POINT('Ctrl Pts',(-12.5927632872927,12.7362032520556,
133.091234472325)) ;
#142499=CARTESIAN_POINT('Ctrl Pts',(-12.5325786259911,12.9562237292826,
132.948303657431)) ;
#142500=CARTESIAN_POINT('Ctrl Pts',(-12.4925362362005,13.2127632851082,
132.864667442093)) ;
#142501=CARTESIAN_POINT('Ctrl Pts',(-12.4758811291573,13.4814740425718,
132.848961259101)) ;
#142502=CARTESIAN_POINT('Ctrl Pts',(-12.482415341822,13.7476021325284,132.901201359878)) ;
#142503=CARTESIAN_POINT('Ctrl Pts',(-12.5113783925367,13.9907503270219,
133.019010135492)) ;
#142504=CARTESIAN_POINT('Ctrl Pts',(-12.5595683982425,14.1921269255571,
133.192821462917)) ;
#142505=CARTESIAN_POINT('Ctrl Pts',(-12.6230623786545,14.3392030791961,
133.411416698859)) ;
#142506=CARTESIAN_POINT('Ctrl Pts',(-12.6970341102038,14.4207500388282,
133.660819657676)) ;
#142507=CARTESIAN_POINT('Ctrl Pts',(-12.774263901664,14.4302362494743,133.919425040572)) ;
#142508=CARTESIAN_POINT('Ctrl Pts',(-12.8494758392042,14.3680282355215,
134.172257690455)) ;
#142509=CARTESIAN_POINT('Ctrl Pts',(-12.9164641133178,14.2375542878188,
134.401162442814)) ;
#142510=CARTESIAN_POINT('Ctrl Pts',(-12.9692941715123,14.0487158820881,
134.588645421394)) ;
#142511=CARTESIAN_POINT('Ctrl Pts',(-13.0035360447327,13.8167882878437,
134.721606270082)) ;
#142512=CARTESIAN_POINT('Ctrl Pts',(-13.0164063281861,13.5548283790035,
134.792403087177)) ;
#142513=CARTESIAN_POINT('Ctrl Pts',(-13.0059798332764,13.2844749263172,
134.794999956039)) ;
#142514=CARTESIAN_POINT('Ctrl Pts',(-12.9721289476738,13.0226682928204,
134.729355118088)) ;
#142515=CARTESIAN_POINT('Ctrl Pts',(-12.917018681203,12.7913019037466,134.601363667181)) ;
#142516=CARTESIAN_POINT('Ctrl Pts',(-12.8433910805977,12.6040506886806,
134.41942655632)) ;
#142517=CARTESIAN_POINT('Ctrl Pts',(-12.7558724866451,12.4756113608574,
134.19692331088)) ;
#142518=CARTESIAN_POINT('Ctrl Pts',(-12.6602458572947,12.4152434806169,
133.950682918633)) ;
#142519=CARTESIAN_POINT('Ctrl Pts',(-12.5625488997366,12.4269403893897,
133.69837573229)) ;
#142520=CARTESIAN_POINT('Ctrl Pts',(-12.4688527527708,12.5099953392157,
133.457802697882)) ;
#142521=CARTESIAN_POINT('Ctrl Pts',(-12.3852338683453,12.6587329493789,
133.246696937566)) ;
#142522=CARTESIAN_POINT('Ctrl Pts',(-12.3171693653744,12.8618952615055,
133.080961556617)) ;
#142523=CARTESIAN_POINT('Ctrl Pts',(-12.2685510182443,13.105407033224,132.972065334935)) ;
#142524=CARTESIAN_POINT('Ctrl Pts',(-12.2422386883744,13.372198744835,132.928388345119)) ;
#142525=CARTESIAN_POINT('Ctrl Pts',(-12.2394516643981,13.6415134475053,
132.953298608277)) ;
#142526=CARTESIAN_POINT('Ctrl Pts',(-12.2594173692579,13.8954057522976,
133.044683143725)) ;
#142527=CARTESIAN_POINT('Ctrl Pts',(-12.3004891041707,14.1169004817223,
133.19795900627)) ;
#142528=CARTESIAN_POINT('Ctrl Pts',(-12.3582400665715,14.2868623314226,
133.399654280047)) ;
#142529=CARTESIAN_POINT('Ctrl Pts',(-12.4284737856363,14.3960130363954,
133.637987808134)) ;
#142530=CARTESIAN_POINT('Ctrl Pts',(-12.5052035539747,14.4351149221843,
133.895287975856)) ;
#142531=CARTESIAN_POINT('Ctrl Pts',(-12.581975793469,14.4019052033915,134.152623117381)) ;
#142532=CARTESIAN_POINT('Ctrl Pts',(-12.6530830929324,14.2983009205314,
134.393547253594)) ;
#142533=CARTESIAN_POINT('Ctrl Pts',(-12.7122527073782,14.1317969233753,
134.599560718346)) ;
#142534=CARTESIAN_POINT('Ctrl Pts',(-12.7545160578287,13.9153433735369,
134.756066454016)) ;
#142535=CARTESIAN_POINT('Ctrl Pts',(-12.7763808920198,13.6633971657659,
134.853037417297)) ;
#142536=CARTESIAN_POINT('Ctrl Pts',(-12.7755195845432,13.3943409356125,
134.883605222402)) ;
#142537=CARTESIAN_POINT('Ctrl Pts',(-12.7509706545826,13.125759479102,134.84518017233)) ;
#142538=CARTESIAN_POINT('Ctrl Pts',(-12.7042295073339,12.8806964502858,
134.741640153808)) ;
#142539=CARTESIAN_POINT('Ctrl Pts',(-12.6376258108186,12.6734733504626,
134.580189987171)) ;
#142540=CARTESIAN_POINT('Ctrl Pts',(-12.5549426142071,12.5195857964099,
134.371866859259)) ;
#142541=CARTESIAN_POINT('Ctrl Pts',(-12.46181515628,12.431093262312,134.13296415491)) ;
#142542=CARTESIAN_POINT('Ctrl Pts',(-12.3646330795371,12.4134132732782,
133.882020752927)) ;
#142543=CARTESIAN_POINT('Ctrl Pts',(-12.2682242070371,12.4681188865971,
133.63362475741)) ;
#142544=CARTESIAN_POINT('Ctrl Pts',(-12.1801451229978,12.5909169952097,
133.409362869367)) ;
#142545=CARTESIAN_POINT('Ctrl Pts',(-12.1051580880957,12.7734489728906,
133.223438258115)) ;
#142546=CARTESIAN_POINT('Ctrl Pts',(-12.0481373858043,13.0028155052197,
133.090024310372)) ;
#142547=CARTESIAN_POINT('Ctrl Pts',(-12.0125481809866,13.2626813874081,
133.01925718553)) ;
#142548=CARTESIAN_POINT('Ctrl Pts',(-12.0001983771847,13.5323092973528,
133.016160648346)) ;
#142549=CARTESIAN_POINT('Ctrl Pts',(-12.0111586092843,13.7963544405994,
133.081441752916)) ;
#142550=CARTESIAN_POINT('Ctrl Pts',(-12.0440275864981,14.0324258924939,
133.210582553837)) ;
#142551=CARTESIAN_POINT('Ctrl Pts',(-12.0953705891647,14.2243212394665,
133.393573736006)) ;
#142552=CARTESIAN_POINT('Ctrl Pts',(-12.1612093656614,14.3597397385498,
133.61903315744)) ;
#142553=CARTESIAN_POINT('Ctrl Pts',(-12.2362126914327,14.4280132276383,
133.871367486346)) ;
#142554=CARTESIAN_POINT('Ctrl Pts',(-12.3137470656388,14.4240026774031,
134.130972884586)) ;
#142555=CARTESIAN_POINT('Ctrl Pts',(-12.38788747333,14.3482148360276,134.380710229016)) ;
#142556=CARTESIAN_POINT('Ctrl Pts',(-12.452286472395,14.2066838492508,134.601870345064)) ;
#142557=CARTESIAN_POINT('Ctrl Pts',(-12.502100488198,14.0084843901798,134.78056124378)) ;
#142558=CARTESIAN_POINT('Ctrl Pts',(-12.5326854037367,13.7679162492584,
134.903106175098)) ;
#142559=CARTESIAN_POINT('Ctrl Pts',(-12.5410969798908,13.5034892563332,
134.960764420724)) ;
#142560=CARTESIAN_POINT('Ctrl Pts',(-12.5262131615707,13.2335993396584,
134.9503397068)) ;
#142561=CARTESIAN_POINT('Ctrl Pts',(-12.4882428296575,12.9764075734903,
134.872572785143)) ;
#142562=CARTESIAN_POINT('Ctrl Pts',(-12.4289044713352,12.7508791959946,
134.732473639261)) ;
#142563=CARTESIAN_POINT('Ctrl Pts',(-12.3527354057446,12.5752390295055,
134.542884388565)) ;
#142564=CARTESIAN_POINT('Ctrl Pts',(-12.2632773386131,12.4588914827239,
134.314708508696)) ;
#142565=CARTESIAN_POINT('Ctrl Pts',(-12.166700002866,12.4118138337187,134.065711798887)) ;
#142566=CARTESIAN_POINT('Ctrl Pts',(-12.0689529096772,12.4374481802068,
133.813382896759)) ;
#142567=CARTESIAN_POINT('Ctrl Pts',(-11.9769702221726,12.5333386761198,
133.577728338921)) ;
#142568=CARTESIAN_POINT('Ctrl Pts',(-11.8956955766465,12.6939673682458,
133.373567679243)) ;
#142569=CARTESIAN_POINT('Ctrl Pts',(-11.8313521769806,12.905003236762,133.218546885697)) ;
#142570=CARTESIAN_POINT('Ctrl Pts',(-11.7866067831211,13.1551454221065,
133.121092437729)) ;
#142571=CARTESIAN_POINT('Ctrl Pts',(-11.7721059446934,13.3338159430811,
133.100771605669)) ;
#142572=CARTESIAN_POINT('Ctrl Pts',(-11.7687201639657,13.423122164697,133.10190161956)) ;
#142573=CARTESIAN_POINT('Ctrl Pts',(-33.2064616283861,13.1551399285885,
127.920719415945)) ;
#142574=CARTESIAN_POINT('Ctrl Pts',(-33.2057227295762,13.1489709760559,
127.919291866388)) ;
#142575=CARTESIAN_POINT('Ctrl Pts',(-33.1936688649743,13.0505875198745,
127.895761948055)) ;
#142576=CARTESIAN_POINT('Ctrl Pts',(-33.160921840628,12.8648901900081,127.82307456361)) ;
#142577=CARTESIAN_POINT('Ctrl Pts',(-33.0921833510773,12.637899642759,127.655294615791)) ;
#142578=CARTESIAN_POINT('Ctrl Pts',(-33.0059288840404,12.4661938429578,
127.436429577543)) ;
#142579=CARTESIAN_POINT('Ctrl Pts',(-32.9070996303315,12.3629468652583,
127.180997914754)) ;
#142580=CARTESIAN_POINT('Ctrl Pts',(-32.8036494006583,12.3360866593215,
126.911722952076)) ;
#142581=CARTESIAN_POINT('Ctrl Pts',(-32.7003181752768,12.3868468010151,
126.643092453762)) ;
#142582=CARTESIAN_POINT('Ctrl Pts',(-32.6050897103573,12.5118616654237,
126.397998146605)) ;
#142583=CARTESIAN_POINT('Ctrl Pts',(-32.5235050196537,12.7022377085439,
126.192812360252)) ;
#142584=CARTESIAN_POINT('Ctrl Pts',(-32.4608859591013,12.9442212424904,
126.043009732538)) ;
#142585=CARTESIAN_POINT('Ctrl Pts',(-32.4209546422374,13.2203923683254,
125.959474453867)) ;
#142586=CARTESIAN_POINT('Ctrl Pts',(-32.405749339523,13.5109002567873,125.948146471616)) ;
#142587=CARTESIAN_POINT('Ctrl Pts',(-32.4158543282408,13.7967279051741,
126.010955365665)) ;
#142588=CARTESIAN_POINT('Ctrl Pts',(-32.44946277106,14.053163616969,126.142095751459)) ;
#142589=CARTESIAN_POINT('Ctrl Pts',(-32.5037010294867,14.2659162320927,
126.333668528097)) ;
#142590=CARTESIAN_POINT('Ctrl Pts',(-32.5739098208083,14.4182156131257,
126.571880763336)) ;
#142591=CARTESIAN_POINT('Ctrl Pts',(-32.6545587102474,14.4993926376335,
126.840688712835)) ;
#142592=CARTESIAN_POINT('Ctrl Pts',(-32.7386970776525,14.5030673759949,
127.119597798947)) ;
#142593=CARTESIAN_POINT('Ctrl Pts',(-32.8196605589341,14.4296657361334,
127.389182606704)) ;
#142594=CARTESIAN_POINT('Ctrl Pts',(-32.891145728035,14.2842404294125,127.631112234882)) ;
#142595=CARTESIAN_POINT('Ctrl Pts',(-32.9473175863939,14.0768884033213,
127.828355609425)) ;
#142596=CARTESIAN_POINT('Ctrl Pts',(-32.9832788532576,13.8219373708246,
127.966631980771)) ;
#142597=CARTESIAN_POINT('Ctrl Pts',(-32.9956260618082,13.5404395793698,
128.035680171597)) ;
#142598=CARTESIAN_POINT('Ctrl Pts',(-32.9830519454183,13.2491901831122,
128.032089979617)) ;
#142599=CARTESIAN_POINT('Ctrl Pts',(-32.9453417855078,12.969918720115,127.955137134767)) ;
#142600=CARTESIAN_POINT('Ctrl Pts',(-32.8850287367867,12.7245501655325,
127.811958868713)) ;
#142601=CARTESIAN_POINT('Ctrl Pts',(-32.8050106729142,12.5279693790049,
127.61140382253)) ;
#142602=CARTESIAN_POINT('Ctrl Pts',(-32.7109505070757,12.3961376577074,
127.369698243799)) ;
#142603=CARTESIAN_POINT('Ctrl Pts',(-32.608093202144,12.3376103607184,127.102453943038)) ;
#142604=CARTESIAN_POINT('Ctrl Pts',(-32.5042165214054,12.3569098768634,
126.832006082133)) ;
#142605=CARTESIAN_POINT('Ctrl Pts',(-32.4047263008834,12.4527690637887,
126.574582317231)) ;
#142606=CARTESIAN_POINT('Ctrl Pts',(-32.317039240674,12.6179594101214,126.35151544099)) ;
#142607=CARTESIAN_POINT('Ctrl Pts',(-32.2462108306946,12.8405880896203,
126.177706544888)) ;
#142608=CARTESIAN_POINT('Ctrl Pts',(-32.1965338574651,13.1065246819692,
126.065865852924)) ;
#142609=CARTESIAN_POINT('Ctrl Pts',(-32.1713639236927,13.3925179969382,
126.02529765245)) ;
#142610=CARTESIAN_POINT('Ctrl Pts',(-32.1711356447092,13.6819916806813,
126.057745187493)) ;
#142611=CARTESIAN_POINT('Ctrl Pts',(-32.1955942855959,13.953724245336,126.16241143608)) ;
#142612=CARTESIAN_POINT('Ctrl Pts',(-32.2420024149265,14.1863734270825,
126.331069844754)) ;
#142613=CARTESIAN_POINT('Ctrl Pts',(-32.3062614393706,14.3643807952629,
126.551845049774)) ;
#142614=CARTESIAN_POINT('Ctrl Pts',(-32.3832731449588,14.4754559836596,
126.809932800703)) ;
#142615=CARTESIAN_POINT('Ctrl Pts',(-32.46693246729,14.5110246745496,127.087529153579)) ;
#142616=CARTESIAN_POINT('Ctrl Pts',(-32.5498802722831,14.468706357864,127.362883365774)) ;
#142617=CARTESIAN_POINT('Ctrl Pts',(-32.6261767345985,14.3514018733064,
127.618935169129)) ;
#142618=CARTESIAN_POINT('Ctrl Pts',(-32.6892389357437,14.1671964526519,
127.836331456435)) ;
#142619=CARTESIAN_POINT('Ctrl Pts',(-32.7336924477987,13.9308607646815,
127.999208617667)) ;
#142620=CARTESIAN_POINT('Ctrl Pts',(-32.7560437331624,13.6570089391064,
128.09768299258)) ;
#142621=CARTESIAN_POINT('Ctrl Pts',(-32.7536233967398,13.3664658768335,
128.123772039366)) ;
#142622=CARTESIAN_POINT('Ctrl Pts',(-32.726020561585,13.0805680543038,128.076234678783)) ;
#142623=CARTESIAN_POINT('Ctrl Pts',(-32.6745478724091,12.8190538509803,
127.958967690888)) ;
#142624=CARTESIAN_POINT('Ctrl Pts',(-32.6016486027217,12.599933753752,127.77927449631)) ;
#142625=CARTESIAN_POINT('Ctrl Pts',(-32.5129827012049,12.4413956885076,
127.553221361994)) ;
#142626=CARTESIAN_POINT('Ctrl Pts',(-32.4129362071219,12.3520377966892,
127.294128922931)) ;
#142627=CARTESIAN_POINT('Ctrl Pts',(-32.3085709639735,12.3397344016033,
127.022370141575)) ;
#142628=CARTESIAN_POINT('Ctrl Pts',(-32.2065472158637,12.4049383820741,
126.757445808132)) ;
#142629=CARTESIAN_POINT('Ctrl Pts',(-32.1134309497632,12.5429636135127,
126.518532052174)) ;
#142630=CARTESIAN_POINT('Ctrl Pts',(-32.0350063547161,12.744355559365,126.322594585157)) ;
#142631=CARTESIAN_POINT('Ctrl Pts',(-31.9764168702957,12.99435234836,126.184578080748)) ;
#142632=CARTESIAN_POINT('Ctrl Pts',(-31.9410923640507,13.2741649900779,
126.114424971979)) ;
#142633=CARTESIAN_POINT('Ctrl Pts',(-31.9306079711779,13.5657204845938,
126.116961809238)) ;
#142634=CARTESIAN_POINT('Ctrl Pts',(-31.945333022402,13.8474317542271,126.1931967302)) ;
#142635=CARTESIAN_POINT('Ctrl Pts',(-31.9830832898237,14.0971651338937,
126.336484257145)) ;
#142636=CARTESIAN_POINT('Ctrl Pts',(-32.0409399787663,14.300212406185,126.538735226936)) ;
#142637=CARTESIAN_POINT('Ctrl Pts',(-32.1136595413229,14.439451037695,126.784306408733)) ;
#142638=CARTESIAN_POINT('Ctrl Pts',(-32.1949128964174,14.5058688377535,
127.05463526644)) ;
#142639=CARTESIAN_POINT('Ctrl Pts',(-32.2791660586006,14.4952594512815,
127.333947782969)) ;
#142640=CARTESIAN_POINT('Ctrl Pts',(-32.3592129092692,14.4071576201155,
127.601021809783)) ;
#142641=CARTESIAN_POINT('Ctrl Pts',(-32.4281419451805,14.2488069359853,
127.835486225876)) ;
#142642=CARTESIAN_POINT('Ctrl Pts',(-32.4805375156639,14.0323324822322,
128.021538873071)) ;
#142643=CARTESIAN_POINT('Ctrl Pts',(-32.512289642295,13.7715184536488,128.147415816655)) ;
#142644=CARTESIAN_POINT('Ctrl Pts',(-32.5201337915764,13.4849967549257,
128.20352710882)) ;
#142645=CARTESIAN_POINT('Ctrl Pts',(-32.5025273372398,13.1936953531143,
128.185335934368)) ;
#142646=CARTESIAN_POINT('Ctrl Pts',(-32.4607259546474,12.9217410379526,
128.096103762869)) ;
#142647=CARTESIAN_POINT('Ctrl Pts',(-32.3960971896468,12.6826992816898,
127.940549532299)) ;
#142648=CARTESIAN_POINT('Ctrl Pts',(-32.3129069984928,12.4976839055064,
127.730706441742)) ;
#142649=CARTESIAN_POINT('Ctrl Pts',(-32.2171411071609,12.37947113767,127.483906316843)) ;
#142650=CARTESIAN_POINT('Ctrl Pts',(-32.1132911001469,12.3351744205894,
127.21381155579)) ;
#142651=CARTESIAN_POINT('Ctrl Pts',(-32.0094764720966,12.3695012767601,
126.943667978939)) ;
#142652=CARTESIAN_POINT('Ctrl Pts',(-31.9122693293976,12.4786183713965,
126.69271538078)) ;
#142653=CARTESIAN_POINT('Ctrl Pts',(-31.827183667738,12.6556201650726,126.477292320838)) ;
#142654=CARTESIAN_POINT('Ctrl Pts',(-31.7599124151507,12.8885376927875,
126.314004677371)) ;
#142655=CARTESIAN_POINT('Ctrl Pts',(-31.714947288412,13.1578672301346,126.215639088923)) ;
#142656=CARTESIAN_POINT('Ctrl Pts',(-31.6941824964107,13.4488181207259,
126.188284587737)) ;
#142657=CARTESIAN_POINT('Ctrl Pts',(-31.698897103108,13.7357351510131,126.235108130151)) ;
#142658=CARTESIAN_POINT('Ctrl Pts',(-31.7274809073415,14.0000244491373,
126.351602120279)) ;
#142659=CARTESIAN_POINT('Ctrl Pts',(-31.7778273453152,14.2248064092014,
126.531934807809)) ;
#142660=CARTESIAN_POINT('Ctrl Pts',(-31.844851717,14.3907221874245,126.760746549466)) ;
#142661=CARTESIAN_POINT('Ctrl Pts',(-31.9236967438235,14.4880878252355,
127.0242463843)) ;
#142662=CARTESIAN_POINT('Ctrl Pts',(-32.0074797583405,14.5090844466389,
127.302065690259)) ;
#142663=CARTESIAN_POINT('Ctrl Pts',(-32.0902772487515,14.4517330875411,
127.577253483703)) ;
#142664=CARTESIAN_POINT('Ctrl Pts',(-32.1640651859993,14.3213872706393,
127.825792981418)) ;
#142665=CARTESIAN_POINT('Ctrl Pts',(-32.2240068107159,14.1266125068475,
128.034020404948)) ;
#142666=CARTESIAN_POINT('Ctrl Pts',(-32.2647640498464,13.8801112237431,
128.186345332148)) ;
#142667=CARTESIAN_POINT('Ctrl Pts',(-32.2823576448507,13.6025838419119,
128.270778674212)) ;
#142668=CARTESIAN_POINT('Ctrl Pts',(-32.2752642468574,13.3122087049322,
128.283106518981)) ;
#142669=CARTESIAN_POINT('Ctrl Pts',(-32.2429269674404,13.0284663697123,
128.221843758155)) ;
#142670=CARTESIAN_POINT('Ctrl Pts',(-32.1871815503845,12.7739763347418,
128.092081411688)) ;
#142671=CARTESIAN_POINT('Ctrl Pts',(-32.111096935218,12.5655227594086,127.902962986094)) ;
#142672=CARTESIAN_POINT('Ctrl Pts',(-32.0195990424995,12.4188417655465,
127.668765531469)) ;
#142673=CARTESIAN_POINT('Ctrl Pts',(-31.9184991684207,12.343819791052,127.406496289624)) ;
#142674=CARTESIAN_POINT('Ctrl Pts',(-31.8137079351686,12.3461750188478,
127.133605889349)) ;
#142675=CARTESIAN_POINT('Ctrl Pts',(-31.7130252080803,12.4256200301873,
126.872547622651)) ;
#142676=CARTESIAN_POINT('Ctrl Pts',(-31.6221469061099,12.5766361181176,
126.640220251546)) ;
#142677=CARTESIAN_POINT('Ctrl Pts',(-31.547220653387,12.7882866055861,126.454465707021)) ;
#142678=CARTESIAN_POINT('Ctrl Pts',(-31.492809784499,13.0452021106171,126.328621831613)) ;
#142679=CARTESIAN_POINT('Ctrl Pts',(-31.4620208452283,13.3293878961544,
126.271809382364)) ;
#142680=CARTESIAN_POINT('Ctrl Pts',(-31.4563957226866,13.6204037391964,
126.288518759348)) ;
#142681=CARTESIAN_POINT('Ctrl Pts',(-31.4756176952845,13.8971497414612,
126.3778003854)) ;
#142682=CARTESIAN_POINT('Ctrl Pts',(-31.5174981860061,14.1397539982186,
126.53324136256)) ;
#142683=CARTESIAN_POINT('Ctrl Pts',(-31.5784731662082,14.3313465280224,
126.744521176888)) ;
#142684=CARTESIAN_POINT('Ctrl Pts',(-31.6531070542541,14.4574458886048,
126.995592910948)) ;
#142685=CARTESIAN_POINT('Ctrl Pts',(-31.7357182581869,14.509972396165,127.27004619928)) ;
#142686=CARTESIAN_POINT('Ctrl Pts',(-31.8197265109475,14.4843439557881,
127.548664482844)) ;
#142687=CARTESIAN_POINT('Ctrl Pts',(-31.8978809400863,14.3827749210334,
127.810067848139)) ;
#142688=CARTESIAN_POINT('Ctrl Pts',(-31.9642304853554,14.2124739765949,
128.037017650735)) ;
#142689=CARTESIAN_POINT('Ctrl Pts',(-32.0131976388995,13.9855789270548,
128.213188860414)) ;
#142690=CARTESIAN_POINT('Ctrl Pts',(-32.0405543494933,13.7185805831256,
128.326209499296)) ;
#142691=CARTESIAN_POINT('Ctrl Pts',(-32.0436331723574,13.4303185672317,
128.368322928117)) ;
#142692=CARTESIAN_POINT('Ctrl Pts',(-32.0215333257744,13.1417758390937,
128.33685233434)) ;
#142693=CARTESIAN_POINT('Ctrl Pts',(-31.9748976328392,12.8725286087569,
128.233815253822)) ;
#142694=CARTESIAN_POINT('Ctrl Pts',(-31.9066058992129,12.6435096250976,
128.067418368168)) ;
#142695=CARTESIAN_POINT('Ctrl Pts',(-31.8206856918917,12.470154617103,127.849547648784)) ;
#142696=CARTESIAN_POINT('Ctrl Pts',(-31.7226433988074,12.3650501816311,
127.596245250201)) ;
#142697=CARTESIAN_POINT('Ctrl Pts',(-31.6184519258737,12.3357586673989,
127.325066885764)) ;
#142698=CARTESIAN_POINT('Ctrl Pts',(-31.5155220134888,12.3843195645159,
127.057439493129)) ;
#142699=CARTESIAN_POINT('Ctrl Pts',(-31.4198179572413,12.5073667033233,
126.811011568101)) ;
#142700=CARTESIAN_POINT('Ctrl Pts',(-31.3378940321144,12.695820098274,126.604784360148)) ;
#142701=CARTESIAN_POINT('Ctrl Pts',(-31.2746568300074,12.9363650189031,
126.453164101291)) ;
#142702=CARTESIAN_POINT('Ctrl Pts',(-31.2339861564669,13.2120463476192,
126.367497677483)) ;
#142703=CARTESIAN_POINT('Ctrl Pts',(-31.218054736522,13.5022482408363,126.354027956631)) ;
#142704=CARTESIAN_POINT('Ctrl Pts',(-31.2274123863003,13.788401757224,126.414636560072)) ;
#142705=CARTESIAN_POINT('Ctrl Pts',(-31.2603056788409,14.0459452112238,
126.543679970572)) ;
#142706=CARTESIAN_POINT('Ctrl Pts',(-31.3142676028335,14.261068186074,126.734589300308)) ;
#142707=CARTESIAN_POINT('Ctrl Pts',(-31.3838448851807,14.4145624952327,
126.970825527176)) ;
#142708=CARTESIAN_POINT('Ctrl Pts',(-31.464268747959,14.4980852442795,127.238979955351)) ;
#142709=CARTESIAN_POINT('Ctrl Pts',(-31.5484155641688,14.5041312509629,
127.517917624269)) ;
#142710=CARTESIAN_POINT('Ctrl Pts',(-31.6297274762448,14.4326961548768,
127.788594379386)) ;
#142711=CARTESIAN_POINT('Ctrl Pts',(-31.7015057073872,14.2894246996344,
128.031337346009)) ;
#142712=CARTESIAN_POINT('Ctrl Pts',(-31.7583243957012,14.0826506129639,
128.230601393984)) ;
#142713=CARTESIAN_POINT('Ctrl Pts',(-31.7946301927493,13.8312289814619,
128.369572219819)) ;
#142714=CARTESIAN_POINT('Ctrl Pts',(-31.8078849388079,13.5479803719868,
128.441553443391)) ;
#142715=CARTESIAN_POINT('Ctrl Pts',(-31.7959085692955,13.257297898438,128.439638332041)) ;
#142716=CARTESIAN_POINT('Ctrl Pts',(-31.7591260014045,12.9781390141801,
128.365290983036)) ;
#142717=CARTESIAN_POINT('Ctrl Pts',(-31.6989001455544,12.7298469956755,
128.222623208126)) ;
#142718=CARTESIAN_POINT('Ctrl Pts',(-31.619935033866,12.5331717504731,128.024890524041)) ;
#142719=CARTESIAN_POINT('Ctrl Pts',(-31.5257553511796,12.3987049958051,
127.783005973355)) ;
#142720=CARTESIAN_POINT('Ctrl Pts',(-31.4236240780026,12.3381977038027,
127.517686726716)) ;
#142721=CARTESIAN_POINT('Ctrl Pts',(-31.3187777933959,12.3556286047268,
127.244711651246)) ;
#142722=CARTESIAN_POINT('Ctrl Pts',(-31.2201199323636,12.4484986932729,
126.989359567954)) ;
#142723=CARTESIAN_POINT('Ctrl Pts',(-31.1314620599124,12.6124652381156,
126.763652129256)) ;
#142724=CARTESIAN_POINT('Ctrl Pts',(-31.0603390629678,12.833019455732,126.588870336055)) ;
#142725=CARTESIAN_POINT('Ctrl Pts',(-31.0098757034308,13.0981217097557,
126.474765888058)) ;
#142726=CARTESIAN_POINT('Ctrl Pts',(-30.9839541223414,13.3840424084956,
126.432032804447)) ;
#142727=CARTESIAN_POINT('Ctrl Pts',(-30.9830184122512,13.673804350161,126.462424161424)) ;
#142728=CARTESIAN_POINT('Ctrl Pts',(-31.0067064338544,13.9458856599705,
126.564772906119)) ;
#142729=CARTESIAN_POINT('Ctrl Pts',(-31.0526563993131,14.1805609779054,
126.732191904978)) ;
#142730=CARTESIAN_POINT('Ctrl Pts',(-31.1163979299656,14.3602096691543,
126.951417205331)) ;
#142731=CARTESIAN_POINT('Ctrl Pts',(-31.1936186238981,14.47371465445,127.210313970921)) ;
#142732=CARTESIAN_POINT('Ctrl Pts',(-31.276626453563,14.5109817362897,127.485775916908)) ;
#142733=CARTESIAN_POINT('Ctrl Pts',(-31.3597859403266,14.4710234549687,
127.761794153221)) ;
#142734=CARTESIAN_POINT('Ctrl Pts',(-31.4362807735142,14.3558611737084,
128.018385473721)) ;
#142735=CARTESIAN_POINT('Ctrl Pts',(-31.4998116237642,14.173605953239,128.237140036393)) ;
#142736=CARTESIAN_POINT('Ctrl Pts',(-31.5449540416273,13.9381264570577,
128.402093551021)) ;
#142737=CARTESIAN_POINT('Ctrl Pts',(-31.5679255836761,13.6651920565378,
128.502359753407)) ;
#142738=CARTESIAN_POINT('Ctrl Pts',(-31.5663255356321,13.3755914390975,
128.530759248685)) ;
#142739=CARTESIAN_POINT('Ctrl Pts',(-31.5392380980967,13.0874856739398,
128.484939106277)) ;
#142740=CARTESIAN_POINT('Ctrl Pts',(-31.4885879922083,12.8264336867777,
128.369908021904)) ;
#142741=CARTESIAN_POINT('Ctrl Pts',(-31.4164911780433,12.6060973636301,
128.192486850099)) ;
#142742=CARTESIAN_POINT('Ctrl Pts',(-31.3280152859864,12.4450312815742,
127.967079585755)) ;
#142743=CARTESIAN_POINT('Ctrl Pts',(-31.2279193062099,12.3534665915943,
127.7079284228)) ;
#142744=CARTESIAN_POINT('Ctrl Pts',(-31.1238917413468,12.3390030026154,
127.437059120732)) ;
#142745=CARTESIAN_POINT('Ctrl Pts',(-31.0214731199007,12.4020393022516,
127.171054081183)) ;
#142746=CARTESIAN_POINT('Ctrl Pts',(-30.9279202793389,12.5385712255671,
126.930915337845)) ;
#142747=CARTESIAN_POINT('Ctrl Pts',(-30.8494032021172,12.7373374755761,
126.734540013757)) ;
#142748=CARTESIAN_POINT('Ctrl Pts',(-30.7900716797921,12.9861208763485,
126.594372908603)) ;
#142749=CARTESIAN_POINT('Ctrl Pts',(-30.7539485891286,13.2660912868939,
126.521974733773)) ;
#142750=CARTESIAN_POINT('Ctrl Pts',(-30.7428010893841,13.5573229974737,
126.522542007644)) ;
#142751=CARTESIAN_POINT('Ctrl Pts',(-30.7566839096316,13.8386954173301,
126.596197928137)) ;
#142752=CARTESIAN_POINT('Ctrl Pts',(-30.7939147647464,14.0906009261112,
126.738098027588)) ;
#142753=CARTESIAN_POINT('Ctrl Pts',(-30.8510431537068,14.2945041038628,
126.938095608529)) ;
#142754=CARTESIAN_POINT('Ctrl Pts',(-30.9233443651782,14.4361574942565,
127.18244958177)) ;
#142755=CARTESIAN_POINT('Ctrl Pts',(-31.0048336013044,14.5051117773277,
127.453630062579)) ;
#142756=CARTESIAN_POINT('Ctrl Pts',(-31.0888759648342,14.4965825882903,
127.732236491623)) ;
#142757=CARTESIAN_POINT('Ctrl Pts',(-31.168865676846,14.4113394048867,127.999016499472)) ;
#142758=CARTESIAN_POINT('Ctrl Pts',(-31.2384933243905,14.2546478359796,
128.235636040619)) ;
#142759=CARTESIAN_POINT('Ctrl Pts',(-31.2915451356608,14.0391437504434,
128.423680114953)) ;
#142760=CARTESIAN_POINT('Ctrl Pts',(-31.3239067519199,13.7793415261531,
128.551331386748)) ;
#142761=CARTESIAN_POINT('Ctrl Pts',(-31.3324639869936,13.4941094654563,
128.609429945624)) ;
#142762=CARTESIAN_POINT('Ctrl Pts',(-31.3156967226184,13.2026873964626,
128.593682895648)) ;
#142763=CARTESIAN_POINT('Ctrl Pts',(-31.274441049515,12.9288332689777,128.506175701619)) ;
#142764=CARTESIAN_POINT('Ctrl Pts',(-31.2102613525706,12.6885083227908,
128.351964103388)) ;
#142765=CARTESIAN_POINT('Ctrl Pts',(-31.1280360942476,12.5026390523848,
128.144753064434)) ;
#142766=CARTESIAN_POINT('Ctrl Pts',(-31.0320401303252,12.3816810142256,
127.897469250246)) ;
#142767=CARTESIAN_POINT('Ctrl Pts',(-30.9288964149733,12.3354826601101,
127.629243583753)) ;
#142768=CARTESIAN_POINT('Ctrl Pts',(-30.8247552318205,12.3671988695935,
127.358221331888)) ;
#142769=CARTESIAN_POINT('Ctrl Pts',(-30.7268557425413,12.4748749590594,
127.105391022476)) ;
#142770=CARTESIAN_POINT('Ctrl Pts',(-30.6416225436775,12.6498955161038,
126.889454161025)) ;
#142771=CARTESIAN_POINT('Ctrl Pts',(-30.5739773175829,12.8801431271714,
126.724918684966)) ;
#142772=CARTESIAN_POINT('Ctrl Pts',(-30.5280533743189,13.1504415256103,
126.623977240751)) ;
#142773=CARTESIAN_POINT('Ctrl Pts',(-30.5067059098186,13.4387392039499,
126.594642314902)) ;
#142774=CARTESIAN_POINT('Ctrl Pts',(-30.5105905683589,13.7280473627643,
126.639272529026)) ;
#142775=CARTESIAN_POINT('Ctrl Pts',(-30.5386531607722,13.9932362270437,
126.754260621585)) ;
#142776=CARTESIAN_POINT('Ctrl Pts',(-30.5881891176015,14.2186784013421,
126.932092352736)) ;
#142777=CARTESIAN_POINT('Ctrl Pts',(-30.6551326283065,14.3872014595801,
127.160834082923)) ;
#142778=CARTESIAN_POINT('Ctrl Pts',(-30.7333872632998,14.4862165376707,
127.422454831296)) ;
#142779=CARTESIAN_POINT('Ctrl Pts',(-30.8174140558742,14.5095010534955,
127.701112767902)) ;
#142780=CARTESIAN_POINT('Ctrl Pts',(-30.8998260095477,14.4548476370639,
127.974954865684)) ;
#142781=CARTESIAN_POINT('Ctrl Pts',(-30.9744919161141,14.3259645840264,
128.226282736462)) ;
#142782=CARTESIAN_POINT('Ctrl Pts',(-31.0349033731148,14.132023950122,128.435947494583)) ;
#142783=CARTESIAN_POINT('Ctrl Pts',(-31.0759430220492,13.8890686102105,
128.588794252599)) ;
#142784=CARTESIAN_POINT('Ctrl Pts',(-31.0944376075796,13.6109286818878,
128.676030610899)) ;
#142785=CARTESIAN_POINT('Ctrl Pts',(-31.0880487774346,13.3205779167508,
128.690415573638)) ;
#142786=CARTESIAN_POINT('Ctrl Pts',(-31.0562963474654,13.0356408417454,
128.630948247247)) ;
#142787=CARTESIAN_POINT('Ctrl Pts',(-31.0013892817443,12.7811566928917,
128.503497528563)) ;
#142788=CARTESIAN_POINT('Ctrl Pts',(-30.9258694959649,12.5709849974497,
128.316035091874)) ;
#142789=CARTESIAN_POINT('Ctrl Pts',(-30.8347412757522,12.4221765780121,
128.082924321767)) ;
#142790=CARTESIAN_POINT('Ctrl Pts',(-30.7333975989525,12.3447406523641,
127.820082767003)) ;
#142791=CARTESIAN_POINT('Ctrl Pts',(-30.6287619755561,12.3451621896592,
127.547596475717)) ;
#142792=CARTESIAN_POINT('Ctrl Pts',(-30.5281543228765,12.4221618578868,
127.286667507964)) ;
#142793=CARTESIAN_POINT('Ctrl Pts',(-30.4368045692654,12.5713294888185,
127.052995432794)) ;
#142794=CARTESIAN_POINT('Ctrl Pts',(-30.361412617843,12.781135912573,126.86584125208)) ;
#142795=CARTESIAN_POINT('Ctrl Pts',(-30.3062767402564,13.0373855963871,
126.73793450979)) ;
#142796=CARTESIAN_POINT('Ctrl Pts',(-30.2748125276942,13.3202249658799,
126.679050724831)) ;
#142797=CARTESIAN_POINT('Ctrl Pts',(-30.2684246244409,13.6126651184226,
126.693687161756)) ;
#142798=CARTESIAN_POINT('Ctrl Pts',(-30.2869050355454,13.8891096825995,
126.780680178363)) ;
#142799=CARTESIAN_POINT('Ctrl Pts',(-30.328241457162,14.1334577296797,126.934603321344)) ;
#142800=CARTESIAN_POINT('Ctrl Pts',(-30.3884948782566,14.3262011562841,
127.143657768574)) ;
#142801=CARTESIAN_POINT('Ctrl Pts',(-30.4632736474801,14.4552702569289,
127.395366894377)) ;
#142802=CARTESIAN_POINT('Ctrl Pts',(-30.5458417500547,14.5094659908496,
127.669716069013)) ;
#142803=CARTESIAN_POINT('Ctrl Pts',(-30.6293554000449,14.4862792648155,
127.946670555011)) ;
#142804=CARTESIAN_POINT('Ctrl Pts',(-30.7080061524191,14.3867194046613,
128.209621341823)) ;
#142805=CARTESIAN_POINT('Ctrl Pts',(-30.7747309805075,14.2183273088974,
128.437642777903)) ;
#142806=CARTESIAN_POINT('Ctrl Pts',(-30.8243935899846,13.992244078071,128.615933560403)) ;
#142807=CARTESIAN_POINT('Ctrl Pts',(-30.8523086752982,13.7260908725509,
128.730577525946)) ;
#142808=CARTESIAN_POINT('Ctrl Pts',(-30.8561418503764,13.4392990631296,
128.774762803047)) ;
#142809=CARTESIAN_POINT('Ctrl Pts',(-30.8346412184545,13.1491383959326,
128.745202054093)) ;
#142810=CARTESIAN_POINT('Ctrl Pts',(-30.7888519514244,12.8801381500525,
128.644497302745)) ;
#142811=CARTESIAN_POINT('Ctrl Pts',(-30.7208398901881,12.64883120769,128.479059560541)) ;
#142812=CARTESIAN_POINT('Ctrl Pts',(-30.6357753911745,12.4746173054018,
128.26351619677)) ;
#142813=CARTESIAN_POINT('Ctrl Pts',(-30.5377496366726,12.3669410554066,
128.010358301652)) ;
#142814=CARTESIAN_POINT('Ctrl Pts',(-30.4336611805425,12.3355244461353,
127.739466951913)) ;
#142815=CARTESIAN_POINT('Ctrl Pts',(-30.3306644329952,12.3818824720289,
127.4716321127)) ;
#142816=CARTESIAN_POINT('Ctrl Pts',(-30.234825873423,12.5024424639559,127.224739910609)) ;
#142817=CARTESIAN_POINT('Ctrl Pts',(-30.1520250480759,12.6900860834509,
127.0161141599)) ;
#142818=CARTESIAN_POINT('Ctrl Pts',(-30.0883858330113,12.9290694340201,
126.863256044418)) ;
#142819=CARTESIAN_POINT('Ctrl Pts',(-30.0470668431947,13.2033803581446,
126.775625804674)) ;
#142820=CARTESIAN_POINT('Ctrl Pts',(-30.0303844725595,13.4938855393019,
126.760016339724)) ;
#142821=CARTESIAN_POINT('Ctrl Pts',(-30.0389475792244,13.7798209622441,
126.818217155643)) ;
#142822=CARTESIAN_POINT('Ctrl Pts',(-30.071382390156,14.0398148496058,126.946107608102)) ;
#142823=CARTESIAN_POINT('Ctrl Pts',(-30.1246984855742,14.2555982023478,
127.135022862139)) ;
#142824=CARTESIAN_POINT('Ctrl Pts',(-30.1938899332028,14.4112165805385,
127.370147971488)) ;
#142825=CARTESIAN_POINT('Ctrl Pts',(-30.2744141343331,14.4969136071728,
127.638712469549)) ;
#142826=CARTESIAN_POINT('Ctrl Pts',(-30.3581226245091,14.5049696606859,
127.916204012444)) ;
#142827=CARTESIAN_POINT('Ctrl Pts',(-30.439571695334,14.4360248987559,128.187259104422)) ;
#142828=CARTESIAN_POINT('Ctrl Pts',(-30.5117927626852,14.2945753095186,
128.431334289227)) ;
#142829=CARTESIAN_POINT('Ctrl Pts',(-30.5691023350333,14.0897547152948,
128.631991536531)) ;
#142830=CARTESIAN_POINT('Ctrl Pts',(-30.6061131460944,13.8386999371902,
128.773119766257)) ;
#142831=CARTESIAN_POINT('Ctrl Pts',(-30.6200817649539,13.557404245294,128.847024010029)) ;
#142832=CARTESIAN_POINT('Ctrl Pts',(-30.6087458782112,13.2644127915957,
128.847242565271)) ;
#142833=CARTESIAN_POINT('Ctrl Pts',(-30.5727419671278,12.9862193835362,
128.774990539839)) ;
#142834=CARTESIAN_POINT('Ctrl Pts',(-30.5133912275406,12.7371110279746,
128.634805043641)) ;
#142835=CARTESIAN_POINT('Ctrl Pts',(-30.4346856662007,12.5380202146654,
128.437941656666)) ;
#142836=CARTESIAN_POINT('Ctrl Pts',(-30.3408137582206,12.4015272035531,
128.196962918917)) ;
#142837=CARTESIAN_POINT('Ctrl Pts',(-30.2387580740374,12.3389469979449,
127.931890728957)) ;
#142838=CARTESIAN_POINT('Ctrl Pts',(-30.1344188320465,12.3537865285607,
127.66021882814)) ;
#142839=CARTESIAN_POINT('Ctrl Pts',(-30.0348799647077,12.4449099781865,
127.402504219006)) ;
#142840=CARTESIAN_POINT('Ctrl Pts',(-29.9458853225937,12.6072328334928,
127.175803032903)) ;
#142841=CARTESIAN_POINT('Ctrl Pts',(-29.8743601595728,12.8259752277409,
126.999791081331)) ;
#142842=CARTESIAN_POINT('Ctrl Pts',(-29.8232788134169,13.0894865992637,
126.883812376946)) ;
#142843=CARTESIAN_POINT('Ctrl Pts',(-29.7965060135308,13.3763086885043,
126.838741513895)) ;
#142844=CARTESIAN_POINT('Ctrl Pts',(-29.7949634120603,13.6661024734113,
126.867343704578)) ;
#142845=CARTESIAN_POINT('Ctrl Pts',(-29.8178316934814,13.9378774690874,
126.967158551912)) ;
#142846=CARTESIAN_POINT('Ctrl Pts',(-29.8633214379128,14.1747933111433,
127.133350479076)) ;
#142847=CARTESIAN_POINT('Ctrl Pts',(-29.9265395417689,14.3556679919274,
127.350985685476)) ;
#142848=CARTESIAN_POINT('Ctrl Pts',(-30.0030508632442,14.4711053285872,
127.6076521516)) ;
#142849=CARTESIAN_POINT('Ctrl Pts',(-30.0865564445511,14.5111709794694,
127.884806852964)) ;
#142850=CARTESIAN_POINT('Ctrl Pts',(-30.1699004127553,14.4729025358904,
128.161406819813)) ;
#142851=CARTESIAN_POINT('Ctrl Pts',(-30.2462983206917,14.3605014207988,
128.417542568319)) ;
#142852=CARTESIAN_POINT('Ctrl Pts',(-30.3106448741099,14.1789799465746,
128.63887062547)) ;
#142853=CARTESIAN_POINT('Ctrl Pts',(-30.3561566067274,13.9453130634453,
128.804803369269)) ;
#142854=CARTESIAN_POINT('Ctrl Pts',(-30.3798024914641,13.6736132719233,
128.906994396133)) ;
#142855=CARTESIAN_POINT('Ctrl Pts',(-30.3789584446791,13.3843416076431,
128.937588844635)) ;
#142856=CARTESIAN_POINT('Ctrl Pts',(-30.3526013931557,13.0956424209517,
128.893923674973)) ;
#142857=CARTESIAN_POINT('Ctrl Pts',(-30.3026011006858,12.8335786861196,
128.780796985994)) ;
#142858=CARTESIAN_POINT('Ctrl Pts',(-30.231053128041,12.611652190356,128.604987703306)) ;
#142859=CARTESIAN_POINT('Ctrl Pts',(-30.1428236509105,12.4486057551385,
128.380351815953)) ;
#142860=CARTESIAN_POINT('Ctrl Pts',(-30.0433319916567,12.3551665725231,
128.12284248329)) ;
#142861=CARTESIAN_POINT('Ctrl Pts',(-29.939015371523,12.338311146402,127.851236266649)) ;
#142862=CARTESIAN_POINT('Ctrl Pts',(-29.8366056665798,12.39913191908,127.585202385857)) ;
#142863=CARTESIAN_POINT('Ctrl Pts',(-29.7427166487443,12.5336134533254,
127.344083270442)) ;
#142864=CARTESIAN_POINT('Ctrl Pts',(-29.663675565517,12.7304748931974,127.146157836652)) ;
#142865=CARTESIAN_POINT('Ctrl Pts',(-29.6033823042093,12.9801495362985,
127.003435636053)) ;
#142866=CARTESIAN_POINT('Ctrl Pts',(-29.5669638511879,13.2569932871313,
126.929866029654)) ;
#142867=CARTESIAN_POINT('Ctrl Pts',(-29.554951047838,13.5493203158773,126.928041183197)) ;
#142868=CARTESIAN_POINT('Ctrl Pts',(-29.5681806364269,13.8310611217576,
126.999765211193)) ;
#142869=CARTESIAN_POINT('Ctrl Pts',(-29.6048343695299,14.0843639820839,
127.14002065473)) ;
#142870=CARTESIAN_POINT('Ctrl Pts',(-29.6614640820528,14.2896245798539,
127.338543409109)) ;
#142871=CARTESIAN_POINT('Ctrl Pts',(-29.7332906010218,14.433006390985,127.581457172281)) ;
#142872=CARTESIAN_POINT('Ctrl Pts',(-29.8146433905983,14.5042107644556,
127.852256910045)) ;
#142873=CARTESIAN_POINT('Ctrl Pts',(-29.8987371113395,14.4979449677576,
128.131024343594)) ;
#142874=CARTESIAN_POINT('Ctrl Pts',(-29.9791604149128,14.4144600975177,
128.399168008958)) ;
#142875=CARTESIAN_POINT('Ctrl Pts',(-30.0490448554192,14.259520873967,128.636505696184)) ;
#142876=CARTESIAN_POINT('Ctrl Pts',(-30.1024733512287,14.0462147796788,
128.825547199947)) ;
#142877=CARTESIAN_POINT('Ctrl Pts',(-30.1355535398746,13.7868051984224,
128.955377427376)) ;
#142878=CARTESIAN_POINT('Ctrl Pts',(-30.1447564168258,13.5027355977882,
129.015276777012)) ;
#142879=CARTESIAN_POINT('Ctrl Pts',(-30.1288158056883,13.2114163358095,
129.001914025961)) ;
#142880=CARTESIAN_POINT('Ctrl Pts',(-30.0880935176902,12.9359342039492,
128.916075180905)) ;
#142881=CARTESIAN_POINT('Ctrl Pts',(-30.0247104416128,12.6951561372944,
128.764080699704)) ;
#142882=CARTESIAN_POINT('Ctrl Pts',(-29.942963545196,12.5073060889563,128.558283375642)) ;
#142883=CARTESIAN_POINT('Ctrl Pts',(-29.8471539839523,12.3841592537523,
128.311585634468)) ;
#142884=CARTESIAN_POINT('Ctrl Pts',(-29.744101814774,12.3356200242118,128.043633158241)) ;
#142885=CARTESIAN_POINT('Ctrl Pts',(-29.6395080858797,12.3655842342963,
127.771418882123)) ;
#142886=CARTESIAN_POINT('Ctrl Pts',(-29.5421036027909,12.4702048662911,
127.519765293934)) ;
#142887=CARTESIAN_POINT('Ctrl Pts',(-29.4557101506611,12.6448837990351,
127.300726057939)) ;
#142888=CARTESIAN_POINT('Ctrl Pts',(-29.3879505080204,12.8725084203653,
127.135649765193)) ;
#142889=CARTESIAN_POINT('Ctrl Pts',(-29.3410790256385,13.1434988264021,
127.03213773474)) ;
#142890=CARTESIAN_POINT('Ctrl Pts',(-29.3192584705184,13.4301737730148,
127.001259274478)) ;
#142891=CARTESIAN_POINT('Ctrl Pts',(-29.3222385561352,13.718779591721,127.043120453796)) ;
#142892=CARTESIAN_POINT('Ctrl Pts',(-29.3498696871251,13.9870154535706,
127.157116456129)) ;
#142893=CARTESIAN_POINT('Ctrl Pts',(-29.3986379964539,14.2124398495338,
127.3325193873)) ;
#142894=CARTESIAN_POINT('Ctrl Pts',(-29.4650553209786,14.3830654639858,
127.559715415461)) ;
#142895=CARTESIAN_POINT('Ctrl Pts',(-29.5434438005476,14.4846609671348,
127.821883558811)) ;
#142896=CARTESIAN_POINT('Ctrl Pts',(-29.6274369403362,14.5097913596576,
128.100451442334)) ;
#142897=CARTESIAN_POINT('Ctrl Pts',(-29.7096257062941,14.4576092834796,
128.373496593985)) ;
#142898=CARTESIAN_POINT('Ctrl Pts',(-29.7848036126788,14.3304830753539,
128.626405753905)) ;
#142899=CARTESIAN_POINT('Ctrl Pts',(-29.845566912938,14.1386182913456,128.837024720556)) ;
#142900=CARTESIAN_POINT('Ctrl Pts',(-29.8872745466126,13.8965845637284,
128.991871079085)) ;
#142901=CARTESIAN_POINT('Ctrl Pts',(-29.9064534682672,13.6198364139058,
129.081022786347)) ;
#142902=CARTESIAN_POINT('Ctrl Pts',(-29.900787063049,13.3288843077371,129.097601934331)) ;
#142903=CARTESIAN_POINT('Ctrl Pts',(-29.8699337024441,13.0447398144614,
129.040604983945)) ;
#142904=CARTESIAN_POINT('Ctrl Pts',(-29.8156278311616,12.7881834818384,
128.91501253398)) ;
#142905=CARTESIAN_POINT('Ctrl Pts',(-29.7402027720901,12.5755908845443,
128.727989057223)) ;
#142906=CARTESIAN_POINT('Ctrl Pts',(-29.6498474075775,12.4257573634701,
128.496978543416)) ;
#142907=CARTESIAN_POINT('Ctrl Pts',(-29.5489205160236,12.3460112100503,
128.235293254381)) ;
#142908=CARTESIAN_POINT('Ctrl Pts',(-29.4441677154177,12.3439532777376,
127.962502290802)) ;
#142909=CARTESIAN_POINT('Ctrl Pts',(-29.3431323111502,12.4188219737117,
127.700394231621)) ;
#142910=CARTESIAN_POINT('Ctrl Pts',(-29.2511415646043,12.5668342389243,
127.464967305872)) ;
#142911=CARTESIAN_POINT('Ctrl Pts',(-29.1756958712415,12.7739567012615,
127.277464266888)) ;
#142912=CARTESIAN_POINT('Ctrl Pts',(-29.1197743038431,13.0292277214245,
127.147296176479)) ;
#142913=CARTESIAN_POINT('Ctrl Pts',(-29.0875900956306,13.3121169680532,
127.086372454532)) ;
#142914=CARTESIAN_POINT('Ctrl Pts',(-29.080439208884,13.603671342882,127.098665686775)) ;
#142915=CARTESIAN_POINT('Ctrl Pts',(-29.0983297264476,13.8822011658837,
127.184109243225)) ;
#142916=CARTESIAN_POINT('Ctrl Pts',(-29.1388833388726,14.1265341471654,
127.335581557334)) ;
#142917=CARTESIAN_POINT('Ctrl Pts',(-29.1987356919885,14.3215277974717,
127.543539347123)) ;
#142918=CARTESIAN_POINT('Ctrl Pts',(-29.273115428844,14.4523872873454,127.794044143669)) ;
#142919=CARTESIAN_POINT('Ctrl Pts',(-29.3554651301705,14.509081275177,128.067728441316)) ;
#142920=CARTESIAN_POINT('Ctrl Pts',(-29.4395851874039,14.4877530377578,
128.346676598338)) ;
#142921=CARTESIAN_POINT('Ctrl Pts',(-29.5179673179766,14.3906972119634,
128.608633598773)) ;
#142922=CARTESIAN_POINT('Ctrl Pts',(-29.5851982952717,14.2242126836462,
128.838160883835)) ;
#142923=CARTESIAN_POINT('Ctrl Pts',(-29.635328017071,14.0000453573048,129.01774887383)) ;
#142924=CARTESIAN_POINT('Ctrl Pts',(-29.6640587815373,13.7349940893193,
129.134772605438)) ;
#142925=CARTESIAN_POINT('Ctrl Pts',(-29.66853047681,13.4462937932098,129.181082266472)) ;
#142926=CARTESIAN_POINT('Ctrl Pts',(-29.6479806661709,13.1586523998495,
129.15397156145)) ;
#142927=CARTESIAN_POINT('Ctrl Pts',(-29.6024908386361,12.8863235955885,
129.05444952426)) ;
#142928=CARTESIAN_POINT('Ctrl Pts',(-29.5354346072489,12.6553854618845,
128.891574893748)) ;
#142929=CARTESIAN_POINT('Ctrl Pts',(-29.450747956121,12.4787538622729,128.677195270721)) ;
#142930=CARTESIAN_POINT('Ctrl Pts',(-29.3526089804549,12.3688114819393,
128.423824114578)) ;
#142931=CARTESIAN_POINT('Ctrl Pts',(-29.2490412806159,12.3354319131045,
128.154314887623)) ;
#142932=CARTESIAN_POINT('Ctrl Pts',(-29.1458394576041,12.3792576345139,
127.885902184127)) ;
#142933=CARTESIAN_POINT('Ctrl Pts',(-29.04916679697,12.4988399158766,127.636776287795)) ;
#142934=CARTESIAN_POINT('Ctrl Pts',(-28.9665629773405,12.6835118837374,
127.428475303792)) ;
#142935=CARTESIAN_POINT('Ctrl Pts',(-28.9021265706556,12.9214924452222,
127.273355660426)) ;
#142936=CARTESIAN_POINT('Ctrl Pts',(-28.8600821072398,13.1954917190088,
127.18365141452)) ;
#142937=CARTESIAN_POINT('Ctrl Pts',(-28.842696665374,13.4865486647074,127.166068582976)) ;
#142938=CARTESIAN_POINT('Ctrl Pts',(-28.850646619642,13.7724716992733,127.222433313962)) ;
#142939=CARTESIAN_POINT('Ctrl Pts',(-28.8822838217838,14.0322260172615,
127.34784163249)) ;
#142940=CARTESIAN_POINT('Ctrl Pts',(-28.9348883192046,14.249618629869,127.534639990214)) ;
#142941=CARTESIAN_POINT('Ctrl Pts',(-29.0041241934943,14.4079187286369,
127.770094835747)) ;
#142942=CARTESIAN_POINT('Ctrl Pts',(-29.0837267477703,14.4951289707047,
128.035675109478)) ;
#142943=CARTESIAN_POINT('Ctrl Pts',(-29.1678434679254,14.5060206612055,
128.314536420415)) ;
#142944=CARTESIAN_POINT('Ctrl Pts',(-29.2497073469964,14.4388851270518,
128.586900356964)) ;
#142945=CARTESIAN_POINT('Ctrl Pts',(-29.3223025667751,14.2990478381217,
128.832099458619)) ;
#142946=CARTESIAN_POINT('Ctrl Pts',(-29.3799249295879,14.0962769263581,
129.033581817066)) ;
#142947=CARTESIAN_POINT('Ctrl Pts',(-29.4176290706378,13.8463550292072,
129.176742685336)) ;
#142948=CARTESIAN_POINT('Ctrl Pts',(-29.4321974247897,13.5643760642883,
129.252539348112)) ;
#142949=CARTESIAN_POINT('Ctrl Pts',(-29.4217829780266,13.2747378724678,
129.255060449538)) ;
#142950=CARTESIAN_POINT('Ctrl Pts',(-29.3862948352972,12.9934295019574,
129.1846062214)) ;
#142951=CARTESIAN_POINT('Ctrl Pts',(-29.3276375405367,12.7438066422354,
129.046365113135)) ;
#142952=CARTESIAN_POINT('Ctrl Pts',(-29.2492689518633,12.542694227186,128.850560073051)) ;
#142953=CARTESIAN_POINT('Ctrl Pts',(-29.156078800014,12.4046935574579,128.611449593072)) ;
#142954=CARTESIAN_POINT('Ctrl Pts',(-29.0539430372178,12.3396331607935,
128.346227666517)) ;
#142955=CARTESIAN_POINT('Ctrl Pts',(-28.9496962563366,12.3522551180279,
128.074782981399)) ;
#142956=CARTESIAN_POINT('Ctrl Pts',(-28.849926492838,12.4411586824075,127.816395883758)) ;
#142957=CARTESIAN_POINT('Ctrl Pts',(-28.7605590312039,12.6013770610415,
127.588581938705)) ;
#142958=CARTESIAN_POINT('Ctrl Pts',(-28.6883543070743,12.819071741669,127.410650651919)) ;
#142959=CARTESIAN_POINT('Ctrl Pts',(-28.6367460501826,13.0807347129293,
127.293025418326)) ;
#142960=CARTESIAN_POINT('Ctrl Pts',(-28.6091712936872,13.3675409458687,
127.245666864385)) ;
#142961=CARTESIAN_POINT('Ctrl Pts',(-28.6067914289987,13.6570979950049,
127.271760239889)) ;
#142962=CARTESIAN_POINT('Ctrl Pts',(-28.6292800088116,13.9319894333905,
127.370771892158)) ;
#142963=CARTESIAN_POINT('Ctrl Pts',(-28.6737114216624,14.1676085516927,
127.5335038352)) ;
#142964=CARTESIAN_POINT('Ctrl Pts',(-28.7369049369059,14.3519029701599,
127.751335315566)) ;
#142965=CARTESIAN_POINT('Ctrl Pts',(-28.8129872581851,14.4687263887883,
128.006656410294)) ;
#142966=CARTESIAN_POINT('Ctrl Pts',(-28.8961104028969,14.5110206737837,
128.282595596457)) ;
#142967=CARTESIAN_POINT('Ctrl Pts',(-28.9795137356919,14.475483911121,128.559339823648)) ;
#142968=CARTESIAN_POINT('Ctrl Pts',(-29.0567266802165,14.3641243915887,
128.818105203385)) ;
#142969=CARTESIAN_POINT('Ctrl Pts',(-29.120945343812,14.185998118253,129.038755013211)) ;
#142970=CARTESIAN_POINT('Ctrl Pts',(-29.1673724631696,13.9527739610766,
129.207530855678)) ;
#142971=CARTESIAN_POINT('Ctrl Pts',(-29.1916772905069,13.6818171752754,
129.311643144904)) ;
#142972=CARTESIAN_POINT('Ctrl Pts',(-29.191513082233,13.392345635537,129.344277671689)) ;
#142973=CARTESIAN_POINT('Ctrl Pts',(-29.1660326258556,13.1044624962765,
129.303028370569)) ;
#142974=CARTESIAN_POINT('Ctrl Pts',(-29.1164519209928,12.8400819723837,
129.191300221752)) ;
#142975=CARTESIAN_POINT('Ctrl Pts',(-29.0456199048285,12.6174282729713,
129.017485608075)) ;
#142976=CARTESIAN_POINT('Ctrl Pts',(-28.9576757901538,12.452181454216,128.793738916405)) ;
#142977=CARTESIAN_POINT('Ctrl Pts',(-28.8583760496555,12.3567834927398,
128.536796874985)) ;
#142978=CARTESIAN_POINT('Ctrl Pts',(-28.7543916660935,12.3377092342152,
128.266071088682)) ;
#142979=CARTESIAN_POINT('Ctrl Pts',(-28.6517324722958,12.396207648245,127.999337715851)) ;
#142980=CARTESIAN_POINT('Ctrl Pts',(-28.5572877270569,12.5290433262916,
127.756671538889)) ;
#142981=CARTESIAN_POINT('Ctrl Pts',(-28.4778718732435,12.7244086521529,
127.557638995965)) ;
#142982=CARTESIAN_POINT('Ctrl Pts',(-28.4172847882494,12.970950220754,127.41382234341)) ;
#142983=CARTESIAN_POINT('Ctrl Pts',(-28.3797659678261,13.24944047257,127.337320504979)) ;
#142984=CARTESIAN_POINT('Ctrl Pts',(-28.3671847047696,13.5418969111079,
127.333850245581)) ;
#142985=CARTESIAN_POINT('Ctrl Pts',(-28.3796755155786,13.8230885860474,
127.403291738133)) ;
#142986=CARTESIAN_POINT('Ctrl Pts',(-28.4156802442814,14.0775912623992,
127.541659056659)) ;
#142987=CARTESIAN_POINT('Ctrl Pts',(-28.4717102355528,14.2842120208938,
127.738388350272)) ;
#142988=CARTESIAN_POINT('Ctrl Pts',(-28.5432604389653,14.4299776255762,
127.980546699844)) ;
#142989=CARTESIAN_POINT('Ctrl Pts',(-28.6248137961591,14.5033310573158,
128.252079015529)) ;
#142990=CARTESIAN_POINT('Ctrl Pts',(-28.7083919312205,14.4992417521952,
128.529128681056)) ;
#142991=CARTESIAN_POINT('Ctrl Pts',(-28.7892681436748,14.4177938992537,
128.79869937182)) ;
#142992=CARTESIAN_POINT('Ctrl Pts',(-28.8593764558841,14.2650804914184,
129.036610653591)) ;
#142993=CARTESIAN_POINT('Ctrl Pts',(-28.9134147220646,14.0529680000281,
129.227490443514)) ;
#142994=CARTESIAN_POINT('Ctrl Pts',(-28.9471011414545,13.7955268691578,
129.3589796482)) ;
#142995=CARTESIAN_POINT('Ctrl Pts',(-28.9570776705698,13.5095707979293,
129.421414389121)) ;
#142996=CARTESIAN_POINT('Ctrl Pts',(-28.9417243006281,13.2189035142274,
129.409677362568)) ;
#142997=CARTESIAN_POINT('Ctrl Pts',(-28.9018277588826,12.9437119836813,
129.326137208322)) ;
#142998=CARTESIAN_POINT('Ctrl Pts',(-28.8391939509021,12.7018112503585,
129.17628858698)) ;
#142999=CARTESIAN_POINT('Ctrl Pts',(-28.7575688794774,12.5115374305282,
128.970987035415)) ;
#143000=CARTESIAN_POINT('Ctrl Pts',(-28.6622219712875,12.3865362301687,
128.725579337275)) ;
#143001=CARTESIAN_POINT('Ctrl Pts',(-28.5587510574966,12.3360647675439,
128.456580284187)) ;
#143002=CARTESIAN_POINT('Ctrl Pts',(-28.4555305358195,12.3630945112241,
128.187903732276)) ;
#143003=CARTESIAN_POINT('Ctrl Pts',(-28.3566879058951,12.466576968382,127.932449994111)) ;
#143004=CARTESIAN_POINT('Ctrl Pts',(-28.2706251997226,12.6378737412179,
127.714064371724)) ;
#143005=CARTESIAN_POINT('Ctrl Pts',(-28.2016344309745,12.8661806777279,
127.545715311069)) ;
#143006=CARTESIAN_POINT('Ctrl Pts',(-28.1545836946371,13.133327748888,127.441304758509)) ;
#143007=CARTESIAN_POINT('Ctrl Pts',(-28.1316798850368,13.4221934769942,
127.407563269515)) ;
#143008=CARTESIAN_POINT('Ctrl Pts',(-28.1340477421079,13.7107571262916,
127.447593177881)) ;
#143009=CARTESIAN_POINT('Ctrl Pts',(-28.1609619636342,13.9798563789946,
127.559489257503)) ;
#143010=CARTESIAN_POINT('Ctrl Pts',(-28.2093006124176,14.2070905645433,
127.733705392524)) ;
#143011=CARTESIAN_POINT('Ctrl Pts',(-28.2752017753927,14.3790287585347,
127.959331880187)) ;
#143012=CARTESIAN_POINT('Ctrl Pts',(-28.3530820320636,14.4826462603949,
128.219918375423)) ;
#143013=CARTESIAN_POINT('Ctrl Pts',(-28.4373112880813,14.5101765741511,
128.49929849806)) ;
#143014=CARTESIAN_POINT('Ctrl Pts',(-28.519474085672,14.4602520915312,128.772202055633)) ;
#143015=CARTESIAN_POINT('Ctrl Pts',(-28.5950471255898,14.3349862853441,
129.026308923663)) ;
#143016=CARTESIAN_POINT('Ctrl Pts',(-28.6560285639578,14.1459035788167,
129.237399512473)) ;
#143017=CARTESIAN_POINT('Ctrl Pts',(-28.698619817941,13.9042673527481,129.394971716019)) ;
#143018=CARTESIAN_POINT('Ctrl Pts',(-28.7184673372425,13.6274932797063,
129.486151626671)) ;
#143019=CARTESIAN_POINT('Ctrl Pts',(-28.7135006465235,13.3375399739688,
129.504678260935)) ;
#143020=CARTESIAN_POINT('Ctrl Pts',(-28.6834932097191,13.0529654851711,
129.450131261485)) ;
#143021=CARTESIAN_POINT('Ctrl Pts',(-28.6292897606013,12.7935418575334,
129.325100800843)) ;
#143022=CARTESIAN_POINT('Ctrl Pts',(-28.5550549856277,12.5815360245405,
129.141238342052)) ;
#143023=CARTESIAN_POINT('Ctrl Pts',(-28.4646576427796,12.4287257654979,
128.910282719979)) ;
#143024=CARTESIAN_POINT('Ctrl Pts',(-28.363677082995,12.3470719681604,128.64850632388)) ;
#143025=CARTESIAN_POINT('Ctrl Pts',(-28.2591488468396,12.3430683476044,
128.376304331127)) ;
#143026=CARTESIAN_POINT('Ctrl Pts',(-28.1582862016969,12.4155936903918,
128.114589342041)) ;
#143027=CARTESIAN_POINT('Ctrl Pts',(-28.0661544614373,12.5608877107137,
127.878647626776)) ;
#143028=CARTESIAN_POINT('Ctrl Pts',(-27.9897622819606,12.76729595803,127.688541378532)) ;
#143029=CARTESIAN_POINT('Ctrl Pts',(-27.9331944991847,13.021989825902,127.556534508152)) ;
#143030=CARTESIAN_POINT('Ctrl Pts',(-27.9004198086109,13.303543839919,127.493791149837)) ;
#143031=CARTESIAN_POINT('Ctrl Pts',(-27.8925042874101,13.5948424473805,
127.503816308611)) ;
#143032=CARTESIAN_POINT('Ctrl Pts',(-27.9096152355407,13.8739531403396,
127.586963478625)) ;
#143033=CARTESIAN_POINT('Ctrl Pts',(-27.9496646620447,14.1203175585331,
127.737068535428)) ;
#143034=CARTESIAN_POINT('Ctrl Pts',(-28.0090231272187,14.3167169570115,
127.943561552684)) ;
#143035=CARTESIAN_POINT('Ctrl Pts',(-28.0828620310095,14.4494067343281,
128.192402472001)) ;
#143036=CARTESIAN_POINT('Ctrl Pts',(-28.1651717407411,14.5084702765568,
128.466017783128)) ;
#143037=CARTESIAN_POINT('Ctrl Pts',(-28.2490683969256,14.4897007225782,
128.744200921648)) ;
#143038=CARTESIAN_POINT('Ctrl Pts',(-28.3280752188241,14.3946105615284,
129.008131391206)) ;
#143039=CARTESIAN_POINT('Ctrl Pts',(-28.3958042440866,14.2294634797175,
129.23917393567)) ;
#143040=CARTESIAN_POINT('Ctrl Pts',(-28.4463272391741,14.0073333338193,
129.419816794305)) ;
#143041=CARTESIAN_POINT('Ctrl Pts',(-28.4757409397969,13.743582797636,129.538801386051)) ;
#143042=CARTESIAN_POINT('Ctrl Pts',(-28.4810001371008,13.4548247152231,
129.587459496954)) ;
#143043=CARTESIAN_POINT('Ctrl Pts',(-28.461059887965,13.1663898310179,129.562197963423)) ;
#143044=CARTESIAN_POINT('Ctrl Pts',(-28.41656739466,12.8948251828515,129.465387320094)) ;
#143045=CARTESIAN_POINT('Ctrl Pts',(-28.3499271169494,12.661361440579,129.303861114263)) ;
#143046=CARTESIAN_POINT('Ctrl Pts',(-28.2654515362701,12.4827884895572,
129.090166702319)) ;
#143047=CARTESIAN_POINT('Ctrl Pts',(-28.1681467304688,12.3713199015498,
128.839048548618)) ;
#143048=CARTESIAN_POINT('Ctrl Pts',(-28.0645799433211,12.3351536533699,
128.569574159567)) ;
#143049=CARTESIAN_POINT('Ctrl Pts',(-27.9607827823663,12.3771106009455,
128.299581621144)) ;
#143050=CARTESIAN_POINT('Ctrl Pts',(-27.8644780082732,12.4937460494275,
128.051299065574)) ;
#143051=CARTESIAN_POINT('Ctrl Pts',(-27.7810699349148,12.6767291591256,
127.840739185193)) ;
#143052=CARTESIAN_POINT('Ctrl Pts',(-27.7157445671607,12.9147363341255,
127.683191915483)) ;
#143053=CARTESIAN_POINT('Ctrl Pts',(-27.6732296957668,13.1870897744472,
127.59199890341)) ;
#143054=CARTESIAN_POINT('Ctrl Pts',(-27.6550770827887,13.4771403047647,
127.572086844516)) ;
#143055=CARTESIAN_POINT('Ctrl Pts',(-27.6622219471036,13.7642377896945,
127.626175179984)) ;
#143056=CARTESIAN_POINT('Ctrl Pts',(-27.6934344667264,14.0261140993903,
127.750502240094)) ;
#143057=CARTESIAN_POINT('Ctrl Pts',(-27.7452532633533,14.2437566933168,
127.934829589344)) ;
#143058=CARTESIAN_POINT('Ctrl Pts',(-27.814130143941,14.4043005148666,128.169276756387)) ;
#143059=CARTESIAN_POINT('Ctrl Pts',(-27.8935228607594,14.4936452056158,
128.434244053094)) ;
#143060=CARTESIAN_POINT('Ctrl Pts',(-27.9775948902962,14.5067755080675,
128.712972810078)) ;
#143061=CARTESIAN_POINT('Ctrl Pts',(-28.0595004608224,14.4421250993153,
128.98539905036)) ;
#143062=CARTESIAN_POINT('Ctrl Pts',(-28.1325782921938,14.3039890578845,
129.232076923519)) ;
#143063=CARTESIAN_POINT('Ctrl Pts',(-28.1904918232912,14.1040920585568,
129.434238070627)) ;
#143064=CARTESIAN_POINT('Ctrl Pts',(-28.2291431873281,13.8535850410252,
129.580412255891)) ;
#143065=CARTESIAN_POINT('Ctrl Pts',(-28.2443210492215,13.573095030684,129.657872655295)) ;
#143066=CARTESIAN_POINT('Ctrl Pts',(-28.2346408638536,13.2829859633842,
129.662599052892)) ;
#143067=CARTESIAN_POINT('Ctrl Pts',(-28.1999752849308,13.0017735288795,
129.594458814166)) ;
#143068=CARTESIAN_POINT('Ctrl Pts',(-28.1417676131385,12.7500889121872,
129.457648777599)) ;
#143069=CARTESIAN_POINT('Ctrl Pts',(-28.0639229564631,12.5475576765503,
129.263351153657)) ;
#143070=CARTESIAN_POINT('Ctrl Pts',(-27.9709828123923,12.4075651763914,
129.02500225527)) ;
#143071=CARTESIAN_POINT('Ctrl Pts',(-27.8693506787333,12.3405227195362,
128.761141757557)) ;
#143072=CARTESIAN_POINT('Ctrl Pts',(-27.7648049873815,12.3506976033877,
128.488907346772)) ;
#143073=CARTESIAN_POINT('Ctrl Pts',(-27.6644555408828,12.4381775614935,
128.228958563771)) ;
#143074=CARTESIAN_POINT('Ctrl Pts',(-27.5751702428162,12.5958828969702,
128.001218540191)) ;
#143075=CARTESIAN_POINT('Ctrl Pts',(-27.502283193488,12.8123888981795,127.821351130497)) ;
#143076=CARTESIAN_POINT('Ctrl Pts',(-27.450031586974,13.0732935402693,127.701864848652)) ;
#143077=CARTESIAN_POINT('Ctrl Pts',(-27.4217776748689,13.3601445566741,
127.652571547418)) ;
#143078=CARTESIAN_POINT('Ctrl Pts',(-27.418773970736,13.6487325565986,127.676717562199)) ;
#143079=CARTESIAN_POINT('Ctrl Pts',(-27.4403379990912,13.9231969676619,
127.772866432049)) ;
#143080=CARTESIAN_POINT('Ctrl Pts',(-27.4843681376287,14.161664923211,127.934621131012)) ;
#143081=CARTESIAN_POINT('Ctrl Pts',(-27.5471256039461,14.3474885312589,
128.151168293149)) ;
#143082=CARTESIAN_POINT('Ctrl Pts',(-27.6228649944064,14.4664584642889,
128.405473991337)) ;
#143083=CARTESIAN_POINT('Ctrl Pts',(-27.7062638841247,14.5109046596075,
128.682368151807)) ;
#143084=CARTESIAN_POINT('Ctrl Pts',(-27.7893507587579,14.4775384051983,
128.958029757662)) ;
#143085=CARTESIAN_POINT('Ctrl Pts',(-27.8669709430451,14.3681997153804,
129.218037882252)) ;
#143086=CARTESIAN_POINT('Ctrl Pts',(-27.9316058833016,14.1916180826176,
129.439912282084)) ;
#143087=CARTESIAN_POINT('Ctrl Pts',(-27.9785106186434,13.9603525000671,
129.610001559058)) ;
#143088=CARTESIAN_POINT('Ctrl Pts',(-28.0035618824634,13.6895220896488,
129.716380788557)) ;
#143089=CARTESIAN_POINT('Ctrl Pts',(-28.0040495835783,13.4007319535163,
129.750868768487)) ;
#143090=CARTESIAN_POINT('Ctrl Pts',(-27.9794449922936,13.1132078069033,
129.712088512607)) ;
#143091=CARTESIAN_POINT('Ctrl Pts',(-27.9302630163752,12.846606824237,129.601692481036)) ;
#143092=CARTESIAN_POINT('Ctrl Pts',(-27.8603417733815,12.623698437481,129.430363738554)) ;
#143093=CARTESIAN_POINT('Ctrl Pts',(-27.772694620763,12.4561011636242,129.207550748791)) ;
#143094=CARTESIAN_POINT('Ctrl Pts',(-27.6737731829943,12.3585967931485,
128.951668241225)) ;
#143095=CARTESIAN_POINT('Ctrl Pts',(-27.5695149442883,12.3371246783343,
128.680247071619)) ;
#143096=CARTESIAN_POINT('Ctrl Pts',(-27.466838847916,12.3935413864574,128.413427301181)) ;
#143097=CARTESIAN_POINT('Ctrl Pts',(-27.3723658112914,12.5236724613545,
128.170561312785)) ;
#143098=CARTESIAN_POINT('Ctrl Pts',(-27.2920858688792,12.7179305396398,
127.969133189608)) ;
#143099=CARTESIAN_POINT('Ctrl Pts',(-27.2307490661673,12.9643002141067,
127.823241817984)) ;
#143100=CARTESIAN_POINT('Ctrl Pts',(-27.1927875893493,13.2410163015689,
127.74530764181)) ;
#143101=CARTESIAN_POINT('Ctrl Pts',(-27.1794002354583,13.5320328266363,
127.739328215748)) ;
#143102=CARTESIAN_POINT('Ctrl Pts',(-27.1911525976807,13.8151978209727,
127.806773844443)) ;
#143103=CARTESIAN_POINT('Ctrl Pts',(-27.226570298699,14.0709652782984,127.943449594362)) ;
#143104=CARTESIAN_POINT('Ctrl Pts',(-27.2822196281639,14.2795163173677,
128.139134706522)) ;
#143105=CARTESIAN_POINT('Ctrl Pts',(-27.3532889376274,14.4266234403896,
128.379816035706)) ;
#143106=CARTESIAN_POINT('Ctrl Pts',(-27.4341580000532,14.5021445242865,
128.649158484748)) ;
#143107=CARTESIAN_POINT('Ctrl Pts',(-27.5183881057503,14.5004798974739,
128.928367380574)) ;
#143108=CARTESIAN_POINT('Ctrl Pts',(-27.5992329747341,14.4210757518903,
129.197760560483)) ;
#143109=CARTESIAN_POINT('Ctrl Pts',(-27.6694923473982,14.2711636067417,
129.435985416657)) ;
#143110=CARTESIAN_POINT('Ctrl Pts',(-27.7243575187803,14.0600318658462,
129.629403124372)) ;
#143111=CARTESIAN_POINT('Ctrl Pts',(-27.7587068568811,13.8025044724255,
129.762955028685)) ;
#143112=CARTESIAN_POINT('Ctrl Pts',(-27.7693309736884,13.5194348559979,
129.827002883379)) ;
#143113=CARTESIAN_POINT('Ctrl Pts',(-27.7548332219261,13.2279296915562,
129.817849904189)) ;
#143114=CARTESIAN_POINT('Ctrl Pts',(-27.7155874618165,12.9514278673655,
129.736271623692)) ;
#143115=CARTESIAN_POINT('Ctrl Pts',(-27.653314484704,12.7076269304905,129.587584820316)) ;
#143116=CARTESIAN_POINT('Ctrl Pts',(-27.572509924976,12.5164543303433,129.384536694103)) ;
#143117=CARTESIAN_POINT('Ctrl Pts',(-27.4772456621855,12.3891143614251,
129.139458063282)) ;
#143118=CARTESIAN_POINT('Ctrl Pts',(-27.3744497556545,12.3364756135891,
128.872254272894)) ;
#143119=CARTESIAN_POINT('Ctrl Pts',(-27.2704082203507,12.3612642379946,
128.601421099459)) ;
#143120=CARTESIAN_POINT('Ctrl Pts',(-27.1713773382745,12.4629839046161,
128.345404662449)) ;
#143121=CARTESIAN_POINT('Ctrl Pts',(-27.0851007677242,12.6321971909499,
128.126327881533)) ;
#143122=CARTESIAN_POINT('Ctrl Pts',(-27.015641032897,12.8584558944589,127.956532197619)) ;
#143123=CARTESIAN_POINT('Ctrl Pts',(-26.9676850720169,13.126164869302,127.84965606525)) ;
#143124=CARTESIAN_POINT('Ctrl Pts',(-26.9442084970736,13.4141234527586,
127.814163915492)) ;
#143125=CARTESIAN_POINT('Ctrl Pts',(-26.9458709815039,13.7023852281616,
127.852074256674)) ;
#143126=CARTESIAN_POINT('Ctrl Pts',(-26.9718751244399,13.9714211958417,
127.961170070242)) ;
#143127=CARTESIAN_POINT('Ctrl Pts',(-27.0200293376702,14.2020200814189,
128.135130194059)) ;
#143128=CARTESIAN_POINT('Ctrl Pts',(-27.0853698779214,14.3750071777218,
128.359015009443)) ;
#143129=CARTESIAN_POINT('Ctrl Pts',(-27.1629746883779,14.4806351397631,
128.618798290785)) ;
#143130=CARTESIAN_POINT('Ctrl Pts',(-27.2467360159308,14.5105855300703,
128.896650717923)) ;
#143131=CARTESIAN_POINT('Ctrl Pts',(-27.3295913980905,14.4625550533332,
129.171811865125)) ;
#143132=CARTESIAN_POINT('Ctrl Pts',(-27.4050082321251,14.3400369090667,
129.425253916033)) ;
#143133=CARTESIAN_POINT('Ctrl Pts',(-27.4667526234034,14.1521956958397,
129.638700651972)) ;
#143134=CARTESIAN_POINT('Ctrl Pts',(-27.509920728559,13.9116488292757,129.797965117592)) ;
#143135=CARTESIAN_POINT('Ctrl Pts',(-27.5304424424998,13.6358543135724,
129.891087447677)) ;
#143136=CARTESIAN_POINT('Ctrl Pts',(-27.5262343520398,13.3459426369887,
129.911837713114)) ;
#143137=CARTESIAN_POINT('Ctrl Pts',(-27.4968203591533,13.0604648346963,
129.859083942663)) ;
#143138=CARTESIAN_POINT('Ctrl Pts',(-27.4436406639866,12.8015142493302,
129.736839092141)) ;
#143139=CARTESIAN_POINT('Ctrl Pts',(-27.3697110305104,12.5868713096869,
129.554007522395)) ;
#143140=CARTESIAN_POINT('Ctrl Pts',(-27.2796913738203,12.432303139715,129.324145798948)) ;
#143141=CARTESIAN_POINT('Ctrl Pts',(-27.1792802958715,12.3486039806668,
129.063923184096)) ;
#143142=CARTESIAN_POINT('Ctrl Pts',(-27.0747302802551,12.3418345477554,
128.791666168228)) ;
#143143=CARTESIAN_POINT('Ctrl Pts',(-26.9730648540773,12.4127258480294,
128.527813593233)) ;
#143144=CARTESIAN_POINT('Ctrl Pts',(-26.8810202662406,12.5554431662894,
128.291966182553)) ;
#143145=CARTESIAN_POINT('Ctrl Pts',(-26.8038302880742,12.7608030962308,
128.099638464274)) ;
#143146=CARTESIAN_POINT('Ctrl Pts',(-26.7467082859449,13.0143081230203,
127.965989241137)) ;
#143147=CARTESIAN_POINT('Ctrl Pts',(-26.713205468323,13.29536631424,127.901127763773)) ;
#143148=CARTESIAN_POINT('Ctrl Pts',(-26.7045894976719,13.5874993963847,
127.909194608933)) ;
#143149=CARTESIAN_POINT('Ctrl Pts',(-26.7211066559591,13.8669340437894,
127.990583783677)) ;
#143150=CARTESIAN_POINT('Ctrl Pts',(-26.7603551603999,14.1134264974216,
128.13820542311)) ;
#143151=CARTESIAN_POINT('Ctrl Pts',(-26.8193522325074,14.312178191849,128.34373825684)) ;
#143152=CARTESIAN_POINT('Ctrl Pts',(-26.8931267445792,14.447005080599,128.592489132649)) ;
#143153=CARTESIAN_POINT('Ctrl Pts',(-26.9751504369521,14.50780864275,128.865206484874)) ;
#143154=CARTESIAN_POINT('Ctrl Pts',(-27.0588159564451,14.4913412466958,
129.142606878717)) ;
#143155=CARTESIAN_POINT('Ctrl Pts',(-27.1380385087885,14.3985298499944,
129.40715742329)) ;
#143156=CARTESIAN_POINT('Ctrl Pts',(-27.2062467307682,14.23537642446,129.639608049856)) ;
#143157=CARTESIAN_POINT('Ctrl Pts',(-27.2575581083356,14.0132823702427,
129.822743994824)) ;
#143158=CARTESIAN_POINT('Ctrl Pts',(-27.2873688840562,13.7517705184138,
129.942709762938)) ;
#143159=CARTESIAN_POINT('Ctrl Pts',(-27.293472251736,13.4639004109061,129.993782745323)) ;
#143160=CARTESIAN_POINT('Ctrl Pts',(-27.2740851665503,13.1736259239267,
129.970325135161)) ;
#143161=CARTESIAN_POINT('Ctrl Pts',(-27.2305215118996,12.9029494163379,
129.876022131441)) ;
#143162=CARTESIAN_POINT('Ctrl Pts',(-27.1642896249734,12.6670694779248,
129.715817346972)) ;
#143163=CARTESIAN_POINT('Ctrl Pts',(-27.0800464564361,12.4867414541686,
129.502856286838)) ;
#143164=CARTESIAN_POINT('Ctrl Pts',(-26.9834820409465,12.3736046966953,
129.253747171097)) ;
#143165=CARTESIAN_POINT('Ctrl Pts',(-26.879418915152,12.3351061358333,128.983013182515)) ;
#143166=CARTESIAN_POINT('Ctrl Pts',(-26.7762312191263,12.3747297398712,
128.714574685413)) ;
#143167=CARTESIAN_POINT('Ctrl Pts',(-26.6793849366064,12.4890530278271,
128.46477378363)) ;
#143168=CARTESIAN_POINT('Ctrl Pts',(-26.5950275521023,12.671847392328,128.251667519718)) ;
#143169=CARTESIAN_POINT('Ctrl Pts',(-26.5296066139418,12.9071471276995,
128.093622284971)) ;
#143170=CARTESIAN_POINT('Ctrl Pts',(-26.4862925849143,13.1791584028572,
128.000158541116)) ;
#143171=CARTESIAN_POINT('Ctrl Pts',(-26.4674803411247,13.4685703859445,
127.978264630818)) ;
#143172=CARTESIAN_POINT('Ctrl Pts',(-26.4738622862666,13.7556866314948,
128.030081960704)) ;
#143173=CARTESIAN_POINT('Ctrl Pts',(-26.5043022522006,14.0184521546514,
128.152120496671)) ;
#143174=CARTESIAN_POINT('Ctrl Pts',(-26.5558322179965,14.2386836272176,
128.335773179578)) ;
#143175=CARTESIAN_POINT('Ctrl Pts',(-26.6243219235215,14.4009245820624,
128.569075258418)) ;
#143176=CARTESIAN_POINT('Ctrl Pts',(-26.7037459041493,14.4923209355322,
128.834232583563)) ;
#143177=CARTESIAN_POINT('Ctrl Pts',(-26.7873700011777,14.5074993707076,
129.111483360412)) ;
#143178=CARTESIAN_POINT('Ctrl Pts',(-26.869769976205,14.4446390736038,129.38550037864)) ;
#143179=CARTESIAN_POINT('Ctrl Pts',(-26.942794278446,14.3090137807522,129.63184995493)) ;
#143180=CARTESIAN_POINT('Ctrl Pts',(-27.001348624657,14.1104147854154,129.835955195458)) ;
#143181=CARTESIAN_POINT('Ctrl Pts',(-27.0405182096425,13.8614586698981,
129.983581974093)) ;
#143182=CARTESIAN_POINT('Ctrl Pts',(-27.0564545067552,13.5819684927305,
130.063220990945)) ;
#143183=CARTESIAN_POINT('Ctrl Pts',(-27.0474617770525,13.2906276884224,
130.070095552532)) ;
#143184=CARTESIAN_POINT('Ctrl Pts',(-27.0134271462375,13.0092431055299,
130.003763417619)) ;
#143185=CARTESIAN_POINT('Ctrl Pts',(-26.9561897398293,12.7575166399562,
129.869627977763)) ;
#143186=CARTESIAN_POINT('Ctrl Pts',(-26.878600427533,12.5525238857448,129.676201545283)) ;
#143187=CARTESIAN_POINT('Ctrl Pts',(-26.786267640891,12.4108769573351,129.439535650803)) ;
#143188=CARTESIAN_POINT('Ctrl Pts',(-26.6844582304523,12.3412908932615,
129.175275636481)) ;
#143189=CARTESIAN_POINT('Ctrl Pts',(-26.5800334572457,12.3493862056845,
128.903348153925)) ;
#143190=CARTESIAN_POINT('Ctrl Pts',(-26.4797393076399,12.434272868394,128.643467145807)) ;
#143191=CARTESIAN_POINT('Ctrl Pts',(-26.3898901908696,12.5900490117304,
128.414124382121)) ;
#143192=CARTESIAN_POINT('Ctrl Pts',(-26.3162603078544,12.8056267290578,
128.232173964895)) ;
#143193=CARTESIAN_POINT('Ctrl Pts',(-26.2634623259816,13.065385008078,128.111066358889)) ;
#143194=CARTESIAN_POINT('Ctrl Pts',(-26.2345041414233,13.3504852311182,
128.059568931144)) ;
#143195=CARTESIAN_POINT('Ctrl Pts',(-26.2307238031498,13.6412799194347,
128.081681426423)) ;
#143196=CARTESIAN_POINT('Ctrl Pts',(-26.2516126185945,13.9155482376954,
128.175749664471)) ;
#143197=CARTESIAN_POINT('Ctrl Pts',(-26.2949893624843,14.1552942576475,
128.335588778516)) ;
#143198=CARTESIAN_POINT('Ctrl Pts',(-26.3572525364643,14.3429102218091,
128.550683951018)) ;
#143199=CARTESIAN_POINT('Ctrl Pts',(-26.4327879058784,14.4639893151741,
128.804436412996)) ;
#143200=CARTESIAN_POINT('Ctrl Pts',(-26.5157245235423,14.5107279947802,
129.079841196809)) ;
#143201=CARTESIAN_POINT('Ctrl Pts',(-26.599342755531,14.4794893711203,129.357238144724)) ;
#143202=CARTESIAN_POINT('Ctrl Pts',(-26.6768758741317,14.3727211556821,
129.616834198873)) ;
#143203=CARTESIAN_POINT('Ctrl Pts',(-26.742126370631,14.1977799605459,129.840578904122)) ;
#143204=CARTESIAN_POINT('Ctrl Pts',(-26.7896263521605,13.9680803092071,
130.012384935134)) ;
#143205=CARTESIAN_POINT('Ctrl Pts',(-26.8154360590847,13.6967826979273,
130.121139587608)) ;
#143206=CARTESIAN_POINT('Ctrl Pts',(-26.8165967221177,13.4094043760134,
130.157455368201)) ;
#143207=CARTESIAN_POINT('Ctrl Pts',(-26.7926969292554,13.1212039235338,
130.120777584093)) ;
#143208=CARTESIAN_POINT('Ctrl Pts',(-26.7444083705524,12.8546896055266,
130.012858824521)) ;
#143209=CARTESIAN_POINT('Ctrl Pts',(-26.6749139207326,12.6293810119528,
129.842883806981)) ;
#143210=CARTESIAN_POINT('Ctrl Pts',(-26.5872220070184,12.4594635136683,
129.62009200021)) ;
#143211=CARTESIAN_POINT('Ctrl Pts',(-26.4890425150724,12.3604529147884,
129.366204449936)) ;
#143212=CARTESIAN_POINT('Ctrl Pts',(-26.3845073686079,12.3366695110087,
129.094084042648)) ;
#143213=CARTESIAN_POINT('Ctrl Pts',(-26.2821289297751,12.3907630911244,
128.827994581518)) ;
#143214=CARTESIAN_POINT('Ctrl Pts',(-26.187128095685,12.5187718172597,128.583638766626)) ;
#143215=CARTESIAN_POINT('Ctrl Pts',(-26.1060949547663,12.7125554078675,
128.380162610462)) ;
#143216=CARTESIAN_POINT('Ctrl Pts',(-26.0447561615951,12.9551209833767,
128.233921001561)) ;
#143217=CARTESIAN_POINT('Ctrl Pts',(-26.0057078064282,13.2325621685243,
128.153002106468)) ;
#143218=CARTESIAN_POINT('Ctrl Pts',(-25.9916571139282,13.5243421587289,
128.145175592515)) ;
#143219=CARTESIAN_POINT('Ctrl Pts',(-26.0026775791259,13.8069928303566,
128.210366181038)) ;
#143220=CARTESIAN_POINT('Ctrl Pts',(-26.0374047644475,14.0639001821586,
128.345024781301)) ;
#143221=CARTESIAN_POINT('Ctrl Pts',(-26.0925147260829,14.274156022816,128.539139181305)) ;
#143222=CARTESIAN_POINT('Ctrl Pts',(-26.1633735273204,14.4234616465823,
128.779279376222)) ;
#143223=CARTESIAN_POINT('Ctrl Pts',(-26.2439599577869,14.5011170980349,
129.047753483437)) ;
#143224=CARTESIAN_POINT('Ctrl Pts',(-26.3285030639104,14.501361448933,129.328007829175)) ;
#143225=CARTESIAN_POINT('Ctrl Pts',(-26.4088108195145,14.4249955787507,
129.595519956069)) ;
#143226=CARTESIAN_POINT('Ctrl Pts',(-26.4800874345285,14.2760170248169,
129.836998320279)) ;
#143227=CARTESIAN_POINT('Ctrl Pts',(-26.5352515744716,14.0665440737742,
130.031218298945)) ;
#143228=CARTESIAN_POINT('Ctrl Pts',(-26.5702400842864,13.8110526556412,
130.166533147419)) ;
#143229=CARTESIAN_POINT('Ctrl Pts',(-26.5815726590234,13.5262784611541,
130.232906371947)) ;
#143230=CARTESIAN_POINT('Ctrl Pts',(-26.5678635340945,13.2368368163846,
130.225803590966)) ;
#143231=CARTESIAN_POINT('Ctrl Pts',(-26.5291217423332,12.9583254451164,
130.145867702787)) ;
#143232=CARTESIAN_POINT('Ctrl Pts',(-26.4678331545185,12.7145798984787,
129.999860683866)) ;
#143233=CARTESIAN_POINT('Ctrl Pts',(-26.3867440068472,12.5201729680917,
129.796286454842)) ;
#143234=CARTESIAN_POINT('Ctrl Pts',(-26.2927852183014,12.3922976801848,
129.554661598127)) ;
#143235=CARTESIAN_POINT('Ctrl Pts',(-26.1895660009278,12.3368042006491,
129.28641664148)) ;
#143236=CARTESIAN_POINT('Ctrl Pts',(-26.0858016380748,12.3594079761625,
129.016280828409)) ;
#143237=CARTESIAN_POINT('Ctrl Pts',(-25.9864031337543,12.458842653819,128.759223963542)) ;
#143238=CARTESIAN_POINT('Ctrl Pts',(-25.8996090906676,12.6263833262832,
128.538666355053)) ;
#143239=CARTESIAN_POINT('Ctrl Pts',(-25.8295827174989,12.8513078347283,
128.367225899866)) ;
#143240=CARTESIAN_POINT('Ctrl Pts',(-25.781006901016,13.1175342113745,128.258472258186)) ;
#143241=CARTESIAN_POINT('Ctrl Pts',(-25.7567380807917,13.4059955031651,
128.220766348)) ;
#143242=CARTESIAN_POINT('Ctrl Pts',(-25.7576446857111,13.6942419631863,
128.256424466659)) ;
#143243=CARTESIAN_POINT('Ctrl Pts',(-25.7832873182616,13.9656571301542,
128.36468485081)) ;
#143244=CARTESIAN_POINT('Ctrl Pts',(-25.8302149885515,14.1945698171883,
128.53461018047)) ;
#143245=CARTESIAN_POINT('Ctrl Pts',(-25.895500840112,14.3711224521538,128.758593840646)) ;
#143246=CARTESIAN_POINT('Ctrl Pts',(-25.9728377548636,14.4785950112144,
129.017572340248)) ;
#143247=CARTESIAN_POINT('Ctrl Pts',(-26.056604347087,14.5108133119048,129.295478786872)) ;
#143248=CARTESIAN_POINT('Ctrl Pts',(-26.1394268468674,14.465039412922,129.570481762383)) ;
#143249=CARTESIAN_POINT('Ctrl Pts',(-26.2151348850256,14.3446919180205,
129.824767484077)) ;
#143250=CARTESIAN_POINT('Ctrl Pts',(-26.2774107699029,14.1586507475217,
130.039773742848)) ;
#143251=CARTESIAN_POINT('Ctrl Pts',(-26.3212982659288,13.9182141888542,
130.201285607756)) ;
#143252=CARTESIAN_POINT('Ctrl Pts',(-26.3423778627286,13.6446893381856,
130.295847000978)) ;
#143253=CARTESIAN_POINT('Ctrl Pts',(-26.3389066565706,13.3538162430507,
130.318882585942)) ;
#143254=CARTESIAN_POINT('Ctrl Pts',(-26.3102603550136,13.0687528103835,
130.268268932066)) ;
#143255=CARTESIAN_POINT('Ctrl Pts',(-26.2576977023151,12.808402450481,130.147871722525)) ;
#143256=CARTESIAN_POINT('Ctrl Pts',(-26.1843413480049,12.5923661463697,
129.966695992935)) ;
#143257=CARTESIAN_POINT('Ctrl Pts',(-26.0945780045174,12.4355966192842,
129.737634921388)) ;
#143258=CARTESIAN_POINT('Ctrl Pts',(-25.9941838470144,12.3498833858894,
129.477517705028)) ;
#143259=CARTESIAN_POINT('Ctrl Pts',(-25.8901883755494,12.3409543002999,
129.206711463543)) ;
#143260=CARTESIAN_POINT('Ctrl Pts',(-25.7882740958192,12.4093757985287,
128.942149411662)) ;
#143261=CARTESIAN_POINT('Ctrl Pts',(-25.6956212849253,12.5505197572112,
128.704612922647)) ;
#143262=CARTESIAN_POINT('Ctrl Pts',(-25.6180396767608,12.7541804700571,
128.511108725249)) ;
#143263=CARTESIAN_POINT('Ctrl Pts',(-25.5604107173287,13.0055269427028,
128.375859916493)) ;
#143264=CARTESIAN_POINT('Ctrl Pts',(-25.526031444965,13.2870727031463,128.308567998837)) ;
#143265=CARTESIAN_POINT('Ctrl Pts',(-25.5167159350328,13.5781356431356,
128.314465472164)) ;
#143266=CARTESIAN_POINT('Ctrl Pts',(-25.532383711498,13.8583664416102,128.393378284334)) ;
#143267=CARTESIAN_POINT('Ctrl Pts',(-25.5712031763481,14.1072756620479,
128.539909138783)) ;
#143268=CARTESIAN_POINT('Ctrl Pts',(-25.6295827662988,14.3069767003197,
128.743547855544)) ;
#143269=CARTESIAN_POINT('Ctrl Pts',(-25.7026733511847,14.4436141295833,
128.990173698217)) ;
#143270=CARTESIAN_POINT('Ctrl Pts',(-25.7848004053856,14.5071928211091,
129.263307294218)) ;
#143271=CARTESIAN_POINT('Ctrl Pts',(-25.8687007298245,14.4928944928021,
129.541467990308)) ;
#143272=CARTESIAN_POINT('Ctrl Pts',(-25.9481227868581,14.4021254320443,
129.80659518902)) ;
#143273=CARTESIAN_POINT('Ctrl Pts',(-26.0165481319324,14.2413769659717,
130.039584245616)) ;
#143274=CARTESIAN_POINT('Ctrl Pts',(-26.0684809468175,14.0210257728375,
130.224528199235)) ;
#143275=CARTESIAN_POINT('Ctrl Pts',(-26.0991009049518,13.7594507578406,
130.346988630004)) ;
#143276=CARTESIAN_POINT('Ctrl Pts',(-26.1058130306325,13.4716752359127,
130.399870698281)) ;
#143277=CARTESIAN_POINT('Ctrl Pts',(-26.0873198572873,13.1827800209618,
130.378837828388)) ;
#143278=CARTESIAN_POINT('Ctrl Pts',(-26.0442075196764,12.9097866027274,
130.286041057869)) ;
#143279=CARTESIAN_POINT('Ctrl Pts',(-25.9789209888468,12.6739760958484,
130.128405961843)) ;
#143280=CARTESIAN_POINT('Ctrl Pts',(-25.8950644284899,12.4911376309814,
129.916641264972)) ;
#143281=CARTESIAN_POINT('Ctrl Pts',(-25.7982306766349,12.375575879239,129.666921135392)) ;
#143282=CARTESIAN_POINT('Ctrl Pts',(-25.6948872153544,12.3352662333604,
129.398091075705)) ;
#143283=CARTESIAN_POINT('Ctrl Pts',(-25.591475557297,12.3722006124299,129.129028993969)) ;
#143284=CARTESIAN_POINT('Ctrl Pts',(-25.4936430630205,12.4858118700224,
128.876611173075)) ;
#143285=CARTESIAN_POINT('Ctrl Pts',(-25.4097931267157,12.6649628036957,
128.664617898589)) ;
#143286=CARTESIAN_POINT('Ctrl Pts',(-25.3434171037584,12.8995424395387,
128.503913243776)) ;
#143287=CARTESIAN_POINT('Ctrl Pts',(-25.2994520917775,13.1707490219764,
128.408538167925)) ;
#143288=CARTESIAN_POINT('Ctrl Pts',(-25.2798667180845,13.4602465795,128.384422935853)) ;
#143289=CARTESIAN_POINT('Ctrl Pts',(-25.2855719032732,13.7479094630808,
128.434283282751)) ;
#143290=CARTESIAN_POINT('Ctrl Pts',(-25.3152873758232,14.0110934234083,
128.554137674801)) ;
#143291=CARTESIAN_POINT('Ctrl Pts',(-25.3662625164448,14.233019589697,128.736189009337)) ;
#143292=CARTESIAN_POINT('Ctrl Pts',(-25.4343591120224,14.3970564643661,
128.968346310512)) ;
#143293=CARTESIAN_POINT('Ctrl Pts',(-25.5132805122452,14.4906411189315,
129.231930680055)) ;
#143294=CARTESIAN_POINT('Ctrl Pts',(-25.5973959591667,14.5080280038905,
129.510833611735)) ;
#143295=CARTESIAN_POINT('Ctrl Pts',(-25.6792022536452,14.4480724922228,
129.782803145259)) ;
#143296=CARTESIAN_POINT('Ctrl Pts',(-25.7531141454623,14.3139469642534,
130.031971871347)) ;
#143297=CARTESIAN_POINT('Ctrl Pts',(-25.8121272678128,14.1169436134283,
130.237401395038)) ;
#143298=CARTESIAN_POINT('Ctrl Pts',(-25.8519851660838,13.8684680278967,
130.387129822211)) ;
#143299=CARTESIAN_POINT('Ctrl Pts',(-25.8685225668081,13.5907241662415,
130.468386340342)) ;
#143300=CARTESIAN_POINT('Ctrl Pts',(-25.8603228056423,13.2994060447749,
130.477583630266)) ;
#143301=CARTESIAN_POINT('Ctrl Pts',(-25.827036095678,13.0173300828137,130.413443066431)) ;
#143302=CARTESIAN_POINT('Ctrl Pts',(-25.7701669280763,12.7634585275692,
130.280523268416)) ;
#143303=CARTESIAN_POINT('Ctrl Pts',(-25.6931351589582,12.5574052301983,
130.088675092408)) ;
#143304=CARTESIAN_POINT('Ctrl Pts',(-25.6014237918118,12.4141337315889,
129.853734516058)) ;
#143305=CARTESIAN_POINT('Ctrl Pts',(-25.4997017590006,12.3422331852162,
129.589762284572)) ;
#143306=CARTESIAN_POINT('Ctrl Pts',(-25.3953738695026,12.3479816705834,
129.318078617136)) ;
#143307=CARTESIAN_POINT('Ctrl Pts',(-25.2947149038502,12.4308509408022,
129.057186959594)) ;
#143308=CARTESIAN_POINT('Ctrl Pts',(-25.2047058731085,12.5841343909331,
128.827278360344)) ;
#143309=CARTESIAN_POINT('Ctrl Pts',(-25.1301965858679,12.7991565720161,
128.642914315101)) ;
#143310=CARTESIAN_POINT('Ctrl Pts',(-25.0769545406197,13.0570001115815,
128.520387169891)) ;
#143311=CARTESIAN_POINT('Ctrl Pts',(-25.0472058635231,13.3421922466227,
128.466652040374)) ;
#143312=CARTESIAN_POINT('Ctrl Pts',(-25.0426624131729,13.6321455836602,
128.486417781107)) ;
#143313=CARTESIAN_POINT('Ctrl Pts',(-25.0629539703241,13.9089726379876,
128.57895542738)) ;
#143314=CARTESIAN_POINT('Ctrl Pts',(-25.1059158440566,14.1498189010042,
128.73760438917)) ;
#143315=CARTESIAN_POINT('Ctrl Pts',(-25.1672896859518,14.3379335627546,
128.949882671248)) ;
#143316=CARTESIAN_POINT('Ctrl Pts',(-25.2427067211349,14.4615825928275,
129.203386921482)) ;
#143317=CARTESIAN_POINT('Ctrl Pts',(-25.3254735430017,14.5104718340286,
129.478271233911)) ;
#143318=CARTESIAN_POINT('Ctrl Pts',(-25.4093890445753,14.4813917007992,
129.756623752072)) ;
#143319=CARTESIAN_POINT('Ctrl Pts',(-25.487125210729,14.376410140061,130.016808097636)) ;
#143320=CARTESIAN_POINT('Ctrl Pts',(-25.5525788833299,14.2041612959408,
130.241003440752)) ;
#143321=CARTESIAN_POINT('Ctrl Pts',(-25.6008773224437,13.974383981629,130.415342708694)) ;
#143322=CARTESIAN_POINT('Ctrl Pts',(-25.6271719709242,13.7063210465707,
130.525219374997)) ;
#143323=CARTESIAN_POINT('Ctrl Pts',(-25.6291300522666,13.4167011729611,
130.56416290139)) ;
#143324=CARTESIAN_POINT('Ctrl Pts',(-25.6058960644918,13.1291677764475,
130.529317082054)) ;
#143325=CARTESIAN_POINT('Ctrl Pts',(-25.5583125907459,12.8617102719658,
130.423460313947)) ;
#143326=CARTESIAN_POINT('Ctrl Pts',(-25.4893078563168,12.6350478347594,
130.254927988591)) ;
#143327=CARTESIAN_POINT('Ctrl Pts',(-25.4024730274085,12.4638699496821,
130.034490107221)) ;
#143328=CARTESIAN_POINT('Ctrl Pts',(-25.3040512171019,12.3621126749229,
129.780067190961)) ;
#143329=CARTESIAN_POINT('Ctrl Pts',(-25.1997380119896,12.336288295009,129.508540465744)) ;
#143330=CARTESIAN_POINT('Ctrl Pts',(-25.0970121081987,12.3882079371413,
129.241501944942)) ;
#143331=CARTESIAN_POINT('Ctrl Pts',(-25.0016211651868,12.5148240574062,
128.996060126096)) ;
#143332=CARTESIAN_POINT('Ctrl Pts',(-24.920756965554,12.7050813508199,128.792787218599)) ;
#143333=CARTESIAN_POINT('Ctrl Pts',(-24.8582697031265,12.9482678416441,
128.64346188212)) ;
#143334=CARTESIAN_POINT('Ctrl Pts',(-24.8187646180453,13.2238579668187,
128.56105516626)) ;
#143335=CARTESIAN_POINT('Ctrl Pts',(-24.803905764497,13.5162934097049,128.550961928654)) ;
#143336=CARTESIAN_POINT('Ctrl Pts',(-24.8142217184009,13.7991654054394,
128.614056451591)) ;
#143337=CARTESIAN_POINT('Ctrl Pts',(-24.848496068521,14.0580269319691,128.747523628204)) ;
#143338=CARTESIAN_POINT('Ctrl Pts',(-24.9028546228909,14.2686029381806,
128.939273431809)) ;
#143339=CARTESIAN_POINT('Ctrl Pts',(-24.9732407127939,14.419961933364,129.178011411683)) ;
#143340=CARTESIAN_POINT('Ctrl Pts',(-25.0537195338019,14.49989585267,129.446209462079)) ;
#143341=CARTESIAN_POINT('Ctrl Pts',(-25.1381655958701,14.5025664525356,
129.726139589141)) ;
#143342=CARTESIAN_POINT('Ctrl Pts',(-25.2188788130462,14.4280651994865,
129.994934028458)) ;
#143343=CARTESIAN_POINT('Ctrl Pts',(-25.2902271151953,14.2819176182956,
130.236459424966)) ;
#143344=CARTESIAN_POINT('Ctrl Pts',(-25.346349360693,14.0723875526179,130.433740928495)) ;
#143345=CARTESIAN_POINT('Ctrl Pts',(-25.3816831121814,13.8191593341655,
130.569884981309)) ;
#143346=CARTESIAN_POINT('Ctrl Pts',(-25.3938278972864,13.5356700868247,
130.638556719779)) ;
#143347=CARTESIAN_POINT('Ctrl Pts',(-25.3808456816373,13.2451624741664,
130.633688514316)) ;
#143348=CARTESIAN_POINT('Ctrl Pts',(-25.3427850618204,12.9658957798679,
130.555749230615)) ;
#143349=CARTESIAN_POINT('Ctrl Pts',(-25.2820224790504,12.7208678253265,
130.41130505217)) ;
#143350=CARTESIAN_POINT('Ctrl Pts',(-25.2019014171005,12.5256177762791,
130.210380825888)) ;
#143351=CARTESIAN_POINT('Ctrl Pts',(-25.1077011701678,12.3947248965929,
129.968261731413)) ;
#143352=CARTESIAN_POINT('Ctrl Pts',(-25.0046214201826,12.3373274071284,
129.700414239671)) ;
#143353=CARTESIAN_POINT('Ctrl Pts',(-24.9009929151909,12.3577351595859,
129.430619982872)) ;
#143354=CARTESIAN_POINT('Ctrl Pts',(-24.8015282893426,12.4546492902735,
129.173300985343)) ;
#143355=CARTESIAN_POINT('Ctrl Pts',(-24.7139128643915,12.6210677035252,
128.950492831251)) ;
#143356=CARTESIAN_POINT('Ctrl Pts',(-24.6434512146242,12.8446767267699,
128.777764271832)) ;
#143357=CARTESIAN_POINT('Ctrl Pts',(-24.5943806100842,13.1088081967542,
128.667427010549)) ;
#143358=CARTESIAN_POINT('Ctrl Pts',(-24.5692555646321,13.3979062800969,
128.627333437601)) ;
#143359=CARTESIAN_POINT('Ctrl Pts',(-24.5695431905959,13.6859097693729,
128.6611363567)) ;
#143360=CARTESIAN_POINT('Ctrl Pts',(-24.594157481065,13.9567565274245,128.766182296297)) ;
#143361=CARTESIAN_POINT('Ctrl Pts',(-24.6411416936085,14.1899349081331,
128.936706868906)) ;
#143362=CARTESIAN_POINT('Ctrl Pts',(-24.7053594546824,14.3662692594446,
129.157216214963)) ;
#143363=CARTESIAN_POINT('Ctrl Pts',(-24.782903699173,14.4768289977238,129.417032620335)) ;
#143364=CARTESIAN_POINT('Ctrl Pts',(-24.866384635766,14.5109207097569,129.694010170453)) ;
#143365=CARTESIAN_POINT('Ctrl Pts',(-24.9494158435752,14.4673589922836,
129.96966777721)) ;
#143366=CARTESIAN_POINT('Ctrl Pts',(-25.0253981397071,14.3490297985362,
130.224741120684)) ;
#143367=CARTESIAN_POINT('Ctrl Pts',(-25.0881434075069,14.1643442277036,
130.441156584524)) ;
#143368=CARTESIAN_POINT('Ctrl Pts',(-25.1323829486443,13.9269540267458,
130.603466456372)) ;
#143369=CARTESIAN_POINT('Ctrl Pts',(-25.1543475264281,13.6529086343547,
130.700783789999)) ;
#143370=CARTESIAN_POINT('Ctrl Pts',(-25.1515873002568,13.3625039506586,
130.725856091348)) ;
#143371=CARTESIAN_POINT('Ctrl Pts',(-25.123624185757,13.0764916582392,130.677299559346)) ;
#143372=CARTESIAN_POINT('Ctrl Pts',(-25.0717015091459,12.8152456791565,
130.558760811629)) ;
#143373=CARTESIAN_POINT('Ctrl Pts',(-24.9988762003653,12.5977359905825,
130.37913851997)) ;
#143374=CARTESIAN_POINT('Ctrl Pts',(-24.9096025778513,12.439230107941,130.151471731367)) ;
#143375=CARTESIAN_POINT('Ctrl Pts',(-24.8094482485441,12.3513755687183,
129.892051831185)) ;
#143376=CARTESIAN_POINT('Ctrl Pts',(-24.7055184930905,12.339931649505,129.621419546249)) ;
#143377=CARTESIAN_POINT('Ctrl Pts',(-24.6026979852918,12.4070555048895,
129.3544642037)) ;
#143378=CARTESIAN_POINT('Ctrl Pts',(-24.510580365153,12.5451371061637,129.118182642952)) ;
#143379=CARTESIAN_POINT('Ctrl Pts',(-24.432124078182,12.7477728516222,128.922258912151)) ;
#143380=CARTESIAN_POINT('Ctrl Pts',(-24.3739511399616,12.9979369346779,
128.785397374143)) ;
#143381=CARTESIAN_POINT('Ctrl Pts',(-24.3388401109884,13.2792373127526,
128.716009070394)) ;
#143382=CARTESIAN_POINT('Ctrl Pts',(-24.3288627638645,13.570158269964,128.719955082171)) ;
#143383=CARTESIAN_POINT('Ctrl Pts',(-24.3438038378766,13.850537969179,128.796691496782)) ;
#143384=CARTESIAN_POINT('Ctrl Pts',(-24.382009729182,14.1007514006134,128.941447794759)) ;
#143385=CARTESIAN_POINT('Ctrl Pts',(-24.4399060508627,14.302171677131,129.143685734349)) ;
#143386=CARTESIAN_POINT('Ctrl Pts',(-24.5128915120813,14.4410638896651,
129.390101505646)) ;
#143387=CARTESIAN_POINT('Ctrl Pts',(-24.5948014466677,14.5064205925433,
129.662568824423)) ;
#143388=CARTESIAN_POINT('Ctrl Pts',(-24.6784736579456,14.4944296430568,
129.939960176772)) ;
#143389=CARTESIAN_POINT('Ctrl Pts',(-24.7583064519586,14.405561123776,130.206367062894)) ;
#143390=CARTESIAN_POINT('Ctrl Pts',(-24.8269294458247,14.2469874685197,
130.439848204688)) ;
#143391=CARTESIAN_POINT('Ctrl Pts',(-24.879425711808,14.0284941679127,130.626407574217)) ;
#143392=CARTESIAN_POINT('Ctrl Pts',(-24.9107857517225,13.7670073728255,
130.751140170549)) ;
#143393=CARTESIAN_POINT('Ctrl Pts',(-24.9181746250829,13.480578033378,130.805889170149)) ;
#143394=CARTESIAN_POINT('Ctrl Pts',(-24.9004718610314,13.1913387346796,
130.787181604797)) ;
#143395=CARTESIAN_POINT('Ctrl Pts',(-24.8579892099205,12.9172330452571,
130.696265791956)) ;
#143396=CARTESIAN_POINT('Ctrl Pts',(-24.7933025062214,12.6799728424888,
130.54038894737)) ;
#143397=CARTESIAN_POINT('Ctrl Pts',(-24.7095184083986,12.4949910313751,
130.328965022333)) ;
#143398=CARTESIAN_POINT('Ctrl Pts',(-24.6137491483049,12.3781840419528,
130.082088557106)) ;
#143399=CARTESIAN_POINT('Ctrl Pts',(-24.5096740314932,12.3352411031327,
129.811395756904)) ;
#143400=CARTESIAN_POINT('Ctrl Pts',(-24.4066670559684,12.3701183951614,
129.543355608262)) ;
#143401=CARTESIAN_POINT('Ctrl Pts',(-24.3084885990164,12.4815908336551,
129.289951677576)) ;
#143402=CARTESIAN_POINT('Ctrl Pts',(-24.2242844198451,12.6586744423265,
129.076874290103)) ;
#143403=CARTESIAN_POINT('Ctrl Pts',(-24.1571513402064,12.8927064520039,
128.914066459456)) ;
#143404=CARTESIAN_POINT('Ctrl Pts',(-24.1127083684764,13.161589606751,128.817110936231)) ;
#143405=CARTESIAN_POINT('Ctrl Pts',(-24.0922448928208,13.452733819126,128.790651846091)) ;
#143406=CARTESIAN_POINT('Ctrl Pts',(-24.0972841912124,13.7397606616034,
128.838449143832)) ;
#143407=CARTESIAN_POINT('Ctrl Pts',(-24.1263977298111,14.0044957325971,
128.95662307499)) ;
#143408=CARTESIAN_POINT('Ctrl Pts',(-24.17672470396,14.2270717509881,129.136685989293)) ;
#143409=CARTESIAN_POINT('Ctrl Pts',(-24.2441033416361,14.3928428929851,
129.366635907636)) ;
#143410=CARTESIAN_POINT('Ctrl Pts',(-24.3234048929595,14.4891680120794,
129.631590444853)) ;
#143411=CARTESIAN_POINT('Ctrl Pts',(-24.4068303427356,14.5086708871169,
129.908215193314)) ;
#143412=CARTESIAN_POINT('Ctrl Pts',(-24.4893464782002,14.4507090768999,
130.182488475895)) ;
#143413=CARTESIAN_POINT('Ctrl Pts',(-24.5633225195788,14.3188233795464,
130.431729758912)) ;
#143414=CARTESIAN_POINT('Ctrl Pts',(-24.6228714288218,14.1234066158898,
130.638750106157)) ;
#143415=CARTESIAN_POINT('Ctrl Pts',(-24.6632253427087,13.8772494948289,
130.789787062655)) ;
#143416=CARTESIAN_POINT('Ctrl Pts',(-24.6806457149312,13.5994496671663,
130.873720819945)) ;
#143417=CARTESIAN_POINT('Ctrl Pts',(-24.6730550166184,13.306728753329,130.884860699526)) ;
#143418=CARTESIAN_POINT('Ctrl Pts',(-24.6405630151421,13.0255130150403,
130.822883930019)) ;
#143419=CARTESIAN_POINT('Ctrl Pts',(-24.5845233822454,12.7708775179562,
130.692326227787)) ;
#143420=CARTESIAN_POINT('Ctrl Pts',(-24.5079734619455,12.5628411654916,
130.50192327057)) ;
#143421=CARTESIAN_POINT('Ctrl Pts',(-24.4164416886935,12.4171763297159,
130.267577824475)) ;
#143422=CARTESIAN_POINT('Ctrl Pts',(-24.3145207569583,12.3431378103405,
130.003142213765)) ;
#143423=CARTESIAN_POINT('Ctrl Pts',(-24.2107870625428,12.346743528454,129.733002482958)) ;
#143424=CARTESIAN_POINT('Ctrl Pts',(-24.1097939762825,12.4272275492429,
129.471168629618)) ;
#143425=CARTESIAN_POINT('Ctrl Pts',(-24.0192589501256,12.5790159402385,
129.23978681913)) ;
#143426=CARTESIAN_POINT('Ctrl Pts',(-23.9444236233476,12.7916689357573,
129.054355997432)) ;
#143427=CARTESIAN_POINT('Ctrl Pts',(-23.8902712760071,13.0498140627792,
128.929343394403)) ;
#143428=CARTESIAN_POINT('Ctrl Pts',(-23.8599875189387,13.3331758335929,
128.873881118229)) ;
#143429=CARTESIAN_POINT('Ctrl Pts',(-23.8546383050908,13.6238936791233,
128.891367979456)) ;
#143430=CARTESIAN_POINT('Ctrl Pts',(-23.8742411013974,13.9010886430072,
128.981854923374)) ;
#143431=CARTESIAN_POINT('Ctrl Pts',(-23.9164786379271,14.1432055625841,
129.138361036176)) ;
#143432=CARTESIAN_POINT('Ctrl Pts',(-23.9778352999634,14.334107077719,129.350811327269)) ;
#143433=CARTESIAN_POINT('Ctrl Pts',(-24.0525075482063,14.4587992015315,
129.601930787677)) ;
#143434=CARTESIAN_POINT('Ctrl Pts',(-24.1351926047194,14.5101605092006,
129.876603495337)) ;
#143435=CARTESIAN_POINT('Ctrl Pts',(-24.2190053195467,14.4834097462587,
130.154588398391)) ;
#143436=CARTESIAN_POINT('Ctrl Pts',(-24.2970658510404,14.3809866888584,
130.415717243842)) ;
#143437=CARTESIAN_POINT('Ctrl Pts',(-24.3633845701292,14.2089571493578,
130.642698748449)) ;
#143438=CARTESIAN_POINT('Ctrl Pts',(-24.4118081071485,13.9828180389134,
130.81707577575)) ;
#143439=CARTESIAN_POINT('Ctrl Pts',(-24.43904614768,13.7132629238328,130.930016793868)) ;
#143440=CARTESIAN_POINT('Ctrl Pts',(-24.4416278169151,13.4258376467274,
130.970551063788)) ;
#143441=CARTESIAN_POINT('Ctrl Pts',(-24.4191648497253,13.1374631126408,
130.938024271275)) ;
#143442=CARTESIAN_POINT('Ctrl Pts',(-24.3722929118948,12.8691197020598,
130.834231842167)) ;
#143443=CARTESIAN_POINT('Ctrl Pts',(-24.3035253027477,12.6403113391648,
130.666529496578)) ;
#143444=CARTESIAN_POINT('Ctrl Pts',(-24.2177440216527,12.4684206936737,
130.448931894944)) ;
#143445=CARTESIAN_POINT('Ctrl Pts',(-24.1189641371196,12.3638000131135,
130.193681090473)) ;
#143446=CARTESIAN_POINT('Ctrl Pts',(-24.0152577190491,12.3359859149595,
129.923747869451)) ;
#143447=CARTESIAN_POINT('Ctrl Pts',(-23.9122225721519,12.3855342860159,
129.655866294705)) ;
#143448=CARTESIAN_POINT('Ctrl Pts',(-23.8167044562249,12.5097023553619,
129.409976684742)) ;
#143449=CARTESIAN_POINT('Ctrl Pts',(-23.7350415696029,12.6987170593864,
129.204483050259)) ;
#143450=CARTESIAN_POINT('Ctrl Pts',(-23.6718214474125,12.9413959891016,
129.053102247864)) ;
#143451=CARTESIAN_POINT('Ctrl Pts',(-23.6317266635016,13.2164085190981,
128.968979209855)) ;
#143452=CARTESIAN_POINT('Ctrl Pts',(-23.6161846853452,13.5077477594262,
128.956775771091)) ;
#143453=CARTESIAN_POINT('Ctrl Pts',(-23.6258623623192,13.7917086517815,
129.018086560944)) ;
#143454=CARTESIAN_POINT('Ctrl Pts',(-23.6591748256657,14.0497091065288,
129.148483877937)) ;
#143455=CARTESIAN_POINT('Ctrl Pts',(-23.7131536163967,14.2632251224131,
129.339292961049)) ;
#143456=CARTESIAN_POINT('Ctrl Pts',(-23.7834103537624,14.4168538521645,
129.577752440174)) ;
#143457=CARTESIAN_POINT('Ctrl Pts',(-23.8637812419505,14.498759930122,129.845665495601)) ;
#143458=CARTESIAN_POINT('Ctrl Pts',(-23.9479867757916,14.5035045472666,
130.124804508874)) ;
#143459=CARTESIAN_POINT('Ctrl Pts',(-24.0289297957099,14.4313229189066,
130.394277457633)) ;
#143460=CARTESIAN_POINT('Ctrl Pts',(-24.1008459108954,14.2860965422893,
130.63760203165)) ;
#143461=CARTESIAN_POINT('Ctrl Pts',(-24.1568860900922,14.0806886832094,
130.834254572376)) ;
#143462=CARTESIAN_POINT('Ctrl Pts',(-24.1932719079745,13.8265803466444,
130.973763090983)) ;
#143463=CARTESIAN_POINT('Ctrl Pts',(-24.2060319927351,13.5441877343299,
131.044150934557)) ;
#143464=CARTESIAN_POINT('Ctrl Pts',(-24.1937444777174,13.2530368711715,
131.041386093533)) ;
#143465=CARTESIAN_POINT('Ctrl Pts',(-24.1565222164124,12.9741112441056,
130.965772544337)) ;
#143466=CARTESIAN_POINT('Ctrl Pts',(-24.0962637236049,12.727211784615,130.82288513937)) ;
#143467=CARTESIAN_POINT('Ctrl Pts',(-24.0167199464712,12.5305676715835,
130.623604426394)) ;
#143468=CARTESIAN_POINT('Ctrl Pts',(-23.9228649380525,12.3976028269524,
130.382495884254)) ;
#143469=CARTESIAN_POINT('Ctrl Pts',(-23.8200059844747,12.3378877483635,
130.115269742189)) ;
#143470=CARTESIAN_POINT('Ctrl Pts',(-23.7161313122626,12.3561146706411,
129.844822206421)) ;
#143471=CARTESIAN_POINT('Ctrl Pts',(-23.6167274273655,12.4504996571453,
129.58757336973)) ;
#143472=CARTESIAN_POINT('Ctrl Pts',(-23.5285438481367,12.6151918757671,
129.363160504632)) ;
#143473=CARTESIAN_POINT('Ctrl Pts',(-23.4575504842079,12.8367628546182,
129.188815787231)) ;
#143474=CARTESIAN_POINT('Ctrl Pts',(-23.4074694454012,13.1024713310692,
129.075832540994)) ;
#143475=CARTESIAN_POINT('Ctrl Pts',(-23.3819286365241,13.3880985112024,
129.034157042022)) ;
#143476=CARTESIAN_POINT('Ctrl Pts',(-23.3813836420094,13.6786302833929,
129.065792225384)) ;
#143477=CARTESIAN_POINT('Ctrl Pts',(-23.4054139281742,13.9495118102634,
129.169053182591)) ;
#143478=CARTESIAN_POINT('Ctrl Pts',(-23.4515197088819,14.1831630718956,
129.33686405637)) ;
#143479=CARTESIAN_POINT('Ctrl Pts',(-23.5155530868319,14.3622887223182,
129.556989419024)) ;
#143480=CARTESIAN_POINT('Ctrl Pts',(-23.5929622025893,14.4748192512671,
129.816455245563)) ;
#143481=CARTESIAN_POINT('Ctrl Pts',(-23.6760665889331,14.5109473635331,
130.092219650908)) ;
#143482=CARTESIAN_POINT('Ctrl Pts',(-23.7591142385176,14.4698938664046,
130.367885685175)) ;
#143483=CARTESIAN_POINT('Ctrl Pts',(-23.8354983853783,14.3536144682459,
130.62417280819)) ;
#143484=CARTESIAN_POINT('Ctrl Pts',(-23.8987831172299,14.1706211200802,
130.84218781578)) ;
#143485=CARTESIAN_POINT('Ctrl Pts',(-23.9436890861957,13.9337365390504,
131.0065426473)) ;
#143486=CARTESIAN_POINT('Ctrl Pts',(-23.9662439925048,13.6617103922721,
131.105431657837)) ;
#143487=CARTESIAN_POINT('Ctrl Pts',(-23.9642309252639,13.3701431433412,
131.132842985535)) ;
#143488=CARTESIAN_POINT('Ctrl Pts',(-23.936880730123,13.0839500606497,131.086055779472)) ;
#143489=CARTESIAN_POINT('Ctrl Pts',(-23.8858072445162,12.8226368169183,
130.969880672048)) ;
#143490=CARTESIAN_POINT('Ctrl Pts',(-23.8135792178995,12.603615233857,130.791996666625)) ;
#143491=CARTESIAN_POINT('Ctrl Pts',(-23.7249031771877,12.443223881209,130.566020018471)) ;
#143492=CARTESIAN_POINT('Ctrl Pts',(-23.6243834508961,12.3525997217998,
130.305729187183)) ;
#143493=CARTESIAN_POINT('Ctrl Pts',(-23.5206245740586,12.339390379435,130.035551590509)) ;
#143494=CARTESIAN_POINT('Ctrl Pts',(-23.4183108359919,12.4034681613504,
129.769849164582)) ;
#143495=CARTESIAN_POINT('Ctrl Pts',(-23.3250195012801,12.5405073209883,
129.530418794464)) ;
#143496=CARTESIAN_POINT('Ctrl Pts',(-23.246128657495,12.742000710491,129.333241435513)) ;
#143497=CARTESIAN_POINT('Ctrl Pts',(-23.1875710322953,12.9900803066021,
129.195131588516)) ;
#143498=CARTESIAN_POINT('Ctrl Pts',(-23.1517255791024,13.2708160842573,
129.123605670452)) ;
#143499=CARTESIAN_POINT('Ctrl Pts',(-23.1410164930884,13.5613606280666,
129.125372551299)) ;
#143500=CARTESIAN_POINT('Ctrl Pts',(-23.1552114470279,13.8428562082264,
129.199981132927)) ;
#143501=CARTESIAN_POINT('Ctrl Pts',(-23.1930535350395,14.0951248182504,
129.343821332079)) ;
#143502=CARTESIAN_POINT('Ctrl Pts',(-23.2501057955293,14.2968155376203,
129.543381940502)) ;
#143503=CARTESIAN_POINT('Ctrl Pts',(-23.3229353073403,14.4382063534547,
129.789446101916)) ;
#143504=CARTESIAN_POINT('Ctrl Pts',(-23.404500721367,14.5055714123115,130.060826591937)) ;
#143505=CARTESIAN_POINT('Ctrl Pts',(-23.4883253092773,14.4957941615493,
130.338720063012)) ;
#143506=CARTESIAN_POINT('Ctrl Pts',(-23.5681456294195,14.4095661599452,
130.604978527462)) ;
#143507=CARTESIAN_POINT('Ctrl Pts',(-23.6377229031392,14.2515334104405,
130.841522721531)) ;
#143508=CARTESIAN_POINT('Ctrl Pts',(-23.6904929025794,14.0347235705321,
131.028791977006)) ;
#143509=CARTESIAN_POINT('Ctrl Pts',(-23.722380178782,13.7751698912538,131.154951237933)) ;
#143510=CARTESIAN_POINT('Ctrl Pts',(-23.7305596953239,13.489554992756,131.211966965207)) ;
#143511=CARTESIAN_POINT('Ctrl Pts',(-23.7134857949628,13.1989623651925,
131.195236364621)) ;
#143512=CARTESIAN_POINT('Ctrl Pts',(-23.6717605104891,12.9245155111551,
131.106471534992)) ;
#143513=CARTESIAN_POINT('Ctrl Pts',(-23.607204735429,12.6850931696754,130.951153837753)) ;
#143514=CARTESIAN_POINT('Ctrl Pts',(-23.5251058801955,12.5007200280461,
130.744179233861)) ;
#143515=CARTESIAN_POINT('Ctrl Pts',(-23.4285456899501,12.3802347954754,
130.495393086658)) ;
#143516=CARTESIAN_POINT('Ctrl Pts',(-23.3255044334404,12.3354177836866,
130.227408711233)) ;
#143517=CARTESIAN_POINT('Ctrl Pts',(-23.2214527235259,12.3682931667049,
129.956637199255)) ;
#143518=CARTESIAN_POINT('Ctrl Pts',(-23.1240214979293,12.4764500212594,
129.705052803222)) ;
#143519=CARTESIAN_POINT('Ctrl Pts',(-23.0386731819847,12.6527561710341,
129.488891430682)) ;
#143520=CARTESIAN_POINT('Ctrl Pts',(-22.9712446345339,12.8841372623909,
129.325039080064)) ;
#143521=CARTESIAN_POINT('Ctrl Pts',(-22.9256685603981,13.1550291138396,
129.225129396424)) ;
#143522=CARTESIAN_POINT('Ctrl Pts',(-22.9047424564583,13.4437302446049,
129.197053986198)) ;
#143523=CARTESIAN_POINT('Ctrl Pts',(-22.9090153289593,13.7319393210826,
129.242714369187)) ;
#143524=CARTESIAN_POINT('Ctrl Pts',(-22.9373439751867,13.996548190544,129.358457399253)) ;
#143525=CARTESIAN_POINT('Ctrl Pts',(-22.9872072567607,14.2215298509627,
129.537280491404)) ;
#143526=CARTESIAN_POINT('Ctrl Pts',(-23.0543476264601,14.38914835891,129.76659166035)) ;
#143527=CARTESIAN_POINT('Ctrl Pts',(-23.132867941208,14.4871687209254,130.029047170173)) ;
#143528=CARTESIAN_POINT('Ctrl Pts',(-23.2167986272204,14.5093408038881,
130.307369504363)) ;
#143529=CARTESIAN_POINT('Ctrl Pts',(-23.2994992889762,14.4530254210031,
130.582212420233)) ;
#143530=CARTESIAN_POINT('Ctrl Pts',(-23.3734144406411,14.3240304850431,
130.831087779391)) ;
#143531=CARTESIAN_POINT('Ctrl Pts',(-23.4337726380514,14.1290978573837,
131.040670220681)) ;
#143532=CARTESIAN_POINT('Ctrl Pts',(-23.4745345852949,13.8855602682148,
131.192702691882)) ;
#143533=CARTESIAN_POINT('Ctrl Pts',(-23.4927384577347,13.605841493294,131.279235002887)) ;
#143534=CARTESIAN_POINT('Ctrl Pts',(-23.4858621472011,13.3160019490386,
131.292133100213)) ;
#143535=CARTESIAN_POINT('Ctrl Pts',(-23.4540121299607,13.0326884812318,
131.232212628337)) ;
#143536=CARTESIAN_POINT('Ctrl Pts',(-23.3983642412574,12.7766370515925,
131.102864082558)) ;
#143537=CARTESIAN_POINT('Ctrl Pts',(-23.3224252508295,12.5676696843858,
130.914179013247)) ;
#143538=CARTESIAN_POINT('Ctrl Pts',(-23.2315623998387,12.4206516952527,
130.681675995429)) ;
#143539=CARTESIAN_POINT('Ctrl Pts',(-23.1301738864212,12.34431502245,130.418692826269)) ;
#143540=CARTESIAN_POINT('Ctrl Pts',(-23.0259203389995,12.345456773331,130.147196189081)) ;
#143541=CARTESIAN_POINT('Ctrl Pts',(-22.9245983595864,12.4241540990105,
129.884450538708)) ;
#143542=CARTESIAN_POINT('Ctrl Pts',(-22.8339604250744,12.5736455946733,
129.652673423447)) ;
#143543=CARTESIAN_POINT('Ctrl Pts',(-22.7586463627445,12.7844245874558,
129.465809714269)) ;
#143544=CARTESIAN_POINT('Ctrl Pts',(-22.7038116606386,13.0412646550238,
129.338784714396)) ;
#143545=CARTESIAN_POINT('Ctrl Pts',(-22.672696634036,13.3250315602578,129.280999683653)) ;
#143546=CARTESIAN_POINT('Ctrl Pts',(-22.6666782489099,13.615649410723,129.296509723596)) ;
#143547=CARTESIAN_POINT('Ctrl Pts',(-22.6854869927878,13.8929004143671,
129.384593069969)) ;
#143548=CARTESIAN_POINT('Ctrl Pts',(-22.7271490627597,14.1366367418866,
129.53946593282)) ;
#143549=CARTESIAN_POINT('Ctrl Pts',(-22.7877716926247,14.3287834464846,
129.749659518345)) ;
#143550=CARTESIAN_POINT('Ctrl Pts',(-22.8624217458546,14.4563288635319,
130.000862719859)) ;
#143551=CARTESIAN_POINT('Ctrl Pts',(-22.9451469435644,14.5097636487804,
130.275713031449)) ;
#143552=CARTESIAN_POINT('Ctrl Pts',(-23.0287793650505,14.4852491667338,
130.553077224357)) ;
#143553=CARTESIAN_POINT('Ctrl Pts',(-23.1070274154926,14.3852131560936,
130.814719834429)) ;
#143554=CARTESIAN_POINT('Ctrl Pts',(-23.1739124562573,14.2148994142931,
131.043403108811)) ;
#143555=CARTESIAN_POINT('Ctrl Pts',(-23.2229394678138,13.9895604970269,
131.219613593883)) ;
#143556=CARTESIAN_POINT('Ctrl Pts',(-23.2507366610269,13.722649621575,131.333978244755)) ;
#143557=CARTESIAN_POINT('Ctrl Pts',(-23.2541372508295,13.4342098870415,
131.377066913897)) ;
#143558=CARTESIAN_POINT('Ctrl Pts',(-23.2324178885211,13.145818281647,131.346673514171)) ;
#143559=CARTESIAN_POINT('Ctrl Pts',(-23.1860426545478,12.8759127187507,
131.244432599894)) ;
#143560=CARTESIAN_POINT('Ctrl Pts',(-23.1182744949016,12.646886857505,131.079457250169)) ;
#143561=CARTESIAN_POINT('Ctrl Pts',(-23.0324041722189,12.4721832267463,
130.861807119644)) ;
#143562=CARTESIAN_POINT('Ctrl Pts',(-22.9347158667363,12.3661739230268,
130.609463902656)) ;
#143563=CARTESIAN_POINT('Ctrl Pts',(-22.8302237560895,12.3355863381279,
130.337518479939)) ;
#143564=CARTESIAN_POINT('Ctrl Pts',(-22.7272957874238,12.383119877217,130.06987449926)) ;
#143565=CARTESIAN_POINT('Ctrl Pts',(-22.6313718290583,12.5053833335783,
129.822838291288)) ;
#143566=CARTESIAN_POINT('Ctrl Pts',(-22.549444806847,12.6923271245218,129.616496226826)) ;
#143567=CARTESIAN_POINT('Ctrl Pts',(-22.4855769767943,12.933586655108,129.46321823843)) ;
#143568=CARTESIAN_POINT('Ctrl Pts',(-22.4447201723286,13.2085815637178,
129.376950905108)) ;
#143569=CARTESIAN_POINT('Ctrl Pts',(-22.428506211567,13.499055887524,129.362699996165)) ;
#143570=CARTESIAN_POINT('Ctrl Pts',(-22.4374411004653,13.7836908824952,
129.421864605484)) ;
#143571=CARTESIAN_POINT('Ctrl Pts',(-22.4701043315475,14.0427282723312,
129.550363332339)) ;
#143572=CARTESIAN_POINT('Ctrl Pts',(-22.5235419982417,14.2577310864089,
129.73959019157)) ;
#143573=CARTESIAN_POINT('Ctrl Pts',(-22.5932633108271,14.4131665395365,
129.976425920683)) ;
#143574=CARTESIAN_POINT('Ctrl Pts',(-22.6735795483315,14.4973756020118,
130.244248302139)) ;
#143575=CARTESIAN_POINT('Ctrl Pts',(-22.7573477862148,14.5046723914937,
130.521938057957)) ;
#143576=CARTESIAN_POINT('Ctrl Pts',(-22.8390722337888,14.4343110972272,
130.793939994731)) ;
#143577=CARTESIAN_POINT('Ctrl Pts',(-22.9110884796083,14.2913902739099,
131.037440280102)) ;
#143578=CARTESIAN_POINT('Ctrl Pts',(-22.9677500828963,14.0872938687907,
131.235968489753)) ;
#143579=CARTESIAN_POINT('Ctrl Pts',(-23.0047032783507,13.8349905737135,
131.377045531599)) ;
#143580=CARTESIAN_POINT('Ctrl Pts',(-23.0182429611947,13.5522016078203,
131.449828390998)) ;
#143581=CARTESIAN_POINT('Ctrl Pts',(-23.0066529011385,13.261176925901,131.449077872334)) ;
#143582=CARTESIAN_POINT('Ctrl Pts',(-22.9700608928401,12.9814105366867,
131.375336701068)) ;
#143583=CARTESIAN_POINT('Ctrl Pts',(-22.9106223405697,12.7341368123324,
131.234734753748)) ;
#143584=CARTESIAN_POINT('Ctrl Pts',(-22.831420465707,12.5351661127334,131.036536297695)) ;
#143585=CARTESIAN_POINT('Ctrl Pts',(-22.7374700882341,12.4000170335594,
130.795280878613)) ;
#143586=CARTESIAN_POINT('Ctrl Pts',(-22.6352599088003,12.3385940998212,
130.529783876629)) ;
#143587=CARTESIAN_POINT('Ctrl Pts',(-22.5311701984334,12.3545286959988,
130.258765286088)) ;
#143588=CARTESIAN_POINT('Ctrl Pts',(-22.4314837094175,12.4469846985816,
130.000709234555)) ;
#143589=CARTESIAN_POINT('Ctrl Pts',(-22.3428054266133,12.6102580102747,
129.774900451722)) ;
#143590=CARTESIAN_POINT('Ctrl Pts',(-22.2716044309603,12.8296978065605,
129.599824238354)) ;
#143591=CARTESIAN_POINT('Ctrl Pts',(-22.220982217263,13.0929764235486,129.485098106775)) ;
#143592=CARTESIAN_POINT('Ctrl Pts',(-22.1944879827316,13.3798715648176,
129.440832558787)) ;
#143593=CARTESIAN_POINT('Ctrl Pts',(-22.1932838176779,13.6705227890218,
129.47053097622)) ;
#143594=CARTESIAN_POINT('Ctrl Pts',(-22.216586984954,13.9421700624616,129.571656651199)) ;
#143595=CARTESIAN_POINT('Ctrl Pts',(-22.2623594128797,14.1780191075409,
129.738634100291)) ;
#143596=CARTESIAN_POINT('Ctrl Pts',(-22.3257673108184,14.3579768131381,
129.956807935287)) ;
#143597=CARTESIAN_POINT('Ctrl Pts',(-22.402693163682,14.4725057536027,130.214788867147)) ;
#143598=CARTESIAN_POINT('Ctrl Pts',(-22.4858525447118,14.5110248787741,
130.490773806693)) ;
#143599=CARTESIAN_POINT('Ctrl Pts',(-22.5690583642843,14.4721191985818,
130.766923866594)) ;
#143600=CARTESIAN_POINT('Ctrl Pts',(-22.6457431338845,14.3577454334386,
131.024102564944)) ;
#143601=CARTESIAN_POINT('Ctrl Pts',(-22.709285526216,14.1770688600788,131.242769537148)) ;
#143602=CARTESIAN_POINT('Ctrl Pts',(-22.7548684342017,13.9416997135302,
131.409099612895)) ;
#143603=CARTESIAN_POINT('Ctrl Pts',(-22.7781477410586,13.6694103999149,
131.510228280328)) ;
#143604=CARTESIAN_POINT('Ctrl Pts',(-22.7768870761297,13.3798585419127,
131.539630839804)) ;
#143605=CARTESIAN_POINT('Ctrl Pts',(-22.750382745593,13.0927639720694,131.495363128211)) ;
#143606=CARTESIAN_POINT('Ctrl Pts',(-22.6997687083182,12.8294541996799,
131.380657407185)) ;
#143607=CARTESIAN_POINT('Ctrl Pts',(-22.6280842619235,12.6090079342562,
131.204355845863)) ;
#143608=CARTESIAN_POINT('Ctrl Pts',(-22.5396228094031,12.4466659033485,
130.979064335721)) ;
#143609=CARTESIAN_POINT('Ctrl Pts',(-22.4399385081326,12.3544265083851,
130.7210134408)) ;
#143610=CARTESIAN_POINT('Ctrl Pts',(-22.3359884293059,12.338485561048,130.450351932456)) ;
#143611=CARTESIAN_POINT('Ctrl Pts',(-22.2329622684113,12.4009576642386,
130.182750802671)) ;
#143612=CARTESIAN_POINT('Ctrl Pts',(-22.1398337600932,12.5356623711056,
129.943638898752)) ;
#143613=CARTESIAN_POINT('Ctrl Pts',(-22.0607017790479,12.7342794409358,
129.745607566337)) ;
#143614=CARTESIAN_POINT('Ctrl Pts',(-22.0011596910477,12.9822472239535,
129.604781893021)) ;
#143615=CARTESIAN_POINT('Ctrl Pts',(-21.9646063758927,13.2626106306711,
129.531211763355)) ;
#143616=CARTESIAN_POINT('Ctrl Pts',(-21.9531801864884,13.5537332478673,
129.530951535747)) ;
#143617=CARTESIAN_POINT('Ctrl Pts',(-21.9667343017209,13.835078244523,129.603615881096)) ;
#143618=CARTESIAN_POINT('Ctrl Pts',(-22.0036132721382,14.0872564093589,
129.744451692133)) ;
#143619=CARTESIAN_POINT('Ctrl Pts',(-22.0605479104735,14.2922554026262,
129.943923349653)) ;
#143620=CARTESIAN_POINT('Ctrl Pts',(-22.1328947465888,14.4349646687422,
130.18849153958)) ;
#143621=CARTESIAN_POINT('Ctrl Pts',(-22.213936585761,14.50455407939,130.458214816929)) ;
#143622=CARTESIAN_POINT('Ctrl Pts',(-22.2981099146983,14.4973581073499,
130.737249362425)) ;
#143623=CARTESIAN_POINT('Ctrl Pts',(-22.3784072001466,14.4126016063702,
131.0050273077)) ;
#143624=CARTESIAN_POINT('Ctrl Pts',(-22.447805875919,14.2578369760295,131.240771109956)) ;
#143625=CARTESIAN_POINT('Ctrl Pts',(-22.5013649795716,14.0423605049128,
131.430430107999)) ;
#143626=CARTESIAN_POINT('Ctrl Pts',(-22.534006961752,13.7833429469769,131.558854833022)) ;
#143627=CARTESIAN_POINT('Ctrl Pts',(-22.5428671924125,13.4972453189194,
131.617966841361)) ;
#143628=CARTESIAN_POINT('Ctrl Pts',(-22.5265920281103,13.2077136867894,
131.603426053842)) ;
#143629=CARTESIAN_POINT('Ctrl Pts',(-22.4854531315834,12.9318530296234,
131.516461855721)) ;
#143630=CARTESIAN_POINT('Ctrl Pts',(-22.4218868621433,12.6922551548189,
131.363858154752)) ;
#143631=CARTESIAN_POINT('Ctrl Pts',(-22.339699493421,12.5046664561304,131.156866750708)) ;
#143632=CARTESIAN_POINT('Ctrl Pts',(-22.2434112650807,12.3825157092279,
130.908862326724)) ;
#143633=CARTESIAN_POINT('Ctrl Pts',(-22.1407022451927,12.3357140446238,
130.641782038687)) ;
#143634=CARTESIAN_POINT('Ctrl Pts',(-22.0367950143925,12.36606795923,130.371356157515)) ;
#143635=CARTESIAN_POINT('Ctrl Pts',(-21.9385800776849,12.4727573842292,
130.117660335976)) ;
#143636=CARTESIAN_POINT('Ctrl Pts',(-21.8530384367553,12.6471452972706,
129.900859802065)) ;
#143637=CARTESIAN_POINT('Ctrl Pts',(-21.7851981669221,12.8766362128536,
129.735734315131)) ;
#143638=CARTESIAN_POINT('Ctrl Pts',(-21.738959998301,13.1457609498557,129.633791333078)) ;
#143639=CARTESIAN_POINT('Ctrl Pts',(-21.7171693051141,13.4362085163513,
129.603423986028)) ;
#143640=CARTESIAN_POINT('Ctrl Pts',(-21.7207505372234,13.7232902090159,
129.646893616354)) ;
#143641=CARTESIAN_POINT('Ctrl Pts',(-21.7484265203704,13.9896012437994,
129.760821659193)) ;
#143642=CARTESIAN_POINT('Ctrl Pts',(-21.7977851645391,14.215929645434,129.938174798434)) ;
#143643=CARTESIAN_POINT('Ctrl Pts',(-21.8643742193588,14.3851342373848,
130.165817724569)) ;
#143644=CARTESIAN_POINT('Ctrl Pts',(-21.9427712554755,14.4854517125692,
130.42796572971)) ;
#143645=CARTESIAN_POINT('Ctrl Pts',(-22.0264764252796,14.5096986582257,
130.705565676572)) ;
#143646=CARTESIAN_POINT('Ctrl Pts',(-22.1091205178272,14.4561737442075,
130.980149885645)) ;
#143647=CARTESIAN_POINT('Ctrl Pts',(-22.1838332613068,14.3282784828902,
131.231578468129)) ;
#143648=CARTESIAN_POINT('Ctrl Pts',(-22.2443137255644,14.1363002885468,
131.441301018419)) ;
#143649=CARTESIAN_POINT('Ctrl Pts',(-22.2859518160171,13.8924838529507,
131.596109073872)) ;
#143650=CARTESIAN_POINT('Ctrl Pts',(-22.3047209382812,13.6154600840217,
131.684045645423)) ;
#143651=CARTESIAN_POINT('Ctrl Pts',(-22.2986702811419,13.3244464776438,
131.699506421331)) ;
#143652=CARTESIAN_POINT('Ctrl Pts',(-22.2674859080266,13.0407280398606,
131.641518038007)) ;
#143653=CARTESIAN_POINT('Ctrl Pts',(-22.2127203231953,12.7843964023836,
131.514637915739)) ;
#143654=CARTESIAN_POINT('Ctrl Pts',(-22.137398507186,12.5734337589229,131.327764159491)) ;
#143655=CARTESIAN_POINT('Ctrl Pts',(-22.0463241028875,12.4236458719393,
131.094850745407)) ;
#143656=CARTESIAN_POINT('Ctrl Pts',(-21.9456019274968,12.3455712337427,
130.833653818815)) ;
#143657=CARTESIAN_POINT('Ctrl Pts',(-21.8410149058486,12.3443023954149,
130.561292129649)) ;
#143658=CARTESIAN_POINT('Ctrl Pts',(-21.7395756953206,12.4209332624995,
130.298180683002)) ;
#143659=CARTESIAN_POINT('Ctrl Pts',(-21.6485359377366,12.5684898191716,
130.065238668739)) ;
#143660=CARTESIAN_POINT('Ctrl Pts',(-21.5725277270908,12.7783873972307,
129.876435053139)) ;
#143661=CARTESIAN_POINT('Ctrl Pts',(-21.5172012263658,13.0341437387016,
129.747950001213)) ;
#143662=CARTESIAN_POINT('Ctrl Pts',(-21.4855037051697,13.3161554584295,
129.68831963719)) ;
#143663=CARTESIAN_POINT('Ctrl Pts',(-21.4786823629391,13.6077103928711,
129.701579568902)) ;
#143664=CARTESIAN_POINT('Ctrl Pts',(-21.4969471387102,13.8863968339185,
129.78817190297)) ;
#143665=CARTESIAN_POINT('Ctrl Pts',(-21.5380140006036,14.1306964208414,
129.941243579544)) ;
#143666=CARTESIAN_POINT('Ctrl Pts',(-21.597955468829,14.3238933798465,130.14933977895)) ;
#143667=CARTESIAN_POINT('Ctrl Pts',(-21.6722368019592,14.4535138148578,
130.399455722399)) ;
#143668=CARTESIAN_POINT('Ctrl Pts',(-21.7548431705078,14.5094099207336,
130.673967122569)) ;
#143669=CARTESIAN_POINT('Ctrl Pts',(-21.8390074433957,14.4867701490887,
130.953075016823)) ;
#143670=CARTESIAN_POINT('Ctrl Pts',(-21.9170393419491,14.3890643501402,
131.213907369447)) ;
#143671=CARTESIAN_POINT('Ctrl Pts',(-21.9843219419799,14.2211868758739,
131.443700982914)) ;
#143672=CARTESIAN_POINT('Ctrl Pts',(-22.034145358508,13.9958857732727,131.622425454293)) ;
#143673=CARTESIAN_POINT('Ctrl Pts',(-22.0624108594708,13.731479333369,131.737954309001)) ;
#143674=CARTESIAN_POINT('Ctrl Pts',(-22.0666539748557,13.44236393195,131.783625544948)) ;
#143675=CARTESIAN_POINT('Ctrl Pts',(-22.0454519447672,13.1530743208287,
131.754824233389)) ;
#143676=CARTESIAN_POINT('Ctrl Pts',(-22.0001608256054,12.884256615766,131.655497903819)) ;
#143677=CARTESIAN_POINT('Ctrl Pts',(-21.9324437444424,12.6519995409111,
131.490940272545)) ;
#143678=CARTESIAN_POINT('Ctrl Pts',(-21.8474698625417,12.4766942451725,
131.275709117702)) ;
#143679=CARTESIAN_POINT('Ctrl Pts',(-21.7498528975863,12.3681120664589,
131.023656849795)) ;
#143680=CARTESIAN_POINT('Ctrl Pts',(-21.6453559537401,12.3353450088633,
130.751717635271)) ;
#143681=CARTESIAN_POINT('Ctrl Pts',(-21.542236103773,12.380878936013,130.483543962322)) ;
#143682=CARTESIAN_POINT('Ctrl Pts',(-21.4463295322367,12.5006496945069,
130.236443567169)) ;
#143683=CARTESIAN_POINT('Ctrl Pts',(-21.3637539981775,12.6862349323656,
130.028280312864)) ;
#143684=CARTESIAN_POINT('Ctrl Pts',(-21.2995009859174,12.9253055935091,
129.873754351436)) ;
#143685=CARTESIAN_POINT('Ctrl Pts',(-21.2578359992807,13.1996775352275,
129.785155353514)) ;
#143686=CARTESIAN_POINT('Ctrl Pts',(-21.2408217231033,13.4900584277301,
129.768572274844)) ;
#143687=CARTESIAN_POINT('Ctrl Pts',(-21.2490712614427,13.7765695978382,
129.825896978974)) ;
#143688=CARTESIAN_POINT('Ctrl Pts',(-21.2812883123373,14.036835781509,129.953150444439)) ;
#143689=CARTESIAN_POINT('Ctrl Pts',(-21.3339524991672,14.2522895995138,
130.139959179499)) ;
#143690=CARTESIAN_POINT('Ctrl Pts',(-21.4036007042656,14.410142724822,130.376724923373)) ;
#143691=CARTESIAN_POINT('Ctrl Pts',(-21.4833190971745,14.4959011671627,
130.642629699404)) ;
#143692=CARTESIAN_POINT('Ctrl Pts',(-21.5672364300302,14.5055615409164,
130.920826895733)) ;
#143693=CARTESIAN_POINT('Ctrl Pts',(-21.6489772963134,14.4373878436055,
131.192815585546)) ;
#143694=CARTESIAN_POINT('Ctrl Pts',(-21.721303833013,14.2968054840673,131.437185325856)) ;
#143695=CARTESIAN_POINT('Ctrl Pts',(-21.7787209509657,14.0934338457394,
131.63806052176)) ;
#143696=CARTESIAN_POINT('Ctrl Pts',(-21.8161626773945,13.8423636115969,
131.780529628432)) ;
#143697=CARTESIAN_POINT('Ctrl Pts',(-21.8304120659341,13.5615575056706,
131.855225921439)) ;
#143698=CARTESIAN_POINT('Ctrl Pts',(-21.8195551963924,13.2694346825445,
131.85674250842)) ;
#143699=CARTESIAN_POINT('Ctrl Pts',(-21.7837797080597,12.9897645897098,
131.785295359872)) ;
#143700=CARTESIAN_POINT('Ctrl Pts',(-21.7247880088678,12.7403850896867,
131.646117143433)) ;
#143701=CARTESIAN_POINT('Ctrl Pts',(-21.6461522200936,12.5401777346667,
131.449526068275)) ;
#143702=CARTESIAN_POINT('Ctrl Pts',(-21.552843515609,12.403253810304,131.2100513829)) ;
#143703=CARTESIAN_POINT('Ctrl Pts',(-21.4506728701617,12.3392654629647,
130.944714192732)) ;
#143704=CARTESIAN_POINT('Ctrl Pts',(-21.3462630111135,12.3529796001613,
130.672847368747)) ;
#143705=CARTESIAN_POINT('Ctrl Pts',(-21.2464552737874,12.4434150313968,
130.414411901)) ;
#143706=CARTESIAN_POINT('Ctrl Pts',(-21.1576935500326,12.6038143238447,
130.188212603758)) ;
#143707=CARTESIAN_POINT('Ctrl Pts',(-21.0854169254923,12.8232747601352,
130.010229428693)) ;
#143708=CARTESIAN_POINT('Ctrl Pts',(-21.0343721327219,13.0848674968843,
129.894160674788)) ;
#143709=CARTESIAN_POINT('Ctrl Pts',(-21.0071238887452,13.3712341167296,
129.847685621154)) ;
#143710=CARTESIAN_POINT('Ctrl Pts',(-21.0051604192748,13.662067069188,129.875157873121)) ;
#143711=CARTESIAN_POINT('Ctrl Pts',(-21.0278323583826,13.9347879566426,
129.974482349287)) ;
#143712=CARTESIAN_POINT('Ctrl Pts',(-21.0727651018897,14.1711547211457,
130.138867819652)) ;
#143713=CARTESIAN_POINT('Ctrl Pts',(-21.1360453755805,14.3538986016763,
130.356852241416)) ;
#143714=CARTESIAN_POINT('Ctrl Pts',(-21.2123321193934,14.4699515412555,
130.612807306947)) ;
#143715=CARTESIAN_POINT('Ctrl Pts',(-21.2955547074011,14.5110117292323,
130.889053219107)) ;
#143716=CARTESIAN_POINT('Ctrl Pts',(-21.3787853405023,14.4745400439387,
131.165237882417)) ;
#143717=CARTESIAN_POINT('Ctrl Pts',(-21.4561885971438,14.3614975022745,
131.424710865457)) ;
#143718=CARTESIAN_POINT('Ctrl Pts',(-21.519893734885,14.1829580281289,131.64373550919)) ;
#143719=CARTESIAN_POINT('Ctrl Pts',(-21.5660558437163,13.94924048582,131.811726969927)) ;
#143720=CARTESIAN_POINT('Ctrl Pts',(-21.5900114787157,13.6775800783231,
131.914852504217)) ;
#143721=CARTESIAN_POINT('Ctrl Pts',(-21.5895481401675,13.3886494305686,
131.946535521547)) ;
#143722=CARTESIAN_POINT('Ctrl Pts',(-21.5635014834957,13.0993477502972,
131.903825726572)) ;
#143723=CARTESIAN_POINT('Ctrl Pts',(-21.513837759379,12.8369457747394,131.791665496349)) ;
#143724=CARTESIAN_POINT('Ctrl Pts',(-21.4424162592507,12.6140529182667,
131.616278760656)) ;
#143725=CARTESIAN_POINT('Ctrl Pts',(-21.3547003822089,12.4507322880218,
131.393022499549)) ;
#143726=CARTESIAN_POINT('Ctrl Pts',(-21.2552473216185,12.3558899058093,
131.135660559877)) ;
#143727=CARTESIAN_POINT('Ctrl Pts',(-21.1505893270676,12.3380969168945,
130.863169991664)) ;
#143728=CARTESIAN_POINT('Ctrl Pts',(-21.0487008205765,12.3976017184894,
130.598472003428)) ;
#143729=CARTESIAN_POINT('Ctrl Pts',(-20.9545575211431,12.5305839180843,
130.356606283238)) ;
#143730=CARTESIAN_POINT('Ctrl Pts',(-20.8747906198652,12.7283491883042,
130.156805436594)) ;
#143731=CARTESIAN_POINT('Ctrl Pts',(-20.814855044514,12.97427729496,130.014714765469)) ;
#143732=CARTESIAN_POINT('Ctrl Pts',(-20.7775537383068,13.2539378203869,
129.938959194661)) ;
#143733=CARTESIAN_POINT('Ctrl Pts',(-20.7653549702161,13.5450905398915,
129.936447089367)) ;
#143734=CARTESIAN_POINT('Ctrl Pts',(-20.778250046486,13.8275789493197,130.007259996117)) ;
#143735=CARTESIAN_POINT('Ctrl Pts',(-20.8144440542377,14.0806196920483,
130.146052159019)) ;
#143736=CARTESIAN_POINT('Ctrl Pts',(-20.8711507634857,14.2877393448121,
130.344989067034)) ;
#143737=CARTESIAN_POINT('Ctrl Pts',(-20.9424498938353,14.4312139219373,
130.586184629812)) ;
#143738=CARTESIAN_POINT('Ctrl Pts',(-21.0239714683594,14.5038738405656,
130.85759121572)) ;
#143739=CARTESIAN_POINT('Ctrl Pts',(-21.1079824326602,14.4984557258389,
131.13608035658)) ;
#143740=CARTESIAN_POINT('Ctrl Pts',(-21.1882743598749,14.4164646007505,
131.403738404483)) ;
#143741=CARTESIAN_POINT('Ctrl Pts',(-21.2585413217483,14.262213927018,131.642274476708)) ;
#143742=CARTESIAN_POINT('Ctrl Pts',(-21.3122078056105,14.0497488038025,
131.831993572367)) ;
#143743=CARTESIAN_POINT('Ctrl Pts',(-21.3456511109205,13.7905256830516,
131.962929341245)) ;
#143744=CARTESIAN_POINT('Ctrl Pts',(-21.3552119916928,13.5064863468517,
132.023892257237)) ;
#143745=CARTESIAN_POINT('Ctrl Pts',(-21.3394492991724,13.2142514411646,
132.011153788034)) ;
#143746=CARTESIAN_POINT('Ctrl Pts',(-21.2993880623109,12.9406231812218,
131.926977857705)) ;
#143747=CARTESIAN_POINT('Ctrl Pts',(-21.236159113355,12.6982138034392,131.775554994669)) ;
#143748=CARTESIAN_POINT('Ctrl Pts',(-21.1546783206131,12.5096111619529,
131.570515351654)) ;
#143749=CARTESIAN_POINT('Ctrl Pts',(-21.0586507848846,12.3850648455084,
131.323305972789)) ;
#143750=CARTESIAN_POINT('Ctrl Pts',(-20.9559564799004,12.3359713262841,
131.056299516685)) ;
#143751=CARTESIAN_POINT('Ctrl Pts',(-20.8519535030408,12.3641515786215,
130.785604464466)) ;
#143752=CARTESIAN_POINT('Ctrl Pts',(-20.7536461523058,12.4683944870956,
130.531571929203)) ;
#143753=CARTESIAN_POINT('Ctrl Pts',(-20.667420355021,12.6414744959111,130.312873391049)) ;
#143754=CARTESIAN_POINT('Ctrl Pts',(-20.5990533195231,12.8692739699043,
130.146164983405)) ;
#143755=CARTESIAN_POINT('Ctrl Pts',(-20.5519947072442,13.1394382776975,
130.042045907124)) ;
#143756=CARTESIAN_POINT('Ctrl Pts',(-20.5297640471579,13.4257125359272,
130.009941561444)) ;
#143757=CARTESIAN_POINT('Ctrl Pts',(-20.5324664686264,13.7153678906251,
130.051102559557)) ;
#143758=CARTESIAN_POINT('Ctrl Pts',(-20.5595324760176,13.9823826139753,
130.163226514843)) ;
#143759=CARTESIAN_POINT('Ctrl Pts',(-20.608371754187,14.2103512804348,130.339101089377)) ;
#143760=CARTESIAN_POINT('Ctrl Pts',(-20.6744261305736,14.3810373660196,
130.565119965549)) ;
#143761=CARTESIAN_POINT('Ctrl Pts',(-20.7525322815134,14.4835203984391,
130.826411205508)) ;
#143762=CARTESIAN_POINT('Ctrl Pts',(-20.8362000596334,14.5102051461734,
131.103908811644)) ;
#143763=CARTESIAN_POINT('Ctrl Pts',(-20.9193142204875,14.4584272237243,
131.380012083211)) ;
#143764=CARTESIAN_POINT('Ctrl Pts',(-20.9939183747902,14.3332271033523,
131.630932788698)) ;
#143765=CARTESIAN_POINT('Ctrl Pts',(-21.0551280057048,14.1422678192608,
131.842918113244)) ;
#143766=CARTESIAN_POINT('Ctrl Pts',(-21.0972229529673,13.9003525396715,
131.998958255873)) ;
#143767=CARTESIAN_POINT('Ctrl Pts',(-21.1167448448093,13.6237174619485,
132.089138962996)) ;
#143768=CARTESIAN_POINT('Ctrl Pts',(-21.1114203041332,13.3329586763548,
132.106702057009)) ;
#143769=CARTESIAN_POINT('Ctrl Pts',(-21.080916791115,13.0482789829305,132.050754538744)) ;
#143770=CARTESIAN_POINT('Ctrl Pts',(-21.0266195937754,12.7905982685052,
131.925298668968)) ;
#143771=CARTESIAN_POINT('Ctrl Pts',(-20.9521997292132,12.5792073074467,
131.7408905552)) ;
#143772=CARTESIAN_POINT('Ctrl Pts',(-20.8615137418709,12.4271419499118,
131.509129299022)) ;
#143773=CARTESIAN_POINT('Ctrl Pts',(-20.7607142920707,12.3466854310429,
131.247794334763)) ;
#143774=CARTESIAN_POINT('Ctrl Pts',(-20.6562427076659,12.3433384713207,
130.975737443275)) ;
#143775=CARTESIAN_POINT('Ctrl Pts',(-20.5549504108213,12.4172569566232,
130.712936540163)) ;
#143776=CARTESIAN_POINT('Ctrl Pts',(-20.4631678141765,12.5633305895845,
130.47795441216)) ;
#143777=CARTESIAN_POINT('Ctrl Pts',(-20.386921679344,12.7708595617965,130.288329923847)) ;
#143778=CARTESIAN_POINT('Ctrl Pts',(-20.3308120046874,13.025326544213,130.157561920011)) ;
#143779=CARTESIAN_POINT('Ctrl Pts',(-20.2982429233288,13.3082180027096,
130.095548052008)) ;
#143780=CARTESIAN_POINT('Ctrl Pts',(-20.2907757621212,13.5990346851552,
130.106831087445)) ;
#143781=CARTESIAN_POINT('Ctrl Pts',(-20.3081537505599,13.8774217687766,
130.190705780526)) ;
#143782=CARTESIAN_POINT('Ctrl Pts',(-20.3486475693887,14.1239850259666,
130.342217744254)) ;
#143783=CARTESIAN_POINT('Ctrl Pts',(-20.40825134073,14.3192777030772,130.549401817463)) ;
#143784=CARTESIAN_POINT('Ctrl Pts',(-20.482206299086,14.450773280104,130.798558182801)) ;
#143785=CARTESIAN_POINT('Ctrl Pts',(-20.5644237207708,14.5087792742394,
131.071837523224)) ;
#143786=CARTESIAN_POINT('Ctrl Pts',(-20.6486285547493,14.4887238114624,
131.351056533869)) ;
#143787=CARTESIAN_POINT('Ctrl Pts',(-20.7272350805244,14.3928284673273,
131.613698351731)) ;
#143788=CARTESIAN_POINT('Ctrl Pts',(-20.794923502291,14.2263681576049,131.844708220877)) ;
#143789=CARTESIAN_POINT('Ctrl Pts',(-20.84507946644,14.0038696004935,132.024217539971)) ;
#143790=CARTESIAN_POINT('Ctrl Pts',(-20.8741779141571,13.7389371650263,
132.142367468664)) ;
#143791=CARTESIAN_POINT('Ctrl Pts',(-20.8790905217415,13.4518073481161,
132.189802522045)) ;
#143792=CARTESIAN_POINT('Ctrl Pts',(-20.858730901802,13.1616327343089,132.163529091199)) ;
#143793=CARTESIAN_POINT('Ctrl Pts',(-20.8137892339047,12.8906304369754,
132.065399389232)) ;
#143794=CARTESIAN_POINT('Ctrl Pts',(-20.7470135686821,12.6585325356575,
131.903393481101)) ;
#143795=CARTESIAN_POINT('Ctrl Pts',(-20.6624947858425,12.4808578781887,
131.689522457705)) ;
#143796=CARTESIAN_POINT('Ctrl Pts',(-20.5643202030253,12.3697949694261,
131.436105306196)) ;
#143797=CARTESIAN_POINT('Ctrl Pts',(-20.4610498700862,12.3353140236409,
131.167379944547)) ;
#143798=CARTESIAN_POINT('Ctrl Pts',(-20.3574082392478,12.3783402030792,
130.89781264628)) ;
#143799=CARTESIAN_POINT('Ctrl Pts',(-20.2612268033925,12.4961138022352,
130.649899660601)) ;
#143800=CARTESIAN_POINT('Ctrl Pts',(-20.1780818919777,12.680095634731,130.440110299312)) ;
#143801=CARTESIAN_POINT('Ctrl Pts',(-20.1132235209398,12.9180877630852,
130.283835936512)) ;
#143802=CARTESIAN_POINT('Ctrl Pts',(-20.0709566929653,13.1911275854678,
130.193411093563)) ;
#143803=CARTESIAN_POINT('Ctrl Pts',(-20.0531602513411,13.4815073291889,
130.174562545783)) ;
#143804=CARTESIAN_POINT('Ctrl Pts',(-20.0607201513665,13.7684315330807,
130.229876234887)) ;
#143805=CARTESIAN_POINT('Ctrl Pts',(-20.0920900302076,14.0290764110969,
130.354550101899)) ;
#143806=CARTESIAN_POINT('Ctrl Pts',(-20.1445760208522,14.247309485019,130.54105507157)) ;
#143807=CARTESIAN_POINT('Ctrl Pts',(-20.2131672327109,14.4057092189414,
130.774419872493)) ;
#143808=CARTESIAN_POINT('Ctrl Pts',(-20.2931490018152,14.4946179014392,
131.041320306837)) ;
#143809=CARTESIAN_POINT('Ctrl Pts',(-20.3770264287286,14.5063975048984,
131.319385004787)) ;
#143810=CARTESIAN_POINT('Ctrl Pts',(-20.4591355130039,14.4401277902918,
131.592540260583)) ;
#143811=CARTESIAN_POINT('Ctrl Pts',(-20.5314992276366,14.3020000140496,
131.836880126924)) ;
#143812=CARTESIAN_POINT('Ctrl Pts',(-20.5894710367744,14.1003807123236,
132.03938198034)) ;
#143813=CARTESIAN_POINT('Ctrl Pts',(-20.6275991795873,13.8504600276244,
132.183862987364)) ;
#143814=CARTESIAN_POINT('Ctrl Pts',(-20.6425877337758,13.5690358349625,
132.260858497093)) ;
#143815=CARTESIAN_POINT('Ctrl Pts',(-20.632372444611,13.2773475296497,132.264198835309)) ;
#143816=CARTESIAN_POINT('Ctrl Pts',(-20.5974164630217,12.9978263790817,
132.19505566985)) ;
#143817=CARTESIAN_POINT('Ctrl Pts',(-20.5390138830624,12.7470236955785,
132.05763095546)) ;
#143818=CARTESIAN_POINT('Ctrl Pts',(-20.4609877883318,12.545343046617,131.862781749307)) ;
#143819=CARTESIAN_POINT('Ctrl Pts',(-20.3678785101158,12.4062332571894,
131.623944714736)) ;
#143820=CARTESIAN_POINT('Ctrl Pts',(-20.2661748246587,12.3400677783264,
131.359872952747)) ;
#143821=CARTESIAN_POINT('Ctrl Pts',(-20.1612567497015,12.3515723275397,
131.086676839459)) ;
#143822=CARTESIAN_POINT('Ctrl Pts',(-20.0615848469451,12.4396026158797,
130.82851586695)) ;
#143823=CARTESIAN_POINT('Ctrl Pts',(-19.9722369368756,12.5983880408564,
130.600675700158)) ;
#143824=CARTESIAN_POINT('Ctrl Pts',(-19.8996242883099,12.8155082856179,
130.421593407092)) ;
#143825=CARTESIAN_POINT('Ctrl Pts',(-19.8475518785741,13.0777481932152,
130.302736870524)) ;
#143826=CARTESIAN_POINT('Ctrl Pts',(-19.8197563730186,13.364000804506,130.254684914467)) ;
#143827=CARTESIAN_POINT('Ctrl Pts',(-19.8170697551175,13.6530970935561,
130.27982574218)) ;
#143828=CARTESIAN_POINT('Ctrl Pts',(-19.839060486369,13.9274411059631,130.377257704675)) ;
#143829=CARTESIAN_POINT('Ctrl Pts',(-19.8833826907644,14.1649405749744,
130.539835176495)) ;
#143830=CARTESIAN_POINT('Ctrl Pts',(-19.946370690104,14.3499177041157,130.757052955588)) ;
#143831=CARTESIAN_POINT('Ctrl Pts',(-20.0223920281984,14.4676736772021,
131.012227837299)) ;
#143832=CARTESIAN_POINT('Ctrl Pts',(-20.1051541931323,14.5109849191037,
131.286985839572)) ;
#143833=CARTESIAN_POINT('Ctrl Pts',(-20.18894891482,14.4763368013962,131.565019086318)) ;
#143834=CARTESIAN_POINT('Ctrl Pts',(-20.2659802707125,14.3664425306899,
131.823111021419)) ;
#143835=CARTESIAN_POINT('Ctrl Pts',(-20.3307357805088,14.188260258707,132.045502355382)) ;
#143836=CARTESIAN_POINT('Ctrl Pts',(-20.3772257856926,13.9563928722856,
132.214338660589)) ;
#143837=CARTESIAN_POINT('Ctrl Pts',(-20.4018956542535,13.6856074997971,
132.319552911824)) ;
#143838=CARTESIAN_POINT('Ctrl Pts',(-20.402087534473,13.3967977975017,132.353162100239)) ;
#143839=CARTESIAN_POINT('Ctrl Pts',(-20.3769488824518,13.1083771825577,
132.312954980926)) ;
#143840=CARTESIAN_POINT('Ctrl Pts',(-20.3277277023517,12.8436200801875,
132.202260047876)) ;
#143841=CARTESIAN_POINT('Ctrl Pts',(-20.2569355974636,12.6197329194616,
132.028657274242)) ;
#143842=CARTESIAN_POINT('Ctrl Pts',(-20.1694662975559,12.4541609796659,
131.80618730668)) ;
#143843=CARTESIAN_POINT('Ctrl Pts',(-20.0700517699011,12.357518085621,131.548991538675)) ;
#143844=CARTESIAN_POINT('Ctrl Pts',(-19.966347191366,12.3374075405641,131.278995876173)) ;
#143845=CARTESIAN_POINT('Ctrl Pts',(-19.8634803419964,12.3950240901617,
131.011711144262)) ;
#143846=CARTESIAN_POINT('Ctrl Pts',(-19.7694521450956,12.5255975503683,
130.770028076305)) ;
#143847=CARTESIAN_POINT('Ctrl Pts',(-19.6889554236045,12.7221237769604,
130.568189360195)) ;
#143848=CARTESIAN_POINT('Ctrl Pts',(-19.6284746226204,12.9666439794892,
130.424467938799)) ;
#143849=CARTESIAN_POINT('Ctrl Pts',(-19.59039372203,13.2467844847395,130.346566394817)) ;
#143850=CARTESIAN_POINT('Ctrl Pts',(-19.5776057553389,13.5364086840901,
130.342163547303)) ;
#143851=CARTESIAN_POINT('Ctrl Pts',(-19.5896981839258,13.8193015445878,
130.410610408146)) ;
#143852=CARTESIAN_POINT('Ctrl Pts',(-19.6252906608147,14.0737432295645,
130.547683639879)) ;
#143853=CARTESIAN_POINT('Ctrl Pts',(-19.6813765478133,14.28233845815,130.744766235332)) ;
#143854=CARTESIAN_POINT('Ctrl Pts',(-19.7525262423754,14.428082061538,130.985623109379)) ;
#143855=CARTESIAN_POINT('Ctrl Pts',(-19.8334644514673,14.5027907453993,
131.255163146721)) ;
#143856=CARTESIAN_POINT('Ctrl Pts',(-19.9181420687845,14.4996008871204,
131.535862402913)) ;
#143857=CARTESIAN_POINT('Ctrl Pts',(-19.9981755813607,14.419843429899,131.802586216274)) ;
#143858=CARTESIAN_POINT('Ctrl Pts',(-20.0687288547216,14.2682254316152,
132.041884513473)) ;
#143859=CARTESIAN_POINT('Ctrl Pts',(-20.1231433501969,14.0566690769085,
132.233899830116)) ;
#143860=CARTESIAN_POINT('Ctrl Pts',(-20.1572405438189,13.7984045254372,
132.366752500805)) ;
#143861=CARTESIAN_POINT('Ctrl Pts',(-20.1674646547526,13.5146253545805,
132.429679127936)) ;
#143862=CARTESIAN_POINT('Ctrl Pts',(-20.1525953490523,13.223790028339,132.419372446335)) ;
#143863=CARTESIAN_POINT('Ctrl Pts',(-20.1130358657083,12.9476428894619,
132.336873395723)) ;
#143864=CARTESIAN_POINT('Ctrl Pts',(-20.0503426230759,12.7041857857084,
132.187005515754)) ;
#143865=CARTESIAN_POINT('Ctrl Pts',(-19.9694659663671,12.5142907834555,
131.983675392732)) ;
#143866=CARTESIAN_POINT('Ctrl Pts',(-19.8739753931397,12.3877724095918,
131.737965648296)) ;
#143867=CARTESIAN_POINT('Ctrl Pts',(-19.7709443029584,12.336191203021,131.470124280929)) ;
#143868=CARTESIAN_POINT('Ctrl Pts',(-19.6669365691679,12.3624798343251,
131.199398785677)) ;
#143869=CARTESIAN_POINT('Ctrl Pts',(-19.5687719098967,12.4640688198504,
130.945644876183)) ;
#143870=CARTESIAN_POINT('Ctrl Pts',(-19.4817848481537,12.6358046378966,
130.724836080655)) ;
#143871=CARTESIAN_POINT('Ctrl Pts',(-19.4130402249853,12.8620488663086,
130.556977640894)) ;
#143872=CARTESIAN_POINT('Ctrl Pts',(-19.3654039404876,13.1294243702491,
130.450960645276)) ;
#143873=CARTESIAN_POINT('Ctrl Pts',(-19.3421969031624,13.4191275485285,
130.416438112994)) ;
#143874=CARTESIAN_POINT('Ctrl Pts',(-19.3442262557683,13.7060585191979,
130.455278759065)) ;
#143875=CARTESIAN_POINT('Ctrl Pts',(-19.3707106093196,13.9758635048128,
130.565935791541)) ;
#143876=CARTESIAN_POINT('Ctrl Pts',(-19.4189272476174,14.2044690848735,
130.739897049957)) ;
#143877=CARTESIAN_POINT('Ctrl Pts',(-19.4846182490666,14.3772046545246,
130.964899352542)) ;
#143878=CARTESIAN_POINT('Ctrl Pts',(-19.5624570312064,14.4817041714967,
131.225395979999)) ;
#143879=CARTESIAN_POINT('Ctrl Pts',(-19.6461425521004,14.5103977603672,
131.502983431525)) ;
#143880=CARTESIAN_POINT('Ctrl Pts',(-19.7288282612474,14.4613877005576,
131.777604673512)) ;
#143881=CARTESIAN_POINT('Ctrl Pts',(-19.8041618277618,14.3378670133984,
132.030826862098)) ;
#143882=CARTESIAN_POINT('Ctrl Pts',(-19.8657702567754,14.1487648805611,
132.243936937615)) ;
#143883=CARTESIAN_POINT('Ctrl Pts',(-19.9085599505618,13.9077123498208,
132.402067970361)) ;
#143884=CARTESIAN_POINT('Ctrl Pts',(-19.9287403578106,13.6318347847728,
132.494161297536)) ;
#143885=CARTESIAN_POINT('Ctrl Pts',(-19.9241285333911,13.3411960486728,
132.513808537463)) ;
#143886=CARTESIAN_POINT('Ctrl Pts',(-19.8943722337192,13.0563345512955,
132.460007505097)) ;
#143887=CARTESIAN_POINT('Ctrl Pts',(-19.8407354442242,12.7976620834808,
132.336477575288)) ;
#143888=CARTESIAN_POINT('Ctrl Pts',(-19.7669398342799,12.5846251876044,
132.153875056264)) ;
#143889=CARTESIAN_POINT('Ctrl Pts',(-19.6758878336454,12.429833205716,131.921298618884)) ;
#143890=CARTESIAN_POINT('Ctrl Pts',(-19.5761959977977,12.3481748441672,
131.662890781629)) ;
#143891=CARTESIAN_POINT('Ctrl Pts',(-19.4713288624757,12.3422836443017,
131.389814015339)) ;
#143892=CARTESIAN_POINT('Ctrl Pts',(-19.3699251221927,12.4141623973689,
131.126663932511)) ;
#143893=CARTESIAN_POINT('Ctrl Pts',(-19.2776778514234,12.5584918127645,
130.890365636612)) ;
#143894=CARTESIAN_POINT('Ctrl Pts',(-19.2009980997659,12.7644626666543,
130.699456378474)) ;
#143895=CARTESIAN_POINT('Ctrl Pts',(-19.1443455018427,13.0174117066364,
130.567048844427)) ;
#143896=CARTESIAN_POINT('Ctrl Pts',(-19.1110423418376,13.2998966428893,
130.502908392849)) ;
#143897=CARTESIAN_POINT('Ctrl Pts',(-19.1028387268705,13.5908801629709,
130.512051029699)) ;
#143898=CARTESIAN_POINT('Ctrl Pts',(-19.1196170916764,13.8706961833489,
130.594271086926)) ;
#143899=CARTESIAN_POINT('Ctrl Pts',(-19.159552960718,14.1180204039502,130.74412111884)) ;
#143900=CARTESIAN_POINT('Ctrl Pts',(-19.2184761004089,14.3143766861394,
130.949213922764)) ;
#143901=CARTESIAN_POINT('Ctrl Pts',(-19.2922787411306,14.4481661316014,
131.198005144871)) ;
#143902=CARTESIAN_POINT('Ctrl Pts',(-19.3741452353846,14.508083869743,131.470174035041)) ;
#143903=CARTESIAN_POINT('Ctrl Pts',(-19.4583253760916,14.490551827571,131.749290337179)) ;
#143904=CARTESIAN_POINT('Ctrl Pts',(-19.5374248602333,14.3964091806781,
132.013482408106)) ;
#143905=CARTESIAN_POINT('Ctrl Pts',(-19.6052930437783,14.2323049271919,
132.244907382024)) ;
#143906=CARTESIAN_POINT('Ctrl Pts',(-19.6560850193192,14.0113006230555,
132.426290968773)) ;
#143907=CARTESIAN_POINT('Ctrl Pts',(-19.6858796266344,13.7469852751569,
132.546516040551)) ;
#143908=CARTESIAN_POINT('Ctrl Pts',(-19.6915477871688,13.4601450927403,
132.596164261453)) ;
#143909=CARTESIAN_POINT('Ctrl Pts',(-19.6717188591123,13.1687002988962,
132.571570210908)) ;
#143910=CARTESIAN_POINT('Ctrl Pts',(-19.6278387509683,12.8989650808956,
132.476275608127)) ;
#143911=CARTESIAN_POINT('Ctrl Pts',(-19.5611246263324,12.6635916502146,
132.314724093995)) ;
#143912=CARTESIAN_POINT('Ctrl Pts',(-19.4773775734119,12.4852398029377,
132.102947245662)) ;
#143913=CARTESIAN_POINT('Ctrl Pts',(-19.3794463063608,12.371925952002,131.850265421701)) ;
#143914=CARTESIAN_POINT('Ctrl Pts',(-19.2764036885513,12.3351771027553,
131.582155999456)) ;
#143915=CARTESIAN_POINT('Ctrl Pts',(-19.1723427206771,12.3762351051066,
131.311472093278)) ;
#143916=CARTESIAN_POINT('Ctrl Pts',(-19.0763723598902,12.4911992471527,
131.06399151218)) ;
#143917=CARTESIAN_POINT('Ctrl Pts',(-18.9922096682478,12.6745749417996,
130.851450255868)) ;
#143918=CARTESIAN_POINT('Ctrl Pts',(-18.9270369780191,12.9105841492293,
130.694139865369)) ;
#143919=CARTESIAN_POINT('Ctrl Pts',(-18.8839823300028,13.1834575977754,
130.601491539362)) ;
#143920=CARTESIAN_POINT('Ctrl Pts',(-18.8655874201825,13.472817267858,130.580799753087)) ;
#143921=CARTESIAN_POINT('Ctrl Pts',(-18.8722524231717,13.7593252919433,
130.633389173602)) ;
#143922=CARTESIAN_POINT('Ctrl Pts',(-18.9032397697211,14.0229112267302,
130.757205209474)) ;
#143923=CARTESIAN_POINT('Ctrl Pts',(-18.9547768664526,14.2409569319606,
130.940675690362)) ;
#143924=CARTESIAN_POINT('Ctrl Pts',(-19.0233923114078,14.4024703207306,
131.174341399345)) ;
#143925=CARTESIAN_POINT('Ctrl Pts',(-19.1029165563042,14.4930253207348,
131.43979044431)) ;
#143926=CARTESIAN_POINT('Ctrl Pts',(-19.1868068466344,14.5071137946879,
131.717918368786)) ;
#143927=CARTESIAN_POINT('Ctrl Pts',(-19.2687479247028,14.4434721690138,
131.99044237149)) ;
#143928=CARTESIAN_POINT('Ctrl Pts',(-19.3417397331137,14.3072990407348,
132.236714912124)) ;
#143929=CARTESIAN_POINT('Ctrl Pts',(-19.4004487381664,14.1061280190249,
132.441533665576)) ;
#143930=CARTESIAN_POINT('Ctrl Pts',(-19.4389556441804,13.8584456467317,
132.586963381329)) ;
#143931=CARTESIAN_POINT('Ctrl Pts',(-19.4547110225428,13.5782525507237,
132.666137792883)) ;
#143932=CARTESIAN_POINT('Ctrl Pts',(-19.445287263111,13.2862403685174,132.671828009305)) ;
#143933=CARTESIAN_POINT('Ctrl Pts',(-19.4110002332987,13.0054671404376,
132.604709517203)) ;
#143934=CARTESIAN_POINT('Ctrl Pts',(-19.3529363497825,12.7527976757228,
132.468391881073)) ;
#143935=CARTESIAN_POINT('Ctrl Pts',(-19.2758383987832,12.5507720823643,
132.276062163398)) ;
#143936=CARTESIAN_POINT('Ctrl Pts',(-19.183036429821,12.4092692851511,132.038156718385)) ;
#143937=CARTESIAN_POINT('Ctrl Pts',(-19.0812978335299,12.3409405879061,
131.774046332401)) ;
#143938=CARTESIAN_POINT('Ctrl Pts',(-18.9767024131274,12.3499819514293,
131.501678448741)) ;
#143939=CARTESIAN_POINT('Ctrl Pts',(-18.8763024196267,12.4363532900494,
131.241564305693)) ;
#143940=CARTESIAN_POINT('Ctrl Pts',(-18.7870104329141,12.592566468637,131.013723468433)) ;
#143941=CARTESIAN_POINT('Ctrl Pts',(-18.7136463936558,12.808517161013,130.832521133127)) ;
#143942=CARTESIAN_POINT('Ctrl Pts',(-18.6610063634179,13.0694867381501,
130.711967777011)) ;
#143943=CARTESIAN_POINT('Ctrl Pts',(-18.632410200303,13.3550372325075,130.661550020128)) ;
#143944=CARTESIAN_POINT('Ctrl Pts',(-18.629052962816,13.6462143914832,130.684953987523)) ;
#143945=CARTESIAN_POINT('Ctrl Pts',(-18.6502970918763,13.9195288326514,
130.779995857368)) ;
#143946=CARTESIAN_POINT('Ctrl Pts',(-18.6939926671848,14.1586151342569,
130.940770034127)) ;
#143947=CARTESIAN_POINT('Ctrl Pts',(-18.7563803737566,14.3449690064031,
131.156166852151)) ;
#143948=CARTESIAN_POINT('Ctrl Pts',(-18.8320450450556,14.4652397459023,
131.410296759735)) ;
#143949=CARTESIAN_POINT('Ctrl Pts',(-18.9153450746737,14.5107689860091,
131.686885139385)) ;
#143950=CARTESIAN_POINT('Ctrl Pts',(-18.9984240823211,14.4787461953136,
131.962499912619)) ;
#143951=CARTESIAN_POINT('Ctrl Pts',(-19.0764363731335,14.3700644333909,
132.223765872129)) ;
#143952=CARTESIAN_POINT('Ctrl Pts',(-19.1411505492463,14.1946408209154,
132.445805538787)) ;
#143953=CARTESIAN_POINT('Ctrl Pts',(-19.1883722206098,13.9639077381356,
132.616845906245)) ;
#143954=CARTESIAN_POINT('Ctrl Pts',(-19.2137492404945,13.6940409342519,
132.724111687935)) ;
#143955=CARTESIAN_POINT('Ctrl Pts',(-19.2145880477621,13.4043243870117,
132.759747994875)) ;
#143956=CARTESIAN_POINT('Ctrl Pts',(-19.1903786530231,13.1175424203496,
132.722018069961)) ;
#143957=CARTESIAN_POINT('Ctrl Pts',(-19.1415408484447,12.8501253800453,
132.612661218455)) ;
#143958=CARTESIAN_POINT('Ctrl Pts',(-19.0716495724154,12.6260375072132,
132.441510922512)) ;
#143959=CARTESIAN_POINT('Ctrl Pts',(-18.9844995837982,12.4581544955602,
132.220034073742)) ;
#143960=CARTESIAN_POINT('Ctrl Pts',(-18.8855629159112,12.3594525317711,
131.964157974244)) ;
#143961=CARTESIAN_POINT('Ctrl Pts',(-18.781568439516,12.3367944106136,131.69342789164)) ;
#143962=CARTESIAN_POINT('Ctrl Pts',(-18.6782922396415,12.3925085766977,
131.425032749455)) ;
#143963=CARTESIAN_POINT('Ctrl Pts',(-18.5839790247587,12.5213899475148,
131.182523412252)) ;
#143964=CARTESIAN_POINT('Ctrl Pts',(-18.5032609434197,12.715572513745,130.979923431317)) ;
#143965=CARTESIAN_POINT('Ctrl Pts',(-18.4420722767198,12.9595222132268,
130.834214989689)) ;
#143966=CARTESIAN_POINT('Ctrl Pts',(-18.40353217852,13.2367790657483,130.754712073368)) ;
#143967=CARTESIAN_POINT('Ctrl Pts',(-18.3897870456702,13.5277645483974,
130.747681760714)) ;
#143968=CARTESIAN_POINT('Ctrl Pts',(-18.4012590895738,13.8120455612361,
130.814415686742)) ;
#143969=CARTESIAN_POINT('Ctrl Pts',(-18.4363207056852,14.0676656402339,
130.949968439689)) ;
#143970=CARTESIAN_POINT('Ctrl Pts',(-18.4917693507281,14.2771421243593,
131.145101016195)) ;
#143971=CARTESIAN_POINT('Ctrl Pts',(-18.5625493538873,14.4250319650245,
131.384885119588)) ;
#143972=CARTESIAN_POINT('Ctrl Pts',(-18.643665197432,14.5017260343279,131.655084520159)) ;
#143973=CARTESIAN_POINT('Ctrl Pts',(-18.7273753185774,14.5010098763796,
131.93256823998)) ;
#143974=CARTESIAN_POINT('Ctrl Pts',(-18.8083279001163,14.4231232861786,
132.202267998652)) ;
#143975=CARTESIAN_POINT('Ctrl Pts',(-18.8790721039087,14.2735699420865,
132.442042706819)) ;
#143976=CARTESIAN_POINT('Ctrl Pts',(-18.934118330524,14.0631259217895,132.635977437453)) ;
#143977=CARTESIAN_POINT('Ctrl Pts',(-18.9687409921237,13.8068511447586,
132.77024180709)) ;
#143978=CARTESIAN_POINT('Ctrl Pts',(-18.9797426090043,13.5229066982492,
132.835523927713)) ;
#143979=CARTESIAN_POINT('Ctrl Pts',(-18.9656045700259,13.2323183656793,
132.827310581068)) ;
#143980=CARTESIAN_POINT('Ctrl Pts',(-18.9267636321704,12.9554622848227,
132.746912610664)) ;
#143981=CARTESIAN_POINT('Ctrl Pts',(-18.8647595657246,12.7108336294588,
132.599034340916)) ;
#143982=CARTESIAN_POINT('Ctrl Pts',(-18.7842026722726,12.5189036240624,
132.396704170719)) ;
#143983=CARTESIAN_POINT('Ctrl Pts',(-18.6893441361919,12.390658589764,132.152733493589)) ;
#143984=CARTESIAN_POINT('Ctrl Pts',(-18.5863020448112,12.3366531307129,
131.884915005918)) ;
#143985=CARTESIAN_POINT('Ctrl Pts',(-18.4823911075163,12.3602977893096,
131.614409397646)) ;
#143986=CARTESIAN_POINT('Ctrl Pts',(-18.3831235087243,12.4609988755096,
131.357739271015)) ;
#143987=CARTESIAN_POINT('Ctrl Pts',(-18.2966708436327,12.6291274896935,
131.13812421699)) ;
#143988=CARTESIAN_POINT('Ctrl Pts',(-18.2267347033546,12.8555169939373,
130.967049610023)) ;
#143989=CARTESIAN_POINT('Ctrl Pts',(-18.178684786641,13.1215885619852,130.859745333703)) ;
#143990=CARTESIAN_POINT('Ctrl Pts',(-18.1547618093871,13.4096083947618,
130.822983784196)) ;
#143991=CARTESIAN_POINT('Ctrl Pts',(-18.1560074176891,13.6982129377788,
130.859689555193)) ;
#143992=CARTESIAN_POINT('Ctrl Pts',(-18.1819407569754,13.969145223664,130.968781097798)) ;
#143993=CARTESIAN_POINT('Ctrl Pts',(-18.2294348519779,14.1982918384811,
131.140518474738)) ;
#143994=CARTESIAN_POINT('Ctrl Pts',(-18.2945663581642,14.3728095638234,
131.363846741243)) ;
#143995=CARTESIAN_POINT('Ctrl Pts',(-18.3722159348404,14.4796622896265,
131.623830517624)) ;
#143996=CARTESIAN_POINT('Ctrl Pts',(-18.4558928969119,14.5107460885462,
131.901416593924)) ;
#143997=CARTESIAN_POINT('Ctrl Pts',(-18.5389249565536,14.4636147877097,
132.177147765495)) ;
#143998=CARTESIAN_POINT('Ctrl Pts',(-18.6142268417918,14.3427084446703,
132.430124576738)) ;
#143999=CARTESIAN_POINT('Ctrl Pts',(-18.6766156566363,14.1545213571348,
132.645670743121)) ;
#144000=CARTESIAN_POINT('Ctrl Pts',(-18.7198818709583,13.9146657038493,
132.805172644963)) ;
#144001=CARTESIAN_POINT('Ctrl Pts',(-18.7406883952545,13.6405171669677,
132.898977954723)) ;
#144002=CARTESIAN_POINT('Ctrl Pts',(-18.7368457016297,13.3501101589506,
132.920865495942)) ;
#144003=CARTESIAN_POINT('Ctrl Pts',(-18.7079487411962,13.0651841999784,
132.869519266352)) ;
#144004=CARTESIAN_POINT('Ctrl Pts',(-18.6546706091732,12.8038875928186,
132.747233558968)) ;
#144005=CARTESIAN_POINT('Ctrl Pts',(-18.5814042568152,12.5899464176031,
132.566132647451)) ;
#144006=CARTESIAN_POINT('Ctrl Pts',(-18.4914287730643,12.4339562439877,
132.336473507997)) ;
#144007=CARTESIAN_POINT('Ctrl Pts',(-18.3911210751021,12.3491846670138,
132.076546495149)) ;
#144008=CARTESIAN_POINT('Ctrl Pts',(-18.2862071161722,12.3415474496416,
131.803348771399)) ;
#144009=CARTESIAN_POINT('Ctrl Pts',(-18.185020267949,12.4110292965116,131.540707750202)) ;
#144010=CARTESIAN_POINT('Ctrl Pts',(-18.0923825798042,12.5533606733183,
131.303276774471)) ;
#144011=CARTESIAN_POINT('Ctrl Pts',(-18.0152756269635,12.7574393223527,
131.111078020155)) ;
#144012=CARTESIAN_POINT('Ctrl Pts',(-17.9578353710385,13.009581913367,130.976421309906)) ;
#144013=CARTESIAN_POINT('Ctrl Pts',(-17.9237910313609,13.2928228925075,
130.910262343832)) ;
#144014=CARTESIAN_POINT('Ctrl Pts',(-17.9149479043077,13.582012204951,130.917325191259)) ;
#144015=CARTESIAN_POINT('Ctrl Pts',(-17.9310342367056,13.8633231100431,
130.997627599138)) ;
#144016=CARTESIAN_POINT('Ctrl Pts',(-17.9702736832324,14.1112604273849,
131.145362804117)) ;
#144017=CARTESIAN_POINT('Ctrl Pts',(-18.0287922044005,14.3095522815314,
131.349330597399)) ;
#144018=CARTESIAN_POINT('Ctrl Pts',(-18.1019911045966,14.44510578155,131.596246152401)) ;
#144019=CARTESIAN_POINT('Ctrl Pts',(-18.1843833903802,14.5076745879146,
131.870226367737)) ;
#144020=CARTESIAN_POINT('Ctrl Pts',(-18.2683793556834,14.4918702238892,
132.148714883584)) ;
#144021=CARTESIAN_POINT('Ctrl Pts',(-18.3474187695467,14.4001695332023,
132.412617942134)) ;
#144022=CARTESIAN_POINT('Ctrl Pts',(-18.4156630172785,14.2383391968108,
132.645098549425)) ;
#144023=CARTESIAN_POINT('Ctrl Pts',(-18.467196959154,14.0178456765348,132.828789503516)) ;
#144024=CARTESIAN_POINT('Ctrl Pts',(-18.4976105450035,13.7549023993413,
132.950761290453)) ;
#144025=CARTESIAN_POINT('Ctrl Pts',(-18.5038507504708,13.4669383110673,
133.002257275435)) ;
#144026=CARTESIAN_POINT('Ctrl Pts',(-18.4851160162367,13.179287796842,132.980385937109)) ;
#144027=CARTESIAN_POINT('Ctrl Pts',(-18.4414836298312,12.9054935054356,
132.886215827744)) ;
#144028=CARTESIAN_POINT('Ctrl Pts',(-18.3759576029619,12.6708451736549,
132.727823306595)) ;
#144029=CARTESIAN_POINT('Ctrl Pts',(-18.2919020242458,12.489010935019,132.515465753891)) ;
#144030=CARTESIAN_POINT('Ctrl Pts',(-18.195291179958,12.3747427452421,132.266277907465)) ;
#144031=CARTESIAN_POINT('Ctrl Pts',(-18.091594831957,12.3351181280502,131.996517106783)) ;
#144032=CARTESIAN_POINT('Ctrl Pts',(-17.9879486999613,12.3735357239234,
131.726863664562)) ;
#144033=CARTESIAN_POINT('Ctrl Pts',(-17.8906852858916,12.4876827047378,
131.475961664461)) ;
#144034=CARTESIAN_POINT('Ctrl Pts',(-17.8067791669803,12.6681438766094,
131.263905063417)) ;
#144035=CARTESIAN_POINT('Ctrl Pts',(-17.7407847508741,12.9033828008646,
131.104296212358)) ;
#144036=CARTESIAN_POINT('Ctrl Pts',(-17.6972166763221,13.1743601977476,
131.010010008373)) ;
#144037=CARTESIAN_POINT('Ctrl Pts',(-17.6779325586506,13.4644840524054,
130.986835357892)) ;
#144038=CARTESIAN_POINT('Ctrl Pts',(-17.6840007503613,13.7518156372007,
131.037738629709)) ;
#144039=CARTESIAN_POINT('Ctrl Pts',(-17.7140670121059,14.0147481121993,
131.158647104721)) ;
#144040=CARTESIAN_POINT('Ctrl Pts',(-17.7653297228469,14.2359323146828,
131.341537689732)) ;
#144041=CARTESIAN_POINT('Ctrl Pts',(-17.8336956152316,14.3990328961567,
131.574504973464)) ;
#144042=CARTESIAN_POINT('Ctrl Pts',(-17.9125313999844,14.4913721477539,
131.83775479626)) ;
#144043=CARTESIAN_POINT('Ctrl Pts',(-17.9968649663334,14.5077030506771,
132.117375597015)) ;
#144044=CARTESIAN_POINT('Ctrl Pts',(-18.0785119061021,14.4466726392651,
132.388843886304)) ;
#144045=CARTESIAN_POINT('Ctrl Pts',(-18.1524693054502,14.3110619945875,
132.638246915545)) ;
#144046=CARTESIAN_POINT('Ctrl Pts',(-18.2110525859729,14.1132679223134,
132.842369697694)) ;
#144047=CARTESIAN_POINT('Ctrl Pts',(-18.2504776017827,13.8656263142686,
132.990662346473)) ;
#144048=CARTESIAN_POINT('Ctrl Pts',(-18.2668284491577,13.5853315264496,
133.071641048268)) ;
#144049=CARTESIAN_POINT('Ctrl Pts',(-18.2580557921982,13.2939510978671,
133.07916650733)) ;
#144050=CARTESIAN_POINT('Ctrl Pts',(-18.2245616027976,13.0136079092844,
133.014252441019)) ;
#144051=CARTESIAN_POINT('Ctrl Pts',(-18.1674098083939,12.7604082845335,
132.880496364703)) ;
#144052=CARTESIAN_POINT('Ctrl Pts',(-18.090494442978,12.5556139237626,132.688861748547)) ;
#144053=CARTESIAN_POINT('Ctrl Pts',(-17.997864980143,12.4121627059908,132.451509225692)) ;
#144054=CARTESIAN_POINT('Ctrl Pts',(-17.8965884139111,12.3419224610127,
132.188653868652)) ;
#144055=CARTESIAN_POINT('Ctrl Pts',(-17.792087088157,12.3485705952627,131.916526485213)) ;
#144056=CARTESIAN_POINT('Ctrl Pts',(-17.6915055460129,12.4325162963297,
131.655862931741)) ;
#144057=CARTESIAN_POINT('Ctrl Pts',(-17.6015237275694,12.5872707160174,
131.42611251694)) ;
#144058=CARTESIAN_POINT('Ctrl Pts',(-17.5277116214108,12.8016743120911,
131.2435792644)) ;
#144059=CARTESIAN_POINT('Ctrl Pts',(-17.474505078703,13.0608928169866,131.121287014814)) ;
#144060=CARTESIAN_POINT('Ctrl Pts',(-17.4451268590908,13.3463628711479,
131.068632504424)) ;
#144061=CARTESIAN_POINT('Ctrl Pts',(-17.4409756319216,13.6367414871714,
131.089604614589)) ;
#144062=CARTESIAN_POINT('Ctrl Pts',(-17.4615369886941,13.9121235287477,
131.182800505553)) ;
#144063=CARTESIAN_POINT('Ctrl Pts',(-17.5047804458157,14.1528033818472,
131.342314267092)) ;
#144064=CARTESIAN_POINT('Ctrl Pts',(-17.5665368051181,14.3402810469184,
131.555772727796)) ;
#144065=CARTESIAN_POINT('Ctrl Pts',(-17.6417901561433,14.4626257228514,
131.808667033106)) ;
#144066=CARTESIAN_POINT('Ctrl Pts',(-17.7250930723354,14.5106364095724,
132.085311240385)) ;
#144067=CARTESIAN_POINT('Ctrl Pts',(-17.8084089248018,14.4805445911802,
132.361688449539)) ;
#144068=CARTESIAN_POINT('Ctrl Pts',(-17.8862294224432,14.3748126734896,
132.62218433143)) ;
#144069=CARTESIAN_POINT('Ctrl Pts',(-17.9517402542539,14.2005693780012,
132.846713355767)) ;
#144070=CARTESIAN_POINT('Ctrl Pts',(-17.9994948910566,13.9714225005758,
133.019271782795)) ;
#144071=CARTESIAN_POINT('Ctrl Pts',(-18.0255718526998,13.7016038518799,
133.128682790687)) ;
#144072=CARTESIAN_POINT('Ctrl Pts',(-18.0271841884768,13.4137877751622,
133.166386118846)) ;
#144073=CARTESIAN_POINT('Ctrl Pts',(-18.0035377111098,13.1249621012608,
133.130508208661)) ;
#144074=CARTESIAN_POINT('Ctrl Pts',(-17.9558148290788,12.8587597894488,
133.024127137134)) ;
#144075=CARTESIAN_POINT('Ctrl Pts',(-17.8859782679843,12.6311848852698,
132.853419690908)) ;
#144076=CARTESIAN_POINT('Ctrl Pts',(-17.7993724447725,12.462061420416,132.633456990691)) ;
#144077=CARTESIAN_POINT('Ctrl Pts',(-17.7005818136129,12.3611529098997,
132.378046477399)) ;
#144078=CARTESIAN_POINT('Ctrl Pts',(-17.5968820347917,12.3364027391132,
132.10810046349)) ;
#144079=CARTESIAN_POINT('Ctrl Pts',(-17.4934737132323,12.3896955050154,
131.839314298154)) ;
#144080=CARTESIAN_POINT('Ctrl Pts',(-17.3986186118639,12.5169546340526,
131.595303735162)) ;
#144081=CARTESIAN_POINT('Ctrl Pts',(-17.3176313423662,12.709001546384,131.391832952582)) ;
#144082=CARTESIAN_POINT('Ctrl Pts',(-17.2557611142785,12.9518210421532,
131.244157189681)) ;
#144083=CARTESIAN_POINT('Ctrl Pts',(-17.2165247568354,13.2283912816006,
131.162618305046)) ;
#144084=CARTESIAN_POINT('Ctrl Pts',(-17.2020566522433,13.5192446194064,
131.153474543528)) ;
#144085=CARTESIAN_POINT('Ctrl Pts',(-17.2127416793211,13.8035931145738,
131.217849752997)) ;
#144086=CARTESIAN_POINT('Ctrl Pts',(-17.2472308211586,14.0607676757129,
131.351799133051)) ;
#144087=CARTESIAN_POINT('Ctrl Pts',(-17.3018010878718,14.2709777793726,
131.544193934465)) ;
#144088=CARTESIAN_POINT('Ctrl Pts',(-17.3726941931638,14.4220258992613,
131.784554671216)) ;
#144089=CARTESIAN_POINT('Ctrl Pts',(-17.4533630606129,14.5004900232679,
132.053331540465)) ;
#144090=CARTESIAN_POINT('Ctrl Pts',(-17.5372064933208,14.5020985489184,
132.331265024116)) ;
#144091=CARTESIAN_POINT('Ctrl Pts',(-17.6181545095247,14.4266675394507,
132.600862510344)) ;
#144092=CARTESIAN_POINT('Ctrl Pts',(-17.6895299584939,14.2786156866751,
132.842598856471)) ;
#144093=CARTESIAN_POINT('Ctrl Pts',(-17.7450422967288,14.0697688504795,
133.037872094707)) ;
#144094=CARTESIAN_POINT('Ctrl Pts',(-17.7803002307335,13.8142974441725,
133.174023505257)) ;
#144095=CARTESIAN_POINT('Ctrl Pts',(-17.7919769771061,13.5318060155786,
133.241168052371)) ;
#144096=CARTESIAN_POINT('Ctrl Pts',(-17.7786061454648,13.2403760089107,
133.235279390626)) ;
#144097=CARTESIAN_POINT('Ctrl Pts',(-17.7401864120296,12.9618560085294,
133.156243590285)) ;
#144098=CARTESIAN_POINT('Ctrl Pts',(-17.6790471041912,12.7173262571543,
133.010725408051)) ;
#144099=CARTESIAN_POINT('Ctrl Pts',(-17.598858303532,12.5233446116289,132.809527661974)) ;
#144100=CARTESIAN_POINT('Ctrl Pts',(-17.5042403431588,12.3931311939353,
132.566278115897)) ;
#144101=CARTESIAN_POINT('Ctrl Pts',(-17.4011692780146,12.3370752417009,
132.298424229784)) ;
#144102=CARTESIAN_POINT('Ctrl Pts',(-17.297611106788,12.35867646463,132.028824194911)) ;
#144103=CARTESIAN_POINT('Ctrl Pts',(-17.1985322921028,12.4563696655718,
131.772543585188)) ;
#144104=CARTESIAN_POINT('Ctrl Pts',(-17.1110977243364,12.6234424548744,
131.550255293278)) ;
#144105=CARTESIAN_POINT('Ctrl Pts',(-17.0406693325323,12.8484690633149,
131.377731534728)) ;
#144106=CARTESIAN_POINT('Ctrl Pts',(-16.9919310653804,13.1134860837276,
131.268405229023)) ;
#144107=CARTESIAN_POINT('Ctrl Pts',(-16.9672563212509,13.4024250602232,
131.229587957196)) ;
#144108=CARTESIAN_POINT('Ctrl Pts',(-16.967880389663,13.6901681965896,131.264353710665)) ;
#144109=CARTESIAN_POINT('Ctrl Pts',(-16.9930208750078,13.9614083334907,
131.371055961702)) ;
#144110=CARTESIAN_POINT('Ctrl Pts',(-17.0400006387744,14.1924050626967,
131.541350722063)) ;
#144111=CARTESIAN_POINT('Ctrl Pts',(-17.1047498618222,14.3688010138631,
131.763584208451)) ;
#144112=CARTESIAN_POINT('Ctrl Pts',(-17.1821740977121,14.4776662108143,
132.022923082352)) ;
#144113=CARTESIAN_POINT('Ctrl Pts',(-17.2655114072571,14.5108828487548,
132.29941621485)) ;
#144114=CARTESIAN_POINT('Ctrl Pts',(-17.3486749040906,14.4662997659133,
132.575529076312)) ;
#144115=CARTESIAN_POINT('Ctrl Pts',(-17.424537978016,14.3468724175,132.830268759673)) ;
#144116=CARTESIAN_POINT('Ctrl Pts',(-17.487015387752,14.1616148952727,133.045867001742)) ;
#144117=CARTESIAN_POINT('Ctrl Pts',(-17.5310816258823,13.9230022148217,
133.20775448503)) ;
#144118=CARTESIAN_POINT('Ctrl Pts',(-17.5526588839964,13.6485313215457,
133.303938527978)) ;
#144119=CARTESIAN_POINT('Ctrl Pts',(-17.5495272912202,13.3583010704495,
133.327897885114)) ;
#144120=CARTESIAN_POINT('Ctrl Pts',(-17.5212236932149,13.0725041550786,
133.278343292719)) ;
#144121=CARTESIAN_POINT('Ctrl Pts',(-17.4689241155059,12.8117565584391,
133.158715640019)) ;
#144122=CARTESIAN_POINT('Ctrl Pts',(-17.3961417753446,12.5955170585835,
132.979103295085)) ;
#144123=CARTESIAN_POINT('Ctrl Pts',(-17.3060142614099,12.4369579838143,
132.749182506099)) ;
#144124=CARTESIAN_POINT('Ctrl Pts',(-17.2063706296485,12.3507869319176,
132.491038212779)) ;
#144125=CARTESIAN_POINT('Ctrl Pts',(-17.1019586891201,12.3404899824772,
132.219157468743)) ;
#144126=CARTESIAN_POINT('Ctrl Pts',(-17.0000872852129,12.4078495192289,
131.954676728806)) ;
#144127=CARTESIAN_POINT('Ctrl Pts',(-16.9070324900772,12.548387321603,131.716050913228)) ;
#144128=CARTESIAN_POINT('Ctrl Pts',(-16.8292801740909,12.7513534766359,
131.522034622583)) ;
#144129=CARTESIAN_POINT('Ctrl Pts',(-16.7714279753808,13.0019415175825,
131.386102341255)) ;
#144130=CARTESIAN_POINT('Ctrl Pts',(-16.7367407995622,13.2828870424453,
131.317874613442)) ;
#144131=CARTESIAN_POINT('Ctrl Pts',(-16.7270336805474,13.5743280761341,
131.322668167423)) ;
#144132=CARTESIAN_POINT('Ctrl Pts',(-16.7424845135658,13.8554589732171,
131.401028165635)) ;
#144133=CARTESIAN_POINT('Ctrl Pts',(-16.7808557497941,14.1037392604584,
131.546099387152)) ;
#144134=CARTESIAN_POINT('Ctrl Pts',(-16.8390183501908,14.3046991320609,
131.749149752379)) ;
#144135=CARTESIAN_POINT('Ctrl Pts',(-16.9122058795314,14.4424189349425,
131.99615822982)) ;
#144136=CARTESIAN_POINT('Ctrl Pts',(-16.993748194292,14.5067209378496,132.267376795982)) ;
#144137=CARTESIAN_POINT('Ctrl Pts',(-17.0779887847319,14.4936392386325,
132.54666448779)) ;
#144138=CARTESIAN_POINT('Ctrl Pts',(-17.1574333119646,14.4040066761143,
132.811811758465)) ;
#144139=CARTESIAN_POINT('Ctrl Pts',(-17.2262595929588,14.2433941808528,
133.046100374082)) ;
#144140=CARTESIAN_POINT('Ctrl Pts',(-17.2781278639299,14.0252992108477,
133.230624486337)) ;
#144141=CARTESIAN_POINT('Ctrl Pts',(-17.3092719455246,13.7626962224851,
133.354817881569)) ;
#144142=CARTESIAN_POINT('Ctrl Pts',(-17.316267594569,13.4766512855246,133.408344106023)) ;
#144143=CARTESIAN_POINT('Ctrl Pts',(-17.2981853151813,13.186696570853,133.388620530966)) ;
#144144=CARTESIAN_POINT('Ctrl Pts',(-17.2551278866597,12.9123106604455,
133.296117275778)) ;
#144145=CARTESIAN_POINT('Ctrl Pts',(-17.1902973642623,12.676940859845,133.139690042966)) ;
#144146=CARTESIAN_POINT('Ctrl Pts',(-17.1069284764214,12.4935889461196,
132.929262064253)) ;
#144147=CARTESIAN_POINT('Ctrl Pts',(-17.010083943622,12.3766908564608,132.679569553018)) ;
#144148=CARTESIAN_POINT('Ctrl Pts',(-16.9066971430059,12.3352383867213,
132.41063861344)) ;
#144149=CARTESIAN_POINT('Ctrl Pts',(-16.8031994099977,12.3713735993149,
132.141348296765)) ;
#144150=CARTESIAN_POINT('Ctrl Pts',(-16.705881826715,12.482759025907,131.890188907889)) ;
#144151=CARTESIAN_POINT('Ctrl Pts',(-16.6209434982664,12.6627224299211,
131.67535070706)) ;
#144152=CARTESIAN_POINT('Ctrl Pts',(-16.5547338499338,12.8955397907263,
131.514942816909)) ;
#144153=CARTESIAN_POINT('Ctrl Pts',(-16.5103062642366,13.1663559129077,
131.418237368089)) ;
#144154=CARTESIAN_POINT('Ctrl Pts',(-16.4903565413196,13.4563321375684,
131.393122535293)) ;
#144155=CARTESIAN_POINT('Ctrl Pts',(-16.4956768644731,13.7435418421396,
131.441783379302)) ;
#144156=CARTESIAN_POINT('Ctrl Pts',(-16.5251249616778,14.0078637990346,
131.560938657713)) ;
#144157=CARTESIAN_POINT('Ctrl Pts',(-16.5757586121628,14.2299792933114,
131.74192799708)) ;
#144158=CARTESIAN_POINT('Ctrl Pts',(-16.6434535774873,14.3948659933446,
131.97284187312)) ;
#144159=CARTESIAN_POINT('Ctrl Pts',(-16.7225810687213,14.489874104301,132.237167095108)) ;
#144160=CARTESIAN_POINT('Ctrl Pts',(-16.806343644156,14.5084149170405,132.514902816577)) ;
#144161=CARTESIAN_POINT('Ctrl Pts',(-16.8886542888971,14.4492458860129,
132.788526102146)) ;
#144162=CARTESIAN_POINT('Ctrl Pts',(-16.9624159138355,14.3166093969371,
133.037110239956)) ;
#144163=CARTESIAN_POINT('Ctrl Pts',(-17.0218381999614,14.1198899210566,
133.243834706)) ;
#144164=CARTESIAN_POINT('Ctrl Pts',(-17.0618275788481,13.8734077643859,
133.393763574749)) ;
#144165=CARTESIAN_POINT('Ctrl Pts',(-17.0788760119436,13.5947692208086,
133.476671089743)) ;
#144166=CARTESIAN_POINT('Ctrl Pts',(-17.0709959555774,13.3033323132003,
133.486812454175)) ;
#144167=CARTESIAN_POINT('Ctrl Pts',(-17.0379682213309,13.0207082772212,
133.423468632668)) ;
#144168=CARTESIAN_POINT('Ctrl Pts',(-16.9816999774438,12.7676285186634,
133.292133333742)) ;
#144169=CARTESIAN_POINT('Ctrl Pts',(-16.9050914223552,12.5604750217273,
133.101504105218)) ;
#144170=CARTESIAN_POINT('Ctrl Pts',(-16.8128546592574,12.4152915919243,
132.865275428246)) ;
#144171=CARTESIAN_POINT('Ctrl Pts',(-16.7117366179799,12.3428120384338,
132.602892096191)) ;
#144172=CARTESIAN_POINT('Ctrl Pts',(-16.6069387357596,12.3473797731266,
132.329986276711)) ;
#144173=CARTESIAN_POINT('Ctrl Pts',(-16.5062600023837,12.4294696184163,
132.069015423166)) ;
#144174=CARTESIAN_POINT('Ctrl Pts',(-16.4162815450884,12.5816149593444,
131.839131113819)) ;
#144175=CARTESIAN_POINT('Ctrl Pts',(-16.3416786434313,12.7949908749712,
131.654383280298)) ;
#144176=CARTESIAN_POINT('Ctrl Pts',(-16.2877499448409,13.0541013315914,
131.530079485041)) ;
#144177=CARTESIAN_POINT('Ctrl Pts',(-16.2578276039007,13.3386275615382,
131.47577302621)) ;
#144178=CARTESIAN_POINT('Ctrl Pts',(-16.2529639798073,13.6281886067776,
131.494556503773)) ;
#144179=CARTESIAN_POINT('Ctrl Pts',(-16.2727902240412,13.9042250282851,
131.585594807978)) ;
#144180=CARTESIAN_POINT('Ctrl Pts',(-16.3153850284575,14.1463904196779,
131.743221904152)) ;
#144181=CARTESIAN_POINT('Ctrl Pts',(-16.3770706873026,14.3364820143999,
131.956663853719)) ;
#144182=CARTESIAN_POINT('Ctrl Pts',(-16.451653444678,14.4598817897301,132.207420357655)) ;
#144183=CARTESIAN_POINT('Ctrl Pts',(-16.5346837427855,14.5104486172097,
132.483217139684)) ;
#144184=CARTESIAN_POINT('Ctrl Pts',(-16.6185369661693,14.4822486282368,
132.761351628534)) ;
#144185=CARTESIAN_POINT('Ctrl Pts',(-16.6961329602209,14.3791732925603,
133.020987830093)) ;
#144186=CARTESIAN_POINT('Ctrl Pts',(-16.7623831735156,14.2063740239316,
133.247798110192)) ;
#144187=CARTESIAN_POINT('Ctrl Pts',(-16.8107019337629,13.977776586442,133.422085314861)) ;
#144188=CARTESIAN_POINT('Ctrl Pts',(-16.8373185524501,13.7109259547803,
133.5328204031)) ;
#144189=CARTESIAN_POINT('Ctrl Pts',(-16.8396831884313,13.4211174219504,
133.572989902815)) ;
#144190=CARTESIAN_POINT('Ctrl Pts',(-16.8168260927309,13.1336909374666,
133.539218220475)) ;
#144191=CARTESIAN_POINT('Ctrl Pts',(-16.7697357035739,12.8658812614538,
133.434767371646)) ;
#144192=CARTESIAN_POINT('Ctrl Pts',(-16.7003932528539,12.6367690077997,
133.265523679042)) ;
#144193=CARTESIAN_POINT('Ctrl Pts',(-16.6141071851622,12.4658337758404,
133.046525912297)) ;
#144194=CARTESIAN_POINT('Ctrl Pts',(-16.5159102908414,12.363124510772,132.792734881814)) ;
#144195=CARTESIAN_POINT('Ctrl Pts',(-16.4120568421875,12.3360466249849,
132.522413241757)) ;
#144196=CARTESIAN_POINT('Ctrl Pts',(-16.3088888182374,12.3868688211213,
132.254206294469)) ;
#144197=CARTESIAN_POINT('Ctrl Pts',(-16.2136026177267,12.5119418808478,
132.008965625596)) ;
#144198=CARTESIAN_POINT('Ctrl Pts',(-16.1320705940404,12.7021784508198,
131.80390923486)) ;
#144199=CARTESIAN_POINT('Ctrl Pts',(-16.0692715430123,12.9449354906641,
131.653682319898)) ;
#144200=CARTESIAN_POINT('Ctrl Pts',(-16.0294330752892,13.2214385193801,
131.570442661055)) ;
#144201=CARTESIAN_POINT('Ctrl Pts',(-16.0143292105081,13.5108149265418,
131.559283090765)) ;
#144202=CARTESIAN_POINT('Ctrl Pts',(-16.024395738529,13.7968085806489,131.621995082752)) ;
#144203=CARTESIAN_POINT('Ctrl Pts',(-16.0581227273194,14.0536577586376,
131.753546869173)) ;
#144204=CARTESIAN_POINT('Ctrl Pts',(-16.1122503754108,14.2659121796834,
131.944720560037)) ;
#144205=CARTESIAN_POINT('Ctrl Pts',(-16.1826593705253,14.4185013343906,
132.183605873283)) ;
#144206=CARTESIAN_POINT('Ctrl Pts',(-16.2630150868534,14.4992712533562,
132.451430959388)) ;
#144207=CARTESIAN_POINT('Ctrl Pts',(-16.3472138704315,14.5031359858994,
132.730542445583)) ;
#144208=CARTESIAN_POINT('Ctrl Pts',(-16.4282278041652,14.42962012524,133.000297431596)) ;
#144209=CARTESIAN_POINT('Ctrl Pts',(-16.4996649079536,14.2844129921914,
133.242054084249)) ;
#144210=CARTESIAN_POINT('Ctrl Pts',(-16.555935794527,14.07647539704,133.439668505005)) ;
#144211=CARTESIAN_POINT('Ctrl Pts',(-16.5917569598566,13.8227945386488,
133.577374015525)) ;
#144212=CARTESIAN_POINT('Ctrl Pts',(-16.6042213644859,13.5398700971536,
133.646937875095)) ;
#144213=CARTESIAN_POINT('Ctrl Pts',(-16.5915381268133,13.2487715870731,
133.643011550727)) ;
#144214=CARTESIAN_POINT('Ctrl Pts',(-16.5539869821841,12.9703360488667,
133.566419364886)) ;
#144215=CARTESIAN_POINT('Ctrl Pts',(-16.4934594117706,12.724109148074,133.422732551231)) ;
#144216=CARTESIAN_POINT('Ctrl Pts',(-16.4135452640998,12.5279170556122,
133.222424143852)) ;
#144217=CARTESIAN_POINT('Ctrl Pts',(-16.3193068200252,12.3959938215062,
132.980258046712)) ;
#144218=CARTESIAN_POINT('Ctrl Pts',(-16.2168484516887,12.3376260911869,
132.714047247702)) ;
#144219=CARTESIAN_POINT('Ctrl Pts',(-16.1125041885171,12.3570498023057,
132.442386064704)) ;
#144220=CARTESIAN_POINT('Ctrl Pts',(-16.0135226857535,12.4525560159372,
132.18628157101)) ;
#144221=CARTESIAN_POINT('Ctrl Pts',(-15.925676910732,12.6176036615847,131.962785188827)) ;
#144222=CARTESIAN_POINT('Ctrl Pts',(-15.8546709466239,12.841094749517,131.788566152118)) ;
#144223=CARTESIAN_POINT('Ctrl Pts',(-15.8052367164706,13.1055203905307,
131.677249540122)) ;
#144224=CARTESIAN_POINT('Ctrl Pts',(-15.7798623786128,13.3928980582864,
131.636249531326)) ;
#144225=CARTESIAN_POINT('Ctrl Pts',(-15.7797414082747,13.682454377304,131.66902224139)) ;
#144226=CARTESIAN_POINT('Ctrl Pts',(-15.8040952873856,13.953269278216,131.773267748027)) ;
#144227=CARTESIAN_POINT('Ctrl Pts',(-15.8505306674575,14.1862511207232,
131.942048548818)) ;
#144228=CARTESIAN_POINT('Ctrl Pts',(-15.9147431639295,14.3643962047435,
132.162676232254)) ;
#144229=CARTESIAN_POINT('Ctrl Pts',(-15.9923526478993,14.4759024798905,
132.42275165957)) ;
#144230=CARTESIAN_POINT('Ctrl Pts',(-16.0753259172169,14.5109062470025,
132.698063584178)) ;
#144231=CARTESIAN_POINT('Ctrl Pts',(-16.1585231199198,14.4687351613561,
132.974244296309)) ;
#144232=CARTESIAN_POINT('Ctrl Pts',(-16.2347182143026,14.3512437869113,
133.229975033208)) ;
#144233=CARTESIAN_POINT('Ctrl Pts',(-16.2976212045528,14.1681343320696,
133.446767765667)) ;
#144234=CARTESIAN_POINT('Ctrl Pts',(-16.342496750101,13.9291093087556,133.611240379679)) ;
#144235=CARTESIAN_POINT('Ctrl Pts',(-16.3645583959615,13.6572014758575,
133.708608822739)) ;
#144236=CARTESIAN_POINT('Ctrl Pts',(-16.3621600211972,13.3659145810937,
133.734856792979)) ;
#144237=CARTESIAN_POINT('Ctrl Pts',(-16.3346204183379,13.0809590498869,
133.687391258314)) ;
#144238=CARTESIAN_POINT('Ctrl Pts',(-16.2830794550255,12.8188858312814,
133.569993158216)) ;
#144239=CARTESIAN_POINT('Ctrl Pts',(-16.2101996415637,12.5999509531083,
133.390335016311)) ;
#144240=CARTESIAN_POINT('Ctrl Pts',(-16.1215938088304,12.441498416931,133.164439212171)) ;
#144241=CARTESIAN_POINT('Ctrl Pts',(-16.0216086754502,12.3520342804443,
132.90550795831)) ;
#144242=CARTESIAN_POINT('Ctrl Pts',(-15.9169354902678,12.339805477818,132.632949304706)) ;
#144243=CARTESIAN_POINT('Ctrl Pts',(-15.8152636813313,12.404786593097,132.368936116434)) ;
#144244=CARTESIAN_POINT('Ctrl Pts',(-15.7218412987795,12.543193504082,132.129236118801)) ;
#144245=CARTESIAN_POINT('Ctrl Pts',(-15.6435355946438,12.7444967223723,
131.933608263687)) ;
#144246=CARTESIAN_POINT('Ctrl Pts',(-15.5849489993876,12.9945027181083,
131.795604404436)) ;
#144247=CARTESIAN_POINT('Ctrl Pts',(-15.5495839140457,13.2745331235142,
131.725353632572)) ;
#144248=CARTESIAN_POINT('Ctrl Pts',(-15.5392180445128,13.5670628518901,
131.72835389432)) ;
#144249=CARTESIAN_POINT('Ctrl Pts',(-15.5537810725356,13.8462372757585,
131.803808377595)) ;
#144250=CARTESIAN_POINT('Ctrl Pts',(-15.5917625445911,14.0979242906841,
131.948022870834)) ;
#144251=CARTESIAN_POINT('Ctrl Pts',(-15.6494094412975,14.299738463193,132.149495635102)) ;
#144252=CARTESIAN_POINT('Ctrl Pts',(-15.7219689570077,14.4393312892027,
132.394565274966)) ;
#144253=CARTESIAN_POINT('Ctrl Pts',(-15.8039842180224,14.5060643737482,
132.667421219409)) ;
#144254=CARTESIAN_POINT('Ctrl Pts',(-15.8876335375387,14.4951758470579,
132.94472806509)) ;
#144255=CARTESIAN_POINT('Ctrl Pts',(-15.9676762287012,14.4072622582047,
133.211792898155)) ;
#144256=CARTESIAN_POINT('Ctrl Pts',(-16.036543722577,14.2495038720977,133.44600603181)) ;
#144257=CARTESIAN_POINT('Ctrl Pts',(-16.089366133658,14.0308220187667,133.633622691749)) ;
#144258=CARTESIAN_POINT('Ctrl Pts',(-16.120792732328,13.7719099555025,133.758281534103)) ;
#144259=CARTESIAN_POINT('Ctrl Pts',(-16.1286533928309,13.4847455489294,
133.814530120636)) ;
#144260=CARTESIAN_POINT('Ctrl Pts',(-16.1113129075323,13.1955424238471,
133.796861187968)) ;
#144261=CARTESIAN_POINT('Ctrl Pts',(-16.0689855848103,12.9200552439899,
133.706524257301)) ;
#144262=CARTESIAN_POINT('Ctrl Pts',(-16.0046877923632,12.6831184051196,
133.551684114638)) ;
#144263=CARTESIAN_POINT('Ctrl Pts',(-15.9217483090797,12.4980281051702,
133.342521067972)) ;
#144264=CARTESIAN_POINT('Ctrl Pts',(-15.8254049942899,12.3791543391629,
133.094225998351)) ;
#144265=CARTESIAN_POINT('Ctrl Pts',(-15.7218252727384,12.3353503724763,
132.824832082411)) ;
#144266=CARTESIAN_POINT('Ctrl Pts',(-15.6183467338859,12.3691099624238,
132.555553737279)) ;
#144267=CARTESIAN_POINT('Ctrl Pts',(-15.5201912749977,12.4795856754925,
132.302167330869)) ;
#144268=CARTESIAN_POINT('Ctrl Pts',(-15.4359387494791,12.655336096254,132.088880801219)) ;
#144269=CARTESIAN_POINT('Ctrl Pts',(-15.3684950766273,12.8882259195335,
131.925126605676)) ;
#144270=CARTESIAN_POINT('Ctrl Pts',(-15.3234771421884,13.1581921439883,
131.826674404974)) ;
#144271=CARTESIAN_POINT('Ctrl Pts',(-15.3027810611371,13.4482190553547,
131.799417903735)) ;
#144272=CARTESIAN_POINT('Ctrl Pts',(-15.3073896332409,13.7352663481711,
131.845937422089)) ;
#144273=CARTESIAN_POINT('Ctrl Pts',(-15.3361366056611,14.0004787801146,
131.963037517509)) ;
#144274=CARTESIAN_POINT('Ctrl Pts',(-15.3861846693765,14.224240187898,132.1423230941)) ;
#144275=CARTESIAN_POINT('Ctrl Pts',(-15.4537984970937,14.391486040761,132.373145815163)) ;
#144276=CARTESIAN_POINT('Ctrl Pts',(-15.5322488697613,14.4880342043903,
132.635302336254)) ;
#144277=CARTESIAN_POINT('Ctrl Pts',(-15.6162814316108,14.508976716731,132.913959445703)) ;
#144278=CARTESIAN_POINT('Ctrl Pts',(-15.6984885960337,14.4520806960152,
133.187177926299)) ;
#144279=CARTESIAN_POINT('Ctrl Pts',(-15.7726891524608,14.3213934161067,
133.437089396067)) ;
#144280=CARTESIAN_POINT('Ctrl Pts',(-15.832567950564,14.1264275067293,133.645128594592)) ;
#144281=CARTESIAN_POINT('Ctrl Pts',(-15.8732541213187,13.8807879238241,
133.797144869293)) ;
#144282=CARTESIAN_POINT('Ctrl Pts',(-15.8909376658887,13.6022564662603,
133.88196368139)) ;
#144283=CARTESIAN_POINT('Ctrl Pts',(-15.8838084227577,13.3123737627951,
133.894129173828)) ;
#144284=CARTESIAN_POINT('Ctrl Pts',(-15.8515754461964,13.0290002093282,
133.833124538385)) ;
#144285=CARTESIAN_POINT('Ctrl Pts',(-15.7957904346099,12.7741269018416,
133.703288589335)) ;
#144286=CARTESIAN_POINT('Ctrl Pts',(-15.7197425124795,12.5657350925596,
133.514264692283)) ;
#144287=CARTESIAN_POINT('Ctrl Pts',(-15.6282416938175,12.4188761283997,
133.28006727262)) ;
#144288=CARTESIAN_POINT('Ctrl Pts',(-15.5269267217761,12.3438128182006,
133.017238568564)) ;
#144289=CARTESIAN_POINT('Ctrl Pts',(-15.4225146726752,12.346102551177,132.745334035542)) ;
#144290=CARTESIAN_POINT('Ctrl Pts',(-15.3215773838207,12.4255736713201,
132.483612778592)) ;
#144291=CARTESIAN_POINT('Ctrl Pts',(-15.2307667619573,12.5765458005785,
132.251460050158)) ;
#144292=CARTESIAN_POINT('Ctrl Pts',(-15.1558846692699,12.7879288159169,
132.065806337038)) ;
#144293=CARTESIAN_POINT('Ctrl Pts',(-15.1014092188235,13.0448055751977,
131.939778233867)) ;
#144294=CARTESIAN_POINT('Ctrl Pts',(-15.0705529522139,13.3297564879043,
131.882857829171)) ;
#144295=CARTESIAN_POINT('Ctrl Pts',(-15.0649638067235,13.6201108686768,
131.899596243117)) ;
#144296=CARTESIAN_POINT('Ctrl Pts',(-15.0841303044588,13.8967555620889,
131.988701102709)) ;
#144297=CARTESIAN_POINT('Ctrl Pts',(-15.1259754124002,14.1394984275279,
132.144042294626)) ;
#144298=CARTESIAN_POINT('Ctrl Pts',(-15.1870982940081,14.3315002121409,
132.355832850618)) ;
#144299=CARTESIAN_POINT('Ctrl Pts',(-15.2616606243926,14.4575223198637,
132.606660509906)) ;
#144300=CARTESIAN_POINT('Ctrl Pts',(-15.3446502895168,14.5099977953481,
132.882369335938)) ;
#144301=CARTESIAN_POINT('Ctrl Pts',(-15.4281132070526,14.4843800737971,
133.159177027372)) ;
#144302=CARTESIAN_POINT('Ctrl Pts',(-15.5064015464553,14.3828781274989,
133.421023569231)) ;
#144303=CARTESIAN_POINT('Ctrl Pts',(-15.5726872563074,14.2128161512202,
133.647745598719)) ;
#144304=CARTESIAN_POINT('Ctrl Pts',(-15.6217981618111,13.9854781588929,
133.824413847127)) ;
#144305=CARTESIAN_POINT('Ctrl Pts',(-15.6491464955149,13.7179644901035,
133.937462255945)) ;
#144306=CARTESIAN_POINT('Ctrl Pts',(-15.6521578575077,13.4301920421151,
133.979322612002)) ;
#144307=CARTESIAN_POINT('Ctrl Pts',(-15.6301625185461,13.1421055702502,
133.948099015158)) ;
#144308=CARTESIAN_POINT('Ctrl Pts',(-15.5832226689965,12.871501287512,133.844351996978)) ;
#144309=CARTESIAN_POINT('Ctrl Pts',(-15.5151730259063,12.6436097972574,
133.678515535288)) ;
#144310=CARTESIAN_POINT('Ctrl Pts',(-15.4290810051553,12.469849836909,133.460215264565)) ;
#144311=CARTESIAN_POINT('Ctrl Pts',(-15.3311482913841,12.3651221790713,
133.207186335415)) ;
#144312=CARTESIAN_POINT('Ctrl Pts',(-15.2272564454248,12.3356922244687,
132.936789720777)) ;
#144313=CARTESIAN_POINT('Ctrl Pts',(-15.1239058803988,12.3844432220599,
132.668069533847)) ;
#144314=CARTESIAN_POINT('Ctrl Pts',(-15.0285056070021,12.5072148267233,
132.422427919904)) ;
#144315=CARTESIAN_POINT('Ctrl Pts',(-14.9464192845507,12.695755079112,132.215771718577)) ;
#144316=CARTESIAN_POINT('Ctrl Pts',(-14.8830378580334,12.9373000432248,
132.063847131515)) ;
#144317=CARTESIAN_POINT('Ctrl Pts',(-14.8425232798133,13.2121500744088,
131.978527590025)) ;
#144318=CARTESIAN_POINT('Ctrl Pts',(-14.8266372192779,13.503246650252,131.96529981272)) ;
#144319=CARTESIAN_POINT('Ctrl Pts',(-14.8358595928672,13.7871081777778,
132.025232619903)) ;
#144320=CARTESIAN_POINT('Ctrl Pts',(-14.8690306285163,14.04691061429,132.155386588116)) ;
#144321=CARTESIAN_POINT('Ctrl Pts',(-14.922645952623,14.260565028937,132.345047723229)) ;
#144322=CARTESIAN_POINT('Ctrl Pts',(-14.9928707940905,14.4153650292754,
132.583485979597)) ;
#144323=CARTESIAN_POINT('Ctrl Pts',(-15.0727028439604,14.4978583100618,
132.849642817734)) ;
#144324=CARTESIAN_POINT('Ctrl Pts',(-15.1568916183296,14.5041773759635,
133.128731323045)) ;
#144325=CARTESIAN_POINT('Ctrl Pts',(-15.2381267118911,14.4329778405108,
133.399139072621)) ;
#144326=CARTESIAN_POINT('Ctrl Pts',(-15.310215281974,14.2890421003468,133.642938749112)) ;
#144327=CARTESIAN_POINT('Ctrl Pts',(-15.3668446015009,14.0827792612075,
133.841549772997)) ;
#144328=CARTESIAN_POINT('Ctrl Pts',(-15.403218936125,13.830933510425,133.980781224856)) ;
#144329=CARTESIAN_POINT('Ctrl Pts',(-15.416422867439,13.5483118095736,134.052537966208)) ;
#144330=CARTESIAN_POINT('Ctrl Pts',(-15.4045116247788,13.2574775512287,
134.050827634668)) ;
#144331=CARTESIAN_POINT('Ctrl Pts',(-15.3675972987209,12.9779695749568,
133.976150837606)) ;
#144332=CARTESIAN_POINT('Ctrl Pts',(-15.3079074469604,12.7311578821155,
133.834812535713)) ;
#144333=CARTESIAN_POINT('Ctrl Pts',(-15.2281264002969,12.5323979618,133.635048294444)) ;
#144334=CARTESIAN_POINT('Ctrl Pts',(-15.1345460077119,12.3989896763175,
133.394682225535)) ;
#144335=CARTESIAN_POINT('Ctrl Pts',(-15.0320366735209,12.3382487508946,
133.128394076734)) ;
#144336=CARTESIAN_POINT('Ctrl Pts',(-14.9280016502807,12.3552058345121,
132.85751876148)) ;
#144337=CARTESIAN_POINT('Ctrl Pts',(-14.828126334543,12.449068120654,132.599017361818)) ;
#144338=CARTESIAN_POINT('Ctrl Pts',(-14.7399179314426,12.6128543666523,
132.374483440093)) ;
#144339=CARTESIAN_POINT('Ctrl Pts',(-14.6688184323609,12.8333918946772,
132.199772246187)) ;
#144340=CARTESIAN_POINT('Ctrl Pts',(-14.6185220942431,13.0975419716129,
132.086034661743)) ;
#144341=CARTESIAN_POINT('Ctrl Pts',(-14.5924589370379,13.38437019925,132.042997984616)) ;
#144342=CARTESIAN_POINT('Ctrl Pts',(-14.5916118196615,13.6749248877936,
132.073736568238)) ;
#144343=CARTESIAN_POINT('Ctrl Pts',(-14.615388619572,13.9463602698171,132.17629151353)) ;
#144344=CARTESIAN_POINT('Ctrl Pts',(-14.6609947039576,14.179832441143,132.34250644721)) ;
#144345=CARTESIAN_POINT('Ctrl Pts',(-14.7251736432412,14.3606302747574,
132.563238264022)) ;
#144346=CARTESIAN_POINT('Ctrl Pts',(-14.8018119805842,14.4733618846649,
132.820176750005)) ;
#144347=CARTESIAN_POINT('Ctrl Pts',(-14.8854691744736,14.5110756603655,
133.097804799088)) ;
#144348=CARTESIAN_POINT('Ctrl Pts',(-14.9682970766034,14.4709889018576,
133.372719303669)) ;
#144349=CARTESIAN_POINT('Ctrl Pts',(-15.0449564076789,14.3556941953622,
133.629862494971)) ;
#144350=CARTESIAN_POINT('Ctrl Pts',(-15.108481062133,14.1731666349653,133.848613132394)) ;
#144351=CARTESIAN_POINT('Ctrl Pts',(-15.1535160847987,13.9378583888153,
134.013218034185)) ;
#144352=CARTESIAN_POINT('Ctrl Pts',(-15.1764968053545,13.665635486159,134.113428205125)) ;
#144353=CARTESIAN_POINT('Ctrl Pts',(-15.1748102635303,13.3744562424158,
134.141758613948)) ;
#144354=CARTESIAN_POINT('Ctrl Pts',(-15.1479237720966,13.0885611024712,
134.096264872109)) ;
#144355=CARTESIAN_POINT('Ctrl Pts',(-15.097140483322,12.8263305673749,133.980986925495)) ;
#144356=CARTESIAN_POINT('Ctrl Pts',(-15.0251820302,12.6063806997543,133.803901483058)) ;
#144357=CARTESIAN_POINT('Ctrl Pts',(-14.9363600437793,12.4447492337382,
133.577614824626)) ;
#144358=CARTESIAN_POINT('Ctrl Pts',(-14.8365909935855,12.353502559508,133.319303022106)) ;
#144359=CARTESIAN_POINT('Ctrl Pts',(-14.7321331307677,12.3391045182876,
133.04731904121)) ;
#144360=CARTESIAN_POINT('Ctrl Pts',(-14.6302798500926,12.4018104838522,
132.782777505341)) ;
#144361=CARTESIAN_POINT('Ctrl Pts',(-14.5362174086835,12.5389587593729,
132.541328494992)) ;
#144362=CARTESIAN_POINT('Ctrl Pts',(-14.4578519480753,12.7377765995817,
132.345359393595)) ;
#144363=CARTESIAN_POINT('Ctrl Pts',(-14.3986096579226,12.9863021610025,
132.205418010863)) ;
#144364=CARTESIAN_POINT('Ctrl Pts',(-14.3624943762826,13.26603407284,132.133014222054)) ;
#144365=CARTESIAN_POINT('Ctrl Pts',(-14.3513554744166,13.5582234410802,
132.133715470598)) ;
#144366=CARTESIAN_POINT('Ctrl Pts',(-14.3652841770306,13.8387406073518,
132.20741478973)) ;
#144367=CARTESIAN_POINT('Ctrl Pts',(-14.402398537324,14.0904926888755,132.348933832789)) ;
#144368=CARTESIAN_POINT('Ctrl Pts',(-14.4599824766091,14.2955137272415,
132.550485329431)) ;
#144369=CARTESIAN_POINT('Ctrl Pts',(-14.5318636954427,14.4360007562524,
132.793394148)) ;
#144370=CARTESIAN_POINT('Ctrl Pts',(-14.6134847888935,14.5051703131075,
133.065024459182)) ;
#144371=CARTESIAN_POINT('Ctrl Pts',(-14.6974445904021,14.4966323444729,
133.34334938671)) ;
#144372=CARTESIAN_POINT('Ctrl Pts',(-14.7777292058018,14.4108290646986,
133.611127666164)) ;
#144373=CARTESIAN_POINT('Ctrl Pts',(-14.8470034884994,14.2547208432748,
133.846555378337)) ;
#144374=CARTESIAN_POINT('Ctrl Pts',(-14.9001526523347,14.0388604849956,
134.034948538747)) ;
#144375=CARTESIAN_POINT('Ctrl Pts',(-14.9324920252192,13.7794054501878,
134.162484960282)) ;
#144376=CARTESIAN_POINT('Ctrl Pts',(-14.9409722546491,13.4926640432345,
134.220533515023)) ;
#144377=CARTESIAN_POINT('Ctrl Pts',(-14.9243598314647,13.2038301120676,
134.204936121479)) ;
#144378=CARTESIAN_POINT('Ctrl Pts',(-14.8828700391429,12.9280759212708,
134.116976868931)) ;
#144379=CARTESIAN_POINT('Ctrl Pts',(-14.8188908380602,12.6887447030163,
133.963216320727)) ;
#144380=CARTESIAN_POINT('Ctrl Pts',(-14.7363827544312,12.5022966098147,
133.755297039805)) ;
#144381=CARTESIAN_POINT('Ctrl Pts',(-14.6407612364118,12.3817639702232,
133.508972013868)) ;
#144382=CARTESIAN_POINT('Ctrl Pts',(-14.5369394844871,12.3354318122153,
133.238985783327)) ;
#144383=CARTESIAN_POINT('Ctrl Pts',(-14.4335611887344,12.3672035542546,
132.969949082775)) ;
#144384=CARTESIAN_POINT('Ctrl Pts',(-14.3356308343994,12.4744264817991,
132.717025526438)) ;
#144385=CARTESIAN_POINT('Ctrl Pts',(-14.2499549471161,12.6503068789,132.499956654344)) ;
#144386=CARTESIAN_POINT('Ctrl Pts',(-14.1823507038926,12.88124813694,132.335597188222)) ;
#144387=CARTESIAN_POINT('Ctrl Pts',(-14.1367086423717,13.1494231043328,
132.235222082954)) ;
#144388=CARTESIAN_POINT('Ctrl Pts',(-14.1151990196335,13.4405328336443,
132.205741664821)) ;
#144389=CARTESIAN_POINT('Ctrl Pts',(-14.1191469684865,13.7272524235385,
132.250255662763)) ;
#144390=CARTESIAN_POINT('Ctrl Pts',(-14.1472055291928,13.9933198018618,
132.365337276901)) ;
#144391=CARTESIAN_POINT('Ctrl Pts',(-14.1966526863445,14.2183989347204,
132.542845561358)) ;
#144392=CARTESIAN_POINT('Ctrl Pts',(-14.263893080412,14.3876287809154,132.772603151364)) ;
#144393=CARTESIAN_POINT('Ctrl Pts',(-14.3419899874594,14.4861871139801,
133.033682078537)) ;
#144394=CARTESIAN_POINT('Ctrl Pts',(-14.4260278724583,14.5095212263095,
133.312380013365)) ;
#144395=CARTESIAN_POINT('Ctrl Pts',(-14.5084628588285,14.4547286941079,
133.586299917709)) ;
#144396=CARTESIAN_POINT('Ctrl Pts',(-14.5829405589946,14.3261104850367,
133.837000847086)) ;
#144397=CARTESIAN_POINT('Ctrl Pts',(-14.6433221281086,14.1327423956962,
134.046521365604)) ;
#144398=CARTESIAN_POINT('Ctrl Pts',(-14.6845889897072,13.8885304573601,
134.200204530242)) ;
#144399=CARTESIAN_POINT('Ctrl Pts',(-14.7029647633418,13.6107522710193,
134.28704040231)) ;
#144400=CARTESIAN_POINT('Ctrl Pts',(-14.6966560072645,13.3210540758006,
134.301585228587)) ;
#144401=CARTESIAN_POINT('Ctrl Pts',(-14.6647660833951,13.0351249391052,
134.241836648231)) ;
#144402=CARTESIAN_POINT('Ctrl Pts',(-14.6100670255446,12.7816148571452,
134.114864586357)) ;
#144403=CARTESIAN_POINT('Ctrl Pts',(-14.534310267785,12.5706516748794,133.926826881026)) ;
#144404=CARTESIAN_POINT('Ctrl Pts',(-14.4432001449626,12.4220918167394,
133.693747165107)) ;
#144405=CARTESIAN_POINT('Ctrl Pts',(-14.3419526728907,12.3448083545055,
133.431156912992)) ;
#144406=CARTESIAN_POINT('Ctrl Pts',(-14.2375927674014,12.3450375900235,
133.159386644344)) ;
#144407=CARTESIAN_POINT('Ctrl Pts',(-14.1366243467377,12.4222141215766,
132.897520934609)) ;
#144408=CARTESIAN_POINT('Ctrl Pts',(-14.0453864330863,12.5713074000372,
132.664137827729)) ;
#144409=CARTESIAN_POINT('Ctrl Pts',(-13.9699446216825,12.7812070105723,
132.47686000557)) ;
#144410=CARTESIAN_POINT('Ctrl Pts',(-13.9147092621739,13.0378488607775,
132.348709030643)) ;
#144411=CARTESIAN_POINT('Ctrl Pts',(-13.8832871777118,13.3220974223082,
132.290103709443)) ;
#144412=CARTESIAN_POINT('Ctrl Pts',(-13.8769825405473,13.611647883706,132.304649018805)) ;
#144413=CARTESIAN_POINT('Ctrl Pts',(-13.8955086499777,13.8896345343945,
132.39196295235)) ;
#144414=CARTESIAN_POINT('Ctrl Pts',(-13.9366753833046,14.1329049356831,
132.54523713465)) ;
#144415=CARTESIAN_POINT('Ctrl Pts',(-13.9972054024135,14.3266158098986,
132.755265210383)) ;
#144416=CARTESIAN_POINT('Ctrl Pts',(-14.0717046716822,14.4550272244897,
133.006018843489)) ;
#144417=CARTESIAN_POINT('Ctrl Pts',(-14.1542914623274,14.5094869188899,
133.280440740806)) ;
#144418=CARTESIAN_POINT('Ctrl Pts',(-14.23786007523,14.4863254941317,133.55757350622)) ;
#144419=CARTESIAN_POINT('Ctrl Pts',(-14.3164953259384,14.3868080621077,
133.820474949002)) ;
#144420=CARTESIAN_POINT('Ctrl Pts',(-14.3832481636959,14.2186053489218,
134.048567565763)) ;
#144421=CARTESIAN_POINT('Ctrl Pts',(-14.433013492223,13.9916146636668,134.227276700998)) ;
#144422=CARTESIAN_POINT('Ctrl Pts',(-14.4608459895121,13.7271394613145,
134.341473276466)) ;
#144423=CARTESIAN_POINT('Ctrl Pts',(-14.4646255722011,13.4373621630931,
134.385853195471)) ;
#144424=CARTESIAN_POINT('Ctrl Pts',(-14.443349249692,13.1504054567353,134.35656690841)) ;
#144425=CARTESIAN_POINT('Ctrl Pts',(-14.3970798767142,12.8786465082132,
134.254813797913)) ;
#144426=CARTESIAN_POINT('Ctrl Pts',(-14.3297712578551,12.6500332847712,
134.091052737694)) ;
#144427=CARTESIAN_POINT('Ctrl Pts',(-14.2443077145905,12.4743183889617,
133.874546811681)) ;
#144428=CARTESIAN_POINT('Ctrl Pts',(-14.1459829063076,12.3668547885935,
133.620592382301)) ;
#144429=CARTESIAN_POINT('Ctrl Pts',(-14.0426593854965,12.3355629410877,
133.35169506941)) ;
#144430=CARTESIAN_POINT('Ctrl Pts',(-13.9392469880479,12.3817108160481,
133.082773805456)) ;
#144431=CARTESIAN_POINT('Ctrl Pts',(-13.843143436717,12.5028398511796,132.835204825882)) ;
#144432=CARTESIAN_POINT('Ctrl Pts',(-13.7605436154981,12.6903514923922,
132.627110847511)) ;
#144433=CARTESIAN_POINT('Ctrl Pts',(-13.6970335294607,12.9285060131068,
132.474531325953)) ;
#144434=CARTESIAN_POINT('Ctrl Pts',(-13.6554462176405,13.2046732930674,
132.386338568047)) ;
#144435=CARTESIAN_POINT('Ctrl Pts',(-13.6389656541903,13.4951334329262,
132.371307889567)) ;
#144436=CARTESIAN_POINT('Ctrl Pts',(-13.6475068620829,13.7795013395347,
132.429266393857)) ;
#144437=CARTESIAN_POINT('Ctrl Pts',(-13.679877816188,14.0394109591315,132.556955498111)) ;
#144438=CARTESIAN_POINT('Ctrl Pts',(-13.7330862586516,14.2552142278511,
132.745523563383)) ;
#144439=CARTESIAN_POINT('Ctrl Pts',(-13.8025719368285,14.4112842986504,
132.981643339771)) ;
#144440=CARTESIAN_POINT('Ctrl Pts',(-13.8823995551984,14.4966304081093,
133.247890097308)) ;
#144441=CARTESIAN_POINT('Ctrl Pts',(-13.9669897571776,14.5049768575903,
133.528313290587)) ;
#144442=CARTESIAN_POINT('Ctrl Pts',(-14.0479944860348,14.4360834976797,
133.797890686312)) ;
#144443=CARTESIAN_POINT('Ctrl Pts',(-14.1203483029127,14.2946512650185,
134.04240392863)) ;
#144444=CARTESIAN_POINT('Ctrl Pts',(-14.1776079248902,14.0899138392311,
134.242893869283)) ;
#144445=CARTESIAN_POINT('Ctrl Pts',(-14.2147355846971,13.8386915040984,
134.384396464482)) ;
#144446=CARTESIAN_POINT('Ctrl Pts',(-14.2285960401478,13.5555689993548,
134.45818874425)) ;
#144447=CARTESIAN_POINT('Ctrl Pts',(-14.2174370565147,13.2663899085958,
134.458484095202)) ;
#144448=CARTESIAN_POINT('Ctrl Pts',(-14.1812851642328,12.9858845454111,
134.386068426283)) ;
#144449=CARTESIAN_POINT('Ctrl Pts',(-14.1220605741677,12.737510093137,134.246152635889)) ;
#144450=CARTESIAN_POINT('Ctrl Pts',(-14.0430821999498,12.5376375211986,
134.048618882787)) ;
#144451=CARTESIAN_POINT('Ctrl Pts',(-13.9493516901009,12.4015826391132,
133.807988055911)) ;
#144452=CARTESIAN_POINT('Ctrl Pts',(-13.847485963073,12.3390360778661,133.543416015632)) ;
#144453=CARTESIAN_POINT('Ctrl Pts',(-13.7431811033581,12.3535754317009,
133.271827404683)) ;
#144454=CARTESIAN_POINT('Ctrl Pts',(-13.6431991335962,12.4452741320202,
133.012975789816)) ;
#144455=CARTESIAN_POINT('Ctrl Pts',(-13.5545881261613,12.6067972439988,
132.78723888543)) ;
#144456=CARTESIAN_POINT('Ctrl Pts',(-13.4825179247784,12.8274893323333,
132.609914210707)) ;
#144457=CARTESIAN_POINT('Ctrl Pts',(-13.4319485828918,13.0891409681253,
132.495170039007)) ;
#144458=CARTESIAN_POINT('Ctrl Pts',(-13.405076521648,13.3757401842095,132.449797594403)) ;
#144459=CARTESIAN_POINT('Ctrl Pts',(-13.403495750014,13.6659116467556,132.478325630475)) ;
#144460=CARTESIAN_POINT('Ctrl Pts',(-13.4264445635729,13.9383430933064,
132.578458762523)) ;
#144461=CARTESIAN_POINT('Ctrl Pts',(-13.4718993493954,14.1747318891546,
132.74449081178)) ;
#144462=CARTESIAN_POINT('Ctrl Pts',(-13.5350003238588,14.3556000253484,
132.961746054639)) ;
#144463=CARTESIAN_POINT('Ctrl Pts',(-13.6120266374697,14.4715471838241,
133.220125893983)) ;
#144464=CARTESIAN_POINT('Ctrl Pts',(-13.6950425828247,14.5109306883494,
133.495651568683)) ;
#144465=CARTESIAN_POINT('Ctrl Pts',(-13.7781244502882,14.4734197529204,
133.771367920486)) ;
#144466=CARTESIAN_POINT('Ctrl Pts',(-13.8553206961182,14.3595613324345,
134.030197068802)) ;
#144467=CARTESIAN_POINT('Ctrl Pts',(-13.9189983306387,14.1794661673076,
134.249255457911)) ;
#144468=CARTESIAN_POINT('Ctrl Pts',(-13.9647465680392,13.945518104717,134.415965062651)) ;
#144469=CARTESIAN_POINT('Ctrl Pts',(-13.9884352930972,13.6723045433651,
134.518446435358)) ;
#144470=CARTESIAN_POINT('Ctrl Pts',(-13.9874200608317,13.3834915419228,
134.548487177175)) ;
#144471=CARTESIAN_POINT('Ctrl Pts',(-13.961292173295,13.096613347718,134.505276795414)) ;
#144472=CARTESIAN_POINT('Ctrl Pts',(-13.9110701574395,12.8330520382444,
134.391683767702)) ;
#144473=CARTESIAN_POINT('Ctrl Pts',(-13.8394412414765,12.611232367513,134.215641479407)) ;
#144474=CARTESIAN_POINT('Ctrl Pts',(-13.7510797643784,12.4482428501487,
133.990655184354)) ;
#144475=CARTESIAN_POINT('Ctrl Pts',(-13.6520098987817,12.3553252132509,
133.734233775121)) ;
#144476=CARTESIAN_POINT('Ctrl Pts',(-13.5477078598646,12.3382107203878,
133.462666865456)) ;
#144477=CARTESIAN_POINT('Ctrl Pts',(-13.4451051943709,12.3992481995866,
133.196136133625)) ;
#144478=CARTESIAN_POINT('Ctrl Pts',(-13.3515020692413,12.533120575299,132.955737055526)) ;
#144479=CARTESIAN_POINT('Ctrl Pts',(-13.2721063140921,12.7309389352082,
132.75693541364)) ;
#144480=CARTESIAN_POINT('Ctrl Pts',(-13.2121057414651,12.9791526214122,
132.614875968898)) ;
#144481=CARTESIAN_POINT('Ctrl Pts',(-13.1753406281424,13.2585792633392,
132.540604769992)) ;
#144482=CARTESIAN_POINT('Ctrl Pts',(-13.1635578925844,13.5499400001449,
132.539336578873)) ;
#144483=CARTESIAN_POINT('Ctrl Pts',(-13.1767327841943,13.831171440361,132.610841057035)) ;
#144484=CARTESIAN_POINT('Ctrl Pts',(-13.2135052261466,14.0848087373092,
132.751501701129)) ;
#144485=CARTESIAN_POINT('Ctrl Pts',(-13.2698735591139,14.2892042753313,
132.949112869563)) ;
#144486=CARTESIAN_POINT('Ctrl Pts',(-13.3419495547469,14.4332159857665,
133.192881784659)) ;
#144487=CARTESIAN_POINT('Ctrl Pts',(-13.4232398552977,14.5042074008981,
133.463464415944)) ;
#144488=CARTESIAN_POINT('Ctrl Pts',(-13.507384649746,14.4978850234615,133.742403717604)) ;
#144489=CARTESIAN_POINT('Ctrl Pts',(-13.5875958441071,14.4145533230364,
134.009844183663)) ;
#144490=CARTESIAN_POINT('Ctrl Pts',(-13.6574499514611,14.2600829811303,
134.24704991028)) ;
#144491=CARTESIAN_POINT('Ctrl Pts',(-13.711063219599,14.0459658246631,134.436755953918)) ;
#144492=CARTESIAN_POINT('Ctrl Pts',(-13.7440726911672,13.7875806302573,
134.566251929894)) ;
#144493=CARTESIAN_POINT('Ctrl Pts',(-13.7533105607091,13.5015007624486,
134.626490095641)) ;
#144494=CARTESIAN_POINT('Ctrl Pts',(-13.7373844729382,13.2119710918027,
134.612963509928)) ;
#144495=CARTESIAN_POINT('Ctrl Pts',(-13.6967466416228,12.9363052863804,
134.527385775247)) ;
#144496=CARTESIAN_POINT('Ctrl Pts',(-13.6333101280341,12.6952735982691,
134.375265595291)) ;
#144497=CARTESIAN_POINT('Ctrl Pts',(-13.5514819956674,12.5071256429724,
134.169269681796)) ;
#144498=CARTESIAN_POINT('Ctrl Pts',(-13.4552564937098,12.383762838378,133.921486273109)) ;
#144499=CARTESIAN_POINT('Ctrl Pts',(-13.3526734621167,12.3357954087545,
133.654750351329)) ;
#144500=CARTESIAN_POINT('Ctrl Pts',(-13.248390208345,12.3652711313032,133.383338134123)) ;
#144501=CARTESIAN_POINT('Ctrl Pts',(-13.1504948799325,12.4705156862028,
133.130424748745)) ;
#144502=CARTESIAN_POINT('Ctrl Pts',(-13.064631594807,12.6439184984734,132.912710120954)) ;
#144503=CARTESIAN_POINT('Ctrl Pts',(-12.9963758778862,12.8730354014428,
132.746418369545)) ;
#144504=CARTESIAN_POINT('Ctrl Pts',(-12.9497883269641,13.1424159380097,
132.643529935982)) ;
#144505=CARTESIAN_POINT('Ctrl Pts',(-12.9277522729892,13.4306391713404,
132.612207026215)) ;
#144506=CARTESIAN_POINT('Ctrl Pts',(-12.9308623319706,13.7191539467883,
132.654442340638)) ;
#144507=CARTESIAN_POINT('Ctrl Pts',(-12.9582863068314,13.9861294006722,
132.767666480281)) ;
#144508=CARTESIAN_POINT('Ctrl Pts',(-13.007269468484,14.2128684177951,132.943873402988)) ;
#144509=CARTESIAN_POINT('Ctrl Pts',(-13.0737783621588,14.3833348165239,
133.171349191452)) ;
#144510=CARTESIAN_POINT('Ctrl Pts',(-13.1520175298029,14.4845639234701,
133.433016513638)) ;
#144511=CARTESIAN_POINT('Ctrl Pts',(-13.2357654256101,14.5099092452808,
133.710770485551)) ;
#144512=CARTESIAN_POINT('Ctrl Pts',(-13.3184724571213,14.4573340950599,
133.985540682199)) ;
#144513=CARTESIAN_POINT('Ctrl Pts',(-13.3932587277117,14.3305257687139,
134.237149673029)) ;
#144514=CARTESIAN_POINT('Ctrl Pts',(-13.453959624611,14.1393929887669,134.447512911923)) ;
#144515=CARTESIAN_POINT('Ctrl Pts',(-13.4959188907949,13.8963011605845,
134.60324810303)) ;
#144516=CARTESIAN_POINT('Ctrl Pts',(-13.5150245929042,13.6185277978384,
134.692292652566)) ;
#144517=CARTESIAN_POINT('Ctrl Pts',(-13.5093297939817,13.3290636880528,
134.708618703529)) ;
#144518=CARTESIAN_POINT('Ctrl Pts',(-13.478487997988,13.0445547365035,134.651695864734)) ;
#144519=CARTESIAN_POINT('Ctrl Pts',(-13.4240438635045,12.7876682378207,
134.525750731676)) ;
#144520=CARTESIAN_POINT('Ctrl Pts',(-13.3486520787745,12.5753841966509,
134.33879441597)) ;
#144521=CARTESIAN_POINT('Ctrl Pts',(-13.2582557575008,12.4255193729721,
134.107675530931)) ;
#144522=CARTESIAN_POINT('Ctrl Pts',(-13.1571893879613,12.3459765323798,
133.845622114518)) ;
#144523=CARTESIAN_POINT('Ctrl Pts',(-13.052964824145,12.3439073605975,133.574205697266)) ;
#144524=CARTESIAN_POINT('Ctrl Pts',(-12.9516198217642,12.4188280799993,
133.3112916701)) ;
#144525=CARTESIAN_POINT('Ctrl Pts',(-12.8596716620883,12.5669348779127,
133.075980414901)) ;
#144526=CARTESIAN_POINT('Ctrl Pts',(-12.7842079537086,12.7740278443755,
132.888427019291)) ;
#144527=CARTESIAN_POINT('Ctrl Pts',(-12.7281316399476,13.0302841857639,
132.757923355197)) ;
#144528=CARTESIAN_POINT('Ctrl Pts',(-12.6960840940017,13.313391034623,132.697410502884)) ;
#144529=CARTESIAN_POINT('Ctrl Pts',(-12.6890448913152,13.603463825877,132.70986693963)) ;
#144530=CARTESIAN_POINT('Ctrl Pts',(-12.7067501795814,13.881303539034,132.794671056419)) ;
#144531=CARTESIAN_POINT('Ctrl Pts',(-12.7476563868859,14.1277804532013,
132.947459523477)) ;
#144532=CARTESIAN_POINT('Ctrl Pts',(-12.807668461047,14.3222500271651,133.155884784261)) ;
#144533=CARTESIAN_POINT('Ctrl Pts',(-12.8815759825536,14.4521801534422,
133.404796235282)) ;
#144534=CARTESIAN_POINT('Ctrl Pts',(-12.9639114339177,14.5090397064551,
133.678440955096)) ;
#144535=CARTESIAN_POINT('Ctrl Pts',(-13.0478748509612,14.4879536180509,
133.956866936907)) ;
#144536=CARTESIAN_POINT('Ctrl Pts',(-13.12663874727,14.3907168838663,134.220082699091)) ;
#144537=CARTESIAN_POINT('Ctrl Pts',(-13.1940374997755,14.2230874548014,
134.450238889046)) ;
#144538=CARTESIAN_POINT('Ctrl Pts',(-13.2437494985685,14.0008520915057,
134.628318458797)) ;
#144539=CARTESIAN_POINT('Ctrl Pts',(-13.2726507285596,13.7343152411408,
134.746038138861)) ;
#144540=CARTESIAN_POINT('Ctrl Pts',(-13.2771331648552,13.4474451384185,
134.7921586958)) ;
#144541=CARTESIAN_POINT('Ctrl Pts',(-13.2564031610437,13.1575373566889,
134.764792024668)) ;
#144542=CARTESIAN_POINT('Ctrl Pts',(-13.2113358398759,12.8878586213282,
134.666175549562)) ;
#144543=CARTESIAN_POINT('Ctrl Pts',(-13.1441355018156,12.6555337208909,
134.503032248599)) ;
#144544=CARTESIAN_POINT('Ctrl Pts',(-13.059137517177,12.4784852889698,134.287843551478)) ;
#144545=CARTESIAN_POINT('Ctrl Pts',(-12.9611258595703,12.3688435118071,
134.034798276015)) ;
#144546=CARTESIAN_POINT('Ctrl Pts',(-12.8576569308719,12.3353790498827,
133.765544543762)) ;
#144547=CARTESIAN_POINT('Ctrl Pts',(-12.7543421492588,12.3794309096132,
133.496846744508)) ;
#144548=CARTESIAN_POINT('Ctrl Pts',(-12.6581868323014,12.4979553163596,
133.249029548583)) ;
#144549=CARTESIAN_POINT('Ctrl Pts',(-12.5748068823933,12.6843641883006,
133.038779090593)) ;
#144550=CARTESIAN_POINT('Ctrl Pts',(-12.5108333068289,12.9208195747622,
132.884779860558)) ;
#144551=CARTESIAN_POINT('Ctrl Pts',(-12.4685180268136,13.1965599985602,
132.794503935178)) ;
#144552=CARTESIAN_POINT('Ctrl Pts',(-12.4513334564237,13.4854151022566,
132.777251050598)) ;
#144553=CARTESIAN_POINT('Ctrl Pts',(-12.4590824100926,13.7715246215189,
132.833039729551)) ;
#144554=CARTESIAN_POINT('Ctrl Pts',(-12.4909465763308,14.0329604460064,
132.959323426921)) ;
#144555=CARTESIAN_POINT('Ctrl Pts',(-12.543481678053,14.2495175049027,133.145827922929)) ;
#144556=CARTESIAN_POINT('Ctrl Pts',(-12.6124777949629,14.4077222066367,
133.380496347068)) ;
#144557=CARTESIAN_POINT('Ctrl Pts',(-12.6927510621182,14.4954975109272,
133.648307749174)) ;
#144558=CARTESIAN_POINT('Ctrl Pts',(-12.7765296871443,14.5058124049383,
133.926043997693)) ;
#144559=CARTESIAN_POINT('Ctrl Pts',(-12.8581519695846,14.4390539454557,
134.197602951378)) ;
#144560=CARTESIAN_POINT('Ctrl Pts',(-12.930945670173,14.2988993787837,134.443466881682)) ;
#144561=CARTESIAN_POINT('Ctrl Pts',(-12.9885263190073,14.0959845150152,
134.644827585225)) ;
#144562=CARTESIAN_POINT('Ctrl Pts',(-13.0261259536014,13.8467236092075,
134.787597338179)) ;
#144563=CARTESIAN_POINT('Ctrl Pts',(-13.0407617343322,13.5651497445093,
134.863551637252)) ;
#144564=CARTESIAN_POINT('Ctrl Pts',(-13.0303516451087,13.2745208567972,
134.866196431429)) ;
#144565=CARTESIAN_POINT('Ctrl Pts',(-12.9947636873513,12.9930479903862,
134.795477148735)) ;
#144566=CARTESIAN_POINT('Ctrl Pts',(-12.9363121229771,12.744268366307,134.657724887669)) ;
#144567=CARTESIAN_POINT('Ctrl Pts',(-12.8579516687104,12.5428868462353,
134.461961866201)) ;
#144568=CARTESIAN_POINT('Ctrl Pts',(-12.764650310326,12.4047082626809,134.222565644588)) ;
#144569=CARTESIAN_POINT('Ctrl Pts',(-12.6626217646199,12.3396945376806,
133.957623570518)) ;
#144570=CARTESIAN_POINT('Ctrl Pts',(-12.5583566636078,12.3521469878651,
133.68612910926)) ;
#144571=CARTESIAN_POINT('Ctrl Pts',(-12.4583830396902,12.4413144196275,
133.42721791323)) ;
#144572=CARTESIAN_POINT('Ctrl Pts',(-12.369233426393,12.6011044167591,133.199955438854)) ;
#144573=CARTESIAN_POINT('Ctrl Pts',(-12.296795109846,12.8194225372239,133.021442997756)) ;
#144574=CARTESIAN_POINT('Ctrl Pts',(-12.245256136277,13.0811435285209,132.904014857809)) ;
#144575=CARTESIAN_POINT('Ctrl Pts',(-12.2176939794846,13.3679218651448,
132.856686794612)) ;
#144576=CARTESIAN_POINT('Ctrl Pts',(-12.2154180287801,13.6574454628282,
132.883090037096)) ;
#144577=CARTESIAN_POINT('Ctrl Pts',(-12.2376037442581,13.9304219315962,
132.980959807401)) ;
#144578=CARTESIAN_POINT('Ctrl Pts',(-12.2824887862547,14.1686008809453,
133.145375342875)) ;
#144579=CARTESIAN_POINT('Ctrl Pts',(-12.3453046157036,14.3514046906987,
133.361866425527)) ;
#144580=CARTESIAN_POINT('Ctrl Pts',(-12.4215524934275,14.4688537021457,
133.617768892991)) ;
#144581=CARTESIAN_POINT('Ctrl Pts',(-12.5047937799249,14.5110084059665,
133.894090918055)) ;
#144582=CARTESIAN_POINT('Ctrl Pts',(-12.5880891539146,14.4754271671864,
134.170481851329)) ;
#144583=CARTESIAN_POINT('Ctrl Pts',(-12.6653082061899,14.3641624837098,
134.429260025213)) ;
#144584=CARTESIAN_POINT('Ctrl Pts',(-12.7297019423071,14.1852632714168,
134.650534523629)) ;
#144585=CARTESIAN_POINT('Ctrl Pts',(-12.7759253627988,13.9526451363771,
134.818608665659)) ;
#144586=CARTESIAN_POINT('Ctrl Pts',(-12.8002263769998,13.6818446977071,
134.922696351685)) ;
#144587=CARTESIAN_POINT('Ctrl Pts',(-12.8000986222463,13.3926206183681,
134.955407057366)) ;
#144588=CARTESIAN_POINT('Ctrl Pts',(-12.7745111191584,13.1038754492096,
134.91394806215)) ;
#144589=CARTESIAN_POINT('Ctrl Pts',(-12.7250570523891,12.840383579606,134.802482892193)) ;
#144590=CARTESIAN_POINT('Ctrl Pts',(-12.6542480453106,12.6175434058043,
134.628747907332)) ;
#144591=CARTESIAN_POINT('Ctrl Pts',(-12.5661484572041,12.452017834643,134.40460207524)) ;
#144592=CARTESIAN_POINT('Ctrl Pts',(-12.466810665612,12.3567780373273,134.147557352768)) ;
#144593=CARTESIAN_POINT('Ctrl Pts',(-12.3630998015103,12.3376561181457,
133.877541645615)) ;
#144594=CARTESIAN_POINT('Ctrl Pts',(-12.2602167543945,12.3963495269004,
133.610232883161)) ;
#144595=CARTESIAN_POINT('Ctrl Pts',(-12.1662740877371,12.5282530119487,
133.36884192798)) ;
#144596=CARTESIAN_POINT('Ctrl Pts',(-12.0863990846921,12.7243874356401,
133.168638276115)) ;
#144597=CARTESIAN_POINT('Ctrl Pts',(-12.0258318101677,12.9708925599776,
133.024863858059)) ;
#144598=CARTESIAN_POINT('Ctrl Pts',(-11.9882998267701,13.2502128136118,
132.948421366033)) ;
#144599=CARTESIAN_POINT('Ctrl Pts',(-11.9757436014194,13.5400585853171,
132.944721817268)) ;
#144600=CARTESIAN_POINT('Ctrl Pts',(-11.9882527010253,13.8239340251458,
133.014527571327)) ;
#144601=CARTESIAN_POINT('Ctrl Pts',(-12.024314175027,14.0777678447128,133.152994495197)) ;
#144602=CARTESIAN_POINT('Ctrl Pts',(-12.0802386867807,14.2841379825029,
133.349369470604)) ;
#144603=CARTESIAN_POINT('Ctrl Pts',(-12.1517568327263,14.4298157397374,
133.591419824173)) ;
#144604=CARTESIAN_POINT('Ctrl Pts',(-12.2331386991357,14.5033259419055,
133.862387548151)) ;
#144605=CARTESIAN_POINT('Ctrl Pts',(-12.3172490667229,14.499135083616,134.141203152847)) ;
#144606=CARTESIAN_POINT('Ctrl Pts',(-12.3977223834432,14.4177797503692,
134.409440590375)) ;
#144607=CARTESIAN_POINT('Ctrl Pts',(-12.4677306111638,14.2657375874764,
134.646986738776)) ;
#144608=CARTESIAN_POINT('Ctrl Pts',(-12.5220714640845,14.0527572687347,
134.838901719408)) ;
#144609=CARTESIAN_POINT('Ctrl Pts',(-12.5557480287328,13.7942042748117,
134.970478170915)) ;
#144610=CARTESIAN_POINT('Ctrl Pts',(-12.5655893514791,13.5099720674089,
135.032313082312)) ;
#144611=CARTESIAN_POINT('Ctrl Pts',(-12.5503883535898,13.2198346279653,
135.020961803302)) ;
#144612=CARTESIAN_POINT('Ctrl Pts',(-12.5103698968678,12.943315390008,134.937211770159)) ;
#144613=CARTESIAN_POINT('Ctrl Pts',(-12.4473782776272,12.7008041601945,
134.786440487952)) ;
#144614=CARTESIAN_POINT('Ctrl Pts',(-12.3662789009973,12.5118987867612,
134.582448501668)) ;
#144615=CARTESIAN_POINT('Ctrl Pts',(-12.2708904646129,12.3867144274878,
134.336948453018)) ;
#144616=CARTESIAN_POINT('Ctrl Pts',(-12.1678380844892,12.3359851179155,
134.069036435236)) ;
#144617=CARTESIAN_POINT('Ctrl Pts',(-12.0635192151034,12.3634203975105,
133.797509645721)) ;
#144618=CARTESIAN_POINT('Ctrl Pts',(-11.9653834956935,12.4663876776292,
133.543880463579)) ;
#144619=CARTESIAN_POINT('Ctrl Pts',(-11.8787531345459,12.638970046877,133.32407434828)) ;
#144620=CARTESIAN_POINT('Ctrl Pts',(-11.8103116788291,12.8657476347374,
133.157082057629)) ;
#144621=CARTESIAN_POINT('Ctrl Pts',(-11.7629363114797,13.1346340040003,
133.051944760251)) ;
#144622=CARTESIAN_POINT('Ctrl Pts',(-11.74782998282,13.3266515427633,133.029855138178)) ;
#144623=CARTESIAN_POINT('Ctrl Pts',(-11.7444305159761,13.4226803244344,
133.030945169693)) ;
#144624=CARTESIAN_POINT('Ctrl Pts',(-33.2300180027834,13.1368456608817,
127.989533782136)) ;
#144625=CARTESIAN_POINT('Ctrl Pts',(-33.2292437520727,13.130243425216,127.988002960232)) ;
#144626=CARTESIAN_POINT('Ctrl Pts',(-33.2166096866017,13.0249708380281,
127.962778125839)) ;
#144627=CARTESIAN_POINT('Ctrl Pts',(-33.182092795898,12.8263019600079,127.884920491647)) ;
#144628=CARTESIAN_POINT('Ctrl Pts',(-33.1092916050684,12.5833994930382,
127.705272326551)) ;
#144629=CARTESIAN_POINT('Ctrl Pts',(-33.0177478422943,12.399626766211,127.470955863714)) ;
#144630=CARTESIAN_POINT('Ctrl Pts',(-32.9127470434696,12.2890731618772,
127.197495494478)) ;
#144631=CARTESIAN_POINT('Ctrl Pts',(-32.8027864649256,12.2602312948732,
126.909202090255)) ;
#144632=CARTESIAN_POINT('Ctrl Pts',(-32.6929501385259,12.3144254522227,
126.621568480859)) ;
#144633=CARTESIAN_POINT('Ctrl Pts',(-32.59177016842,12.4480642946114,126.359088261639)) ;
#144634=CARTESIAN_POINT('Ctrl Pts',(-32.5051791199469,12.6516399899179,
126.139277587465)) ;
#144635=CARTESIAN_POINT('Ctrl Pts',(-32.4388702329151,12.9104453038702,
125.97869600614)) ;
#144636=CARTESIAN_POINT('Ctrl Pts',(-32.3968275748835,13.2058492691314,
125.888992944671)) ;
#144637=CARTESIAN_POINT('Ctrl Pts',(-32.3812336706731,13.5166185684314,
125.876529755364)) ;
#144638=CARTESIAN_POINT('Ctrl Pts',(-32.3927205422695,13.8224101024019,
125.943375492965)) ;
#144639=CARTESIAN_POINT('Ctrl Pts',(-32.4293470746311,14.0967865746008,
126.083332512321)) ;
#144640=CARTESIAN_POINT('Ctrl Pts',(-32.4880514233328,14.3244563595429,
126.287951913574)) ;
#144641=CARTESIAN_POINT('Ctrl Pts',(-32.5638474430166,14.4874742407207,
126.54248591268)) ;
#144642=CARTESIAN_POINT('Ctrl Pts',(-32.6508225706577,14.5744205093284,
126.829774468175)) ;
#144643=CARTESIAN_POINT('Ctrl Pts',(-32.7415381559199,14.5784621609188,
127.127897337849)) ;
#144644=CARTESIAN_POINT('Ctrl Pts',(-32.8288658284697,14.5000469368875,
127.416073622444)) ;
#144645=CARTESIAN_POINT('Ctrl Pts',(-32.9060635890902,14.344572658684,127.67469123317)) ;
#144646=CARTESIAN_POINT('Ctrl Pts',(-32.9668884901517,14.1228337492368,
127.88552736943)) ;
#144647=CARTESIAN_POINT('Ctrl Pts',(-33.0061004434272,13.8501516005036,
128.033299850844)) ;
#144648=CARTESIAN_POINT('Ctrl Pts',(-33.0200491726642,13.5490422759736,
128.107026504832)) ;
#144649=CARTESIAN_POINT('Ctrl Pts',(-33.0073427737607,13.2374716075454,
128.103049880758)) ;
#144650=CARTESIAN_POINT('Ctrl Pts',(-32.9677468015857,12.9386843836575,
128.020588082111)) ;
#144651=CARTESIAN_POINT('Ctrl Pts',(-32.9039626552368,12.6761376580761,
127.867269826708)) ;
#144652=CARTESIAN_POINT('Ctrl Pts',(-32.8190967106854,12.4657586342273,
127.652552845677)) ;
#144653=CARTESIAN_POINT('Ctrl Pts',(-32.7191980487996,12.3246285440834,
127.39379148403)) ;
#144654=CARTESIAN_POINT('Ctrl Pts',(-32.6098826596707,12.2619062203987,
127.107681420346)) ;
#144655=CARTESIAN_POINT('Ctrl Pts',(-32.4994620023921,12.282438847825,126.818116882423)) ;
#144656=CARTESIAN_POINT('Ctrl Pts',(-32.3937285710348,12.3848777791117,
126.542455056202)) ;
#144657=CARTESIAN_POINT('Ctrl Pts',(-32.3006102621747,12.5614992054213,
126.303522073794)) ;
#144658=CARTESIAN_POINT('Ctrl Pts',(-32.2255196684499,12.7995868451149,
126.117262217641)) ;
#144659=CARTESIAN_POINT('Ctrl Pts',(-32.1730545330911,13.0840300183346,
125.99727657049)) ;
#144660=CARTESIAN_POINT('Ctrl Pts',(-32.1467969822621,13.3899587420559,
125.953531154388)) ;
#144661=CARTESIAN_POINT('Ctrl Pts',(-32.147224199752,13.6996411471026,125.987893566941)) ;
#144662=CARTESIAN_POINT('Ctrl Pts',(-32.1740653691313,13.9903747367888,
126.099519807881)) ;
#144663=CARTESIAN_POINT('Ctrl Pts',(-32.2243898321981,14.2393240379775,
126.279618857538)) ;
#144664=CARTESIAN_POINT('Ctrl Pts',(-32.2938170416811,14.4298400275378,
126.51549169053)) ;
#144665=CARTESIAN_POINT('Ctrl Pts',(-32.3768965968871,14.5487685200995,
126.791305226358)) ;
#144666=CARTESIAN_POINT('Ctrl Pts',(-32.4670988147272,14.5869290465038,
127.088015098191)) ;
#144667=CARTESIAN_POINT('Ctrl Pts',(-32.5565456830465,14.5417666874379,
127.382354784027)) ;
#144668=CARTESIAN_POINT('Ctrl Pts',(-32.6388889719656,14.4163781165351,
127.656070958631)) ;
#144669=CARTESIAN_POINT('Ctrl Pts',(-32.70708269963,14.2194053123055,127.888457784894)) ;
#144670=CARTESIAN_POINT('Ctrl Pts',(-32.7553721885115,13.966643682879,128.06254084362)) ;
#144671=CARTESIAN_POINT('Ctrl Pts',(-32.7800253727878,13.6737230006816,
128.167739670936)) ;
#144672=CARTESIAN_POINT('Ctrl Pts',(-32.7781801610669,13.3629182756251,
128.195508808425)) ;
#144673=CARTESIAN_POINT('Ctrl Pts',(-32.7493936429457,13.0570540996615,
128.144513598679)) ;
#144674=CARTESIAN_POINT('Ctrl Pts',(-32.6950690343676,12.7772473921445,
128.018915404156)) ;
#144675=CARTESIAN_POINT('Ctrl Pts',(-32.6178215190404,12.5427680100154,
127.826519840422)) ;
#144676=CARTESIAN_POINT('Ctrl Pts',(-32.5236936545369,12.3730788139632,
127.584510875552)) ;
#144677=CARTESIAN_POINT('Ctrl Pts',(-32.4173873681917,12.2773830368376,
127.307131936776)) ;
#144678=CARTESIAN_POINT('Ctrl Pts',(-32.306450665399,12.2641121803462,127.016176193277)) ;
#144679=CARTESIAN_POINT('Ctrl Pts',(-32.1980092860901,12.3337583656513,
126.732504271029)) ;
#144680=CARTESIAN_POINT('Ctrl Pts',(-32.0990876968215,12.4813161327732,
126.476631639078)) ;
#144681=CARTESIAN_POINT('Ctrl Pts',(-32.0158761927489,12.6966780658121,
126.266710351662)) ;
#144682=CARTESIAN_POINT('Ctrl Pts',(-31.9538770228678,12.9640585789761,
126.118733259147)) ;
#144683=CARTESIAN_POINT('Ctrl Pts',(-31.9167599552358,13.263362217281,126.043343607058)) ;
#144684=CARTESIAN_POINT('Ctrl Pts',(-31.9062170544741,13.5752569117425,
126.045709527399)) ;
#144685=CARTESIAN_POINT('Ctrl Pts',(-31.9226445076029,13.8766503644376,
126.126917612135)) ;
#144686=CARTESIAN_POINT('Ctrl Pts',(-31.9637029016732,14.1438627014427,
126.279869047209)) ;
#144687=CARTESIAN_POINT('Ctrl Pts',(-32.0262809227179,14.3611558948339,
126.495912269976)) ;
#144688=CARTESIAN_POINT('Ctrl Pts',(-32.1047645421015,14.5102071341288,
126.758321777945)) ;
#144689=CARTESIAN_POINT('Ctrl Pts',(-32.1923828176935,14.5813677967462,
127.047244242667)) ;
#144690=CARTESIAN_POINT('Ctrl Pts',(-32.2832244888106,14.5701314848988,
127.34580352681)) ;
#144691=CARTESIAN_POINT('Ctrl Pts',(-32.3695772610759,14.4759918680502,
127.631298809263)) ;
#144692=CARTESIAN_POINT('Ctrl Pts',(-32.4440427734201,14.3066892261713,
127.881936729274)) ;
#144693=CARTESIAN_POINT('Ctrl Pts',(-32.5008263829426,14.0751878259722,
128.080807992668)) ;
#144694=CARTESIAN_POINT('Ctrl Pts',(-32.5355347715382,13.7962286301239,
128.215320954955)) ;
#144695=CARTESIAN_POINT('Ctrl Pts',(-32.5446721574957,13.489739255107,128.275210131471)) ;
#144696=CARTESIAN_POINT('Ctrl Pts',(-32.5265849289817,13.1781056591445,
128.255614488998)) ;
#144697=CARTESIAN_POINT('Ctrl Pts',(-32.4826045749206,12.8871394405402,
128.160016968544)) ;
#144698=CARTESIAN_POINT('Ctrl Pts',(-32.4142077175318,12.6313542948275,
127.993455148727)) ;
#144699=CARTESIAN_POINT('Ctrl Pts',(-32.3259460356126,12.4333423799844,
127.768796899427)) ;
#144700=CARTESIAN_POINT('Ctrl Pts',(-32.2242180820195,12.3067788244502,
127.504580022225)) ;
#144701=CARTESIAN_POINT('Ctrl Pts',(-32.1138392452441,12.2592790120272,
127.215412831883)) ;
#144702=CARTESIAN_POINT('Ctrl Pts',(-32.003485063804,12.2958890745914,126.926165499256)) ;
#144703=CARTESIAN_POINT('Ctrl Pts',(-31.9001877061898,12.412515961838,126.657421781237)) ;
#144704=CARTESIAN_POINT('Ctrl Pts',(-31.8098515533927,12.6017795181092,
126.426660655506)) ;
#144705=CARTESIAN_POINT('Ctrl Pts',(-31.7385681295902,12.8508820386888,
126.251652404541)) ;
#144706=CARTESIAN_POINT('Ctrl Pts',(-31.6911379315082,13.1389626270395,
126.146085694306)) ;
#144707=CARTESIAN_POINT('Ctrl Pts',(-31.6696008199509,13.4502019217322,
126.116475044646)) ;
#144708=CARTESIAN_POINT('Ctrl Pts',(-31.675316072249,13.7571545307035,126.166221736191)) ;
#144709=CARTESIAN_POINT('Ctrl Pts',(-31.706567429285,14.0399279839555,126.290508349871)) ;
#144710=CARTESIAN_POINT('Ctrl Pts',(-31.7611102860572,14.2804627639154,
126.483099880761)) ;
#144711=CARTESIAN_POINT('Ctrl Pts',(-31.8334965665926,14.4580430592262,
126.727575168769)) ;
#144712=CARTESIAN_POINT('Ctrl Pts',(-31.9185397988038,14.5623041916472,
127.009181592164)) ;
#144713=CARTESIAN_POINT('Ctrl Pts',(-32.0088724260903,14.5848738279965,
127.306134040065)) ;
#144714=CARTESIAN_POINT('Ctrl Pts',(-32.0981654325802,14.5236285085623,
127.60029694483)) ;
#144715=CARTESIAN_POINT('Ctrl Pts',(-32.1778221198332,14.3842858340258,
127.865980605226)) ;
#144716=CARTESIAN_POINT('Ctrl Pts',(-32.2426771957791,14.1760036072079,
128.088561512435)) ;
#144717=CARTESIAN_POINT('Ctrl Pts',(-32.2870187656786,13.9123644757914,
128.251357212827)) ;
#144718=CARTESIAN_POINT('Ctrl Pts',(-32.3065797695472,13.6155078278093,
128.341537873815)) ;
#144719=CARTESIAN_POINT('Ctrl Pts',(-32.299733398088,13.3048785674805,128.354587348161)) ;
#144720=CARTESIAN_POINT('Ctrl Pts',(-32.2658846348396,13.0013157661824,
128.288909145549)) ;
#144721=CARTESIAN_POINT('Ctrl Pts',(-32.2069886942351,12.7290184016179,
128.1499432911)) ;
#144722=CARTESIAN_POINT('Ctrl Pts',(-32.1263303751001,12.5059452399051,
127.947463873129)) ;
#144723=CARTESIAN_POINT('Ctrl Pts',(-32.0291748251866,12.3489356287849,
127.696738913591)) ;
#144724=CARTESIAN_POINT('Ctrl Pts',(-31.9217381388589,12.2685725543234,
127.415958176252)) ;
#144725=CARTESIAN_POINT('Ctrl Pts',(-31.8103465441405,12.2709800429639,
127.123786383864)) ;
#144726=CARTESIAN_POINT('Ctrl Pts',(-31.7033367406482,12.3558597729099,
126.844245062595)) ;
#144727=CARTESIAN_POINT('Ctrl Pts',(-31.6068083151779,12.5173149603475,
126.595412194401)) ;
#144728=CARTESIAN_POINT('Ctrl Pts',(-31.5273365282627,12.7436533990505,
126.396378948702)) ;
#144729=CARTESIAN_POINT('Ctrl Pts',(-31.4698051340278,13.0184391558732,
126.261419197798)) ;
#144730=CARTESIAN_POINT('Ctrl Pts',(-31.4375406438131,13.3224259864685,
126.200296275979)) ;
#144731=CARTESIAN_POINT('Ctrl Pts',(-31.4321948009819,13.6337497242247,
126.217821502333)) ;
#144732=CARTESIAN_POINT('Ctrl Pts',(-31.4534309715984,13.9298382282655,
126.312987130498)) ;
#144733=CARTESIAN_POINT('Ctrl Pts',(-31.4989100448319,14.189430649662,126.47894051365)) ;
#144734=CARTESIAN_POINT('Ctrl Pts',(-31.564823476328,14.394475769408,126.704646843122)) ;
#144735=CARTESIAN_POINT('Ctrl Pts',(-31.6453547625781,14.5294751555696,
126.972946428523)) ;
#144736=CARTESIAN_POINT('Ctrl Pts',(-31.7344309707167,14.5857784692471,
127.266285694623)) ;
#144737=CARTESIAN_POINT('Ctrl Pts',(-31.8250135034699,14.5584757915825,
127.564109179261)) ;
#144738=CARTESIAN_POINT('Ctrl Pts',(-31.9093410315124,14.4499269428434,
127.843545790168)) ;
#144739=CARTESIAN_POINT('Ctrl Pts',(-31.9810494756834,14.2678362353556,
128.086150346001)) ;
#144740=CARTESIAN_POINT('Ctrl Pts',(-32.034169894188,14.025181457992,128.274454335045)) ;
#144741=CARTESIAN_POINT('Ctrl Pts',(-32.0641766159735,13.7395989373351,
128.395216353623)) ;
#144742=CARTESIAN_POINT('Ctrl Pts',(-32.0682143772273,13.4312396323536,
128.440131093672)) ;
#144743=CARTESIAN_POINT('Ctrl Pts',(-32.0453158611644,13.1225497358479,
128.406327376222)) ;
#144744=CARTESIAN_POINT('Ctrl Pts',(-31.996169151728,12.8344723691042,128.295954955988)) ;
#144745=CARTESIAN_POINT('Ctrl Pts',(-31.9238482595544,12.5894057797878,
128.117787838384)) ;
#144746=CARTESIAN_POINT('Ctrl Pts',(-31.832662535924,12.403866954954,127.884535160831)) ;
#144747=CARTESIAN_POINT('Ctrl Pts',(-31.7285002227895,12.2913271395126,
127.613354573894)) ;
#144748=CARTESIAN_POINT('Ctrl Pts',(-31.6177523868802,12.2598830910024,
127.32302334867)) ;
#144749=CARTESIAN_POINT('Ctrl Pts',(-31.5083419637065,12.3117248800856,
127.036464679432)) ;
#144750=CARTESIAN_POINT('Ctrl Pts',(-31.4066545343474,12.4432581969561,
126.772557747754)) ;
#144751=CARTESIAN_POINT('Ctrl Pts',(-31.3196996717147,12.6447768479475,
126.551633848093)) ;
#144752=CARTESIAN_POINT('Ctrl Pts',(-31.2527294004413,12.9020427023331,
126.389108312362)) ;
#144753=CARTESIAN_POINT('Ctrl Pts',(-31.2098964874748,13.1969220955149,
126.297125418566)) ;
#144754=CARTESIAN_POINT('Ctrl Pts',(-31.1935254547332,13.5073634201221,
126.282371473235)) ;
#144755=CARTESIAN_POINT('Ctrl Pts',(-31.2042125321738,13.8135028677167,
126.346863684754)) ;
#144756=CARTESIAN_POINT('Ctrl Pts',(-31.2400738263031,14.0890635163078,
126.484577408742)) ;
#144757=CARTESIAN_POINT('Ctrl Pts',(-31.2984854067219,14.3192685446141,
126.688485355535)) ;
#144758=CARTESIAN_POINT('Ctrl Pts',(-31.3736030379443,14.4835637983032,
126.940906398959)) ;
#144759=CARTESIAN_POINT('Ctrl Pts',(-31.4603373040575,14.5730188285823,
127.227495175343)) ;
#144760=CARTESIAN_POINT('Ctrl Pts',(-31.5510617389729,14.5795967764284,
127.52564779883)) ;
#144761=CARTESIAN_POINT('Ctrl Pts',(-31.6387634374852,14.5032853646564,
127.814990801029)) ;
#144762=CARTESIAN_POINT('Ctrl Pts',(-31.7162734788817,14.3501151249434,
128.074477893202)) ;
#144763=CARTESIAN_POINT('Ctrl Pts',(-31.7777929390999,14.1289951799062,
128.287474132469)) ;
#144764=CARTESIAN_POINT('Ctrl Pts',(-31.8173663026795,13.8600883343583,
128.435990379675)) ;
#144765=CARTESIAN_POINT('Ctrl Pts',(-31.8322919438319,13.5571075891159,
128.512852727312)) ;
#144766=CARTESIAN_POINT('Ctrl Pts',(-31.82022330572,13.246144038551,128.51066807506)) ;
#144767=CARTESIAN_POINT('Ctrl Pts',(-31.7816172657033,12.9474784018938,
128.430993884236)) ;
#144768=CARTESIAN_POINT('Ctrl Pts',(-31.7179322198423,12.6818049804595,
128.278220905245)) ;
#144769=CARTESIAN_POINT('Ctrl Pts',(-31.6341871853082,12.4713261551404,
128.06652480907)) ;
#144770=CARTESIAN_POINT('Ctrl Pts',(-31.5341646889309,12.3273775060339,
127.807571862483)) ;
#144771=CARTESIAN_POINT('Ctrl Pts',(-31.4256220530774,12.2625380401702,
127.523523338818)) ;
#144772=CARTESIAN_POINT('Ctrl Pts',(-31.3141710264018,12.2810707697993,
127.231254074188)) ;
#144773=CARTESIAN_POINT('Ctrl Pts',(-31.2093207416978,12.3803129449242,
126.957812292313)) ;
#144774=CARTESIAN_POINT('Ctrl Pts',(-31.1151683157107,12.5556239471542,
126.716053817191)) ;
#144775=CARTESIAN_POINT('Ctrl Pts',(-31.0397604821061,12.7914917481058,
126.528754888834)) ;
#144776=CARTESIAN_POINT('Ctrl Pts',(-30.9864549257893,13.0750410185669,
126.406347636205)) ;
#144777=CARTESIAN_POINT('Ctrl Pts',(-30.9593938888774,13.3808908825506,
126.360285902276)) ;
#144778=CARTESIAN_POINT('Ctrl Pts',(-30.9590643989393,13.6908805105498,
126.392448187648)) ;
#144779=CARTESIAN_POINT('Ctrl Pts',(-30.985079519922,13.9819858860809,126.501595001656)) ;
#144780=CARTESIAN_POINT('Ctrl Pts',(-31.0349155333376,14.2331023170552,
126.680366168729)) ;
#144781=CARTESIAN_POINT('Ctrl Pts',(-31.103787873337,14.425373738482,126.914579912793)) ;
#144782=CARTESIAN_POINT('Ctrl Pts',(-31.1870948720038,14.5469025467051,
127.191256375485)) ;
#144783=CARTESIAN_POINT('Ctrl Pts',(-31.2765949077209,14.5868798002751,
127.48568376315)) ;
#144784=CARTESIAN_POINT('Ctrl Pts',(-31.3662691064729,14.544243012127,127.780733186927)) ;
#144785=CARTESIAN_POINT('Ctrl Pts',(-31.4488236582154,14.4211466682183,
128.055026539422)) ;
#144786=CARTESIAN_POINT('Ctrl Pts',(-31.5175184584452,14.2262607668007,
128.28886635848)) ;
#144787=CARTESIAN_POINT('Ctrl Pts',(-31.566546342217,13.9744157440355,128.465170341222)) ;
#144788=CARTESIAN_POINT('Ctrl Pts',(-31.5918626188502,13.6824769956245,
128.572286130259)) ;
#144789=CARTESIAN_POINT('Ctrl Pts',(-31.5908930328258,13.3726811075526,
128.602527371079)) ;
#144790=CARTESIAN_POINT('Ctrl Pts',(-31.5626626632348,13.0644552653701,
128.553368423674)) ;
#144791=CARTESIAN_POINT('Ctrl Pts',(-31.5092143642815,12.7851437456734,
128.430163081405)) ;
#144792=CARTESIAN_POINT('Ctrl Pts',(-31.4328238022929,12.5493640024945,
128.240198742894)) ;
#144793=CARTESIAN_POINT('Ctrl Pts',(-31.3389013828092,12.376970726474,127.998880739351)) ;
#144794=CARTESIAN_POINT('Ctrl Pts',(-31.2325442048154,12.2789142943649,
127.721438969545)) ;
#144795=CARTESIAN_POINT('Ctrl Pts',(-31.1219668459032,12.2633331335236,
127.431435996235)) ;
#144796=CARTESIAN_POINT('Ctrl Pts',(-31.0131048658682,12.3306602868788,
127.146608211436)) ;
#144797=CARTESIAN_POINT('Ctrl Pts',(-30.9137175361845,12.4766203405944,
126.889425390704)) ;
#144798=CARTESIAN_POINT('Ctrl Pts',(-30.8304038367424,12.6891737116268,
126.679037871423)) ;
#144799=CARTESIAN_POINT('Ctrl Pts',(-30.7676114855164,12.9552556025245,
126.528760774747)) ;
#144800=CARTESIAN_POINT('Ctrl Pts',(-30.7296421112751,13.2547271279824,
126.450969119973)) ;
#144801=CARTESIAN_POINT('Ctrl Pts',(-30.7183893110639,13.5662747472623,
126.451228783518)) ;
#144802=CARTESIAN_POINT('Ctrl Pts',(-30.733913444231,13.8673047437589,126.529679410817)) ;
#144803=CARTESIAN_POINT('Ctrl Pts',(-30.7744187831049,14.1368397654386,
126.681145138688)) ;
#144804=CARTESIAN_POINT('Ctrl Pts',(-30.8362150266428,14.3550474854522,
126.894778750719)) ;
#144805=CARTESIAN_POINT('Ctrl Pts',(-30.9142509625502,14.5066809969925,
127.155885362528)) ;
#144806=CARTESIAN_POINT('Ctrl Pts',(-31.0021246618732,14.5805550021418,
127.445716539722)) ;
#144807=CARTESIAN_POINT('Ctrl Pts',(-31.0927386419464,14.5715434154247,
127.743520389293)) ;
#144808=CARTESIAN_POINT('Ctrl Pts',(-31.1790271767305,14.4804614253832,
128.028700915286)) ;
#144809=CARTESIAN_POINT('Ctrl Pts',(-31.2542421356505,14.3129344322758,
128.281642462591)) ;
#144810=CARTESIAN_POINT('Ctrl Pts',(-31.3117291376772,14.0824719348205,
128.482642895694)) ;
#144811=CARTESIAN_POINT('Ctrl Pts',(-31.3470892051773,13.8045959520742,
128.619053432175)) ;
#144812=CARTESIAN_POINT('Ctrl Pts',(-31.3569871658133,13.4994871825109,
128.681068602957)) ;
#144813=CARTESIAN_POINT('Ctrl Pts',(-31.3397975278184,13.1877258357311,
128.664087688354)) ;
#144814=CARTESIAN_POINT('Ctrl Pts',(-31.2964040254458,12.8947281462995,
128.570335332532)) ;
#144815=CARTESIAN_POINT('Ctrl Pts',(-31.2284884597744,12.6375710279023,
128.405210278833)) ;
#144816=CARTESIAN_POINT('Ctrl Pts',(-31.1412553171242,12.4386468610117,
128.183369892293)) ;
#144817=CARTESIAN_POINT('Ctrl Pts',(-31.0392856803408,12.3091460957756,
127.918635408139)) ;
#144818=CARTESIAN_POINT('Ctrl Pts',(-30.9296587376181,12.2596124823544,
127.631470528942)) ;
#144819=CARTESIAN_POINT('Ctrl Pts',(-30.8189572509962,12.2934287608505,
127.341283904815)) ;
#144820=CARTESIAN_POINT('Ctrl Pts',(-30.7149224451956,12.4085128327331,
127.070530721846)) ;
#144821=CARTESIAN_POINT('Ctrl Pts',(-30.6244270191123,12.5956557289105,
126.839221510393)) ;
#144822=CARTESIAN_POINT('Ctrl Pts',(-30.552740348961,12.8419007225992,126.662879913109)) ;
#144823=CARTESIAN_POINT('Ctrl Pts',(-30.5042887818973,13.1310174961036,
126.554554614901)) ;
#144824=CARTESIAN_POINT('Ctrl Pts',(-30.4821225458649,13.4394174357417,
126.522827842075)) ;
#144825=CARTESIAN_POINT('Ctrl Pts',(-30.4869544585416,13.7489280911395,
126.570225234814)) ;
#144826=CARTESIAN_POINT('Ctrl Pts',(-30.5176484397562,14.0326636377924,
126.692900306353)) ;
#144827=CARTESIAN_POINT('Ctrl Pts',(-30.5713213184817,14.2739040852335,
126.882817074721)) ;
#144828=CARTESIAN_POINT('Ctrl Pts',(-30.6436244084103,14.4542739196418,
127.127215545827)) ;
#144829=CARTESIAN_POINT('Ctrl Pts',(-30.7280326162985,14.5602989728585,
127.406812499474)) ;
#144830=CARTESIAN_POINT('Ctrl Pts',(-30.8186285442324,14.5853165149043,
127.704660608665)) ;
#144831=CARTESIAN_POINT('Ctrl Pts',(-30.9075041976881,14.5269566975762,
127.997384873959)) ;
#144832=CARTESIAN_POINT('Ctrl Pts',(-30.9881047297177,14.3891797557674,
128.266049347008)) ;
#144833=CARTESIAN_POINT('Ctrl Pts',(-31.0534636981104,14.1817902541555,
128.490167087522)) ;
#144834=CARTESIAN_POINT('Ctrl Pts',(-31.0981004770551,13.9219441435514,
128.653522008646)) ;
#144835=CARTESIAN_POINT('Ctrl Pts',(-31.1186289612997,13.6244332360091,
128.746699920256)) ;
#144836=CARTESIAN_POINT('Ctrl Pts',(-31.1125361857991,13.3138307533241,
128.761949736596)) ;
#144837=CARTESIAN_POINT('Ctrl Pts',(-31.0793149773615,13.0089906490168,
128.698191722049)) ;
#144838=CARTESIAN_POINT('Ctrl Pts',(-31.0213127924495,12.7367004546504,
128.56169934609)) ;
#144839=CARTESIAN_POINT('Ctrl Pts',(-30.9412589328357,12.5117902226442,
128.360991687097)) ;
#144840=CARTESIAN_POINT('Ctrl Pts',(-30.8444991744712,12.3525055718321,
128.111429712698)) ;
#144841=CARTESIAN_POINT('Ctrl Pts',(-30.736804998274,12.2695603422194,127.830036678703)) ;
#144842=CARTESIAN_POINT('Ctrl Pts',(-30.6255790074019,12.2698997587057,
127.538298190404)) ;
#144843=CARTESIAN_POINT('Ctrl Pts',(-30.5186478948904,12.3521640390818,
127.258896733062)) ;
#144844=CARTESIAN_POINT('Ctrl Pts',(-30.4216161503203,12.5116415634716,
127.008626067595)) ;
#144845=CARTESIAN_POINT('Ctrl Pts',(-30.3416456644303,12.7360069700772,
126.808096783249)) ;
#144846=CARTESIAN_POINT('Ctrl Pts',(-30.2833400695677,13.0100796293743,
126.670930462911)) ;
#144847=CARTESIAN_POINT('Ctrl Pts',(-30.250351362489,13.3126253374921,126.607593228363)) ;
#144848=CARTESIAN_POINT('Ctrl Pts',(-30.2441927566021,13.6254715524663,
126.622899503079)) ;
#144849=CARTESIAN_POINT('Ctrl Pts',(-30.2646331156608,13.9212365418522,
126.715618043122)) ;
#144850=CARTESIAN_POINT('Ctrl Pts',(-30.3095314842463,14.1826934673073,
126.879946570036)) ;
#144851=CARTESIAN_POINT('Ctrl Pts',(-30.3746703453055,14.3889686584202,
127.103272672401)) ;
#144852=CARTESIAN_POINT('Ctrl Pts',(-30.4553607437768,14.5271450156122,
127.372251222131)) ;
#144853=CARTESIAN_POINT('Ctrl Pts',(-30.5443910347089,14.5852339348323,
127.665478148695)) ;
#144854=CARTESIAN_POINT('Ctrl Pts',(-30.6344393567166,14.5605427661762,
127.96152213049)) ;
#144855=CARTESIAN_POINT('Ctrl Pts',(-30.7192995987514,14.4541441537073,
128.242612469861)) ;
#144856=CARTESIAN_POINT('Ctrl Pts',(-30.791408695709,14.2740963281162,128.486362771515)) ;
#144857=CARTESIAN_POINT('Ctrl Pts',(-30.8452749040731,14.0323112919108,
128.676933371986)) ;
#144858=CARTESIAN_POINT('Ctrl Pts',(-30.8758787528105,13.747634010638,128.799431922669)) ;
#144859=CARTESIAN_POINT('Ctrl Pts',(-30.8807206526435,13.4408490944308,
128.846563950046)) ;
#144860=CARTESIAN_POINT('Ctrl Pts',(-30.8584669743735,13.1304291630284,
128.814803354541)) ;
#144861=CARTESIAN_POINT('Ctrl Pts',(-30.8102230492694,12.8426172833002,
128.706927901223)) ;
#144862=CARTESIAN_POINT('Ctrl Pts',(-30.738204665558,12.5951022439345,128.529786637205)) ;
#144863=CARTESIAN_POINT('Ctrl Pts',(-30.6479308981306,12.4086451367459,
128.299025630122)) ;
#144864=CARTESIAN_POINT('Ctrl Pts',(-30.5437885246526,12.2933533526165,
128.027999482058)) ;
#144865=CARTESIAN_POINT('Ctrl Pts',(-30.4331507484022,12.2596356642452,
127.737975845541)) ;
#144866=CARTESIAN_POINT('Ctrl Pts',(-30.3236687251324,12.3091205579985,
127.451195810082)) ;
#144867=CARTESIAN_POINT('Ctrl Pts',(-30.2218360682073,12.4379929419073,
127.186793272986)) ;
#144868=CARTESIAN_POINT('Ctrl Pts',(-30.133946584772,12.6386445208212,126.963302213587)) ;
#144869=CARTESIAN_POINT('Ctrl Pts',(-30.0665450383509,12.8942395319149,
126.799453338661)) ;
#144870=CARTESIAN_POINT('Ctrl Pts',(-30.0230172306372,13.1876524015431,
126.705370560951)) ;
#144871=CARTESIAN_POINT('Ctrl Pts',(-30.0058439958763,13.4984175352415,
126.688327152923)) ;
#144872=CARTESIAN_POINT('Ctrl Pts',(-30.0156793479209,13.804322978022,126.750244532428)) ;
#144873=CARTESIAN_POINT('Ctrl Pts',(-30.0510539190333,14.0825044690989,
126.886722797835)) ;
#144874=CARTESIAN_POINT('Ctrl Pts',(-30.1087723520417,14.3134151939565,
127.08849843816)) ;
#144875=CARTESIAN_POINT('Ctrl Pts',(-30.1834773985359,14.4799820430956,
127.339730220267)) ;
#144876=CARTESIAN_POINT('Ctrl Pts',(-30.2703212530767,14.5717629111611,
127.626756088476)) ;
#144877=CARTESIAN_POINT('Ctrl Pts',(-30.3605730980817,14.5804902345133,
127.923362492144)) ;
#144878=CARTESIAN_POINT('Ctrl Pts',(-30.4484207426051,14.5068426017295,
128.213109501132)) ;
#144879=CARTESIAN_POINT('Ctrl Pts',(-30.5264050460669,14.3556215142155,
128.474020614704)) ;
#144880=CARTESIAN_POINT('Ctrl Pts',(-30.5884484413862,14.1365915328991,
128.68850660419)) ;
#144881=CARTESIAN_POINT('Ctrl Pts',(-30.6287779145481,13.8680779330351,
128.839329518904)) ;
#144882=CARTESIAN_POINT('Ctrl Pts',(-30.6444633950159,13.567186800724,128.918249167054)) ;
#144883=CARTESIAN_POINT('Ctrl Pts',(-30.6330856943008,13.2537545062593,
128.918345572643)) ;
#144884=CARTESIAN_POINT('Ctrl Pts',(-30.5953085614819,12.9561224404112,
128.840913500029)) ;
#144885=CARTESIAN_POINT('Ctrl Pts',(-30.5325580838653,12.6895769772328,
128.690796474662)) ;
#144886=CARTESIAN_POINT('Ctrl Pts',(-30.4490933643888,12.4765148457442,
128.480030334778)) ;
#144887=CARTESIAN_POINT('Ctrl Pts',(-30.3494005172327,12.3303992852147,
128.22204710236)) ;
#144888=CARTESIAN_POINT('Ctrl Pts',(-30.2409395974139,12.2633426599666,
127.938263534079)) ;
#144889=CARTESIAN_POINT('Ctrl Pts',(-30.1300275403306,12.279103982185,127.647390711244)) ;
#144890=CARTESIAN_POINT('Ctrl Pts',(-30.0242396310796,12.3764767576561,
127.371421006722)) ;
#144891=CARTESIAN_POINT('Ctrl Pts',(-29.9297270127892,12.5500289101503,
127.128600360507)) ;
#144892=CARTESIAN_POINT('Ctrl Pts',(-29.8538880485749,12.7839578561676,
126.939986660771)) ;
#144893=CARTESIAN_POINT('Ctrl Pts',(-29.799920152433,13.0658041228342,126.815575584381)) ;
#144894=CARTESIAN_POINT('Ctrl Pts',(-29.7719515457904,13.3726170647806,
126.767011455076)) ;
#144895=CARTESIAN_POINT('Ctrl Pts',(-29.7709724043549,13.6826397531364,
126.797259660595)) ;
#144896=CARTESIAN_POINT('Ctrl Pts',(-29.7961074976013,13.9734160289762,
126.903696461442)) ;
#144897=CARTESIAN_POINT('Ctrl Pts',(-29.8454532437699,14.2269288377743,
127.081152783863)) ;
#144898=CARTESIAN_POINT('Ctrl Pts',(-29.9137639793214,14.4205112274409,
127.313664906998)) ;
#144899=CARTESIAN_POINT('Ctrl Pts',(-29.9963081148544,14.5441065971854,
127.58795480985)) ;
#144900=CARTESIAN_POINT('Ctrl Pts',(-30.0863453943646,14.5870792664814,
127.884190319798)) ;
#144901=CARTESIAN_POINT('Ctrl Pts',(-30.1762178473104,14.5462510463569,
128.179861707913)) ;
#144902=CARTESIAN_POINT('Ctrl Pts',(-30.2586647603345,14.426108976537,128.453668191511)) ;
#144903=CARTESIAN_POINT('Ctrl Pts',(-30.3282364972307,14.2320089292168,
128.690260384184)) ;
#144904=CARTESIAN_POINT('Ctrl Pts',(-30.3776572255911,13.9821034896837,
128.867612332903)) ;
#144905=CARTESIAN_POINT('Ctrl Pts',(-30.4036939249744,13.6914860951574,
128.976787558372)) ;
#144906=CARTESIAN_POINT('Ctrl Pts',(-30.4035328494657,13.3820426901867,
129.00937714575)) ;
#144907=CARTESIAN_POINT('Ctrl Pts',(-30.3760843784156,13.0731824495073,
128.962523652732)) ;
#144908=CARTESIAN_POINT('Ctrl Pts',(-30.3233314713119,12.7927891220342,
128.841355852443)) ;
#144909=CARTESIAN_POINT('Ctrl Pts',(-30.2475283569067,12.5553086793863,
128.653116181517)) ;
#144910=CARTESIAN_POINT('Ctrl Pts',(-30.1538708216962,12.3807971317929,
128.412623508798)) ;
#144911=CARTESIAN_POINT('Ctrl Pts',(-30.0481576035752,12.2807361314401,
128.136939366239)) ;
#144912=CARTESIAN_POINT('Ctrl Pts',(-29.9372735731522,12.2625961547027,
127.846148016714)) ;
#144913=CARTESIAN_POINT('Ctrl Pts',(-29.8284201756463,12.3275534841213,
127.561290415052)) ;
#144914=CARTESIAN_POINT('Ctrl Pts',(-29.7286735000512,12.4713200428819,
127.303059540576)) ;
#144915=CARTESIAN_POINT('Ctrl Pts',(-29.6447991067587,12.6818354528321,
127.091014736761)) ;
#144916=CARTESIAN_POINT('Ctrl Pts',(-29.5809833693557,12.9488696704077,
126.938002457017)) ;
#144917=CARTESIAN_POINT('Ctrl Pts',(-29.5426918772744,13.2449965342222,
126.858961210863)) ;
#144918=CARTESIAN_POINT('Ctrl Pts',(-29.5305163141329,13.5577147943103,
126.856660900313)) ;
#144919=CARTESIAN_POINT('Ctrl Pts',(-29.5453412160275,13.85913805832,126.933045258162)) ;
#144920=CARTESIAN_POINT('Ctrl Pts',(-29.5852299850096,14.1301670031634,
127.082751092509)) ;
#144921=CARTESIAN_POINT('Ctrl Pts',(-29.6464922978866,14.3498259886228,
127.294806891139)) ;
#144922=CARTESIAN_POINT('Ctrl Pts',(-29.7240191450472,14.5033075932482,
127.554372812427)) ;
#144923=CARTESIAN_POINT('Ctrl Pts',(-29.811746984037,14.5795881010438,127.84379574646)) ;
#144924=CARTESIAN_POINT('Ctrl Pts',(-29.902415821184,14.5729975043218,128.141770824574)) ;
#144925=CARTESIAN_POINT('Ctrl Pts',(-29.989169947926,14.4837968036715,128.428408489667)) ;
#144926=CARTESIAN_POINT('Ctrl Pts',(-30.0646586440251,14.3181445279312,
128.682117681586)) ;
#144927=CARTESIAN_POINT('Ctrl Pts',(-30.1225460634505,14.0900336140832,
128.884184874073)) ;
#144928=CARTESIAN_POINT('Ctrl Pts',(-30.1586763891653,13.812578673719,129.02292535409)) ;
#144929=CARTESIAN_POINT('Ctrl Pts',(-30.1692630060862,13.5087142835403,
129.086866972052)) ;
#144930=CARTESIAN_POINT('Ctrl Pts',(-30.1529569913643,13.1970641651478,
129.072436780848)) ;
#144931=CARTESIAN_POINT('Ctrl Pts',(-30.1101366557487,12.9023258221912,
128.98046898665)) ;
#144932=CARTESIAN_POINT('Ctrl Pts',(-30.0430710583863,12.644685125118,128.817716891912)) ;
#144933=CARTESIAN_POINT('Ctrl Pts',(-29.9563503393959,12.4436426605292,
128.597389723599)) ;
#144934=CARTESIAN_POINT('Ctrl Pts',(-29.8545813873611,12.3118006025232,
128.333283034123)) ;
#144935=CARTESIAN_POINT('Ctrl Pts',(-29.745052917924,12.2597626712743,128.046411581091)) ;
#144936=CARTESIAN_POINT('Ctrl Pts',(-29.6338703610585,12.291703918078,127.754949605098)) ;
#144937=CARTESIAN_POINT('Ctrl Pts',(-29.5303599253894,12.4035190278675,
127.485458923152)) ;
#144938=CARTESIAN_POINT('Ctrl Pts',(-29.4386293109041,12.5902948833878,
127.250828431852)) ;
#144939=CARTESIAN_POINT('Ctrl Pts',(-29.3668161784755,12.8337324563932,
127.07391082911)) ;
#144940=CARTESIAN_POINT('Ctrl Pts',(-29.317354785249,13.1235886445067,126.962832987765)) ;
#144941=CARTESIAN_POINT('Ctrl Pts',(-29.2946790039063,13.4302519414742,
126.929456186755)) ;
#144942=CARTESIAN_POINT('Ctrl Pts',(-29.2985403929367,13.7390104772614,
126.97389188522)) ;
#144943=CARTESIAN_POINT('Ctrl Pts',(-29.328778151289,14.0260062302898,127.095502531862)) ;
#144944=CARTESIAN_POINT('Ctrl Pts',(-29.3816257655434,14.267226902407,127.282822185877)) ;
#144945=CARTESIAN_POINT('Ctrl Pts',(-29.453365562884,14.4498458952908,127.525566557357)) ;
#144946=CARTESIAN_POINT('Ctrl Pts',(-29.5379200931215,14.5586319352592,
127.805747356859)) ;
#144947=CARTESIAN_POINT('Ctrl Pts',(-29.6284800570067,14.5856242088894,
128.103498661156)) ;
#144948=CARTESIAN_POINT('Ctrl Pts',(-29.7171136257346,14.5299078181027,
128.395370777147)) ;
#144949=CARTESIAN_POINT('Ctrl Pts',(-29.7982635715947,14.3940107606991,
128.665725835528)) ;
#144950=CARTESIAN_POINT('Ctrl Pts',(-29.8639971373026,14.1888420463645,
128.890864255151)) ;
#144951=CARTESIAN_POINT('Ctrl Pts',(-29.9093494029208,13.9299824320437,
129.056357542449)) ;
#144952=CARTESIAN_POINT('Ctrl Pts',(-29.9306079583778,13.6339608398866,
129.151584407244)) ;
#144953=CARTESIAN_POINT('Ctrl Pts',(-29.9252897878826,13.3227158538243,
129.16918084059)) ;
#144954=CARTESIAN_POINT('Ctrl Pts',(-29.8930268090175,13.018724359071,129.10806602458)) ;
#144955=CARTESIAN_POINT('Ctrl Pts',(-29.8356700823935,12.7442183705068,
128.973561223721)) ;
#144956=CARTESIAN_POINT('Ctrl Pts',(-29.7557212807804,12.5167188464288,
128.773322705119)) ;
#144957=CARTESIAN_POINT('Ctrl Pts',(-29.6597849157997,12.3563385813199,
128.526008620895)) ;
#144958=CARTESIAN_POINT('Ctrl Pts',(-29.5525354882502,12.2709228201269,
128.245853541108)) ;
#144959=CARTESIAN_POINT('Ctrl Pts',(-29.4411852696987,12.2686101214329,
127.953789784267)) ;
#144960=CARTESIAN_POINT('Ctrl Pts',(-29.3337984112996,12.3485946759632,
127.673127456804)) ;
#144961=CARTESIAN_POINT('Ctrl Pts',(-29.2360837324195,12.5068357117029,
127.420979418989)) ;
#144962=CARTESIAN_POINT('Ctrl Pts',(-29.1560520154867,12.7283302241023,
127.220079398763)) ;
#144963=CARTESIAN_POINT('Ctrl Pts',(-29.0969069082964,13.0013551128606,
127.080494500603)) ;
#144964=CARTESIAN_POINT('Ctrl Pts',(-29.0631494426447,13.3039532563625,
127.014974879755)) ;
#144965=CARTESIAN_POINT('Ctrl Pts',(-29.056172402243,13.6158509275634,127.027775962805)) ;
#144966=CARTESIAN_POINT('Ctrl Pts',(-29.0759852253016,13.9138456123568,
127.118835079156)) ;
#144967=CARTESIAN_POINT('Ctrl Pts',(-29.1200427275785,14.1752853033959,
127.280543177125)) ;
#144968=CARTESIAN_POINT('Ctrl Pts',(-29.184753849063,14.3839669210711,127.502694707301)) ;
#144969=CARTESIAN_POINT('Ctrl Pts',(-29.2650162806971,14.5240578631267,
127.770384402593)) ;
#144970=CARTESIAN_POINT('Ctrl Pts',(-29.3538119622672,14.584818935146,128.062899104014)) ;
#144971=CARTESIAN_POINT('Ctrl Pts',(-29.4445134401354,14.5621167265827,
128.3610733218)) ;
#144972=CARTESIAN_POINT('Ctrl Pts',(-29.5290814497335,14.4583966229727,
128.641100901953)) ;
#144973=CARTESIAN_POINT('Ctrl Pts',(-29.6017322946948,14.2803903749363,
128.886461046025)) ;
#144974=CARTESIAN_POINT('Ctrl Pts',(-29.6560964939787,14.0406559377366,
129.078419058495)) ;
#144975=CARTESIAN_POINT('Ctrl Pts',(-29.687572797519,13.7571590105316,129.203463231829)) ;
#144976=CARTESIAN_POINT('Ctrl Pts',(-29.6931036600313,13.4483332581187,
129.252866998852)) ;
#144977=CARTESIAN_POINT('Ctrl Pts',(-29.6718600493204,13.140610392606,129.223729521239)) ;
#144978=CARTESIAN_POINT('Ctrl Pts',(-29.6239436216886,12.8492377200964,
129.117118746748)) ;
#144979=CARTESIAN_POINT('Ctrl Pts',(-29.5529432008373,12.6021186062381,
128.942722101255)) ;
#144980=CARTESIAN_POINT('Ctrl Pts',(-29.4630752370502,12.4130744443633,
128.713206500985)) ;
#144981=CARTESIAN_POINT('Ctrl Pts',(-29.3588143740803,12.2953575363629,
128.441951701695)) ;
#144982=CARTESIAN_POINT('Ctrl Pts',(-29.2487309441084,12.259540004683,128.153408313109)) ;
#144983=CARTESIAN_POINT('Ctrl Pts',(-29.1390301351818,12.3063152851138,
127.866010362267)) ;
#144984=CARTESIAN_POINT('Ctrl Pts',(-29.0363094353862,12.4341408318063,
127.599216552733)) ;
#144985=CARTESIAN_POINT('Ctrl Pts',(-28.9486256458988,12.6316134862806,
127.376075640592)) ;
#144986=CARTESIAN_POINT('Ctrl Pts',(-28.8803727387758,12.8861350461837,
127.209806995649)) ;
#144987=CARTESIAN_POINT('Ctrl Pts',(-28.8360698049953,13.179213941093,127.113505163863)) ;
#144988=CARTESIAN_POINT('Ctrl Pts',(-28.818146099152,13.4905687882747,127.094349921822)) ;
#144989=CARTESIAN_POINT('Ctrl Pts',(-28.8273246021898,13.7964604527636,
127.154303567097)) ;
#144990=CARTESIAN_POINT('Ctrl Pts',(-28.8618427799844,14.0743848720617,
127.288127973483)) ;
#144991=CARTESIAN_POINT('Ctrl Pts',(-28.9187990753972,14.3070163090694,
127.487639078043)) ;
#144992=CARTESIAN_POINT('Ctrl Pts',(-28.9935556217395,14.4764518819419,
127.739221259018)) ;
#144993=CARTESIAN_POINT('Ctrl Pts',(-29.0794072904876,14.5698501931718,
128.023056840081)) ;
#144994=CARTESIAN_POINT('Ctrl Pts',(-29.1700992616621,14.5816111155488,
128.321126188998)) ;
#144995=CARTESIAN_POINT('Ctrl Pts',(-29.2583924640271,14.5098991366122,
128.612271870243)) ;
#144996=CARTESIAN_POINT('Ctrl Pts',(-29.3367774377786,14.3604029768198,
128.874384366338)) ;
#144997=CARTESIAN_POINT('Ctrl Pts',(-29.3991532586463,14.1435656071336,
129.089752826229)) ;
#144998=CARTESIAN_POINT('Ctrl Pts',(-29.4402243229761,13.8762645151226,
129.24274936311)) ;
#144999=CARTESIAN_POINT('Ctrl Pts',(-29.4565543469436,13.5746433207973,
129.323692326844)) ;
#145000=CARTESIAN_POINT('Ctrl Pts',(-29.446153488638,13.2647985797715,129.326253123723)) ;
#145001=CARTESIAN_POINT('Ctrl Pts',(-29.4089346093494,12.9638355607027,
129.250742958793)) ;
#145002=CARTESIAN_POINT('Ctrl Pts',(-29.3469241765837,12.6967406329269,
129.102706452313)) ;
#145003=CARTESIAN_POINT('Ctrl Pts',(-29.2638217308112,12.4815166817384,
128.89307257032)) ;
#145004=CARTESIAN_POINT('Ctrl Pts',(-29.1648556934516,12.3337893264045,
128.637089209316)) ;
#145005=CARTESIAN_POINT('Ctrl Pts',(-29.0563112696507,12.2640797848313,
128.353145898042)) ;
#145006=CARTESIAN_POINT('Ctrl Pts',(-28.9454975257324,12.2774691635847,
128.06251738632)) ;
#145007=CARTESIAN_POINT('Ctrl Pts',(-28.8394630097651,12.3724670755757,
127.785829298635)) ;
#145008=CARTESIAN_POINT('Ctrl Pts',(-28.74455141607,12.5437674769879,127.541819485266)) ;
#145009=CARTESIAN_POINT('Ctrl Pts',(-28.667987089546,12.7765747381498,127.351152652953)) ;
#145010=CARTESIAN_POINT('Ctrl Pts',(-28.6134535091621,13.056442748956,127.224981779766)) ;
#145011=CARTESIAN_POINT('Ctrl Pts',(-28.5846281837057,13.3632374806636,
127.173969984753)) ;
#145012=CARTESIAN_POINT('Ctrl Pts',(-28.5827519865197,13.6730055446753,
127.201534705381)) ;
#145013=CARTESIAN_POINT('Ctrl Pts',(-28.6074869894877,13.9671153512335,
127.30710875043)) ;
#145014=CARTESIAN_POINT('Ctrl Pts',(-28.6556926253068,14.2192391234479,
127.480866191476)) ;
#145015=CARTESIAN_POINT('Ctrl Pts',(-28.7239822741008,14.4164802375927,
127.713584818354)) ;
#145016=CARTESIAN_POINT('Ctrl Pts',(-28.8060651324488,14.5415580398573,
127.986435060222)) ;
#145017=CARTESIAN_POINT('Ctrl Pts',(-28.8956906557492,14.5869148378636,
128.281369404631)) ;
#145018=CARTESIAN_POINT('Ctrl Pts',(-28.98562546963,14.549009953407,128.577193806147)) ;
#145019=CARTESIAN_POINT('Ctrl Pts',(-29.0689498515829,14.4299835709606,
128.853812302228)) ;
#145020=CARTESIAN_POINT('Ctrl Pts',(-29.1383779103369,14.2395160277486,
129.089680125683)) ;
#145021=CARTESIAN_POINT('Ctrl Pts',(-29.1887817833045,13.9900850952094,
129.270073111603)) ;
#145022=CARTESIAN_POINT('Ctrl Pts',(-29.2155234000854,13.7002631098511,
129.381303903886)) ;
#145023=CARTESIAN_POINT('Ctrl Pts',(-29.2160909046462,13.3906063370585,
129.41607595645)) ;
#145024=CARTESIAN_POINT('Ctrl Pts',(-29.1895770572792,13.0826197342829,
129.371807848553)) ;
#145025=CARTESIAN_POINT('Ctrl Pts',(-29.1372769875413,12.7997480934514,
129.252135719739)) ;
#145026=CARTESIAN_POINT('Ctrl Pts',(-29.0622377639789,12.5614902723847,
129.066030746683)) ;
#145027=CARTESIAN_POINT('Ctrl Pts',(-28.9688868831584,12.3846250062646,
128.826489468998)) ;
#145028=CARTESIAN_POINT('Ctrl Pts',(-28.863379279089,12.2824687795427,128.551412625249)) ;
#145029=CARTESIAN_POINT('Ctrl Pts',(-28.7528489225533,12.2619556367439,
128.26156433009)) ;
#145030=CARTESIAN_POINT('Ctrl Pts',(-28.6437294898597,12.3244285368361,
127.975958900215)) ;
#145031=CARTESIAN_POINT('Ctrl Pts',(-28.543390154748,12.4664340564494,127.7160730758)) ;
#145032=CARTESIAN_POINT('Ctrl Pts',(-28.45911478577,12.6753487848156,127.502844610872)) ;
#145033=CARTESIAN_POINT('Ctrl Pts',(-28.3949800858147,12.9390315175275,
127.348664441927)) ;
#145034=CARTESIAN_POINT('Ctrl Pts',(-28.3555174386426,13.2369183961831,
127.266484174329)) ;
#145035=CARTESIAN_POINT('Ctrl Pts',(-28.3427341604387,13.5497744886041,
127.262423775639)) ;
#145036=CARTESIAN_POINT('Ctrl Pts',(-28.3567662936906,13.8506095454533,
127.336367876544)) ;
#145037=CARTESIAN_POINT('Ctrl Pts',(-28.3959609227216,14.1229210683533,
127.484053733088)) ;
#145038=CARTESIAN_POINT('Ctrl Pts',(-28.4565807352272,14.3440341407498,
127.694191101912)) ;
#145039=CARTESIAN_POINT('Ctrl Pts',(-28.533812846294,14.5000650906738,127.95294779839)) ;
#145040=CARTESIAN_POINT('Ctrl Pts',(-28.6217580585773,14.5786444747034,
128.243152404162)) ;
#145041=CARTESIAN_POINT('Ctrl Pts',(-28.7118706340383,14.5743811476286,
128.539290888972)) ;
#145042=CARTESIAN_POINT('Ctrl Pts',(-28.7991111237447,14.4873598311618,
128.82745330766)) ;
#145043=CARTESIAN_POINT('Ctrl Pts',(-28.8748372539666,14.3240886154077,
129.081775713549)) ;
#145044=CARTESIAN_POINT('Ctrl Pts',(-28.9333779405285,14.0972552260208,
129.285808257697)) ;
#145045=CARTESIAN_POINT('Ctrl Pts',(-28.9701540565685,13.8219066558181,
129.426323278948)) ;
#145046=CARTESIAN_POINT('Ctrl Pts',(-28.9815743172463,13.516025574875,129.492975539389)) ;
#145047=CARTESIAN_POINT('Ctrl Pts',(-28.9658944739719,13.2050736952722,
129.480284798213)) ;
#145048=CARTESIAN_POINT('Ctrl Pts',(-28.9239550053985,12.9106473531297,
129.390776717177)) ;
#145049=CARTESIAN_POINT('Ctrl Pts',(-28.8576902058508,12.6518068036689,
129.230321014171)) ;
#145050=CARTESIAN_POINT('Ctrl Pts',(-28.7711031640628,12.4481718276841,
129.010524241751)) ;
#145051=CARTESIAN_POINT('Ctrl Pts',(-28.6698281713027,12.3143466020562,
128.747799049023)) ;
#145052=CARTESIAN_POINT('Ctrl Pts',(-28.5598558153291,12.2602411283263,
128.459807572917)) ;
#145053=CARTESIAN_POINT('Ctrl Pts',(-28.4501327796536,12.289044221804,128.172135467012)) ;
#145054=CARTESIAN_POINT('Ctrl Pts',(-28.3450924897601,12.3996399121577,
127.898576733604)) ;
#145055=CARTESIAN_POINT('Ctrl Pts',(-28.2537095920121,12.5827969137066,
127.664649432031)) ;
#145056=CARTESIAN_POINT('Ctrl Pts',(-28.1805860737797,12.8269629913892,
127.4842275229)) ;
#145057=CARTESIAN_POINT('Ctrl Pts',(-28.1309253611483,13.1127056194501,
127.372192542966)) ;
#145058=CARTESIAN_POINT('Ctrl Pts',(-28.1070965691472,13.4217118754633,
127.335748937024)) ;
#145059=CARTESIAN_POINT('Ctrl Pts',(-28.1103019107213,13.7304251092952,
127.378225357934)) ;
#145060=CARTESIAN_POINT('Ctrl Pts',(-28.1397723896426,14.0183443121755,
127.497588937897)) ;
#145061=CARTESIAN_POINT('Ctrl Pts',(-28.1921615804711,14.2615012050008,
127.68363777181)) ;
#145062=CARTESIAN_POINT('Ctrl Pts',(-28.2633477193032,14.4455241702922,
127.924703064281)) ;
#145063=CARTESIAN_POINT('Ctrl Pts',(-28.3473562951541,14.5564730573808,
128.20319199203)) ;
#145064=CARTESIAN_POINT('Ctrl Pts',(-28.4381713240423,14.5860332568258,
128.501810889804)) ;
#145065=CARTESIAN_POINT('Ctrl Pts',(-28.5267754984946,14.5327319791753,
128.79353140372)) ;
#145066=CARTESIAN_POINT('Ctrl Pts',(-28.6083489557468,14.3988254927601,
129.065167069407)) ;
#145067=CARTESIAN_POINT('Ctrl Pts',(-28.674312050933,14.1966329256883,129.290810388347)) ;
#145068=CARTESIAN_POINT('Ctrl Pts',(-28.7206126327925,13.9381994026002,
129.459218514531)) ;
#145069=CARTESIAN_POINT('Ctrl Pts',(-28.7425880079729,13.6421506980583,
129.55661445211)) ;
#145070=CARTESIAN_POINT('Ctrl Pts',(-28.7380161215275,13.3319747136995,
129.576294413639)) ;
#145071=CARTESIAN_POINT('Ctrl Pts',(-28.7066575696832,13.0275240722509,
129.517800451875)) ;
#145072=CARTESIAN_POINT('Ctrl Pts',(-28.6494163393576,12.7499512402199,
129.383895833374)) ;
#145073=CARTESIAN_POINT('Ctrl Pts',(-28.570733840793,12.5230805349149,129.187040404072)) ;
#145074=CARTESIAN_POINT('Ctrl Pts',(-28.4747567031311,12.3595163071095,
128.939784733654)) ;
#145075=CARTESIAN_POINT('Ctrl Pts',(-28.3674514892643,12.2720600916224,
128.659532359337)) ;
#145076=CARTESIAN_POINT('Ctrl Pts',(-28.2563402590024,12.2676665525214,
128.36809970917)) ;
#145077=CARTESIAN_POINT('Ctrl Pts',(-28.1491360838674,12.3451448696153,
128.08785944284)) ;
#145078=CARTESIAN_POINT('Ctrl Pts',(-28.0512687436739,12.5004783202174,
127.835162531413)) ;
#145079=CARTESIAN_POINT('Ctrl Pts',(-27.9702282254497,12.7212078449696,
127.631477262919)) ;
#145080=CARTESIAN_POINT('Ctrl Pts',(-27.9103930589021,12.9936146304865,
127.489925505009)) ;
#145081=CARTESIAN_POINT('Ctrl Pts',(-27.8760021682395,13.2947838231295,
127.422460801043)) ;
#145082=CARTESIAN_POINT('Ctrl Pts',(-27.8682065706614,13.6064069014527,
127.432836288194)) ;
#145083=CARTESIAN_POINT('Ctrl Pts',(-27.8871850592498,13.9050218268895,
127.521439035055)) ;
#145084=CARTESIAN_POINT('Ctrl Pts',(-27.9307052432448,14.1686337353897,
127.681683087378)) ;
#145085=CARTESIAN_POINT('Ctrl Pts',(-27.9948873964674,14.3788183161701,
127.902267366194)) ;
#145086=CARTESIAN_POINT('Ctrl Pts',(-28.0745692281525,14.520866298431,128.168177014756)) ;
#145087=CARTESIAN_POINT('Ctrl Pts',(-28.1633227835529,14.5841620003351,
128.460616494003)) ;
#145088=CARTESIAN_POINT('Ctrl Pts',(-28.2537824709229,14.5641966090762,
128.757971972895)) ;
#145089=CARTESIAN_POINT('Ctrl Pts',(-28.3390215958204,14.4625801801971,
129.040108638781)) ;
#145090=CARTESIAN_POINT('Ctrl Pts',(-28.4122062994549,14.2860054922745,
129.287088654733)) ;
#145091=CARTESIAN_POINT('Ctrl Pts',(-28.466988907218,14.0484511491475,129.480174962356)) ;
#145092=CARTESIAN_POINT('Ctrl Pts',(-28.4991949158601,13.7663469405247,
129.607316620214)) ;
#145093=CARTESIAN_POINT('Ctrl Pts',(-28.5055693504399,13.4574607709576,
129.659232632401)) ;
#145094=CARTESIAN_POINT('Ctrl Pts',(-28.4849795148332,13.1488899250601,
129.632073485812)) ;
#145095=CARTESIAN_POINT('Ctrl Pts',(-28.438125868901,12.8583365008137,129.528365294442)) ;
#145096=CARTESIAN_POINT('Ctrl Pts',(-28.3675738014983,12.6085157648157,
129.355411721836)) ;
#145097=CARTESIAN_POINT('Ctrl Pts',(-28.2779335638049,12.4173946912655,
129.126629988132)) ;
#145098=CARTESIAN_POINT('Ctrl Pts',(-28.1745614589347,12.2980452527152,
128.857787657823)) ;
#145099=CARTESIAN_POINT('Ctrl Pts',(-28.0644798746441,12.2592457777712,
128.569281832608)) ;
#145100=CARTESIAN_POINT('Ctrl Pts',(-27.9541455681162,12.3040208605449,
128.280192572425)) ;
#145101=CARTESIAN_POINT('Ctrl Pts',(-27.8518137736169,12.4286939369855,
128.01430350491)) ;
#145102=CARTESIAN_POINT('Ctrl Pts',(-27.7632715398407,12.6243590090332,
127.788745391501)) ;
#145103=CARTESIAN_POINT('Ctrl Pts',(-27.6940711138233,12.8789083522399,
127.619878057419)) ;
#145104=CARTESIAN_POINT('Ctrl Pts',(-27.6492626440896,13.1702261318585,
127.521984841382)) ;
#145105=CARTESIAN_POINT('Ctrl Pts',(-27.6305164470897,13.4805037318096,
127.500338767568)) ;
#145106=CARTESIAN_POINT('Ctrl Pts',(-27.638835187958,13.7876511812746,127.557856305416)) ;
#145107=CARTESIAN_POINT('Ctrl Pts',(-27.6729022423348,14.0678452982214,
127.690522212597)) ;
#145108=CARTESIAN_POINT('Ctrl Pts',(-27.7290143253781,14.3007432991358,
127.887391380954)) ;
#145109=CARTESIAN_POINT('Ctrl Pts',(-27.8033875281781,14.472578666663,128.137894751171)) ;
#145110=CARTESIAN_POINT('Ctrl Pts',(-27.8890145289959,14.5682598997855,
128.42107403151)) ;
#145111=CARTESIAN_POINT('Ctrl Pts',(-27.9796584294107,14.5824152858443,
128.719000952207)) ;
#145112=CARTESIAN_POINT('Ctrl Pts',(-28.0679946971491,14.5133614382036,
129.010212950777)) ;
#145113=CARTESIAN_POINT('Ctrl Pts',(-28.1468971665483,14.3656854854221,
129.273906123905)) ;
#145114=CARTESIAN_POINT('Ctrl Pts',(-28.209580420455,14.1519222579812,129.490000886093)) ;
#145115=CARTESIAN_POINT('Ctrl Pts',(-28.2516699552296,13.8839964820202,
129.646218872573)) ;
#145116=CARTESIAN_POINT('Ctrl Pts',(-28.268649225353,13.5839684953717,129.728941659316)) ;
#145117=CARTESIAN_POINT('Ctrl Pts',(-28.2590350628778,13.2736209953703,
129.733860927166)) ;
#145118=CARTESIAN_POINT('Ctrl Pts',(-28.2226940752123,12.9727615411734,
129.66082637878)) ;
#145119=CARTESIAN_POINT('Ctrl Pts',(-28.1611673220689,12.7034620049653,
129.514320432465)) ;
#145120=CARTESIAN_POINT('Ctrl Pts',(-28.0786249670964,12.4867211493109,
129.306299596008)) ;
#145121=CARTESIAN_POINT('Ctrl Pts',(-27.9799272757244,12.3368636809282,
129.051131387346)) ;
#145122=CARTESIAN_POINT('Ctrl Pts',(-27.8719194784827,12.2650346838616,
128.768645899096)) ;
#145123=CARTESIAN_POINT('Ctrl Pts',(-27.7607881458193,12.2758062745913,
128.477173097563)) ;
#145124=CARTESIAN_POINT('Ctrl Pts',(-27.6541366047843,12.3692807546481,
128.198814238508)) ;
#145125=CARTESIAN_POINT('Ctrl Pts',(-27.5593097138098,12.5378929706017,
127.954885764186)) ;
#145126=CARTESIAN_POINT('Ctrl Pts',(-27.4820169207693,12.7694277831183,
127.762148018036)) ;
#145127=CARTESIAN_POINT('Ctrl Pts',(-27.4267956575346,13.0484836383152,
127.633986587578)) ;
#145128=CARTESIAN_POINT('Ctrl Pts',(-27.3972448682813,13.3553252345684,
127.580904766868)) ;
#145129=CARTESIAN_POINT('Ctrl Pts',(-27.3946987479372,13.6640556396721,
127.606387504147)) ;
#145130=CARTESIAN_POINT('Ctrl Pts',(-27.4184411975963,13.9577070644724,
127.708900115504)) ;
#145131=CARTESIAN_POINT('Ctrl Pts',(-27.4662212855069,14.2128779960594,
127.881609402868)) ;
#145132=CARTESIAN_POINT('Ctrl Pts',(-27.5340439011821,14.4117544272494,
128.112953198524)) ;
#145133=CARTESIAN_POINT('Ctrl Pts',(-27.6157591745542,14.5391283033453,
128.384716022554)) ;
#145134=CARTESIAN_POINT('Ctrl Pts',(-27.7056825536617,14.5867879380275,
128.680669932691)) ;
#145135=CARTESIAN_POINT('Ctrl Pts',(-27.7952749803668,14.5512051546367,
128.975335967388)) ;
#145136=CARTESIAN_POINT('Ctrl Pts',(-27.879035841241,14.4343419889086,129.253282623546)) ;
#145137=CARTESIAN_POINT('Ctrl Pts',(-27.9489094001948,14.2455278937518,
129.490460406613)) ;
#145138=CARTESIAN_POINT('Ctrl Pts',(-27.999822466142,13.9981929158514,129.672259071705)) ;
#145139=CARTESIAN_POINT('Ctrl Pts',(-28.027364677321,13.7085066698523,129.785915013751)) ;
#145140=CARTESIAN_POINT('Ctrl Pts',(-28.0286285492022,13.3995793870564,
129.822670392743)) ;
#145141=CARTESIAN_POINT('Ctrl Pts',(-28.0030498332934,13.0919774585784,
129.781044462692)) ;
#145142=CARTESIAN_POINT('Ctrl Pts',(-27.9511801663322,12.8067303604848,
129.662796978732)) ;
#145143=CARTESIAN_POINT('Ctrl Pts',(-27.8771115641797,12.5682008646981,
129.479352709281)) ;
#145144=CARTESIAN_POINT('Ctrl Pts',(-27.7840799881775,12.3888212047449,
129.240810402594)) ;
#145145=CARTESIAN_POINT('Ctrl Pts',(-27.6789762774325,12.2844119375082,
128.966867849549)) ;
#145146=CARTESIAN_POINT('Ctrl Pts',(-27.5681554143404,12.2613333969067,
128.676275527954)) ;
#145147=CARTESIAN_POINT('Ctrl Pts',(-27.4590172958769,12.3215794743214,
128.390578491288)) ;
#145148=CARTESIAN_POINT('Ctrl Pts',(-27.3586454587107,12.4606919481936,
128.13048055496)) ;
#145149=CARTESIAN_POINT('Ctrl Pts',(-27.2734486429436,12.6684214506416,
127.914688951451)) ;
#145150=CARTESIAN_POINT('Ctrl Pts',(-27.2085144692729,12.9319196123432,
127.758288713112)) ;
#145151=CARTESIAN_POINT('Ctrl Pts',(-27.1685755827829,13.2279083302756,
127.674578003213)) ;
#145152=CARTESIAN_POINT('Ctrl Pts',(-27.1549269841447,13.5392234184095,
127.667835412627)) ;
#145153=CARTESIAN_POINT('Ctrl Pts',(-27.1681724778946,13.8421684111979,
127.73964287137)) ;
#145154=CARTESIAN_POINT('Ctrl Pts',(-27.2067395795055,14.1158321070144,
127.885518848952)) ;
#145155=CARTESIAN_POINT('Ctrl Pts',(-27.2669534578115,14.339009376798,128.094538209038)) ;
#145156=CARTESIAN_POINT('Ctrl Pts',(-27.3436695138408,14.4964746049257,
128.351715170359)) ;
#145157=CARTESIAN_POINT('Ctrl Pts',(-27.4308784775676,14.5773715889881,
128.639578138836)) ;
#145158=CARTESIAN_POINT('Ctrl Pts',(-27.5216935080159,14.5757025147149,
128.93802333203)) ;
#145159=CARTESIAN_POINT('Ctrl Pts',(-27.6088983693204,14.490867072331,129.225995722479)) ;
#145160=CARTESIAN_POINT('Ctrl Pts',(-27.6847829789678,14.330592253299,129.48065337557)) ;
#145161=CARTESIAN_POINT('Ctrl Pts',(-27.7442105909782,14.1048089901007,
129.687399172449)) ;
#145162=CARTESIAN_POINT('Ctrl Pts',(-27.7816984625605,13.8293690778141,
129.830119558559)) ;
#145163=CARTESIAN_POINT('Ctrl Pts',(-27.7938050924863,13.526576284789,129.898498223956)) ;
#145164=CARTESIAN_POINT('Ctrl Pts',(-27.7790423798048,13.2147294294983,
129.888571224088)) ;
#145165=CARTESIAN_POINT('Ctrl Pts',(-27.7378005231724,12.9189024654219,
129.801161820441)) ;
#145166=CARTESIAN_POINT('Ctrl Pts',(-27.6719242811303,12.6580299108607,
129.641948932191)) ;
#145167=CARTESIAN_POINT('Ctrl Pts',(-27.5862120750185,12.4534345481142,
129.424564279788)) ;
#145168=CARTESIAN_POINT('Ctrl Pts',(-27.4850277388239,12.3171076600088,
129.162191557086)) ;
#145169=CARTESIAN_POINT('Ctrl Pts',(-27.3757741136007,12.2606844017973,
128.876123071525)) ;
#145170=CARTESIAN_POINT('Ctrl Pts',(-27.2651782726929,12.2870889602567,
128.586143047142)) ;
#145171=CARTESIAN_POINT('Ctrl Pts',(-27.1599366275124,12.3957983185939,
128.311983337171)) ;
#145172=CARTESIAN_POINT('Ctrl Pts',(-27.068323828863,12.576725714127,128.07731803016)) ;
#145173=CARTESIAN_POINT('Ctrl Pts',(-26.9946972364049,12.8186993235838,
127.895349858883)) ;
#145174=CARTESIAN_POINT('Ctrl Pts',(-26.9440717391415,13.1050418168408,
127.780675308402)) ;
#145175=CARTESIAN_POINT('Ctrl Pts',(-26.9196285238679,13.4130762749516,
127.742359347898)) ;
#145176=CARTESIAN_POINT('Ctrl Pts',(-26.9220777684625,13.7214651862128,
127.782568022446)) ;
#145177=CARTESIAN_POINT('Ctrl Pts',(-26.9505714061639,14.0093161749257,
127.898936305092)) ;
#145178=CARTESIAN_POINT('Ctrl Pts',(-27.0027689908232,14.2560736746896,
128.084708180528)) ;
#145179=CARTESIAN_POINT('Ctrl Pts',(-27.0733529928704,14.4412184365536,
128.323910527195)) ;
#145180=CARTESIAN_POINT('Ctrl Pts',(-27.1570667414105,14.5543182537731,
128.601539623747)) ;
#145181=CARTESIAN_POINT('Ctrl Pts',(-27.2473775377621,14.5864671229327,
128.89852477223)) ;
#145182=CARTESIAN_POINT('Ctrl Pts',(-27.3367275624371,14.5351930359694,
129.19265847879)) ;
#145183=CARTESIAN_POINT('Ctrl Pts',(-27.4181292069275,14.4042256510203,
129.463583735512)) ;
#145184=CARTESIAN_POINT('Ctrl Pts',(-27.4849111444952,14.2033619799806,
129.691746469449)) ;
#145185=CARTESIAN_POINT('Ctrl Pts',(-27.5318288818491,13.9460942692561,
129.861964597238)) ;
#145186=CARTESIAN_POINT('Ctrl Pts',(-27.5545247889339,13.6510939576202,
129.96143831759)) ;
#145187=CARTESIAN_POINT('Ctrl Pts',(-27.550764534156,13.3409631929891,129.983496828996)) ;
#145188=CARTESIAN_POINT('Ctrl Pts',(-27.5200421487155,13.0355468372364,
129.926920899871)) ;
#145189=CARTESIAN_POINT('Ctrl Pts',(-27.463891512529,12.7584809477333,129.795997149247)) ;
#145190=CARTESIAN_POINT('Ctrl Pts',(-27.3855386705038,12.5287898024968,
129.600244223915)) ;
#145191=CARTESIAN_POINT('Ctrl Pts',(-27.2899654965722,12.3633456659364,
129.35415921584)) ;
#145192=CARTESIAN_POINT('Ctrl Pts',(-27.1832672774182,12.2737023197767,
129.075570207765)) ;
#145193=CARTESIAN_POINT('Ctrl Pts',(-27.0721332475999,12.2663504667095,
128.784079554544)) ;
#145194=CARTESIAN_POINT('Ctrl Pts',(-26.9640750440213,12.34208017502,128.501551995175)) ;
#145195=CARTESIAN_POINT('Ctrl Pts',(-26.8662978136907,12.4946576903152,
128.248958027811)) ;
#145196=CARTESIAN_POINT('Ctrl Pts',(-26.7844064413056,12.7142650578431,
128.042896300319)) ;
#145197=CARTESIAN_POINT('Ctrl Pts',(-26.7239781458071,12.9853995961956,
127.899588524508)) ;
#145198=CARTESIAN_POINT('Ctrl Pts',(-26.6888087161657,13.2860375673385,
127.829858435003)) ;
#145199=CARTESIAN_POINT('Ctrl Pts',(-26.6802656934047,13.5985523264733,
127.838138380085)) ;
#145200=CARTESIAN_POINT('Ctrl Pts',(-26.6986085159139,13.8975129640997,
127.924860800194)) ;
#145201=CARTESIAN_POINT('Ctrl Pts',(-26.7412689213863,14.1612607305214,
128.082449499982)) ;
#145202=CARTESIAN_POINT('Ctrl Pts',(-26.8050662272223,14.3739608986485,
128.302005079039)) ;
#145203=CARTESIAN_POINT('Ctrl Pts',(-26.8846809635726,14.5182947311408,
128.567816786118)) ;
#145204=CARTESIAN_POINT('Ctrl Pts',(-26.9731269723443,14.5834512891337,
128.859295413823)) ;
#145205=CARTESIAN_POINT('Ctrl Pts',(-27.063336767471,14.5659482056826,129.155813358164)) ;
#145206=CARTESIAN_POINT('Ctrl Pts',(-27.1488060860294,14.4667697468738,
129.438612349934)) ;
#145207=CARTESIAN_POINT('Ctrl Pts',(-27.2225032558955,14.2923285358451,
129.68709763699)) ;
#145208=CARTESIAN_POINT('Ctrl Pts',(-27.2781332705648,14.0548140143778,
129.882849456784)) ;
#145209=CARTESIAN_POINT('Ctrl Pts',(-27.3107599426325,13.7751053966171,
130.011041198749)) ;
#145210=CARTESIAN_POINT('Ctrl Pts',(-27.3180362901016,13.4671706685235,
130.065540763481)) ;
#145211=CARTESIAN_POINT('Ctrl Pts',(-27.298042554253,13.1566326629542,130.040310967005)) ;
#145212=CARTESIAN_POINT('Ctrl Pts',(-27.2521782342998,12.8670308580196,
129.939287114639)) ;
#145213=CARTESIAN_POINT('Ctrl Pts',(-27.1820662948561,12.614625742012,129.767747675979)) ;
#145214=CARTESIAN_POINT('Ctrl Pts',(-27.0926762160904,12.4216271710516,
129.539751137083)) ;
#145215=CARTESIAN_POINT('Ctrl Pts',(-26.9900934748709,12.3004936351809,
129.273060908702)) ;
#145216=CARTESIAN_POINT('Ctrl Pts',(-26.8794850458073,12.2591976942699,
128.983206367494)) ;
#145217=CARTESIAN_POINT('Ctrl Pts',(-26.769798191186,12.3014766458867,128.695782118538)) ;
#145218=CARTESIAN_POINT('Ctrl Pts',(-26.6668884802955,12.4236752425343,
128.428268347536)) ;
#145219=CARTESIAN_POINT('Ctrl Pts',(-26.5773353042428,12.6191375618547,
128.199983809857)) ;
#145220=CARTESIAN_POINT('Ctrl Pts',(-26.5080282119653,12.8707902517674,
128.030586096778)) ;
#145221=CARTESIAN_POINT('Ctrl Pts',(-26.4623661086803,13.1617413465553,
127.930263010471)) ;
#145222=CARTESIAN_POINT('Ctrl Pts',(-26.4429131084249,13.4713353015044,
127.906497282117)) ;
#145223=CARTESIAN_POINT('Ctrl Pts',(-26.4504147849802,13.7785022490456,
127.961585642172)) ;
#145224=CARTESIAN_POINT('Ctrl Pts',(-26.4836546467707,14.0596469751513,
128.091803410612)) ;
#145225=CARTESIAN_POINT('Ctrl Pts',(-26.5394610982308,14.2953142931135,
128.287948833244)) ;
#145226=CARTESIAN_POINT('Ctrl Pts',(-26.6134196928557,14.468964761841,128.537226975926)) ;
#145227=CARTESIAN_POINT('Ctrl Pts',(-26.6990820403619,14.566840747798,128.820608211893)) ;
#145228=CARTESIAN_POINT('Ctrl Pts',(-26.7892429864435,14.5831863557758,
129.116954844477)) ;
#145229=CARTESIAN_POINT('Ctrl Pts',(-26.8781110470037,14.5160478882273,
129.409866842151)) ;
#145230=CARTESIAN_POINT('Ctrl Pts',(-26.956952315364,14.3710572999732,129.673209306742)) ;
#145231=CARTESIAN_POINT('Ctrl Pts',(-27.0203223929184,14.1586831437498,
129.891382565407)) ;
#145232=CARTESIAN_POINT('Ctrl Pts',(-27.0629647324315,13.8924167167611,
130.049154173624)) ;
#145233=CARTESIAN_POINT('Ctrl Pts',(-27.0807543092698,13.5934589593166,
130.134207108121)) ;
#145234=CARTESIAN_POINT('Ctrl Pts',(-27.0718785730549,13.2817948443867,
130.141423438504)) ;
#145235=CARTESIAN_POINT('Ctrl Pts',(-27.036211707864,12.9807519837477,130.070323117634)) ;
#145236=CARTESIAN_POINT('Ctrl Pts',(-26.9757193317698,12.7114087835464,
129.926679055096)) ;
#145237=CARTESIAN_POINT('Ctrl Pts',(-26.8934530739077,12.4920355070178,
129.71959003431)) ;
#145238=CARTESIAN_POINT('Ctrl Pts',(-26.7954032837469,12.340409192469,129.466223268637)) ;
#145239=CARTESIAN_POINT('Ctrl Pts',(-26.6872087381884,12.2658594126602,
129.183310594939)) ;
#145240=CARTESIAN_POINT('Ctrl Pts',(-26.5762060450296,12.2744067953506,
128.892167277779)) ;
#145241=CARTESIAN_POINT('Ctrl Pts',(-26.4696120195096,12.3651074088565,
128.61388267482)) ;
#145242=CARTESIAN_POINT('Ctrl Pts',(-26.3741832777799,12.5316553295761,
128.368240358776)) ;
#145243=CARTESIAN_POINT('Ctrl Pts',(-26.2960979131251,12.7621962066438,
128.173274307522)) ;
#145244=CARTESIAN_POINT('Ctrl Pts',(-26.2402918341511,13.0400249877383,
128.043379258454)) ;
#145245=CARTESIAN_POINT('Ctrl Pts',(-26.209984773203,13.3449925663018,127.987941407805)) ;
#145246=CARTESIAN_POINT('Ctrl Pts',(-26.2066126024052,13.6560824874518,
128.01124626749)) ;
#145247=CARTESIAN_POINT('Ctrl Pts',(-26.2296304118587,13.949523069505,128.111533856934)) ;
#145248=CARTESIAN_POINT('Ctrl Pts',(-26.2767111329634,14.2060602321428,
128.282193262609)) ;
#145249=CARTESIAN_POINT('Ctrl Pts',(-26.3440044394362,14.4068533843326,
128.511982775146)) ;
#145250=CARTESIAN_POINT('Ctrl Pts',(-26.4255019943792,14.5364834537221,
128.783152349287)) ;
#145251=CARTESIAN_POINT('Ctrl Pts',(-26.5149273646816,14.5865952294226,
129.077512486312)) ;
#145252=CARTESIAN_POINT('Ctrl Pts',(-26.6050918737861,14.5532896916384,
129.374032831588)) ;
#145253=CARTESIAN_POINT('Ctrl Pts',(-26.6887557362477,14.4391769961996,
129.651538401177)) ;
#145254=CARTESIAN_POINT('Ctrl Pts',(-26.7592891858962,14.2521193934998,
129.890716002212)) ;
#145255=CARTESIAN_POINT('Ctrl Pts',(-26.8108385572124,14.0064610043906,
130.074351365964)) ;
#145256=CARTESIAN_POINT('Ctrl Pts',(-26.8391959482818,13.7162751862111,
130.190548474023)) ;
#145257=CARTESIAN_POINT('Ctrl Pts',(-26.8411767728426,13.4088590372399,
130.229260162228)) ;
#145258=CARTESIAN_POINT('Ctrl Pts',(-26.8163531916444,13.10053389726,130.189883749462)) ;
#145259=CARTESIAN_POINT('Ctrl Pts',(-26.7654365125188,12.8153801351655,
130.07428755891)) ;
#145260=CARTESIAN_POINT('Ctrl Pts',(-26.6918270487183,12.5742829301141,
129.892291503174)) ;
#145261=CARTESIAN_POINT('Ctrl Pts',(-26.5987510300196,12.3924207645517,
129.653771309622)) ;
#145262=CARTESIAN_POINT('Ctrl Pts',(-26.494437484084,12.2864008460228,129.381964574177)) ;
#145263=CARTESIAN_POINT('Ctrl Pts',(-26.3833229207034,12.2608494094795,
129.090623959521)) ;
#145264=CARTESIAN_POINT('Ctrl Pts',(-26.2745004596113,12.318610673207,128.805709814383)) ;
#145265=CARTESIAN_POINT('Ctrl Pts',(-26.1735653192533,12.4554523498405,
128.544018330009)) ;
#145266=CARTESIAN_POINT('Ctrl Pts',(-26.0875660779443,12.6626735869421,
128.326034888429)) ;
#145267=CARTESIAN_POINT('Ctrl Pts',(-26.0226228583949,12.9221026671482,
128.169263802032)) ;
#145268=CARTESIAN_POINT('Ctrl Pts',(-25.9815253480016,13.2188659560216,
128.082358785624)) ;
#145269=CARTESIAN_POINT('Ctrl Pts',(-25.9671690642881,13.5309970504502,
128.073639559481)) ;
#145270=CARTESIAN_POINT('Ctrl Pts',(-25.9796292863015,13.833391117926,128.143036056483)) ;
#145271=CARTESIAN_POINT('Ctrl Pts',(-26.0174576883516,14.1082733327472,
128.286754126692)) ;
#145272=CARTESIAN_POINT('Ctrl Pts',(-26.0770945744703,14.333273457915,128.494092864001)) ;
#145273=CARTESIAN_POINT('Ctrl Pts',(-26.1535867878669,14.493089968581,128.750689737769)) ;
#145274=CARTESIAN_POINT('Ctrl Pts',(-26.240492285696,14.5762694878071,129.037623503028)) ;
#145275=CARTESIAN_POINT('Ctrl Pts',(-26.3316446527599,14.5766426332955,
129.337185238566)) ;
#145276=CARTESIAN_POINT('Ctrl Pts',(-26.4182679904325,14.4950561386841,
129.623146842004)) ;
#145277=CARTESIAN_POINT('Ctrl Pts',(-26.4952465067177,14.3357812086937,
129.881281959693)) ;
#145278=CARTESIAN_POINT('Ctrl Pts',(-26.5549921587296,14.1117725486506,
130.08888574024)) ;
#145279=CARTESIAN_POINT('Ctrl Pts',(-26.5931611985058,13.8385111509001,
130.233491753311)) ;
#145280=CARTESIAN_POINT('Ctrl Pts',(-26.6060312661162,13.5338961508562,
130.304356398855)) ;
#145281=CARTESIAN_POINT('Ctrl Pts',(-26.5921064352985,13.224257482388,130.296623484146)) ;
#145282=CARTESIAN_POINT('Ctrl Pts',(-26.5514075441165,12.9262818286679,
130.210970393599)) ;
#145283=CARTESIAN_POINT('Ctrl Pts',(-26.4865801356298,12.6654697880194,
130.054625548478)) ;
#145284=CARTESIAN_POINT('Ctrl Pts',(-26.4005704729957,12.4574145749278,
129.836677200713)) ;
#145285=CARTESIAN_POINT('Ctrl Pts',(-26.3007750838948,12.3205165370977,
129.578002098338)) ;
#145286=CARTESIAN_POINT('Ctrl Pts',(-26.1910732522884,12.2610390449612,
129.290819720059)) ;
#145287=CARTESIAN_POINT('Ctrl Pts',(-26.0807718810186,12.2851065235111,
129.00158758569)) ;
#145288=CARTESIAN_POINT('Ctrl Pts',(-25.9751380722918,12.3913707658575,
128.726315756247)) ;
#145289=CARTESIAN_POINT('Ctrl Pts',(-25.8829725862754,12.5705078939367,
128.490066749863)) ;
#145290=CARTESIAN_POINT('Ctrl Pts',(-25.8087402089946,12.8110531024917,
128.306339450124)) ;
#145291=CARTESIAN_POINT('Ctrl Pts',(-25.7574503041843,13.0958081066442,
128.189657242365)) ;
#145292=CARTESIAN_POINT('Ctrl Pts',(-25.7321614965632,13.4043791396556,
128.148971680577)) ;
#145293=CARTESIAN_POINT('Ctrl Pts',(-25.7338009498791,13.7127503611852,
128.186770642114)) ;
#145294=CARTESIAN_POINT('Ctrl Pts',(-25.7619120955808,14.0031465384866,
128.302242202483)) ;
#145295=CARTESIAN_POINT('Ctrl Pts',(-25.8127877498031,14.2480984869967,
128.483700631739)) ;
#145296=CARTESIAN_POINT('Ctrl Pts',(-25.883318478156,14.4370589144751,128.723005956744)) ;
#145297=CARTESIAN_POINT('Ctrl Pts',(-25.9667449820352,14.5521322480481,
128.999773748139)) ;
#145298=CARTESIAN_POINT('Ctrl Pts',(-26.0570620921973,14.5867077636068,
129.296815980901)) ;
#145299=CARTESIAN_POINT('Ctrl Pts',(-26.1463754355628,14.5378478925882,
129.59078041807)) ;
#145300=CARTESIAN_POINT('Ctrl Pts',(-26.2280883194995,14.409203021957,129.862607874009)) ;
#145301=CARTESIAN_POINT('Ctrl Pts',(-26.2954388715456,14.2102655044933,
130.092438570625)) ;
#145302=CARTESIAN_POINT('Ctrl Pts',(-26.3431293730661,13.9531164546974,
130.265060015164)) ;
#145303=CARTESIAN_POINT('Ctrl Pts',(-26.3664177483922,13.6605444903127,
130.366073831618)) ;
#145304=CARTESIAN_POINT('Ctrl Pts',(-26.3634487238989,13.3493859295917,
130.390576421491)) ;
#145305=CARTESIAN_POINT('Ctrl Pts',(-26.3335452830324,13.0444134847032,
130.336290333141)) ;
#145306=CARTESIAN_POINT('Ctrl Pts',(-26.2780557893883,12.7658508385772,
130.207343051435)) ;
#145307=CARTESIAN_POINT('Ctrl Pts',(-26.2003158885766,12.5346698137633,
130.013361829543)) ;
#145308=CARTESIAN_POINT('Ctrl Pts',(-26.1050182124943,12.3668712653983,
129.768133516794)) ;
#145309=CARTESIAN_POINT('Ctrl Pts',(-25.9983394998777,12.2750736353354,
129.489657461887)) ;
#145310=CARTESIAN_POINT('Ctrl Pts',(-25.8877952399973,12.2654123935104,
129.19972048684)) ;
#145311=CARTESIAN_POINT('Ctrl Pts',(-25.7794715126841,12.3385001490515,
128.916434752625)) ;
#145312=CARTESIAN_POINT('Ctrl Pts',(-25.6810457853793,12.4893941605664,
128.662034056247)) ;
#145313=CARTESIAN_POINT('Ctrl Pts',(-25.5987350438462,12.7071836242874,
128.454714816302)) ;
#145314=CARTESIAN_POINT('Ctrl Pts',(-25.5377622535892,12.976008781698,128.309697798118)) ;
#145315=CARTESIAN_POINT('Ctrl Pts',(-25.5016580962441,13.2771672423765,
128.237367037692)) ;
#145316=CARTESIAN_POINT('Ctrl Pts',(-25.4923643066174,13.5885364783272,
128.24332796172)) ;
#145317=CARTESIAN_POINT('Ctrl Pts',(-25.5097986358348,13.8883475892356,
128.32740133913)) ;
#145318=CARTESIAN_POINT('Ctrl Pts',(-25.5520032926188,14.1546798103871,
128.483821229637)) ;
#145319=CARTESIAN_POINT('Ctrl Pts',(-25.6151380635207,14.3683945721778,
128.701351080741)) ;
#145320=CARTESIAN_POINT('Ctrl Pts',(-25.6940182660661,14.5146640723976,
128.964889919477)) ;
#145321=CARTESIAN_POINT('Ctrl Pts',(-25.7825768658118,14.5827891637854,
129.256811751722)) ;
#145322=CARTESIAN_POINT('Ctrl Pts',(-25.8730390891615,14.5676065821518,
129.554141480536)) ;
#145323=CARTESIAN_POINT('Ctrl Pts',(-25.9587213698666,14.4706130851543,
129.837556439225)) ;
#145324=CARTESIAN_POINT('Ctrl Pts',(-26.03264838451,14.2987448591994,130.086617319719)) ;
#145325=CARTESIAN_POINT('Ctrl Pts',(-26.0889427361501,14.063095759129,130.284302469339)) ;
#145326=CARTESIAN_POINT('Ctrl Pts',(-26.1224378317549,13.7833207941159,
130.415161932836)) ;
#145327=CARTESIAN_POINT('Ctrl Pts',(-26.1303660621799,13.4754882889809,
130.471596562787)) ;
#145328=CARTESIAN_POINT('Ctrl Pts',(-26.111324532664,13.1664272505894,130.448961800146)) ;
#145329=CARTESIAN_POINT('Ctrl Pts',(-26.0659474183763,12.8743475054809,
130.349549021052)) ;
#145330=CARTESIAN_POINT('Ctrl Pts',(-25.9968429052108,12.6220180592587,
130.180760594169)) ;
#145331=CARTESIAN_POINT('Ctrl Pts',(-25.9078683759823,12.4263341461984,
129.954044963807)) ;
#145332=CARTESIAN_POINT('Ctrl Pts',(-25.8050016005084,12.3026056592769,
129.686700785145)) ;
#145333=CARTESIAN_POINT('Ctrl Pts',(-25.6951594284179,12.2593725249827,
129.398886281629)) ;
#145334=CARTESIAN_POINT('Ctrl Pts',(-25.5852338552597,12.2987734012192,
129.110795340355)) ;
#145335=CARTESIAN_POINT('Ctrl Pts',(-25.4812744222043,12.4202091762236,
128.84047911961)) ;
#145336=CARTESIAN_POINT('Ctrl Pts',(-25.3922566652092,12.611773656706,128.613389281527)) ;
#145337=CARTESIAN_POINT('Ctrl Pts',(-25.3219304478952,12.8626551620978,
128.44114506998)) ;
#145338=CARTESIAN_POINT('Ctrl Pts',(-25.2755717009999,13.1527448434828,
128.338777264869)) ;
#145339=CARTESIAN_POINT('Ctrl Pts',(-25.2552923109432,13.4624298007765,
128.312634628559)) ;
#145340=CARTESIAN_POINT('Ctrl Pts',(-25.2620703386305,13.7701811084813,
128.365629030765)) ;
#145341=CARTESIAN_POINT('Ctrl Pts',(-25.2945336713983,14.0517728674994,
128.493510645481)) ;
#145342=CARTESIAN_POINT('Ctrl Pts',(-25.3497468545249,14.2892527094167,
128.687942417164)) ;
#145343=CARTESIAN_POINT('Ctrl Pts',(-25.423284853834,14.4648240462418,128.935995490194)) ;
#145344=CARTESIAN_POINT('Ctrl Pts',(-25.5084071558922,14.5650403206084,
129.217694325303)) ;
#145345=CARTESIAN_POINT('Ctrl Pts',(-25.5990981080236,14.583748953291,129.515806037567)) ;
#145346=CARTESIAN_POINT('Ctrl Pts',(-25.6873241508409,14.5197167656378,
129.806529344841)) ;
#145347=CARTESIAN_POINT('Ctrl Pts',(-25.7671195219414,14.3763314306489,
130.072885261732)) ;
#145348=CARTESIAN_POINT('Ctrl Pts',(-25.8309798067965,14.1656644644825,
130.292474622263)) ;
#145349=CARTESIAN_POINT('Ctrl Pts',(-25.874360274551,13.8999127599495,130.452493401639)) ;
#145350=CARTESIAN_POINT('Ctrl Pts',(-25.8927896275635,13.6028234452547,
130.53927681015)) ;
#145351=CARTESIAN_POINT('Ctrl Pts',(-25.8847621742614,13.291184455058,130.548977456738)) ;
#145352=CARTESIAN_POINT('Ctrl Pts',(-25.8498954972506,12.9894029525186,
130.480221393588)) ;
#145353=CARTESIAN_POINT('Ctrl Pts',(-25.7898002281872,12.717765879006,130.337877304595)) ;
#145354=CARTESIAN_POINT('Ctrl Pts',(-25.708129365045,12.4972589130398,130.132477114614)) ;
#145355=CARTESIAN_POINT('Ctrl Pts',(-25.6107425249076,12.3438957008414,
129.880956988692)) ;
#145356=CARTESIAN_POINT('Ctrl Pts',(-25.5026424369846,12.2668705096983,
129.598352780418)) ;
#145357=CARTESIAN_POINT('Ctrl Pts',(-25.3917428525325,12.2729078297229,
129.30747146326)) ;
#145358=CARTESIAN_POINT('Ctrl Pts',(-25.2847600750955,12.3614501849398,
129.028106287917)) ;
#145359=CARTESIAN_POINT('Ctrl Pts',(-25.1891585260755,12.5253315667214,
128.781860471565)) ;
#145360=CARTESIAN_POINT('Ctrl Pts',(-25.110135939089,12.7552771114224,128.584311890392)) ;
#145361=CARTESIAN_POINT('Ctrl Pts',(-25.0538525122355,13.0310570491295,
128.45290006936)) ;
#145362=CARTESIAN_POINT('Ctrl Pts',(-25.0227014081751,13.3361218325012,
128.395068081625)) ;
#145363=CARTESIAN_POINT('Ctrl Pts',(-25.0185105180042,13.6463105662156,
128.415863743252)) ;
#145364=CARTESIAN_POINT('Ctrl Pts',(-25.040893647384,13.9424874348681,128.514511422021)) ;
#145365=CARTESIAN_POINT('Ctrl Pts',(-25.0875308435713,14.2002009461362,
128.683896967344)) ;
#145366=CARTESIAN_POINT('Ctrl Pts',(-25.1538679221218,14.4015262761072,
128.910674169156)) ;
#145367=CARTESIAN_POINT('Ctrl Pts',(-25.23524054031,14.5339055048123,129.181576243816)) ;
#145368=CARTESIAN_POINT('Ctrl Pts',(-25.3244833479966,14.5863178640293,
129.475378614211)) ;
#145369=CARTESIAN_POINT('Ctrl Pts',(-25.4149673875239,14.55532217226,129.772919559462)) ;
#145370=CARTESIAN_POINT('Ctrl Pts',(-25.4988480768799,14.4431215003341,
130.051053673527)) ;
#145371=CARTESIAN_POINT('Ctrl Pts',(-25.5695954221607,14.2589451908106,
130.290713226978)) ;
#145372=CARTESIAN_POINT('Ctrl Pts',(-25.6220034125225,14.0132050933504,
130.477057575067)) ;
#145373=CARTESIAN_POINT('Ctrl Pts',(-25.6508730043343,13.7264814781089,
130.594456328158)) ;
#145374=CARTESIAN_POINT('Ctrl Pts',(-25.6537138653535,13.4166671262314,
130.635978686215)) ;
#145375=CARTESIAN_POINT('Ctrl Pts',(-25.6296001905431,13.1090562119369,
130.598563069686)) ;
#145376=CARTESIAN_POINT('Ctrl Pts',(-25.5794380606441,12.8228936687179,
130.485173368709)) ;
#145377=CARTESIAN_POINT('Ctrl Pts',(-25.5063529307715,12.5803482500096,
130.304721134994)) ;
#145378=CARTESIAN_POINT('Ctrl Pts',(-25.414190730486,12.3971382780487,130.068720600588)) ;
#145379=CARTESIAN_POINT('Ctrl Pts',(-25.3096218748052,12.2881794710329,
129.796340547925)) ;
#145380=CARTESIAN_POINT('Ctrl Pts',(-25.1987437257025,12.260444774343,129.505635894546)) ;
#145381=CARTESIAN_POINT('Ctrl Pts',(-25.0895511480794,12.3158800590199,
129.219706518543)) ;
#145382=CARTESIAN_POINT('Ctrl Pts',(-24.9881999358306,12.4512316435153,
128.956853185564)) ;
#145383=CARTESIAN_POINT('Ctrl Pts',(-24.9023755881761,12.6546809911043,
128.739090381038)) ;
#145384=CARTESIAN_POINT('Ctrl Pts',(-24.8362095298155,12.9147731891358,
128.579018314088)) ;
#145385=CARTESIAN_POINT('Ctrl Pts',(-24.7946204028052,13.2095560207855,
128.490523563663)) ;
#145386=CARTESIAN_POINT('Ctrl Pts',(-24.7794015918992,13.5223875094378,
128.479378796091)) ;
#145387=CARTESIAN_POINT('Ctrl Pts',(-24.7911074196154,13.8250175828272,
128.54653350614)) ;
#145388=CARTESIAN_POINT('Ctrl Pts',(-24.8284540425988,14.1019896446971,
128.688975600091)) ;
#145389=CARTESIAN_POINT('Ctrl Pts',(-24.8872835848728,14.3273313285593,
128.893786335539)) ;
#145390=CARTESIAN_POINT('Ctrl Pts',(-24.9632695041877,14.4893435909273,
129.148882890249)) ;
#145391=CARTESIAN_POINT('Ctrl Pts',(-25.0500604547885,14.5749600250314,
129.435520331663)) ;
#145392=CARTESIAN_POINT('Ctrl Pts',(-25.1411078657764,14.5779281119493,
129.734734735459)) ;
#145393=CARTESIAN_POINT('Ctrl Pts',(-25.2281667322443,14.4983364866609,
130.022066485608)) ;
#145394=CARTESIAN_POINT('Ctrl Pts',(-25.3052181042423,14.3420895520869,
130.280252049349)) ;
#145395=CARTESIAN_POINT('Ctrl Pts',(-25.3659941264421,14.1180210697834,
130.491128458774)) ;
#145396=CARTESIAN_POINT('Ctrl Pts',(-25.4045283220153,13.8471807636704,
130.636621850606)) ;
#145397=CARTESIAN_POINT('Ctrl Pts',(-25.4182653820351,13.5439412036153,
130.709945042882)) ;
#145398=CARTESIAN_POINT('Ctrl Pts',(-25.4051205680015,13.2331633714353,
130.704601844684)) ;
#145399=CARTESIAN_POINT('Ctrl Pts',(-25.3651505354746,12.9343807646982,
130.621084664061)) ;
#145400=CARTESIAN_POINT('Ctrl Pts',(-25.3008865115351,12.6721977503837,
130.466411854782)) ;
#145401=CARTESIAN_POINT('Ctrl Pts',(-25.2159087492335,12.4632419123552,
130.25129992907)) ;
#145402=CARTESIAN_POINT('Ctrl Pts',(-25.1158600119201,12.3231158449139,
129.992095855596)) ;
#145403=CARTESIAN_POINT('Ctrl Pts',(-25.0063074780256,12.2616017868531,
129.70533965919)) ;
#145404=CARTESIAN_POINT('Ctrl Pts',(-24.8961505989959,12.2833201930426,
129.416474304397)) ;
#145405=CARTESIAN_POINT('Ctrl Pts',(-24.7904450068508,12.3868877539332,
129.14092380243)) ;
#145406=CARTESIAN_POINT('Ctrl Pts',(-24.6974041889648,12.5648231593225,
128.90226664825)) ;
#145407=CARTESIAN_POINT('Ctrl Pts',(-24.6227059932372,12.8039602386114,
128.7171620235)) ;
#145408=CARTESIAN_POINT('Ctrl Pts',(-24.5708840649089,13.0864729218444,
128.598787421566)) ;
#145409=CARTESIAN_POINT('Ctrl Pts',(-24.5446815137269,13.3957238551008,
128.55554617079)) ;
#145410=CARTESIAN_POINT('Ctrl Pts',(-24.545657676478,13.7038340489926,128.591360486886)) ;
#145411=CARTESIAN_POINT('Ctrl Pts',(-24.5726639326172,13.9936201437027,
128.703393987333)) ;
#145412=CARTESIAN_POINT('Ctrl Pts',(-24.623608766435,14.2431366533872,128.885488576488)) ;
#145413=CARTESIAN_POINT('Ctrl Pts',(-24.6929890285264,14.4318623911142,
129.121078946022)) ;
#145414=CARTESIAN_POINT('Ctrl Pts',(-24.7766421491609,14.5502397440411,
129.398740985602)) ;
#145415=CARTESIAN_POINT('Ctrl Pts',(-24.8666514693775,14.5868194748713,
129.694789661665)) ;
#145416=CARTESIAN_POINT('Ctrl Pts',(-24.9561889353879,14.5403267777303,
129.989453760209)) ;
#145417=CARTESIAN_POINT('Ctrl Pts',(-25.0381948159731,14.4138414860088,
130.262123578507)) ;
#145418=CARTESIAN_POINT('Ctrl Pts',(-25.1060482756281,14.2163546818928,
130.493461414613)) ;
#145419=CARTESIAN_POINT('Ctrl Pts',(-25.1541101693659,13.9624647587777,
130.666937384025)) ;
#145420=CARTESIAN_POINT('Ctrl Pts',(-25.1783490492856,13.6693367218364,
130.770898552611)) ;
#145421=CARTESIAN_POINT('Ctrl Pts',(-25.1761396925621,13.3586797958361,
130.797580088685)) ;
#145422=CARTESIAN_POINT('Ctrl Pts',(-25.146968494634,13.0526929008547,130.745494427357)) ;
#145423=CARTESIAN_POINT('Ctrl Pts',(-25.0921634279591,12.7731727546938,
130.618535460199)) ;
#145424=CARTESIAN_POINT('Ctrl Pts',(-25.0149917609423,12.5404161552581,
130.426216312955)) ;
#145425=CARTESIAN_POINT('Ctrl Pts',(-24.9202173073984,12.370760764573,130.182480150042)) ;
#145426=CARTESIAN_POINT('Ctrl Pts',(-24.813795268409,12.2766729448487,129.904750621267)) ;
#145427=CARTESIAN_POINT('Ctrl Pts',(-24.7033211856258,12.2643218542415,
129.615000634789)) ;
#145428=CARTESIAN_POINT('Ctrl Pts',(-24.5940336951667,12.336020687125,129.329153534857)) ;
#145429=CARTESIAN_POINT('Ctrl Pts',(-24.4961741879793,12.4836397645111,
129.076098411666)) ;
#145430=CARTESIAN_POINT('Ctrl Pts',(-24.4129309013941,12.7003320009064,
128.866190595829)) ;
#145431=CARTESIAN_POINT('Ctrl Pts',(-24.3513759196075,12.9678918714247,
128.719449218943)) ;
#145432=CARTESIAN_POINT('Ctrl Pts',(-24.3144899988947,13.2687870375049,
128.644875989553)) ;
#145433=CARTESIAN_POINT('Ctrl Pts',(-24.3044879537029,13.5800036106842,
128.648749851774)) ;
#145434=CARTESIAN_POINT('Ctrl Pts',(-24.3211438511778,13.8799730706512,
128.730495716788)) ;
#145435=CARTESIAN_POINT('Ctrl Pts',(-24.3626924443883,14.1476994881547,
128.885016926294)) ;
#145436=CARTESIAN_POINT('Ctrl Pts',(-24.4253103124442,14.3632525192321,
129.101047744803)) ;
#145437=CARTESIAN_POINT('Ctrl Pts',(-24.5040798325508,14.5119336191473,
129.364360273537)) ;
#145438=CARTESIAN_POINT('Ctrl Pts',(-24.5924052510114,14.5819602234039,
129.655568908214)) ;
#145439=CARTESIAN_POINT('Ctrl Pts',(-24.682620944481,14.5692454166129,129.952075493236)) ;
#145440=CARTESIAN_POINT('Ctrl Pts',(-24.7687439856791,14.4742854326631,
130.236857845916)) ;
#145441=CARTESIAN_POINT('Ctrl Pts',(-24.8428802815619,14.3047438743695,
130.48644479307)) ;
#145442=CARTESIAN_POINT('Ctrl Pts',(-24.8997764198948,14.0710830609088,
130.68585734697)) ;
#145443=CARTESIAN_POINT('Ctrl Pts',(-24.9340655234998,13.7914035953126,
130.819146508686)) ;
#145444=CARTESIAN_POINT('Ctrl Pts',(-24.9427151855598,13.48501227345,130.877578603568)) ;
#145445=CARTESIAN_POINT('Ctrl Pts',(-24.9245196442458,13.1755843630713,
130.85743150607)) ;
#145446=CARTESIAN_POINT('Ctrl Pts',(-24.8798172615573,12.8823157457974,
130.760031273221)) ;
#145447=CARTESIAN_POINT('Ctrl Pts',(-24.8113548753546,12.6284362839445,
130.593124666697)) ;
#145448=CARTESIAN_POINT('Ctrl Pts',(-24.7224609989211,12.4304595143626,
130.366773734036)) ;
#145449=CARTESIAN_POINT('Ctrl Pts',(-24.6207277818397,12.3053999518157,
130.102474981531)) ;
#145450=CARTESIAN_POINT('Ctrl Pts',(-24.510109071113,12.2593484399968,129.812666622082)) ;
#145451=CARTESIAN_POINT('Ctrl Pts',(-24.4006135039195,12.2965483921961,
129.52567159029)) ;
#145452=CARTESIAN_POINT('Ctrl Pts',(-24.2962846439716,12.4156949295869,
129.25430071454)) ;
#145453=CARTESIAN_POINT('Ctrl Pts',(-24.2068868760499,12.6050470782002,
129.026051488153)) ;
#145454=CARTESIAN_POINT('Ctrl Pts',(-24.1357528972809,12.85534209768,128.851555978763)) ;
#145455=CARTESIAN_POINT('Ctrl Pts',(-24.0888790413308,13.1429454569684,
128.747499203338)) ;
#145456=CARTESIAN_POINT('Ctrl Pts',(-24.0676646556075,13.4543917047447,
128.718846507491)) ;
#145457=CARTESIAN_POINT('Ctrl Pts',(-24.0737278362457,13.7614620059086,
128.769634834732)) ;
#145458=CARTESIAN_POINT('Ctrl Pts',(-24.1055487068068,14.0447128346805,
128.895717594865)) ;
#145459=CARTESIAN_POINT('Ctrl Pts',(-24.1600664153194,14.2828873109444,
129.088022746766)) ;
#145460=CARTESIAN_POINT('Ctrl Pts',(-24.2328338887739,14.4603132478387,
129.333714872122)) ;
#145461=CARTESIAN_POINT('Ctrl Pts',(-24.3183681463858,14.5634617520393,
129.61687678413)) ;
#145462=CARTESIAN_POINT('Ctrl Pts',(-24.4083151971696,14.5844329879889,
129.912552844779)) ;
#145463=CARTESIAN_POINT('Ctrl Pts',(-24.4973052919974,14.5225343310152,
130.205738265823)) ;
#145464=CARTESIAN_POINT('Ctrl Pts',(-24.5771666052191,14.381544806336,130.472171976175)) ;
#145465=CARTESIAN_POINT('Ctrl Pts',(-24.6416003829867,14.1725754677665,
130.693462309482)) ;
#145466=CARTESIAN_POINT('Ctrl Pts',(-24.6855081480157,13.9093040451571,
130.854881000139)) ;
#145467=CARTESIAN_POINT('Ctrl Pts',(-24.7048840428278,13.6121558294026,
130.944527353415)) ;
#145468=CARTESIAN_POINT('Ctrl Pts',(-24.6975117007538,13.2990170967779,
130.956305109112)) ;
#145469=CARTESIAN_POINT('Ctrl Pts',(-24.6634915622585,12.9981565078101,
130.889864249442)) ;
#145470=CARTESIAN_POINT('Ctrl Pts',(-24.6042823318373,12.7257032392755,
130.75004731912)) ;
#145471=CARTESIAN_POINT('Ctrl Pts',(-24.5231278871429,12.50307580565,130.546193334941)) ;
#145472=CARTESIAN_POINT('Ctrl Pts',(-24.4259349379458,12.3471529691752,
130.295310104727)) ;
#145473=CARTESIAN_POINT('Ctrl Pts',(-24.317624894329,12.2678408556735,130.012210217516)) ;
#145474=CARTESIAN_POINT('Ctrl Pts',(-24.2073570412543,12.2715869300384,
129.722982490408)) ;
#145475=CARTESIAN_POINT('Ctrl Pts',(-24.1000179362842,12.3575776259723,
129.442610247021)) ;
#145476=CARTESIAN_POINT('Ctrl Pts',(-24.0038553412902,12.5198592417277,
129.194788827538)) ;
#145477=CARTESIAN_POINT('Ctrl Pts',(-23.9244819040808,12.7472701152985,
128.996100991408)) ;
#145478=CARTESIAN_POINT('Ctrl Pts',(-23.8672284776034,13.0233715005783,
128.862029320355)) ;
#145479=CARTESIAN_POINT('Ctrl Pts',(-23.8355017571013,13.3264775703159,
128.80235176831)) ;
#145480=CARTESIAN_POINT('Ctrl Pts',(-23.8304504639882,13.6374829528976,
128.82070893424)) ;
#145481=CARTESIAN_POINT('Ctrl Pts',(-23.8520959271135,13.9340523066843,
128.917163045102)) ;
#145482=CARTESIAN_POINT('Ctrl Pts',(-23.8979574875289,14.1931239778517,
129.084255884832)) ;
#145483=CARTESIAN_POINT('Ctrl Pts',(-23.9642805338681,14.3974304902421,
129.311214290723)) ;
#145484=CARTESIAN_POINT('Ctrl Pts',(-24.0448517026705,14.5309245532204,
129.579566049685)) ;
#145485=CARTESIAN_POINT('Ctrl Pts',(-24.1340072017482,14.5859814539265,
129.873140621991)) ;
#145486=CARTESIAN_POINT('Ctrl Pts',(-24.2243794169451,14.5574777806989,
130.17028755097)) ;
#145487=CARTESIAN_POINT('Ctrl Pts',(-24.3086066368753,14.4480150523887,
130.449430915378)) ;
#145488=CARTESIAN_POINT('Ctrl Pts',(-24.3802849882229,14.2640746902433,
130.692069315547)) ;
#145489=CARTESIAN_POINT('Ctrl Pts',(-24.4328192725426,14.0222278683344,
130.878454916982)) ;
#145490=CARTESIAN_POINT('Ctrl Pts',(-24.4627050818997,13.7339092296597,
130.99913076425)) ;
#145491=CARTESIAN_POINT('Ctrl Pts',(-24.4662080301879,13.4264443376891,
131.042356332604)) ;
#145492=CARTESIAN_POINT('Ctrl Pts',(-24.4429209579648,13.1179337351116,
131.007422112503)) ;
#145493=CARTESIAN_POINT('Ctrl Pts',(-24.3935199440539,12.8308236558004,
130.896241586922)) ;
#145494=CARTESIAN_POINT('Ctrl Pts',(-24.3206916784442,12.5859821192932,
130.716676995717)) ;
#145495=CARTESIAN_POINT('Ctrl Pts',(-24.2296516192907,12.4020104607834,
130.483717120117)) ;
#145496=CARTESIAN_POINT('Ctrl Pts',(-24.1247045576579,12.2899875616105,
130.21045036919)) ;
#145497=CARTESIAN_POINT('Ctrl Pts',(-24.0144718993948,12.260124778228,129.921452283938)) ;
#145498=CARTESIAN_POINT('Ctrl Pts',(-23.9049499602136,12.3130229090721,
129.634621082704)) ;
#145499=CARTESIAN_POINT('Ctrl Pts',(-23.8034612745574,12.445755568189,129.371289868144)) ;
#145500=CARTESIAN_POINT('Ctrl Pts',(-23.716785016583,12.6478749143986,129.151150857304)) ;
#145501=CARTESIAN_POINT('Ctrl Pts',(-23.6498368401481,12.9074235529971,
128.988879427975)) ;
#145502=CARTESIAN_POINT('Ctrl Pts',(-23.6076171016782,13.201587990353,128.898548838853)) ;
#145503=CARTESIAN_POINT('Ctrl Pts',(-23.5916652550101,13.5132462797945,
128.885148066507)) ;
#145504=CARTESIAN_POINT('Ctrl Pts',(-23.6026899469641,13.8170405083281,
128.950393841574)) ;
#145505=CARTESIAN_POINT('Ctrl Pts',(-23.6390022908284,14.0930904717493,
129.089554598804)) ;
#145506=CARTESIAN_POINT('Ctrl Pts',(-23.6974288966858,14.3215765569393,
129.293356920021)) ;
#145507=CARTESIAN_POINT('Ctrl Pts',(-23.7732783266701,14.4860164684736,
129.548154125562)) ;
#145508=CARTESIAN_POINT('Ctrl Pts',(-23.8599542560027,14.5737422146348,
129.834485864806)) ;
#145509=CARTESIAN_POINT('Ctrl Pts',(-23.9507422758738,14.5789283273619,
130.13285405137)) ;
#145510=CARTESIAN_POINT('Ctrl Pts',(-24.0380468092121,14.5018179973275,
130.420910654275)) ;
#145511=CARTESIAN_POINT('Ctrl Pts',(-24.1157083841933,14.3465570817491,
130.68101922773)) ;
#145512=CARTESIAN_POINT('Ctrl Pts',(-24.176387817006,14.1268974135735,130.891224248633)) ;
#145513=CARTESIAN_POINT('Ctrl Pts',(-24.2160535934832,13.8551171351805,
131.04031438907)) ;
#145514=CARTESIAN_POINT('Ctrl Pts',(-24.2304468988952,13.5530512913373,
131.115473299743)) ;
#145515=CARTESIAN_POINT('Ctrl Pts',(-24.2180467938604,13.2415863722887,
131.112379553594)) ;
#145516=CARTESIAN_POINT('Ctrl Pts',(-24.1789708219546,12.9431696446184,
131.031350828024)) ;
#145517=CARTESIAN_POINT('Ctrl Pts',(-24.1152480411839,12.6789855652346,
130.878343326519)) ;
#145518=CARTESIAN_POINT('Ctrl Pts',(-24.0308870684906,12.4685393411929,
130.664990318022)) ;
#145519=CARTESIAN_POINT('Ctrl Pts',(-23.9312079738808,12.3261974567536,
130.406868087954)) ;
#145520=CARTESIAN_POINT('Ctrl Pts',(-23.8218914930888,12.2622045863294,
130.12077781006)) ;
#145521=CARTESIAN_POINT('Ctrl Pts',(-23.711473023475,12.2815898353466,129.831214120587)) ;
#145522=CARTESIAN_POINT('Ctrl Pts',(-23.605830521001,12.3824517800912,129.55574064071)) ;
#145523=CARTESIAN_POINT('Ctrl Pts',(-23.5121833804525,12.5585397023802,
129.31536727562)) ;
#145524=CARTESIAN_POINT('Ctrl Pts',(-23.4369153209714,12.7954955062998,
129.128535047897)) ;
#145525=CARTESIAN_POINT('Ctrl Pts',(-23.3840187660153,13.0796940190917,
129.007326938172)) ;
#145526=CARTESIAN_POINT('Ctrl Pts',(-23.3573639658812,13.3852304458179,
128.962397177592)) ;
#145527=CARTESIAN_POINT('Ctrl Pts',(-23.3574546179297,13.69604445911,128.995889251632)) ;
#145528=CARTESIAN_POINT('Ctrl Pts',(-23.3838342563352,13.985866733445,129.106013284641)) ;
#145529=CARTESIAN_POINT('Ctrl Pts',(-23.4338358205724,14.2358877356182,
129.285204766825)) ;
#145530=CARTESIAN_POINT('Ctrl Pts',(-23.5030215875279,14.4275999337175,
129.520381613063)) ;
#145531=CARTESIAN_POINT('Ctrl Pts',(-23.586530885337,14.5480862858471,129.79766767603)) ;
#145532=CARTESIAN_POINT('Ctrl Pts',(-23.6761347345792,14.5868446718797,
130.092418722233)) ;
#145533=CARTESIAN_POINT('Ctrl Pts',(-23.7656887691914,14.5430357670067,
130.387091618743)) ;
#145534=CARTESIAN_POINT('Ctrl Pts',(-23.8481253493012,14.41874401797,130.66105949148)) ;
#145535=CARTESIAN_POINT('Ctrl Pts',(-23.9165563901983,14.2230681528207,
130.894108221658)) ;
#145536=CARTESIAN_POINT('Ctrl Pts',(-23.9653333847544,13.9697197453762,
131.069771337352)) ;
#145537=CARTESIAN_POINT('Ctrl Pts',(-23.990200337815,13.6787523324498,131.175414444762)) ;
#145538=CARTESIAN_POINT('Ctrl Pts',(-23.9887937953144,13.3668522755562,
131.204597590958)) ;
#145539=CARTESIAN_POINT('Ctrl Pts',(-23.9602778328738,13.060672465625,131.154404872108)) ;
#145540=CARTESIAN_POINT('Ctrl Pts',(-23.9063786521122,12.7810810976344,
131.029975165967)) ;
#145541=CARTESIAN_POINT('Ctrl Pts',(-23.8298459002734,12.5467077229853,
130.839515925952)) ;
#145542=CARTESIAN_POINT('Ctrl Pts',(-23.7357096542374,12.375036029875,130.597588581862)) ;
#145543=CARTESIAN_POINT('Ctrl Pts',(-23.6289012337717,12.2779852364334,
130.318926820808)) ;
#145544=CARTESIAN_POINT('Ctrl Pts',(-23.5186091664602,12.263745955446,130.029664056281)) ;
#145545=CARTESIAN_POINT('Ctrl Pts',(-23.409859192313,12.3321871906188,129.745159691814)) ;
#145546=CARTESIAN_POINT('Ctrl Pts',(-23.3107503409185,12.4786900321498,
129.488734825247)) ;
#145547=CARTESIAN_POINT('Ctrl Pts',(-23.2270427134099,12.6941599570478,
129.277486374064)) ;
#145548=CARTESIAN_POINT('Ctrl Pts',(-23.1650738676188,12.9594898311094,
129.129411454435)) ;
#145549=CARTESIAN_POINT('Ctrl Pts',(-23.127402651992,13.2597802878034,129.052552004075)) ;
#145550=CARTESIAN_POINT('Ctrl Pts',(-23.1166171147694,13.5705933911082,
129.054095550851)) ;
#145551=CARTESIAN_POINT('Ctrl Pts',(-23.1324759418215,13.8717555022921,
129.133564743532)) ;
#145552=CARTESIAN_POINT('Ctrl Pts',(-23.1736382839865,14.1416796956212,
129.287104278442)) ;
#145553=CARTESIAN_POINT('Ctrl Pts',(-23.2353487963013,14.3575208853318,
129.500272865785)) ;
#145554=CARTESIAN_POINT('Ctrl Pts',(-23.3139533929537,14.5088742851846,
129.763207569102)) ;
#145555=CARTESIAN_POINT('Ctrl Pts',(-23.4019083074391,14.5810485932283,
130.05325347066)) ;
#145556=CARTESIAN_POINT('Ctrl Pts',(-23.4922878921798,14.5707018107426,
130.350295811704)) ;
#145557=CARTESIAN_POINT('Ctrl Pts',(-23.5783948195674,14.4785662345022,
130.634919109524)) ;
#145558=CARTESIAN_POINT('Ctrl Pts',(-23.6535576314426,14.3096045878152,
130.887780129686)) ;
#145559=CARTESIAN_POINT('Ctrl Pts',(-23.7107444191254,14.0777449679159,
131.087951985329)) ;
#145560=CARTESIAN_POINT('Ctrl Pts',(-23.7455948140687,13.8001341455209,
131.222767295429)) ;
#145561=CARTESIAN_POINT('Ctrl Pts',(-23.7550892236747,13.4946152703642,
131.283624171076)) ;
#145562=CARTESIAN_POINT('Ctrl Pts',(-23.7375695842205,13.1837406589244,
131.265591449185)) ;
#145563=CARTESIAN_POINT('Ctrl Pts',(-23.6936762044173,12.8901082273082,
131.170493042617)) ;
#145564=CARTESIAN_POINT('Ctrl Pts',(-23.625357982327,12.6339160706406,131.004184247701)) ;
#145565=CARTESIAN_POINT('Ctrl Pts',(-23.5382570077213,12.4365925645623,
130.782597137202)) ;
#145566=CARTESIAN_POINT('Ctrl Pts',(-23.4356867081835,12.3075969590058,
130.516253879618)) ;
#145567=CARTESIAN_POINT('Ctrl Pts',(-23.3261678971312,12.2595413699531,
130.229346863333)) ;
#145568=CARTESIAN_POINT('Ctrl Pts',(-23.2155616867436,12.2945981250866,
129.939427931191)) ;
#145569=CARTESIAN_POINT('Ctrl Pts',(-23.112025204016,12.4101972577176,129.670008473014)) ;
#145570=CARTESIAN_POINT('Ctrl Pts',(-23.0214087797488,12.598715944425,129.438457570237)) ;
#145571=CARTESIAN_POINT('Ctrl Pts',(-22.9499549148632,12.8461743706132,
129.262846208528)) ;
#145572=CARTESIAN_POINT('Ctrl Pts',(-22.9018759435203,13.1359262374288,
129.155624903807)) ;
#145573=CARTESIAN_POINT('Ctrl Pts',(-22.8801611636247,13.4447581529336,
129.125245563724)) ;
#145574=CARTESIAN_POINT('Ctrl Pts',(-22.8854063684676,13.7530929209566,
129.17374638537)) ;
#145575=CARTESIAN_POINT('Ctrl Pts',(-22.916384591562,14.0362080508941,129.297229526547)) ;
#145576=CARTESIAN_POINT('Ctrl Pts',(-22.9704084490522,14.2769560090218,
129.488206755545)) ;
#145577=CARTESIAN_POINT('Ctrl Pts',(-23.0429220897085,14.4563581984587,
129.733214662571)) ;
#145578=CARTESIAN_POINT('Ctrl Pts',(-23.1276158497506,14.5613193565883,
130.013704430188)) ;
#145579=CARTESIAN_POINT('Ctrl Pts',(-23.2181078723221,14.5851466740993,
130.311194154607)) ;
#145580=CARTESIAN_POINT('Ctrl Pts',(-23.3072958781627,14.5250094201889,
130.604988309245)) ;
#145581=CARTESIAN_POINT('Ctrl Pts',(-23.3870877454623,14.3871118872338,
130.87103110078)) ;
#145582=CARTESIAN_POINT('Ctrl Pts',(-23.4523914097116,14.1786613146333,
131.095060551793)) ;
#145583=CARTESIAN_POINT('Ctrl Pts',(-23.4967311352243,13.9181921404444,
131.25754465457)) ;
#145584=CARTESIAN_POINT('Ctrl Pts',(-23.5169519482374,13.6189922621126,
131.349968979705)) ;
#145585=CARTESIAN_POINT('Ctrl Pts',(-23.5103363565515,13.3089360963624,
131.363628705452)) ;
#145586=CARTESIAN_POINT('Ctrl Pts',(-23.4770069966206,13.0058324971489,
131.29938668452)) ;
#145587=CARTESIAN_POINT('Ctrl Pts',(-23.4182183181683,12.7318651916952,
131.160863065766)) ;
#145588=CARTESIAN_POINT('Ctrl Pts',(-23.3377159966076,12.5082426234418,
130.958847305866)) ;
#145589=CARTESIAN_POINT('Ctrl Pts',(-23.2412362943228,12.3508732167538,
130.709935987911)) ;
#145590=CARTESIAN_POINT('Ctrl Pts',(-23.1334938059766,12.2691036353101,
130.428391186563)) ;
#145591=CARTESIAN_POINT('Ctrl Pts',(-23.0226736892661,12.2702137418504,
130.137711873116)) ;
#145592=CARTESIAN_POINT('Ctrl Pts',(-22.9149840860042,12.3542930287051,
129.856364718422)) ;
#145593=CARTESIAN_POINT('Ctrl Pts',(-22.8187097041837,12.5141177100409,
129.608122057843)) ;
#145594=CARTESIAN_POINT('Ctrl Pts',(-22.7388237334191,12.7395234896818,
129.407902601402)) ;
#145595=CARTESIAN_POINT('Ctrl Pts',(-22.6808402251335,13.0142280160873,
129.271679110281)) ;
#145596=CARTESIAN_POINT('Ctrl Pts',(-22.6482265628477,13.3177663479764,
129.209516170382)) ;
#145597=CARTESIAN_POINT('Ctrl Pts',(-22.6424590310294,13.6286638171374,
129.22575901871)) ;
#145598=CARTESIAN_POINT('Ctrl Pts',(-22.6632532943469,13.925291931835,129.319642589528)) ;
#145599=CARTESIAN_POINT('Ctrl Pts',(-22.7085000580716,14.1860950196788,
129.484987285644)) ;
#145600=CARTESIAN_POINT('Ctrl Pts',(-22.7740352615984,14.3917324528471,
129.709531790955)) ;
#145601=CARTESIAN_POINT('Ctrl Pts',(-22.8545854265937,14.5282787585867,
129.977970770821)) ;
#145602=CARTESIAN_POINT('Ctrl Pts',(-22.9437848131845,14.585553871015,130.271733891018)) ;
#145603=CARTESIAN_POINT('Ctrl Pts',(-23.0339617592761,14.5594424124574,
130.568216361715)) ;
#145604=CARTESIAN_POINT('Ctrl Pts',(-23.1183884658679,14.452533822029,130.847908451577)) ;
#145605=CARTESIAN_POINT('Ctrl Pts',(-23.1906734144242,14.2704301815678,
131.092366276915)) ;
#145606=CARTESIAN_POINT('Ctrl Pts',(-23.2438547431658,14.0294404722423,
131.280712615189)) ;
#145607=CARTESIAN_POINT('Ctrl Pts',(-23.2743339500446,13.7439522492757,
131.402912133382)) ;
#145608=CARTESIAN_POINT('Ctrl Pts',(-23.2787167666675,13.4354033023599,
131.448870145367)) ;
#145609=CARTESIAN_POINT('Ctrl Pts',(-23.2562246361759,13.1268757917154,
131.416219286457)) ;
#145610=CARTESIAN_POINT('Ctrl Pts',(-23.2073574714543,12.8380942366352,
131.306698786949)) ;
#145611=CARTESIAN_POINT('Ctrl Pts',(-23.1355944667206,12.5930207366324,
131.130053443896)) ;
#145612=CARTESIAN_POINT('Ctrl Pts',(-23.0444638356501,12.406038861412,130.897036568901)) ;
#145613=CARTESIAN_POINT('Ctrl Pts',(-22.9406787300405,12.292531234905,130.626882995043)) ;
#145614=CARTESIAN_POINT('Ctrl Pts',(-22.8296117127798,12.259700175239,130.335730540699)) ;
#145615=CARTESIAN_POINT('Ctrl Pts',(-22.7202029855353,12.3104428593725,
130.049154559549)) ;
#145616=CARTESIAN_POINT('Ctrl Pts',(-22.6182810864586,12.4411375655696,
129.784596789139)) ;
#145617=CARTESIAN_POINT('Ctrl Pts',(-22.5313208064023,12.6410412802729,
129.563551254626)) ;
#145618=CARTESIAN_POINT('Ctrl Pts',(-22.4636797384928,12.8990710258353,
129.399250646078)) ;
#145619=CARTESIAN_POINT('Ctrl Pts',(-22.4206465720963,13.1932159520557,
129.306625587208)) ;
#145620=CARTESIAN_POINT('Ctrl Pts',(-22.4039742026336,13.5039484440362,
129.291035546014)) ;
#145621=CARTESIAN_POINT('Ctrl Pts',(-22.4142047859484,13.8084630693567,
129.353985219695)) ;
#145622=CARTESIAN_POINT('Ctrl Pts',(-22.4498225285243,14.0856215831729,
129.491114851947)) ;
#145623=CARTESIAN_POINT('Ctrl Pts',(-22.507670146175,14.3156974837171,129.693224338099)) ;
#145624=CARTESIAN_POINT('Ctrl Pts',(-22.5829454215261,14.482069329469,129.946284653554)) ;
#145625=CARTESIAN_POINT('Ctrl Pts',(-22.6695641165245,14.5722583544091,
130.232518171332)) ;
#145626=CARTESIAN_POINT('Ctrl Pts',(-22.7598804555675,14.5801736799871,
130.529336653199)) ;
#145627=CARTESIAN_POINT('Ctrl Pts',(-22.8480258383558,14.5050113517495,
130.820095830851)) ;
#145628=CARTESIAN_POINT('Ctrl Pts',(-22.9257917436902,14.3522164750112,
131.080392384164)) ;
#145629=CARTESIAN_POINT('Ctrl Pts',(-22.987136965067,14.1339602612738,131.292602674308)) ;
#145630=CARTESIAN_POINT('Ctrl Pts',(-23.0274074755232,13.8641112712326,
131.443370465904)) ;
#145631=CARTESIAN_POINT('Ctrl Pts',(-23.0426371790203,13.5616225014003,
131.521090320168)) ;
#145632=CARTESIAN_POINT('Ctrl Pts',(-23.0309825577039,13.2502934236062,
131.520151201035)) ;
#145633=CARTESIAN_POINT('Ctrl Pts',(-22.9925814825968,12.9509782560257,
131.441125269672)) ;
#145634=CARTESIAN_POINT('Ctrl Pts',(-22.9297334436235,12.6863948819192,
131.290563314743)) ;
#145635=CARTESIAN_POINT('Ctrl Pts',(-22.8457402853658,12.4734606146631,
131.078368259428)) ;
#145636=CARTESIAN_POINT('Ctrl Pts',(-22.7459623009365,12.3287823734524,
130.820088867329)) ;
#145637=CARTESIAN_POINT('Ctrl Pts',(-22.6373365168631,12.262963408062,130.535850196423)) ;
#145638=CARTESIAN_POINT('Ctrl Pts',(-22.5266895904036,12.2798963364109,
130.245676252651)) ;
#145639=CARTESIAN_POINT('Ctrl Pts',(-22.4207454828677,12.3786944152069,
129.96934005118)) ;
#145640=CARTESIAN_POINT('Ctrl Pts',(-22.3265704318192,12.5532637477409,
129.727473762186)) ;
#145641=CARTESIAN_POINT('Ctrl Pts',(-22.2510778917587,12.7879392173085,
129.539860818582)) ;
#145642=CARTESIAN_POINT('Ctrl Pts',(-22.1975992748365,13.0695371613245,
129.416790381634)) ;
#145643=CARTESIAN_POINT('Ctrl Pts',(-22.1699284873186,13.3764287313842,
129.369087812723)) ;
#145644=CARTESIAN_POINT('Ctrl Pts',(-22.1693136310075,13.6873693944069,
129.400507755856)) ;
#145645=CARTESIAN_POINT('Ctrl Pts',(-22.1949149197245,13.9780097537181,
129.508346847974)) ;
#145646=CARTESIAN_POINT('Ctrl Pts',(-22.2445624596995,14.2303816916052,
129.686644518596)) ;
#145647=CARTESIAN_POINT('Ctrl Pts',(-22.3130761042801,14.4229832275646,
129.919733582549)) ;
#145648=CARTESIAN_POINT('Ctrl Pts',(-22.3960662366792,14.545607197334,130.195429870093)) ;
#145649=CARTESIAN_POINT('Ctrl Pts',(-22.4857299738979,14.5869244372964,
130.490415745043)) ;
#145650=CARTESIAN_POINT('Ctrl Pts',(-22.575453626079,14.545413999477,130.785606108546)) ;
#145651=CARTESIAN_POINT('Ctrl Pts',(-22.6582120497049,14.4231615318539,
131.060527548057)) ;
#145652=CARTESIAN_POINT('Ctrl Pts',(-22.7269164368304,14.2299646003197,
131.294274065008)) ;
#145653=CARTESIAN_POINT('Ctrl Pts',(-22.7764175593052,13.9782380349311,
131.47205027609)) ;
#145654=CARTESIAN_POINT('Ctrl Pts',(-22.8020622548463,13.6869896701315,
131.58008886622)) ;
#145655=CARTESIAN_POINT('Ctrl Pts',(-22.8014560080435,13.3772462280803,
131.611403153323)) ;
#145656=CARTESIAN_POINT('Ctrl Pts',(-22.7738460874784,13.0701026348063,
131.563905722585)) ;
#145657=CARTESIAN_POINT('Ctrl Pts',(-22.7204413399783,12.7883757721948,
131.441047603048)) ;
#145658=CARTESIAN_POINT('Ctrl Pts',(-22.6444900848234,12.5524788061311,
131.252281571094)) ;
#145659=CARTESIAN_POINT('Ctrl Pts',(-22.5505848182462,12.3787205922408,
131.011087248236)) ;
#145660=CARTESIAN_POINT('Ctrl Pts',(-22.4446658828603,12.2799428361804,
130.734823347179)) ;
#145661=CARTESIAN_POINT('Ctrl Pts',(-22.3341711628268,12.26278144672,130.445043220403)) ;
#145662=CARTESIAN_POINT('Ctrl Pts',(-22.2246631880983,12.3295044441556,
130.158507007516)) ;
#145663=CARTESIAN_POINT('Ctrl Pts',(-22.1257254050998,12.4735104762095,
129.902424684196)) ;
#145664=CARTESIAN_POINT('Ctrl Pts',(-22.0417569838295,12.6859036202202,
129.690264837747)) ;
#145665=CARTESIAN_POINT('Ctrl Pts',(-21.9787385701834,12.9511128750471,
129.539283902845)) ;
#145666=CARTESIAN_POINT('Ctrl Pts',(-21.9403107768235,13.2510042881428,
129.460237929327)) ;
#145667=CARTESIAN_POINT('Ctrl Pts',(-21.9287596101754,13.5624349033162,
129.459612610358)) ;
#145668=CARTESIAN_POINT('Ctrl Pts',(-21.9439314898076,13.8634351893562,
129.537002871099)) ;
#145669=CARTESIAN_POINT('Ctrl Pts',(-21.9840596405432,14.1332614315187,
129.687330392558)) ;
#145670=CARTESIAN_POINT('Ctrl Pts',(-22.0456493591576,14.3526410215066,
129.900400764091)) ;
#145671=CARTESIAN_POINT('Ctrl Pts',(-22.1237356790095,14.5054039917793,
130.161735495758)) ;
#145672=CARTESIAN_POINT('Ctrl Pts',(-22.2111275537692,14.5799567731311,
130.450008897407)) ;
#145673=CARTESIAN_POINT('Ctrl Pts',(-22.3018824052644,14.572371407252,130.74826980151)) ;
#145674=CARTESIAN_POINT('Ctrl Pts',(-22.3885019784228,14.4818104179813,
131.034516812178)) ;
#145675=CARTESIAN_POINT('Ctrl Pts',(-22.4634673589328,14.3163442533983,
131.286522423217)) ;
#145676=CARTESIAN_POINT('Ctrl Pts',(-22.5214998076607,14.0859120132609,
131.489249238818)) ;
#145677=CARTESIAN_POINT('Ctrl Pts',(-22.5571587027642,13.8088757639041,
131.62648715997)) ;
#145678=CARTESIAN_POINT('Ctrl Pts',(-22.5673836208744,13.5028415696086,
131.68958577917)) ;
#145679=CARTESIAN_POINT('Ctrl Pts',(-22.5507152273552,13.1931030740132,
131.673896265537)) ;
#145680=CARTESIAN_POINT('Ctrl Pts',(-22.5074512192622,12.8979592088334,
131.58072405734)) ;
#145681=CARTESIAN_POINT('Ctrl Pts',(-22.4401878872421,12.6415806575113,
131.417320263901)) ;
#145682=CARTESIAN_POINT('Ctrl Pts',(-22.3529978608748,12.4408172036161,
131.195714780762)) ;
#145683=CARTESIAN_POINT('Ctrl Pts',(-22.2507185667645,12.3100401552364,
130.930208877523)) ;
#145684=CARTESIAN_POINT('Ctrl Pts',(-22.1415541397393,12.2598615756175,
130.644270647017)) ;
#145685=CARTESIAN_POINT('Ctrl Pts',(-22.0311013361464,12.2922205464447,
130.354723425766)) ;
#145686=CARTESIAN_POINT('Ctrl Pts',(-21.9267303945298,12.40624849515,130.083044294425)) ;
#145687=CARTESIAN_POINT('Ctrl Pts',(-21.8359058461118,12.5927140641391,
129.850810997993)) ;
#145688=CARTESIAN_POINT('Ctrl Pts',(-21.7640101840432,12.8381488954601,
129.673838643522)) ;
#145689=CARTESIAN_POINT('Ctrl Pts',(-21.7152207007081,13.1260095358548,
129.564442600056)) ;
#145690=CARTESIAN_POINT('Ctrl Pts',(-21.6925855604333,13.4367097241923,
129.531608400982)) ;
#145691=CARTESIAN_POINT('Ctrl Pts',(-21.6970872221281,13.7438376773702,
129.577766848317)) ;
#145692=CARTESIAN_POINT('Ctrl Pts',(-21.7273689275802,14.0287736558089,
129.699306891545)) ;
#145693=CARTESIAN_POINT('Ctrl Pts',(-21.7808528667027,14.2709621799374,
129.888711102644)) ;
#145694=CARTESIAN_POINT('Ctrl Pts',(-21.8527753379124,14.4520608011874,
130.131934341161)) ;
#145695=CARTESIAN_POINT('Ctrl Pts',(-21.937338148521,14.5594794464979,130.412094195668)) ;
#145696=CARTESIAN_POINT('Ctrl Pts',(-22.0275873885439,14.5855261750269,
130.708811093224)) ;
#145697=CARTESIAN_POINT('Ctrl Pts',(-22.1167126461185,14.5283738687936,
131.002328490394)) ;
#145698=CARTESIAN_POINT('Ctrl Pts',(-22.1973624162769,14.3916536122689,
131.271100689726)) ;
#145699=CARTESIAN_POINT('Ctrl Pts',(-22.2627919222655,14.1863632945959,
131.495280692911)) ;
#145700=CARTESIAN_POINT('Ctrl Pts',(-22.3080735207915,13.9255968041967,
131.660732394034)) ;
#145701=CARTESIAN_POINT('Ctrl Pts',(-22.3288933669282,13.6292800303555,
131.754659669598)) ;
#145702=CARTESIAN_POINT('Ctrl Pts',(-22.3231642846892,13.3179689166563,
131.771059850504)) ;
#145703=CARTESIAN_POINT('Ctrl Pts',(-22.2905466843428,13.0144328238462,
131.70888463353)) ;
#145704=CARTESIAN_POINT('Ctrl Pts',(-22.232699413988,12.7401667038842,131.573002097289)) ;
#145705=CARTESIAN_POINT('Ctrl Pts',(-22.1528576217879,12.5144106692782,
131.37292430167)) ;
#145706=CARTESIAN_POINT('Ctrl Pts',(-22.0561564026532,12.3540784251448,
131.123573481352)) ;
#145707=CARTESIAN_POINT('Ctrl Pts',(-21.9491234057288,12.2704506674806,
130.843940985009)) ;
#145708=CARTESIAN_POINT('Ctrl Pts',(-21.8379492349739,12.2689821034606,
130.552336500549)) ;
#145709=CARTESIAN_POINT('Ctrl Pts',(-21.7301340097967,12.350850990926,130.270599037869)) ;
#145710=CARTESIAN_POINT('Ctrl Pts',(-21.6334302854589,12.5086055972373,
130.02111108677)) ;
#145711=CARTESIAN_POINT('Ctrl Pts',(-21.5528038582257,12.7330677829212,
129.818816445627)) ;
#145712=CARTESIAN_POINT('Ctrl Pts',(-21.4942939691824,13.0066124889692,
129.68103187895)) ;
#145713=CARTESIAN_POINT('Ctrl Pts',(-21.4610544217535,13.308272601369,129.616896850597)) ;
#145714=CARTESIAN_POINT('Ctrl Pts',(-21.4544299431771,13.6201713325224,
129.630731872719)) ;
#145715=CARTESIAN_POINT('Ctrl Pts',(-21.474644249058,13.9183341039009,129.72301929693)) ;
#145716=CARTESIAN_POINT('Ctrl Pts',(-21.5192529028078,14.1797388278147,
129.886437479066)) ;
#145717=CARTESIAN_POINT('Ctrl Pts',(-21.5840569958028,14.3864987369051,
130.108738684431)) ;
#145718=CARTESIAN_POINT('Ctrl Pts',(-21.6642121862485,14.5252641755352,
130.376013710086)) ;
#145719=CARTESIAN_POINT('Ctrl Pts',(-21.7532842228128,14.5851721038055,
130.669413027174)) ;
#145720=CARTESIAN_POINT('Ctrl Pts',(-21.8440338817864,14.5610669162746,
130.967758566311)) ;
#145721=CARTESIAN_POINT('Ctrl Pts',(-21.9282251617535,14.4566509798001,
131.246584092179)) ;
#145722=CARTESIAN_POINT('Ctrl Pts',(-22.0009339264215,14.2771545198569,
131.492228959747)) ;
#145723=CARTESIAN_POINT('Ctrl Pts',(-22.0549712796414,14.0362065305465,
131.683263448546)) ;
#145724=CARTESIAN_POINT('Ctrl Pts',(-22.0859468214144,13.753398715095,131.806709045245)) ;
#145725=CARTESIAN_POINT('Ctrl Pts',(-22.0912337993049,13.4441283585126,
131.855429678035)) ;
#145726=CARTESIAN_POINT('Ctrl Pts',(-22.0692970894306,13.1346408966579,
131.824482173486)) ;
#145727=CARTESIAN_POINT('Ctrl Pts',(-22.0215845589901,12.8470251737848,
131.718082264569)) ;
#145728=CARTESIAN_POINT('Ctrl Pts',(-21.9498823449809,12.5984937869307,
131.541883011935)) ;
#145729=CARTESIAN_POINT('Ctrl Pts',(-21.859706635381,12.4108688278635,131.311455950053)) ;
#145730=CARTESIAN_POINT('Ctrl Pts',(-21.7559998278931,12.2946081096869,
131.041613650211)) ;
#145731=CARTESIAN_POINT('Ctrl Pts',(-21.6449281923886,12.2594450533974,
130.750468031976)) ;
#145732=CARTESIAN_POINT('Ctrl Pts',(-21.5353149765672,12.30804814686,130.463325529376)) ;
#145733=CARTESIAN_POINT('Ctrl Pts',(-21.433409422968,12.4360760991486,130.198700529688)) ;
#145734=CARTESIAN_POINT('Ctrl Pts',(-21.3457569994458,12.634525822386,129.975706345904)) ;
#145735=CARTESIAN_POINT('Ctrl Pts',(-21.2777014430076,12.8902137015407,
129.810072152823)) ;
#145736=CARTESIAN_POINT('Ctrl Pts',(-21.2338043784698,13.1836915440523,
129.714952668352)) ;
#145737=CARTESIAN_POINT('Ctrl Pts',(-21.2162760126707,13.4943234250401,
129.69686779882)) ;
#145738=CARTESIAN_POINT('Ctrl Pts',(-21.2257767207619,13.8008444914087,
129.757847499092)) ;
#145739=CARTESIAN_POINT('Ctrl Pts',(-21.260918305411,14.0793170573489,129.893644297111)) ;
#145740=CARTESIAN_POINT('Ctrl Pts',(-21.3179351568953,14.3098745304063,
130.093168310721)) ;
#145741=CARTESIAN_POINT('Ctrl Pts',(-21.393135043171,14.4788324739109,130.346151975855)) ;
#145742=CARTESIAN_POINT('Ctrl Pts',(-21.4791104654225,14.5706780118123,
130.630335180623)) ;
#145743=CARTESIAN_POINT('Ctrl Pts',(-21.569587551734,14.5811216563982,130.92769514245)) ;
#145744=CARTESIAN_POINT('Ctrl Pts',(-21.6577489493399,14.5082991498853,
131.218439893283)) ;
#145745=CARTESIAN_POINT('Ctrl Pts',(-21.7358456781333,14.3580057871193,
131.479665882624)) ;
#145746=CARTESIAN_POINT('Ctrl Pts',(-21.798001885849,14.1405256903455,131.694385206399)) ;
#145747=CARTESIAN_POINT('Ctrl Pts',(-21.8387940212521,13.8719961113424,
131.846641739039)) ;
#145748=CARTESIAN_POINT('Ctrl Pts',(-21.8547791588512,13.5716289607196,
131.926408611645)) ;
#145749=CARTESIAN_POINT('Ctrl Pts',(-21.8439115520657,13.2591262832754,
131.927893832288)) ;
#145750=CARTESIAN_POINT('Ctrl Pts',(-21.8063818672718,12.9599151059205,
131.851322214392)) ;
#145751=CARTESIAN_POINT('Ctrl Pts',(-21.7440145809282,12.6930800437845,
131.702283019861)) ;
#145752=CARTESIAN_POINT('Ctrl Pts',(-21.660626104627,12.4788237616548,131.491808094147)) ;
#145753=CARTESIAN_POINT('Ctrl Pts',(-21.5615327330444,12.332247898292,131.235434874409)) ;
#145754=CARTESIAN_POINT('Ctrl Pts',(-21.4529505571654,12.2636849567094,
130.951367917164)) ;
#145755=CARTESIAN_POINT('Ctrl Pts',(-21.3419633703332,12.2782423804387,
130.660286988405)) ;
#145756=CARTESIAN_POINT('Ctrl Pts',(-21.2358893379918,12.3748788763276,
130.383546024411)) ;
#145757=CARTESIAN_POINT('Ctrl Pts',(-21.141622326909,12.5463735135204,130.141264334557)) ;
#145758=CARTESIAN_POINT('Ctrl Pts',(-21.0649842164547,12.7810696956234,
129.950540111674)) ;
#145759=CARTESIAN_POINT('Ctrl Pts',(-21.0110514658407,13.0608633683861,
129.82603487308)) ;
#145760=CARTESIAN_POINT('Ctrl Pts',(-20.9825739767851,13.3671883117348,
129.775968871056)) ;
#145761=CARTESIAN_POINT('Ctrl Pts',(-20.9811465718423,13.6783221132163,
129.805007108354)) ;
#145762=CARTESIAN_POINT('Ctrl Pts',(-21.0060732680338,13.9701100820096,
129.910918322944)) ;
#145763=CARTESIAN_POINT('Ctrl Pts',(-21.0548192698872,14.2230345342298,
130.086443323896)) ;
#145764=CARTESIAN_POINT('Ctrl Pts',(-21.1231998537938,14.4186168912711,
130.319327093341)) ;
#145765=CARTESIAN_POINT('Ctrl Pts',(-21.2055023955591,14.5428705870382,
130.592855887077)) ;
#145766=CARTESIAN_POINT('Ctrl Pts',(-21.2952349104155,14.5869069845901,
130.888119007957)) ;
#145767=CARTESIAN_POINT('Ctrl Pts',(-21.3849839588049,14.5480013185182,
131.183345676982)) ;
#145768=CARTESIAN_POINT('Ctrl Pts',(-21.4685154515025,14.4271740783889,
131.460720849614)) ;
#145769=CARTESIAN_POINT('Ctrl Pts',(-21.5373912518205,14.2362638793065,
131.694850358935)) ;
#145770=CARTESIAN_POINT('Ctrl Pts',(-21.5875113438075,13.9863048350813,
131.874404129707)) ;
#145771=CARTESIAN_POINT('Ctrl Pts',(-21.6138800887913,13.6957298115947,
131.984578993146)) ;
#145772=CARTESIAN_POINT('Ctrl Pts',(-21.614125788485,13.3866515588876,132.018333297806)) ;
#145773=CARTESIAN_POINT('Ctrl Pts',(-21.5870104977058,13.0771469470951,
131.972501741679)) ;
#145774=CARTESIAN_POINT('Ctrl Pts',(-21.5346173255377,12.7963920748989,
131.852368075822)) ;
#145775=CARTESIAN_POINT('Ctrl Pts',(-21.4589507416269,12.5578779077828,
131.664580333898)) ;
#145776=CARTESIAN_POINT('Ctrl Pts',(-21.3658400631902,12.3830735450268,
131.425564438929)) ;
#145777=CARTESIAN_POINT('Ctrl Pts',(-21.2601690090166,12.2815115080033,
131.150038104503)) ;
#145778=CARTESIAN_POINT('Ctrl Pts',(-21.1489223139169,12.262368243914,130.858300208979)) ;
#145779=CARTESIAN_POINT('Ctrl Pts',(-21.0406225843969,12.3259184462842,
130.574873351895)) ;
#145780=CARTESIAN_POINT('Ctrl Pts',(-20.940603983949,12.4680809705656,130.315844332064)) ;
#145781=CARTESIAN_POINT('Ctrl Pts',(-20.8559583287252,12.6795623808911,
130.101791361904)) ;
#145782=CARTESIAN_POINT('Ctrl Pts',(-20.7925168040744,12.9425895546652,
129.949458890712)) ;
#145783=CARTESIAN_POINT('Ctrl Pts',(-20.7532890269665,13.2417283918,129.868075591736)) ;
#145784=CARTESIAN_POINT('Ctrl Pts',(-20.7409116210845,13.5531903661268,
129.865041638529)) ;
#145785=CARTESIAN_POINT('Ctrl Pts',(-20.7553800380265,13.8554129193782,
129.940450687303)) ;
#145786=CARTESIAN_POINT('Ctrl Pts',(-20.7947745520951,14.1261609524352,
130.088592371087)) ;
#145787=CARTESIAN_POINT('Ctrl Pts',(-20.8561230143057,14.3478085326463,
130.30108906054)) ;
#145788=CARTESIAN_POINT('Ctrl Pts',(-20.9330819717435,14.5013887047212,
130.558818467068)) ;
#145789=CARTESIAN_POINT('Ctrl Pts',(-21.0209925763894,14.5792263128841,
130.848889090578)) ;
#145790=CARTESIAN_POINT('Ctrl Pts',(-21.1115720077452,14.5735423168914,
131.146566451509)) ;
#145791=CARTESIAN_POINT('Ctrl Pts',(-21.1981832466757,14.4859391814988,
131.432684871179)) ;
#145792=CARTESIAN_POINT('Ctrl Pts',(-21.2740827223277,14.3210239309704,
131.687674997692)) ;
#145793=CARTESIAN_POINT('Ctrl Pts',(-21.3322242178944,14.0938128758495,
131.890466779621)) ;
#145794=CARTESIAN_POINT('Ctrl Pts',(-21.3687438781438,13.8165579042321,
132.030389390382)) ;
#145795=CARTESIAN_POINT('Ctrl Pts',(-21.3797138200489,13.5127263915299,
132.095468544481)) ;
#145796=CARTESIAN_POINT('Ctrl Pts',(-21.3636004734543,13.2000971209204,
132.081705722308)) ;
#145797=CARTESIAN_POINT('Ctrl Pts',(-21.3214813309677,12.907342662141,131.991518108208)) ;
#145798=CARTESIAN_POINT('Ctrl Pts',(-21.2545834330948,12.6479572241649,
131.829377280071)) ;
#145799=CARTESIAN_POINT('Ctrl Pts',(-21.1681470865365,12.4461100173765,
131.609861160652)) ;
#145800=CARTESIAN_POINT('Ctrl Pts',(-21.0661478275666,12.3127706189861,
131.345206807129)) ;
#145801=CARTESIAN_POINT('Ctrl Pts',(-20.9570001828304,12.2601401087974,
131.059348447915)) ;
#145802=CARTESIAN_POINT('Ctrl Pts',(-20.8464455495092,12.2901733256143,
130.769514283601)) ;
#145803=CARTESIAN_POINT('Ctrl Pts',(-20.7419747378729,12.4015833067204,
130.497476657603)) ;
#145804=CARTESIAN_POINT('Ctrl Pts',(-20.6504205693361,12.5866483791686,
130.263212545272)) ;
#145805=CARTESIAN_POINT('Ctrl Pts',(-20.5779605821059,12.8302723289068,
130.084547548889)) ;
#145806=CARTESIAN_POINT('Ctrl Pts',(-20.5282977949781,13.1192440261277,
129.97282099279)) ;
#145807=CARTESIAN_POINT('Ctrl Pts',(-20.5051826159402,13.4254781915307,
129.938132734578)) ;
#145808=CARTESIAN_POINT('Ctrl Pts',(-20.5087491589204,13.7353596810941,
129.981818058974)) ;
#145809=CARTESIAN_POINT('Ctrl Pts',(-20.538377675736,14.0210482002996,130.10142777843)) ;
#145810=CARTESIAN_POINT('Ctrl Pts',(-20.5913066213589,14.2649914716046,
130.289249347501)) ;
#145811=CARTESIAN_POINT('Ctrl Pts',(-20.66265561167,14.4476747030691,130.53073518382)) ;
#145812=CARTESIAN_POINT('Ctrl Pts',(-20.7469069028372,14.5574100040251,
130.809977995015)) ;
#145813=CARTESIAN_POINT('Ctrl Pts',(-20.8371160932442,14.5860647514156,
131.106584787319)) ;
#145814=CARTESIAN_POINT('Ctrl Pts',(-20.9267472282309,14.5307819261163,
131.401725854825)) ;
#145815=CARTESIAN_POINT('Ctrl Pts',(-21.0072764966253,14.3969445095406,
131.669955377324)) ;
#145816=CARTESIAN_POINT('Ctrl Pts',(-21.0734887878382,14.1927448984532,
131.896554788733)) ;
#145817=CARTESIAN_POINT('Ctrl Pts',(-21.1192566993192,13.93401239778,132.063324626172)) ;
#145818=CARTESIAN_POINT('Ctrl Pts',(-21.1408827040485,13.6381121003486,
132.159652000683)) ;
#145819=CARTESIAN_POINT('Ctrl Pts',(-21.1359298836086,13.3270742285028,
132.178300987423)) ;
#145820=CARTESIAN_POINT('Ctrl Pts',(-21.1040417699142,13.0225106106699,
132.118308686489)) ;
#145821=CARTESIAN_POINT('Ctrl Pts',(-21.046696839129,12.7468019660475,131.983949585715)) ;
#145822=CARTESIAN_POINT('Ctrl Pts',(-20.9678162020651,12.5205887293237,
131.786510382128)) ;
#145823=CARTESIAN_POINT('Ctrl Pts',(-20.8715310603488,12.3578209293796,
131.538392523229)) ;
#145824=CARTESIAN_POINT('Ctrl Pts',(-20.7644175602374,12.2716454717833,
131.258612557137)) ;
#145825=CARTESIAN_POINT('Ctrl Pts',(-20.6533664144399,12.2679543097138,
130.967335036085)) ;
#145826=CARTESIAN_POINT('Ctrl Pts',(-20.5457061292773,12.3469222200597,
130.685931563992)) ;
#145827=CARTESIAN_POINT('Ctrl Pts',(-20.4482108374109,12.503089881748,130.434261150502)) ;
#145828=CARTESIAN_POINT('Ctrl Pts',(-20.3673275506228,12.7250182855012,
130.231090321485)) ;
#145829=CARTESIAN_POINT('Ctrl Pts',(-20.3079802630187,12.9971829063299,
130.090864398519)) ;
#145830=CARTESIAN_POINT('Ctrl Pts',(-20.2738118580622,13.2997829333183,
130.024178485513)) ;
#145831=CARTESIAN_POINT('Ctrl Pts',(-20.2664947685224,13.6108911186927,
130.035899919689)) ;
#145832=CARTESIAN_POINT('Ctrl Pts',(-20.2857578508788,13.9087324272285,
130.125281467885)) ;
#145833=CARTESIAN_POINT('Ctrl Pts',(-20.3297556724829,14.1725576742086,
130.287029545329)) ;
#145834=CARTESIAN_POINT('Ctrl Pts',(-20.3941998282761,14.3815588265502,
130.508353654678)) ;
#145835=CARTESIAN_POINT('Ctrl Pts',(-20.474005477433,14.5223296073452,130.774601426749)) ;
#145836=CARTESIAN_POINT('Ctrl Pts',(-20.5626590610956,14.5844939687617,
131.066682489216)) ;
#145837=CARTESIAN_POINT('Ctrl Pts',(-20.6534515210062,14.5631534202887,
131.365145687928)) ;
#145838=CARTESIAN_POINT('Ctrl Pts',(-20.7382600278816,14.4606750911625,
131.645905123897)) ;
#145839=CARTESIAN_POINT('Ctrl Pts',(-20.8114033440883,14.2826953933965,
131.892850174446)) ;
#145840=CARTESIAN_POINT('Ctrl Pts',(-20.8657920624794,14.0447463333177,
132.084724481994)) ;
#145841=CARTESIAN_POINT('Ctrl Pts',(-20.8976628106915,13.7613771036905,
132.21097302955)) ;
#145842=CARTESIAN_POINT('Ctrl Pts',(-20.9036617211628,13.4542323232824,
132.261581459296)) ;
#145843=CARTESIAN_POINT('Ctrl Pts',(-20.8826279491425,13.143799460901,132.233338652764)) ;
#145844=CARTESIAN_POINT('Ctrl Pts',(-20.8352934217348,12.8538469192422,
132.128218778633)) ;
#145845=CARTESIAN_POINT('Ctrl Pts',(-20.7645944475466,12.6054873495862,
131.954751852928)) ;
#145846=CARTESIAN_POINT('Ctrl Pts',(-20.6749066761871,12.4153273206803,
131.725780854323)) ;
#145847=CARTESIAN_POINT('Ctrl Pts',(-20.5706090003662,12.2964112458501,
131.454476537484)) ;
#145848=CARTESIAN_POINT('Ctrl Pts',(-20.4608420339056,12.2594155900217,
131.166772800409)) ;
#145849=CARTESIAN_POINT('Ctrl Pts',(-20.3506734795636,12.3053349442499,
130.878138641754)) ;
#145850=CARTESIAN_POINT('Ctrl Pts',(-20.2484737854587,12.4312259098382,
130.612644740711)) ;
#145851=CARTESIAN_POINT('Ctrl Pts',(-20.1602130981831,12.6279597260861,
130.387910852536)) ;
#145852=CARTESIAN_POINT('Ctrl Pts',(-20.0915104002888,12.8824933120028,
130.220406199881)) ;
#145853=CARTESIAN_POINT('Ctrl Pts',(-20.0469681651641,13.1745455822002,
130.123334294232)) ;
#145854=CARTESIAN_POINT('Ctrl Pts',(-20.0286034664188,13.485175620818,130.102825718079)) ;
#145855=CARTESIAN_POINT('Ctrl Pts',(-20.0373664825325,13.7921379938219,
130.161654025936)) ;
#145856=CARTESIAN_POINT('Ctrl Pts',(-20.0715995929942,14.0710148384314,
130.294692145833)) ;
#145857=CARTESIAN_POINT('Ctrl Pts',(-20.1284301538696,14.3045452555015,
130.493888748158)) ;
#145858=CARTESIAN_POINT('Ctrl Pts',(-20.2024927177133,14.4740866338348,
130.743236807604)) ;
#145859=CARTESIAN_POINT('Ctrl Pts',(-20.2887543569043,14.5693022561264,
131.028482394559)) ;
#145860=CARTESIAN_POINT('Ctrl Pts',(-20.3791881951362,14.582012624519,131.325700094759)) ;
#145861=CARTESIAN_POINT('Ctrl Pts',(-20.4677451846558,14.5112270801159,
131.617691378033)) ;
#145862=CARTESIAN_POINT('Ctrl Pts',(-20.5458784428509,14.3635590913307,
131.878885598879)) ;
#145863=CARTESIAN_POINT('Ctrl Pts',(-20.6086278771025,14.1479538826623,
132.095344152089)) ;
#145864=CARTESIAN_POINT('Ctrl Pts',(-20.6501541988264,13.8806546187411,
132.249752133656)) ;
#145865=CARTESIAN_POINT('Ctrl Pts',(-20.6669329941746,13.5796272829373,
132.331977408768)) ;
#145866=CARTESIAN_POINT('Ctrl Pts',(-20.6567504793002,13.2675901061276,
132.335413489308)) ;
#145867=CARTESIAN_POINT('Ctrl Pts',(-20.6200953900451,12.9685391977506,
132.261306783387)) ;
#145868=CARTESIAN_POINT('Ctrl Pts',(-20.5583590983708,12.7001826766663,
132.114143420094)) ;
#145869=CARTESIAN_POINT('Ctrl Pts',(-20.4756221157238,12.4843513272629,
131.905532471069)) ;
#145870=CARTESIAN_POINT('Ctrl Pts',(-20.3767435277783,12.3354377542164,
131.649841765062)) ;
#145871=CARTESIAN_POINT('Ctrl Pts',(-20.2686590300988,12.2645466478322,
131.367129971997)) ;
#145872=CARTESIAN_POINT('Ctrl Pts',(-20.1571318808931,12.276740062036,131.074627014157)) ;
#145873=CARTESIAN_POINT('Ctrl Pts',(-20.0512008838517,12.3708039289104,
130.79818158066)) ;
#145874=CARTESIAN_POINT('Ctrl Pts',(-19.9563086255669,12.5405714665883,
130.554144914128)) ;
#145875=CARTESIAN_POINT('Ctrl Pts',(-19.8793088986638,12.7727637010119,
130.362246811073)) ;
#145876=CARTESIAN_POINT('Ctrl Pts',(-19.8242814025798,13.0532482908803,
130.234757689759)) ;
#145877=CARTESIAN_POINT('Ctrl Pts',(-19.7952189624458,13.3594504233503,
130.183004684366)) ;
#145878=CARTESIAN_POINT('Ctrl Pts',(-19.7930134578907,13.6687251009062,
130.209550970589)) ;
#145879=CARTESIAN_POINT('Ctrl Pts',(-19.817213216908,13.9622484425501,130.313436084114)) ;
#145880=CARTESIAN_POINT('Ctrl Pts',(-19.8653052839122,14.2163837439272,
130.487026316147)) ;
#145881=CARTESIAN_POINT('Ctrl Pts',(-19.9333746488485,14.4143549492585,
130.719088100669)) ;
#145882=CARTESIAN_POINT('Ctrl Pts',(-20.0153927997561,14.5404303849103,
130.991781249979)) ;
#145883=CARTESIAN_POINT('Ctrl Pts',(-20.1046291781112,14.5868747911533,
131.285452132637)) ;
#145884=CARTESIAN_POINT('Ctrl Pts',(-20.1949857625837,14.5499212467829,
131.582654306618)) ;
#145885=CARTESIAN_POINT('Ctrl Pts',(-20.2781124905757,14.4324626312606,
131.858552426998)) ;
#145886=CARTESIAN_POINT('Ctrl Pts',(-20.3481188112535,14.2419356966938,
132.096282760798)) ;
#145887=CARTESIAN_POINT('Ctrl Pts',(-20.3985871619512,13.9939564791264,
132.276740859809)) ;
#145888=CARTESIAN_POINT('Ctrl Pts',(-20.425720129423,13.7043181769273,132.389150470966)) ;
#145889=CARTESIAN_POINT('Ctrl Pts',(-20.426667137121,13.395369790062,132.424965585476)) ;
#145890=CARTESIAN_POINT('Ctrl Pts',(-20.4005199781611,13.086808383261,132.381812352242)) ;
#145891=CARTESIAN_POINT('Ctrl Pts',(-20.3486042070597,12.8035341555048,
132.263245810191)) ;
#145892=CARTESIAN_POINT('Ctrl Pts',(-20.2736098470821,12.5639567351557,
132.077367144187)) ;
#145893=CARTESIAN_POINT('Ctrl Pts',(-20.1807645712942,12.3867441251715,
131.839192537053)) ;
#145894=CARTESIAN_POINT('Ctrl Pts',(-20.0751360357646,12.2832559633923,
131.563844017608)) ;
#145895=CARTESIAN_POINT('Ctrl Pts',(-19.964903232874,12.2616345665819,131.274777694618)) ;
#145896=CARTESIAN_POINT('Ctrl Pts',(-19.8555629286285,12.3231638960011,
130.98858229832)) ;
#145897=CARTESIAN_POINT('Ctrl Pts',(-19.7556644206763,12.4627500215576,
130.729750507701)) ;
#145898=CARTESIAN_POINT('Ctrl Pts',(-19.6702402237526,12.6729053974916,
130.513517339829)) ;
#145899=CARTESIAN_POINT('Ctrl Pts',(-19.6062148535559,12.9344260822497,
130.35944129945)) ;
#145900=CARTESIAN_POINT('Ctrl Pts',(-19.5661559405149,13.234077565713,130.27576146091)) ;
#145901=CARTESIAN_POINT('Ctrl Pts',(-19.5531448999268,13.5439039553039,
130.270706955932)) ;
#145902=CARTESIAN_POINT('Ctrl Pts',(-19.5667543120863,13.8465582342306,
130.343585324908)) ;
#145903=CARTESIAN_POINT('Ctrl Pts',(-19.6055060890507,14.1188040415087,
130.489887703278)) ;
#145904=CARTESIAN_POINT('Ctrl Pts',(-19.6661894867969,14.3420291426398,
130.700400837048)) ;
#145905=CARTESIAN_POINT('Ctrl Pts',(-19.7429904163147,14.4980360771653,
130.957766454984)) ;
#145906=CARTESIAN_POINT('Ctrl Pts',(-19.8302733403421,14.5780642539032,
131.245841073644)) ;
#145907=CARTESIAN_POINT('Ctrl Pts',(-19.921571119927,14.5747644514925,131.545879565233)) ;
#145908=CARTESIAN_POINT('Ctrl Pts',(-20.007901843405,14.489550077403,131.830999188099)) ;
#145909=CARTESIAN_POINT('Ctrl Pts',(-20.0841056157462,14.3274511232625,
132.086804079126)) ;
#145910=CARTESIAN_POINT('Ctrl Pts',(-20.1430494283501,14.10121310871,132.292050722471)) ;
#145911=CARTESIAN_POINT('Ctrl Pts',(-20.1802685099669,13.8249843797631,
132.434023249095)) ;
#145912=CARTESIAN_POINT('Ctrl Pts',(-20.1919483927985,13.5214320860101,
132.501202568774)) ;
#145913=CARTESIAN_POINT('Ctrl Pts',(-20.1767867112314,13.2103011439188,
132.490041780221)) ;
#145914=CARTESIAN_POINT('Ctrl Pts',(-20.1352091335675,12.9148531024708,
132.401647345103)) ;
#145915=CARTESIAN_POINT('Ctrl Pts',(-20.0688842605853,12.6543477240414,
132.24117051739)) ;
#145916=CARTESIAN_POINT('Ctrl Pts',(-19.983093218714,12.4511188454898,132.023484182445)) ;
#145917=CARTESIAN_POINT('Ctrl Pts',(-19.8816672758417,12.3156705346788,
131.760435661779)) ;
#145918=CARTESIAN_POINT('Ctrl Pts',(-19.7721629217621,12.2603783289395,
131.473684187594)) ;
#145919=CARTESIAN_POINT('Ctrl Pts',(-19.6616031715542,12.2883877322888,
131.183818528714)) ;
#145920=CARTESIAN_POINT('Ctrl Pts',(-19.5572825092889,12.396958266653,130.912081314997)) ;
#145921=CARTESIAN_POINT('Ctrl Pts',(-19.4649165468607,12.5805839766397,
130.675559335482)) ;
#145922=CARTESIAN_POINT('Ctrl Pts',(-19.3920517907422,12.8225431268309,
130.49566490348)) ;
#145923=CARTESIAN_POINT('Ctrl Pts',(-19.3417667776537,13.1085293602313,
130.381910274806)) ;
#145924=CARTESIAN_POINT('Ctrl Pts',(-19.3176156777269,13.4184312820959,
130.344629887277)) ;
#145925=CARTESIAN_POINT('Ctrl Pts',(-19.3204546895957,13.725396855158,130.38583576103)) ;
#145926=CARTESIAN_POINT('Ctrl Pts',(-19.3494655025508,14.0140710233184,
130.503873246052)) ;
#145927=CARTESIAN_POINT('Ctrl Pts',(-19.4017261950081,14.2586953082214,
130.689648250537)) ;
#145928=CARTESIAN_POINT('Ctrl Pts',(-19.4726871937748,14.4435712393275,
130.930045601665)) ;
#145929=CARTESIAN_POINT('Ctrl Pts',(-19.5566519911389,14.5554638081498,
131.208437931173)) ;
#145930=CARTESIAN_POINT('Ctrl Pts',(-19.6468808266438,14.5862678501096,
131.505140126049)) ;
#145931=CARTESIAN_POINT('Ctrl Pts',(-19.7360484351444,14.5339455279845,
131.798696701267)) ;
#145932=CARTESIAN_POINT('Ctrl Pts',(-19.8173615669052,14.4019055584218,
132.069386773039)) ;
#145933=CARTESIAN_POINT('Ctrl Pts',(-19.8839994555415,14.1996929308369,
132.297189223288)) ;
#145934=CARTESIAN_POINT('Ctrl Pts',(-19.9305118128425,13.9418839763085,
132.466195135576)) ;
#145935=CARTESIAN_POINT('Ctrl Pts',(-19.9528419276723,13.6467945517117,
132.56456832424)) ;
#145936=CARTESIAN_POINT('Ctrl Pts',(-19.9486515206637,13.3358857358536,
132.585446635425)) ;
#145937=CARTESIAN_POINT('Ctrl Pts',(-19.9175619038722,13.0311283359512,
132.527750633158)) ;
#145938=CARTESIAN_POINT('Ctrl Pts',(-19.8609233985763,12.7543595067604,
132.395451902013)) ;
#145939=CARTESIAN_POINT('Ctrl Pts',(-19.7827102679386,12.5263863833961,
132.199944643095)) ;
#145940=CARTESIAN_POINT('Ctrl Pts',(-19.6860393622514,12.3607017684255,
131.950953906113)) ;
#145941=CARTESIAN_POINT('Ctrl Pts',(-19.580104111669,12.2732420029804,131.674307412116)) ;
#145942=CARTESIAN_POINT('Ctrl Pts',(-19.4686330724515,12.2668291294782,
131.381938905443)) ;
#145943=CARTESIAN_POINT('Ctrl Pts',(-19.3608533291528,12.3436152480751,
131.100162840615)) ;
#145944=CARTESIAN_POINT('Ctrl Pts',(-19.2628621236054,12.4979168003383,
130.84708500029)) ;
#145945=CARTESIAN_POINT('Ctrl Pts',(-19.1815148595947,12.7181781437397,
130.642540710761)) ;
#145946=CARTESIAN_POINT('Ctrl Pts',(-19.1215859229779,12.9887185054322,
130.500562129518)) ;
#145947=CARTESIAN_POINT('Ctrl Pts',(-19.0866327913616,13.2908827967775,
130.431601676791)) ;
#145948=CARTESIAN_POINT('Ctrl Pts',(-19.0785282040241,13.6021684785122,
130.441033599336)) ;
#145949=CARTESIAN_POINT('Ctrl Pts',(-19.0971518047465,13.901537415506,130.52864407598)) ;
#145950=CARTESIAN_POINT('Ctrl Pts',(-19.1405520283606,14.1661758295122,
130.6886143988)) ;
#145951=CARTESIAN_POINT('Ctrl Pts',(-19.2042657866774,14.3763137224392,
130.907701859825)) ;
#145952=CARTESIAN_POINT('Ctrl Pts',(-19.2839098721216,14.5195379343594,
131.173557478438)) ;
#145953=CARTESIAN_POINT('Ctrl Pts',(-19.3721859569991,14.5837467777198,
131.464450468761)) ;
#145954=CARTESIAN_POINT('Ctrl Pts',(-19.4629509428763,14.5651055472896,
131.762802835642)) ;
#145955=CARTESIAN_POINT('Ctrl Pts',(-19.5482888539825,14.4645028537766,
132.045218992615)) ;
#145956=CARTESIAN_POINT('Ctrl Pts',(-19.6216217472489,14.2890439615902,
132.292607820973)) ;
#145957=CARTESIAN_POINT('Ctrl Pts',(-19.6766909799852,14.0526944517644,
132.486486401001)) ;
#145958=CARTESIAN_POINT('Ctrl Pts',(-19.7093072750895,13.7699865640071,
132.6149543649)) ;
#145959=CARTESIAN_POINT('Ctrl Pts',(-19.7161146198736,13.4631529119525,
132.667930442523)) ;
#145960=CARTESIAN_POINT('Ctrl Pts',(-19.6956515836537,13.1513620896954,
132.641483995069)) ;
#145961=CARTESIAN_POINT('Ctrl Pts',(-19.6494470974551,12.8627668245119,
132.539399272476)) ;
#145962=CARTESIAN_POINT('Ctrl Pts',(-19.5788203474868,12.6109028721184,
132.366417950411)) ;
#145963=CARTESIAN_POINT('Ctrl Pts',(-19.4899551594223,12.4200193080497,
132.139689682939)) ;
#145964=CARTESIAN_POINT('Ctrl Pts',(-19.3859186787791,12.298694725006,131.869172924049)) ;
#145965=CARTESIAN_POINT('Ctrl Pts',(-19.2763944386609,12.2592723921271,
131.582128978046)) ;
#145966=CARTESIAN_POINT('Ctrl Pts',(-19.165779613809,12.3030853474822,131.29229953169)) ;
#145967=CARTESIAN_POINT('Ctrl Pts',(-19.0638020603307,12.4259705793417,
131.027270360588)) ;
#145968=CARTESIAN_POINT('Ctrl Pts',(-18.9744571168751,12.6220550039555,
130.799590383652)) ;
#145969=CARTESIAN_POINT('Ctrl Pts',(-18.9054157982143,12.8744669424422,
130.630978711971)) ;
#145970=CARTESIAN_POINT('Ctrl Pts',(-18.8600323634942,13.1663406139675,
130.531527387548)) ;
#145971=CARTESIAN_POINT('Ctrl Pts',(-18.8410254999906,13.475878892664,130.509047923724)) ;
#145972=CARTESIAN_POINT('Ctrl Pts',(-18.848828895151,13.7823953075606,130.564962887383)) ;
#145973=CARTESIAN_POINT('Ctrl Pts',(-18.8826580153594,14.064418215805,130.69708049184)) ;
#145974=CARTESIAN_POINT('Ctrl Pts',(-18.9384679926998,14.2977471414108,
130.893033181098)) ;
#145975=CARTESIAN_POINT('Ctrl Pts',(-19.0125610674894,14.4706194179794,
131.142700487904)) ;
#145976=CARTESIAN_POINT('Ctrl Pts',(-19.09833071192,14.5675955159237,131.426393987923)) ;
#145977=CARTESIAN_POINT('Ctrl Pts',(-19.1887786220764,14.5827755983601,
131.723678445035)) ;
#145978=CARTESIAN_POINT('Ctrl Pts',(-19.2771526394746,14.5148008413574,
132.014994755847)) ;
#145979=CARTESIAN_POINT('Ctrl Pts',(-19.3559595938276,14.3692242855325,
132.278254867564)) ;
#145980=CARTESIAN_POINT('Ctrl Pts',(-19.4195009826797,14.1540994204916,
132.497190285371)) ;
#145981=CARTESIAN_POINT('Ctrl Pts',(-19.4614287947386,13.889194577701,132.652613367611)) ;
#145982=CARTESIAN_POINT('Ctrl Pts',(-19.479026321897,13.5894848313417,132.737169180434)) ;
#145983=CARTESIAN_POINT('Ctrl Pts',(-19.469691253169,13.2771021698192,132.743118485761)) ;
#145984=CARTESIAN_POINT('Ctrl Pts',(-19.4337533195738,12.9767128859996,
132.67117726944)) ;
#145985=CARTESIAN_POINT('Ctrl Pts',(-19.3723820364147,12.7063601582146,
132.525197848911)) ;
#145986=CARTESIAN_POINT('Ctrl Pts',(-19.2906337460424,12.4901609157503,
132.319283266615)) ;
#145987=CARTESIAN_POINT('Ctrl Pts',(-19.1920848992532,12.338688213011,132.064589679679)) ;
#145988=CARTESIAN_POINT('Ctrl Pts',(-19.0839647079271,12.2654833215425,
131.781836975828)) ;
#145989=CARTESIAN_POINT('Ctrl Pts',(-18.9727805931348,12.2750423939134,
131.490221782582)) ;
#145990=CARTESIAN_POINT('Ctrl Pts',(-18.8660747623374,12.3673309477628,
131.211686629903)) ;
#145991=CARTESIAN_POINT('Ctrl Pts',(-18.771239184174,12.5343469793072,130.96765150365)) ;
#145992=CARTESIAN_POINT('Ctrl Pts',(-18.693437502563,12.7652871615339,130.773485647564)) ;
#145993=CARTESIAN_POINT('Ctrl Pts',(-18.6378021901779,13.0444119641298,
130.644182284215)) ;
#145994=CARTESIAN_POINT('Ctrl Pts',(-18.6078827874849,13.3498617711502,
130.58989899629)) ;
#145995=CARTESIAN_POINT('Ctrl Pts',(-18.6049643640782,13.6613615410962,
130.614584854872)) ;
#145996=CARTESIAN_POINT('Ctrl Pts',(-18.6283610363628,13.9537822456917,
130.715914869578)) ;
#145997=CARTESIAN_POINT('Ctrl Pts',(-18.6757830396079,14.2096141723503,
130.887574922432)) ;
#145998=CARTESIAN_POINT('Ctrl Pts',(-18.7432084588704,14.4090573352496,
131.117688224262)) ;
#145999=CARTESIAN_POINT('Ctrl Pts',(-18.8248444961312,14.5378227777349,
131.389262062474)) ;
#146000=CARTESIAN_POINT('Ctrl Pts',(-18.9146615446444,14.5866410232384,
131.684888368504)) ;
#146001=CARTESIAN_POINT('Ctrl Pts',(-19.0042448193372,14.5524956968184,
131.979503816669)) ;
#146002=CARTESIAN_POINT('Ctrl Pts',(-19.0884275166112,14.4363359787846,
132.258795156506)) ;
#146003=CARTESIAN_POINT('Ctrl Pts',(-19.158384232285,14.2487612531945,132.496149660261)) ;
#146004=CARTESIAN_POINT('Ctrl Pts',(-19.2096369480705,14.0019963672536,
132.678965768853)) ;
#146005=CARTESIAN_POINT('Ctrl Pts',(-19.2375262292726,13.7133413750086,
132.793570526747)) ;
#146006=CARTESIAN_POINT('Ctrl Pts',(-19.2391685265025,13.4034231078491,
132.831554039307)) ;
#146007=CARTESIAN_POINT('Ctrl Pts',(-19.2140103146631,13.0966156009071,
132.791052370135)) ;
#146008=CARTESIAN_POINT('Ctrl Pts',(-19.1625096709922,12.8104956204696,
132.673916665319)) ;
#146009=CARTESIAN_POINT('Ctrl Pts',(-19.08847519723,12.5707042349948,132.490662999038)) ;
#146010=CARTESIAN_POINT('Ctrl Pts',(-18.9959730199521,12.3910193657153,
132.253550999424)) ;
#146011=CARTESIAN_POINT('Ctrl Pts',(-18.8908542141825,12.285328864528,131.979615249099)) ;
#146012=CARTESIAN_POINT('Ctrl Pts',(-18.7803139240097,12.2609818529467,
131.6897631227)) ;
#146013=CARTESIAN_POINT('Ctrl Pts',(-18.6705377025057,12.3204757590526,
131.402379707675)) ;
#146014=CARTESIAN_POINT('Ctrl Pts',(-18.5703346082798,12.4582515921679,
131.14266448369)) ;
#146015=CARTESIAN_POINT('Ctrl Pts',(-18.4846714167296,12.6658998652864,
130.92561853516)) ;
#146016=CARTESIAN_POINT('Ctrl Pts',(-18.4198906462997,12.9268096194457,
130.769416613743)) ;
#146017=CARTESIAN_POINT('Ctrl Pts',(-18.3793353527382,13.2233761882574,
130.684026781784)) ;
#146018=CARTESIAN_POINT('Ctrl Pts',(-18.3653039385833,13.5346577028184,
130.67616016624)) ;
#146019=CARTESIAN_POINT('Ctrl Pts',(-18.37825174114,13.8387961550216,130.747205171599)) ;
#146020=CARTESIAN_POINT('Ctrl Pts',(-18.416436223305,14.1123018093557,130.891880637841)) ;
#146021=CARTESIAN_POINT('Ctrl Pts',(-18.4764360525695,14.3364687446635,
131.100308420715)) ;
#146022=CARTESIAN_POINT('Ctrl Pts',(-18.5528414616942,14.494770833943,131.356525814744)) ;
#146023=CARTESIAN_POINT('Ctrl Pts',(-18.6403171302965,14.5769227995843,
131.645303937294)) ;
#146024=CARTESIAN_POINT('Ctrl Pts',(-18.7305714826929,14.5762675412157,
131.941905078074)) ;
#146025=CARTESIAN_POINT('Ctrl Pts',(-18.8178911875836,14.4930554177443,
132.23020487892)) ;
#146026=CARTESIAN_POINT('Ctrl Pts',(-18.8942971692305,14.3331650364545,
132.4865191295)) ;
#146027=CARTESIAN_POINT('Ctrl Pts',(-18.9539181012747,14.1081176093321,
132.693817778015)) ;
#146028=CARTESIAN_POINT('Ctrl Pts',(-18.9916963349415,13.8340178637995,
132.837300403657)) ;
#146029=CARTESIAN_POINT('Ctrl Pts',(-19.0042096670202,13.5302898798933,
132.90699864193)) ;
#146030=CARTESIAN_POINT('Ctrl Pts',(-18.989829242128,13.2194241455141,132.898077222158)) ;
#146031=CARTESIAN_POINT('Ctrl Pts',(-18.949020417078,12.9232187981691,132.811930535479)) ;
#146032=CARTESIAN_POINT('Ctrl Pts',(-18.8834324422067,12.6614612454166,
132.653582726297)) ;
#146033=CARTESIAN_POINT('Ctrl Pts',(-18.7979851633379,12.4560560128417,
132.436966453739)) ;
#146034=CARTESIAN_POINT('Ctrl Pts',(-18.6972333502297,12.3187614460116,
132.17577996401)) ;
#146035=CARTESIAN_POINT('Ctrl Pts',(-18.5877188076482,12.2608758912203,
131.889053743613)) ;
#146036=CARTESIAN_POINT('Ctrl Pts',(-18.4772617072998,12.2860567579314,
131.599425070931)) ;
#146037=CARTESIAN_POINT('Ctrl Pts',(-18.3717678028048,12.3936760882031,
131.324566267309)) ;
#146038=CARTESIAN_POINT('Ctrl Pts',(-18.2799662634484,12.5734427246259,
131.08932574441)) ;
#146039=CARTESIAN_POINT('Ctrl Pts',(-18.205832390456,12.8155556850103,130.905988455816)) ;
#146040=CARTESIAN_POINT('Ctrl Pts',(-18.1551033037978,13.1001458972495,
130.790857619227)) ;
#146041=CARTESIAN_POINT('Ctrl Pts',(-18.1301831955087,13.4082451879306,
130.751183187586)) ;
#146042=CARTESIAN_POINT('Ctrl Pts',(-18.1321866015327,13.7170001803432,
130.790102685016)) ;
#146043=CARTESIAN_POINT('Ctrl Pts',(-18.160608589631,14.0068803402206,130.906464225431)) ;
#146044=CARTESIAN_POINT('Ctrl Pts',(-18.2120937054126,14.2520830293328,
131.089860423946)) ;
#146045=CARTESIAN_POINT('Ctrl Pts',(-18.2824550721689,14.4388654830233,
131.328466488959)) ;
#146046=CARTESIAN_POINT('Ctrl Pts',(-18.3662181188831,14.5532758732377,
131.606309319578)) ;
#146047=CARTESIAN_POINT('Ctrl Pts',(-18.4564381360141,14.5866372920254,
131.903009380992)) ;
#146048=CARTESIAN_POINT('Ctrl Pts',(-18.5459782715731,14.5363254176441,
132.197752354425)) ;
#146049=CARTESIAN_POINT('Ctrl Pts',(-18.6272540069243,14.4070821621483,
132.46818035341)) ;
#146050=CARTESIAN_POINT('Ctrl Pts',(-18.6947300760767,14.2058492083664,
132.698587728027)) ;
#146051=CARTESIAN_POINT('Ctrl Pts',(-18.7417516398663,13.9493209948446,
132.869059993674)) ;
#146052=CARTESIAN_POINT('Ctrl Pts',(-18.7647488489571,13.6560816427411,
132.969264870124)) ;
#146053=CARTESIAN_POINT('Ctrl Pts',(-18.7613810278091,13.3454213686902,
132.992539638917)) ;
#146054=CARTESIAN_POINT('Ctrl Pts',(-18.7312094393375,13.0405957785926,
132.937469885673)) ;
#146055=CARTESIAN_POINT('Ctrl Pts',(-18.6749590606351,12.761020315257,132.806501464058)) ;
#146056=CARTESIAN_POINT('Ctrl Pts',(-18.5973111868101,12.5320804704421,
132.612600975859)) ;
#146057=CARTESIAN_POINT('Ctrl Pts',(-18.5017869925786,12.3651153247515,
132.366732593609)) ;
#146058=CARTESIAN_POINT('Ctrl Pts',(-18.3951993341836,12.2743249868604,
132.08846016447)) ;
#146059=CARTESIAN_POINT('Ctrl Pts',(-18.2836787398034,12.2660445265336,
131.795962720769)) ;
#146060=CARTESIAN_POINT('Ctrl Pts',(-18.1761286055653,12.3402671637665,
131.514732867287)) ;
#146061=CARTESIAN_POINT('Ctrl Pts',(-18.0777202181115,12.492431210345,131.260444160921)) ;
#146062=CARTESIAN_POINT('Ctrl Pts',(-17.9959153741565,12.7106681794057,
131.054521630885)) ;
#146063=CARTESIAN_POINT('Ctrl Pts',(-17.9351451797697,12.9803450583886,
130.910137294443)) ;
#146064=CARTESIAN_POINT('Ctrl Pts',(-17.8994023316142,13.2833171432177,
130.83901653828)) ;
#146065=CARTESIAN_POINT('Ctrl Pts',(-17.8906094381936,13.5926828813481,
130.846226131332)) ;
#146066=CARTESIAN_POINT('Ctrl Pts',(-17.9084948671421,13.8936498651441,
130.931784173422)) ;
#146067=CARTESIAN_POINT('Ctrl Pts',(-17.9511483769507,14.1589431067745,
131.089492755246)) ;
#146068=CARTESIAN_POINT('Ctrl Pts',(-18.0144302964997,14.3711507970921,
131.307375688141)) ;
#146069=CARTESIAN_POINT('Ctrl Pts',(-18.0934259365928,14.5162610816314,
131.571225045128)) ;
#146070=CARTESIAN_POINT('Ctrl Pts',(-18.182269930839,14.583306350133,131.864052397872)) ;
#146071=CARTESIAN_POINT('Ctrl Pts',(-18.272835722527,14.5665129586633,132.161733104664)) ;
#146072=CARTESIAN_POINT('Ctrl Pts',(-18.3581065810839,14.4685223967189,
132.443839852237)) ;
#146073=CARTESIAN_POINT('Ctrl Pts',(-18.4318404880964,14.2954966012034,
132.692357198206)) ;
#146074=CARTESIAN_POINT('Ctrl Pts',(-18.4877063256743,14.0596946296019,
132.888702759001)) ;
#146075=CARTESIAN_POINT('Ctrl Pts',(-18.5209832839551,13.7784555956093,
133.019039209871)) ;
#146076=CARTESIAN_POINT('Ctrl Pts',(-18.5284065230371,13.4704205391721,
133.073991147064)) ;
#146077=CARTESIAN_POINT('Ctrl Pts',(-18.5091035543004,13.1626906793203,
133.050459846182)) ;
#146078=CARTESIAN_POINT('Ctrl Pts',(-18.4631732366913,12.8697533216184,
132.949576875133)) ;
#146079=CARTESIAN_POINT('Ctrl Pts',(-18.3938110455771,12.6186668370347,
132.77997790901)) ;
#146080=CARTESIAN_POINT('Ctrl Pts',(-18.3046231204081,12.4240570551779,
132.552627422137)) ;
#146081=CARTESIAN_POINT('Ctrl Pts',(-18.2019920844373,12.301712902155,132.285853012118)) ;
#146082=CARTESIAN_POINT('Ctrl Pts',(-18.0917742767469,12.2592124433866,
131.997041312157)) ;
#146083=CARTESIAN_POINT('Ctrl Pts',(-17.9815995706875,12.3002004237818,
131.708316187743)) ;
#146084=CARTESIAN_POINT('Ctrl Pts',(-17.8782460339929,12.4222100081088,
131.439623337485)) ;
#146085=CARTESIAN_POINT('Ctrl Pts',(-17.7891702075967,12.6151763804986,
131.212464661044)) ;
#146086=CARTESIAN_POINT('Ctrl Pts',(-17.7192518879757,12.866763553233,131.041393055734)) ;
#146087=CARTESIAN_POINT('Ctrl Pts',(-17.6733163828393,13.1566083036236,
130.940190964357)) ;
#146088=CARTESIAN_POINT('Ctrl Pts',(-17.6533605413985,13.4669635155183,
130.91505403219)) ;
#146089=CARTESIAN_POINT('Ctrl Pts',(-17.660526594431,13.7743605860558,130.969164445883)) ;
#146090=CARTESIAN_POINT('Ctrl Pts',(-17.6933658448605,14.0556835712851,
131.098173550433)) ;
#146091=CARTESIAN_POINT('Ctrl Pts',(-17.7488867045143,14.2923698679386,
131.293503308698)) ;
#146092=CARTESIAN_POINT('Ctrl Pts',(-17.8227133439083,14.4669398360514,
131.54242287109)) ;
#146093=CARTESIAN_POINT('Ctrl Pts',(-17.9077423757333,14.5658237204842,
131.823764797856)) ;
#146094=CARTESIAN_POINT('Ctrl Pts',(-17.9986684570008,14.5834030750835,
132.122644069035)) ;
#146095=CARTESIAN_POINT('Ctrl Pts',(-18.0867233838671,14.5182209369221,
132.412831774384)) ;
#146096=CARTESIAN_POINT('Ctrl Pts',(-18.1665697451038,14.3732472228341,
132.679438010564)) ;
#146097=CARTESIAN_POINT('Ctrl Pts',(-18.2299692526917,14.161734042983,132.897630258977)) ;
#146098=CARTESIAN_POINT('Ctrl Pts',(-18.2728829473476,13.8968738672396,
133.056114256463)) ;
#146099=CARTESIAN_POINT('Ctrl Pts',(-18.2911187814473,13.5970560174392,
133.142599500408)) ;
#146100=CARTESIAN_POINT('Ctrl Pts',(-18.2824786204777,13.285349771455,133.150512015157)) ;
#146101=CARTESIAN_POINT('Ctrl Pts',(-18.2473862581819,12.9854213227035,
133.080929265439)) ;
#146102=CARTESIAN_POINT('Ctrl Pts',(-18.1869883996118,12.7145025865389,
132.937690581817)) ;
#146103=CARTESIAN_POINT('Ctrl Pts',(-18.1054391959301,12.4953422149561,
132.732519305131)) ;
#146104=CARTESIAN_POINT('Ctrl Pts',(-18.0070761592923,12.3417857538749,
132.478417504927)) ;
#146105=CARTESIAN_POINT('Ctrl Pts',(-17.8994483905022,12.2665368093941,
132.197008614467)) ;
#146106=CARTESIAN_POINT('Ctrl Pts',(-17.7883645178934,12.2735361740405,
131.905651880035)) ;
#146107=CARTESIAN_POINT('Ctrl Pts',(-17.6814644389021,12.3632299565235,
131.626530218229)) ;
#146108=CARTESIAN_POINT('Ctrl Pts',(-17.5858934658356,12.5286847950401,
131.380452412425)) ;
#146109=CARTESIAN_POINT('Ctrl Pts',(-17.5076122654555,12.7579694730324,
131.18486375994)) ;
#146110=CARTESIAN_POINT('Ctrl Pts',(-17.4513694267864,13.0352202971202,
131.053701691009)) ;
#146111=CARTESIAN_POINT('Ctrl Pts',(-17.4206145070061,13.3405829184085,
130.99702547713)) ;
#146112=CARTESIAN_POINT('Ctrl Pts',(-17.4168444194452,13.6512271972451,
131.019110996205)) ;
#146113=CARTESIAN_POINT('Ctrl Pts',(-17.4395135787806,13.9458587168303,
131.118464332761)) ;
#146114=CARTESIAN_POINT('Ctrl Pts',(-17.4864529506928,14.2033946727232,
131.288774833455)) ;
#146115=CARTESIAN_POINT('Ctrl Pts',(-17.5532007112171,14.4040391264647,
131.51681448999)) ;
#146116=CARTESIAN_POINT('Ctrl Pts',(-17.6343956033889,14.5350227428464,
131.787065599792)) ;
#146117=CARTESIAN_POINT('Ctrl Pts',(-17.7242162985725,14.5864958766325,
132.082749953862)) ;
#146118=CARTESIAN_POINT('Ctrl Pts',(-17.8140541710382,14.5544169233344,
132.37817969897)) ;
#146119=CARTESIAN_POINT('Ctrl Pts',(-17.8980266225735,14.4414134366696,
132.656647056367)) ;
#146120=CARTESIAN_POINT('Ctrl Pts',(-17.968839016247,14.2551029691134,132.896663337422)) ;
#146121=CARTESIAN_POINT('Ctrl Pts',(-18.0206609436882,14.0100365412081,
133.081103390275)) ;
#146122=CARTESIAN_POINT('Ctrl Pts',(-18.0493014678381,13.7214335751914,
133.198003238596)) ;
#146123=CARTESIAN_POINT('Ctrl Pts',(-18.051767121632,13.4135493095884,133.23819933318)) ;
#146124=CARTESIAN_POINT('Ctrl Pts',(-18.0272159345045,13.1045553543373,
133.199678527869)) ;
#146125=CARTESIAN_POINT('Ctrl Pts',(-17.9769019731203,12.819735905808,133.085728232042)) ;
#146126=CARTESIAN_POINT('Ctrl Pts',(-17.9029324475278,12.5762135123813,
132.902947309471)) ;
#146127=CARTESIAN_POINT('Ctrl Pts',(-17.8110109172599,12.3952019865551,
132.66745603075)) ;
#146128=CARTESIAN_POINT('Ctrl Pts',(-17.7060493534379,12.2871509096393,
132.394018600026)) ;
#146129=CARTESIAN_POINT('Ctrl Pts',(-17.5958228629102,12.2605661260812,
132.105006344478)) ;
#146130=CARTESIAN_POINT('Ctrl Pts',(-17.4859053807389,12.3174696156297,
131.817205208931)) ;
#146131=CARTESIAN_POINT('Ctrl Pts',(-17.385124499541,12.4535095799729,131.555883884411)) ;
#146132=CARTESIAN_POINT('Ctrl Pts',(-17.2991717616446,12.6588731415835,
131.337907662609)) ;
#146133=CARTESIAN_POINT('Ctrl Pts',(-17.2336625509736,12.9185733098552,
131.179601474472)) ;
#146134=CARTESIAN_POINT('Ctrl Pts',(-17.1923625242315,13.2144047799764,
131.09203406909)) ;
#146135=CARTESIAN_POINT('Ctrl Pts',(-17.1775577739653,13.5255442513147,
131.081906877128)) ;
#146136=CARTESIAN_POINT('Ctrl Pts',(-17.18966249855,13.8297540824603,131.150429396587)) ;
#146137=CARTESIAN_POINT('Ctrl Pts',(-17.227235954351,14.1049218673864,131.293388869168)) ;
#146138=CARTESIAN_POINT('Ctrl Pts',(-17.2862925400434,14.3298724417038,
131.498889388524)) ;
#146139=CARTESIAN_POINT('Ctrl Pts',(-17.3628237983981,14.4915528402348,
131.755720653574)) ;
#146140=CARTESIAN_POINT('Ctrl Pts',(-17.449818689308,14.5755974614276,132.042977501466)) ;
#146141=CARTESIAN_POINT('Ctrl Pts',(-17.5402166301667,14.5774288175943,
132.340058427624)) ;
#146142=CARTESIAN_POINT('Ctrl Pts',(-17.6275292470889,14.4968431022692,
132.628248586778)) ;
#146143=CARTESIAN_POINT('Ctrl Pts',(-17.7046127069172,14.3385595023236,
132.886659534106)) ;
#146144=CARTESIAN_POINT('Ctrl Pts',(-17.7647314828476,14.1152209980979,
133.095389388544)) ;
#146145=CARTESIAN_POINT('Ctrl Pts',(-17.8031897569592,13.8419813754815,
133.240889834337)) ;
#146146=CARTESIAN_POINT('Ctrl Pts',(-17.8164226854489,13.5398084238246,
133.3125803987)) ;
#146147=CARTESIAN_POINT('Ctrl Pts',(-17.8028647743182,13.2280435028726,
133.306145228451)) ;
#146148=CARTESIAN_POINT('Ctrl Pts',(-17.762509518981,12.9300590292135,133.221455259361)) ;
#146149=CARTESIAN_POINT('Ctrl Pts',(-17.6978430232198,12.6684083848218,
133.065633233242)) ;
#146150=CARTESIAN_POINT('Ctrl Pts',(-17.6127910105085,12.4608091208846,
132.850228765349)) ;
#146151=CARTESIAN_POINT('Ctrl Pts',(-17.5122972473823,12.3214093347923,
132.589814453629)) ;
#146152=CARTESIAN_POINT('Ctrl Pts',(-17.4027531001663,12.2613302981185,
132.303050991841)) ;
#146153=CARTESIAN_POINT('Ctrl Pts',(-17.2926710306357,12.2843255086961,
132.014392933773)) ;
#146154=CARTESIAN_POINT('Ctrl Pts',(-17.187376124559,12.3887269891781,131.73995348577)) ;
#146155=CARTESIAN_POINT('Ctrl Pts',(-17.094528490589,12.567362762576,131.501852203403)) ;
#146156=CARTESIAN_POINT('Ctrl Pts',(-17.0198679665341,12.8080166965812,
131.316965273115)) ;
#146157=CARTESIAN_POINT('Ctrl Pts',(-16.9684023291972,13.0914774469774,
131.199671601539)) ;
#146158=CARTESIAN_POINT('Ctrl Pts',(-16.9426807542661,13.4005589719555,
131.157796261443)) ;
#146159=CARTESIAN_POINT('Ctrl Pts',(-16.9440165303375,13.7083911607305,
131.194641100135)) ;
#146160=CARTESIAN_POINT('Ctrl Pts',(-16.9715883950981,13.9985991355892,
131.308446049961)) ;
#146161=CARTESIAN_POINT('Ctrl Pts',(-17.0225241829903,14.2457812535683,
131.490297397422)) ;
#146162=CARTESIAN_POINT('Ctrl Pts',(-17.0924768410808,14.434573414283,131.727731486366)) ;
#146163=CARTESIAN_POINT('Ctrl Pts',(-17.1759989243048,14.5511370884747,
132.004883776446)) ;
#146164=CARTESIAN_POINT('Ctrl Pts',(-17.2658532219854,14.5867802191552,
132.300414745677)) ;
#146165=CARTESIAN_POINT('Ctrl Pts',(-17.3555337669737,14.5391948457713,
132.595565619242)) ;
#146166=CARTESIAN_POINT('Ctrl Pts',(-17.4374124666097,14.4115345320068,
132.867878527861)) ;
#146167=CARTESIAN_POINT('Ctrl Pts',(-17.5049786238165,14.2134355726879,
133.098342340037)) ;
#146168=CARTESIAN_POINT('Ctrl Pts',(-17.5528570162914,13.958237750451,133.271366129121)) ;
#146169=CARTESIAN_POINT('Ctrl Pts',(-17.5766815250463,13.6646542433851,
133.374114982498)) ;
#146170=CARTESIAN_POINT('Ctrl Pts',(-17.5740742648385,13.3541836423797,
133.399606053148)) ;
#146171=CARTESIAN_POINT('Ctrl Pts',(-17.5445387474705,13.0484268899304,
133.346452700391)) ;
#146172=CARTESIAN_POINT('Ctrl Pts',(-17.4893307298857,12.769439556936,133.218328729894)) ;
#146173=CARTESIAN_POINT('Ctrl Pts',(-17.4122024226174,12.538041732005,133.026020671942)) ;
#146174=CARTESIAN_POINT('Ctrl Pts',(-17.3165197740753,12.3683285737822,
132.77987187364)) ;
#146175=CARTESIAN_POINT('Ctrl Pts',(-17.2106392056921,12.2760420146323,
132.503507847891)) ;
#146176=CARTESIAN_POINT('Ctrl Pts',(-17.0996526659154,12.2649172046645,
132.212420970085)) ;
#146177=CARTESIAN_POINT('Ctrl Pts',(-16.9913739789809,12.3368690960139,
131.929222871054)) ;
#146178=CARTESIAN_POINT('Ctrl Pts',(-16.8925201645751,12.4871143046054,
131.67365659481)) ;
#146179=CARTESIAN_POINT('Ctrl Pts',(-16.8100266244737,12.7041606562746,
131.465789941374)) ;
#146180=CARTESIAN_POINT('Ctrl Pts',(-16.7488144744473,12.9721743226057,
131.320042358429)) ;
#146181=CARTESIAN_POINT('Ctrl Pts',(-16.7123802766638,13.2726903984431,
131.246711119902)) ;
#146182=CARTESIAN_POINT('Ctrl Pts',(-16.7026684240063,13.5844635777056,
131.251490845653)) ;
#146183=CARTESIAN_POINT('Ctrl Pts',(-16.7198723144853,13.8852371899129,
131.334971985811)) ;
#146184=CARTESIAN_POINT('Ctrl Pts',(-16.7615944094477,14.1508961258859,
131.489831947096)) ;
#146185=CARTESIAN_POINT('Ctrl Pts',(-16.8244978834266,14.3659570919706,
131.706731651083)) ;
#146186=CARTESIAN_POINT('Ctrl Pts',(-16.903483751971,14.5133844766524,131.970678602505)) ;
#146187=CARTESIAN_POINT('Ctrl Pts',(-16.9914123716409,14.5822824975676,
132.26055324515)) ;
#146188=CARTESIAN_POINT('Ctrl Pts',(-17.0822412219883,14.5684017551043,
132.559086977075)) ;
#146189=CARTESIAN_POINT('Ctrl Pts',(-17.1679464043999,14.4726240030268,
132.842523268284)) ;
#146190=CARTESIAN_POINT('Ctrl Pts',(-17.2423050049178,14.3009017831871,
133.092973244359)) ;
#146191=CARTESIAN_POINT('Ctrl Pts',(-17.2985250729578,14.0676661547484,
133.290210100475)) ;
#146192=CARTESIAN_POINT('Ctrl Pts',(-17.3325852755681,13.7867922981234,
133.422922252114)) ;
#146193=CARTESIAN_POINT('Ctrl Pts',(-17.340812658842,13.4808115386222,133.480046696113)) ;
#146194=CARTESIAN_POINT('Ctrl Pts',(-17.322213176098,13.1706177086878,133.458812233851)) ;
#146195=CARTESIAN_POINT('Ctrl Pts',(-17.2768978369704,12.877048394192,133.35971302766)) ;
#146196=CARTESIAN_POINT('Ctrl Pts',(-17.2082784989992,12.6251910446387,
133.192217667791)) ;
#146197=CARTESIAN_POINT('Ctrl Pts',(-17.1198239714151,12.4289584730978,
132.966933197476)) ;
#146198=CARTESIAN_POINT('Ctrl Pts',(-17.016947151482,12.3038002385442,132.699618788606)) ;
#146199=CARTESIAN_POINT('Ctrl Pts',(-16.9070593349269,12.2593442702032,
132.411696671294)) ;
#146200=CARTESIAN_POINT('Ctrl Pts',(-16.7970423402235,12.2978898762746,
132.123361876262)) ;
#146201=CARTESIAN_POINT('Ctrl Pts',(-16.6936288501025,12.4169444265874,
131.854394739963)) ;
#146202=CARTESIAN_POINT('Ctrl Pts',(-16.6034534816505,12.6093773192219,
131.624257767718)) ;
#146203=CARTESIAN_POINT('Ctrl Pts',(-16.5333014451683,12.8583734151229,
131.452333124793)) ;
#146204=CARTESIAN_POINT('Ctrl Pts',(-16.4864482413194,13.1480449796925,
131.348541807378)) ;
#146205=CARTESIAN_POINT('Ctrl Pts',(-16.4657803621371,13.4582418088587,
131.321329051345)) ;
#146206=CARTESIAN_POINT('Ctrl Pts',(-16.4721450959125,13.7655079341762,
131.373040893652)) ;
#146207=CARTESIAN_POINT('Ctrl Pts',(-16.5043240159691,14.048316994012,131.500173624113)) ;
#146208=CARTESIAN_POINT('Ctrl Pts',(-16.55917049357,14.2859990299988,131.693469739828)) ;
#146209=CARTESIAN_POINT('Ctrl Pts',(-16.6322772804353,14.4624790722787,
131.940192970349)) ;
#146210=CARTESIAN_POINT('Ctrl Pts',(-16.7176228652551,14.5642184031824,
132.222682879556)) ;
#146211=CARTESIAN_POINT('Ctrl Pts',(-16.8079333251705,14.584160945988,132.519546694171)) ;
#146212=CARTESIAN_POINT('Ctrl Pts',(-16.8967026449305,14.5209707107522,
132.812037468598)) ;
#146213=CARTESIAN_POINT('Ctrl Pts',(-16.9763340125269,14.3791778899535,
133.077768668898)) ;
#146214=CARTESIAN_POINT('Ctrl Pts',(-17.0406340695259,14.1688150689694,
133.298742386899)) ;
#146215=CARTESIAN_POINT('Ctrl Pts',(-17.0841510266317,13.9051956236196,
133.458976239671)) ;
#146216=CARTESIAN_POINT('Ctrl Pts',(-17.1031304829445,13.6071499712881,
133.547524781534)) ;
#146217=CARTESIAN_POINT('Ctrl Pts',(-17.095445226368,13.2953842790605,133.55823520747)) ;
#146218=CARTESIAN_POINT('Ctrl Pts',(-17.0608564828447,12.9930168542047,
133.49033126729)) ;
#146219=CARTESIAN_POINT('Ctrl Pts',(-17.0014002167995,12.722227284065,133.349682917051)) ;
#146220=CARTESIAN_POINT('Ctrl Pts',(-16.920181788314,12.5005440271994,133.145587035709)) ;
#146221=CARTESIAN_POINT('Ctrl Pts',(-16.822238500183,12.3451352919228,132.892688097985)) ;
#146222=CARTESIAN_POINT('Ctrl Pts',(-16.7147807681509,12.2674914162103,
132.611784861536)) ;
#146223=CARTESIAN_POINT('Ctrl Pts',(-16.603381855895,12.2722652816386,132.319595696845)) ;
#146224=CARTESIAN_POINT('Ctrl Pts',(-16.4963775783064,12.3599738875374,
132.040146264629)) ;
#146225=CARTESIAN_POINT('Ctrl Pts',(-16.40080748811,12.522637910065,131.793927324611)) ;
#146226=CARTESIAN_POINT('Ctrl Pts',(-16.321682629452,12.7508223350777,131.595969665067)) ;
#146227=CARTESIAN_POINT('Ctrl Pts',(-16.2646694657802,13.0279566235447,
131.462655335791)) ;
#146228=CARTESIAN_POINT('Ctrl Pts',(-16.2333313099527,13.3323088318152,
131.40421290911)) ;
#146229=CARTESIAN_POINT('Ctrl Pts',(-16.2287969756995,13.6420774787073,
131.423958328797)) ;
#146230=CARTESIAN_POINT('Ctrl Pts',(-16.2506794474225,13.9374078863426,
131.521003414245)) ;
#146231=CARTESIAN_POINT('Ctrl Pts',(-16.2969248519444,14.1965319765984,
131.68929487346)) ;
#146232=CARTESIAN_POINT('Ctrl Pts',(-16.3636006492136,14.3999725992787,
131.917314329854)) ;
#146233=CARTESIAN_POINT('Ctrl Pts',(-16.4440741066575,14.5320840225921,
132.185279118148)) ;
#146234=CARTESIAN_POINT('Ctrl Pts',(-16.5336015824952,14.5862914481746,
132.480055865257)) ;
#146235=CARTESIAN_POINT('Ctrl Pts',(-16.6240180686935,14.5562373139742,
132.777363371128)) ;
#146236=CARTESIAN_POINT('Ctrl Pts',(-16.7077455074844,14.446076002877,133.054911135565)) ;
#146237=CARTESIAN_POINT('Ctrl Pts',(-16.7793513256384,14.2613118658137,
133.29736654614)) ;
#146238=CARTESIAN_POINT('Ctrl Pts',(-16.8317784891826,14.0168342944467,
133.483655477492)) ;
#146239=CARTESIAN_POINT('Ctrl Pts',(-16.8609906465943,13.7314084945653,
133.601972817066)) ;
#146240=CARTESIAN_POINT('Ctrl Pts',(-16.8642673995017,13.4213927806631,
133.644806850243)) ;
#146241=CARTESIAN_POINT('Ctrl Pts',(-16.8405564164842,13.1138964829047,
133.608540738459)) ;
#146242=CARTESIAN_POINT('Ctrl Pts',(-16.7909211560091,12.8273574952535,
133.496655651129)) ;
#146243=CARTESIAN_POINT('Ctrl Pts',(-16.7174808384362,12.5821904217373,
133.315441011606)) ;
#146244=CARTESIAN_POINT('Ctrl Pts',(-16.6259022245879,12.3992406566731,
133.080982325427)) ;
#146245=CARTESIAN_POINT('Ctrl Pts',(-16.5215735406818,12.2892635320147,
132.809278724701)) ;
#146246=CARTESIAN_POINT('Ctrl Pts',(-16.4111844090626,12.2601882735182,
132.519864635604)) ;
#146247=CARTESIAN_POINT('Ctrl Pts',(-16.3015215656193,12.3144490437337,
132.232684612256)) ;
#146248=CARTESIAN_POINT('Ctrl Pts',(-16.200280314493,12.4481500552587,131.970047674196)) ;
#146249=CARTESIAN_POINT('Ctrl Pts',(-16.113745113496,12.6515765738091,131.750375686591)) ;
#146250=CARTESIAN_POINT('Ctrl Pts',(-16.047245764908,12.911209097722,131.589339229255)) ;
#146251=CARTESIAN_POINT('Ctrl Pts',(-16.0053029062974,13.2069681338802,
131.499952091212)) ;
#146252=CARTESIAN_POINT('Ctrl Pts',(-15.9898149035429,13.5165271467016,
131.487670352965)) ;
#146253=CARTESIAN_POINT('Ctrl Pts',(-16.0012609274539,13.8224961920609,
131.554412215482)) ;
#146254=CARTESIAN_POINT('Ctrl Pts',(-16.0380155767778,14.0973150821475,
131.694808594853)) ;
#146255=CARTESIAN_POINT('Ctrl Pts',(-16.0966000359878,14.3244518569206,
131.899001803462)) ;
#146256=CARTESIAN_POINT('Ctrl Pts',(-16.1726120215274,14.4877799967397,
132.15425492571)) ;
#146257=CARTESIAN_POINT('Ctrl Pts',(-16.2592709157759,14.5742905029568,
132.440493252649)) ;
#146258=CARTESIAN_POINT('Ctrl Pts',(-16.3500516483461,14.5785355282753,
132.738832343294)) ;
#146259=CARTESIAN_POINT('Ctrl Pts',(-16.4374337885806,14.4999982805016,
133.02719053569)) ;
#146260=CARTESIAN_POINT('Ctrl Pts',(-16.5145794309264,14.344757358462,133.28562333112)) ;
#146261=CARTESIAN_POINT('Ctrl Pts',(-16.5755120854339,14.1223923332962,
133.49685600228)) ;
#146262=CARTESIAN_POINT('Ctrl Pts',(-16.6145706090846,13.8510685521418,
133.644018688014)) ;
#146263=CARTESIAN_POINT('Ctrl Pts',(-16.6286485860927,13.5484335086258,
133.718296216895)) ;
#146264=CARTESIAN_POINT('Ctrl Pts',(-16.6158251047736,13.2370240609784,
133.713960203863)) ;
#146265=CARTESIAN_POINT('Ctrl Pts',(-16.5763969172709,12.9391310692164,
133.631884681932)) ;
#146266=CARTESIAN_POINT('Ctrl Pts',(-16.5123859500824,12.6756659712694,
133.478021949865)) ;
#146267=CARTESIAN_POINT('Ctrl Pts',(-16.427629899397,12.4657027471288,133.263569069972)) ;
#146268=CARTESIAN_POINT('Ctrl Pts',(-16.3275418282825,12.3244745287068,
133.004314673347)) ;
#146269=CARTESIAN_POINT('Ctrl Pts',(-16.2186503349576,12.2619232724697,
132.719311023849)) ;
#146270=CARTESIAN_POINT('Ctrl Pts',(-16.1077327239437,12.2825882461712,
132.428447362504)) ;
#146271=CARTESIAN_POINT('Ctrl Pts',(-16.0025399530748,12.3846501373822,
132.154198120639)) ;
#146272=CARTESIAN_POINT('Ctrl Pts',(-15.9092526009268,12.5611187376007,
131.914805460089)) ;
#146273=CARTESIAN_POINT('Ctrl Pts',(-15.8339742586128,12.8001289118654,
131.72810568261)) ;
#146274=CARTESIAN_POINT('Ctrl Pts',(-15.7817650558556,13.0829558583446,
131.608682645535)) ;
#146275=CARTESIAN_POINT('Ctrl Pts',(-15.7552921984508,13.3903655570018,
131.564473572041)) ;
#146276=CARTESIAN_POINT('Ctrl Pts',(-15.7558344968402,13.7001366244489,
131.599183864421)) ;
#146277=CARTESIAN_POINT('Ctrl Pts',(-15.7825612660351,13.9898881879969,
131.710361207101)) ;
#146278=CARTESIAN_POINT('Ctrl Pts',(-15.8329158030238,14.2391934604651,
131.890590896131)) ;
#146279=CARTESIAN_POINT('Ctrl Pts',(-15.902293018607,14.4298567276207,132.126306082656)) ;
#146280=CARTESIAN_POINT('Ctrl Pts',(-15.9860173892895,14.5492471456149,
132.404244702619)) ;
#146281=CARTESIAN_POINT('Ctrl Pts',(-16.0754794895065,14.5868020959289,
132.698512209234)) ;
#146282=CARTESIAN_POINT('Ctrl Pts',(-16.1651952894194,14.5417975153692,
132.99373545863)) ;
#146283=CARTESIAN_POINT('Ctrl Pts',(-16.2474295569201,14.4162088209851,
133.26710820894)) ;
#146284=CARTESIAN_POINT('Ctrl Pts',(-16.3154498224604,14.2204083214859,
133.498849848744)) ;
#146285=CARTESIAN_POINT('Ctrl Pts',(-16.364198904732,13.9647701024183,133.674638082656)) ;
#146286=CARTESIAN_POINT('Ctrl Pts',(-16.3885363920283,13.6739288437871,
133.77865485733)) ;
#146287=CARTESIAN_POINT('Ctrl Pts',(-16.3867167940381,13.362328471029,133.806593586957)) ;
#146288=CARTESIAN_POINT('Ctrl Pts',(-16.3579953894516,13.0574724209015,
133.755675698701)) ;
#146289=CARTESIAN_POINT('Ctrl Pts',(-16.3035992847228,12.7770676806865,
133.629936979636)) ;
#146290=CARTESIAN_POINT('Ctrl Pts',(-16.2263721109659,12.5427864739332,
133.437579054895)) ;
#146291=CARTESIAN_POINT('Ctrl Pts',(-16.1323081173652,12.3731888111629,
133.195738527186)) ;
#146292=CARTESIAN_POINT('Ctrl Pts',(-16.0260671047681,12.2773794230824,
132.918532204642)) ;
#146293=CARTESIAN_POINT('Ctrl Pts',(-15.9148031459185,12.2641879723106,
132.626720167564)) ;
#146294=CARTESIAN_POINT('Ctrl Pts',(-15.8067357439252,12.3335960858358,
132.34402376968)) ;
#146295=CARTESIAN_POINT('Ctrl Pts',(-15.7074889808104,12.4815617101667,
132.087309224399)) ;
#146296=CARTESIAN_POINT('Ctrl Pts',(-15.6244038386482,12.6968288003286,
131.87771937363)) ;
#146297=CARTESIAN_POINT('Ctrl Pts',(-15.5624078276461,12.9642191171328,
131.729755714177)) ;
#146298=CARTESIAN_POINT('Ctrl Pts',(-15.5252477520953,13.2637556030546,
131.654261303762)) ;
#146299=CARTESIAN_POINT('Ctrl Pts',(-15.51483397363,13.5766924952844,131.657121610923)) ;
#146300=CARTESIAN_POINT('Ctrl Pts',(-15.5310818707384,13.8753723119149,
131.737498039997)) ;
#146301=CARTESIAN_POINT('Ctrl Pts',(-15.5723926579611,14.1446746282912,
131.891438338589)) ;
#146302=CARTESIAN_POINT('Ctrl Pts',(-15.6347429021983,14.3606486732163,
132.106650818172)) ;
#146303=CARTESIAN_POINT('Ctrl Pts',(-15.7130545539066,14.510078619128,132.368523960334)) ;
#146304=CARTESIAN_POINT('Ctrl Pts',(-15.8014941644787,14.5815775918547,
132.66014711967)) ;
#146305=CARTESIAN_POINT('Ctrl Pts',(-15.8916848447273,14.5700419701179,
132.956563000691)) ;
#146306=CARTESIAN_POINT('Ctrl Pts',(-15.9780332182577,14.4761037327312,
133.242048390542)) ;
#146307=CARTESIAN_POINT('Ctrl Pts',(-16.0524313118317,14.3074346005472,
133.492417860637)) ;
#146308=CARTESIAN_POINT('Ctrl Pts',(-16.1096785706815,14.073572566118,133.6929606647)) ;
#146309=CARTESIAN_POINT('Ctrl Pts',(-16.1440328164937,13.7966474057212,
133.82617193438)) ;
#146310=CARTESIAN_POINT('Ctrl Pts',(-16.1531898468542,13.4894704941488,
133.886207558095)) ;
#146311=CARTESIAN_POINT('Ctrl Pts',(-16.1353814446473,13.1800818047294,
133.867171716919)) ;
#146312=CARTESIAN_POINT('Ctrl Pts',(-16.0908480942642,12.8853355952022,
133.770390398962)) ;
#146313=CARTESIAN_POINT('Ctrl Pts',(-16.0227996234303,12.6318025855322,
133.604593537981)) ;
#146314=CARTESIAN_POINT('Ctrl Pts',(-15.9348050473155,12.4337108442548,
133.380663235259)) ;
#146315=CARTESIAN_POINT('Ctrl Pts',(-15.8324634579182,12.3064394695167,
133.114845627519)) ;
#146316=CARTESIAN_POINT('Ctrl Pts',(-15.7223718021778,12.259467253753,132.826428638725)) ;
#146317=CARTESIAN_POINT('Ctrl Pts',(-15.61237482116,12.2954707770716,132.538108209265)) ;
#146318=CARTESIAN_POINT('Ctrl Pts',(-15.5080697165881,12.4135506736779,
132.266757070083)) ;
#146319=CARTESIAN_POINT('Ctrl Pts',(-15.4186188949712,12.6014761688176,
132.038284950102)) ;
#146320=CARTESIAN_POINT('Ctrl Pts',(-15.3471518246755,12.8505488617132,
131.862777352297)) ;
#146321=CARTESIAN_POINT('Ctrl Pts',(-15.2996665374583,13.1393106642719,
131.75711736515)) ;
#146322=CARTESIAN_POINT('Ctrl Pts',(-15.2782008897368,13.4495612707078,
131.727612757336)) ;
#146323=CARTESIAN_POINT('Ctrl Pts',(-15.2838028221544,13.7566531065693,
131.777034142582)) ;
#146324=CARTESIAN_POINT('Ctrl Pts',(-15.3152314145327,14.0404143617275,
131.901967955441)) ;
#146325=CARTESIAN_POINT('Ctrl Pts',(-15.369451427365,14.2798568103851,132.093440892985)) ;
#146326=CARTESIAN_POINT('Ctrl Pts',(-15.4424743213,14.4588607973601,132.34006491953)) ;
#146327=CARTESIAN_POINT('Ctrl Pts',(-15.5270913631344,14.5622468207321,
132.620235903549)) ;
#146328=CARTESIAN_POINT('Ctrl Pts',(-15.6176932560271,14.5847589284177,
132.918083757224)) ;
#146329=CARTESIAN_POINT('Ctrl Pts',(-15.7063494799737,14.5239999294188,
133.210141637278)) ;
#146330=CARTESIAN_POINT('Ctrl Pts',(-15.7864511470471,14.3842925756614,
133.4772918037)) ;
#146331=CARTESIAN_POINT('Ctrl Pts',(-15.8512389369364,14.1758058754008,
133.699671458692)) ;
#146332=CARTESIAN_POINT('Ctrl Pts',(-15.8955022373477,13.9130883833925,
133.862137470225)) ;
#146333=CARTESIAN_POINT('Ctrl Pts',(-15.9151622120142,13.6151579335754,
133.952729954653)) ;
#146334=CARTESIAN_POINT('Ctrl Pts',(-15.9082762302878,13.3050553518441,
133.965606077722)) ;
#146335=CARTESIAN_POINT('Ctrl Pts',(-15.8745380140857,13.0018870987347,
133.900204241411)) ;
#146336=CARTESIAN_POINT('Ctrl Pts',(-15.8156006902136,12.7291797299788,
133.761159559006)) ;
#146337=CARTESIAN_POINT('Ctrl Pts',(-15.7349813594489,12.5061726224373,
133.558781374846)) ;
#146338=CARTESIAN_POINT('Ctrl Pts',(-15.6378228988285,12.3489725905771,
133.308056494779)) ;
#146339=CARTESIAN_POINT('Ctrl Pts',(-15.530157628843,12.2685649990364,133.026676899959)) ;
#146340=CARTESIAN_POINT('Ctrl Pts',(-15.4191690111872,12.2709027590492,
132.735560480177)) ;
#146341=CARTESIAN_POINT('Ctrl Pts',(-15.3118886403359,12.3558100715775,
132.455309412101)) ;
#146342=CARTESIAN_POINT('Ctrl Pts',(-15.2154321019517,12.5172182560686,
132.206663476268)) ;
#146343=CARTESIAN_POINT('Ctrl Pts',(-15.1360069622019,12.743270611073,132.007738327536)) ;
#146344=CARTESIAN_POINT('Ctrl Pts',(-15.0784065694775,13.0180148278647,
131.872581445848)) ;
#146345=CARTESIAN_POINT('Ctrl Pts',(-15.0460718420616,13.3228200342207,
131.811342068092)) ;
#146346=CARTESIAN_POINT('Ctrl Pts',(-15.0407629253236,13.6334362897112,
131.828899103818)) ;
#146347=CARTESIAN_POINT('Ctrl Pts',(-15.0619394460524,13.929416387864,131.923875769177)) ;
#146348=CARTESIAN_POINT('Ctrl Pts',(-15.1073807241388,14.1891570751448,
132.089722319927)) ;
#146349=CARTESIAN_POINT('Ctrl Pts',(-15.173454010653,14.3946402332245,132.315974310693)) ;
#146350=CARTESIAN_POINT('Ctrl Pts',(-15.2539080167936,14.5295569095383,
132.584013104552)) ;
#146351=CARTESIAN_POINT('Ctrl Pts',(-15.3433923457211,14.5858061320267,
132.878694551811)) ;
#146352=CARTESIAN_POINT('Ctrl Pts',(-15.4333868311324,14.5585141684262,
133.174582671032)) ;
#146353=CARTESIAN_POINT('Ctrl Pts',(-15.5178587338625,14.4500372102403,
133.45449302783)) ;
#146354=CARTESIAN_POINT('Ctrl Pts',(-15.5894979700118,14.268202012558,133.696854115771)) ;
#146355=CARTESIAN_POINT('Ctrl Pts',(-15.6427738964284,14.0250734119471,
133.885689485768)) ;
#146356=CARTESIAN_POINT('Ctrl Pts',(-15.6727728261184,13.7389393518604,
134.006480982623)) ;
#146357=CARTESIAN_POINT('Ctrl Pts',(-15.6767371037588,13.4311037036194,
134.051125055907)) ;
#146358=CARTESIAN_POINT('Ctrl Pts',(-15.6539490538312,13.1229020321195,
134.017585741783)) ;
#146359=CARTESIAN_POINT('Ctrl Pts',(-15.6044808421572,12.8333723855065,
133.906452712776)) ;
#146360=CARTESIAN_POINT('Ctrl Pts',(-15.5324157004818,12.5895126789185,
133.72888592348)) ;
#146361=CARTESIAN_POINT('Ctrl Pts',(-15.4410477383866,12.4035404975601,
133.495173240331)) ;
#146362=CARTESIAN_POINT('Ctrl Pts',(-15.3370016478281,12.2914040477839,
133.224285529547)) ;
#146363=CARTESIAN_POINT('Ctrl Pts',(-15.2265724109178,12.259812265838,132.934791476383)) ;
#146364=CARTESIAN_POINT('Ctrl Pts',(-15.1167148533907,12.3118570241587,
132.647062652829)) ;
#146365=CARTESIAN_POINT('Ctrl Pts',(-15.0153503169405,12.4430958843788,
132.383997857726)) ;
#146366=CARTESIAN_POINT('Ctrl Pts',(-14.9282226918438,12.6447072746916,
132.162614685402)) ;
#146367=CARTESIAN_POINT('Ctrl Pts',(-14.8611005268562,12.9030427397014,
131.999762417432)) ;
#146368=CARTESIAN_POINT('Ctrl Pts',(-14.8184323691343,13.1970329557463,
131.90815170385)) ;
#146369=CARTESIAN_POINT('Ctrl Pts',(-14.8021120725842,13.5084313502234,
131.893655409077)) ;
#146370=CARTESIAN_POINT('Ctrl Pts',(-14.8126487298977,13.8121188302543,
131.957427584863)) ;
#146371=CARTESIAN_POINT('Ctrl Pts',(-14.8488131994512,14.0900962513971,
132.096326161093)) ;
#146372=CARTESIAN_POINT('Ctrl Pts',(-14.906849179233,14.31872996458,132.298901194403)) ;
#146373=CARTESIAN_POINT('Ctrl Pts',(-14.9826658905836,14.484422730659,132.553674773777)) ;
#146374=CARTESIAN_POINT('Ctrl Pts',(-15.0687615290781,14.5727758927101,
132.838129202005)) ;
#146375=CARTESIAN_POINT('Ctrl Pts',(-15.1595314097221,14.5796460422286,
133.136442849992)) ;
#146376=CARTESIAN_POINT('Ctrl Pts',(-15.2471499676657,14.5035865487986,
133.425498378262)) ;
#146377=CARTESIAN_POINT('Ctrl Pts',(-15.3249952354103,14.3497062950072,
133.686114882967)) ;
#146378=CARTESIAN_POINT('Ctrl Pts',(-15.3863099770745,14.1291329679128,
133.898413257429)) ;
#146379=CARTESIAN_POINT('Ctrl Pts',(-15.4259580102792,13.8597726326946,
134.047208043984)) ;
#146380=CARTESIAN_POINT('Ctrl Pts',(-15.4408276270026,13.557462341525,134.123830690541)) ;
#146381=CARTESIAN_POINT('Ctrl Pts',(-15.4288290015519,13.2463365194833,
134.121865090828)) ;
#146382=CARTESIAN_POINT('Ctrl Pts',(-15.3900832769036,12.9472973154242,
134.041838296647)) ;
#146383=CARTESIAN_POINT('Ctrl Pts',(-15.3269663434198,12.6832077780023,
133.890488587454)) ;
#146384=CARTESIAN_POINT('Ctrl Pts',(-15.2423563366193,12.4704982394892,
133.676617683217)) ;
#146385=CARTESIAN_POINT('Ctrl Pts',(-15.1429697800888,12.3276823235439,
133.419290281986)) ;
#146386=CARTESIAN_POINT('Ctrl Pts',(-15.034025656949,12.2625925201889,133.13420442183)) ;
#146387=CARTESIAN_POINT('Ctrl Pts',(-14.9234367169736,12.280619224966,132.844183391634)) ;
#146388=CARTESIAN_POINT('Ctrl Pts',(-14.8172926653969,12.3809214756921,
132.567369365397)) ;
#146389=CARTESIAN_POINT('Ctrl Pts',(-14.7236180638936,12.556040128184,132.326867240074)) ;
#146390=CARTESIAN_POINT('Ctrl Pts',(-14.6482354062739,12.7918901581632,
132.13964381325)) ;
#146391=CARTESIAN_POINT('Ctrl Pts',(-14.5951060569914,13.0744209862709,
132.017630257796)) ;
#146392=CARTESIAN_POINT('Ctrl Pts',(-14.5678958064568,13.3812416833702,
131.971242619165)) ;
#146393=CARTESIAN_POINT('Ctrl Pts',(-14.5676629123474,13.6920797161949,
132.003775510376)) ;
#146394=CARTESIAN_POINT('Ctrl Pts',(-14.5937720069054,13.9824941766623,
132.113143701743)) ;
#146395=CARTESIAN_POINT('Ctrl Pts',(-14.6432359699896,14.2323227471641,
132.290628513848)) ;
#146396=CARTESIAN_POINT('Ctrl Pts',(-14.7125811656434,14.4258243482768,
132.526452324439)) ;
#146397=CARTESIAN_POINT('Ctrl Pts',(-14.795259617687,14.5465247223938,132.801035574304)) ;
#146398=CARTESIAN_POINT('Ctrl Pts',(-14.8854602664183,14.5869806833893,
133.097778776266)) ;
#146399=CARTESIAN_POINT('Ctrl Pts',(-14.9747767120066,14.5442058476213,
133.391648023159)) ;
#146400=CARTESIAN_POINT('Ctrl Pts',(-15.0575087952615,14.4209679586328,
133.666531321112)) ;
#146401=CARTESIAN_POINT('Ctrl Pts',(-15.126197252713,14.2257906516459,133.900366785556)) ;
#146402=CARTESIAN_POINT('Ctrl Pts',(-15.1751094293477,13.9741287595616,
134.0762978741)) ;
#146403=CARTESIAN_POINT('Ctrl Pts',(-15.2004336399251,13.6829512293512,
134.183353995983)) ;
#146404=CARTESIAN_POINT('Ctrl Pts',(-15.1993756323757,13.37146650651,134.213520518934)) ;
#146405=CARTESIAN_POINT('Ctrl Pts',(-15.1713543841638,13.0656058260286,
134.164711854186)) ;
#146406=CARTESIAN_POINT('Ctrl Pts',(-15.1177667999354,12.7850334229127,
134.041241823021)) ;
#146407=CARTESIAN_POINT('Ctrl Pts',(-15.0415227466297,12.5496672671412,
133.851637015263)) ;
#146408=CARTESIAN_POINT('Ctrl Pts',(-14.9472330050277,12.3766688304073,
133.6093776058)) ;
#146409=CARTESIAN_POINT('Ctrl Pts',(-14.8412230464008,12.2789529109886,
133.332834468204)) ;
#146410=CARTESIAN_POINT('Ctrl Pts',(-14.7301884575418,12.2634413575716,
133.041638140652)) ;
#146411=CARTESIAN_POINT('Ctrl Pts',(-14.6219272251922,12.3304157181155,
132.758377292415)) ;
#146412=CARTESIAN_POINT('Ctrl Pts',(-14.5219985404227,12.4770344340702,
132.499791442207)) ;
#146413=CARTESIAN_POINT('Ctrl Pts',(-14.438846216414,12.6896430839443,132.289838653687)) ;
#146414=CARTESIAN_POINT('Ctrl Pts',(-14.3761485768327,12.9554492280344,
132.139803286405)) ;
#146415=CARTESIAN_POINT('Ctrl Pts',(-14.3381869562118,13.2546656267019,
132.062005855799)) ;
#146416=CARTESIAN_POINT('Ctrl Pts',(-14.3269455293927,13.5672375771819,
132.062407602021)) ;
#146417=CARTESIAN_POINT('Ctrl Pts',(-14.3425168856217,13.8673528503954,
132.140905544475)) ;
#146418=CARTESIAN_POINT('Ctrl Pts',(-14.3828967515057,14.1367236573279,
132.29196398836)) ;
#146419=CARTESIAN_POINT('Ctrl Pts',(-14.4451848472743,14.3561277006207,
132.507257563492)) ;
#146420=CARTESIAN_POINT('Ctrl Pts',(-14.5227670474163,14.5065131900063,
132.766820448084)) ;
#146421=CARTESIAN_POINT('Ctrl Pts',(-14.6107831313521,14.5806176996537,
133.05713220862)) ;
#146422=CARTESIAN_POINT('Ctrl Pts',(-14.7013079495486,14.5715966835969,
133.354635276761)) ;
#146423=CARTESIAN_POINT('Ctrl Pts',(-14.7879149238724,14.4799160450286,
133.640882829627)) ;
#146424=CARTESIAN_POINT('Ctrl Pts',(-14.8627484547883,14.3130125765193,
133.892550568111)) ;
#146425=CARTESIAN_POINT('Ctrl Pts',(-14.9203410309572,14.0821691302311,
134.093924104667)) ;
#146426=CARTESIAN_POINT('Ctrl Pts',(-14.9556762161135,13.8046644835193,
134.230212081773)) ;
#146427=CARTESIAN_POINT('Ctrl Pts',(-14.9654957367169,13.4979410489725,
134.292173058157)) ;
#146428=CARTESIAN_POINT('Ctrl Pts',(-14.9484649563509,13.1889483563346,
134.275353533116)) ;
#146429=CARTESIAN_POINT('Ctrl Pts',(-14.9048261853835,12.8939178220345,
134.181116548468)) ;
#146430=CARTESIAN_POINT('Ctrl Pts',(-14.8371220940663,12.6378239154038,
134.016474615887)) ;
#146431=CARTESIAN_POINT('Ctrl Pts',(-14.7495889434489,12.4382802078468,
133.793875792288)) ;
#146432=CARTESIAN_POINT('Ctrl Pts',(-14.6480169552468,12.3092349638881,
133.530167877536)) ;
#146433=CARTESIAN_POINT('Ctrl Pts',(-14.5376692614152,12.2595575251469,
133.241117653867)) ;
#146434=CARTESIAN_POINT('Ctrl Pts',(-14.427778786874,12.2934341319413,132.953057165944)) ;
#146435=CARTESIAN_POINT('Ctrl Pts',(-14.3237109603852,12.4080333826879,
132.68220443888)) ;
#146436=CARTESIAN_POINT('Ctrl Pts',(-14.2327451779127,12.5960960403323,
132.449682391364)) ;
#146437=CARTESIAN_POINT('Ctrl Pts',(-14.1611034981059,12.843083593107,132.27352851092)) ;
#146438=CARTESIAN_POINT('Ctrl Pts',(-14.1129483862029,13.1299282656209,
132.165812124441)) ;
#146439=CARTESIAN_POINT('Ctrl Pts',(-14.0906153604259,13.4413370847319,
132.133926329516)) ;
#146440=CARTESIAN_POINT('Ctrl Pts',(-14.095508888872,13.7480777848253,132.181202614268)) ;
#146441=CARTESIAN_POINT('Ctrl Pts',(-14.1262007162312,14.0327532963684,
132.303976693101)) ;
#146442=CARTESIAN_POINT('Ctrl Pts',(-14.1797772693749,14.2736050959338,
132.493548029621)) ;
#146443=CARTESIAN_POINT('Ctrl Pts',(-14.2524010625293,14.4547314296563,
132.739031944661)) ;
#146444=CARTESIAN_POINT('Ctrl Pts',(-14.336638830989,14.5602675742185,133.018049943511)) ;
#146445=CARTESIAN_POINT('Ctrl Pts',(-14.4272467643914,14.5853381801731,
133.315940718168)) ;
#146446=CARTESIAN_POINT('Ctrl Pts',(-14.5161472798392,14.5268295873478,
133.608748133879)) ;
#146447=CARTESIAN_POINT('Ctrl Pts',(-14.5965447904337,14.3893357497607,
133.876742386898)) ;
#146448=CARTESIAN_POINT('Ctrl Pts',(-14.6618705056622,14.1825586684621,
134.100706056936)) ;
#146449=CARTESIAN_POINT('Ctrl Pts',(-14.7067541737627,13.9213687845982,
134.264954864919)) ;
#146450=CARTESIAN_POINT('Ctrl Pts',(-14.7271543963702,13.6242447212575,
134.357704685103)) ;
#146451=CARTESIAN_POINT('Ctrl Pts',(-14.7211456285122,13.3143403284212,
134.373125855975)) ;
#146452=CARTESIAN_POINT('Ctrl Pts',(-14.6877800682829,13.0084389968774,
134.309066553768)) ;
#146453=CARTESIAN_POINT('Ctrl Pts',(-14.6299975192762,12.7371908431784,
134.173086803152)) ;
#146454=CARTESIAN_POINT('Ctrl Pts',(-14.5496928088176,12.5114337629303,
133.971763331707)) ;
#146455=CARTESIAN_POINT('Ctrl Pts',(-14.4529519278489,12.3524149247727,
133.722234690091)) ;
#146456=CARTESIAN_POINT('Ctrl Pts',(-14.3453600058295,12.2696327934899,
133.441110630772)) ;
#146457=CARTESIAN_POINT('Ctrl Pts',(-14.234427034219,12.2697667408868,133.150138706916)) ;
#146458=CARTESIAN_POINT('Ctrl Pts',(-14.1271125200423,12.3522197325102,
132.869734388649)) ;
#146459=CARTESIAN_POINT('Ctrl Pts',(-14.0301995863744,12.5116177862274,
132.619773055426)) ;
#146460=CARTESIAN_POINT('Ctrl Pts',(-13.9501762091569,12.736082772034,132.419111274269)) ;
#146461=CARTESIAN_POINT('Ctrl Pts',(-13.8917651248445,13.0105747690242,
132.281683171717)) ;
#146462=CARTESIAN_POINT('Ctrl Pts',(-13.8588245965078,13.3146279151312,
132.218642076419)) ;
#146463=CARTESIAN_POINT('Ctrl Pts',(-13.8527482583037,13.6243832359542,
132.233854307006)) ;
#146464=CARTESIAN_POINT('Ctrl Pts',(-13.8732412974156,13.9217978697246,
132.326914159419)) ;
#146465=CARTESIAN_POINT('Ctrl Pts',(-13.9179550084861,14.1821018677862,
132.49054999663)) ;
#146466=CARTESIAN_POINT('Ctrl Pts',(-13.9833931661554,14.3894123612741,
132.714916036037)) ;
#146467=CARTESIAN_POINT('Ctrl Pts',(-14.0637817030373,14.5268848445949,
132.982873768876)) ;
#146468=CARTESIAN_POINT('Ctrl Pts',(-14.1528323479007,14.585256166508,133.276178284537)) ;
#146469=CARTESIAN_POINT('Ctrl Pts',(-14.2429398570225,14.5605921317333,
133.572412885749)) ;
#146470=CARTESIAN_POINT('Ctrl Pts',(-14.327783437094,14.4542388415829,133.853450491557)) ;
#146471=CARTESIAN_POINT('Ctrl Pts',(-14.3999222529145,14.2743936202259,
134.0972769669)) ;
#146472=CARTESIAN_POINT('Ctrl Pts',(-14.4539010120162,14.0316377152924,
134.288294641039)) ;
#146473=CARTESIAN_POINT('Ctrl Pts',(-14.4844118562612,13.7487556087195,
134.410315372432)) ;
#146474=CARTESIAN_POINT('Ctrl Pts',(-14.4892042813141,13.4387761357976,
134.457654070306)) ;
#146475=CARTESIAN_POINT('Ctrl Pts',(-14.4671820256302,13.131784657343,134.426188716179)) ;
#146476=CARTESIAN_POINT('Ctrl Pts',(-14.4184322168324,12.8410201909971,
134.317189600133)) ;
#146477=CARTESIAN_POINT('Ctrl Pts',(-14.3471581146507,12.5963886012332,
134.141844320016)) ;
#146478=CARTESIAN_POINT('Ctrl Pts',(-14.2564618620465,12.4083250161853,
133.910052273587)) ;
#146479=CARTESIAN_POINT('Ctrl Pts',(-14.1520011623539,12.2932606214,133.638173291436)) ;
#146480=CARTESIAN_POINT('Ctrl Pts',(-14.0421766856827,12.2596773190563,
133.350284976464)) ;
#146481=CARTESIAN_POINT('Ctrl Pts',(-13.9322527165775,12.3089369873083,
133.062341698944)) ;
#146482=CARTESIAN_POINT('Ctrl Pts',(-13.8301386015647,12.4384179192494,
132.797214281908)) ;
#146483=CARTESIAN_POINT('Ctrl Pts',(-13.7424630213586,12.6389284665683,
132.574292676507)) ;
#146484=CARTESIAN_POINT('Ctrl Pts',(-13.6751976177911,12.8936369055523,
132.410742884719)) ;
#146485=CARTESIAN_POINT('Ctrl Pts',(-13.6313872780528,13.1890353554826,
132.316056077679)) ;
#146486=CARTESIAN_POINT('Ctrl Pts',(-13.6144296986492,13.4997524264947,
132.299631910272)) ;
#146487=CARTESIAN_POINT('Ctrl Pts',(-13.6242379968661,13.8039809535807,
132.36129191884)) ;
#146488=CARTESIAN_POINT('Ctrl Pts',(-13.6595439406371,14.0820722250227,
132.497554900109)) ;
#146489=CARTESIAN_POINT('Ctrl Pts',(-13.7171465091326,14.3130041304952,
132.698959363541)) ;
#146490=CARTESIAN_POINT('Ctrl Pts',(-13.7921690834901,14.4800545558914,
132.951253870289)) ;
#146491=CARTESIAN_POINT('Ctrl Pts',(-13.8782618612207,14.5714592047604,
133.235802806482)) ;
#146492=CARTESIAN_POINT('Ctrl Pts',(-13.9694643431118,14.580498376248,133.535542208868)) ;
#146493=CARTESIAN_POINT('Ctrl Pts',(-14.0568328810788,14.5069052062207,
133.823709965073)) ;
#146494=CARTESIAN_POINT('Ctrl Pts',(-14.1349602526621,14.355702929433,134.085089279489)) ;
#146495=CARTESIAN_POINT('Ctrl Pts',(-14.1969497713178,14.1367618967332,
134.299396492582)) ;
#146496=CARTESIAN_POINT('Ctrl Pts',(-14.237404970337,13.8680692745211,134.450619705146)) ;
#146497=CARTESIAN_POINT('Ctrl Pts',(-14.2529793616564,13.5652241802336,
134.529418842422)) ;
#146498=CARTESIAN_POINT('Ctrl Pts',(-14.2417810472862,13.2558695648544,
134.529599297919)) ;
#146499=CARTESIAN_POINT('Ctrl Pts',(-14.2038516719789,12.9557645621013,
134.451991133453)) ;
#146500=CARTESIAN_POINT('Ctrl Pts',(-14.1412339441975,12.6900041384903,
134.302163095143)) ;
#146501=CARTESIAN_POINT('Ctrl Pts',(-14.0574802284815,12.4761054960812,
134.090679313259)) ;
#146502=CARTESIAN_POINT('Ctrl Pts',(-13.9579371786143,12.330458638013,133.833068527865)) ;
#146503=CARTESIAN_POINT('Ctrl Pts',(-13.8496782688255,12.2634381555471,
133.54982031889)) ;
#146504=CARTESIAN_POINT('Ctrl Pts',(-13.7388026570335,12.2788783725225,
133.259036812535)) ;
#146505=CARTESIAN_POINT('Ctrl Pts',(-13.6325440380496,12.3768660101259,
132.981849454036)) ;
#146506=CARTESIAN_POINT('Ctrl Pts',(-13.5384385408213,12.5495630530058,
132.740061699469)) ;
#146507=CARTESIAN_POINT('Ctrl Pts',(-13.4620222411141,12.7855771799242,
132.550040928112)) ;
#146508=CARTESIAN_POINT('Ctrl Pts',(-13.4085967067531,13.0654345443907,
132.426953066734)) ;
#146509=CARTESIAN_POINT('Ctrl Pts',(-13.3805216983346,13.3720089515071,
132.378066496838)) ;
#146510=CARTESIAN_POINT('Ctrl Pts',(-13.3795024819761,13.6824357040732,
132.408234983439)) ;
#146511=CARTESIAN_POINT('Ctrl Pts',(-13.4047254545112,13.9739144872618,
132.515011531949)) ;
#146512=CARTESIAN_POINT('Ctrl Pts',(-13.4540326672827,14.2268633761364,
132.692297533583)) ;
#146513=CARTESIAN_POINT('Ctrl Pts',(-13.5222172871231,14.4204385567601,
132.924403441781)) ;
#146514=CARTESIAN_POINT('Ctrl Pts',(-13.6053169565128,14.5445800980489,
133.200525150877)) ;
#146515=CARTESIAN_POINT('Ctrl Pts',(-13.69482615905,14.5868220517618,133.495019337852)) ;
#146516=CARTESIAN_POINT('Ctrl Pts',(-13.7844155042831,14.5468039115563,
133.789745744027)) ;
#146517=CARTESIAN_POINT('Ctrl Pts',(-13.8677245925165,14.4251034056979,
134.066432113054)) ;
#146518=CARTESIAN_POINT('Ctrl Pts',(-13.9365735484581,14.2325286559051,
134.300597292436)) ;
#146519=CARTESIAN_POINT('Ctrl Pts',(-13.9862491962028,13.9823226082249,
134.478779895998)) ;
#146520=CARTESIAN_POINT('Ctrl Pts',(-14.0123354158408,13.6900857614276,
134.588264981185)) ;
#146521=CARTESIAN_POINT('Ctrl Pts',(-14.0119899662679,13.3811329933267,
134.620262334553)) ;
#146522=CARTESIAN_POINT('Ctrl Pts',(-13.9847818385877,13.0742211924304,
134.573896287318)) ;
#146523=CARTESIAN_POINT('Ctrl Pts',(-13.9317957915014,12.7922255681548,
134.452228797447)) ;
#146524=CARTESIAN_POINT('Ctrl Pts',(-13.8559061607881,12.5548593941868,
134.263739840746)) ;
#146525=CARTESIAN_POINT('Ctrl Pts',(-13.7621081879575,12.3804086208566,
134.022872111731)) ;
#146526=CARTESIAN_POINT('Ctrl Pts',(-13.6568430418593,12.2809059673708,
133.748352658593)) ;
#146527=CARTESIAN_POINT('Ctrl Pts',(-13.5459745763591,12.2624888540407,
133.457603489706)) ;
#146528=CARTESIAN_POINT('Ctrl Pts',(-13.4369161855102,12.3276777325191,
133.172213886062)) ;
#146529=CARTESIAN_POINT('Ctrl Pts',(-13.3374729301959,12.4707929525642,
132.914754251539)) ;
#146530=CARTESIAN_POINT('Ctrl Pts',(-13.2532224546344,12.6823314867526,
132.701770694391)) ;
#146531=CARTESIAN_POINT('Ctrl Pts',(-13.1897158468007,12.9478032750239,
132.549469198639)) ;
#146532=CARTESIAN_POINT('Ctrl Pts',(-13.1510598607848,13.2466924677811,
132.469674263269)) ;
#146533=CARTESIAN_POINT('Ctrl Pts',(-13.1391280106543,13.5583773879723,
132.467970469312)) ;
#146534=CARTESIAN_POINT('Ctrl Pts',(-13.1538931724907,13.8592557726353,
132.544120545162)) ;
#146535=CARTESIAN_POINT('Ctrl Pts',(-13.1939100913278,14.1306426193177,
132.69425915972)) ;
#146536=CARTESIAN_POINT('Ctrl Pts',(-13.2548897709125,14.3493760513521,
132.905341284647)) ;
#146537=CARTESIAN_POINT('Ctrl Pts',(-13.3326860582841,14.5035317935641,
133.165820676624)) ;
#146538=CARTESIAN_POINT('Ctrl Pts',(-13.4203463467915,14.5795845166173,
133.455011718327)) ;
#146539=CARTESIAN_POINT('Ctrl Pts',(-13.5110703082225,14.5729335427119,
133.753170497346)) ;
#146540=CARTESIAN_POINT('Ctrl Pts',(-13.5975957735246,14.4838964505683,
134.039056609727)) ;
#146541=CARTESIAN_POINT('Ctrl Pts',(-13.6730510545671,14.3187457002778,
134.292624837989)) ;
#146542=CARTESIAN_POINT('Ctrl Pts',(-13.7311388935659,14.0897675242826,
134.495402280048)) ;
#146543=CARTESIAN_POINT('Ctrl Pts',(-13.7671907435101,13.8134082052382,
134.633785843446)) ;
#146544=CARTESIAN_POINT('Ctrl Pts',(-13.7778201049083,13.5073935686165,
134.698088922778)) ;
#146545=CARTESIAN_POINT('Ctrl Pts',(-13.7615250080495,13.1976576575877,
134.683484364323)) ;
#146546=CARTESIAN_POINT('Ctrl Pts',(-13.7187953498613,12.902722923634,134.591795852928)) ;
#146547=CARTESIAN_POINT('Ctrl Pts',(-13.6516732615037,12.6448108187769,
134.428909139399)) ;
#146548=CARTESIAN_POINT('Ctrl Pts',(-13.5648664921481,12.4434495534872,
134.208369317472)) ;
#146549=CARTESIAN_POINT('Ctrl Pts',(-13.4626553121334,12.3113759719957,
133.943100168444)) ;
#146550=CARTESIAN_POINT('Ctrl Pts',(-13.3536253569139,12.2599503304337,
133.65753108676)) ;
#146551=CARTESIAN_POINT('Ctrl Pts',(-13.2427727916244,12.291369325937,133.366928182391)) ;
#146552=CARTESIAN_POINT('Ctrl Pts',(-13.1387408123296,12.4038516063155,
133.096088025424)) ;
#146553=CARTESIAN_POINT('Ctrl Pts',(-13.0475728337221,12.5892626492753,
132.862876992473)) ;
#146554=CARTESIAN_POINT('Ctrl Pts',(-12.9752337296433,12.8342966688913,
132.684656592976)) ;
#146555=CARTESIAN_POINT('Ctrl Pts',(-12.9260719761757,13.122430564087,132.574248236609)) ;
#146556=CARTESIAN_POINT('Ctrl Pts',(-12.903169430825,13.4307504301952,132.540394077624)) ;
#146557=CARTESIAN_POINT('Ctrl Pts',(-12.9071698221294,13.7394115406098,
132.585230287027)) ;
#146558=CARTESIAN_POINT('Ctrl Pts',(-12.9371825249084,14.0250582572476,
132.70601678198)) ;
#146559=CARTESIAN_POINT('Ctrl Pts',(-12.9902636541603,14.2676857637035,
132.894194946137)) ;
#146560=CARTESIAN_POINT('Ctrl Pts',(-13.0621016867333,14.4501343866895,
133.137238551309)) ;
#146561=CARTESIAN_POINT('Ctrl Pts',(-13.1464951100618,14.5585281733049,
133.416884073386)) ;
#146562=CARTESIAN_POINT('Ctrl Pts',(-13.2367905862396,14.5857500263022,
133.713765250072)) ;
#146563=CARTESIAN_POINT('Ctrl Pts',(-13.3259831356628,14.5296138137444,
134.00748135074)) ;
#146564=CARTESIAN_POINT('Ctrl Pts',(-13.4067107227604,14.3940563365778,
134.276446490129)) ;
#146565=CARTESIAN_POINT('Ctrl Pts',(-13.4723758800565,14.1896705870724,
134.501311639645)) ;
#146566=CARTESIAN_POINT('Ctrl Pts',(-13.5180007326056,13.929679500594,134.667754972924)) ;
#146567=CARTESIAN_POINT('Ctrl Pts',(-13.5391833761276,13.6325613008054,
134.762866814829)) ;
#146568=CARTESIAN_POINT('Ctrl Pts',(-13.5338310344752,13.3229079041448,
134.780193273664)) ;
#146569=CARTESIAN_POINT('Ctrl Pts',(-13.5015813505085,13.0185266052724,
134.719157623872)) ;
#146570=CARTESIAN_POINT('Ctrl Pts',(-13.4440778905347,12.7436673209471,
134.584275396389)) ;
#146571=CARTESIAN_POINT('Ctrl Pts',(-13.364164023709,12.5164978313935,134.384108889428)) ;
#146572=CARTESIAN_POINT('Ctrl Pts',(-13.2681841114513,12.3560839841268,
134.136678866392)) ;
#146573=CARTESIAN_POINT('Ctrl Pts',(-13.1607863258833,12.2708854639731,
133.856129718307)) ;
#146574=CARTESIAN_POINT('Ctrl Pts',(-13.0499975081774,12.2685612257957,
133.565537388716)) ;
#146575=CARTESIAN_POINT('Ctrl Pts',(-12.9422815963831,12.3486010166685,
133.28401225927)) ;
#146576=CARTESIAN_POINT('Ctrl Pts',(-12.8446122552014,12.5069431442139,
133.031987927892)) ;
#146577=CARTESIAN_POINT('Ctrl Pts',(-12.7645613027564,12.7284060361604,
132.831033985649)) ;
#146578=CARTESIAN_POINT('Ctrl Pts',(-12.705253017919,13.0024846524795,132.691088883789)) ;
#146579=CARTESIAN_POINT('Ctrl Pts',(-12.6716419222305,13.3053157268251,
132.6260084913)) ;
#146580=CARTESIAN_POINT('Ctrl Pts',(-12.6647810266749,13.6156287863426,
132.638985809996)) ;
#146581=CARTESIAN_POINT('Ctrl Pts',(-12.6843936920298,13.9128850712382,
132.729361876897)) ;
#146582=CARTESIAN_POINT('Ctrl Pts',(-12.7288341766348,14.1766185876755,
132.892474897501)) ;
#146583=CARTESIAN_POINT('Ctrl Pts',(-12.7937162436498,14.3847399014371,
133.115126688338)) ;
#146584=CARTESIAN_POINT('Ctrl Pts',(-12.8734691079153,14.5238361204557,
133.381113923067)) ;
#146585=CARTESIAN_POINT('Ctrl Pts',(-12.9622495766178,14.5847743037998,
133.673586233755)) ;
#146586=CARTESIAN_POINT('Ctrl Pts',(-13.0527820859063,14.562330930931,133.971202261872)) ;
#146587=CARTESIAN_POINT('Ctrl Pts',(-13.1377615990323,14.4584177990408,
134.252575475658)) ;
#146588=CARTESIAN_POINT('Ctrl Pts',(-13.2105950760868,14.2791868588028,
134.498607925464)) ;
#146589=CARTESIAN_POINT('Ctrl Pts',(-13.2645059669396,14.0415186925473,
134.688953563355)) ;
#146590=CARTESIAN_POINT('Ctrl Pts',(-13.2961690615346,13.7564325224017,
134.814741376284)) ;
#146591=CARTESIAN_POINT('Ctrl Pts',(-13.3017064519511,13.4495648486799,
134.863943731619)) ;
#146592=CARTESIAN_POINT('Ctrl Pts',(-13.2802760759038,13.1394167822153,
134.83453108885)) ;
#146593=CARTESIAN_POINT('Ctrl Pts',(-13.2328043241826,12.8508801279426,
134.728890639548)) ;
#146594=CARTESIAN_POINT('Ctrl Pts',(-13.1616530962339,12.6022770183791,
134.554205749892)) ;
#146595=CARTESIAN_POINT('Ctrl Pts',(-13.0714541468405,12.4127865792607,
134.323823666599)) ;
#146596=CARTESIAN_POINT('Ctrl Pts',(-12.9673285301535,12.2953916608247,
134.052917908426)) ;
#146597=CARTESIAN_POINT('Ctrl Pts',(-12.8573500994989,12.2594835078991,
133.764648208685)) ;
#146598=CARTESIAN_POINT('Ctrl Pts',(-12.7475293975293,12.3065006928956,
133.476944904768)) ;
#146599=CARTESIAN_POINT('Ctrl Pts',(-12.6453580244396,12.4331949975966,
133.211553226454)) ;
#146600=CARTESIAN_POINT('Ctrl Pts',(-12.5568504774939,12.6325251245457,
132.986323708861)) ;
#146601=CARTESIAN_POINT('Ctrl Pts',(-12.4890879876667,12.8854154202419,
132.821256063685)) ;
#146602=CARTESIAN_POINT('Ctrl Pts',(-12.4444998174266,13.1803567120122,
132.724340428263)) ;
#146603=CARTESIAN_POINT('Ctrl Pts',(-12.4267857836901,13.4893561619414,
132.705540842095)) ;
#146604=CARTESIAN_POINT('Ctrl Pts',(-12.4357494783633,13.7954471105094,
132.764878099224)) ;
#146605=CARTESIAN_POINT('Ctrl Pts',(-12.470514760125,14.0751705649909,132.899636718351)) ;
#146606=CARTESIAN_POINT('Ctrl Pts',(-12.5273949578635,14.3069080842483,
133.098834382941)) ;
#146607=CARTESIAN_POINT('Ctrl Pts',(-12.6018932112712,14.4762413340772,
133.349575995276)) ;
#146608=CARTESIAN_POINT('Ctrl Pts',(-12.6884680140324,14.5702449830263,
133.635795840671)) ;
#146609=CARTESIAN_POINT('Ctrl Pts',(-12.7787954726246,14.5813885604022,
133.932662954814)) ;
#146610=CARTESIAN_POINT('Ctrl Pts',(-12.8668280999648,14.5100796553899,
134.222948212301)) ;
#146611=CARTESIAN_POINT('Ctrl Pts',(-12.9454272270282,14.3602444697485,
134.48577132055)) ;
#146612=CARTESIAN_POINT('Ctrl Pts',(-13.0077584665022,14.1432531479422,
134.701009749057)) ;
#146613=CARTESIAN_POINT('Ctrl Pts',(-13.04871586247,13.8766589305714,134.853588406275)) ;
#146614=CARTESIAN_POINT('Ctrl Pts',(-13.0651171404783,13.575471110015,134.934700187327)) ;
#146615=CARTESIAN_POINT('Ctrl Pts',(-13.0547234569409,13.2645667872771,
134.937392906819)) ;
#146616=CARTESIAN_POINT('Ctrl Pts',(-13.0173984270287,12.9634276879521,
134.861599179382)) ;
#146617=CARTESIAN_POINT('Ctrl Pts',(-12.9556055647511,12.6972348288673,
134.714086108156)) ;
#146618=CARTESIAN_POINT('Ctrl Pts',(-12.8725122568232,12.4817230037899,
134.504497176081)) ;
#146619=CARTESIAN_POINT('Ctrl Pts',(-12.773428134007,12.3338051645045,134.248207978296)) ;
#146620=CARTESIAN_POINT('Ctrl Pts',(-12.664997671945,12.2641455947444,133.964564222402)) ;
#146621=CARTESIAN_POINT('Ctrl Pts',(-12.5541644274789,12.2773535863406,
133.673882486229)) ;
#146622=CARTESIAN_POINT('Ctrl Pts',(-12.4479133266097,12.3726335000392,
133.396633128579)) ;
#146623=CARTESIAN_POINT('Ctrl Pts',(-12.3532329844408,12.5434758841393,
133.153213940141)) ;
#146624=CARTESIAN_POINT('Ctrl Pts',(-12.2764208543176,12.7769498129424,
132.961924438896)) ;
#146625=CARTESIAN_POINT('Ctrl Pts',(-12.2219612543097,13.0568800238177,
132.835964380683)) ;
#146626=CARTESIAN_POINT('Ctrl Pts',(-12.1931492705949,13.3636449854545,
132.784985244105)) ;
#146627=CARTESIAN_POINT('Ctrl Pts',(-12.1913843931622,13.6733774781512,
132.812881465914)) ;
#146628=CARTESIAN_POINT('Ctrl Pts',(-12.2157901192583,13.9654381108949,
132.917236471078)) ;
#146629=CARTESIAN_POINT('Ctrl Pts',(-12.2644884683387,14.2203012801684,
133.092791679479)) ;
#146630=CARTESIAN_POINT('Ctrl Pts',(-12.3323691648357,14.4159470499748,
133.324078571007)) ;
#146631=CARTESIAN_POINT('Ctrl Pts',(-12.4146312012186,14.541694367896,133.597549977849)) ;
#146632=CARTESIAN_POINT('Ctrl Pts',(-12.504384005875,14.5869018897487,133.892893860253)) ;
#146633=CARTESIAN_POINT('Ctrl Pts',(-12.5942025143602,14.5489491309812,
134.188340585277)) ;
#146634=CARTESIAN_POINT('Ctrl Pts',(-12.6775333194475,14.4300240468882,
134.464972796832)) ;
#146635=CARTESIAN_POINT('Ctrl Pts',(-12.7471511772361,14.2387296194583,
134.701508328912)) ;
#146636=CARTESIAN_POINT('Ctrl Pts',(-12.7973346677689,13.9899468992174,
134.881150877303)) ;
#146637=CARTESIAN_POINT('Ctrl Pts',(-12.8240718619797,13.7002922296482,
134.992355286073)) ;
#146638=CARTESIAN_POINT('Ctrl Pts',(-12.8246776599493,13.3909003011237,
135.027208892331)) ;
#146639=CARTESIAN_POINT('Ctrl Pts',(-12.7980515837342,13.0819914193172,
134.982715951971)) ;
#146640=CARTESIAN_POINT('Ctrl Pts',(-12.7458845974443,12.8000707089261,
134.863325630578)) ;
#146641=CARTESIAN_POINT('Ctrl Pts',(-12.6708702798026,12.561613461146,134.677305827493)) ;
#146642=CARTESIAN_POINT('Ctrl Pts',(-12.5773543002011,12.3844498728761,
134.437337291221)) ;
#146643=CARTESIAN_POINT('Ctrl Pts',(-12.471806174944,12.2824628123426,134.162150550627)) ;
#146644=CARTESIAN_POINT('Ctrl Pts',(-12.3615665234835,12.2618989630133,
133.873062538303)) ;
#146645=CARTESIAN_POINT('Ctrl Pts',(-12.2522093017518,12.3245801672036,
133.586841008912)) ;
#146646=CARTESIAN_POINT('Ctrl Pts',(-12.1524030524764,12.4655890286878,
133.328320986593)) ;
#146647=CARTESIAN_POINT('Ctrl Pts',(-12.0676400812886,12.6753258983896,
133.113838294116)) ;
#146648=CARTESIAN_POINT('Ctrl Pts',(-12.0035262345311,12.9389696147355,
132.959703405746)) ;
#146649=CARTESIAN_POINT('Ctrl Pts',(-11.9640514725537,13.2377442398154,
132.877585546536)) ;
#146650=CARTESIAN_POINT('Ctrl Pts',(-11.951288825654,13.5478078732814,132.87328298619)) ;
#146651=CARTESIAN_POINT('Ctrl Pts',(-11.9653467927663,13.8515136096922,
132.947613389739)) ;
#146652=CARTESIAN_POINT('Ctrl Pts',(-12.0046007635559,14.1231097969316,
133.095406436556)) ;
#146653=CARTESIAN_POINT('Ctrl Pts',(-12.0651067843966,14.3439547255393,
133.305165205202)) ;
#146654=CARTESIAN_POINT('Ctrl Pts',(-12.1423042997912,14.4998917409251,
133.563806490907)) ;
#146655=CARTESIAN_POINT('Ctrl Pts',(-12.2300647068386,14.5786386561727,
133.853407609955)) ;
#146656=CARTESIAN_POINT('Ctrl Pts',(-12.3207510678068,14.574267489829,134.151433421108)) ;
#146657=CARTESIAN_POINT('Ctrl Pts',(-12.4075572935563,14.4873446647109,
134.438170951734)) ;
#146658=CARTESIAN_POINT('Ctrl Pts',(-12.4831747499324,14.3247913257021,
134.692103132489)) ;
#146659=CARTESIAN_POINT('Ctrl Pts',(-12.542042439971,14.0970301472897,134.897242195035)) ;
#146660=CARTESIAN_POINT('Ctrl Pts',(-12.5788106537289,13.820492300365,135.037850166732)) ;
#146661=CARTESIAN_POINT('Ctrl Pts',(-12.5900817230675,13.5164548784845,
135.103861743899)) ;
#146662=CARTESIAN_POINT('Ctrl Pts',(-12.5745635456089,13.2060699162722,
135.091583899804)) ;
#146663=CARTESIAN_POINT('Ctrl Pts',(-12.5324969640781,12.9102232065258,
135.001850755175)) ;
#146664=CARTESIAN_POINT('Ctrl Pts',(-12.4658520839193,12.6507291243944,
134.840407336644)) ;
#146665=CARTESIAN_POINT('Ctrl Pts',(-12.3798223962499,12.4485585440169,
134.622012614771)) ;
#146666=CARTESIAN_POINT('Ctrl Pts',(-12.2785035906128,12.3145373722517,
134.359188397339)) ;
#146667=CARTESIAN_POINT('Ctrl Pts',(-12.1689761661125,12.2601564021124,
134.072361071585)) ;
#146668=CARTESIAN_POINT('Ctrl Pts',(-12.0580855205296,12.2893926148143,
133.781636394683)) ;
#146669=CARTESIAN_POINT('Ctrl Pts',(-11.9537967692143,12.3994366791386,
133.510032588238)) ;
#146670=CARTESIAN_POINT('Ctrl Pts',(-11.8618106924454,12.5839727255082,
133.274581017316)) ;
#146671=CARTESIAN_POINT('Ctrl Pts',(-11.7892711806775,12.8264920327129,
133.095617229562)) ;
#146672=CARTESIAN_POINT('Ctrl Pts',(-11.7392658398382,13.1141225858941,
132.982797082773)) ;
#146673=CARTESIAN_POINT('Ctrl Pts',(-11.7235540209465,13.3194871424456,
132.958938670686)) ;
#146674=CARTESIAN_POINT('Ctrl Pts',(-11.7201408679865,13.4222384841719,
132.959988719826)) ;
#146675=CARTESIAN_POINT('Ctrl Pts',(-33.3012851433477,13.1368456608817,
127.965137779698)) ;
#146676=CARTESIAN_POINT('Ctrl Pts',(-33.3005108918432,13.1302434176427,
127.963606955475)) ;
#146677=CARTESIAN_POINT('Ctrl Pts',(-33.2878768464891,13.0249710001428,
127.93838217985)) ;
#146678=CARTESIAN_POINT('Ctrl Pts',(-33.253359927881,12.826301888656,127.860524464141)) ;
#146679=CARTESIAN_POINT('Ctrl Pts',(-33.180558749092,12.5833995163819,127.680876334219)) ;
#146680=CARTESIAN_POINT('Ctrl Pts',(-33.0890149852688,12.3996267668574,
127.446559868317)) ;
#146681=CARTESIAN_POINT('Ctrl Pts',(-32.9840141902935,12.289073168245,127.173099510327)) ;
#146682=CARTESIAN_POINT('Ctrl Pts',(-32.8740536137075,12.2602312941192,
126.884806111823)) ;
#146683=CARTESIAN_POINT('Ctrl Pts',(-32.7642172899274,12.3144254424815,
126.597172510079)) ;
#146684=CARTESIAN_POINT('Ctrl Pts',(-32.6630373208337,12.4480642715863,
126.334692293817)) ;
#146685=CARTESIAN_POINT('Ctrl Pts',(-32.576446271887,12.6516399513856,126.114881618259)) ;
#146686=CARTESIAN_POINT('Ctrl Pts',(-32.5101373823508,12.9104452496318,
125.954300029618)) ;
#146687=CARTESIAN_POINT('Ctrl Pts',(-32.4680947198103,13.2058492015505,
125.864596954978)) ;
#146688=CARTESIAN_POINT('Ctrl Pts',(-32.4525008094708,13.5166184921212,
125.852133747766)) ;
#146689=CARTESIAN_POINT('Ctrl Pts',(-32.4639876735504,13.8224100223415,
125.918979463408)) ;
#146690=CARTESIAN_POINT('Ctrl Pts',(-32.5006141983944,14.0967865008827,
126.058936460803)) ;
#146691=CARTESIAN_POINT('Ctrl Pts',(-32.5593185399482,14.3244562986112,
126.263555841175)) ;
#146692=CARTESIAN_POINT('Ctrl Pts',(-32.6351145538659,14.4874741997871,
126.518089823437)) ;
#146693=CARTESIAN_POINT('Ctrl Pts',(-32.7220896777706,14.5744204937736,
126.805378368018)) ;
#146694=CARTESIAN_POINT('Ctrl Pts',(-32.8128052621322,14.5784621737365,
127.10350123506)) ;
#146695=CARTESIAN_POINT('Ctrl Pts',(-32.900132936634,14.5000469778991,127.391677525357)) ;
#146696=CARTESIAN_POINT('Ctrl Pts',(-32.977330701875,14.3445727249932,127.650295149581)) ;
#146697=CARTESIAN_POINT('Ctrl Pts',(-33.0381556098337,14.122833835347,127.861131305989)) ;
#146698=CARTESIAN_POINT('Ctrl Pts',(-33.0773675715877,13.8501516984393,
128.008903812172)) ;
#146699=CARTESIAN_POINT('Ctrl Pts',(-33.0913163097499,13.5490423779197,
128.082630492233)) ;
#146700=CARTESIAN_POINT('Ctrl Pts',(-33.0786099195809,13.2374717045801,
128.078653893675)) ;
#146701=CARTESIAN_POINT('Ctrl Pts',(-33.0390139547928,12.9386844676289,
127.996192116606)) ;
#146702=CARTESIAN_POINT('Ctrl Pts',(-32.975229814111,12.6761377246457,127.842873877758)) ;
#146703=CARTESIAN_POINT('Ctrl Pts',(-32.8903638726636,12.4657586790897,
127.628156905795)) ;
#146704=CARTESIAN_POINT('Ctrl Pts',(-32.7904652117052,12.3246285674056,
127.369395546857)) ;
#146705=CARTESIAN_POINT('Ctrl Pts',(-32.6811498208371,12.2619062239342,
127.083285478092)) ;
#146706=CARTESIAN_POINT('Ctrl Pts',(-32.5707291608164,12.282438835861,126.793720932159)) ;
#146707=CARTESIAN_POINT('Ctrl Pts',(-32.4649957249968,12.3848777571664,
126.518059092902)) ;
#146708=CARTESIAN_POINT('Ctrl Pts',(-32.3718774118045,12.5614991790326,
126.279126097839)) ;
#146709=CARTESIAN_POINT('Ctrl Pts',(-32.2967868140066,12.7995868191894,
126.092866229788)) ;
#146710=CARTESIAN_POINT('Ctrl Pts',(-32.2443216753795,13.084029998422,125.972880573089)) ;
#146711=CARTESIAN_POINT('Ctrl Pts',(-32.2180641227937,13.3899587273314,
125.929135151855)) ;
#146712=CARTESIAN_POINT('Ctrl Pts',(-32.2184913394978,13.6996411393276,
125.963497562112)) ;
#146713=CARTESIAN_POINT('Ctrl Pts',(-32.2453325092191,13.9903747350237,
126.075123804051)) ;
#146714=CARTESIAN_POINT('Ctrl Pts',(-32.2956569729903,14.2393240390192,
126.255222855766)) ;
#146715=CARTESIAN_POINT('Ctrl Pts',(-32.3650841831038,14.429840029191,126.4910956906)) ;
#146716=CARTESIAN_POINT('Ctrl Pts',(-32.448163738453,14.5487685207819,126.766909226846)) ;
#146717=CARTESIAN_POINT('Ctrl Pts',(-32.5383659554756,14.5869290462078,
127.063619096291)) ;
#146718=CARTESIAN_POINT('Ctrl Pts',(-32.6278128226021,14.5417666879112,
127.357958778643)) ;
#146719=CARTESIAN_POINT('Ctrl Pts',(-32.7101561099796,14.4163781206347,
127.631674948744)) ;
#146720=CARTESIAN_POINT('Ctrl Pts',(-32.7783498364979,14.2194053236093,
127.864061771658)) ;
#146721=CARTESIAN_POINT('Ctrl Pts',(-32.8266393254659,13.9666437025949,
128.038144830637)) ;
#146722=CARTESIAN_POINT('Ctrl Pts',(-32.851292510915,13.6737230311142,128.143343661379)) ;
#146723=CARTESIAN_POINT('Ctrl Pts',(-32.8494473020655,13.3629183159293,
128.171112807256)) ;
#146724=CARTESIAN_POINT('Ctrl Pts',(-32.8206607882665,13.0570541461369,
128.120117610136)) ;
#146725=CARTESIAN_POINT('Ctrl Pts',(-32.7663361849904,12.7772474401736,
127.994519431102)) ;
#146726=CARTESIAN_POINT('Ctrl Pts',(-32.6890886758744,12.542768054334,127.802123885512)) ;
#146727=CARTESIAN_POINT('Ctrl Pts',(-32.5949608164813,12.3730788461159,
127.560114935571)) ;
#146728=CARTESIAN_POINT('Ctrl Pts',(-32.4886545346452,12.2773830517675,
127.282736009967)) ;
#146729=CARTESIAN_POINT('Ctrl Pts',(-32.3777178343667,12.2641121727855,
126.991780273813)) ;
#146730=CARTESIAN_POINT('Ctrl Pts',(-32.269276455156,12.3337583329821,126.708108351852)) ;
#146731=CARTESIAN_POINT('Ctrl Pts',(-32.1703548633399,12.4813160749921,
126.452235712459)) ;
#146732=CARTESIAN_POINT('Ctrl Pts',(-32.0871433542004,12.6966779854676,
126.242314410242)) ;
#146733=CARTESIAN_POINT('Ctrl Pts',(-32.0251441770006,12.964058481658,126.094337296347)) ;
#146734=CARTESIAN_POINT('Ctrl Pts',(-31.9880271005956,13.2633621106785,
126.01894761863)) ;
#146735=CARTESIAN_POINT('Ctrl Pts',(-31.9774841904215,13.5752568041736,
126.021313511474)) ;
#146736=CARTESIAN_POINT('Ctrl Pts',(-31.9939116345013,13.8766502651513,
126.102521569776)) ;
#146737=CARTESIAN_POINT('Ctrl Pts',(-32.0349700208106,14.1438626179913,
126.255472982178)) ;
#146738=CARTESIAN_POINT('Ctrl Pts',(-32.0975480361989,14.3611558339141,
126.471516188421)) ;
#146739=CARTESIAN_POINT('Ctrl Pts',(-32.1760316525525,14.5102070990302,
126.733925687538)) ;
#146740=CARTESIAN_POINT('Ctrl Pts',(-32.2636499274558,14.5813677878946,
127.022848150248)) ;
#146741=CARTESIAN_POINT('Ctrl Pts',(-32.3544916008583,14.5701315008181,
127.321407441068)) ;
#146742=CARTESIAN_POINT('Ctrl Pts',(-32.4408443777509,14.4759919036324,
127.606902737038)) ;
#146743=CARTESIAN_POINT('Ctrl Pts',(-32.5153098957686,14.3066892752371,
127.857540673623)) ;
#146744=CARTESIAN_POINT('Ctrl Pts',(-32.572093511354,14.0751878826871,128.056411954729)) ;
#146745=CARTESIAN_POINT('Ctrl Pts',(-32.606801906154,13.7962286869884,128.19092493514)) ;
#146746=CARTESIAN_POINT('Ctrl Pts',(-32.6159392974398,13.4897393053989,
128.250814127221)) ;
#146747=CARTESIAN_POINT('Ctrl Pts',(-32.5978520725212,13.1781056984616,
128.231218495251)) ;
#146748=CARTESIAN_POINT('Ctrl Pts',(-32.5538717207945,12.8871394706553,
128.135620981617)) ;
#146749=CARTESIAN_POINT('Ctrl Pts',(-32.4854748637565,12.6313543123433,
127.969059162825)) ;
#146750=CARTESIAN_POINT('Ctrl Pts',(-32.3972131808472,12.4333423882355,
127.744400910633)) ;
#146751=CARTESIAN_POINT('Ctrl Pts',(-32.2954852260653,12.3067788270204,
127.480184029957)) ;
#146752=CARTESIAN_POINT('Ctrl Pts',(-32.1851063871179,12.2592790115486,
127.191016833271)) ;
#146753=CARTESIAN_POINT('Ctrl Pts',(-32.0747522042955,12.2958890743791,
126.901769496605)) ;
#146754=CARTESIAN_POINT('Ctrl Pts',(-31.9714548460177,12.412515962942,126.633025776648)) ;
#146755=CARTESIAN_POINT('Ctrl Pts',(-31.8811186931709,12.6017795206287,
126.402264650772)) ;
#146756=CARTESIAN_POINT('Ctrl Pts',(-31.8098352699652,12.850882040149,126.227256401551)) ;
#146757=CARTESIAN_POINT('Ctrl Pts',(-31.762405072303,13.1389626258658,126.121689692541)) ;
#146758=CARTESIAN_POINT('Ctrl Pts',(-31.7408679606482,13.4502019142914,
126.092079042597)) ;
#146759=CARTESIAN_POINT('Ctrl Pts',(-31.7465832117125,13.7571545177325,
126.141825730537)) ;
#146760=CARTESIAN_POINT('Ctrl Pts',(-31.7778345667064,14.0399279671086,
126.266112338252)) ;
#146761=CARTESIAN_POINT('Ctrl Pts',(-31.832377419942,14.2804627439869,126.458703858811)) ;
#146762=CARTESIAN_POINT('Ctrl Pts',(-31.9047636968708,14.4580430421026,
126.703179136283)) ;
#146763=CARTESIAN_POINT('Ctrl Pts',(-31.9898069250853,14.5623041816762,
126.984785548002)) ;
#146764=CARTESIAN_POINT('Ctrl Pts',(-32.0801395493773,14.5848738304735,
127.281737987156)) ;
#146765=CARTESIAN_POINT('Ctrl Pts',(-32.1694325535098,14.5236285286568,
127.575900885035)) ;
#146766=CARTESIAN_POINT('Ctrl Pts',(-32.2490892414091,14.3842858734187,
127.841584547318)) ;
#146767=CARTESIAN_POINT('Ctrl Pts',(-32.3139443197535,14.176003666528,128.064165461533)) ;
#146768=CARTESIAN_POINT('Ctrl Pts',(-32.3582858943054,13.9123645540699,
128.226961175517)) ;
#146769=CARTESIAN_POINT('Ctrl Pts',(-32.3778469050749,13.6155079184588,
128.317141856664)) ;
#146770=CARTESIAN_POINT('Ctrl Pts',(-32.3710005417205,13.3048786639477,
128.330191354686)) ;
#146771=CARTESIAN_POINT('Ctrl Pts',(-32.337151787263,13.0013158611206,128.264513177756)) ;
#146772=CARTESIAN_POINT('Ctrl Pts',(-32.2782558550222,12.7290184859203,
128.125547347738)) ;
#146773=CARTESIAN_POINT('Ctrl Pts',(-32.1975975430178,12.5059453059748,
127.923067950598)) ;
#146774=CARTESIAN_POINT('Ctrl Pts',(-32.1004419981188,12.3489356704195,
127.672343005709)) ;
#146775=CARTESIAN_POINT('Ctrl Pts',(-31.9930053142448,12.2685725679141,
127.391562275537)) ;
#146776=CARTESIAN_POINT('Ctrl Pts',(-31.8816137190197,12.2709800275436,
127.099390481669)) ;
#146777=CARTESIAN_POINT('Ctrl Pts',(-31.7746039123214,12.3558597307768,
126.819849151034)) ;
#146778=CARTESIAN_POINT('Ctrl Pts',(-31.6780754812207,12.5173148963124,
126.571016266393)) ;
#146779=CARTESIAN_POINT('Ctrl Pts',(-31.5986036870283,12.7436533200346,
126.371982999436)) ;
#146780=CARTESIAN_POINT('Ctrl Pts',(-31.5410722847427,13.018439069694,126.237023225013)) ;
#146781=CARTESIAN_POINT('Ctrl Pts',(-31.5088077865552,13.3224259013371,
126.175900279904)) ;
#146782=CARTESIAN_POINT('Ctrl Pts',(-31.5034619367311,13.6337496474671,
126.193425485829)) ;
#146783=CARTESIAN_POINT('Ctrl Pts',(-31.5246981020183,13.9298381651934,
126.288591098426)) ;
#146784=CARTESIAN_POINT('Ctrl Pts',(-31.5701771718773,14.1894306031692,
126.454544471721)) ;
#146785=CARTESIAN_POINT('Ctrl Pts',(-31.6360906022642,14.3944757405405,
126.680250797952)) ;
#146786=CARTESIAN_POINT('Ctrl Pts',(-31.7166218889976,14.5294751420936,
126.948550384764)) ;
#146787=CARTESIAN_POINT('Ctrl Pts',(-31.8056980992989,14.5857784683659,
127.241889657182)) ;
#146788=CARTESIAN_POINT('Ctrl Pts',(-31.8962806353445,14.5584757984426,
127.539713151438)) ;
#146789=CARTESIAN_POINT('Ctrl Pts',(-31.9806081664582,14.4499269528594,
127.819149771317)) ;
#146790=CARTESIAN_POINT('Ctrl Pts',(-32.0523166133892,14.2678362445854,
128.061754335213)) ;
#146791=CARTESIAN_POINT('Ctrl Pts',(-32.1054370338036,14.0251814638135,
128.250058329836)) ;
#146792=CARTESIAN_POINT('Ctrl Pts',(-32.1354437565122,13.7395989389894,
128.370820351111)) ;
#146793=CARTESIAN_POINT('Ctrl Pts',(-32.1394815178705,13.4312396305714,
128.415735091465)) ;
#146794=CARTESIAN_POINT('Ctrl Pts',(-32.1165830014567,13.122549732562,128.38193137299)) ;
#146795=CARTESIAN_POINT('Ctrl Pts',(-32.0674362918147,12.8344723669187,
128.271558952154)) ;
#146796=CARTESIAN_POINT('Ctrl Pts',(-31.9951154000811,12.5894057801397,
128.093391835837)) ;
#146797=CARTESIAN_POINT('Ctrl Pts',(-31.9039296777277,12.403866957567,127.860139162014)) ;
#146798=CARTESIAN_POINT('Ctrl Pts',(-31.7997673665532,12.2913271425025,
127.588958580803)) ;
#146799=CARTESIAN_POINT('Ctrl Pts',(-31.6890195332233,12.2598830910493,
127.298627363114)) ;
#146800=CARTESIAN_POINT('Ctrl Pts',(-31.5796091120672,12.3117248733074,
127.012068699769)) ;
#146801=CARTESIAN_POINT('Ctrl Pts',(-31.4779216841838,12.443258179484,126.748161772403)) ;
#146802=CARTESIAN_POINT('Ctrl Pts',(-31.3909668215143,12.6447768173015,
126.527237872634)) ;
#146803=CARTESIAN_POINT('Ctrl Pts',(-31.3239965485428,12.9020426575426,
126.364712331942)) ;
#146804=CARTESIAN_POINT('Ctrl Pts',(-31.2811636319815,13.1969220375029,
126.272729427645)) ;
#146805=CARTESIAN_POINT('Ctrl Pts',(-31.2647925939637,13.5073633530841,
126.257975466901)) ;
#146806=CARTESIAN_POINT('Ctrl Pts',(-31.2754796646211,13.8135027955519,
126.322467658605)) ;
#146807=CARTESIAN_POINT('Ctrl Pts',(-31.3113409517686,14.0890634485619,
126.460181362196)) ;
#146808=CARTESIAN_POINT('Ctrl Pts',(-31.3697525249587,14.3192684868255,
126.664089287873)) ;
#146809=CARTESIAN_POINT('Ctrl Pts',(-31.444870150607,14.4835637589644,126.916510315013)) ;
#146810=CARTESIAN_POINT('Ctrl Pts',(-31.5316044126137,14.5730188127273,
127.203099079401)) ;
#146811=CARTESIAN_POINT('Ctrl Pts',(-31.6223288461193,14.57959678794,127.50125169877)) ;
#146812=CARTESIAN_POINT('Ctrl Pts',(-31.7100305460252,14.5032854042053,
127.79059470504)) ;
#146813=CARTESIAN_POINT('Ctrl Pts',(-31.7875405915815,14.3501151902807,
128.050081809365)) ;
#146814=CARTESIAN_POINT('Ctrl Pts',(-31.8490600583958,14.1289952661381,
128.2630780679)) ;
#146815=CARTESIAN_POINT('Ctrl Pts',(-31.8886334301929,13.8600884343622,
128.411594339113)) ;
#146816=CARTESIAN_POINT('Ctrl Pts',(-31.9035590805538,13.5571076942101,
128.48845671365)) ;
#146817=CARTESIAN_POINT('Ctrl Pts',(-31.891490451461,13.2461441401465,128.486272087745)) ;
#146818=CARTESIAN_POINT('Ctrl Pts',(-31.8528844195338,12.9474784920459,
128.406597920553)) ;
#146819=CARTESIAN_POINT('Ctrl Pts',(-31.7891993797209,12.6818050518092,
128.253824959229)) ;
#146820=CARTESIAN_POINT('Ctrl Pts',(-31.7054543493643,12.4713262054323,
128.042128875258)) ;
#146821=CARTESIAN_POINT('Ctrl Pts',(-31.6054318541548,12.3273775325765,
127.783175932083)) ;
#146822=CARTESIAN_POINT('Ctrl Pts',(-31.4968892175325,12.2625380449618,
127.499127406172)) ;
#146823=CARTESIAN_POINT('Ctrl Pts',(-31.3854381872944,12.2810707567545,
127.206858131135)) ;
#146824=CARTESIAN_POINT('Ctrl Pts',(-31.2805878990866,12.3803129183538,
126.933416339024)) ;
#146825=CARTESIAN_POINT('Ctrl Pts',(-31.1864354677024,12.5556239144648,
126.691657848135)) ;
#146826=CARTESIAN_POINT('Ctrl Pts',(-31.111027629603,12.7914917134663,126.504358906648)) ;
#146827=CARTESIAN_POINT('Ctrl Pts',(-31.0577220690262,13.0750409894439,
126.381951641574)) ;
#146828=CARTESIAN_POINT('Ctrl Pts',(-31.0306610295189,13.3808908591526,
126.335889900064)) ;
#146829=CARTESIAN_POINT('Ctrl Pts',(-31.0303315381077,13.6908804953288,
126.368052181132)) ;
#146830=CARTESIAN_POINT('Ctrl Pts',(-31.0563466589472,13.9819858786258,
126.477198994722)) ;
#146831=CARTESIAN_POINT('Ctrl Pts',(-31.1061826731212,14.2331023151693,
126.655970164011)) ;
#146832=CARTESIAN_POINT('Ctrl Pts',(-31.1750550140311,14.4253737390559,
126.890183910735)) ;
#146833=CARTESIAN_POINT('Ctrl Pts',(-31.2583620135867,14.5469025476726,
127.166860376023)) ;
#146834=CARTESIAN_POINT('Ctrl Pts',(-31.347862049284,14.5868798001592,127.46128776363)) ;
#146835=CARTESIAN_POINT('Ctrl Pts',(-31.4375362474262,14.5442430115436,
127.756337185626)) ;
#146836=CARTESIAN_POINT('Ctrl Pts',(-31.520090798019,14.4211466691175,128.030630534762)) ;
#146837=CARTESIAN_POINT('Ctrl Pts',(-31.5887855970849,14.2262607722871,
128.26447035042)) ;
#146838=CARTESIAN_POINT('Ctrl Pts',(-31.637813480413,13.9744157563079,128.440774331866)) ;
#146839=CARTESIAN_POINT('Ctrl Pts',(-31.6631297576241,13.6824770169396,
128.547890122591)) ;
#146840=CARTESIAN_POINT('Ctrl Pts',(-31.6621601735374,13.3726811372132,
128.578131369071)) ;
#146841=CARTESIAN_POINT('Ctrl Pts',(-31.6339298075738,13.0644553037201,
128.528972432263)) ;
#146842=CARTESIAN_POINT('Ctrl Pts',(-31.5804815129814,12.7851437851833,
128.405767102733)) ;
#146843=CARTESIAN_POINT('Ctrl Pts',(-31.5040909563557,12.5493640401518,
128.215802779888)) ;
#146844=CARTESIAN_POINT('Ctrl Pts',(-31.4101685419032,12.3769707551736,
127.974484791043)) ;
#146845=CARTESIAN_POINT('Ctrl Pts',(-31.3038113686885,12.2789143084507,
127.697043035198)) ;
#146846=CARTESIAN_POINT('Ctrl Pts',(-31.1932340122808,12.2633331273902,
127.407040069204)) ;
#146847=CARTESIAN_POINT('Ctrl Pts',(-31.0843720330517,12.3306602572705,
127.12221228676)) ;
#146848=CARTESIAN_POINT('Ctrl Pts',(-30.9849847014499,12.476620286477,126.865029460424)) ;
#146849=CARTESIAN_POINT('Ctrl Pts',(-30.9016709973712,12.6891736358698,
126.654641927599)) ;
#146850=CARTESIAN_POINT('Ctrl Pts',(-30.8388786394785,12.9552555089657,
126.504364811448)) ;
#146851=CARTESIAN_POINT('Ctrl Pts',(-30.8009092568263,13.2547270236638,
126.426573132103)) ;
#146852=CARTESIAN_POINT('Ctrl Pts',(-30.7896564473616,13.5662746405731,
126.426832768617)) ;
#146853=CARTESIAN_POINT('Ctrl Pts',(-30.8051805713809,13.8673046435887,
126.505283369193)) ;
#146854=CARTESIAN_POINT('Ctrl Pts',(-30.8456859021479,14.1368396800883,
126.656749073381)) ;
#146855=CARTESIAN_POINT('Ctrl Pts',(-30.9074821394584,14.3550474216671,
126.87038266722)) ;
#146856=CARTESIAN_POINT('Ctrl Pts',(-30.9855180716348,14.5066809592571,
127.13148926813)) ;
#146857=CARTESIAN_POINT('Ctrl Pts',(-31.0733917700147,14.5805549920085,
127.421320442569)) ;
#146858=CARTESIAN_POINT('Ctrl Pts',(-31.1640057518086,14.5715434315125,
127.719124297166)) ;
#146859=CARTESIAN_POINT('Ctrl Pts',(-31.250294290685,14.480461463905,128.004304835114)) ;
#146860=CARTESIAN_POINT('Ctrl Pts',(-31.325509255673,14.3129344866538,128.257246400145)) ;
#146861=CARTESIAN_POINT('Ctrl Pts',(-31.3829962643348,14.0824719984918,
128.458246852631)) ;
#146862=CARTESIAN_POINT('Ctrl Pts',(-31.4183563386291,13.8045960176135,
128.59465740896)) ;
#146863=CARTESIAN_POINT('Ctrl Pts',(-31.4282543053624,13.4994872434927,
128.656672597553)) ;
#146864=CARTESIAN_POINT('Ctrl Pts',(-31.4110646719943,13.1877258858405,
128.639691696467)) ;
#146865=CARTESIAN_POINT('Ctrl Pts',(-31.3676711726817,12.8947281848912,
128.545939349583)) ;
#146866=CARTESIAN_POINT('Ctrl Pts',(-31.2997556078703,12.6375710521211,
128.380814298397)) ;
#146867=CARTESIAN_POINT('Ctrl Pts',(-31.2125224650725,12.4386468746083,
128.158973911426)) ;
#146868=CARTESIAN_POINT('Ctrl Pts',(-31.110552826707,12.3091461004709,127.89423942265)) ;
#146869=CARTESIAN_POINT('Ctrl Pts',(-31.0009258819824,12.259612482053,127.607074537605)) ;
#146870=CARTESIAN_POINT('Ctrl Pts',(-30.8902243931203,12.2934287591009,
127.316887906934)) ;
#146871=CARTESIAN_POINT('Ctrl Pts',(-30.7861895858125,12.4085128322788,
127.046134719561)) ;
#146872=CARTESIAN_POINT('Ctrl Pts',(-30.6956941591112,12.5956557303843,
126.814825506304)) ;
#146873=CARTESIAN_POINT('Ctrl Pts',(-30.6240074889673,12.8419007256208,
126.638483909041)) ;
#146874=CARTESIAN_POINT('Ctrl Pts',(-30.5755559223467,13.1310174981793,
126.530158612128)) ;
#146875=CARTESIAN_POINT('Ctrl Pts',(-30.5533896865543,13.4394174350743,
126.498431840003)) ;
#146876=CARTESIAN_POINT('Ctrl Pts',(-30.558221598687,13.7489280848763,126.545829231152)) ;
#146877=CARTESIAN_POINT('Ctrl Pts',(-30.588915578463,14.0326636274873,126.668504298489)) ;
#146878=CARTESIAN_POINT('Ctrl Pts',(-30.6425884547498,14.2739040718616,
126.858421059732)) ;
#146879=CARTESIAN_POINT('Ctrl Pts',(-30.7148915412408,14.4542739063911,
127.102819520797)) ;
#146880=CARTESIAN_POINT('Ctrl Pts',(-30.7992997459529,14.5602989647872,
127.382416465165)) ;
#146881=CARTESIAN_POINT('Ctrl Pts',(-30.8898956705548,14.5853165165248,
127.680264564623)) ;
#146882=CARTESIAN_POINT('Ctrl Pts',(-30.9787713220706,14.5269567135038,
127.97298882425)) ;
#146883=CARTESIAN_POINT('Ctrl Pts',(-31.059371853488,14.3891797896351,128.24165329551)) ;
#146884=CARTESIAN_POINT('Ctrl Pts',(-31.1247308236064,14.1817903074031,
128.465771041066)) ;
#146885=CARTESIAN_POINT('Ctrl Pts',(-31.1693676067746,13.9219442128278,
128.629125974528)) ;
#146886=CARTESIAN_POINT('Ctrl Pts',(-31.1898960969392,13.6244333194243,
128.722303903431)) ;
#146887=CARTESIAN_POINT('Ctrl Pts',(-31.1838033289645,13.3138308436316,
128.737553741756)) ;
#146888=CARTESIAN_POINT('Ctrl Pts',(-31.1505821290089,13.0089907399567,
128.673795751988)) ;
#146889=CARTESIAN_POINT('Ctrl Pts',(-31.0925799521882,12.7367005360714,
128.537303399666)) ;
#146890=CARTESIAN_POINT('Ctrl Pts',(-31.0125260998317,12.5117902877451,
128.336595761873)) ;
#146891=CARTESIAN_POINT('Ctrl Pts',(-30.9157663468451,12.3525056138097,
128.087033803185)) ;
#146892=CARTESIAN_POINT('Ctrl Pts',(-30.8080721736054,12.2695603566645,
127.80564077783)) ;
#146893=CARTESIAN_POINT('Ctrl Pts',(-30.6968461827106,12.2698997440141,
127.513902289464)) ;
#146894=CARTESIAN_POINT('Ctrl Pts',(-30.5899150674534,12.352163996818,127.234500824101)) ;
#146895=CARTESIAN_POINT('Ctrl Pts',(-30.4928833175223,12.5116414977634,
126.984230142973)) ;
#146896=CARTESIAN_POINT('Ctrl Pts',(-30.4129128244218,12.7360068873482,
126.783700837563)) ;
#146897=CARTESIAN_POINT('Ctrl Pts',(-30.3546072212312,13.0100795378332,
126.646534492897)) ;
#146898=CARTESIAN_POINT('Ctrl Pts',(-30.3216185057163,13.3126252447019,
126.583197233705)) ;
#146899=CARTESIAN_POINT('Ctrl Pts',(-30.315459892126,13.6254714681501,126.598503485917)) ;
#146900=CARTESIAN_POINT('Ctrl Pts',(-30.3359002449836,13.921236470121,126.691222007845)) ;
#146901=CARTESIAN_POINT('Ctrl Pts',(-30.3807986094703,14.1826934134292,
126.855550522785)) ;
#146902=CARTESIAN_POINT('Ctrl Pts',(-30.4459374684072,14.3889686231296,
127.07887661895)) ;
#146903=CARTESIAN_POINT('Ctrl Pts',(-30.5266278674902,14.5271449992224,
127.347855170467)) ;
#146904=CARTESIAN_POINT('Ctrl Pts',(-30.6156581605218,14.5852339330884,
127.641082103165)) ;
#146905=CARTESIAN_POINT('Ctrl Pts',(-30.7057064852132,14.5605427750385,
127.9371260928)) ;
#146906=CARTESIAN_POINT('Ctrl Pts',(-30.7905667310835,14.4541441679249,
128.218216443374)) ;
#146907=CARTESIAN_POINT('Ctrl Pts',(-30.862675831402,14.2740963431477,128.461966754846)) ;
#146908=CARTESIAN_POINT('Ctrl Pts',(-30.9165420426013,14.0323113034301,
128.6525373636)) ;
#146909=CARTESIAN_POINT('Ctrl Pts',(-30.9471458928728,13.7476340175603,
128.775035918765)) ;
#146910=CARTESIAN_POINT('Ctrl Pts',(-30.9519877933255,13.4408490970619,
128.822167947952)) ;
#146911=CARTESIAN_POINT('Ctrl Pts',(-30.9297341148964,13.1304291613817,
128.790407351982)) ;
#146912=CARTESIAN_POINT('Ctrl Pts',(-30.8814901893038,12.8426172804035,
128.682531897237)) ;
#146913=CARTESIAN_POINT('Ctrl Pts',(-30.8094718054732,12.5951022421241,
128.505390632872)) ;
#146914=CARTESIAN_POINT('Ctrl Pts',(-30.7191980384741,12.4086451366849,
128.274629627039)) ;
#146915=CARTESIAN_POINT('Ctrl Pts',(-30.6150556663668,12.2933533540089,
128.003603482979)) ;
#146916=CARTESIAN_POINT('Ctrl Pts',(-30.5044178921979,12.259635664544,127.713579852543)) ;
#146917=CARTESIAN_POINT('Ctrl Pts',(-30.3949358707502,12.3091205538474,
127.426799822407)) ;
#146918=CARTESIAN_POINT('Ctrl Pts',(-30.2931032152827,12.4379929301553,
127.162397289569)) ;
#146919=CARTESIAN_POINT('Ctrl Pts',(-30.2052137326913,12.6386444970783,
126.938906232635)) ;
#146920=CARTESIAN_POINT('Ctrl Pts',(-30.137812185091,12.8942394959608,126.775057354265)) ;
#146921=CARTESIAN_POINT('Ctrl Pts',(-30.0942843746289,13.1876523538433,
126.680974568525)) ;
#146922=CARTESIAN_POINT('Ctrl Pts',(-30.0771111354794,13.4984174777635,
126.663931147677)) ;
#146923=CARTESIAN_POINT('Ctrl Pts',(-30.0869464816408,13.804322914882,126.725848509996)) ;
#146924=CARTESIAN_POINT('Ctrl Pts',(-30.1223210460623,14.0825044071424,
126.862326755857)) ;
#146925=CARTESIAN_POINT('Ctrl Pts',(-30.1800394723012,14.3134151405244,
127.064102376406)) ;
#146926=CARTESIAN_POINT('Ctrl Pts',(-30.2547445132516,14.4799820056889,
127.315334142319)) ;
#146927=CARTESIAN_POINT('Ctrl Pts',(-30.3415883631799,14.5717628953294,
127.602359997053)) ;
#146928=CARTESIAN_POINT('Ctrl Pts',(-30.4318402066912,14.5804902446719,
127.898966396358)) ;
#146929=CARTESIAN_POINT('Ctrl Pts',(-30.5196878520343,14.5068426391239,
128.188713407741)) ;
#146930=CARTESIAN_POINT('Ctrl Pts',(-30.5976721590961,14.3556215775595,
128.449624531829)) ;
#146931=CARTESIAN_POINT('Ctrl Pts',(-30.6597155605127,14.1365916181852,
128.664110539127)) ;
#146932=CARTESIAN_POINT('Ctrl Pts',(-30.7000450417134,13.8680780332019,
128.814933477325)) ;
#146933=CARTESIAN_POINT('Ctrl Pts',(-30.7157305313142,13.5671869080058,
128.893853152154)) ;
#146934=CARTESIAN_POINT('Ctrl Pts',(-30.7043528399412,13.2537546109161,
128.893949585034)) ;
#146935=CARTESIAN_POINT('Ctrl Pts',(-30.6665757156128,12.9561225351469,
128.816517537223)) ;
#146936=CARTESIAN_POINT('Ctrl Pts',(-30.6038252448511,12.6895770541959,
128.666400531881)) ;
#146937=CARTESIAN_POINT('Ctrl Pts',(-30.5203605300861,12.4765149005577,
128.45563440576)) ;
#146938=CARTESIAN_POINT('Ctrl Pts',(-30.4206676847351,12.3303993150384,
128.197651178616)) ;
#146939=CARTESIAN_POINT('Ctrl Pts',(-30.3122067645033,12.2633426661684,
127.913867609128)) ;
#146940=CARTESIAN_POINT('Ctrl Pts',(-30.2012947046513,12.2791039677748,
127.622994778204)) ;
#146941=CARTESIAN_POINT('Ctrl Pts',(-30.0955067911406,12.3764767274057,
127.34702506124)) ;
#146942=CARTESIAN_POINT('Ctrl Pts',(-30.0009941671484,12.5500288715812,
127.104204398368)) ;
#146943=CARTESIAN_POINT('Ctrl Pts',(-29.9251551979687,12.78395781333,126.915590684127)) ;
#146944=CARTESIAN_POINT('Ctrl Pts',(-29.871187296773,13.0658040836913,126.791179592973)) ;
#146945=CARTESIAN_POINT('Ctrl Pts',(-29.8432186865559,13.3726170327576,
126.742615453226)) ;
#146946=CARTESIAN_POINT('Ctrl Pts',(-29.8422395429821,13.6826397298667,
126.772863652498)) ;
#146947=CARTESIAN_POINT('Ctrl Pts',(-29.8673746353157,13.9734160140871,
126.879300450678)) ;
#146948=CARTESIAN_POINT('Ctrl Pts',(-29.9167203821773,14.2269288316592,
127.056756775125)) ;
#146949=CARTESIAN_POINT('Ctrl Pts',(-29.9850311185671,14.4205112254327,
127.289268900708)) ;
#146950=CARTESIAN_POINT('Ctrl Pts',(-30.0675752554345,14.5441065975964,
127.563558807458)) ;
#146951=CARTESIAN_POINT('Ctrl Pts',(-30.1576125359038,14.5870792666042,
127.859794320208)) ;
#146952=CARTESIAN_POINT('Ctrl Pts',(-30.2474849888597,14.5462510454972,
128.155465708352)) ;
#146953=CARTESIAN_POINT('Ctrl Pts',(-30.3299319014001,14.4261089753038,
128.429272190537)) ;
#146954=CARTESIAN_POINT('Ctrl Pts',(-30.3995036371057,14.2320089308133,
128.665864379733)) ;
#146955=CARTESIAN_POINT('Ctrl Pts',(-30.4489243649137,13.9821034957132,
128.843216326838)) ;
#146956=CARTESIAN_POINT('Ctrl Pts',(-30.4749610643755,13.6914861079863,
128.952391552536)) ;
#146957=CARTESIAN_POINT('Ctrl Pts',(-30.4747999900052,13.3820427102498,
128.98498114324)) ;
#146958=CARTESIAN_POINT('Ctrl Pts',(-30.4473515216857,13.0731824784138,
128.938127658199)) ;
#146959=CARTESIAN_POINT('Ctrl Pts',(-30.3945986181408,12.7927891532511,
128.816959868306)) ;
#146960=CARTESIAN_POINT('Ctrl Pts',(-30.3187955084458,12.555308710761,128.628720211139)) ;
#146961=CARTESIAN_POINT('Ctrl Pts',(-30.2251379780315,12.3807971567645,
128.388227552432)) ;
#146962=CARTESIAN_POINT('Ctrl Pts',(-30.1194247642222,12.2807361442519,
128.112543422468)) ;
#146963=CARTESIAN_POINT('Ctrl Pts',(-30.0085407368298,12.2625961499198,
127.821752081797)) ;
#146964=CARTESIAN_POINT('Ctrl Pts',(-29.8996873404426,12.3275534579407,
127.536894483403)) ;
#146965=CARTESIAN_POINT('Ctrl Pts',(-29.7999406635735,12.4713199935408,
127.278663605204)) ;
#146966=CARTESIAN_POINT('Ctrl Pts',(-29.7160662663461,12.6818353825156,
127.066618789895)) ;
#146967=CARTESIAN_POINT('Ctrl Pts',(-29.6522505230359,12.9488695805188,
126.913606492894)) ;
#146968=CARTESIAN_POINT('Ctrl Pts',(-29.6139590229148,13.2449964341876,
126.834565223254)) ;
#146969=CARTESIAN_POINT('Ctrl Pts',(-29.6017834508264,13.5577146897345,
126.832264886568)) ;
#146970=CARTESIAN_POINT('Ctrl Pts',(-29.6166083435889,13.8591379588549,
126.90864921774)) ;
#146971=CARTESIAN_POINT('Ctrl Pts',(-29.6564971042397,14.1301669170847,
127.058355027748)) ;
#146972=CARTESIAN_POINT('Ctrl Pts',(-29.7177594105147,14.3498259232659,
127.270410807092)) ;
#146973=CARTESIAN_POINT('Ctrl Pts',(-29.7952862533984,14.5033075535996,
127.529976715887)) ;
#146974=CARTESIAN_POINT('Ctrl Pts',(-29.8830140909099,14.5795880895815,
127.819399645601)) ;
#146975=CARTESIAN_POINT('Ctrl Pts',(-29.9736829293594,14.5729975204269,
128.11737472752)) ;
#146976=CARTESIAN_POINT('Ctrl Pts',(-30.0604370601336,14.4837968438998,
128.404012404392)) ;
#146977=CARTESIAN_POINT('Ctrl Pts',(-30.1359257622124,14.3181445860539,
128.65772161378)) ;
#146978=CARTESIAN_POINT('Ctrl Pts',(-30.1938131883798,14.0900336842333,
128.859788825961)) ;
#146979=CARTESIAN_POINT('Ctrl Pts',(-30.2299435215445,13.8125787469842,
128.998529327741)) ;
#146980=CARTESIAN_POINT('Ctrl Pts',(-30.2405301452034,13.5087143541534,
129.062470965387)) ;
#146981=CARTESIAN_POINT('Ctrl Pts',(-30.2242241360838,13.1970642256003,
129.048040790549)) ;
#146982=CARTESIAN_POINT('Ctrl Pts',(-30.1814038042651,12.9023258693894,
128.956073007442)) ;
#146983=CARTESIAN_POINT('Ctrl Pts',(-30.1143382086823,12.6446851573858,
128.793320917903)) ;
#146984=CARTESIAN_POINT('Ctrl Pts',(-30.0276174900689,12.4436426796563,
128.572993750691)) ;
#146985=CARTESIAN_POINT('Ctrl Pts',(-29.9258485365255,12.3118006099846,
128.308887056809)) ;
#146986=CARTESIAN_POINT('Ctrl Pts',(-29.8163200649129,12.259762671147,128.022015597421)) ;
#146987=CARTESIAN_POINT('Ctrl Pts',(-29.7051375050554,12.2917039149137,
127.730553612688)) ;
#146988=CARTESIAN_POINT('Ctrl Pts',(-29.6016270677381,12.4035190243102,
127.461062925927)) ;
#146989=CARTESIAN_POINT('Ctrl Pts',(-29.5098964515148,12.5902948826821,
127.22643242955)) ;
#146990=CARTESIAN_POINT('Ctrl Pts',(-29.4380833187018,12.8337324578526,
127.049514825685)) ;
#146991=CARTESIAN_POINT('Ctrl Pts',(-29.3886219255085,13.1235886478701,
126.938436984437)) ;
#146992=CARTESIAN_POINT('Ctrl Pts',(-29.3659461445248,13.4302519439914,
126.905060184476)) ;
#146993=CARTESIAN_POINT('Ctrl Pts',(-29.3698075336204,13.7390104771059,
126.949495883131)) ;
#146994=CARTESIAN_POINT('Ctrl Pts',(-29.4000452910278,14.0260062251914,
127.071106527012)) ;
#146995=CARTESIAN_POINT('Ctrl Pts',(-29.4528929037883,14.267226894927,127.258426176664)) ;
#146996=CARTESIAN_POINT('Ctrl Pts',(-29.5246326985309,14.4498458863908,
127.501170540554)) ;
#146997=CARTESIAN_POINT('Ctrl Pts',(-29.6091872255536,14.5586319287784,
127.781351330665)) ;
#146998=CARTESIAN_POINT('Ctrl Pts',(-29.6997471862202,14.5856242099091,
128.07910262556)) ;
#146999=CARTESIAN_POINT('Ctrl Pts',(-29.7883807533192,14.5299078303726,
128.370974736792)) ;
#147000=CARTESIAN_POINT('Ctrl Pts',(-29.8695306978399,14.3940107888909,
128.641329791261)) ;
#147001=CARTESIAN_POINT('Ctrl Pts',(-29.9352642647434,14.1888420918384,
128.866468214376)) ;
#147002=CARTESIAN_POINT('Ctrl Pts',(-29.9806165337135,13.9299824930108,
129.031961511465)) ;
#147003=CARTESIAN_POINT('Ctrl Pts',(-30.0018750942867,13.6339609144374,
129.127188391206)) ;
#147004=CARTESIAN_POINT('Ctrl Pts',(-29.9965569305934,13.3227159368467,
129.144784844423)) ;
#147005=CARTESIAN_POINT('Ctrl Pts',(-29.9642939595592,13.0187244434426,
129.083670051289)) ;
#147006=CARTESIAN_POINT('Ctrl Pts',(-29.9069372408107,12.7442184480219,
128.949165273436)) ;
#147007=CARTESIAN_POINT('Ctrl Pts',(-29.826988446716,12.516718909921,128.748926776798)) ;
#147008=CARTESIAN_POINT('Ctrl Pts',(-29.7310520871085,12.3563386228632,
128.50161270827)) ;
#147009=CARTESIAN_POINT('Ctrl Pts',(-29.6238026629605,12.2709228353889,
128.22145763842)) ;
#147010=CARTESIAN_POINT('Ctrl Pts',(-29.5124524449978,12.2686101077704,
127.929393883299)) ;
#147011=CARTESIAN_POINT('Ctrl Pts',(-29.4050655842839,12.3485946341444,
127.648731549074)) ;
#147012=CARTESIAN_POINT('Ctrl Pts',(-29.307350900322,12.5068356453483,127.396583496414)) ;
#147013=CARTESIAN_POINT('Ctrl Pts',(-29.2273191764511,12.728330138996,127.195683455919)) ;
#147014=CARTESIAN_POINT('Ctrl Pts',(-29.1681740607996,13.0013550169445,
127.056098533042)) ;
#147015=CARTESIAN_POINT('Ctrl Pts',(-29.134416586331,13.303953158046,126.990578886437)) ;
#147016=CARTESIAN_POINT('Ctrl Pts',(-29.1274395375994,13.6158508355622,
127.003379945153)) ;
#147017=CARTESIAN_POINT('Ctrl Pts',(-29.1472523538254,13.9138455338492,
127.094439041545)) ;
#147018=CARTESIAN_POINT('Ctrl Pts',(-29.1913098510349,14.1752852419692,
127.256147124711)) ;
#147019=CARTESIAN_POINT('Ctrl Pts',(-29.2560209697753,14.3839668801463,
127.47829864687)) ;
#147020=CARTESIAN_POINT('Ctrl Pts',(-29.3362834013603,14.5240578429112,
127.745988342019)) ;
#147021=CARTESIAN_POINT('Ctrl Pts',(-29.4250790846387,14.584818932524,128.038503048431)) ;
#147022=CARTESIAN_POINT('Ctrl Pts',(-29.5157805659722,14.5621167369362,
128.33667727634)) ;
#147023=CARTESIAN_POINT('Ctrl Pts',(-29.6003485790494,14.4583966415937,
128.616704866655)) ;
#147024=CARTESIAN_POINT('Ctrl Pts',(-29.672999428089,14.2803903963779,128.862065022642)) ;
#147025=CARTESIAN_POINT('Ctrl Pts',(-29.7273636308734,14.0406559571458,
129.054023045337)) ;
#147026=CARTESIAN_POINT('Ctrl Pts',(-29.7588399368944,13.7571590252373,
129.179067225918)) ;
#147027=CARTESIAN_POINT('Ctrl Pts',(-29.7643708007054,13.4483332658606,
129.228470996735)) ;
#147028=CARTESIAN_POINT('Ctrl Pts',(-29.7431271902945,13.1406103959238,
129.199333519999)) ;
#147029=CARTESIAN_POINT('Ctrl Pts',(-29.6952107620917,12.849237718573,129.092722743839)) ;
#147030=CARTESIAN_POINT('Ctrl Pts',(-29.6242103407272,12.6021186040621,
128.918326096847)) ;
#147031=CARTESIAN_POINT('Ctrl Pts',(-29.534342376669,12.4130744428075,128.688810495785)) ;
#147032=CARTESIAN_POINT('Ctrl Pts',(-29.4300815144381,12.295357536539,128.417555698654)) ;
#147033=CARTESIAN_POINT('Ctrl Pts',(-29.3199980857374,12.2595400049776,
128.129012313781)) ;
#147034=CARTESIAN_POINT('Ctrl Pts',(-29.2102972783543,12.3063152833776,
127.841614367448)) ;
#147035=CARTESIAN_POINT('Ctrl Pts',(-29.1075765805156,12.4341408238282,
127.57482056363)) ;
#147036=CARTESIAN_POINT('Ctrl Pts',(-29.0198927916179,12.6316134700122,
127.351679653212)) ;
#147037=CARTESIAN_POINT('Ctrl Pts',(-28.9516398841463,12.8861350192124,
127.185411007251)) ;
#147038=CARTESIAN_POINT('Ctrl Pts',(-28.9073369484727,13.1792139028364,
127.089109169935)) ;
#147039=CARTESIAN_POINT('Ctrl Pts',(-28.8894132390635,13.490568739432,127.069953917477)) ;
#147040=CARTESIAN_POINT('Ctrl Pts',(-28.8985917369534,13.7964603979055,
127.129907547714)) ;
#147041=CARTESIAN_POINT('Ctrl Pts',(-28.933109908976,14.0743848180785,127.263731937239)) ;
#147042=CARTESIAN_POINT('Ctrl Pts',(-28.9900661981856,14.3070162611111,
127.463243023677)) ;
#147043=CARTESIAN_POINT('Ctrl Pts',(-29.0648227386281,14.476451846962,127.714825187418)) ;
#147044=CARTESIAN_POINT('Ctrl Pts',(-29.1506744032719,14.569850177848,127.998660756491)) ;
#147045=CARTESIAN_POINT('Ctrl Pts',(-29.2413663721334,14.5816111241078,
128.296730098651)) ;
#147046=CARTESIAN_POINT('Ctrl Pts',(-29.3296595746276,14.5098991717079,
128.587875780273)) ;
#147047=CARTESIAN_POINT('Ctrl Pts',(-29.4080445514393,14.360403037698,128.849988285308)) ;
#147048=CARTESIAN_POINT('Ctrl Pts',(-29.4704203779367,14.143565690272,129.065356761645)) ;
#147049=CARTESIAN_POINT('Ctrl Pts',(-29.5114914499604,13.8762646142661,
129.218353321002)) ;
#147050=CARTESIAN_POINT('Ctrl Pts',(-29.527821482954,13.5746434283165,129.299296311103)) ;
#147051=CARTESIAN_POINT('Ctrl Pts',(-29.5174206340191,13.2647986868619,
129.301857135357)) ;
#147052=CARTESIAN_POINT('Ctrl Pts',(-29.4802017636136,12.9638356585252,
129.226346996376)) ;
#147053=CARTESIAN_POINT('Ctrl Pts',(-29.4181913382434,12.696740713892,129.0783105115)) ;
#147054=CARTESIAN_POINT('Ctrl Pts',(-29.3350888977121,12.4815167402667,
128.868676644818)) ;
#147055=CARTESIAN_POINT('Ctrl Pts',(-29.2361228630141,12.3337893595149,
128.61269329159)) ;
#147056=CARTESIAN_POINT('Ctrl Pts',(-29.1275784391396,12.2640797923872,
128.3287499801)) ;
#147057=CARTESIAN_POINT('Ctrl Pts',(-29.0167646928416,12.2774691483239,
128.038121461427)) ;
#147058=CARTESIAN_POINT('Ctrl Pts',(-28.9107301726355,12.3724670418659,
127.761433361359)) ;
#147059=CARTESIAN_POINT('Ctrl Pts',(-28.8158185730082,12.543767432119,127.517423530661)) ;
#147060=CARTESIAN_POINT('Ctrl Pts',(-28.7392542408097,12.7765746874498,
127.32675668177)) ;
#147061=CARTESIAN_POINT('Ctrl Pts',(-28.6847206547343,13.056442699504,127.200585791957)) ;
#147062=CARTESIAN_POINT('Ctrl Pts',(-28.6558953247287,13.3632374383365,
127.149573983655)) ;
#147063=CARTESIAN_POINT('Ctrl Pts',(-28.6540191244132,13.6730055112077,
127.177138695141)) ;
#147064=CARTESIAN_POINT('Ctrl Pts',(-28.6787541261639,13.9671153301203,
127.282712736634)) ;
#147065=CARTESIAN_POINT('Ctrl Pts',(-28.726959761685,14.2192391105439,127.456470176809)) ;
#147066=CARTESIAN_POINT('Ctrl Pts',(-28.7952494116795,14.4164802327196,
127.689188807195)) ;
#147067=CARTESIAN_POINT('Ctrl Pts',(-28.8773322714303,14.5415580388922,
127.96203905316)) ;
#147068=CARTESIAN_POINT('Ctrl Pts',(-28.966957796165,14.5869148382087,128.25697340176)) ;
#147069=CARTESIAN_POINT('Ctrl Pts',(-29.056892610989,14.5490099529441,128.55279780603)) ;
#147070=CARTESIAN_POINT('Ctrl Pts',(-29.1402169930976,14.4299835692337,
128.829416302567)) ;
#147071=CARTESIAN_POINT('Ctrl Pts',(-29.2096450513186,14.2395160261302,
129.065284124465)) ;
#147072=CARTESIAN_POINT('Ctrl Pts',(-29.2600489235632,13.9900850961344,
129.245677108272)) ;
#147073=CARTESIAN_POINT('Ctrl Pts',(-29.2867905400275,13.7002631156838,
129.356907899631)) ;
#147074=CARTESIAN_POINT('Ctrl Pts',(-29.2873580451206,13.3906063492619,
129.391679953749)) ;
#147075=CARTESIAN_POINT('Ctrl Pts',(-29.2608441995176,13.0826197535591,
129.347411851006)) ;
#147076=CARTESIAN_POINT('Ctrl Pts',(-29.2085441327409,12.7997481172877,
129.227739730843)) ;
#147077=CARTESIAN_POINT('Ctrl Pts',(-29.1335049130153,12.5614902971475,
129.041634768994)) ;
#147078=CARTESIAN_POINT('Ctrl Pts',(-29.0401540366399,12.3846250273346,
128.802093504295)) ;
#147079=CARTESIAN_POINT('Ctrl Pts',(-28.9346464367386,12.2824687909252,
128.527016672722)) ;
#147080=CARTESIAN_POINT('Ctrl Pts',(-28.824116083048,12.2619556332192,128.237168385874)) ;
#147081=CARTESIAN_POINT('Ctrl Pts',(-28.7149966519967,12.3244285143439,
127.951562960797)) ;
#147082=CARTESIAN_POINT('Ctrl Pts',(-28.6146573164258,12.4664340119557,
127.691677135041)) ;
#147083=CARTESIAN_POINT('Ctrl Pts',(-28.5303819440555,12.675348720281,127.478448660203)) ;
#147084=CARTESIAN_POINT('Ctrl Pts',(-28.4662472388225,12.9390314346698,
127.32426847584)) ;
#147085=CARTESIAN_POINT('Ctrl Pts',(-28.426784584346,13.2369183007794,127.242088186904)) ;
#147086=CARTESIAN_POINT('Ctrl Pts',(-28.414001297498,13.549774387286,127.238027762963)) ;
#147087=CARTESIAN_POINT('Ctrl Pts',(-28.4280334218581,13.850609448165,127.311971837892)) ;
#147088=CARTESIAN_POINT('Ctrl Pts',(-28.4672280424493,14.1229209827014,
127.459657669781)) ;
#147089=CARTESIAN_POINT('Ctrl Pts',(-28.5278478480601,14.3440340746158,
127.669795018464)) ;
#147090=CARTESIAN_POINT('Ctrl Pts',(-28.6050799543434,14.5000650496519,
127.928551700968)) ;
#147091=CARTESIAN_POINT('Ctrl Pts',(-28.6930251647457,14.578644462167,128.218756301245)) ;
#147092=CARTESIAN_POINT('Ctrl Pts',(-28.7831377408782,14.5743811633841,
128.514894788016)) ;
#147093=CARTESIAN_POINT('Ctrl Pts',(-28.8703782343565,14.4873598726622,
128.803057217724)) ;
#147094=CARTESIAN_POINT('Ctrl Pts',(-28.9461043703451,14.3240886770746,
129.057379640458)) ;
#147095=CARTESIAN_POINT('Ctrl Pts',(-29.0046450639296,14.0972553014586,
129.261412205121)) ;
#147096=CARTESIAN_POINT('Ctrl Pts',(-29.041421187763,13.8219067372358,129.401927249139)) ;
#147097=CARTESIAN_POINT('Ctrl Pts',(-29.0528414560578,13.5160256526642,
129.468579531831)) ;
#147098=CARTESIAN_POINT('Ctrl Pts',(-29.0371616190134,13.2050737641674,
129.455888808854)) ;
#147099=CARTESIAN_POINT('Ctrl Pts',(-28.9952221551934,12.9106474096039,
129.366380741704)) ;
#147100=CARTESIAN_POINT('Ctrl Pts',(-28.9289573583744,12.6518068441283,
129.205925046669)) ;
#147101=CARTESIAN_POINT('Ctrl Pts',(-28.8423703172031,12.4481718520534,
128.986128276051)) ;
#147102=CARTESIAN_POINT('Ctrl Pts',(-28.7410953233907,12.3143466124611,
128.723403080249)) ;
#147103=CARTESIAN_POINT('Ctrl Pts',(-28.6311229647181,12.2602411287431,
128.435411596259)) ;
#147104=CARTESIAN_POINT('Ctrl Pts',(-28.521399927036,12.289044216294,128.147739484492)) ;
#147105=CARTESIAN_POINT('Ctrl Pts',(-28.4163596339001,12.3996399053781,
127.874180741612)) ;
#147106=CARTESIAN_POINT('Ctrl Pts',(-28.3249767341809,12.5827969083002,
127.64025343428)) ;
#147107=CARTESIAN_POINT('Ctrl Pts',(-28.2518532145278,12.826962989628,127.459831520999)) ;
#147108=CARTESIAN_POINT('Ctrl Pts',(-28.2021925015218,13.1127056207623,
127.34779653997)) ;
#147109=CARTESIAN_POINT('Ctrl Pts',(-28.178363709681,13.421711878802,127.311352934498)) ;
#147110=CARTESIAN_POINT('Ctrl Pts',(-28.1815690515954,13.7304251120726,
127.353829356402)) ;
#147111=CARTESIAN_POINT('Ctrl Pts',(-28.211039530244,14.018344311728,127.473192935567)) ;
#147112=CARTESIAN_POINT('Ctrl Pts',(-28.2634287201407,14.2615012017521,
127.659241766758)) ;
#147113=CARTESIAN_POINT('Ctrl Pts',(-28.3346148571528,14.4455241651706,
127.900307053913)) ;
#147114=CARTESIAN_POINT('Ctrl Pts',(-28.418623430654,14.5564730529287,128.178795974798)) ;
#147115=CARTESIAN_POINT('Ctrl Pts',(-28.5094384562439,14.58603325722,128.477414862936)) ;
#147116=CARTESIAN_POINT('Ctrl Pts',(-28.5980426291786,14.5327319880778,
128.769135372419)) ;
#147117=CARTESIAN_POINT('Ctrl Pts',(-28.6796160846217,14.3988255152791,
129.040771032821)) ;
#147118=CARTESIAN_POINT('Ctrl Pts',(-28.745579180709,14.1966329622431,129.266414354394)) ;
#147119=CARTESIAN_POINT('Ctrl Pts',(-28.7918797647502,13.9381994545952,
129.434822486951)) ;
#147120=CARTESIAN_POINT('Ctrl Pts',(-28.8138551442112,13.6421507642692,
129.532218437035)) ;
#147121=CARTESIAN_POINT('Ctrl Pts',(-28.8092832638101,13.3319747880892,
129.551898416221)) ;
#147122=CARTESIAN_POINT('Ctrl Pts',(-28.7779247190653,13.0275241495644,
129.493404475197)) ;
#147123=CARTESIAN_POINT('Ctrl Pts',(-28.7206834966505,12.7499513139427,
129.359499879805)) ;
#147124=CARTESIAN_POINT('Ctrl Pts',(-28.6420010050341,12.5230805952481,
129.162644470801)) ;
#147125=CARTESIAN_POINT('Ctrl Pts',(-28.5460238731504,12.3595163479197,
128.915388817262)) ;
#147126=CARTESIAN_POINT('Ctrl Pts',(-28.4387186631021,12.2720601072795,
128.6351364541)) ;
#147127=CARTESIAN_POINT('Ctrl Pts',(-28.3276074338221,12.2676665398888,
128.343703806802)) ;
#147128=CARTESIAN_POINT('Ctrl Pts',(-28.2204032567713,12.3451448289758,
128.063463534875)) ;
#147129=CARTESIAN_POINT('Ctrl Pts',(-28.1225359120705,12.5004782540512,
127.810766610281)) ;
#147130=CARTESIAN_POINT('Ctrl Pts',(-28.0414953870407,12.7212077587515,
127.607081321906)) ;
#147131=CARTESIAN_POINT('Ctrl Pts',(-27.9816602120392,12.9936145319541,
127.4655295393)) ;
#147132=CARTESIAN_POINT('Ctrl Pts',(-27.9472693123842,13.2947837203187,
127.398064809065)) ;
#147133=CARTESIAN_POINT('Ctrl Pts',(-27.9394737059955,13.6064068032795,
127.408440270478)) ;
#147134=CARTESIAN_POINT('Ctrl Pts',(-27.9584521870025,13.9050217412781,
127.497042995191)) ;
#147135=CARTESIAN_POINT('Ctrl Pts',(-28.0019723652954,14.1686336677941,
127.657287030857)) ;
#147136=CARTESIAN_POINT('Ctrl Pts',(-28.0661545150661,14.3788182698461,
127.877871299589)) ;
#147137=CARTESIAN_POINT('Ctrl Pts',(-28.1458363458335,14.5208662743525,
128.14378094547)) ;
#147138=CARTESIAN_POINT('Ctrl Pts',(-28.2345899026998,14.5841619964858,
128.436220428999)) ;
#147139=CARTESIAN_POINT('Ctrl Pts',(-28.3250495930938,14.5641966212731,
128.733575916725)) ;
#147140=CARTESIAN_POINT('Ctrl Pts',(-28.4102887222356,14.4625802031817,
129.01571259501)) ;
#147141=CARTESIAN_POINT('Ctrl Pts',(-28.4834734306057,14.286005519678,129.262692624796)) ;
#147142=CARTESIAN_POINT('Ctrl Pts',(-28.5382560423696,14.0484511766116,
129.455778944107)) ;
#147143=CARTESIAN_POINT('Ctrl Pts',(-28.5704620543408,13.7663469641466,
129.58292061169)) ;
#147144=CARTESIAN_POINT('Ctrl Pts',(-28.5768364910779,13.4574607862846,
129.634836630178)) ;
#147145=CARTESIAN_POINT('Ctrl Pts',(-28.5562466562937,13.1488899343714,
129.607677485992)) ;
#147146=CARTESIAN_POINT('Ctrl Pts',(-28.5093930101883,12.8583365038161,
129.503969294116)) ;
#147147=CARTESIAN_POINT('Ctrl Pts',(-28.4388409420063,12.6085157642258,
129.331015719234)) ;
#147148=CARTESIAN_POINT('Ctrl Pts',(-28.349200703581,12.417394689709,129.102233983392)) ;
#147149=CARTESIAN_POINT('Ctrl Pts',(-28.2458285984717,12.2980452519264,
128.833391652384)) ;
#147150=CARTESIAN_POINT('Ctrl Pts',(-28.1357470146788,12.2592457780577,
128.544885828624)) ;
#147151=CARTESIAN_POINT('Ctrl Pts',(-28.0254127094965,12.304020860261,128.255796572371)) ;
#147152=CARTESIAN_POINT('Ctrl Pts',(-27.9230809162868,12.4286939335528,
127.989907508623)) ;
#147153=CARTESIAN_POINT('Ctrl Pts',(-27.8345386835555,12.6243589997422,
127.764349398266)) ;
#147154=CARTESIAN_POINT('Ctrl Pts',(-27.7653382579701,12.878908332841,127.595482065447)) ;
#147155=CARTESIAN_POINT('Ctrl Pts',(-27.7205297869088,13.1702261034011,
127.497588845532)) ;
#147156=CARTESIAN_POINT('Ctrl Pts',(-27.7017835873121,13.4805036941569,
127.475942764132)) ;
#147157=CARTESIAN_POINT('Ctrl Pts',(-27.710102323973,13.7876511360062,127.533460289688)) ;
#147158=CARTESIAN_POINT('Ctrl Pts',(-27.7441693729637,14.0678452510403,
127.666126181136)) ;
#147159=CARTESIAN_POINT('Ctrl Pts',(-27.8002814506919,14.3007432572347,
127.862995333965)) ;
#147160=CARTESIAN_POINT('Ctrl Pts',(-27.8746546477273,14.4725786347777,
128.113498687342)) ;
#147161=CARTESIAN_POINT('Ctrl Pts',(-27.9602816443766,14.5682598851549,
128.396677955504)) ;
#147162=CARTESIAN_POINT('Ctrl Pts',(-28.0509255421651,14.5824152929646,
128.69460486853)) ;
#147163=CARTESIAN_POINT('Ctrl Pts',(-28.1392618095582,14.5133614701989,
128.98581686609)) ;
#147164=CARTESIAN_POINT('Ctrl Pts',(-28.2181642812926,14.3656855427812,
129.249510046041)) ;
#147165=CARTESIAN_POINT('Ctrl Pts',(-28.2808475403188,14.1519223371762,
129.465604823184)) ;
#147166=CARTESIAN_POINT('Ctrl Pts',(-28.3229370821972,13.8839965789022,
129.621822830416)) ;
#147167=CARTESIAN_POINT('Ctrl Pts',(-28.3399163611,13.5839686018203,129.704545642806)) ;
#147168=CARTESIAN_POINT('Ctrl Pts',(-28.3303022079607,13.2736211027787,
129.709464937928)) ;
#147169=CARTESIAN_POINT('Ctrl Pts',(-28.2939612293933,12.9727616409807,
129.636430416121)) ;
#147170=CARTESIAN_POINT('Ctrl Pts',(-28.2324344840821,12.7034620887289,
129.489924492685)) ;
#147171=CARTESIAN_POINT('Ctrl Pts',(-28.1498921349049,12.4867212109574,
129.281903673158)) ;
#147172=CARTESIAN_POINT('Ctrl Pts',(-28.0511944467291,12.3368637166341,
129.026735473833)) ;
#147173=CARTESIAN_POINT('Ctrl Pts',(-27.9431866501433,12.265034692949,128.744249987499)) ;
#147174=CARTESIAN_POINT('Ctrl Pts',(-27.8320553152906,12.2758062586622,
128.45277717957)) ;
#147175=CARTESIAN_POINT('Ctrl Pts',(-27.725403769765,12.3692807185403,128.174418307397)) ;
#147176=CARTESIAN_POINT('Ctrl Pts',(-27.6305768731226,12.5378929203228,
127.930489816518)) ;
#147177=CARTESIAN_POINT('Ctrl Pts',(-27.5532840737938,12.7694277251572,
127.737752051998)) ;
#147178=CARTESIAN_POINT('Ctrl Pts',(-27.4980628041724,13.0484835802669,
127.609590602882)) ;
#147179=CARTESIAN_POINT('Ctrl Pts',(-27.468512009568,13.3553251834758,127.556508766541)) ;
#147180=CARTESIAN_POINT('Ctrl Pts',(-27.4659658852971,13.664055596243,127.581991492348)) ;
#147181=CARTESIAN_POINT('Ctrl Pts',(-27.4897083326271,13.9577070332473,
127.684504096901)) ;
#147182=CARTESIAN_POINT('Ctrl Pts',(-27.537488419938,14.2128779767414,127.857213382513)) ;
#147183=CARTESIAN_POINT('Ctrl Pts',(-27.6053110365793,14.4117544181439,
128.088557180992)) ;
#147184=CARTESIAN_POINT('Ctrl Pts',(-27.6870263113948,14.539128300591,128.360320009239)) ;
#147185=CARTESIAN_POINT('Ctrl Pts',(-27.776949692643,14.5867879384206,128.656273925629)) ;
#147186=CARTESIAN_POINT('Ctrl Pts',(-27.866542120589,14.5512051552351,128.950939963951)) ;
#147187=CARTESIAN_POINT('Ctrl Pts',(-27.9503029825462,14.4343419878625,
129.228886623273)) ;
#147188=CARTESIAN_POINT('Ctrl Pts',(-28.0201765415202,14.2455278913779,
129.466064406398)) ;
#147189=CARTESIAN_POINT('Ctrl Pts',(-28.071089607046,13.9981929136205,129.647863070259)) ;
#147190=CARTESIAN_POINT('Ctrl Pts',(-28.0986318176994,13.7085066706188,
129.76151901077)) ;
#147191=CARTESIAN_POINT('Ctrl Pts',(-28.099895689668,13.3995793923712,129.798274390018)) ;
#147192=CARTESIAN_POINT('Ctrl Pts',(-28.0743169746615,13.0919774693214,
129.756648462602)) ;
#147193=CARTESIAN_POINT('Ctrl Pts',(-28.0224473100631,12.8067303773131,
129.638400985545)) ;
#147194=CARTESIAN_POINT('Ctrl Pts',(-27.9483787106709,12.5682008824759,
129.454956724157)) ;
#147195=CARTESIAN_POINT('Ctrl Pts',(-27.8553471386476,12.3888212214355,
129.216414429093)) ;
#147196=CARTESIAN_POINT('Ctrl Pts',(-27.7502434316432,12.2844119471438,
128.942471886976)) ;
#147197=CARTESIAN_POINT('Ctrl Pts',(-27.6394225717743,12.2613333945147,
128.651879574797)) ;
#147198=CARTESIAN_POINT('Ctrl Pts',(-27.5302844551379,12.3215794553672,
128.366182543468)) ;
#147199=CARTESIAN_POINT('Ctrl Pts',(-27.4299126178422,12.4606919099578,
128.106084606762)) ;
#147200=CARTESIAN_POINT('Ctrl Pts',(-27.3447157997432,12.6684213928488,
127.890292996441)) ;
#147201=CARTESIAN_POINT('Ctrl Pts',(-27.2797816216191,12.9319195354802,
127.733892745092)) ;
#147202=CARTESIAN_POINT('Ctrl Pts',(-27.2398427283627,13.2279082414743,
127.650182015427)) ;
#147203=CARTESIAN_POINT('Ctrl Pts',(-27.226194121743,13.5392233230321,127.643439401524)) ;
#147204=CARTESIAN_POINT('Ctrl Pts',(-27.2394396068356,13.8421683173594,
127.715246834978)) ;
#147205=CARTESIAN_POINT('Ctrl Pts',(-27.2780066999911,14.1158320229517,
127.861122787859)) ;
#147206=CARTESIAN_POINT('Ctrl Pts',(-27.3382205711599,14.3390093108208,
128.070142127096)) ;
#147207=CARTESIAN_POINT('Ctrl Pts',(-27.4149366221091,14.4964745631391,
128.327319073576)) ;
#147208=CARTESIAN_POINT('Ctrl Pts',(-27.5021455833055,14.5773715751741,
128.615182034661)) ;
#147209=CARTESIAN_POINT('Ctrl Pts',(-27.5929606140918,14.5757025299613,
128.913627228843)) ;
#147210=CARTESIAN_POINT('Ctrl Pts',(-27.6801654786792,14.4908671144554,
129.201599628883)) ;
#147211=CARTESIAN_POINT('Ctrl Pts',(-27.7560500937159,14.3305923177535,
129.456257297716)) ;
#147212=CARTESIAN_POINT('Ctrl Pts',(-27.8154777130251,14.1048090701634,
129.663003115917)) ;
#147213=CARTESIAN_POINT('Ctrl Pts',(-27.8529655928213,13.8293691647795,
129.805723526022)) ;
#147214=CARTESIAN_POINT('Ctrl Pts',(-27.8650722307394,13.5265763718341,
129.874102214767)) ;
#147215=CARTESIAN_POINT('Ctrl Pts',(-27.8503095252252,13.2147295079812,
129.864175235836)) ;
#147216=CARTESIAN_POINT('Ctrl Pts',(-27.8090676741835,12.9189025307067,
129.776765848521)) ;
#147217=CARTESIAN_POINT('Ctrl Pts',(-27.7431914354456,12.6580299583616,
129.617552969924)) ;
#147218=CARTESIAN_POINT('Ctrl Pts',(-27.6574792309469,12.4534345786707,
129.400168322233)) ;
#147219=CARTESIAN_POINT('Ctrl Pts',(-27.5562948938853,12.3171076737635,
129.137795596999)) ;
#147220=CARTESIAN_POINT('Ctrl Pts',(-27.4470412666183,12.2606844029487,
128.851727105467)) ;
#147221=CARTESIAN_POINT('Ctrl Pts',(-27.3364454227257,12.2870889528383,
128.561747072364)) ;
#147222=CARTESIAN_POINT('Ctrl Pts',(-27.2312037738575,12.3957983082861,
128.28758735162)) ;
#147223=CARTESIAN_POINT('Ctrl Pts',(-27.1395909727778,12.5767257036487,
128.05292203751)) ;
#147224=CARTESIAN_POINT('Ctrl Pts',(-27.0659643781722,12.818699316301,127.870953859959)) ;
#147225=CARTESIAN_POINT('Ctrl Pts',(-27.0153388797732,13.105041814552,127.756279306161)) ;
#147226=CARTESIAN_POINT('Ctrl Pts',(-26.9908956643554,13.4130762761878,
127.717963345236)) ;
#147227=CARTESIAN_POINT('Ctrl Pts',(-26.9933449092516,13.7214651892491,
127.758172020665)) ;
#147228=CARTESIAN_POINT('Ctrl Pts',(-27.0218385472917,14.0093161776234,
127.8745403043)) ;
#147229=CARTESIAN_POINT('Ctrl Pts',(-27.074036131509,14.2560736746046,128.060312178445)) ;
#147230=CARTESIAN_POINT('Ctrl Pts',(-27.1446201324908,14.4412184345139,
128.299514522)) ;
#147231=CARTESIAN_POINT('Ctrl Pts',(-27.2283338792895,14.5543182512014,
128.577143613464)) ;
#147232=CARTESIAN_POINT('Ctrl Pts',(-27.3186446732475,14.5864671227743,
128.874128754955)) ;
#147233=CARTESIAN_POINT('Ctrl Pts',(-27.4079946957503,14.5351930421584,
129.16826245517)) ;
#147234=CARTESIAN_POINT('Ctrl Pts',(-27.4893963387798,14.4042256673591,
129.439187707624)) ;
#147235=CARTESIAN_POINT('Ctrl Pts',(-27.556178276305,14.2033620088234,129.667350441437)) ;
#147236=CARTESIAN_POINT('Ctrl Pts',(-27.6030960151028,13.9460943123355,
129.837568573444)) ;
#147237=CARTESIAN_POINT('Ctrl Pts',(-27.625791925615,13.651094014162,129.937042303808)) ;
#147238=CARTESIAN_POINT('Ctrl Pts',(-27.6220316760032,13.340963258282,129.959100830306)) ;
#147239=CARTESIAN_POINT('Ctrl Pts',(-27.5913092970485,13.0355469071403,
129.902524920128)) ;
#147240=CARTESIAN_POINT('Ctrl Pts',(-27.5351586679639,12.7584810147084,
129.771601190251)) ;
#147241=CARTESIAN_POINT('Ctrl Pts',(-27.456805832877,12.5287898592304,129.575848285187)) ;
#147242=CARTESIAN_POINT('Ctrl Pts',(-27.3612326647653,12.3633457050948,
129.329763294114)) ;
#147243=CARTESIAN_POINT('Ctrl Pts',(-27.2545344495649,12.2737023356338,
129.051174297588)) ;
#147244=CARTESIAN_POINT('Ctrl Pts',(-27.1434004213349,12.2663504555484,
128.759683649007)) ;
#147245=CARTESIAN_POINT('Ctrl Pts',(-27.0353422164726,12.3420801358765,
128.477156085888)) ;
#147246=CARTESIAN_POINT('Ctrl Pts',(-26.9375649820687,12.4946576254463,
128.224562106625)) ;
#147247=CARTESIAN_POINT('Ctrl Pts',(-26.8556736032525,12.7142649717312,
128.018500360345)) ;
#147248=CARTESIAN_POINT('Ctrl Pts',(-26.7952452994607,12.9853994961716,
127.875192560308)) ;
#147249=CARTESIAN_POINT('Ctrl Pts',(-26.7600758607061,13.2860374615536,
127.805462444181)) ;
#147250=CARTESIAN_POINT('Ctrl Pts',(-26.7515328287848,13.5985522242575,
127.813742362503)) ;
#147251=CARTESIAN_POINT('Ctrl Pts',(-26.7698756432365,13.8975128735152,
127.900464759074)) ;
#147252=CARTESIAN_POINT('Ctrl Pts',(-26.8125360422085,14.1612606569833,
128.058053439872)) ;
#147253=CARTESIAN_POINT('Ctrl Pts',(-26.8763333439844,14.3739608476098,
128.277609007069)) ;
#147254=CARTESIAN_POINT('Ctrl Pts',(-26.9559480791001,14.518294704107,128.543420710541)) ;
#147255=CARTESIAN_POINT('Ctrl Pts',(-27.0443940887923,14.5834512840226,
128.834899340936)) ;
#147256=CARTESIAN_POINT('Ctrl Pts',(-27.1346038864515,14.5659482192211,
129.131417292674)) ;
#147257=CARTESIAN_POINT('Ctrl Pts',(-27.2200732093609,14.4667697740707,
129.414216297154)) ;
#147258=CARTESIAN_POINT('Ctrl Pts',(-27.2937703844988,14.2923285700355,
129.662701599611)) ;
#147259=CARTESIAN_POINT('Ctrl Pts',(-27.3494004042238,14.0548140486651,
129.858453434174)) ;
#147260=CARTESIAN_POINT('Ctrl Pts',(-27.3820270800496,13.7751054294997,
129.986645187117)) ;
#147261=CARTESIAN_POINT('Ctrl Pts',(-27.3893034306534,13.4671706932676,
130.041144761007)) ;
#147262=CARTESIAN_POINT('Ctrl Pts',(-27.3693096962278,13.1566326789877,
130.015914968687)) ;
#147263=CARTESIAN_POINT('Ctrl Pts',(-27.3234453767361,12.8670308674408,
129.91489111767)) ;
#147264=CARTESIAN_POINT('Ctrl Pts',(-27.2533334364548,12.6146257445343,
129.743351676563)) ;
#147265=CARTESIAN_POINT('Ctrl Pts',(-27.1639433566548,12.4216271707414,
129.515355134645)) ;
#147266=CARTESIAN_POINT('Ctrl Pts',(-27.0613606146514,12.3004936343569,
129.248664903975)) ;
#147267=CARTESIAN_POINT('Ctrl Pts',(-26.9507521852777,12.2591976943178,
128.958810361861)) ;
#147268=CARTESIAN_POINT('Ctrl Pts',(-26.8410653311802,12.3014766465694,
128.671386114435)) ;
#147269=CARTESIAN_POINT('Ctrl Pts',(-26.7381556212626,12.4236752423031,
128.403872346275)) ;
#147270=CARTESIAN_POINT('Ctrl Pts',(-26.6486024466278,12.6191375568078,
128.175587812738)) ;
#147271=CARTESIAN_POINT('Ctrl Pts',(-26.5792953547801,12.8707902400354,
128.006190100915)) ;
#147272=CARTESIAN_POINT('Ctrl Pts',(-26.5336332509194,13.1617413268143,
127.905867012926)) ;
#147273=CARTESIAN_POINT('Ctrl Pts',(-26.5141802488474,13.4713352737269,
127.882101279265)) ;
#147274=CARTESIAN_POINT('Ctrl Pts',(-26.5216819221517,13.7785022138413,
127.937189629823)) ;
#147275=CARTESIAN_POINT('Ctrl Pts',(-26.5549217794985,14.0596469368124,
128.067407385282)) ;
#147276=CARTESIAN_POINT('Ctrl Pts',(-26.610728225856,14.2953142567661,128.263552793007)) ;
#147277=CARTESIAN_POINT('Ctrl Pts',(-26.684686815018,14.4689647332084,128.512830919732)) ;
#147278=CARTESIAN_POINT('Ctrl Pts',(-26.7703491580962,14.5668407340065,
128.796212142762)) ;
#147279=CARTESIAN_POINT('Ctrl Pts',(-26.8605101017941,14.5831863615057,
129.092558768383)) ;
#147280=CARTESIAN_POINT('Ctrl Pts',(-26.9493781611684,14.5160479174659,
129.385470762593)) ;
#147281=CARTESIAN_POINT('Ctrl Pts',(-27.0282194316067,14.3710573530436,
129.648813233255)) ;
#147282=CARTESIAN_POINT('Ctrl Pts',(-27.0915895135471,14.1586832186318,
129.866986504732)) ;
#147283=CARTESIAN_POINT('Ctrl Pts',(-27.1342318596262,13.8924168097658,
130.02475813213)) ;
#147284=CARTESIAN_POINT('Ctrl Pts',(-27.1520214448119,13.5934590630732,
130.109811091012)) ;
#147285=CARTESIAN_POINT('Ctrl Pts',(-27.1431457178143,13.2817949508325,
130.117027448321)) ;
#147286=CARTESIAN_POINT('Ctrl Pts',(-27.107478861766,12.9807520838768,130.045927154159)) ;
#147287=CARTESIAN_POINT('Ctrl Pts',(-27.0469864938312,12.7114088692144,
129.902283115458)) ;
#147288=CARTESIAN_POINT('Ctrl Pts',(-26.9647202422579,12.4920355710748,
129.695194113043)) ;
#147289=CARTESIAN_POINT('Ctrl Pts',(-26.8666704559515,12.3404092306431,
129.441827358629)) ;
#147290=CARTESIAN_POINT('Ctrl Pts',(-26.7584759114317,12.2658594230555,
129.158914687965)) ;
#147291=CARTESIAN_POINT('Ctrl Pts',(-26.647473216562,12.2744067792623,128.867771365807)) ;
#147292=CARTESIAN_POINT('Ctrl Pts',(-26.5408791869932,12.3651073701196,
128.58948675102)) ;
#147293=CARTESIAN_POINT('Ctrl Pts',(-26.4454504393884,12.5316552741645,
128.343844417814)) ;
#147294=CARTESIAN_POINT('Ctrl Pts',(-26.3673650678726,12.7621961418758,
128.148878346518)) ;
#147295=CARTESIAN_POINT('Ctrl Pts',(-26.3115589819965,13.0400249210017,
128.018983277286)) ;
#147296=CARTESIAN_POINT('Ctrl Pts',(-26.2812519148647,13.3449925039121,
127.963545408573)) ;
#147297=CARTESIAN_POINT('Ctrl Pts',(-26.2778797392448,13.6560824350963,
127.986850254171)) ;
#147298=CARTESIAN_POINT('Ctrl Pts',(-26.3008975455134,13.9495230290834,
128.087137834312)) ;
#147299=CARTESIAN_POINT('Ctrl Pts',(-26.3479782652609,14.2060602053469,
128.257797236022)) ;
#147300=CARTESIAN_POINT('Ctrl Pts',(-26.415271572287,14.4068533701998,128.487586750175)) ;
#147301=CARTESIAN_POINT('Ctrl Pts',(-26.4967691286776,14.5364834485285,
128.758756328545)) ;
#147302=CARTESIAN_POINT('Ctrl Pts',(-26.586194501111,14.5865952297017,129.053116471795)) ;
#147303=CARTESIAN_POINT('Ctrl Pts',(-26.6763590123459,14.553289693682,129.349636823295)) ;
#147304=CARTESIAN_POINT('Ctrl Pts',(-26.7600228764154,14.4391769973074,
129.627142397581)) ;
#147305=CARTESIAN_POINT('Ctrl Pts',(-26.8305563269227,14.2521193924325,
129.866320001124)) ;
#147306=CARTESIAN_POINT('Ctrl Pts',(-26.8821056983442,14.0064610013992,
130.049955365184)) ;
#147307=CARTESIAN_POINT('Ctrl Pts',(-26.9104630889835,13.7162751839027,
130.166152471987)) ;
#147308=CARTESIAN_POINT('Ctrl Pts',(-26.9124439133158,13.4088590372776,
130.204864159524)) ;
#147309=CARTESIAN_POINT('Ctrl Pts',(-26.8876203324447,13.1005339015723,
130.165487747714)) ;
#147310=CARTESIAN_POINT('Ctrl Pts',(-26.8367036547029,12.8153801442626,
130.049891561204)) ;
#147311=CARTESIAN_POINT('Ctrl Pts',(-26.7630941930023,12.5742829419459,
129.867895511603)) ;
#147312=CARTESIAN_POINT('Ctrl Pts',(-26.6700181781098,12.3924207775489,
129.62937532917)) ;
#147313=CARTESIAN_POINT('Ctrl Pts',(-26.5657046350372,12.2864008537638,
129.357568602088)) ;
#147314=CARTESIAN_POINT('Ctrl Pts',(-26.4545900751574,12.2608494079679,
129.066227997659)) ;
#147315=CARTESIAN_POINT('Ctrl Pts',(-26.345767615669,12.3186106579848,128.781313857206)) ;
#147316=CARTESIAN_POINT('Ctrl Pts',(-26.2448324759386,12.4554523175926,
128.519622374665)) ;
#147317=CARTESIAN_POINT('Ctrl Pts',(-26.1588332332188,12.6626735352652,
128.301638928963)) ;
#147318=CARTESIAN_POINT('Ctrl Pts',(-26.0938900095568,12.9221025997255,
128.144867830553)) ;
#147319=CARTESIAN_POINT('Ctrl Pts',(-26.0527924934696,13.2188658748081,
128.057962797512)) ;
#147320=CARTESIAN_POINT('Ctrl Pts',(-26.0384362022978,13.5309969609299,
128.049243549581)) ;
#147321=CARTESIAN_POINT('Ctrl Pts',(-26.0508964161626,13.8333910291505,
128.118640022779)) ;
#147322=CARTESIAN_POINT('Ctrl Pts',(-26.0887248099249,14.1082732516314,
128.262358068777)) ;
#147323=CARTESIAN_POINT('Ctrl Pts',(-26.1483616887784,14.3332733930533,
128.469696784862)) ;
#147324=CARTESIAN_POINT('Ctrl Pts',(-26.2248538967359,14.4930899265818,
128.726293642741)) ;
#147325=CARTESIAN_POINT('Ctrl Pts',(-26.3117593915966,14.5762694731203,
129.013227399328)) ;
#147326=CARTESIAN_POINT('Ctrl Pts',(-26.4029117585351,14.5766426477847,
129.3127891345)) ;
#147327=CARTESIAN_POINT('Ctrl Pts',(-26.4895350988602,14.4950561808568,
129.598750745687)) ;
#147328=CARTESIAN_POINT('Ctrl Pts',(-26.5665136204875,14.3357812745788,
129.856885878982)) ;
#147329=CARTESIAN_POINT('Ctrl Pts',(-26.6262592796755,14.1117726317635,
130.064489680492)) ;
#147330=CARTESIAN_POINT('Ctrl Pts',(-26.664428327791,13.8385112435954,130.209095717924)) ;
#147331=CARTESIAN_POINT('Ctrl Pts',(-26.6772984039839,13.5338962434735,
130.27996038854)) ;
#147332=CARTESIAN_POINT('Ctrl Pts',(-26.6633735809435,13.2242575692473,
130.272227496551)) ;
#147333=CARTESIAN_POINT('Ctrl Pts',(-26.6226746960282,12.9262819012927,
130.18657442431)) ;
#147334=CARTESIAN_POINT('Ctrl Pts',(-26.5578472919816,12.6654698435916,
130.03022959216)) ;
#147335=CARTESIAN_POINT('Ctrl Pts',(-26.4718376309163,12.4574146101121,
129.812281248977)) ;
#147336=CARTESIAN_POINT('Ctrl Pts',(-26.3720422424379,12.3205165550688,
129.553606148421)) ;
#147337=CARTESIAN_POINT('Ctrl Pts',(-26.2623404084189,12.2610390468186,
129.266423763094)) ;
#147338=CARTESIAN_POINT('Ctrl Pts',(-26.1520390344193,12.2851065141721,
128.97719162075)) ;
#147339=CARTESIAN_POINT('Ctrl Pts',(-26.0464052214175,12.3913707511119,
128.701919778819)) ;
#147340=CARTESIAN_POINT('Ctrl Pts',(-25.9542397322552,12.5705078775683,
128.465670763245)) ;
#147341=CARTESIAN_POINT('Ctrl Pts',(-25.8800073520596,12.8110530886845,
128.281943454991)) ;
#147342=CARTESIAN_POINT('Ctrl Pts',(-25.8287174453691,13.0958080980136,
128.16526124174)) ;
#147343=CARTESIAN_POINT('Ctrl Pts',(-25.8034286370072,13.4043791366155,
128.124575677788)) ;
#147344=CARTESIAN_POINT('Ctrl Pts',(-25.8050680904062,13.7127503618814,
128.162374639568)) ;
#147345=CARTESIAN_POINT('Ctrl Pts',(-25.8331792366338,14.0031465413693,
128.277846201473)) ;
#147346=CARTESIAN_POINT('Ctrl Pts',(-25.8840548911354,14.2480984891944,
128.459304631545)) ;
#147347=CARTESIAN_POINT('Ctrl Pts',(-25.9545856190801,14.4370589148149,
128.698609955357)) ;
#147348=CARTESIAN_POINT('Ctrl Pts',(-26.0380121218444,14.5521322470153,
128.975377743495)) ;
#147349=CARTESIAN_POINT('Ctrl Pts',(-26.1283292300662,14.5867077632741,
129.272419970589)) ;
#147350=CARTESIAN_POINT('Ctrl Pts',(-26.2176425716056,14.5378478961583,
129.566384402424)) ;
#147351=CARTESIAN_POINT('Ctrl Pts',(-26.2993554539816,14.4092030329905,
129.838211853804)) ;
#147352=CARTESIAN_POINT('Ctrl Pts',(-26.3667060054575,14.2102655256447,
130.068042548754)) ;
#147353=CARTESIAN_POINT('Ctrl Pts',(-26.4143965075339,13.953116489833,130.240663994916)) ;
#147354=CARTESIAN_POINT('Ctrl Pts',(-26.4376848856322,13.6605445363077,
130.341677819469)) ;
#147355=CARTESIAN_POINT('Ctrl Pts',(-26.4347158653785,13.3493859858442,
130.366180421727)) ;
#147356=CARTESIAN_POINT('Ctrl Pts',(-26.4048124301675,13.0444135456855,
130.311894349898)) ;
#147357=CARTESIAN_POINT('Ctrl Pts',(-26.3493229430599,12.7658508988887,
130.182947087287)) ;
#147358=CARTESIAN_POINT('Ctrl Pts',(-26.2715830488278,12.5346698659633,
129.988965884616)) ;
#147359=CARTESIAN_POINT('Ctrl Pts',(-26.1762853786461,12.3668713025773,
129.743737589104)) ;
#147360=CARTESIAN_POINT('Ctrl Pts',(-26.069606670302,12.2750736510529,129.465261546678)) ;
#147361=CARTESIAN_POINT('Ctrl Pts',(-25.9590624120991,12.2654123837922,
129.175324576531)) ;
#147362=CARTESIAN_POINT('Ctrl Pts',(-25.8507386841537,12.3385001121927,
128.89203884047)) ;
#147363=CARTESIAN_POINT('Ctrl Pts',(-25.7523129533691,12.4893940977294,
128.637638133927)) ;
#147364=CARTESIAN_POINT('Ctrl Pts',(-25.6700022058392,12.7071835395625,
128.430318876464)) ;
#147365=CARTESIAN_POINT('Ctrl Pts',(-25.6090294076232,12.9760086815988,
128.285301835029)) ;
#147366=CARTESIAN_POINT('Ctrl Pts',(-25.5729252411528,13.2771671350434,
128.212971047945)) ;
#147367=CARTESIAN_POINT('Ctrl Pts',(-25.5636314421838,13.5885363726329,
128.218931944683)) ;
#147368=CARTESIAN_POINT('Ctrl Pts',(-25.5810657627957,13.8883474938027,
128.303005296954)) ;
#147369=CARTESIAN_POINT('Ctrl Pts',(-25.6232704125892,14.1546797324028,
128.45942516704)) ;
#147370=CARTESIAN_POINT('Ctrl Pts',(-25.6864051786995,14.3683945164845,
128.676955004146)) ;
#147371=CARTESIAN_POINT('Ctrl Pts',(-25.7652853789973,14.5146640414989,
128.940493836316)) ;
#147372=CARTESIAN_POINT('Ctrl Pts',(-25.8538439793988,14.5827891573481,
129.232415670476)) ;
#147373=CARTESIAN_POINT('Ctrl Pts',(-25.9443062053087,14.5676065967762,
129.52974540677)) ;
#147374=CARTESIAN_POINT('Ctrl Pts',(-26.0299884903879,14.4706131159399,
129.813160378237)) ;
#147375=CARTESIAN_POINT('Ctrl Pts',(-26.1039155103848,14.2987449000821,
130.062221274369)) ;
#147376=CARTESIAN_POINT('Ctrl Pts',(-26.1602098677861,14.063095802434,130.259906440819)) ;
#147377=CARTESIAN_POINT('Ctrl Pts',(-26.1937049681925,13.7833208359645,
130.390765918343)) ;
#147378=CARTESIAN_POINT('Ctrl Pts',(-26.2016332025184,13.4754883225496,
130.447200559689)) ;
#147379=CARTESIAN_POINT('Ctrl Pts',(-26.182591675332,13.1664272763286,130.424565803854)) ;
#147380=CARTESIAN_POINT('Ctrl Pts',(-26.1372145619655,12.8743475214726,
130.325153027451)) ;
#147381=CARTESIAN_POINT('Ctrl Pts',(-26.0681100485298,12.6220180673462,
130.156364599778)) ;
#147382=CARTESIAN_POINT('Ctrl Pts',(-25.9791355180504,12.4263341483682,
129.929648965762)) ;
#147383=CARTESIAN_POINT('Ctrl Pts',(-25.8762687412122,12.302605659073,129.662304783115)) ;
#147384=CARTESIAN_POINT('Ctrl Pts',(-25.7664265682515,12.2593725247806,
129.374490277057)) ;
#147385=CARTESIAN_POINT('Ctrl Pts',(-25.6565009947126,12.2987734021689,
129.086399334671)) ;
#147386=CARTESIAN_POINT('Ctrl Pts',(-25.5525415623039,12.4202091773167,
128.816083115814)) ;
#147387=CARTESIAN_POINT('Ctrl Pts',(-25.463523806087,12.6117736562181,128.588993280005)) ;
#147388=CARTESIAN_POINT('Ctrl Pts',(-25.3931975895658,12.8626551569237,
128.416749070774)) ;
#147389=CARTESIAN_POINT('Ctrl Pts',(-25.3468388426278,13.1527448320073,
128.314381265538)) ;
#147390=CARTESIAN_POINT('Ctrl Pts',(-25.3265594515291,13.4624297819909,
128.288238626184)) ;
#147391=CARTESIAN_POINT('Ctrl Pts',(-25.333337476772,13.7701810821573,128.34123302125)) ;
#147392=CARTESIAN_POINT('Ctrl Pts',(-25.3658008060248,14.0517728376964,
128.469114625698)) ;
#147393=CARTESIAN_POINT('Ctrl Pts',(-25.4210139847123,14.2892526795151,
128.663546384413)) ;
#147394=CARTESIAN_POINT('Ctrl Pts',(-25.4945519789554,14.4648240216747,
128.911599442644)) ;
#147395=CARTESIAN_POINT('Ctrl Pts',(-25.579674277019,14.5650403080843,129.193298266083)) ;
#147396=CARTESIAN_POINT('Ctrl Pts',(-25.67036522595,14.5837489578772,129.491409968998)) ;
#147397=CARTESIAN_POINT('Ctrl Pts',(-25.7585912679521,14.519716790758,129.782133273891)) ;
#147398=CARTESIAN_POINT('Ctrl Pts',(-25.8383866398907,14.3763314788885,
130.04848919323)) ;
#147399=CARTESIAN_POINT('Ctrl Pts',(-25.9022469285143,14.1656645339802,
130.26807856477)) ;
#147400=CARTESIAN_POINT('Ctrl Pts',(-25.9456274021111,13.8999128484359,
130.428097361213)) ;
#147401=CARTESIAN_POINT('Ctrl Pts',(-25.9640567630253,13.6028235446839,
130.514880792807)) ;
#147402=CARTESIAN_POINT('Ctrl Pts',(-25.9560293185912,13.291184558806,130.5245814653)) ;
#147403=CARTESIAN_POINT('Ctrl Pts',(-25.9211626506794,12.9894030516706,
130.455825428731)) ;
#147404=CARTESIAN_POINT('Ctrl Pts',(-25.8610673900144,12.7177659651588,
130.313481364272)) ;
#147405=CARTESIAN_POINT('Ctrl Pts',(-25.7793965335319,12.49725897855,130.108081193746)) ;
#147406=CARTESIAN_POINT('Ctrl Pts',(-25.6820096977712,12.3438957408669,
129.856561080609)) ;
#147407=CARTESIAN_POINT('Ctrl Pts',(-25.5739096114305,12.2668705214432,
129.573956876957)) ;
#147408=CARTESIAN_POINT('Ctrl Pts',(-25.4630100257819,12.2729078136877,
129.283075556305)) ;
#147409=CARTESIAN_POINT('Ctrl Pts',(-25.356027244478,12.3614501444855,129.003710369665)) ;
#147410=CARTESIAN_POINT('Ctrl Pts',(-25.2604256897816,12.5253315069565,
128.757464536731)) ;
#147411=CARTESIAN_POINT('Ctrl Pts',(-25.1814030954091,12.75527704082,128.559915933982)) ;
#147412=CARTESIAN_POINT('Ctrl Pts',(-25.1251196612894,13.0310569738766,
128.428504091722)) ;
#147413=CARTESIAN_POINT('Ctrl Pts',(-25.0939685502416,13.336121760913,128.370672083575)) ;
#147414=CARTESIAN_POINT('Ctrl Pts',(-25.089777654312,13.6463105031288,128.39146772838)) ;
#147415=CARTESIAN_POINT('Ctrl Pts',(-25.1121607797936,13.942487386476,128.490115395761)) ;
#147416=CARTESIAN_POINT('Ctrl Pts',(-25.1587979741093,14.2002009126819,
128.659500935617)) ;
#147417=CARTESIAN_POINT('Ctrl Pts',(-25.2251350521265,14.4015262560108,
128.886278135871)) ;
#147418=CARTESIAN_POINT('Ctrl Pts',(-25.3065076717985,14.5339054968789,
129.157180214865)) ;
#147419=CARTESIAN_POINT('Ctrl Pts',(-25.3957504816741,14.5863178640126,
129.450982591655)) ;
#147420=CARTESIAN_POINT('Ctrl Pts',(-25.4862345240099,14.5553221759541,
129.748523545111)) ;
#147421=CARTESIAN_POINT('Ctrl Pts',(-25.5701152155034,14.4431215041297,
130.026657665419)) ;
#147422=CARTESIAN_POINT('Ctrl Pts',(-25.6408625622055,14.2589451929284,
130.266317223022)) ;
#147423=CARTESIAN_POINT('Ctrl Pts',(-25.6932705534346,14.0132050920919,
130.452661573645)) ;
#147424=CARTESIAN_POINT('Ctrl Pts',(-25.7221401451884,13.7264814749198,
130.570060326567)) ;
#147425=CARTESIAN_POINT('Ctrl Pts',(-25.7249810058714,13.4166671234753,
130.611582683641)) ;
#147426=CARTESIAN_POINT('Ctrl Pts',(-25.7008673309746,13.1090562116308,
130.57416706686)) ;
#147427=CARTESIAN_POINT('Ctrl Pts',(-25.650705201746,12.82289367226,130.460777367842)) ;
#147428=CARTESIAN_POINT('Ctrl Pts',(-25.5776200733177,12.5803482566307,
130.280325138346)) ;
#147429=CARTESIAN_POINT('Ctrl Pts',(-25.4854578756859,12.3971382864686,
130.044324611692)) ;
#147430=CARTESIAN_POINT('Ctrl Pts',(-25.3808890229052,12.2881794770673,
129.771944567501)) ;
#147431=CARTESIAN_POINT('Ctrl Pts',(-25.2700108769558,12.2604447735571,
129.481239923333)) ;
#147432=CARTESIAN_POINT('Ctrl Pts',(-25.1608183013244,12.3158800471475,
129.195310553149)) ;
#147433=CARTESIAN_POINT('Ctrl Pts',(-25.0594670901994,12.4512316162553,
128.932457223453)) ;
#147434=CARTESIAN_POINT('Ctrl Pts',(-24.9736427412008,12.6546809483565,
128.714694415)) ;
#147435=CARTESIAN_POINT('Ctrl Pts',(-24.9074766800191,12.9147731293523,
128.554622339809)) ;
#147436=CARTESIAN_POINT('Ctrl Pts',(-24.8658875479562,13.2095559485039,
128.466127574624)) ;
#147437=CARTESIAN_POINT('Ctrl Pts',(-24.850668730366,13.5223874270332,128.454982787526)) ;
#147438=CARTESIAN_POINT('Ctrl Pts',(-24.862374550478,13.825017500004,128.522137475361)) ;
#147439=CARTESIAN_POINT('Ctrl Pts',(-24.899721165262,14.1019895669497,128.66457954536)) ;
#147440=CARTESIAN_POINT('Ctrl Pts',(-24.9585507005245,14.3273312659445,
128.869390260325)) ;
#147441=CARTESIAN_POINT('Ctrl Pts',(-25.0345366141788,14.4893435493457,
129.124486798499)) ;
#147442=CARTESIAN_POINT('Ctrl Pts',(-25.1213275613785,14.5749600096558,
129.411124229977)) ;
#147443=CARTESIAN_POINT('Ctrl Pts',(-25.2123749716485,14.5779281254001,
129.710338631677)) ;
#147444=CARTESIAN_POINT('Ctrl Pts',(-25.2994338403886,14.4983365281884,
129.997670388463)) ;
#147445=CARTESIAN_POINT('Ctrl Pts',(-25.3764852172115,14.3420896185929,
130.255855966299)) ;
#147446=CARTESIAN_POINT('Ctrl Pts',(-25.4372612466155,14.1180211548404,
130.466732396769)) ;
#147447=CARTESIAN_POINT('Ctrl Pts',(-25.4757954504626,13.8471808602615,
130.612225812772)) ;
#147448=CARTESIAN_POINT('Ctrl Pts',(-25.4895325193993,13.5439413026185,
130.685549031096)) ;
#147449=CARTESIAN_POINT('Ctrl Pts',(-25.4763877137705,13.2331634650753,
130.680205857451)) ;
#147450=CARTESIAN_POINT('Ctrl Pts',(-25.436417688245,12.9343808446189,130.59668869728)) ;
#147451=CARTESIAN_POINT('Ctrl Pts',(-25.3721536694258,12.672197812707,130.442015902959)) ;
#147452=CARTESIAN_POINT('Ctrl Pts',(-25.2871759098898,12.4632419540624,
130.226903985326)) ;
#147453=CARTESIAN_POINT('Ctrl Pts',(-25.1871271731951,12.3231158661213,
129.96769991366)) ;
#147454=CARTESIAN_POINT('Ctrl Pts',(-25.0775746371766,12.2616017897263,
129.680943711049)) ;
#147455=CARTESIAN_POINT('Ctrl Pts',(-24.9674177556154,12.2833201820527,
129.392078348861)) ;
#147456=CARTESIAN_POINT('Ctrl Pts',(-24.8617121590519,12.3868877345153,
129.116527833986)) ;
#147457=CARTESIAN_POINT('Ctrl Pts',(-24.7686713370083,12.5648231371291,
128.877870667661)) ;
#147458=CARTESIAN_POINT('Ctrl Pts',(-24.6939731377639,12.8039602179339,
128.692766032637)) ;
#147459=CARTESIAN_POINT('Ctrl Pts',(-24.6421512068702,13.0864729050957,
128.57439142321)) ;
#147460=CARTESIAN_POINT('Ctrl Pts',(-24.6159486541681,13.3957238460679,
128.531150167993)) ;
#147461=CARTESIAN_POINT('Ctrl Pts',(-24.6169248165692,13.7038340446914,
128.566964483066)) ;
#147462=CARTESIAN_POINT('Ctrl Pts',(-24.6439310731031,13.9936201440332,
128.678997984667)) ;
#147463=CARTESIAN_POINT('Ctrl Pts',(-24.694875907643,14.2431366555827,128.861092575931)) ;
#147464=CARTESIAN_POINT('Ctrl Pts',(-24.7642561700479,14.4318623927357,
129.096682946381)) ;
#147465=CARTESIAN_POINT('Ctrl Pts',(-24.847909290222,14.5502397441639,129.374344984616)) ;
#147466=CARTESIAN_POINT('Ctrl Pts',(-24.9379186092033,14.5868194745111,
129.670393657069)) ;
#147467=CARTESIAN_POINT('Ctrl Pts',(-25.0274560736447,14.5403267792944,
129.96505775103)) ;
#147468=CARTESIAN_POINT('Ctrl Pts',(-25.1094619526943,14.4138414926087,
130.237727564842)) ;
#147469=CARTESIAN_POINT('Ctrl Pts',(-25.1773154114334,14.2163546967306,
130.469065398273)) ;
#147470=CARTESIAN_POINT('Ctrl Pts',(-25.2253773054646,13.962464783628,130.642541368542)) ;
#147471=CARTESIAN_POINT('Ctrl Pts',(-25.24961618706,13.6693367580008,130.746502542024)) ;
#147472=CARTESIAN_POINT('Ctrl Pts',(-25.2474068337107,13.3586798418074,
130.773184087954)) ;
#147473=CARTESIAN_POINT('Ctrl Pts',(-25.2182356406182,13.0526929530247,
130.721098440752)) ;
#147474=CARTESIAN_POINT('Ctrl Pts',(-25.1634305798166,12.7731728077457,
130.594139490751)) ;
#147475=CARTESIAN_POINT('Ctrl Pts',(-25.0862589189529,12.5404162023862,
130.401820361483)) ;
#147476=CARTESIAN_POINT('Ctrl Pts',(-24.9914844710839,12.3707607989948,
130.158084215147)) ;
#147477=CARTESIAN_POINT('Ctrl Pts',(-24.8850624365054,12.2766729601255,
129.880354699258)) ;
#147478=CARTESIAN_POINT('Ctrl Pts',(-24.7745883557454,12.2643218460961,
129.59060471869)) ;
#147479=CARTESIAN_POINT('Ctrl Pts',(-24.665300865596,12.3360206522436,129.304757619663)) ;
#147480=CARTESIAN_POINT('Ctrl Pts',(-24.5674413550508,12.4836397048973,
129.051702486663)) ;
#147481=CARTESIAN_POINT('Ctrl Pts',(-24.4841980631826,12.7003319185399,
128.841794655393)) ;
#147482=CARTESIAN_POINT('Ctrl Pts',(-24.4226430737707,12.9678917727225,
128.695053256231)) ;
#147483=CARTESIAN_POINT('Ctrl Pts',(-24.3857571441025,13.2687869300656,
128.62048000068)) ;
#147484=CARTESIAN_POINT('Ctrl Pts',(-24.3757550894969,13.5800035034693,
128.624353835401)) ;
#147485=CARTESIAN_POINT('Ctrl Pts',(-24.3924109780588,13.8799729722643,
128.706099674378)) ;
#147486=CARTESIAN_POINT('Ctrl Pts',(-24.4339595637666,14.14769940646,128.860620861967)) ;
#147487=CARTESIAN_POINT('Ctrl Pts',(-24.4965774264268,14.3632524598664,
129.076651664713)) ;
#147488=CARTESIAN_POINT('Ctrl Pts',(-24.5753469438563,14.511933585639,129.339964185627)) ;
#147489=CARTESIAN_POINT('Ctrl Pts',(-24.6636723624433,14.5819602156047,
129.631172820673)) ;
#147490=CARTESIAN_POINT('Ctrl Pts',(-24.7538880579223,14.5692454320411,
129.927679411565)) ;
#147491=CARTESIAN_POINT('Ctrl Pts',(-24.8400111036722,14.4742854665662,
130.212461777541)) ;
#147492=CARTESIAN_POINT('Ctrl Pts',(-24.9141474049248,14.3047439211162,
130.462048740383)) ;
#147493=CARTESIAN_POINT('Ctrl Pts',(-24.9710435495452,14.0710831127117,
130.66146131265)) ;
#147494=CARTESIAN_POINT('Ctrl Pts',(-25.0053326588705,13.7914036460412,
130.794750491077)) ;
#147495=CARTESIAN_POINT('Ctrl Pts',(-25.0139823256091,13.4850123175133,
130.853182599625)) ;
#147496=CARTESIAN_POINT('Ctrl Pts',(-24.9957867875723,13.1755843986706,
130.833035511702)) ;
#147497=CARTESIAN_POINT('Ctrl Pts',(-24.9510844064904,12.8823157698566,
130.735635283545)) ;
#147498=CARTESIAN_POINT('Ctrl Pts',(-24.8826220204888,12.628436297888,130.568728677609)) ;
#147499=CARTESIAN_POINT('Ctrl Pts',(-24.7937281426364,12.4304595196238,
130.342377740803)) ;
#147500=CARTESIAN_POINT('Ctrl Pts',(-24.6919949244802,12.3053999531995,
130.078078985158)) ;
#147501=CARTESIAN_POINT('Ctrl Pts',(-24.5813762118716,12.2593484395974,
129.788270620212)) ;
#147502=CARTESIAN_POINT('Ctrl Pts',(-24.4718806439112,12.2965483924972,
129.501275586179)) ;
#147503=CARTESIAN_POINT('Ctrl Pts',(-24.3675517835472,12.4156949312687,
129.229904709214)) ;
#147504=CARTESIAN_POINT('Ctrl Pts',(-24.2781540160857,12.6050470802083,
129.001655484171)) ;
#147505=CARTESIAN_POINT('Ctrl Pts',(-24.2070200380848,12.8553420969347,
128.827159977025)) ;
#147506=CARTESIAN_POINT('Ctrl Pts',(-24.1601461823753,13.14294545291,128.723103202303)) ;
#147507=CARTESIAN_POINT('Ctrl Pts',(-24.1389317962829,13.4543916932758,
128.694450505378)) ;
#147508=CARTESIAN_POINT('Ctrl Pts',(-24.1449949752851,13.7614619882681,
128.745238827839)) ;
#147509=CARTESIAN_POINT('Ctrl Pts',(-24.1768158430516,14.0447128123048,
128.871321579809)) ;
#147510=CARTESIAN_POINT('Ctrl Pts',(-24.231333547993,14.2828872878416,129.063626721277)) ;
#147511=CARTESIAN_POINT('Ctrl Pts',(-24.3041010172989,14.4603132279032,
129.309318834514)) ;
#147512=CARTESIAN_POINT('Ctrl Pts',(-24.3896352702838,14.5634617408265,
129.592480733006)) ;
#147513=CARTESIAN_POINT('Ctrl Pts',(-24.4795823186102,14.5844329912441,
129.888156786475)) ;
#147514=CARTESIAN_POINT('Ctrl Pts',(-24.5685724115342,14.5225343527704,
130.181342201958)) ;
#147515=CARTESIAN_POINT('Ctrl Pts',(-24.6484337252993,14.3815448492318,
130.447775913898)) ;
#147516=CARTESIAN_POINT('Ctrl Pts',(-24.7128675060765,14.172575531033,130.669066255997)) ;
#147517=CARTESIAN_POINT('Ctrl Pts',(-24.7567752762927,13.9093041266096,
130.830484961807)) ;
#147518=CARTESIAN_POINT('Ctrl Pts',(-24.7761511782523,13.6121559231782,
130.920131335962)) ;
#147519=CARTESIAN_POINT('Ctrl Pts',(-24.7687788447022,13.2990171970743,
130.93190911656)) ;
#147520=CARTESIAN_POINT('Ctrl Pts',(-24.7347587150341,12.998156604328,130.865468282676)) ;
#147521=CARTESIAN_POINT('Ctrl Pts',(-24.6755494930383,12.7257033246492,
130.725651376967)) ;
#147522=CARTESIAN_POINT('Ctrl Pts',(-24.5943950553872,12.5030758718665,
130.521797413364)) ;
#147523=CARTESIAN_POINT('Ctrl Pts',(-24.4972021110052,12.3471530104355,
130.270914197217)) ;
#147524=CARTESIAN_POINT('Ctrl Pts',(-24.3888920694182,12.2678408684918,
129.987814315935)) ;
#147525=CARTESIAN_POINT('Ctrl Pts',(-24.2786242157361,12.2715869144481,
129.698586587052)) ;
#147526=CARTESIAN_POINT('Ctrl Pts',(-24.1712851072626,12.3575775842601,
129.41821433343)) ;
#147527=CARTESIAN_POINT('Ctrl Pts',(-24.075122506587,12.5198591790598,129.170392897351)) ;
#147528=CARTESIAN_POINT('Ctrl Pts',(-23.9957490620432,12.7472700388984,
128.971705039795)) ;
#147529=CARTESIAN_POINT('Ctrl Pts',(-23.9384956276451,13.0233714187906,
128.837633345603)) ;
#147530=CARTESIAN_POINT('Ctrl Pts',(-23.906768899648,13.3264774895314,128.777955771663)) ;
#147531=CARTESIAN_POINT('Ctrl Pts',(-23.9017175998981,13.6374828806093,
128.796312918205)) ;
#147532=CARTESIAN_POINT('Ctrl Pts',(-23.9233630582439,13.9340522489258,
128.892767015105)) ;
#147533=CARTESIAN_POINT('Ctrl Pts',(-23.9692246158357,14.1931239362593,
129.059859846587)) ;
#147534=CARTESIAN_POINT('Ctrl Pts',(-24.0355476616512,14.3974304653898,
129.286818250949)) ;
#147535=CARTESIAN_POINT('Ctrl Pts',(-24.1161188310183,14.5309245418109,
129.55517001156)) ;
#147536=CARTESIAN_POINT('Ctrl Pts',(-24.2052743323323,14.5859814534191,
129.848744590398)) ;
#147537=CARTESIAN_POINT('Ctrl Pts',(-24.2956465504689,14.5574777864012,
130.145891527965)) ;
#147538=CARTESIAN_POINT('Ctrl Pts',(-24.3798737732299,14.448015060185,130.425034900643)) ;
#147539=CARTESIAN_POINT('Ctrl Pts',(-24.4515521270911,14.2640746959558,
130.667673308155)) ;
#147540=CARTESIAN_POINT('Ctrl Pts',(-24.504086412636,14.0222278715719,130.854058913168)) ;
#147541=CARTESIAN_POINT('Ctrl Pts',(-24.5339722227007,13.733909228241,130.974734762504)) ;
#147542=CARTESIAN_POINT('Ctrl Pts',(-24.5374751707681,13.4264443346404,
131.017960330213)) ;
#147543=CARTESIAN_POINT('Ctrl Pts',(-24.5141880982397,13.1179337320863,
130.98302610922)) ;
#147544=CARTESIAN_POINT('Ctrl Pts',(-24.4647870843601,12.8308236550973,
130.87184558373)) ;
#147545=CARTESIAN_POINT('Ctrl Pts',(-24.3919588197093,12.5859821218942,
130.692280995326)) ;
#147546=CARTESIAN_POINT('Ctrl Pts',(-24.3009187620074,12.4020104650746,
130.459321123967)) ;
#147547=CARTESIAN_POINT('Ctrl Pts',(-24.1959717032129,12.289987565929,130.186054381331)) ;
#147548=CARTESIAN_POINT('Ctrl Pts',(-24.0857390473135,12.2601247779834,
129.897056302984)) ;
#147549=CARTESIAN_POINT('Ctrl Pts',(-23.9762171103296,12.3130229005744,
129.610225108169)) ;
#147550=CARTESIAN_POINT('Ctrl Pts',(-23.8747284259677,12.4457555473525,
129.34689389739)) ;
#147551=CARTESIAN_POINT('Ctrl Pts',(-23.7880521676098,12.6478748794645,
129.12675488543)) ;
#147552=CARTESIAN_POINT('Ctrl Pts',(-23.721103989264,12.9074235012635,128.964483450518)) ;
#147553=CARTESIAN_POINT('Ctrl Pts',(-23.6788842464701,13.2015879263547,
128.874152848765)) ;
#147554=CARTESIAN_POINT('Ctrl Pts',(-23.6629323939292,13.5132462059268,
128.860752059264)) ;
#147555=CARTESIAN_POINT('Ctrl Pts',(-23.6739570788282,13.8170404321959,
128.925997813721)) ;
#147556=CARTESIAN_POINT('Ctrl Pts',(-23.7102694152644,14.0930904001558,
129.065158549252)) ;
#147557=CARTESIAN_POINT('Ctrl Pts',(-23.7686960140215,14.3215764972773,
129.268960849726)) ;
#147558=CARTESIAN_POINT('Ctrl Pts',(-23.8445454380153,14.4860164278212,
129.523758037768)) ;
#147559=CARTESIAN_POINT('Ctrl Pts',(-23.9312213636041,14.573742198897,129.810089766075)) ;
#147560=CARTESIAN_POINT('Ctrl Pts',(-24.0220093823538,14.5789283396522,
130.108457949363)) ;
#147561=CARTESIAN_POINT('Ctrl Pts',(-24.109313917463,14.5018180377366,130.396514557441)) ;
#147562=CARTESIAN_POINT('Ctrl Pts',(-24.1869754969046,14.346557147794,130.656623143926)) ;
#147563=CARTESIAN_POINT('Ctrl Pts',(-24.2476549364385,14.1268974997841,
130.866828184463)) ;
#147564=CARTESIAN_POINT('Ctrl Pts',(-24.2873207213174,13.8551172342444,
131.015918349445)) ;
#147565=CARTESIAN_POINT('Ctrl Pts',(-24.3017140358187,13.5530513946411,
131.091077286669)) ;
#147566=CARTESIAN_POINT('Ctrl Pts',(-24.2893139396289,13.2415864711832,
131.087983566359)) ;
#147567=CARTESIAN_POINT('Ctrl Pts',(-24.250237975428,12.9431697313624,131.006954863297)) ;
#147568=CARTESIAN_POINT('Ctrl Pts',(-24.1865152004602,12.6789856337564,
130.853947378745)) ;
#147569=CARTESIAN_POINT('Ctrl Pts',(-24.1021542313126,12.4685393883903,
130.640594380605)) ;
#147570=CARTESIAN_POINT('Ctrl Pts',(-24.0024751379339,12.3261974816525,
130.382472154133)) ;
#147571=CARTESIAN_POINT('Ctrl Pts',(-23.8931586555059,12.2622045903834,
130.09638187146)) ;
#147572=CARTESIAN_POINT('Ctrl Pts',(-23.7827401832175,12.2815898228841,
129.806818174174)) ;
#147573=CARTESIAN_POINT('Ctrl Pts',(-23.6770976764349,12.3824517560788,
129.53134468171)) ;
#147574=CARTESIAN_POINT('Ctrl Pts',(-23.5834505310389,12.5585396734663,
129.290971302459)) ;
#147575=CARTESIAN_POINT('Ctrl Pts',(-23.508182467316,12.7954954768117,129.104139062345)) ;
#147576=CARTESIAN_POINT('Ctrl Pts',(-23.455285908669,13.0796939956766,128.982930941838)) ;
#147577=CARTESIAN_POINT('Ctrl Pts',(-23.4286311064434,13.3852304275537,
128.938001175148)) ;
#147578=CARTESIAN_POINT('Ctrl Pts',(-23.4287217575004,13.6960444491442,
128.971493246291)) ;
#147579=CARTESIAN_POINT('Ctrl Pts',(-23.4551013960019,13.9858667293059,
129.081617279581)) ;
#147580=CARTESIAN_POINT('Ctrl Pts',(-23.5051029609528,14.2358877355362,
129.26080876385)) ;
#147581=CARTESIAN_POINT('Ctrl Pts',(-23.5742887287595,14.4275999351318,
129.495985612575)) ;
#147582=CARTESIAN_POINT('Ctrl Pts',(-23.6577980269704,14.5480862866817,
129.773271676715)) ;
#147583=CARTESIAN_POINT('Ctrl Pts',(-23.7474018757379,14.5868446716621,
130.068022721532)) ;
#147584=CARTESIAN_POINT('Ctrl Pts',(-23.8369559093925,14.5430357669594,
130.362695615245)) ;
#147585=CARTESIAN_POINT('Ctrl Pts',(-23.9193924881052,14.4187440206734,
130.6366634839)) ;
#147586=CARTESIAN_POINT('Ctrl Pts',(-23.9878235278518,14.2230681613756,
130.869712210717)) ;
#147587=CARTESIAN_POINT('Ctrl Pts',(-24.0366005220974,13.9697197628044,
131.045375325504)) ;
#147588=CARTESIAN_POINT('Ctrl Pts',(-24.0614674762417,13.6787523584359,
131.15101843608)) ;
#147589=CARTESIAN_POINT('Ctrl Pts',(-24.0600609361775,13.3668523124778,
131.180201589393)) ;
#147590=CARTESIAN_POINT('Ctrl Pts',(-24.0315449778296,13.0606725090592,
131.130008882499)) ;
#147591=CARTESIAN_POINT('Ctrl Pts',(-23.9776458019882,12.7810811423454,
131.005579190731)) ;
#147592=CARTESIAN_POINT('Ctrl Pts',(-23.9011130557165,12.5467077639777,
130.815119966979)) ;
#147593=CARTESIAN_POINT('Ctrl Pts',(-23.8069768149252,12.3750360607571,
130.573192638211)) ;
#147594=CARTESIAN_POINT('Ctrl Pts',(-23.7001683995269,12.2779852511976,
130.29453089196)) ;
#147595=CARTESIAN_POINT('Ctrl Pts',(-23.5898763343155,12.2637459485192,
130.005268133567)) ;
#147596=CARTESIAN_POINT('Ctrl Pts',(-23.4811263606614,12.3321871592446,
129.720763770541)) ;
#147597=CARTESIAN_POINT('Ctrl Pts',(-23.3820175069721,12.4786899759448,
129.46433889727)) ;
#147598=CARTESIAN_POINT('Ctrl Pts',(-23.2983098747109,12.6941598777831,
129.253090432204)) ;
#147599=CARTESIAN_POINT('Ctrl Pts',(-23.2363410217116,12.9594897352697,
129.105015491517)) ;
#147600=CARTESIAN_POINT('Ctrl Pts',(-23.1986697974538,13.2597801817525,
129.028156015944)) ;
#147601=CARTESIAN_POINT('Ctrl Pts',(-23.1878842508862,13.5705932837916,
129.029699535421)) ;
#147602=CARTESIAN_POINT('Ctrl Pts',(-23.2037430688038,13.8717554022753,
129.109168701418)) ;
#147603=CARTESIAN_POINT('Ctrl Pts',(-23.2449054031129,14.1416796116284,
129.262708213378)) ;
#147604=CARTESIAN_POINT('Ctrl Pts',(-23.3066159094202,14.3575208228019,
129.475876783172)) ;
#147605=CARTESIAN_POINT('Ctrl Pts',(-23.3852205028398,14.5088742490897,
129.738811477045)) ;
#147606=CARTESIAN_POINT('Ctrl Pts',(-23.4731754167806,14.5810485839828,
130.028857377012)) ;
#147607=CARTESIAN_POINT('Ctrl Pts',(-23.5635550033295,14.57070182657,130.325899723339)) ;
#147608=CARTESIAN_POINT('Ctrl Pts',(-23.6496619348552,14.4785662715794,
130.610523033247)) ;
#147609=CARTESIAN_POINT('Ctrl Pts',(-23.7248247529453,14.3096046389662,
130.863384071564)) ;
#147610=CARTESIAN_POINT('Ctrl Pts',(-23.7820115470691,14.0777450263891,
131.063555946023)) ;
#147611=CARTESIAN_POINT('Ctrl Pts',(-23.8168619482178,13.8001342055984,
131.198371274251)) ;
#147612=CARTESIAN_POINT('Ctrl Pts',(-23.8263563634216,13.4946153250832,
131.25922816625)) ;
#147613=CARTESIAN_POINT('Ctrl Pts',(-23.8088367280898,13.1837407036183,
131.241195456402)) ;
#147614=CARTESIAN_POINT('Ctrl Pts',(-23.7649433507423,12.8901082598339,
131.146097057007)) ;
#147615=CARTESIAN_POINT('Ctrl Pts',(-23.6966251290329,12.6339160902113,
130.979788263205)) ;
#147616=CARTESIAN_POINT('Ctrl Pts',(-23.6095241543669,12.4365925755612,
130.758201152529)) ;
#147617=CARTESIAN_POINT('Ctrl Pts',(-23.5069538528283,12.3075969620248,
130.4918578891)) ;
#147618=CARTESIAN_POINT('Ctrl Pts',(-23.3974350400682,12.2595413696365,
130.204950867827)) ;
#147619=CARTESIAN_POINT('Ctrl Pts',(-23.2868288278412,12.294598124244,129.915031930311)) ;
#147620=CARTESIAN_POINT('Ctrl Pts',(-23.1832923441451,12.4101972582257,
129.645612469305)) ;
#147621=CARTESIAN_POINT('Ctrl Pts',(-23.0926759195256,12.5987159467278,
129.414061565499)) ;
#147622=CARTESIAN_POINT('Ctrl Pts',(-23.0212220550139,12.8461743732165,
129.238450204882)) ;
#147623=CARTESIAN_POINT('Ctrl Pts',(-22.9731430841991,13.1359262373299,
129.131228901704)) ;
#147624=CARTESIAN_POINT('Ctrl Pts',(-22.9514283043162,13.4447581486374,
129.100849561658)) ;
#147625=CARTESIAN_POINT('Ctrl Pts',(-22.9566735082346,13.7530929107791,
129.149350380603)) ;
#147626=CARTESIAN_POINT('Ctrl Pts',(-22.9876517295182,14.0362080368137,
129.27283351649)) ;
#147627=CARTESIAN_POINT('Ctrl Pts',(-23.0416755840538,14.2769559920641,
129.463810736857)) ;
#147628=CARTESIAN_POINT('Ctrl Pts',(-23.1141892209063,14.4563581826417,
129.708818632771)) ;
#147629=CARTESIAN_POINT('Ctrl Pts',(-23.1988829773585,14.5613193473425,
129.989308389901)) ;
#147630=CARTESIAN_POINT('Ctrl Pts',(-23.2893749967103,14.5851466761501,
130.286798104915)) ;
#147631=CARTESIAN_POINT('Ctrl Pts',(-23.3785630002914,14.5250094388502,
130.580592252952)) ;
#147632=CARTESIAN_POINT('Ctrl Pts',(-23.4583548680528,14.3871119239881,
130.846635045836)) ;
#147633=CARTESIAN_POINT('Ctrl Pts',(-23.5236585342063,14.1786613718342,
131.070664502412)) ;
#147634=CARTESIAN_POINT('Ctrl Pts',(-23.5679982643713,13.9181922141156,
131.233148618779)) ;
#147635=CARTESIAN_POINT('Ctrl Pts',(-23.5882190837167,13.6189923508217,
131.325572962413)) ;
#147636=CARTESIAN_POINT('Ctrl Pts',(-23.5816035000313,13.3089361907061,
131.339232711532)) ;
#147637=CARTESIAN_POINT('Ctrl Pts',(-23.5482741486513,13.0058325903369,
131.274990715579)) ;
#147638=CARTESIAN_POINT('Ctrl Pts',(-23.4894854786624,12.7318652754408,
131.136467121549)) ;
#147639=CARTESIAN_POINT('Ctrl Pts',(-23.4089831642771,12.5082426893396,
130.93445138261)) ;
#147640=CARTESIAN_POINT('Ctrl Pts',(-23.3125034670551,12.3508732586718,
130.685540079445)) ;
#147641=CARTESIAN_POINT('Ctrl Pts',(-23.2047609813718,12.269103649341,130.403995285876)) ;
#147642=CARTESIAN_POINT('Ctrl Pts',(-23.0939408644455,12.2702137268432,
130.113315971798)) ;
#147643=CARTESIAN_POINT('Ctrl Pts',(-22.98625125803,12.3542929865281,129.831968807891)) ;
#147644=CARTESIAN_POINT('Ctrl Pts',(-22.8899768708341,12.5141176451976,
129.583726131609)) ;
#147645=CARTESIAN_POINT('Ctrl Pts',(-22.8100908927799,12.739523408871,129.383506653874)) ;
#147646=CARTESIAN_POINT('Ctrl Pts',(-22.7521073762579,13.0142279275944,
129.247283138693)) ;
#147647=CARTESIAN_POINT('Ctrl Pts',(-22.7194937058142,13.3177662597612,
129.185120174962)) ;
#147648=CARTESIAN_POINT('Ctrl Pts',(-22.7137261666825,13.6286637364164,
129.201363001925)) ;
#147649=CARTESIAN_POINT('Ctrl Pts',(-22.7345204242546,13.925291864832,129.295246555959)) ;
#147650=CARTESIAN_POINT('Ctrl Pts',(-22.7797671843805,14.1860949701751,
129.460591241563)) ;
#147651=CARTESIAN_POINT('Ctrl Pts',(-22.8453023863681,14.39173242129,129.685135742378)) ;
#147652=CARTESIAN_POINT('Ctrl Pts',(-22.9258525518916,14.5282787439252,
129.953574723786)) ;
#147653=CARTESIAN_POINT('Ctrl Pts',(-23.0150519408169,14.5855538698207,
130.247337850803)) ;
#147654=CARTESIAN_POINT('Ctrl Pts',(-23.1052288897223,14.5594424200451,
130.54382032972)) ;
#147655=CARTESIAN_POINT('Ctrl Pts',(-23.1896555995475,14.4525338341733,
130.823512429026)) ;
#147656=CARTESIAN_POINT('Ctrl Pts',(-23.2619405515289,14.2704301925612,
131.067970264371)) ;
#147657=CARTESIAN_POINT('Ctrl Pts',(-23.3151218822301,14.029440480781,131.25631660837)) ;
#147658=CARTESIAN_POINT('Ctrl Pts',(-23.3456010904319,13.743952252976,131.378516130427)) ;
#147659=CARTESIAN_POINT('Ctrl Pts',(-23.3499839073277,13.4354033018238,
131.424474143209)) ;
#147660=CARTESIAN_POINT('Ctrl Pts',(-23.3274917765377,13.1268757888795,
131.391823283427)) ;
#147661=CARTESIAN_POINT('Ctrl Pts',(-23.2786246114809,12.8380942338867,
131.28230278294)) ;
#147662=CARTESIAN_POINT('Ctrl Pts',(-23.20686160686,12.5930207357232,131.105657440217)) ;
#147663=CARTESIAN_POINT('Ctrl Pts',(-23.1157309768258,12.406038862873,130.872640568249)) ;
#147664=CARTESIAN_POINT('Ctrl Pts',(-23.0119458727502,12.2925312371157,
130.602486998872)) ;
#147665=CARTESIAN_POINT('Ctrl Pts',(-22.9008788581356,12.2597001754449,
130.311334552258)) ;
#147666=CARTESIAN_POINT('Ctrl Pts',(-22.7914701328309,12.3104428537015,
130.024758576775)) ;
#147667=CARTESIAN_POINT('Ctrl Pts',(-22.6895482353747,12.4411375499462,
129.760200811099)) ;
#147668=CARTESIAN_POINT('Ctrl Pts',(-22.6025879552657,12.6410412531594,
129.539155276432)) ;
#147669=CARTESIAN_POINT('Ctrl Pts',(-22.5349468862704,12.8990709835383,
129.374854664712)) ;
#147670=CARTESIAN_POINT('Ctrl Pts',(-22.4919137164626,13.1932158971754,
129.282229595877)) ;
#147671=CARTESIAN_POINT('Ctrl Pts',(-22.4752413419626,13.5039483796779,
129.266639539968)) ;
#147672=CARTESIAN_POINT('Ctrl Pts',(-22.4854719189725,13.8084630012421,
129.32958919523)) ;
#147673=CARTESIAN_POINT('Ctrl Pts',(-22.5210896546395,14.0856215177356,
129.4667188073)) ;
#147674=CARTESIAN_POINT('Ctrl Pts',(-22.5789372654531,14.3156974280267,
129.668828273479)) ;
#147675=CARTESIAN_POINT('Ctrl Pts',(-22.6542125348602,14.4820692905758,
129.92188857157)) ;
#147676=CARTESIAN_POINT('Ctrl Pts',(-22.7408312256979,14.5722583385509,
130.208122077193)) ;
#147677=CARTESIAN_POINT('Ctrl Pts',(-22.8311475633563,14.5801736907429,
130.504940555016)) ;
#147678=CARTESIAN_POINT('Ctrl Pts',(-22.919292947113,14.5050113905237,130.795699735496)) ;
#147679=CARTESIAN_POINT('Ctrl Pts',(-22.9970588564607,14.3522165397239,
131.055996300533)) ;
#147680=CARTESIAN_POINT('Ctrl Pts',(-23.0584040842159,14.1339603470577,
131.26820660931)) ;
#147681=CARTESIAN_POINT('Ctrl Pts',(-23.0986746028439,13.8641113715177,
131.418974424778)) ;
#147682=CARTESIAN_POINT('Ctrl Pts',(-23.1139043155525,13.5616226074544,
131.496694305952)) ;
#147683=CARTESIAN_POINT('Ctrl Pts',(-23.1022497033995,13.2502935266874,
131.495755213587)) ;
#147684=CARTESIAN_POINT('Ctrl Pts',(-23.0638486364948,12.9509783477542,
131.416729306186)) ;
#147685=CARTESIAN_POINT('Ctrl Pts',(-23.0010006040838,12.686394956267,131.266167370427)) ;
#147686=CARTESIAN_POINT('Ctrl Pts',(-22.9170074500105,12.4734606665479,
131.053972327335)) ;
#147687=CARTESIAN_POINT('Ctrl Pts',(-22.8172294670306,12.3287824012662,
130.79569293947)) ;
#147688=CARTESIAN_POINT('Ctrl Pts',(-22.7086036821982,12.2629634134795,
130.511454266347)) ;
#147689=CARTESIAN_POINT('Ctrl Pts',(-22.5979567530543,12.2798963226628,
130.221280314733)) ;
#147690=CARTESIAN_POINT('Ctrl Pts',(-22.4920126410245,12.3786943874465,
129.944944100135)) ;
#147691=CARTESIAN_POINT('Ctrl Pts',(-22.3978375846003,12.5532637132079,
129.703077795437)) ;
#147692=CARTESIAN_POINT('Ctrl Pts',(-22.3223450400085,12.7879391796142,
129.515464838595)) ;
#147693=CARTESIAN_POINT('Ctrl Pts',(-22.2688664186441,13.0695371271683,
129.392394388671)) ;
#147694=CARTESIAN_POINT('Ctrl Pts',(-22.2411956279741,13.3764287043337,
129.344691810552)) ;
#147695=CARTESIAN_POINT('Ctrl Pts',(-22.2405807700061,13.6873693766845,
129.376111748844)) ;
#147696=CARTESIAN_POINT('Ctrl Pts',(-22.266182058288,13.9780097436375,129.483950839692)) ;
#147697=CARTESIAN_POINT('Ctrl Pts',(-22.3158295990549,14.2303816884254,
129.662248512627)) ;
#147698=CARTESIAN_POINT('Ctrl Pts',(-22.3843432444658,14.4229832272402,
129.895337579006)) ;
#147699=CARTESIAN_POINT('Ctrl Pts',(-22.467333378006,14.5456071982134,130.171033869882)) ;
#147700=CARTESIAN_POINT('Ctrl Pts',(-22.5569971155474,14.5869244372791,
130.466019745775)) ;
#147701=CARTESIAN_POINT('Ctrl Pts',(-22.6467207673819,14.5454139986495,
130.761210108266)) ;
#147702=CARTESIAN_POINT('Ctrl Pts',(-22.7294791899913,14.423161531977,131.036131544807)) ;
#147703=CARTESIAN_POINT('Ctrl Pts',(-22.7981835761643,14.2299646036066,
131.269878058976)) ;
#147704=CARTESIAN_POINT('Ctrl Pts',(-22.8476846979566,13.9782380445369,
131.447654268064)) ;
#147705=CARTESIAN_POINT('Ctrl Pts',(-22.8733293938664,13.6869896878631,
131.555692859271)) ;
#147706=CARTESIAN_POINT('Ctrl Pts',(-22.8727231487113,13.3772462538757,
131.587007151188)) ;
#147707=CARTESIAN_POINT('Ctrl Pts',(-22.8451132311897,13.0701026679002,
131.539509729341)) ;
#147708=CARTESIAN_POINT('Ctrl Pts',(-22.7917084880126,12.7883758090077,
131.416651622432)) ;
#147709=CARTESIAN_POINT('Ctrl Pts',(-22.715757237827,12.5524788411572,131.227885604995)) ;
#147710=CARTESIAN_POINT('Ctrl Pts',(-22.6218519763286,12.3787206196838,
130.986691296974)) ;
#147711=CARTESIAN_POINT('Ctrl Pts',(-22.5159330453895,12.2799428497071,
130.710427408907)) ;
#147712=CARTESIAN_POINT('Ctrl Pts',(-22.4054383279324,12.262781441409,130.420647289657)) ;
#147713=CARTESIAN_POINT('Ctrl Pts',(-22.2959303546471,12.3295044155471,
130.134111080986)) ;
#147714=CARTESIAN_POINT('Ctrl Pts',(-22.1969925695421,12.4735104244077,
129.878028751513)) ;
#147715=CARTESIAN_POINT('Ctrl Pts',(-22.1130241441533,12.6859035463297,
129.665868893032)) ;
#147716=CARTESIAN_POINT('Ctrl Pts',(-22.0500057240316,12.9511127833356,
129.514887939214)) ;
#147717=CARTESIAN_POINT('Ctrl Pts',(-22.0115779224571,13.2510041848706,
129.435841941698)) ;
#147718=CARTESIAN_POINT('Ctrl Pts',(-22.0000267466205,13.5624347972365,
129.435216595887)) ;
#147719=CARTESIAN_POINT('Ctrl Pts',(-22.0151986171199,13.8634350892771,
129.512606829949)) ;
#147720=CARTESIAN_POINT('Ctrl Pts',(-22.0553267596581,14.1332613456827,
129.662934327461)) ;
#147721=CARTESIAN_POINT('Ctrl Pts',(-22.1169164718532,14.352640956948,129.876004680242)) ;
#147722=CARTESIAN_POINT('Ctrl Pts',(-22.1950027878672,14.5054039533886,
130.137339400697)) ;
#147723=CARTESIAN_POINT('Ctrl Pts',(-22.2823946613197,14.5799567622948,
130.425612798528)) ;
#147724=CARTESIAN_POINT('Ctrl Pts',(-22.3731495143974,14.5723714233898,
130.723873707253)) ;
#147725=CARTESIAN_POINT('Ctrl Pts',(-22.4597690917796,14.4818104569399,
131.010120730261)) ;
#147726=CARTESIAN_POINT('Ctrl Pts',(-22.5347344779201,14.3163443098713,
131.262126357748)) ;
#147727=CARTESIAN_POINT('Ctrl Pts',(-22.5927669336754,14.085912079338,131.464853193877)) ;
#147728=CARTESIAN_POINT('Ctrl Pts',(-22.6284258357542,13.8088758328653,
131.602091135406)) ;
#147729=CARTESIAN_POINT('Ctrl Pts',(-22.6386507602744,13.502841633218,131.66518977333)) ;
#147730=CARTESIAN_POINT('Ctrl Pts',(-22.6219823717775,13.1931031291703,
131.649500274369)) ;
#147731=CARTESIAN_POINT('Ctrl Pts',(-22.5787183669213,12.8979592502217,
131.556328075628)) ;
#147732=CARTESIAN_POINT('Ctrl Pts',(-22.5114550363443,12.6415806855276,
131.392924286405)) ;
#147733=CARTESIAN_POINT('Ctrl Pts',(-22.4242650098309,12.4408172190554,
131.171318802838)) ;
#147734=CARTESIAN_POINT('Ctrl Pts',(-22.3219857137763,12.3100401605785,
130.90581289392)) ;
#147735=CARTESIAN_POINT('Ctrl Pts',(-22.2128212850724,12.2598615755304,
130.61987465851)) ;
#147736=CARTESIAN_POINT('Ctrl Pts',(-22.1023684792295,12.2922205439251,
130.330327430686)) ;
#147737=CARTESIAN_POINT('Ctrl Pts',(-21.9979975356662,12.4062484936796,
130.058648293658)) ;
#147738=CARTESIAN_POINT('Ctrl Pts',(-21.9071729863386,12.5927140648452,
129.826414994569)) ;
#147739=CARTESIAN_POINT('Ctrl Pts',(-21.8352773240707,12.8381488980971,
129.649442639516)) ;
#147740=CARTESIAN_POINT('Ctrl Pts',(-21.7864878410526,13.1260095389923,
129.540046596977)) ;
#147741=CARTESIAN_POINT('Ctrl Pts',(-21.763852701103,13.4367097243977,129.507212398852)) ;
#147742=CARTESIAN_POINT('Ctrl Pts',(-21.7683543624926,13.7438376738668,
129.553370845295)) ;
#147743=CARTESIAN_POINT('Ctrl Pts',(-21.7986360668358,14.0287736481255,
129.674910885284)) ;
#147744=CARTESIAN_POINT('Ctrl Pts',(-21.8521200037136,14.2709621687312,
129.864315089826)) ;
#147745=CARTESIAN_POINT('Ctrl Pts',(-21.9240424719339,14.4520607897228,
130.10753831961)) ;
#147746=CARTESIAN_POINT('Ctrl Pts',(-22.0086052791843,14.5594794390157,
130.387698164307)) ;
#147747=CARTESIAN_POINT('Ctrl Pts',(-22.0988545163125,14.5855261762896,
130.684415053406)) ;
#147748=CARTESIAN_POINT('Ctrl Pts',(-22.1879797716456,14.5283738832722,
130.977932444029)) ;
#147749=CARTESIAN_POINT('Ctrl Pts',(-22.268629541142,14.391653643749,131.246704641427)) ;
#147750=CARTESIAN_POINT('Ctrl Pts',(-22.3340590487769,14.1863633435458,
131.470884649421)) ;
#147751=CARTESIAN_POINT('Ctrl Pts',(-22.3793406508304,13.9255968705726,
131.636336360849)) ;
#147752=CARTESIAN_POINT('Ctrl Pts',(-22.4001605026576,13.6292801101744,
131.730263653037)) ;
#147753=CARTESIAN_POINT('Ctrl Pts',(-22.3944314276688,13.3179690043923,
131.746663855123)) ;
#147754=CARTESIAN_POINT('Ctrl Pts',(-22.3618138354626,13.0144329118731,
131.684488661927)) ;
#147755=CARTESIAN_POINT('Ctrl Pts',(-22.3039665732409,12.7401667840787,
131.548606149446)) ;
#147756=CARTESIAN_POINT('Ctrl Pts',(-22.2241247883536,12.5144107338462,
131.34852837519)) ;
#147757=CARTESIAN_POINT('Ctrl Pts',(-22.1274235747229,12.3540784671315,
131.09917757095)) ;
#147758=CARTESIAN_POINT('Ctrl Pts',(-22.0203905808136,12.2704506823876,
130.819545083415)) ;
#147759=CARTESIAN_POINT('Ctrl Pts',(-21.9092164103805,12.2689820893059,
130.527940599895)) ;
#147760=CARTESIAN_POINT('Ctrl Pts',(-21.8014011825293,12.3508509488233,
130.246203129404)) ;
#147761=CARTESIAN_POINT('Ctrl Pts',(-21.7046974530704,12.5086055311564,
129.996715163344)) ;
#147762=CARTESIAN_POINT('Ctrl Pts',(-21.6240710185452,12.7330676993537,
129.7944205009)) ;
#147763=CARTESIAN_POINT('Ctrl Pts',(-21.5655611211422,13.0066123960221,
129.656635909801)) ;
#147764=CARTESIAN_POINT('Ctrl Pts',(-21.5323215652133,13.3082725062707,
129.592500856618)) ;
#147765=CARTESIAN_POINT('Ctrl Pts',(-21.5256970786124,13.6201712444572,
129.606335855298)) ;
#147766=CARTESIAN_POINT('Ctrl Pts',(-21.5459113781207,13.9183340301052,
129.698623260894)) ;
#147767=CARTESIAN_POINT('Ctrl Pts',(-21.5905200274983,14.1797387715242,
129.862041430257)) ;
#147768=CARTESIAN_POINT('Ctrl Pts',(-21.6553241180103,14.3864986993276,
130.084342628369)) ;
#147769=CARTESIAN_POINT('Ctrl Pts',(-21.7354793084019,14.5252641571149,
130.351617653865)) ;
#147770=CARTESIAN_POINT('Ctrl Pts',(-21.8245513470897,14.5851721018435,
130.645016977157)) ;
#147771=CARTESIAN_POINT('Ctrl Pts',(-21.9153010096144,14.5610669254243,
130.943362526667)) ;
#147772=CARTESIAN_POINT('Ctrl Pts',(-21.9994922925595,14.4566509961662,
131.222188061234)) ;
#147773=CARTESIAN_POINT('Ctrl Pts',(-22.0722010613077,14.2771545373181,
131.467832940722)) ;
#147774=CARTESIAN_POINT('Ctrl Pts',(-22.1262384175291,14.0362065449594,
131.658867438289)) ;
#147775=CARTESIAN_POINT('Ctrl Pts',(-22.1572139611432,13.7533987258428,
131.782313040366)) ;
#147776=CARTESIAN_POINT('Ctrl Pts',(-22.1625009400224,13.4441283625548,
131.831033676045)) ;
#147777=CARTESIAN_POINT('Ctrl Pts',(-22.140564230066,13.1346408964387,131.800086171256)) ;
#147778=CARTESIAN_POINT('Ctrl Pts',(-22.0928516991892,12.8470251714903,
131.693686261064)) ;
#147779=CARTESIAN_POINT('Ctrl Pts',(-22.0211494847611,12.5984937845751,
131.517487007206)) ;
#147780=CARTESIAN_POINT('Ctrl Pts',(-21.9309737753859,12.4108688271007,
131.287059945981)) ;
#147781=CARTESIAN_POINT('Ctrl Pts',(-21.8272669687951,12.2946081104034,
131.01721764876)) ;
#147782=CARTESIAN_POINT('Ctrl Pts',(-21.7161953353961,12.2594450538074,
130.726072036675)) ;
#147783=CARTESIAN_POINT('Ctrl Pts',(-21.60658212141,12.308048143484,130.438929539437)) ;
#147784=CARTESIAN_POINT('Ctrl Pts',(-21.5046765692389,12.4360760888544,
130.174304543921)) ;
#147785=CARTESIAN_POINT('Ctrl Pts',(-21.4170241462741,12.6345258024436,
129.951310361765)) ;
#147786=CARTESIAN_POINT('Ctrl Pts',(-21.3489685892398,12.8902136692482,
129.785676166942)) ;
#147787=CARTESIAN_POINT('Ctrl Pts',(-21.3050715222795,13.1836914998379,
129.690556675395)) ;
#147788=CARTESIAN_POINT('Ctrl Pts',(-21.2875431524177,13.4943233710872,
129.672471793995)) ;
#147789=CARTESIAN_POINT('Ctrl Pts',(-21.2970438548803,13.8008444309758,
129.733451477825)) ;
#147790=CARTESIAN_POINT('Ctrl Pts',(-21.3321854329995,14.0793169977329,
129.869248256768)) ;
#147791=CARTESIAN_POINT('Ctrl Pts',(-21.3892022783264,14.3098744793808,
130.06877225239)) ;
#147792=CARTESIAN_POINT('Ctrl Pts',(-21.4644021583777,14.4788324369104,
130.321755899341)) ;
#147793=CARTESIAN_POINT('Ctrl Pts',(-21.5503775766376,14.5706779961945,
130.605939092449)) ;
#147794=CARTESIAN_POINT('Ctrl Pts',(-21.6408546610516,14.5811216657767,
130.903299048732)) ;
#147795=CARTESIAN_POINT('Ctrl Pts',(-21.7290160591459,14.508299186415,131.194043800993)) ;
#147796=CARTESIAN_POINT('Ctrl Pts',(-21.8071127913757,14.3580058494818,
131.455269800372)) ;
#147797=CARTESIAN_POINT('Ctrl Pts',(-21.8692690049898,14.1405257747425,
131.669989141378)) ;
#147798=CARTESIAN_POINT('Ctrl Pts',(-21.9100611483019,13.8719962112454,
131.822245697122)) ;
#147799=CARTESIAN_POINT('Ctrl Pts',(-21.9260462949812,13.571629068225,131.902012596254)) ;
#147800=CARTESIAN_POINT('Ctrl Pts',(-21.9151786975918,13.2591263892434,
131.903497844346)) ;
#147801=CARTESIAN_POINT('Ctrl Pts',(-21.8776490214524,12.9599152020145,
131.826926251731)) ;
#147802=CARTESIAN_POINT('Ctrl Pts',(-21.8152817422074,12.693080122514,131.677887077937)) ;
#147803=CARTESIAN_POINT('Ctrl Pts',(-21.7318932707648,12.478823817929,131.467412166417)) ;
#147804=CARTESIAN_POINT('Ctrl Pts',(-21.6327999015098,12.3322479297148,
131.211038953478)) ;
#147805=CARTESIAN_POINT('Ctrl Pts',(-21.5242177252989,12.2636849635138,
130.926971995263)) ;
#147806=CARTESIAN_POINT('Ctrl Pts',(-21.4132305357613,12.2782423656434,
130.635891058601)) ;
#147807=CARTESIAN_POINT('Ctrl Pts',(-21.3071564989926,12.3748788450642,
130.359150081673)) ;
#147808=CARTESIAN_POINT('Ctrl Pts',(-21.2128894825434,12.5463734718221,
130.116868376143)) ;
#147809=CARTESIAN_POINT('Ctrl Pts',(-21.1362513663819,12.7810696504838,
129.926144136588)) ;
#147810=CARTESIAN_POINT('Ctrl Pts',(-21.0823186107827,13.0608633247241,
129.80163888343)) ;
#147811=CARTESIAN_POINT('Ctrl Pts',(-21.053841117646,13.3671882747387,129.751572869485)) ;
#147812=CARTESIAN_POINT('Ctrl Pts',(-21.052413710193,13.6783220863787,129.78061109945)) ;
#147813=CARTESIAN_POINT('Ctrl Pts',(-21.0773404053595,13.970110064652,129.886522311045)) ;
#147814=CARTESIAN_POINT('Ctrl Pts',(-21.1260864074651,14.223034525395,130.062047312734)) ;
#147815=CARTESIAN_POINT('Ctrl Pts',(-21.1944669924731,14.4186168883369,
130.294931085397)) ;
#147816=CARTESIAN_POINT('Ctrl Pts',(-21.2767695355892,14.5428705869547,
130.568459883078)) ;
#147817=CARTESIAN_POINT('Ctrl Pts',(-21.3665020515511,14.5869069848455,
130.863723007188)) ;
#147818=CARTESIAN_POINT('Ctrl Pts',(-21.4562511004557,14.5480013176435,
131.158949677718)) ;
#147819=CARTESIAN_POINT('Ctrl Pts',(-21.5397825926928,14.4271740770577,
131.436324849005)) ;
#147820=CARTESIAN_POINT('Ctrl Pts',(-21.6086583923119,14.2362638791343,
131.670454356284)) ;
#147821=CARTESIAN_POINT('Ctrl Pts',(-21.6587784835505,13.9863048386446,
131.85000812487)) ;
#147822=CARTESIAN_POINT('Ctrl Pts',(-21.6851472284161,13.6957298215624,
131.960182987964)) ;
#147823=CARTESIAN_POINT('Ctrl Pts',(-21.6853929289674,13.3866515753752,
131.993937295129)) ;
#147824=CARTESIAN_POINT('Ctrl Pts',(-21.6582776406114,13.0771469727204,
131.948105746081)) ;
#147825=CARTESIAN_POINT('Ctrl Pts',(-21.605884471671,12.796392103063,131.827972089653)) ;
#147826=CARTESIAN_POINT('Ctrl Pts',(-21.5302178923545,12.5578779370545,
131.640184361149)) ;
#147827=CARTESIAN_POINT('Ctrl Pts',(-21.4371072181925,12.383073568111,131.401168478668)) ;
#147828=CARTESIAN_POINT('Ctrl Pts',(-21.3314361683633,12.2815115204251,
131.125642156933)) ;
#147829=CARTESIAN_POINT('Ctrl Pts',(-21.220189476718,12.2623682395224,130.833904271501)) ;
#147830=CARTESIAN_POINT('Ctrl Pts',(-21.111889747899,12.3259184217804,130.550477416465)) ;
#147831=CARTESIAN_POINT('Ctrl Pts',(-21.0118711465864,12.4680809238775,
130.291448394108)) ;
#147832=CARTESIAN_POINT('Ctrl Pts',(-20.9272254879945,12.6795623120404,
130.077395414109)) ;
#147833=CARTESIAN_POINT('Ctrl Pts',(-20.8637839574138,12.9425894685416,
129.925062925594)) ;
#147834=CARTESIAN_POINT('Ctrl Pts',(-20.8245561726934,13.2417282929866,
129.843679604379)) ;
#147835=CARTESIAN_POINT('Ctrl Pts',(-20.8121787579524,13.5531902629317,
129.840645625293)) ;
#147836=CARTESIAN_POINT('Ctrl Pts',(-20.826647165812,13.8554128204607,129.916054647535)) ;
#147837=CARTESIAN_POINT('Ctrl Pts',(-20.8660416715249,14.1261608663375,
130.06419630691)) ;
#147838=CARTESIAN_POINT('Ctrl Pts',(-20.9273901269622,14.3478084668955,
130.276692976576)) ;
#147839=CARTESIAN_POINT('Ctrl Pts',(-21.0043490799319,14.5013886643306,
130.534422370052)) ;
#147840=CARTESIAN_POINT('Ctrl Pts',(-21.0922596829206,14.5792263009218,
130.82449298872)) ;
#147841=CARTESIAN_POINT('Ctrl Pts',(-21.1828391154011,14.5735423327803,
131.122170352937)) ;
#147842=CARTESIAN_POINT('Ctrl Pts',(-21.2694503580301,14.4859392223761,
131.408288783411)) ;
#147843=CARTESIAN_POINT('Ctrl Pts',(-21.345349839766,14.32102399054,131.663278927697)) ;
#147844=CARTESIAN_POINT('Ctrl Pts',(-21.4034913421488,14.0938129483377,
131.866070729537)) ;
#147845=CARTESIAN_POINT('Ctrl Pts',(-21.4400110100887,13.8165579803482,
132.005993362765)) ;
#147846=CARTESIAN_POINT('Ctrl Pts',(-21.4509809590389,13.5127264652926,
132.071072537445)) ;
#147847=CARTESIAN_POINT('Ctrl Pts',(-21.4348676182243,13.2000971837,132.057309732157)) ;
#147848=CARTESIAN_POINT('Ctrl Pts',(-21.3927484801215,12.9073427141145,
131.967122130863)) ;
#147849=CARTESIAN_POINT('Ctrl Pts',(-21.3258505842354,12.6479572594797,
131.804981308529)) ;
#147850=CARTESIAN_POINT('Ctrl Pts',(-21.2394142383129,12.4461100388149,
131.585465190968)) ;
#147851=CARTESIAN_POINT('Ctrl Pts',(-21.1374149775603,12.3127706272653,
131.320810832237)) ;
#147852=CARTESIAN_POINT('Ctrl Pts',(-21.0282673309725,12.2601401090579,
131.034952467614)) ;
#147853=CARTESIAN_POINT('Ctrl Pts',(-20.9177126950044,12.2901733213181,
130.745118295567)) ;
#147854=CARTESIAN_POINT('Ctrl Pts',(-20.8132418808532,12.4015833019759,
130.473080662222)) ;
#147855=CARTESIAN_POINT('Ctrl Pts',(-20.7216877105118,12.586648376757,130.238816544621)) ;
#147856=CARTESIAN_POINT('Ctrl Pts',(-20.6492277224844,12.8302723293176,
130.060151545908)) ;
#147857=CARTESIAN_POINT('Ctrl Pts',(-20.5995649352274,13.1192440292328,
129.948424989432)) ;
#147858=CARTESIAN_POINT('Ctrl Pts',(-20.5764497565438,13.4254781947616,
129.913736732255)) ;
#147859=CARTESIAN_POINT('Ctrl Pts',(-20.5800162996611,13.73535968212,129.957422057051)) ;
#147860=CARTESIAN_POINT('Ctrl Pts',(-20.6096448160032,14.0210481979202,
130.077031775124)) ;
#147861=CARTESIAN_POINT('Ctrl Pts',(-20.6625737600944,14.2649914654817,
130.264853339721)) ;
#147862=CARTESIAN_POINT('Ctrl Pts',(-20.7339227482206,14.4476746957159,
130.506339169657)) ;
#147863=CARTESIAN_POINT('Ctrl Pts',(-20.8181740365747,14.5574099985375,
130.785581972635)) ;
#147864=CARTESIAN_POINT('Ctrl Pts',(-20.9083832242606,14.5860647518339,
131.082188756989)) ;
#147865=CARTESIAN_POINT('Ctrl Pts',(-20.9980143564362,14.5307819376324,
131.377329816283)) ;
#147866=CARTESIAN_POINT('Ctrl Pts',(-21.0785436243018,14.3969445347875,
131.645559337238)) ;
#147867=CARTESIAN_POINT('Ctrl Pts',(-21.144755916161,14.1927449402103,131.872158750535)) ;
#147868=CARTESIAN_POINT('Ctrl Pts',(-21.1905238305556,13.9340124552338,
132.038928596485)) ;
#147869=CARTESIAN_POINT('Ctrl Pts',(-21.2121498400583,13.638112171606,132.135255984941)) ;
#147870=CARTESIAN_POINT('Ctrl Pts',(-21.2071970261272,13.3270743083993,
132.153904990694)) ;
#147871=CARTESIAN_POINT('Ctrl Pts',(-21.1753089200448,13.0225106928389,
132.093912711997)) ;
#147872=CARTESIAN_POINT('Ctrl Pts',(-21.1179639971965,12.7468020423806,
131.959553634409)) ;
#147873=CARTESIAN_POINT('Ctrl Pts',(-21.0390833671459,12.520588791344,131.76211445131)) ;
#147874=CARTESIAN_POINT('Ctrl Pts',(-20.9427982312011,12.3578209708367,
131.51399660927)) ;
#147875=CARTESIAN_POINT('Ctrl Pts',(-20.8356847345824,12.2716454872787,
131.234216653382)) ;
#147876=CARTESIAN_POINT('Ctrl Pts',(-20.7246335895613,12.26795429664,130.942939134598)) ;
#147877=CARTESIAN_POINT('Ctrl Pts',(-20.616973302296,12.3469221787347,130.661535656363)) ;
#147878=CARTESIAN_POINT('Ctrl Pts',(-20.5194780056374,12.5030898153774,
130.409865228873)) ;
#147879=CARTESIAN_POINT('Ctrl Pts',(-20.4385947118709,12.725018199882,130.20669437947)) ;
#147880=CARTESIAN_POINT('Ctrl Pts',(-20.3792474158337,12.997182809166,130.066468431869)) ;
#147881=CARTESIAN_POINT('Ctrl Pts',(-20.3450790019387,13.2997828332168,
129.999782492752)) ;
#147882=CARTESIAN_POINT('Ctrl Pts',(-20.3377619039051,13.6108910238796,
130.011503902114)) ;
#147883=CARTESIAN_POINT('Ctrl Pts',(-20.3570249789921,13.9087323450299,
130.100885429075)) ;
#147884=CARTESIAN_POINT('Ctrl Pts',(-20.4010227954552,14.1725576107312,
130.2626334915)) ;
#147885=CARTESIAN_POINT('Ctrl Pts',(-20.4654669482324,14.3815587835512,
130.483957592039)) ;
#147886=CARTESIAN_POINT('Ctrl Pts',(-20.5452725967779,14.522329585323,130.750205362324)) ;
#147887=CARTESIAN_POINT('Ctrl Pts',(-20.6339261819108,14.5844939655697,
131.042286429086)) ;
#147888=CARTESIAN_POINT('Ctrl Pts',(-20.7247186453383,14.5631534313931,
131.340749638072)) ;
#147889=CARTESIAN_POINT('Ctrl Pts',(-20.809527155941,14.4606751117259,131.62150908493)) ;
#147890=CARTESIAN_POINT('Ctrl Pts',(-20.8826704768018,14.2826954166288,
131.868454149074)) ;
#147891=CARTESIAN_POINT('Ctrl Pts',(-20.9370591986332,14.0447463561046,
132.060328466672)) ;
#147892=CARTESIAN_POINT('Ctrl Pts',(-20.9689299497297,13.7613771216005,
132.186577022654)) ;
#147893=CARTESIAN_POINT('Ctrl Pts',(-20.9749288618211,13.4542323350155,
132.237185457133)) ;
#147894=CARTESIAN_POINT('Ctrl Pts',(-20.9538950902724,13.1437994657192,
132.208942651979)) ;
#147895=CARTESIAN_POINT('Ctrl Pts',(-20.9065605624444,12.8538469194028,
132.103822776619)) ;
#147896=CARTESIAN_POINT('Ctrl Pts',(-20.8358615876408,12.6054873478473,
131.930355849117)) ;
#147897=CARTESIAN_POINT('Ctrl Pts',(-20.7461738157483,12.4153273189239,
131.701384848955)) ;
#147898=CARTESIAN_POINT('Ctrl Pts',(-20.6418761403516,12.2964112456076,
131.430080533355)) ;
#147899=CARTESIAN_POINT('Ctrl Pts',(-20.5321091748032,12.2594155903617,
131.142376798945)) ;
#147900=CARTESIAN_POINT('Ctrl Pts',(-20.4219406220952,12.3053349430094,
130.853742645064)) ;
#147901=CARTESIAN_POINT('Ctrl Pts',(-20.3197409294041,12.431225904051,130.58824874815)) ;
#147902=CARTESIAN_POINT('Ctrl Pts',(-20.2314802430667,12.6279597128561,
130.363514862716)) ;
#147903=CARTESIAN_POINT('Ctrl Pts',(-20.162777545172,12.8824932881055,130.19601021006)) ;
#147904=CARTESIAN_POINT('Ctrl Pts',(-20.1182353083601,13.1745455481659,
130.098938299482)) ;
#147905=CARTESIAN_POINT('Ctrl Pts',(-20.0998706065,13.4851755770177,130.078429714229)) ;
#147906=CARTESIAN_POINT('Ctrl Pts',(-20.1086336178108,13.7921379427258,
130.137258008057)) ;
#147907=CARTESIAN_POINT('Ctrl Pts',(-20.14286672269,14.0710147871215,130.270296111646)) ;
#147908=CARTESIAN_POINT('Ctrl Pts',(-20.1996972773832,14.3045452092941,
130.469492695911)) ;
#147909=CARTESIAN_POINT('Ctrl Pts',(-20.273759835946,14.4740866003594,130.71884073993)) ;
#147910=CARTESIAN_POINT('Ctrl Pts',(-20.3600214704323,14.5693022408221,
131.004086313141)) ;
#147911=CARTESIAN_POINT('Ctrl Pts',(-20.4504553064572,14.5820126324711,
131.301304006894)) ;
#147912=CARTESIAN_POINT('Ctrl Pts',(-20.5390122957554,14.5112271142504,
131.593295289522)) ;
#147913=CARTESIAN_POINT('Ctrl Pts',(-20.617145557028,14.3635591504594,131.854489519357)) ;
#147914=CARTESIAN_POINT('Ctrl Pts',(-20.6798949965578,14.147953964214,132.070948087986)) ;
#147915=CARTESIAN_POINT('Ctrl Pts',(-20.7214213257657,13.88065471692,132.225356091417)) ;
#147916=CARTESIAN_POINT('Ctrl Pts',(-20.7382001300279,13.5796273902736,
132.307581392569)) ;
#147917=CARTESIAN_POINT('Ctrl Pts',(-20.72801762459,13.2675902134212,132.311017500675)) ;
#147918=CARTESIAN_POINT('Ctrl Pts',(-20.6913625442672,12.9685392965924,
132.236910820847)) ;
#147919=CARTESIAN_POINT('Ctrl Pts',(-20.6296262601908,12.7001827589766,
132.08974747975)) ;
#147920=CARTESIAN_POINT('Ctrl Pts',(-20.5468892830631,12.4843513873254,
131.881136546848)) ;
#147921=CARTESIAN_POINT('Ctrl Pts',(-20.4480106979793,12.3354377885734,
131.625445849201)) ;
#147922=CARTESIAN_POINT('Ctrl Pts',(-20.3399262007123,12.2645466561417,
131.342734057341)) ;
#147923=CARTESIAN_POINT('Ctrl Pts',(-20.2283990487693,12.2767400465521,
131.050231091505)) ;
#147924=CARTESIAN_POINT('Ctrl Pts',(-20.122468047658,12.3708038942679,130.773785646118)) ;
#147925=CARTESIAN_POINT('Ctrl Pts',(-20.0275757835949,12.540571419273,130.529748962707)) ;
#147926=CARTESIAN_POINT('Ctrl Pts',(-19.9505760506739,12.7727636471261,
130.337850842071)) ;
#147927=CARTESIAN_POINT('Ctrl Pts',(-19.895548548468,13.0532482388654,130.210361702874)) ;
#147928=CARTESIAN_POINT('Ctrl Pts',(-19.8664861035887,13.3594503778047,
130.158608683618)) ;
#147929=CARTESIAN_POINT('Ctrl Pts',(-19.8642805955961,13.6687250636368,
130.185154959799)) ;
#147930=CARTESIAN_POINT('Ctrl Pts',(-19.8884803528754,13.9622484171183,
130.289040068247)) ;
#147931=CARTESIAN_POINT('Ctrl Pts',(-19.9365724196129,14.2163837288721,
130.462630299501)) ;
#147932=CARTESIAN_POINT('Ctrl Pts',(-20.004641785684,14.4143549429609,130.694692087338)) ;
#147933=CARTESIAN_POINT('Ctrl Pts',(-20.0866599380791,14.5404303833534,
130.967385240993)) ;
#147934=CARTESIAN_POINT('Ctrl Pts',(-20.1758963178231,14.5868747915152,
131.261056127709)) ;
#147935=CARTESIAN_POINT('Ctrl Pts',(-20.2662529036822,14.5499212466532,
131.558258305741)) ;
#147936=CARTESIAN_POINT('Ctrl Pts',(-20.3493796320755,14.4324626296397,
131.834156427293)) ;
#147937=CARTESIAN_POINT('Ctrl Pts',(-20.4193859524165,14.2419356946445,
132.071886760109)) ;
#147938=CARTESIAN_POINT('Ctrl Pts',(-20.4698543024917,13.9939564786199,
132.252344857302)) ;
#147939=CARTESIAN_POINT('Ctrl Pts',(-20.4969872695557,13.7043181806052,
132.364754467268)) ;
#147940=CARTESIAN_POINT('Ctrl Pts',(-20.497934277569,13.3953697990708,132.400569582699)) ;
#147941=CARTESIAN_POINT('Ctrl Pts',(-20.4717871200725,13.0868083993376,
132.35741635374)) ;
#147942=CARTESIAN_POINT('Ctrl Pts',(-20.4198713515675,12.8035341762303,
132.238849819273)) ;
#147943=CARTESIAN_POINT('Ctrl Pts',(-20.3448769953812,12.5639567579486,
132.052971164344)) ;
#147944=CARTESIAN_POINT('Ctrl Pts',(-20.2520317235411,12.3867441444795,
131.814796568743)) ;
#147945=CARTESIAN_POINT('Ctrl Pts',(-20.1464031923312,12.2832559742793,
131.539448061917)) ;
#147946=CARTESIAN_POINT('Ctrl Pts',(-20.0361703920393,12.2616345635869,
131.250381746518)) ;
#147947=CARTESIAN_POINT('Ctrl Pts',(-19.926830089703,12.3231638748032,130.964186355798)) ;
#147948=CARTESIAN_POINT('Ctrl Pts',(-19.8269315810433,12.4627499804897,
130.705354563112)) ;
#147949=CARTESIAN_POINT('Ctrl Pts',(-19.7415073817147,12.6729053346686,
130.489121388215)) ;
#147950=CARTESIAN_POINT('Ctrl Pts',(-19.6774820062394,12.9344260025205,
130.335045332416)) ;
#147951=CARTESIAN_POINT('Ctrl Pts',(-19.6374230862404,13.2340774716611,
130.25136547355)) ;
#147952=CARTESIAN_POINT('Ctrl Pts',(-19.6244120372296,13.5439038566318,
130.246310943966)) ;
#147953=CARTESIAN_POINT('Ctrl Pts',(-19.6380214405693,13.8465581380597,
130.319189287178)) ;
#147954=CARTESIAN_POINT('Ctrl Pts',(-19.6767732091256,14.1188039564303,
130.465491640985)) ;
#147955=CARTESIAN_POINT('Ctrl Pts',(-19.7374565997598,14.3420290763671,
130.67600475398)) ;
#147956=CARTESIAN_POINT('Ctrl Pts',(-19.8142575244507,14.4980360356998,
130.933370357815)) ;
#147957=CARTESIAN_POINT('Ctrl Pts',(-19.9015404461652,14.5780642406309,
131.221444969718)) ;
#147958=CARTESIAN_POINT('Ctrl Pts',(-19.9928382265916,14.574764467068,131.521483463765)) ;
#147959=CARTESIAN_POINT('Ctrl Pts',(-20.0791689532746,14.4895501192037,
131.806603095994)) ;
#147960=CARTESIAN_POINT('Ctrl Pts',(-20.1553727313655,14.3274511862454,
132.062408003817)) ;
#147961=CARTESIAN_POINT('Ctrl Pts',(-20.2143165511384,14.1012131862614,
132.267654668105)) ;
#147962=CARTESIAN_POINT('Ctrl Pts',(-20.251535640847,13.8249844629114,132.409627218368)) ;
#147963=CARTESIAN_POINT('Ctrl Pts',(-20.2632155313294,13.5214321679055,
132.476806560396)) ;
#147964=CARTESIAN_POINT('Ctrl Pts',(-20.2480538564404,13.2103012172843,
132.465645791352)) ;
#147965=CARTESIAN_POINT('Ctrl Pts',(-20.2064762839106,12.914853162699,132.377251371231)) ;
#147966=CARTESIAN_POINT('Ctrl Pts',(-20.140151413628,12.6543477666719,132.216774551405)) ;
#147967=CARTESIAN_POINT('Ctrl Pts',(-20.0543603731437,12.4511188727926,
131.999088220512)) ;
#147968=CARTESIAN_POINT('Ctrl Pts',(-19.9529344290796,12.3156705463735,
131.736039696364)) ;
#147969=CARTESIAN_POINT('Ctrl Pts',(-19.8434300726974,12.2603783295909,
131.449288215452)) ;
#147970=CARTESIAN_POINT('Ctrl Pts',(-19.7328703196566,12.2883877263298,
131.159422548297)) ;
#147971=CARTESIAN_POINT('Ctrl Pts',(-19.6285496546779,12.396958257867,130.887685326654)) ;
#147972=CARTESIAN_POINT('Ctrl Pts',(-19.5361836894076,12.5805839699868,
130.651163338837)) ;
#147973=CARTESIAN_POINT('Ctrl Pts',(-19.4633189319576,12.8225431227576,
130.471268902944)) ;
#147974=CARTESIAN_POINT('Ctrl Pts',(-19.4130339180868,13.1085293602937,
130.357514271986)) ;
#147975=CARTESIAN_POINT('Ctrl Pts',(-19.3888828182431,13.4184312850536,
130.320233884699)) ;
#147976=CARTESIAN_POINT('Ctrl Pts',(-19.391721830465,13.725396858395,130.361439759483)) ;
#147977=CARTESIAN_POINT('Ctrl Pts',(-19.4207326434381,14.0140710244904,
130.479477244557)) ;
#147978=CARTESIAN_POINT('Ctrl Pts',(-19.472993335133,14.2586953063536,130.665252246815)) ;
#147979=CARTESIAN_POINT('Ctrl Pts',(-19.5439543323498,14.4435712353924,
130.905649593416)) ;
#147980=CARTESIAN_POINT('Ctrl Pts',(-19.6279191274748,14.5554638044199,
131.184041916383)) ;
#147981=CARTESIAN_POINT('Ctrl Pts',(-19.718147960445,14.5862678502014,131.480744103854)) ;
#147982=CARTESIAN_POINT('Ctrl Pts',(-19.807315566859,14.5339455357937,131.774300672977)) ;
#147983=CARTESIAN_POINT('Ctrl Pts',(-19.8886286972119,14.4019055778879,
132.044990740636)) ;
#147984=CARTESIAN_POINT('Ctrl Pts',(-19.9552665859861,14.1996929646046,
132.272793191288)) ;
#147985=CARTESIAN_POINT('Ctrl Pts',(-20.0017789452845,13.9418840250199,
132.441799109411)) ;
#147986=CARTESIAN_POINT('Ctrl Pts',(-20.0241090640634,13.6467946138759,
132.540172309611)) ;
#147987=CARTESIAN_POINT('Ctrl Pts',(-20.0199186627607,13.3358858072713,
132.561050637465)) ;
#147988=CARTESIAN_POINT('Ctrl Pts',(-19.9888290528914,13.0311284107843,
132.503354655419)) ;
#147989=CARTESIAN_POINT('Ctrl Pts',(-19.9321905550994,12.7543595776973,
132.371055946195)) ;
#147990=CARTESIAN_POINT('Ctrl Pts',(-19.8539774312581,12.5263864421984,
132.175548707132)) ;
#147991=CARTESIAN_POINT('Ctrl Pts',(-19.7573065319154,12.360701809008,131.926557988683)) ;
#147992=CARTESIAN_POINT('Ctrl Pts',(-19.6513712846264,12.2732420187478,
131.649911504307)) ;
#147993=CARTESIAN_POINT('Ctrl Pts',(-19.5399002468881,12.2668291176247,
131.357543001955)) ;
#147994=CARTESIAN_POINT('Ctrl Pts',(-19.4321205019427,12.3436152080196,
131.075766932317)) ;
#147995=CARTESIAN_POINT('Ctrl Pts',(-19.3341292920677,12.4979167345461,
130.82268907935)) ;
#147996=CARTESIAN_POINT('Ctrl Pts',(-19.2527820213521,12.7181780575431,
130.618144770234)) ;
#147997=CARTESIAN_POINT('Ctrl Pts',(-19.1928530764132,12.9887184060059,
130.47616616468)) ;
#147998=CARTESIAN_POINT('Ctrl Pts',(-19.1578999356697,13.2908826927602,
130.40720568529)) ;
#147999=CARTESIAN_POINT('Ctrl Pts',(-19.1497953394028,13.6021683784905,
130.416637581749)) ;
#148000=CARTESIAN_POINT('Ctrl Pts',(-19.1684189323087,13.9015373279121,
130.50424803556)) ;
#148001=CARTESIAN_POINT('Ctrl Pts',(-19.2118191501217,14.1661757603649,
130.664218341433)) ;
#148002=CARTESIAN_POINT('Ctrl Pts',(-19.275532904537,14.3763136740977,130.883305791061)) ;
#148003=CARTESIAN_POINT('Ctrl Pts',(-19.3551769889654,14.519537909018,131.149161406706)) ;
#148004=CARTESIAN_POINT('Ctrl Pts',(-19.4434530746954,14.5837467731856,
131.44005439952)) ;
#148005=CARTESIAN_POINT('Ctrl Pts',(-19.5342180638581,14.5651055600629,
131.738406775999)) ;
#148006=CARTESIAN_POINT('Ctrl Pts',(-19.6195559792533,14.4645028782859,
132.020822945501)) ;
#148007=CARTESIAN_POINT('Ctrl Pts',(-19.6928888773536,14.2890439916082,
132.26821178798)) ;
#148008=CARTESIAN_POINT('Ctrl Pts',(-19.7479581143454,14.0526944829589,
132.46209038044)) ;
#148009=CARTESIAN_POINT('Ctrl Pts',(-19.7805744132292,13.7699865905546,
132.59055835538)) ;
#148010=CARTESIAN_POINT('Ctrl Pts',(-19.7873817604731,13.4631529317897,
132.643534440188)) ;
#148011=CARTESIAN_POINT('Ctrl Pts',(-19.7669187252397,13.1513621002968,
132.617087995616)) ;
#148012=CARTESIAN_POINT('Ctrl Pts',(-19.7207142391698,12.8627668300252,
132.515003273399)) ;
#148013=CARTESIAN_POINT('Ctrl Pts',(-19.65008748828,12.6109028722605,132.342021948642)) ;
#148014=CARTESIAN_POINT('Ctrl Pts',(-19.561222299513,12.4200193070119,132.115293679117)) ;
#148015=CARTESIAN_POINT('Ctrl Pts',(-19.4571858182592,12.2986947240349,
131.844776918444)) ;
#148016=CARTESIAN_POINT('Ctrl Pts',(-19.3476615783916,12.2592723923921,
131.557732973173)) ;
#148017=CARTESIAN_POINT('Ctrl Pts',(-19.2370467547134,12.3030853474788,
131.267903530246)) ;
#148018=CARTESIAN_POINT('Ctrl Pts',(-19.1350692021642,12.4259705775221,
131.002874361858)) ;
#148019=CARTESIAN_POINT('Ctrl Pts',(-19.0457242601456,12.6220549960923,
130.77519438912)) ;
#148020=CARTESIAN_POINT('Ctrl Pts',(-18.9766829417426,12.8744669266435,
130.606582718191)) ;
#148021=CARTESIAN_POINT('Ctrl Pts',(-18.9312995061322,13.1663405887179,
130.507131391168)) ;
#148022=CARTESIAN_POINT('Ctrl Pts',(-18.9122926402712,13.4758788590996,
130.484651920458)) ;
#148023=CARTESIAN_POINT('Ctrl Pts',(-18.9200960317738,13.7823952671727,
130.540566873431)) ;
#148024=CARTESIAN_POINT('Ctrl Pts',(-18.9539251467135,14.0644181714752,
130.672684462497)) ;
#148025=CARTESIAN_POINT('Ctrl Pts',(-19.0097351190021,14.2977471019388,
130.868637136998)) ;
#148026=CARTESIAN_POINT('Ctrl Pts',(-19.0838281882075,14.4706193874242,
131.11830442749)) ;
#148027=CARTESIAN_POINT('Ctrl Pts',(-19.1695978281786,14.5675955014972,
131.401997914482)) ;
#148028=CARTESIAN_POINT('Ctrl Pts',(-19.2600457357947,14.5827756049051,
131.699282364173)) ;
#148029=CARTESIAN_POINT('Ctrl Pts',(-19.3484197526924,14.5148008720864,
131.990598673523)) ;
#148030=CARTESIAN_POINT('Ctrl Pts',(-19.4272267092737,14.3692243405837,
132.253858791749)) ;
#148031=CARTESIAN_POINT('Ctrl Pts',(-19.4907681026563,14.1540994987709,
132.472794222791)) ;
#148032=CARTESIAN_POINT('Ctrl Pts',(-19.5326959218197,13.8891946725912,
132.628217325786)) ;
#148033=CARTESIAN_POINT('Ctrl Pts',(-19.5502934574863,13.5894849367596,
132.712773163463)) ;
#148034=CARTESIAN_POINT('Ctrl Pts',(-19.5409583981256,13.2771022770821,
132.718722496154)) ;
#148035=CARTESIAN_POINT('Ctrl Pts',(-19.5050204736514,12.9767129861419,
132.646781306479)) ;
#148036=CARTESIAN_POINT('Ctrl Pts',(-19.4436491984434,12.7063602426885,
132.500801909177)) ;
#148037=CARTESIAN_POINT('Ctrl Pts',(-19.3619009141506,12.490160978819,132.294887344641)) ;
#148038=CARTESIAN_POINT('Ctrl Pts',(-19.2633520708704,12.3386882499648,
132.040193767955)) ;
#148039=CARTESIAN_POINT('Ctrl Pts',(-19.1552318803299,12.2654833312748,
131.757441066399)) ;
#148040=CARTESIAN_POINT('Ctrl Pts',(-19.0440477635001,12.2750423779192,
131.465825867201)) ;
#148041=CARTESIAN_POINT('Ctrl Pts',(-18.937341928339,12.3673309106593,131.187290701774)) ;
#148042=CARTESIAN_POINT('Ctrl Pts',(-18.8425063446484,12.534346926541,130.943255559375)) ;
#148043=CARTESIAN_POINT('Ctrl Pts',(-18.7647046564001,12.7652871002756,
130.749089683899)) ;
#148044=CARTESIAN_POINT('Ctrl Pts',(-18.709069337308,13.0444119027006,130.619786300958)) ;
#148045=CARTESIAN_POINT('Ctrl Pts',(-18.6791499289154,13.3498617149792,
130.565502996383)) ;
#148046=CARTESIAN_POINT('Ctrl Pts',(-18.6762315013032,13.6613614956128,
130.590188842679)) ;
#148047=CARTESIAN_POINT('Ctrl Pts',(-18.6996281709069,13.9537822109427,
130.691518849554)) ;
#148048=CARTESIAN_POINT('Ctrl Pts',(-18.7470501732347,14.2096141501914,
130.863178899728)) ;
#148049=CARTESIAN_POINT('Ctrl Pts',(-18.8144755931522,14.409057323901,131.093292203471)) ;
#148050=CARTESIAN_POINT('Ctrl Pts',(-18.8961116319339,14.5378227740497,
131.364866046126)) ;
#148051=CARTESIAN_POINT('Ctrl Pts',(-18.9859286827012,14.5866410235712,
131.660492358741)) ;
#148052=CARTESIAN_POINT('Ctrl Pts',(-19.0755119588269,14.5524956980778,
131.955107811092)) ;
#148053=CARTESIAN_POINT('Ctrl Pts',(-19.1596946576678,14.436335978299,132.234399155507)) ;
#148054=CARTESIAN_POINT('Ctrl Pts',(-19.229651373559,14.2487612510743,132.471753659897)) ;
#148055=CARTESIAN_POINT('Ctrl Pts',(-19.2809040891234,14.0019963644833,
132.654569767843)) ;
#148056=CARTESIAN_POINT('Ctrl Pts',(-19.3087933698156,13.7133413739479,
132.769174524247)) ;
#148057=CARTESIAN_POINT('Ctrl Pts',(-19.3104356669662,13.4034231112183,
132.807158036576)) ;
#148058=CARTESIAN_POINT('Ctrl Pts',(-19.2852774557655,13.0966156086416,
132.766656369269)) ;
#148059=CARTESIAN_POINT('Ctrl Pts',(-19.2337768140943,12.8104956344232,
132.649520670295)) ;
#148060=CARTESIAN_POINT('Ctrl Pts',(-19.1597423430483,12.5707042508866,
132.466267011948)) ;
#148061=CARTESIAN_POINT('Ctrl Pts',(-19.0672401692143,12.3910193805736,
132.229155022395)) ;
#148062=CARTESIAN_POINT('Ctrl Pts',(-18.9621213671864,12.2853288734926,
131.955219283)) ;
#148063=CARTESIAN_POINT('Ctrl Pts',(-18.8515810799726,12.2609818511097,
131.665367165245)) ;
#148064=CARTESIAN_POINT('Ctrl Pts',(-18.7418048609671,12.3204757411683,
131.377983757519)) ;
#148065=CARTESIAN_POINT('Ctrl Pts',(-18.6416017664951,12.4582515561699,
131.118268532816)) ;
#148066=CARTESIAN_POINT('Ctrl Pts',(-18.5559385730554,12.665899809485,130.901222578766)) ;
#148067=CARTESIAN_POINT('Ctrl Pts',(-18.491157798158,12.926809546633,130.745020644298)) ;
#148068=CARTESIAN_POINT('Ctrl Pts',(-18.4506024983066,13.2233761024273,
130.659630793965)) ;
#148069=CARTESIAN_POINT('Ctrl Pts',(-18.4365710763997,13.5346576099115,
130.651764155775)) ;
#148070=CARTESIAN_POINT('Ctrl Pts',(-18.4495188703671,13.8387960624651,
130.722809136042)) ;
#148071=CARTESIAN_POINT('Ctrl Pts',(-18.4877033441777,14.1123017262305,
130.867484577879)) ;
#148072=CARTESIAN_POINT('Ctrl Pts',(-18.5477031662279,14.3364686788982,
131.075912339679)) ;
#148073=CARTESIAN_POINT('Ctrl Pts',(-18.6241085701617,14.4947707919197,
131.332129718544)) ;
#148074=CARTESIAN_POINT('Ctrl Pts',(-18.711584236043,14.5769227854228,131.620907833145)) ;
#148075=CARTESIAN_POINT('Ctrl Pts',(-18.8018385885695,14.5762675559882,
131.917508974305)) ;
#148076=CARTESIAN_POINT('Ctrl Pts',(-18.8891582964534,14.4930554599536,
132.205808783895)) ;
#148077=CARTESIAN_POINT('Ctrl Pts',(-18.965564283553,14.3331651015145,132.462123050403)) ;
#148078=CARTESIAN_POINT('Ctrl Pts',(-19.0251852228589,14.1081176905962,
132.669421720131)) ;
#148079=CARTESIAN_POINT('Ctrl Pts',(-19.0629634647551,13.8340179533061,
132.812904369814)) ;
#148080=CARTESIAN_POINT('Ctrl Pts',(-19.0754768051102,13.5302899691965,
132.882602632264)) ;
#148081=CARTESIAN_POINT('Ctrl Pts',(-19.0610963876099,13.2194242274908,
132.873681234086)) ;
#148082=CARTESIAN_POINT('Ctrl Pts',(-19.0202875685388,12.9232188670747,
132.787534564873)) ;
#148083=CARTESIAN_POINT('Ctrl Pts',(-18.9546995972872,12.661461296016,132.629186766265)) ;
#148084=CARTESIAN_POINT('Ctrl Pts',(-18.8692523203122,12.4560560459253,
132.41257049924)) ;
#148085=CARTESIAN_POINT('Ctrl Pts',(-18.7685005068051,12.3187614615208,
132.151384008345)) ;
#148086=CARTESIAN_POINT('Ctrl Pts',(-18.6589859619205,12.2608758926762,
131.86465778122)) ;
#148087=CARTESIAN_POINT('Ctrl Pts',(-18.5485288587057,12.2860567497161,
131.575029100165)) ;
#148088=CARTESIAN_POINT('Ctrl Pts',(-18.4430349502106,12.3936760762178,
131.300170284857)) ;
#148089=CARTESIAN_POINT('Ctrl Pts',(-18.3512334081958,12.5734427117125,
131.064929754193)) ;
#148090=CARTESIAN_POINT('Ctrl Pts',(-18.2770995326014,12.8155556757963,
130.881592457997)) ;
#148091=CARTESIAN_POINT('Ctrl Pts',(-18.2263704446761,13.1001458923633,
130.766461617706)) ;
#148092=CARTESIAN_POINT('Ctrl Pts',(-18.2014503359618,13.4082451874709,
130.726787184823)) ;
#148093=CARTESIAN_POINT('Ctrl Pts',(-18.2034537422446,13.7170001828003,
130.765706683009)) ;
#148094=CARTESIAN_POINT('Ctrl Pts',(-18.2318757307596,14.0068803431456,
130.882068224642)) ;
#148095=CARTESIAN_POINT('Ctrl Pts',(-18.2833608464469,14.2520830304775,
131.065464422881)) ;
#148096=CARTESIAN_POINT('Ctrl Pts',(-18.3537222124873,14.4388654821964,
131.304070485803)) ;
#148097=CARTESIAN_POINT('Ctrl Pts',(-18.437485257584,14.5532758713035,131.581913311696)) ;
#148098=CARTESIAN_POINT('Ctrl Pts',(-18.5277052725611,14.5866372917137,
131.878613366819)) ;
#148099=CARTESIAN_POINT('Ctrl Pts',(-18.6172454058676,14.5363254229255,
132.173356333672)) ;
#148100=CARTESIAN_POINT('Ctrl Pts',(-18.698521140024,14.4070821758454,132.443784329166)) ;
#148101=CARTESIAN_POINT('Ctrl Pts',(-18.7659972083928,14.2058492351143,
132.674191701494)) ;
#148102=CARTESIAN_POINT('Ctrl Pts',(-18.8130187735829,13.9493210351354,
132.844663971232)) ;
#148103=CARTESIAN_POINT('Ctrl Pts',(-18.8360159858587,13.6560816946818,
132.944868856986)) ;
#148104=CARTESIAN_POINT('Ctrl Pts',(-18.8326481694973,13.345421430163,132.968143639762)) ;
#148105=CARTESIAN_POINT('Ctrl Pts',(-18.802476587049,13.040595844376,132.913073904114)) ;
#148106=CARTESIAN_POINT('Ctrl Pts',(-18.746226215621,12.7610203807177,132.782105503749)) ;
#148107=CARTESIAN_POINT('Ctrl Pts',(-18.66857834825,12.5320805251594,132.588205034405)) ;
#148108=CARTESIAN_POINT('Ctrl Pts',(-18.5730541599684,12.3651153632671,
132.342336669536)) ;
#148109=CARTESIAN_POINT('Ctrl Pts',(-18.4664665056406,12.2743250028136,
132.064064252278)) ;
#148110=CARTESIAN_POINT('Ctrl Pts',(-18.3549459131847,12.2660445158075,
131.771566814198)) ;
#148111=CARTESIAN_POINT('Ctrl Pts',(-18.2473957776497,12.3402671255805,
131.490336956928)) ;
#148112=CARTESIAN_POINT('Ctrl Pts',(-18.1489873864352,12.4924311460887,
131.236048239576)) ;
#148113=CARTESIAN_POINT('Ctrl Pts',(-18.0671825361654,12.7106680938423,
131.030125691093)) ;
#148114=CARTESIAN_POINT('Ctrl Pts',(-18.0064123336501,12.9803449580317,
130.885741330905)) ;
#148115=CARTESIAN_POINT('Ctrl Pts',(-17.9706694762708,13.2833170370261,
130.814620547797)) ;
#148116=CARTESIAN_POINT('Ctrl Pts',(-17.9618765736868,13.5926827772034,
130.82183011408)) ;
#148117=CARTESIAN_POINT('Ctrl Pts',(-17.9797619942938,13.8936497726217,
130.907388131803)) ;
#148118=CARTESIAN_POINT('Ctrl Pts',(-18.0224154975657,14.1589430320387,
131.065096694531)) ;
#148119=CARTESIAN_POINT('Ctrl Pts',(-18.0856974126482,14.3711507440271,
131.282979614378)) ;
#148120=CARTESIAN_POINT('Ctrl Pts',(-18.1646930507973,14.5162610526243,
131.546828965686)) ;
#148121=CARTESIAN_POINT('Ctrl Pts',(-18.2535370462115,14.5833063446483,
131.839656321843)) ;
#148122=CARTESIAN_POINT('Ctrl Pts',(-18.3441028407741,14.566512972423,132.137337037032)) ;
#148123=CARTESIAN_POINT('Ctrl Pts',(-18.4293737033493,14.4685224251672,
132.419443796344)) ;
#148124=CARTESIAN_POINT('Ctrl Pts',(-18.503107615546,14.295496638092,132.667961157457)) ;
#148125=CARTESIAN_POINT('Ctrl Pts',(-18.5589734583344,14.0596946684097,
132.864306733473)) ;
#148126=CARTESIAN_POINT('Ctrl Pts',(-18.5922504211388,13.7784556311811,
132.994643197558)) ;
#148127=CARTESIAN_POINT('Ctrl Pts',(-18.5996736634581,13.4704205664196,
133.049595144208)) ;
#148128=CARTESIAN_POINT('Ctrl Pts',(-18.5803706966428,13.1626907003778,
133.026063848939)) ;
#148129=CARTESIAN_POINT('Ctrl Pts',(-18.5344403794479,12.8697533326654,
132.9251808791)) ;
#148130=CARTESIAN_POINT('Ctrl Pts',(-18.4650781878909,12.6186668419938,
132.755581911683)) ;
#148131=CARTESIAN_POINT('Ctrl Pts',(-18.3758902615424,12.4240570557475,
132.528231421364)) ;
#148132=CARTESIAN_POINT('Ctrl Pts',(-18.2732592245776,12.3017129015635,
132.261457008441)) ;
#148133=CARTESIAN_POINT('Ctrl Pts',(-18.1630414162269,12.259212443294,131.972645306552)) ;
#148134=CARTESIAN_POINT('Ctrl Pts',(-18.0528667103631,12.3002004247184,
131.683920182709)) ;
#148135=CARTESIAN_POINT('Ctrl Pts',(-17.9495131746608,12.4222100082891,
131.41522733535)) ;
#148136=CARTESIAN_POINT('Ctrl Pts',(-17.8604373492352,12.6151763777399,
131.188068661744)) ;
#148137=CARTESIAN_POINT('Ctrl Pts',(-17.7905190303083,12.8667635442981,
131.016997058462)) ;
#148138=CARTESIAN_POINT('Ctrl Pts',(-17.7445835247863,13.156608287975,130.915794965958)) ;
#148139=CARTESIAN_POINT('Ctrl Pts',(-17.7246276819165,13.4669634913823,
130.890658029617)) ;
#148140=CARTESIAN_POINT('Ctrl Pts',(-17.7317937319993,13.7743605544172,
130.944768434693)) ;
#148141=CARTESIAN_POINT('Ctrl Pts',(-17.7646329783859,14.0556835364492,
131.073777527433)) ;
#148142=CARTESIAN_POINT('Ctrl Pts',(-17.8201538331759,14.2923698340539,
131.269107271489)) ;
#148143=CARTESIAN_POINT('Ctrl Pts',(-17.8939804671672,14.4669398089711,
131.518026818099)) ;
#148144=CARTESIAN_POINT('Ctrl Pts',(-17.9790094951731,14.5658237072004,
131.799368733708)) ;
#148145=CARTESIAN_POINT('Ctrl Pts',(-18.0699355731019,14.5834030804103,
132.098247995134)) ;
#148146=CARTESIAN_POINT('Ctrl Pts',(-18.1579904994827,14.5182209640518,
132.388435699064)) ;
#148147=CARTESIAN_POINT('Ctrl Pts',(-18.2378368617494,14.3732472744243,
132.655041938253)) ;
#148148=CARTESIAN_POINT('Ctrl Pts',(-18.3012363737009,14.1617341160313,
132.873234199414)) ;
#148149=CARTESIAN_POINT('Ctrl Pts',(-18.3441500746653,13.8968739581495,
133.031718215328)) ;
#148150=CARTESIAN_POINT('Ctrl Pts',(-18.36238591691,13.5970561201623,133.118203483067)) ;
#148151=CARTESIAN_POINT('Ctrl Pts',(-18.353745765101,13.2853498772371,133.126116024577)) ;
#148152=CARTESIAN_POINT('Ctrl Pts',(-18.3186534118777,12.9854214225964,
133.056533301362)) ;
#148153=CARTESIAN_POINT('Ctrl Pts',(-18.2582555615791,12.7145026725385,
132.913294641903)) ;
#148154=CARTESIAN_POINT('Ctrl Pts',(-18.1767063643979,12.4953422799607,
132.708123384207)) ;
#148155=CARTESIAN_POINT('Ctrl Pts',(-18.0783433317562,12.341785792788,132.454021595677)) ;
#148156=CARTESIAN_POINT('Ctrl Pts',(-17.9707155643602,12.2665368205457,
132.172612709289)) ;
#148157=CARTESIAN_POINT('Ctrl Pts',(-17.8596316902576,12.2735361579836,
131.881255970493)) ;
#148158=CARTESIAN_POINT('Ctrl Pts',(-17.7527316072051,12.3632299170458,
131.602134296824)) ;
#148159=CARTESIAN_POINT('Ctrl Pts',(-17.6571606283092,12.5286847379392,
131.356056473991)) ;
#148160=CARTESIAN_POINT('Ctrl Pts',(-17.5788794210432,12.7579694052531,
131.16046780139)) ;
#148161=CARTESIAN_POINT('Ctrl Pts',(-17.5226365751704,13.0352202264865,
131.029305711414)) ;
#148162=CARTESIAN_POINT('Ctrl Pts',(-17.4918816488371,13.3405828522819,
130.972629478393)) ;
#148163=CARTESIAN_POINT('Ctrl Pts',(-17.4881115560766,13.6512271404406,
130.994714982278)) ;
#148164=CARTESIAN_POINT('Ctrl Pts',(-17.5107807119142,13.945858673121,131.094068308616)) ;
#148165=CARTESIAN_POINT('Ctrl Pts',(-17.5577200823908,14.2033946436315,
131.264378805117)) ;
#148166=CARTESIAN_POINT('Ctrl Pts',(-17.6244678428917,14.4040391097263,
131.492418461584)) ;
#148167=CARTESIAN_POINT('Ctrl Pts',(-17.7056627363047,14.5350227363909,
131.762669575012)) ;
#148168=CARTESIAN_POINT('Ctrl Pts',(-17.7954834341729,14.5864958768454,
132.058353936923)) ;
#148169=CARTESIAN_POINT('Ctrl Pts',(-17.885321308586,14.554416926093,132.353783687721)) ;
#148170=CARTESIAN_POINT('Ctrl Pts',(-17.9692937621649,14.4414134388981,
132.632251051087)) ;
#148171=CARTESIAN_POINT('Ctrl Pts',(-18.0401061570019,14.2551029689439,
132.872267335541)) ;
#148172=CARTESIAN_POINT('Ctrl Pts',(-18.0919280847591,14.0100365387615,
133.056707389317)) ;
#148173=CARTESIAN_POINT('Ctrl Pts',(-18.120568608652,13.7214335720741,133.173607236888)) ;
#148174=CARTESIAN_POINT('Ctrl Pts',(-18.1230342621043,13.4135493080175,
133.213803330473)) ;
#148175=CARTESIAN_POINT('Ctrl Pts',(-18.0984830751662,13.1045553567054,
133.175282525716)) ;
#148176=CARTESIAN_POINT('Ctrl Pts',(-18.0481691146944,12.8197359120567,
133.061332232554)) ;
#148177=CARTESIAN_POINT('Ctrl Pts',(-17.9741995914314,12.576213522993,132.878551316788)) ;
#148178=CARTESIAN_POINT('Ctrl Pts',(-17.882278063881,12.3952019972504,132.643060046006)) ;
#148179=CARTESIAN_POINT('Ctrl Pts',(-17.7773165034846,12.2871509168402,
132.369622625289)) ;
#148180=CARTESIAN_POINT('Ctrl Pts',(-17.6670900155522,12.2605661250461,
132.080610377323)) ;
#148181=CARTESIAN_POINT('Ctrl Pts',(-17.5571725360923,12.3174696014915,
131.792809249696)) ;
#148182=CARTESIAN_POINT('Ctrl Pts',(-17.4563916553665,12.45350954949,131.531487926555)) ;
#148183=CARTESIAN_POINT('Ctrl Pts',(-17.3704389160813,12.6588730933983,
131.313511700696)) ;
#148184=CARTESIAN_POINT('Ctrl Pts',(-17.3049297018148,12.9185732452431,
131.155205502056)) ;
#148185=CARTESIAN_POINT('Ctrl Pts',(-17.2636296695763,13.2144047021654,
131.067638080618)) ;
#148186=CARTESIAN_POINT('Ctrl Pts',(-17.2488249122446,13.5255441654578,
131.057510868015)) ;
#148187=CARTESIAN_POINT('Ctrl Pts',(-17.2609296287798,13.8297539954917,
131.126033363959)) ;
#148188=CARTESIAN_POINT('Ctrl Pts',(-17.2985030763623,14.1049217876101,
131.268992812532)) ;
#148189=CARTESIAN_POINT('Ctrl Pts',(-17.3575596549785,14.329872377713,131.474493311217)) ;
#148190=CARTESIAN_POINT('Ctrl Pts',(-17.4340909075981,14.491552798162,131.731324559513)) ;
#148191=CARTESIAN_POINT('Ctrl Pts',(-17.5210857954015,14.5755974464537,
132.01858139833)) ;
#148192=CARTESIAN_POINT('Ctrl Pts',(-17.6114837359406,14.5774288314458,
132.315662323554)) ;
#148193=CARTESIAN_POINT('Ctrl Pts',(-17.698796355316,14.4968431442199,132.603852489875)) ;
#148194=CARTESIAN_POINT('Ctrl Pts',(-17.775879820333,14.3385595684728,132.862263452361)) ;
#148195=CARTESIAN_POINT('Ctrl Pts',(-17.835998603421,14.1152210821619,133.070993327708)) ;
#148196=CARTESIAN_POINT('Ctrl Pts',(-17.874456885931,13.8419814694385,133.216493798034)) ;
#148197=CARTESIAN_POINT('Ctrl Pts',(-17.8876898230409,13.5398085198315,
133.28818438758)) ;
#148198=CARTESIAN_POINT('Ctrl Pts',(-17.8741319200142,13.2280435921434,
133.281749241004)) ;
#148199=CARTESIAN_POINT('Ctrl Pts',(-17.8337766712165,12.9300591046375,
133.197059291018)) ;
#148200=CARTESIAN_POINT('Ctrl Pts',(-17.7691101800502,12.6684084427586,
133.041237278321)) ;
#148201=CARTESIAN_POINT('Ctrl Pts',(-17.6840581698328,12.4608091594121,
132.825832817714)) ;
#148202=CARTESIAN_POINT('Ctrl Pts',(-17.5835644067408,12.3214093535999,
132.565418506094)) ;
#148203=CARTESIAN_POINT('Ctrl Pts',(-17.4740202572772,12.261330300397,132.27865503774)) ;
#148204=CARTESIAN_POINT('Ctrl Pts',(-17.3639381852683,12.2843254988424,
131.989996972432)) ;
#148205=CARTESIAN_POINT('Ctrl Pts',(-17.2586432752413,12.3887269721217,
131.71555751289)) ;
#148206=CARTESIAN_POINT('Ctrl Pts',(-17.1657956374155,12.5673627436567,
131.477456219259)) ;
#148207=CARTESIAN_POINT('Ctrl Pts',(-17.0911351100522,12.8080166806353,
131.292569279306)) ;
#148208=CARTESIAN_POINT('Ctrl Pts',(-17.0396694706571,13.0914774354823,
131.175275601717)) ;
#148209=CARTESIAN_POINT('Ctrl Pts',(-17.0139478947046,13.4005589670674,
131.133400258637)) ;
#148210=CARTESIAN_POINT('Ctrl Pts',(-17.0152836707085,13.7083911596742,
131.170245097133)) ;
#148211=CARTESIAN_POINT('Ctrl Pts',(-17.0428555359998,13.9985991378762,
131.284050048509)) ;
#148212=CARTESIAN_POINT('Ctrl Pts',(-17.0937913243256,14.2457812559265,
131.465901397237)) ;
#148213=CARTESIAN_POINT('Ctrl Pts',(-17.1637439823567,14.4345734153115,
131.703335486007)) ;
#148214=CARTESIAN_POINT('Ctrl Pts',(-17.2472660646445,14.5511370879547,
131.980487773352)) ;
#148215=CARTESIAN_POINT('Ctrl Pts',(-17.337120360927,14.5867802187907,132.276018738499)) ;
#148216=CARTESIAN_POINT('Ctrl Pts',(-17.4268009039852,14.5391948483821,
132.571169606425)) ;
#148217=CARTESIAN_POINT('Ctrl Pts',(-17.50867960202,14.411534541166,132.843482510367)) ;
#148218=CARTESIAN_POINT('Ctrl Pts',(-17.5762457585438,14.2134355911455,
133.073946320548)) ;
#148219=CARTESIAN_POINT('Ctrl Pts',(-17.6241241514975,13.9582377807151,
133.246970111031)) ;
#148220=CARTESIAN_POINT('Ctrl Pts',(-17.6479486624558,13.6646542857207,
133.349718970844)) ;
#148221=CARTESIAN_POINT('Ctrl Pts',(-17.6453414061695,13.354183694307,133.375210052951)) ;
#148222=CARTESIAN_POINT('Ctrl Pts',(-17.6158058941285,13.0484269475921,
133.322056715755)) ;
#148223=CARTESIAN_POINT('Ctrl Pts',(-17.560597882875,12.7694396144753,133.193932763753)) ;
#148224=CARTESIAN_POINT('Ctrl Pts',(-17.4834695817437,12.5380417818578,
133.001624723729)) ;
#148225=CARTESIAN_POINT('Ctrl Pts',(-17.3877869395594,12.3683286103215,
132.755475944)) ;
#148226=CARTESIAN_POINT('Ctrl Pts',(-17.2819063750014,12.2760420301782,
132.479111929425)) ;
#148227=CARTESIAN_POINT('Ctrl Pts',(-17.1709198373748,12.2649171956023,
132.1880250579)) ;
#148228=CARTESIAN_POINT('Ctrl Pts',(-17.0626411499466,12.3368690602114,
131.904826957427)) ;
#148229=CARTESIAN_POINT('Ctrl Pts',(-16.9637873323835,12.4871142426883,
131.64926067196)) ;
#148230=CARTESIAN_POINT('Ctrl Pts',(-16.8812937864313,12.7041605723025,
131.441394001432)) ;
#148231=CARTESIAN_POINT('Ctrl Pts',(-16.8200816285751,12.9721742229255,
131.295646395614)) ;
#148232=CARTESIAN_POINT('Ctrl Pts',(-16.7836474217345,13.2726902909237,
131.222315130629)) ;
#148233=CARTESIAN_POINT('Ctrl Pts',(-16.773935559665,13.5844634712024,131.227094828885)) ;
#148234=CARTESIAN_POINT('Ctrl Pts',(-16.7911394414361,13.8852370935213,
131.310575943605)) ;
#148235=CARTESIAN_POINT('Ctrl Pts',(-16.8328615291614,14.1508960461137,
131.465435883749)) ;
#148236=CARTESIAN_POINT('Ctrl Pts',(-16.8957649980785,14.3659570347197,
131.682335572948)) ;
#148237=CARTESIAN_POINT('Ctrl Pts',(-16.9747508643797,14.513384444757,131.946282517817)) ;
#148238=CARTESIAN_POINT('Ctrl Pts',(-17.0626794840163,14.58228249035,132.236157160365)) ;
#148239=CARTESIAN_POINT('Ctrl Pts',(-17.1535083371299,14.5684017700248,
132.534690900371)) ;
#148240=CARTESIAN_POINT('Ctrl Pts',(-17.2392135238107,14.4726240352221,
132.818127204052)) ;
#148241=CARTESIAN_POINT('Ctrl Pts',(-17.3135721300852,14.3009018256013,
133.068577196943)) ;
#148242=CARTESIAN_POINT('Ctrl Pts',(-17.3697922036115,14.0676662021592,
133.265814069086)) ;
#148243=CARTESIAN_POINT('Ctrl Pts',(-17.4038524116641,13.7867923428731,
133.398526236623)) ;
#148244=CARTESIAN_POINT('Ctrl Pts',(-17.4120797990217,13.4808115770732,
133.455650692552)) ;
#148245=CARTESIAN_POINT('Ctrl Pts',(-17.393480319056,13.1706177379304,133.434416238406)) ;
#148246=CARTESIAN_POINT('Ctrl Pts',(-17.3481649808676,12.8770484120512,
133.335317034958)) ;
#148247=CARTESIAN_POINT('Ctrl Pts',(-17.2795456429539,12.6251910549939,
133.167821675258)) ;
#148248=CARTESIAN_POINT('Ctrl Pts',(-17.191091114337,12.4289584768191,132.942537201925)) ;
#148249=CARTESIAN_POINT('Ctrl Pts',(-17.0882142927875,12.3038002387545,
132.675222788334)) ;
#148250=CARTESIAN_POINT('Ctrl Pts',(-16.978326475091,12.2593442699651,132.387300667687)) ;
#148251=CARTESIAN_POINT('Ctrl Pts',(-16.8683094798042,12.2978898769658,
132.098965870951)) ;
#148252=CARTESIAN_POINT('Ctrl Pts',(-16.7648959897926,12.4169444283248,
131.829998734971)) ;
#148253=CARTESIAN_POINT('Ctrl Pts',(-16.6747206222422,12.6093773195972,
131.599861765361)) ;
#148254=CARTESIAN_POINT('Ctrl Pts',(-16.6045685863941,12.8583734122104,
131.427937124288)) ;
#148255=CARTESIAN_POINT('Ctrl Pts',(-16.5577153827191,13.1480449714035,
131.324145807381)) ;
#148256=CARTESIAN_POINT('Ctrl Pts',(-16.5370475027575,13.4582417931766,
131.296933049071)) ;
#148257=CARTESIAN_POINT('Ctrl Pts',(-16.5434122344791,13.7655079117814,
131.348644885379)) ;
#148258=CARTESIAN_POINT('Ctrl Pts',(-16.57559115125,14.0483169670967,131.475777606241)) ;
#148259=CARTESIAN_POINT('Ctrl Pts',(-16.6304376248013,14.285999002941,131.669073710126)) ;
#148260=CARTESIAN_POINT('Ctrl Pts',(-16.7035444070544,14.4624790496655,
131.915796927174)) ;
#148261=CARTESIAN_POINT('Ctrl Pts',(-16.788889987511,14.5642183911393,132.198286823634)) ;
#148262=CARTESIAN_POINT('Ctrl Pts',(-16.8792004445873,14.5841609498882,
132.495150629956)) ;
#148263=CARTESIAN_POINT('Ctrl Pts',(-16.9679697628479,14.520970734674,132.787641400003)) ;
#148264=CARTESIAN_POINT('Ctrl Pts',(-17.0476011313862,14.3791779358065,
133.053372603054)) ;
#148265=CARTESIAN_POINT('Ctrl Pts',(-17.1119011916955,14.1688151362551,
133.274346330725)) ;
#148266=CARTESIAN_POINT('Ctrl Pts',(-17.1554181544879,13.9051957088918,
133.43458020011)) ;
#148267=CARTESIAN_POINT('Ctrl Pts',(-17.1743976183435,13.60715006879,133.523128764007)) ;
#148268=CARTESIAN_POINT('Ctrl Pts',(-17.1667123705159,13.2953843814918,
133.533839215501)) ;
#148269=CARTESIAN_POINT('Ctrl Pts',(-17.1321236360563,12.9930169526984,
133.465935301798)) ;
#148270=CARTESIAN_POINT('Ctrl Pts',(-17.0726673783466,12.7222273700058,
133.325286975909)) ;
#148271=CARTESIAN_POINT('Ctrl Pts',(-16.991448956747,12.500544093303,133.121191114684)) ;
#148272=CARTESIAN_POINT('Ctrl Pts',(-16.8935056731294,12.3451353324325,
132.868292190144)) ;
#148273=CARTESIAN_POINT('Ctrl Pts',(-16.7860479429717,12.2674914285865,
132.587388959171)) ;
#148274=CARTESIAN_POINT('Ctrl Pts',(-16.6746490295685,12.2722652657277,
132.295199791128)) ;
#148275=CARTESIAN_POINT('Ctrl Pts',(-16.5676447482205,12.3599738467364,
132.01575034793)) ;
#148276=CARTESIAN_POINT('Ctrl Pts',(-16.4720746525094,12.5226378491769,
131.769531391802)) ;
#148277=CARTESIAN_POINT('Ctrl Pts',(-16.3929497865683,12.7508222616319,
131.571573710982)) ;
#148278=CARTESIAN_POINT('Ctrl Pts',(-16.3359366151232,13.0279565462644,
131.438259358999)) ;
#148279=CARTESIAN_POINT('Ctrl Pts',(-16.3045984521949,13.3323087573567,
131.379816911574)) ;
#148280=CARTESIAN_POINT('Ctrl Pts',(-16.3000641118992,13.6420774120511,
131.399562313609)) ;
#148281=CARTESIAN_POINT('Ctrl Pts',(-16.3219465791947,13.9374078331077,
131.496607386123)) ;
#148282=CARTESIAN_POINT('Ctrl Pts',(-16.3681919814467,14.1965319396346,
131.664898838707)) ;
#148283=CARTESIAN_POINT('Ctrl Pts',(-16.4348677786798,14.3999725779251,
131.892918294996)) ;
#148284=CARTESIAN_POINT('Ctrl Pts',(-16.5153412365751,14.5320840128439,
132.160883084608)) ;
#148285=CARTESIAN_POINT('Ctrl Pts',(-16.6048687150457,14.5862914481129,
132.455659839408)) ;
#148286=CARTESIAN_POINT('Ctrl Pts',(-16.6952852040637,14.5562373183141,
132.752967353517)) ;
#148287=CARTESIAN_POINT('Ctrl Pts',(-16.7790126449957,14.4460760086482,
133.030515124208)) ;
#148288=CARTESIAN_POINT('Ctrl Pts',(-16.8506184653848,14.2613118690052,
133.272970541313)) ;
#148289=CARTESIAN_POINT('Ctrl Pts',(-16.9030456298473,14.0168342944471,
133.459259475347)) ;
#148290=CARTESIAN_POINT('Ctrl Pts',(-16.9322577874261,13.7314084921459,
133.57757681541)) ;
#148291=CARTESIAN_POINT('Ctrl Pts',(-16.9355345400515,13.4213927772855,
133.620410847763)) ;
#148292=CARTESIAN_POINT('Ctrl Pts',(-16.9118235568279,13.1138964811438,
133.584144735377)) ;
#148293=CARTESIAN_POINT('Ctrl Pts',(-16.8621882966479,12.8273574964974,
133.472259648909)) ;
#148294=CARTESIAN_POINT('Ctrl Pts',(-16.7887479806333,12.5821904273637,
133.291045013938)) ;
#148295=CARTESIAN_POINT('Ctrl Pts',(-16.6971693689497,12.3992406636329,
133.056586334083)) ;
#148296=CARTESIAN_POINT('Ctrl Pts',(-16.592840687638,12.2892635372044,132.784882740936)) ;
#148297=CARTESIAN_POINT('Ctrl Pts',(-16.4824515586233,12.2601882731061,
132.495468659447)) ;
#148298=CARTESIAN_POINT('Ctrl Pts',(-16.3727887175883,12.3144490332909,
132.208288643135)) ;
#148299=CARTESIAN_POINT('Ctrl Pts',(-16.2715474674814,12.4481500310982,
131.945651708052)) ;
#148300=CARTESIAN_POINT('Ctrl Pts',(-16.1850122658441,12.6515765338915,
131.725979718577)) ;
#148301=CARTESIAN_POINT('Ctrl Pts',(-16.1185129147627,12.9112090409297,
131.564943253957)) ;
#148302=CARTESIAN_POINT('Ctrl Pts',(-16.0765700513496,13.2069680634014,
131.475556101884)) ;
#148303=CARTESIAN_POINT('Ctrl Pts',(-16.0610820422751,13.5165270688446,
131.463274345175)) ;
#148304=CARTESIAN_POINT('Ctrl Pts',(-16.0725280585734,13.8224961105202,
131.530016185453)) ;
#148305=CARTESIAN_POINT('Ctrl Pts',(-16.1092827001771,14.0973150070006,
131.670412542272)) ;
#148306=CARTESIAN_POINT('Ctrl Pts',(-16.1678671523189,14.3244517952957,
131.874605730233)) ;
#148307=CARTESIAN_POINT('Ctrl Pts',(-16.2438791319829,14.4877799553715,
132.129858835317)) ;
#148308=CARTESIAN_POINT('Ctrl Pts',(-16.3305380227414,14.5742904873528,
132.416097152061)) ;
#148309=CARTESIAN_POINT('Ctrl Pts',(-16.4213187544321,14.5785355411289,
132.714436240136)) ;
#148310=CARTESIAN_POINT('Ctrl Pts',(-16.5087008967038,14.4999983215905,
133.002794438483)) ;
#148311=CARTESIAN_POINT('Ctrl Pts',(-16.5858465437254,14.3447574247582,
133.261227247573)) ;
#148312=CARTESIAN_POINT('Ctrl Pts',(-16.6467792052261,14.1223924190304,
133.472459939162)) ;
#148313=CARTESIAN_POINT('Ctrl Pts',(-16.6858377372559,13.8510686498015,
133.619622649373)) ;
#148314=CARTESIAN_POINT('Ctrl Pts',(-16.6999157232596,13.5484336095185,
133.693900204533)) ;
#148315=CARTESIAN_POINT('Ctrl Pts',(-16.6870922505193,13.2370241566132,
133.689564216562)) ;
#148316=CARTESIAN_POINT('Ctrl Pts',(-16.6476640703555,12.9391311523709,
133.60748871607)) ;
#148317=CARTESIAN_POINT('Ctrl Pts',(-16.5836531085729,12.6756660362993,
133.453625999795)) ;
#148318=CARTESIAN_POINT('Ctrl Pts',(-16.4988970609242,12.4657027909829,
133.239173128773)) ;
#148319=CARTESIAN_POINT('Ctrl Pts',(-16.3988089904537,12.324474551251,132.979918734029)) ;
#148320=CARTESIAN_POINT('Ctrl Pts',(-16.2899174957269,12.2619232759168,
132.694915080436)) ;
#148321=CARTESIAN_POINT('Ctrl Pts',(-16.1789998814677,12.2825882347195,
132.40405140961)) ;
#148322=CARTESIAN_POINT('Ctrl Pts',(-16.0738071067368,12.3846501160854,
132.129802156463)) ;
#148323=CARTESIAN_POINT('Ctrl Pts',(-15.9805197501771,12.5611187121008,
131.890409483026)) ;
#148324=CARTESIAN_POINT('Ctrl Pts',(-15.9052414037615,12.800128888062,131.703709693564)) ;
#148325=CARTESIAN_POINT('Ctrl Pts',(-15.8530321981078,13.0829558390025,
131.584286648028)) ;
#148326=CARTESIAN_POINT('Ctrl Pts',(-15.8265593389286,13.3903655442342,
131.540077569351)) ;
#148327=CARTESIAN_POINT('Ctrl Pts',(-15.8271016367445,13.7001366182577,
131.574787860055)) ;
#148328=CARTESIAN_POINT('Ctrl Pts',(-15.853828406241,13.9898881867711,131.685965203616)) ;
#148329=CARTESIAN_POINT('Ctrl Pts',(-15.9041829439333,14.2391934618933,
131.866194894701)) ;
#148330=CARTESIAN_POINT('Ctrl Pts',(-15.9735601601396,14.4298567293758,
132.101910083047)) ;
#148331=CARTESIAN_POINT('Ctrl Pts',(-16.0572845306013,14.5492471460414,
132.379848702365)) ;
#148332=CARTESIAN_POINT('Ctrl Pts',(-16.1467466300587,14.5868020956478,
132.674116206761)) ;
#148333=CARTESIAN_POINT('Ctrl Pts',(-16.2364624285869,14.5417975160937,
132.969339452112)) ;
#148334=CARTESIAN_POINT('Ctrl Pts',(-16.3186966945366,14.416208825978,133.242712197891)) ;
#148335=CARTESIAN_POINT('Ctrl Pts',(-16.3867169591892,14.22040833296,133.474453835102)) ;
#148336=CARTESIAN_POINT('Ctrl Pts',(-16.4354660410799,13.9647701256438,
133.650242067901)) ;
#148337=CARTESIAN_POINT('Ctrl Pts',(-16.4598035300757,13.6739288758575,
133.75425884754)) ;
#148338=CARTESIAN_POINT('Ctrl Pts',(-16.4579839350789,13.3623285139176,
133.782197585911)) ;
#148339=CARTESIAN_POINT('Ctrl Pts',(-16.4292625349313,13.0574724687543,
133.731279710622)) ;
#148340=CARTESIAN_POINT('Ctrl Pts',(-16.374866435716,12.7770677304932,133.605541007664)) ;
#148341=CARTESIAN_POINT('Ctrl Pts',(-16.2976392682529,12.5427865194022,
133.413183101308)) ;
#148342=CARTESIAN_POINT('Ctrl Pts',(-16.2035752797556,12.3731888439483,
133.171342588508)) ;
#148343=CARTESIAN_POINT('Ctrl Pts',(-16.0973342716302,12.2773794382998,
132.894136279027)) ;
#148344=CARTESIAN_POINT('Ctrl Pts',(-15.9860703154779,12.2641879645069,
132.602324249829)) ;
#148345=CARTESIAN_POINT('Ctrl Pts',(-15.8780029132509,12.3335960528712,
132.319627851263)) ;
#148346=CARTESIAN_POINT('Ctrl Pts',(-15.7787561476632,12.4815616516049,
132.062913298757)) ;
#148347=CARTESIAN_POINT('Ctrl Pts',(-15.6956710002437,12.6968287193189,
131.85332343263)) ;
#148348=CARTESIAN_POINT('Ctrl Pts',(-15.6336749818423,12.9642190193072,
131.705359751562)) ;
#148349=CARTESIAN_POINT('Ctrl Pts',(-15.5965148974486,13.2637554960381,
131.629865315315)) ;
#148350=CARTESIAN_POINT('Ctrl Pts',(-15.5861011095343,13.5766923878532,
131.632725594872)) ;
#148351=CARTESIAN_POINT('Ctrl Pts',(-15.6023489976743,13.875372212648,131.713101997748)) ;
#148352=CARTESIAN_POINT('Ctrl Pts',(-15.6436597772124,14.1446745454968,
131.86704227389)) ;
#148353=CARTESIAN_POINT('Ctrl Pts',(-15.7060100158634,14.3606486125631,
132.082254737154)) ;
#148354=CARTESIAN_POINT('Ctrl Pts',(-15.7843216644605,14.5100785842148,
132.344127870228)) ;
#148355=CARTESIAN_POINT('Ctrl Pts',(-15.8727612750498,14.581577583442,132.635751029614)) ;
#148356=CARTESIAN_POINT('Ctrl Pts',(-15.9629519571558,14.5700419857243,
132.932166916061)) ;
#148357=CARTESIAN_POINT('Ctrl Pts',(-16.0493003352905,14.4761037677004,
133.217652319363)) ;
#148358=CARTESIAN_POINT('Ctrl Pts',(-16.1236984343831,14.3074346492421,
133.468021805579)) ;
#148359=CARTESIAN_POINT('Ctrl Pts',(-16.1809456998344,14.0735726196759,
133.668564628927)) ;
#148360=CARTESIAN_POINT('Ctrl Pts',(-16.2152999512208,13.7966474612173,
133.801775914891)) ;
#148361=CARTESIAN_POINT('Ctrl Pts',(-16.2244569868023,13.4894705422107,
133.861811553858)) ;
#148362=CARTESIAN_POINT('Ctrl Pts',(-16.2066485882241,13.1800818443726,
133.842775723282)) ;
#148363=CARTESIAN_POINT('Ctrl Pts',(-16.1621152395961,12.8853356216509,
133.745994410451)) ;
#148364=CARTESIAN_POINT('Ctrl Pts',(-16.0940667692907,12.6318026022688,
133.580197551014)) ;
#148365=CARTESIAN_POINT('Ctrl Pts',(-16.0060721923492,12.4337108519891,
133.356267245877)) ;
#148366=CARTESIAN_POINT('Ctrl Pts',(-15.903730601277,12.3064394714406,133.090449633245)) ;
#148367=CARTESIAN_POINT('Ctrl Pts',(-15.7936389437268,12.2594672533841,
132.802032639163)) ;
#148368=CARTESIAN_POINT('Ctrl Pts',(-15.6836419614988,12.2954707769561,
132.513712206169)) ;
#148369=CARTESIAN_POINT('Ctrl Pts',(-15.5793368562183,12.4135506751844,
132.242361064916)) ;
#148370=CARTESIAN_POINT('Ctrl Pts',(-15.489886034823,12.6014761711869,132.013888945583)) ;
#148371=CARTESIAN_POINT('Ctrl Pts',(-15.4184189651294,12.8505488628237,
131.838381349536)) ;
#148372=CARTESIAN_POINT('Ctrl Pts',(-15.3709336783578,13.1393106619413,
131.732721363692)) ;
#148373=CARTESIAN_POINT('Ctrl Pts',(-15.3494680304114,13.4495612623856,
131.70321675522)) ;
#148374=CARTESIAN_POINT('Ctrl Pts',(-15.3550699615667,13.756653092605,131.752638136779)) ;
#148375=CARTESIAN_POINT('Ctrl Pts',(-15.3864985515293,14.0404143429371,
131.877571942581)) ;
#148376=CARTESIAN_POINT('Ctrl Pts',(-15.4407185610853,14.279856789825,132.069044870554)) ;
#148377=CARTESIAN_POINT('Ctrl Pts',(-15.5137414504908,14.458860778503,132.315668883867)) ;
#148378=CARTESIAN_POINT('Ctrl Pts',(-15.5983584888055,14.5622468104248,
132.595839857605)) ;
#148379=CARTESIAN_POINT('Ctrl Pts',(-15.6889603783722,14.5847589311911,
132.893687701564)) ;
#148380=CARTESIAN_POINT('Ctrl Pts',(-15.7776166007816,14.5239999496504,
133.185745577127)) ;
#148381=CARTESIAN_POINT('Ctrl Pts',(-15.8577182680662,14.3842926160759,
133.452895744165)) ;
#148382=CARTESIAN_POINT('Ctrl Pts',(-15.9225060605763,14.1758059361387,
133.675275406814)) ;
#148383=CARTESIAN_POINT('Ctrl Pts',(-15.9667693658469,13.9130884623637,
133.837741432542)) ;
#148384=CARTESIAN_POINT('Ctrl Pts',(-15.9864293474601,13.6151580257587,
133.928333937263)) ;
#148385=CARTESIAN_POINT('Ctrl Pts',(-15.9795433739699,13.3050554492312,
133.941210084392)) ;
#148386=CARTESIAN_POINT('Ctrl Pts',(-15.9458051665583,13.0018871941951,
133.87580827376)) ;
#148387=CARTESIAN_POINT('Ctrl Pts',(-15.886867851103,12.7291798147193,133.736763615943)) ;
#148388=CARTESIAN_POINT('Ctrl Pts',(-15.8062485274327,12.5061726886818,
133.534385452508)) ;
#148389=CARTESIAN_POINT('Ctrl Pts',(-15.709090071799,12.3489726322612,133.283660587009)) ;
#148390=CARTESIAN_POINT('Ctrl Pts',(-15.6014248041649,12.2685650125514,
133.002280999057)) ;
#148391=CARTESIAN_POINT('Ctrl Pts',(-15.4904361859871,12.2709027437165,
132.711164577751)) ;
#148392=CARTESIAN_POINT('Ctrl Pts',(-15.3831558118205,12.3558100296643,
132.43091349999)) ;
#148393=CARTESIAN_POINT('Ctrl Pts',(-15.2866992677918,12.5172181925544,
132.182267547668)) ;
#148394=CARTESIAN_POINT('Ctrl Pts',(-15.2072741208272,12.7432705327431,
131.983342377859)) ;
#148395=CARTESIAN_POINT('Ctrl Pts',(-15.1496737200748,13.0180147425716,
131.848185472719)) ;
#148396=CARTESIAN_POINT('Ctrl Pts',(-15.117338984736,13.3228199509295,131.786946071819)) ;
#148397=CARTESIAN_POINT('Ctrl Pts',(-15.1120300611744,13.6334362143055,
131.804503087611)) ;
#148398=CARTESIAN_POINT('Ctrl Pts',(-15.133206576665,13.9294163259488,131.899479737668)) ;
#148399=CARTESIAN_POINT('Ctrl Pts',(-15.1786478514763,14.18915702975,132.06532627885)) ;
#148400=CARTESIAN_POINT('Ctrl Pts',(-15.2447211372006,14.3946402056162,
132.291578267309)) ;
#148401=CARTESIAN_POINT('Ctrl Pts',(-15.3251751438084,14.5295568967571,
132.559617062532)) ;
#148402=CARTESIAN_POINT('Ctrl Pts',(-15.4146594754138,14.5858061312981,
132.854298517614)) ;
#148403=CARTESIAN_POINT('Ctrl Pts',(-15.5046539633587,14.5585141748975,
133.150186644236)) ;
#148404=CARTESIAN_POINT('Ctrl Pts',(-15.5891258692447,14.4500372195652,
133.430097010254)) ;
#148405=CARTESIAN_POINT('Ctrl Pts',(-15.6607651079543,14.268202021056,133.672458105674)) ;
#148406=CARTESIAN_POINT('Ctrl Pts',(-15.7140410362885,14.0250734165881,
133.861293481273)) ;
#148407=CARTESIAN_POINT('Ctrl Pts',(-15.7440399667486,13.7389393522913,
133.982084980378)) ;
#148408=CARTESIAN_POINT('Ctrl Pts',(-15.7480042443892,13.4311037013635,
134.026729053662)) ;
#148409=CARTESIAN_POINT('Ctrl Pts',(-15.725216194089,13.1229020286871,133.99318973845)) ;
#148410=CARTESIAN_POINT('Ctrl Pts',(-15.6757479823679,12.8333723840705,
133.882056709305)) ;
#148411=CARTESIAN_POINT('Ctrl Pts',(-15.6036828412038,12.5895126798869,
133.704489921503)) ;
#148412=CARTESIAN_POINT('Ctrl Pts',(-15.5123148806256,12.4035405009807,
133.470777242786)) ;
#148413=CARTESIAN_POINT('Ctrl Pts',(-15.4082687921079,12.2914040510789,
133.199889537963)) ;
#148414=CARTESIAN_POINT('Ctrl Pts',(-15.2978395575661,12.2598122659222,
132.910395491718)) ;
#148415=CARTESIAN_POINT('Ctrl Pts',(-15.1879820024828,12.3118570167027,
132.622666675303)) ;
#148416=CARTESIAN_POINT('Ctrl Pts',(-15.0866174671626,12.4430958660728,
132.359601883501)) ;
#148417=CARTESIAN_POINT('Ctrl Pts',(-14.9994898421019,12.6447072426792,
132.138218711282)) ;
#148418=CARTESIAN_POINT('Ctrl Pts',(-14.9323676753914,12.9030426920416,
131.97536643828)) ;
#148419=CARTESIAN_POINT('Ctrl Pts',(-14.889699513773,13.1970328957413,131.883755713314)) ;
#148420=CARTESIAN_POINT('Ctrl Pts',(-14.8733792116843,13.5084312803207,
131.869259402362)) ;
#148421=CARTESIAN_POINT('Ctrl Pts',(-14.8839158623484,13.8121187578149,
131.933031558723)) ;
#148422=CARTESIAN_POINT('Ctrl Pts',(-14.9200803244134,14.0900961815241,
132.071930113077)) ;
#148423=CARTESIAN_POINT('Ctrl Pts',(-14.9781162973069,14.318729906323,132.274505126265)) ;
#148424=CARTESIAN_POINT('Ctrl Pts',(-15.0539330025022,14.4844226904234,
132.529278687657)) ;
#148425=CARTESIAN_POINT('Ctrl Pts',(-15.1400286374453,14.5727758768623,
132.813733105511)) ;
#148426=CARTESIAN_POINT('Ctrl Pts',(-15.2307985166822,14.5796460537581,
133.112046749388)) ;
#148427=CARTESIAN_POINT('Ctrl Pts',(-15.3184170761058,14.5035865884274,
133.401102281981)) ;
#148428=CARTESIAN_POINT('Ctrl Pts',(-15.3962623480525,14.3497063605797,
133.661718798962)) ;
#148429=CARTESIAN_POINT('Ctrl Pts',(-15.4575770963959,14.1291330540675,
133.874017192935)) ;
#148430=CARTESIAN_POINT('Ctrl Pts',(-15.4972251378502,13.8597727323871,
134.022812003589)) ;
#148431=CARTESIAN_POINT('Ctrl Pts',(-15.5120947637313,13.5574624461298,
134.099434676898)) ;
#148432=CARTESIAN_POINT('Ctrl Pts',(-15.5000961472788,13.2463366204199,
134.097469103472)) ;
#148433=CARTESIAN_POINT('Ctrl Pts',(-15.4613504305426,12.9472974044437,
134.017442332404)) ;
#148434=CARTESIAN_POINT('Ctrl Pts',(-15.3982335033183,12.6832078495132,
133.866092641497)) ;
#148435=CARTESIAN_POINT('Ctrl Pts',(-15.3136235000347,12.4704982882043,
133.652221747533)) ;
#148436=CARTESIAN_POINT('Ctrl Pts',(-15.214236945017,12.3276823498278,133.394894350722)) ;
#148437=CARTESIAN_POINT('Ctrl Pts',(-15.1052928206969,12.2625925248945,
133.109808487118)) ;
#148438=CARTESIAN_POINT('Ctrl Pts',(-14.9947038779737,12.2806192118825,
132.819787448895)) ;
#148439=CARTESIAN_POINT('Ctrl Pts',(-14.8885598216415,12.3809214505585,
132.542973408766)) ;
#148440=CARTESIAN_POINT('Ctrl Pts',(-14.7948852153021,12.5560400972574,
132.302471269315)) ;
#148441=CARTESIAN_POINT('Ctrl Pts',(-14.7195025533567,12.7918901255773,
132.115247829854)) ;
#148442=CARTESIAN_POINT('Ctrl Pts',(-14.6663732001335,13.0744209582552,
131.993234262889)) ;
#148443=CARTESIAN_POINT('Ctrl Pts',(-14.6391629470329,13.3812416621058,
131.946846616762)) ;
#148444=CARTESIAN_POINT('Ctrl Pts',(-14.6389300517192,13.6920797035989,
131.979379504455)) ;
#148445=CARTESIAN_POINT('Ctrl Pts',(-14.6650391462422,13.9824941706661,
132.088747695719)) ;
#148446=CARTESIAN_POINT('Ctrl Pts',(-14.7145031098689,14.2323227455577,
132.266232509409)) ;
#148447=CARTESIAN_POINT('Ctrl Pts',(-14.7838483066136,14.4258243493526,
132.502056323187)) ;
#148448=CARTESIAN_POINT('Ctrl Pts',(-14.866526759289,14.5465247232896,132.776639574897)) ;
#148449=CARTESIAN_POINT('Ctrl Pts',(-14.9567274078562,14.5869806832562,
133.073382776381)) ;
#148450=CARTESIAN_POINT('Ctrl Pts',(-15.0460438527412,14.5442058471831,
133.367252021219)) ;
#148451=CARTESIAN_POINT('Ctrl Pts',(-15.1287759346931,14.4209679601538,
133.642135315366)) ;
#148452=CARTESIAN_POINT('Ctrl Pts',(-15.1974643909208,14.2257906584797,
133.875970776234)) ;
#148453=CARTESIAN_POINT('Ctrl Pts',(-15.2463765672829,13.9741287735189,
134.051901863982)) ;
#148454=CARTESIAN_POINT('Ctrl Pts',(-15.2717007785664,13.6829512518686,
134.158957987928)) ;
#148455=CARTESIAN_POINT('Ctrl Pts',(-15.2706427731617,13.3714665393579,
134.189124517144)) ;
#148456=CARTESIAN_POINT('Ctrl Pts',(-15.2426215285773,13.0656058649526,
134.140315862993)) ;
#148457=CARTESIAN_POINT('Ctrl Pts',(-15.1890339489811,12.7850334641615,
134.01684584536)) ;
#148458=CARTESIAN_POINT('Ctrl Pts',(-15.1127899010191,12.5496673057456,
133.827241053212)) ;
#148459=CARTESIAN_POINT('Ctrl Pts',(-15.0185001648777,12.3766688601944,
133.584981659701)) ;
#148460=CARTESIAN_POINT('Ctrl Pts',(-14.912490210718,12.2789529253499,133.308438535154)) ;
#148461=CARTESIAN_POINT('Ctrl Pts',(-14.8014556247031,12.2634413511376,
133.017242215912)) ;
#148462=CARTESIAN_POINT('Ctrl Pts',(-14.6931943926143,12.330415688247,132.733981368436)) ;
#148463=CARTESIAN_POINT('Ctrl Pts',(-14.5932657061769,12.4770343788681,
132.475395513356)) ;
#148464=CARTESIAN_POINT('Ctrl Pts',(-14.5101133772823,12.6896430070817,
132.265442710562)) ;
#148465=CARTESIAN_POINT('Ctrl Pts',(-14.4474157308921,12.9554491336733,
132.11540732339)) ;
#148466=CARTESIAN_POINT('Ctrl Pts',(-14.4094541017876,13.2546655218149,
132.037609868002)) ;
#148467=CARTESIAN_POINT('Ctrl Pts',(-14.3982126656332,13.5672374700513,
132.038011586952)) ;
#148468=CARTESIAN_POINT('Ctrl Pts',(-14.4137840127669,13.8673527502542,
132.116509502837)) ;
#148469=CARTESIAN_POINT('Ctrl Pts',(-14.4541638705567,14.1367235720608,
132.267567923076)) ;
#148470=CARTESIAN_POINT('Ctrl Pts',(-14.5164519603104,14.3561276375805,
132.482861480637)) ;
#148471=CARTESIAN_POINT('Ctrl Pts',(-14.5940341567091,14.5065131525026,
132.742424354294)) ;
#148472=CARTESIAN_POINT('Ctrl Pts',(-14.6820502398555,14.58061768968,133.032736112524)) ;
#148473=CARTESIAN_POINT('Ctrl Pts',(-14.772575059781,14.5715966995796,133.330239185716)) ;
#148474=CARTESIAN_POINT('Ctrl Pts',(-14.8591820385415,14.4799160826423,
133.616486751543)) ;
#148475=CARTESIAN_POINT('Ctrl Pts',(-14.9340155751519,14.3130126299592,
133.868154506662)) ;
#148476=CARTESIAN_POINT('Ctrl Pts',(-14.991608157995,14.0821691922297,134.069528062715)) ;
#148477=CARTESIAN_POINT('Ctrl Pts',(-15.0269433497899,13.8046645474474,
134.205816059215)) ;
#148478=CARTESIAN_POINT('Ctrl Pts',(-15.0367628763332,13.4979411063597,
134.26777705295)) ;
#148479=CARTESIAN_POINT('Ctrl Pts',(-15.0197321004595,13.1889484059184,
134.250957541032)) ;
#148480=CARTESIAN_POINT('Ctrl Pts',(-14.9760933322257,12.8939178579835,
134.15672056437)) ;
#148481=CARTESIAN_POINT('Ctrl Pts',(-14.9083892418113,12.637823938518,133.992078634426)) ;
#148482=CARTESIAN_POINT('Ctrl Pts',(-14.8208560907062,12.4382802201008,
133.769479809402)) ;
#148483=CARTESIAN_POINT('Ctrl Pts',(-14.7192841012341,12.3092349682175,
133.50577189094)) ;
#148484=CARTESIAN_POINT('Ctrl Pts',(-14.6089364049052,12.2595575247746,
133.216721659976)) ;
#148485=CARTESIAN_POINT('Ctrl Pts',(-14.4990459288312,12.2934341304884,
132.928661167576)) ;
#148486=CARTESIAN_POINT('Ctrl Pts',(-14.3949781008443,12.4080333824313,
132.657808436135)) ;
#148487=CARTESIAN_POINT('Ctrl Pts',(-14.3040123177586,12.5960960423707,
132.425286386828)) ;
#148488=CARTESIAN_POINT('Ctrl Pts',(-14.2323706381693,12.8430835958632,
132.249132507019)) ;
#148489=CARTESIAN_POINT('Ctrl Pts',(-14.1842155266943,13.1299282675871,
132.14141612179)) ;
#148490=CARTESIAN_POINT('Ctrl Pts',(-14.1618825011132,13.4413370820985,
132.109530327437)) ;
#148491=CARTESIAN_POINT('Ctrl Pts',(-14.1667760289367,13.7480777778484,
132.156806610371)) ;
#148492=CARTESIAN_POINT('Ctrl Pts',(-14.1974678546853,14.0327532847483,
132.279580684498)) ;
#148493=CARTESIAN_POINT('Ctrl Pts',(-14.2510444053685,14.2736050816731,
132.469152013831)) ;
#148494=CARTESIAN_POINT('Ctrl Pts',(-14.323668194567,14.454731415087,132.714635917315)) ;
#148495=CARTESIAN_POINT('Ctrl Pts',(-14.4079059599784,14.5602675657722,
132.99365390726)) ;
#148496=CARTESIAN_POINT('Ctrl Pts',(-14.4985138900094,14.5853381818847,
133.291544672069)) ;
#148497=CARTESIAN_POINT('Ctrl Pts',(-14.5874144035252,14.5268296040502,
133.584352082136)) ;
#148498=CARTESIAN_POINT('Ctrl Pts',(-14.6678119138476,14.3893357844739,
133.852346334359)) ;
#148499=CARTESIAN_POINT('Ctrl Pts',(-14.7331376309536,14.1825587222419,
134.076310009883)) ;
#148500=CARTESIAN_POINT('Ctrl Pts',(-14.7780213031554,13.9213688559687,
134.240558829846)) ;
#148501=CARTESIAN_POINT('Ctrl Pts',(-14.7984215319615,13.6242448062503,
134.333308668138)) ;
#148502=CARTESIAN_POINT('Ctrl Pts',(-14.7924127716866,13.3143404196874,
134.348729861162)) ;
#148503=CARTESIAN_POINT('Ctrl Pts',(-14.7590472201161,13.0084390891239,
134.28467058425)) ;
#148504=CARTESIAN_POINT('Ctrl Pts',(-14.7012646791225,12.7371909250803,
134.148690857043)) ;
#148505=CARTESIAN_POINT('Ctrl Pts',(-14.6209599760378,12.5114338285413,
133.947367407138)) ;
#148506=CARTESIAN_POINT('Ctrl Pts',(-14.5242191003668,12.3524149668545,
133.697838780998)) ;
#148507=CARTESIAN_POINT('Ctrl Pts',(-14.4166271811855,12.2696328079286,
133.416714729971)) ;
#148508=CARTESIAN_POINT('Ctrl Pts',(-14.3056942095112,12.2697667262583,
133.125742805927)) ;
#148509=CARTESIAN_POINT('Ctrl Pts',(-14.1983796924837,12.352219690353,132.845338479333)) ;
#148510=CARTESIAN_POINT('Ctrl Pts',(-14.1014667534168,12.5116177208884,
132.595377130338)) ;
#148511=CARTESIAN_POINT('Ctrl Pts',(-14.0214433689727,12.7360826900141,
132.39471532807)) ;
#148512=CARTESIAN_POINT('Ctrl Pts',(-13.9630322762884,13.0105746787141,
132.257287201062)) ;
#148513=CARTESIAN_POINT('Ctrl Pts',(-13.9300917396253,13.3146278251872,
132.194246081439)) ;
#148514=CARTESIAN_POINT('Ctrl Pts',(-13.9240153938967,13.6243831521928,
132.209458290046)) ;
#148515=CARTESIAN_POINT('Ctrl Pts',(-13.944508427021,13.9217978,132.302518124968)) ;
#148516=CARTESIAN_POINT('Ctrl Pts',(-13.9892221339268,14.1821018146301,
132.466153950012)) ;
#148517=CARTESIAN_POINT('Ctrl Pts',(-14.0546602899526,14.389412327527,132.690519984618)) ;
#148518=CARTESIAN_POINT('Ctrl Pts',(-14.1350488271771,14.5268848285114,
132.958477718458)) ;
#148519=CARTESIAN_POINT('Ctrl Pts',(-14.2240994741948,14.5852561648766,
133.251782240412)) ;
#148520=CARTESIAN_POINT('Ctrl Pts',(-14.3142069860548,14.5605921402289,
133.548016849623)) ;
#148521=CARTESIAN_POINT('Ctrl Pts',(-14.3990505698622,14.4542388550499,
133.829054466345)) ;
#148522=CARTESIAN_POINT('Ctrl Pts',(-14.4711893889587,14.2743936343232,
134.072880951258)) ;
#148523=CARTESIAN_POINT('Ctrl Pts',(-14.5251681508735,14.0316377250169,
134.263898633615)) ;
#148524=CARTESIAN_POINT('Ctrl Pts',(-14.5556789963755,13.7487556151288,
134.38591936868)) ;
#148525=CARTESIAN_POINT('Ctrl Pts',(-14.5604714220069,13.4387761363986,
134.433258068243)) ;
#148526=CARTESIAN_POINT('Ctrl Pts',(-14.5384491661002,13.1317846555727,
134.401792713465)) ;
#148527=CARTESIAN_POINT('Ctrl Pts',(-14.4896993568433,12.8410201879509,
134.292793596079)) ;
#148528=CARTESIAN_POINT('Ctrl Pts',(-14.418425254601,12.5963885995688,134.117448315784)) ;
#148529=CARTESIAN_POINT('Ctrl Pts',(-14.3277290025618,12.4083250165559,
133.885656271006)) ;
#148530=CARTESIAN_POINT('Ctrl Pts',(-14.2232683046687,12.2932606232103,
133.613777294112)) ;
#148531=CARTESIAN_POINT('Ctrl Pts',(-14.1134438296,12.2596773192959,133.325888983821)) ;
#148532=CARTESIAN_POINT('Ctrl Pts',(-14.0035198626591,12.3089369828892,
133.037945712624)) ;
#148533=CARTESIAN_POINT('Ctrl Pts',(-13.9014057493695,12.4384179061081,
132.772818300622)) ;
#148534=CARTESIAN_POINT('Ctrl Pts',(-13.8137301697272,12.6389284410988,
132.549896696867)) ;
#148535=CARTESIAN_POINT('Ctrl Pts',(-13.7464647647404,12.893636868565,132.386346900933)) ;
#148536=CARTESIAN_POINT('Ctrl Pts',(-13.7026544223093,13.1890353043008,
132.291660086028)) ;
#148537=CARTESIAN_POINT('Ctrl Pts',(-13.6856968381069,13.4997523656822,
132.275235904602)) ;
#148538=CARTESIAN_POINT('Ctrl Pts',(-13.6955051304073,13.8039808891053,
132.336895895886)) ;
#148539=CARTESIAN_POINT('Ctrl Pts',(-13.730811067449,14.0820721620834,132.473158857497)) ;
#148540=CARTESIAN_POINT('Ctrl Pts',(-13.7884136291909,14.3130040763869,
132.6745633012)) ;
#148541=CARTESIAN_POINT('Ctrl Pts',(-13.8634361976948,14.4800545179009,
132.926857790848)) ;
#148542=CARTESIAN_POINT('Ctrl Pts',(-13.9495289714166,14.5714591887958,
133.211406715331)) ;
#148543=CARTESIAN_POINT('Ctrl Pts',(-14.0407314511908,14.5804983866051,
133.511146111532)) ;
#148544=CARTESIAN_POINT('Ctrl Pts',(-14.1280999903725,14.5069052438345,
133.799313871286)) ;
#148545=CARTESIAN_POINT('Ctrl Pts',(-14.2062273655573,14.3557029930728,
134.060693196223)) ;
#148546=CARTESIAN_POINT('Ctrl Pts',(-14.2682168904107,14.1367619821381,
134.275000427421)) ;
#148547=CARTESIAN_POINT('Ctrl Pts',(-14.308672097508,13.868069374817,134.426223663583)) ;
#148548=CARTESIAN_POINT('Ctrl Pts',(-14.3242464980369,13.5652242868234,
134.505022827762)) ;
#148549=CARTESIAN_POINT('Ctrl Pts',(-14.3130481928678,13.2558696695954,
134.505203310138)) ;
#148550=CARTESIAN_POINT('Ctrl Pts',(-14.2751188260239,12.9557646560496,
134.427595170396)) ;
#148551=CARTESIAN_POINT('Ctrl Pts',(-14.2125011050347,12.6900042149153,
134.277767151928)) ;
#148552=CARTESIAN_POINT('Ctrl Pts',(-14.1287473937729,12.4761055498728,
134.066283383056)) ;
#148553=CARTESIAN_POINT('Ctrl Pts',(-14.0292043456581,12.3304586673531,
133.808672602781)) ;
#148554=CARTESIAN_POINT('Ctrl Pts',(-13.9209454355513,12.2634381617438,
133.525424392877)) ;
#148555=CARTESIAN_POINT('Ctrl Pts',(-13.8100698210139,12.278878358219,133.234640878502)) ;
#148556=CARTESIAN_POINT('Ctrl Pts',(-13.7038111973288,12.3768659810513,
132.957453506269)) ;
#148557=CARTESIAN_POINT('Ctrl Pts',(-13.6097056948675,12.5495630151977,
132.715665736416)) ;
#148558=CARTESIAN_POINT('Ctrl Pts',(-13.5332893897392,12.7855771404834,
132.525644949222)) ;
#148559=CARTESIAN_POINT('Ctrl Pts',(-13.4798638510241,13.0654345066809,
132.402557075124)) ;
#148560=CARTESIAN_POINT('Ctrl Pts',(-13.4517888390726,13.3720089206918,
132.353670494908)) ;
#148561=CARTESIAN_POINT('Ctrl Pts',(-13.4507696207002,13.682435682329,132.383838975626)) ;
#148562=CARTESIAN_POINT('Ctrl Pts',(-13.4759925925544,13.9739144742565,
132.490615522146)) ;
#148563=CARTESIAN_POINT('Ctrl Pts',(-13.5252998059987,14.2268633708939,
132.667901525746)) ;
#148564=CARTESIAN_POINT('Ctrl Pts',(-13.5934844266385,14.4204385553042,
132.900007436279)) ;
#148565=CARTESIAN_POINT('Ctrl Pts',(-13.6765840975396,14.5445800987763,
133.176129149791)) ;
#148566=CARTESIAN_POINT('Ctrl Pts',(-13.7660933005895,14.5868220518321,
133.470623338263)) ;
#148567=CARTESIAN_POINT('Ctrl Pts',(-13.8556826458728,14.5468039105965,
133.765349744584)) ;
#148568=CARTESIAN_POINT('Ctrl Pts',(-13.9389917331868,14.4251034051228,
134.042036110926)) ;
#148569=CARTESIAN_POINT('Ctrl Pts',(-14.0078406882011,14.2325286580178,
134.276201287599)) ;
#148570=CARTESIAN_POINT('Ctrl Pts',(-14.0575163353173,13.9823226151408,
134.454383889325)) ;
#148571=CARTESIAN_POINT('Ctrl Pts',(-14.0836025549971,13.6900857770298,
134.563868974634)) ;
#148572=CARTESIAN_POINT('Ctrl Pts',(-14.0832571069024,13.3811330160851,
134.595866332321)) ;
#148573=CARTESIAN_POINT('Ctrl Pts',(-14.0560489819167,13.0742212220075,
134.549500292957)) ;
#148574=CARTESIAN_POINT('Ctrl Pts',(-14.0030629387518,12.7922256015956,
134.427832814541)) ;
#148575=CARTESIAN_POINT('Ctrl Pts',(-13.9271733129843,12.5548594273492,
134.239343872288)) ;
#148576=CARTESIAN_POINT('Ctrl Pts',(-13.8333753451746,12.3804086470547,
133.99847615794)) ;
#148577=CARTESIAN_POINT('Ctrl Pts',(-13.7281102029634,12.2809059803651,
133.723956716157)) ;
#148578=CARTESIAN_POINT('Ctrl Pts',(-13.617241740478,12.2624888492441,133.433207556077)) ;
#148579=CARTESIAN_POINT('Ctrl Pts',(-13.5081833508386,12.3276777056696,
133.147817955966)) ;
#148580=CARTESIAN_POINT('Ctrl Pts',(-13.4087400939355,12.4707929028479,
132.890358316802)) ;
#148581=CARTESIAN_POINT('Ctrl Pts',(-13.3244896145502,12.6823314150819,
132.677374748484)) ;
#148582=CARTESIAN_POINT('Ctrl Pts',(-13.2609830005564,12.9478031848441,
132.525073234737)) ;
#148583=CARTESIAN_POINT('Ctrl Pts',(-13.2223270064774,13.2466923660168,
132.445278275813)) ;
#148584=CARTESIAN_POINT('Ctrl Pts',(-13.2103951472699,13.5583772827196,
132.44357445534)) ;
#148585=CARTESIAN_POINT('Ctrl Pts',(-13.2251602999981,13.8592556728242,
132.519724504582)) ;
#148586=CARTESIAN_POINT('Ctrl Pts',(-13.2651772105284,14.1306425332548,
132.669863094874)) ;
#148587=CARTESIAN_POINT('Ctrl Pts',(-13.3261568835758,14.3493759860233,
132.880945200703)) ;
#148588=CARTESIAN_POINT('Ctrl Pts',(-13.4039531667767,14.5035317541652,
133.141424580497)) ;
#148589=CARTESIAN_POINT('Ctrl Pts',(-13.4916134539024,14.5795845052791,
133.430615618163)) ;
#148590=CARTESIAN_POINT('Ctrl Pts',(-13.5823374167532,14.5729335586883,
133.72877440133)) ;
#148591=CARTESIAN_POINT('Ctrl Pts',(-13.6688628859832,14.4838964903463,
134.014660525185)) ;
#148592=CARTESIAN_POINT('Ctrl Pts',(-13.7443181729218,14.3187457579905,
134.268228770671)) ;
#148593=CARTESIAN_POINT('Ctrl Pts',(-13.8024060188236,14.0897675929633,
134.471006232896)) ;
#148594=CARTESIAN_POINT('Ctrl Pts',(-13.8384578759884,13.8134082777409,
134.609389817387)) ;
#148595=CARTESIAN_POINT('Ctrl Pts',(-13.8490872441391,13.5073936360873,
134.673692916445)) ;
#148596=CARTESIAN_POINT('Ctrl Pts',(-13.832792152632,13.1976577168155,134.659088373623)) ;
#148597=CARTESIAN_POINT('Ctrl Pts',(-13.7900624981885,12.9027229695694,
134.567399873167)) ;
#148598=CARTESIAN_POINT('Ctrl Pts',(-13.7229404114228,12.6448108497487,
134.404513164289)) ;
#148599=CARTESIAN_POINT('Ctrl Pts',(-13.6361336422572,12.4434495713625,
134.183973342917)) ;
#148600=CARTESIAN_POINT('Ctrl Pts',(-13.5339224602791,12.311375978469,133.918704188154)) ;
#148601=CARTESIAN_POINT('Ctrl Pts',(-13.4248925033934,12.2599503304442,
133.633135101603)) ;
#148602=CARTESIAN_POINT('Ctrl Pts',(-13.3140399354172,12.2913693228783,
133.342532189384)) ;
#148603=CARTESIAN_POINT('Ctrl Pts',(-13.2100079542354,12.4038516035479,
133.071692026905)) ;
#148604=CARTESIAN_POINT('Ctrl Pts',(-13.1188399743127,12.5892626487071,
132.838480990112)) ;
#148605=CARTESIAN_POINT('Ctrl Pts',(-13.0465008697508,12.8342966709516,
132.660260589203)) ;
#148606=CARTESIAN_POINT('Ctrl Pts',(-12.9973391164619,13.122430567382,132.549852233358)) ;
#148607=CARTESIAN_POINT('Ctrl Pts',(-12.9744365714638,13.4307504322514,
132.515998075404)) ;
#148608=CARTESIAN_POINT('Ctrl Pts',(-12.9784369626985,13.7394115392885,
132.560834284604)) ;
#148609=CARTESIAN_POINT('Ctrl Pts',(-13.0084496645794,14.0250582517609,
132.681620776933)) ;
#148610=CARTESIAN_POINT('Ctrl Pts',(-13.0615307919976,14.2676857548662,
132.869798935733)) ;
#148611=CARTESIAN_POINT('Ctrl Pts',(-13.1333688217039,14.4501343766899,
133.112842532531)) ;
#148612=CARTESIAN_POINT('Ctrl Pts',(-13.2177622418928,14.5585281665325,
133.392488045436)) ;
#148613=CARTESIAN_POINT('Ctrl Pts',(-13.3080577151419,14.5857500272389,
133.689369213566)) ;
#148614=CARTESIAN_POINT('Ctrl Pts',(-13.3972502622619,14.5296138269876,
133.983085307506)) ;
#148615=CARTESIAN_POINT('Ctrl Pts',(-13.4779778486236,14.3940563657681,
134.252050444746)) ;
#148616=CARTESIAN_POINT('Ctrl Pts',(-13.5436430073141,14.1896706330216,
134.476915598335)) ;
#148617=CARTESIAN_POINT('Ctrl Pts',(-13.5892678630379,13.9296795635546,
134.643358940888)) ;
#148618=CARTESIAN_POINT('Ctrl Pts',(-13.6104505119164,13.6325613783442,
134.738470798441)) ;
#148619=CARTESIAN_POINT('Ctrl Pts',(-13.6050981772493,13.3229079884786,
134.755797277682)) ;
#148620=CARTESIAN_POINT('Ctrl Pts',(-13.5728485012099,13.018526691074,134.694761651048)) ;
#148621=CARTESIAN_POINT('Ctrl Pts',(-13.5153450492774,12.7436673997071,
134.559879447056)) ;
#148622=CARTESIAN_POINT('Ctrl Pts',(-13.4354311899252,12.5164978954953,
134.359712961926)) ;
#148623=CARTESIAN_POINT('Ctrl Pts',(-13.3394512830422,12.3560840259889,
134.112282954591)) ;
#148624=CARTESIAN_POINT('Ctrl Pts',(-13.2320535007894,12.2708854791944,
133.831733816191)) ;
#148625=CARTESIAN_POINT('Ctrl Pts',(-13.1212646835022,12.2685612121641,
133.541141487823)) ;
#148626=CARTESIAN_POINT('Ctrl Pts',(-13.0135487693522,12.3486009748257,
133.259616351496)) ;
#148627=CARTESIAN_POINT('Ctrl Pts',(-12.9158794229883,12.5069430780995,
133.007592004978)) ;
#148628=CARTESIAN_POINT('Ctrl Pts',(-12.8358284635978,12.7284059514765,
132.806638042446)) ;
#148629=CARTESIAN_POINT('Ctrl Pts',(-12.7765201702019,13.0024845577893,
132.666692915585)) ;
#148630=CARTESIAN_POINT('Ctrl Pts',(-12.7429090658184,13.3053156304276,
132.601612497695)) ;
#148631=CARTESIAN_POINT('Ctrl Pts',(-12.7360481621408,13.6156286955051,
132.614589792664)) ;
#148632=CARTESIAN_POINT('Ctrl Pts',(-12.7556608206096,13.9128849931579,
132.70496583945)) ;
#148633=CARTESIAN_POINT('Ctrl Pts',(-12.8001013006508,14.1766185287715,
132.868078846721)) ;
#148634=CARTESIAN_POINT('Ctrl Pts',(-12.8649833652883,14.3847398624139,
133.090730630613)) ;
#148635=CARTESIAN_POINT('Ctrl Pts',(-12.9447362290285,14.5238361005913,
133.356717863807)) ;
#148636=CARTESIAN_POINT('Ctrl Pts',(-13.0335166994612,14.5847743012247,
133.649190179549)) ;
#148637=CARTESIAN_POINT('Ctrl Pts',(-13.1240492119926,14.5623309410939,
133.94680621714)) ;
#148638=CARTESIAN_POINT('Ctrl Pts',(-13.2090287290572,14.4584178167976,
134.228179442432)) ;
#148639=CARTESIAN_POINT('Ctrl Pts',(-13.281862210307,14.2791868777477,134.474211904493)) ;
#148640=CARTESIAN_POINT('Ctrl Pts',(-13.335773103936,14.0415187113142,134.664557550494)) ;
#148641=CARTESIAN_POINT('Ctrl Pts',(-13.3674362011174,13.7564325349983,
134.790345370979)) ;
#148642=CARTESIAN_POINT('Ctrl Pts',(-13.3729735926156,13.4495648560064,
134.839547729474)) ;
#148643=CARTESIAN_POINT('Ctrl Pts',(-13.3515432167407,13.1394167838631,
134.810135087209)) ;
#148644=CARTESIAN_POINT('Ctrl Pts',(-13.3040714645819,12.8508801265976,
134.704494636628)) ;
#148645=CARTESIAN_POINT('Ctrl Pts',(-13.2329202360563,12.6022770159485,
134.529809745286)) ;
#148646=CARTESIAN_POINT('Ctrl Pts',(-13.1427212865503,12.4127865779696,
134.299427661665)) ;
#148647=CARTESIAN_POINT('Ctrl Pts',(-13.0385956707939,12.2953916612225,
134.02852190621)) ;
#148648=CARTESIAN_POINT('Ctrl Pts',(-12.9286172414397,12.2594835082488,
133.740252210268)) ;
#148649=CARTESIAN_POINT('Ctrl Pts',(-12.8187965411872,12.3065006906036,
133.452548911367)) ;
#148650=CARTESIAN_POINT('Ctrl Pts',(-12.7166251696081,12.4331949897075,
133.187157237466)) ;
#148651=CARTESIAN_POINT('Ctrl Pts',(-12.6281176238896,12.6325251060339,
132.961927723459)) ;
#148652=CARTESIAN_POINT('Ctrl Pts',(-12.5603551331913,12.8854153923965,
132.796860075738)) ;
#148653=CARTESIAN_POINT('Ctrl Pts',(-12.5157669611184,13.1803566705807,
132.699944434962)) ;
#148654=CARTESIAN_POINT('Ctrl Pts',(-12.498052923534,13.4893561125358,132.681144837552)) ;
#148655=CARTESIAN_POINT('Ctrl Pts',(-12.5070166131313,13.7954470549273,
132.740482079854)) ;
#148656=CARTESIAN_POINT('Ctrl Pts',(-12.5417818886109,14.0751705086754,
132.875240680629)) ;
#148657=CARTESIAN_POINT('Ctrl Pts',(-12.5986620801991,14.3069080353192,
133.074438327252)) ;
#148658=CARTESIAN_POINT('Ctrl Pts',(-12.673160327911,14.4762412985565,133.325179922949)) ;
#148659=CARTESIAN_POINT('Ctrl Pts',(-12.7597351258917,14.5702449672957,
133.611399754379)) ;
#148660=CARTESIAN_POINT('Ctrl Pts',(-12.8500625826259,14.5813885693018,
133.908266863094)) ;
#148661=CARTESIAN_POINT('Ctrl Pts',(-12.9380952103393,14.5100796907114,
134.198552121671)) ;
#148662=CARTESIAN_POINT('Ctrl Pts',(-13.0166943404508,14.3602445312062,
134.461375238824)) ;
#148663=CARTESIAN_POINT('Ctrl Pts',(-13.079025585699,14.143253231573,134.676613684199)) ;
#148664=CARTESIAN_POINT('Ctrl Pts',(-13.1199829894282,13.8766590298569,
134.82919236409)) ;
#148665=CARTESIAN_POINT('Ctrl Pts',(-13.1363842764657,13.575471217549,134.910304171519)) ;
#148666=CARTESIAN_POINT('Ctrl Pts',(-13.1259906023331,13.2645668941717,
134.912996918485)) ;
#148667=CARTESIAN_POINT('Ctrl Pts',(-13.0886655812232,12.9634277851347,
134.837203216762)) ;
#148668=CARTESIAN_POINT('Ctrl Pts',(-13.0268727262915,12.6972349094739,
134.689690166995)) ;
#148669=CARTESIAN_POINT('Ctrl Pts',(-12.9437794235418,12.4817230619034,
134.480101250047)) ;
#148670=CARTESIAN_POINT('Ctrl Pts',(-12.8446953032213,12.3338051971936,
134.223812059553)) ;
#148671=CARTESIAN_POINT('Ctrl Pts',(-12.736264841077,12.2641456022445,133.940168303419)) ;
#148672=CARTESIAN_POINT('Ctrl Pts',(-12.6254315941907,12.2773535712523,
133.649486560175)) ;
#148673=CARTESIAN_POINT('Ctrl Pts',(-12.519180488884,12.3726334671979,133.372237189562)) ;
#148674=CARTESIAN_POINT('Ctrl Pts',(-12.424500141051,12.5434758401697,133.128817984578)) ;
#148675=CARTESIAN_POINT('Ctrl Pts',(-12.3476880051171,12.7769497642035,
132.937528466358)) ;
#148676=CARTESIAN_POINT('Ctrl Pts',(-12.2932283996367,13.0568799766939,
132.811568392158)) ;
#148677=CARTESIAN_POINT('Ctrl Pts',(-12.2644164115581,13.3636449455261,
132.760589242832)) ;
#148678=CARTESIAN_POINT('Ctrl Pts',(-12.2626515312786,13.6733774469028,
132.788485456325)) ;
#148679=CARTESIAN_POINT('Ctrl Pts',(-12.287057255896,13.9654380896254,132.892840457169)) ;
#148680=CARTESIAN_POINT('Ctrl Pts',(-12.3357556053458,14.220301269476,133.06839566665)) ;
#148681=CARTESIAN_POINT('Ctrl Pts',(-12.4036363026361,14.415947045335,133.299682560496)) ;
#148682=CARTESIAN_POINT('Ctrl Pts',(-12.4858983405842,14.5416943673476,
133.573153971909)) ;
#148683=CARTESIAN_POINT('Ctrl Pts',(-12.5756511466147,14.586901890039,133.868497858328)) ;
#148684=CARTESIAN_POINT('Ctrl Pts',(-12.6654696558363,14.5489491303822,
134.163944585503)) ;
#148685=CARTESIAN_POINT('Ctrl Pts',(-12.7488004609279,14.4300240451422,
134.44057679707)) ;
#148686=CARTESIAN_POINT('Ctrl Pts',(-12.8184183179855,14.2387296185005,
134.677112327015)) ;
#148687=CARTESIAN_POINT('Ctrl Pts',(-12.8686018078536,13.9899469010905,
134.856754873464)) ;
#148688=CARTESIAN_POINT('Ctrl Pts',(-12.8953390018291,13.7002922366985,
134.967959281547)) ;
#148689=CARTESIAN_POINT('Ctrl Pts',(-12.8959448004099,13.3909003145637,
135.00281288959)) ;
#148690=CARTESIAN_POINT('Ctrl Pts',(-12.8693187261974,13.0819914408663,
134.95831995508)) ;
#148691=CARTESIAN_POINT('Ctrl Pts',(-12.8171517429198,12.8000707339927,
134.838929642487)) ;
#148692=CARTESIAN_POINT('Ctrl Pts',(-12.7421374292196,12.5616134870626,
134.652909850917)) ;
#148693=CARTESIAN_POINT('Ctrl Pts',(-12.6486214543391,12.384449895012,134.412941328436)) ;
#148694=CARTESIAN_POINT('Ctrl Pts',(-12.5430733333332,12.2824628240901,
134.137754600261)) ;
#148695=CARTESIAN_POINT('Ctrl Pts',(-12.4328336844289,12.2618989594336,
133.848666595403)) ;
#148696=CARTESIAN_POINT('Ctrl Pts',(-12.3234764644886,12.3245801439636,
133.562445071246)) ;
#148697=CARTESIAN_POINT('Ctrl Pts',(-12.2236702142189,12.4655889841413,
133.303925046023)) ;
#148698=CARTESIAN_POINT('Ctrl Pts',(-12.1389072399167,12.6753258327154,
133.089442344447)) ;
#148699=CARTESIAN_POINT('Ctrl Pts',(-12.0747933877151,12.9389695306945,
132.935307440174)) ;
#148700=CARTESIAN_POINT('Ctrl Pts',(-12.0353186182838,13.2377441429055,
132.853189559189)) ;
#148701=CARTESIAN_POINT('Ctrl Pts',(-12.0225559627654,13.5478077720715,
132.848886973666)) ;
#148702=CARTESIAN_POINT('Ctrl Pts',(-12.0366139208027,13.8515135114459,
132.923217350704)) ;
#148703=CARTESIAN_POINT('Ctrl Pts',(-12.0758678831878,14.1231097110526,
133.07101037297)) ;
#148704=CARTESIAN_POINT('Ctrl Pts',(-12.1363738971983,14.3439546593352,
133.280769121662)) ;
#148705=CARTESIAN_POINT('Ctrl Pts',(-12.2135714078888,14.4998916999394,
133.539410393626)) ;
#148706=CARTESIAN_POINT('Ctrl Pts',(-12.3013318130591,14.5786386436238,
133.82901150719)) ;
#148707=CARTESIAN_POINT('Ctrl Pts',(-12.3920181749816,14.5742675055765,
134.127037321131)) ;
#148708=CARTESIAN_POINT('Ctrl Pts',(-12.4788244044002,14.4873447057953,
134.413774862475)) ;
#148709=CARTESIAN_POINT('Ctrl Pts',(-12.5544418663992,14.324791387065,134.667707059656)) ;
#148710=CARTESIAN_POINT('Ctrl Pts',(-12.6133095637089,14.0970302215938,
134.872846143443)) ;
#148711=CARTESIAN_POINT('Ctrl Pts',(-12.6500777852611,13.8204923791666,
135.013454137909)) ;
#148712=CARTESIAN_POINT('Ctrl Pts',(-12.6613488618547,13.5164549549645,
135.07946573627)) ;
#148713=CARTESIAN_POINT('Ctrl Pts',(-12.6458306906024,13.2060699844781,
135.067187910305)) ;
#148714=CARTESIAN_POINT('Ctrl Pts',(-12.6037641136263,12.9102232608784,
134.977454778982)) ;
#148715=CARTESIAN_POINT('Ctrl Pts',(-12.5371192356222,12.6507291621381,
134.816011366745)) ;
#148716=CARTESIAN_POINT('Ctrl Pts',(-12.4510895491266,12.4485585677655,
134.597616648301)) ;
#148717=CARTESIAN_POINT('Ctrl Pts',(-12.349770741895,12.3145373825205,134.334792426212)) ;
#148718=CARTESIAN_POINT('Ctrl Pts',(-12.2402433163891,12.2601564012495,
134.047965097519)) ;
#148719=CARTESIAN_POINT('Ctrl Pts',(-12.1293526644653,12.2893926145907,
133.757240402094)) ;
#148720=CARTESIAN_POINT('Ctrl Pts',(-12.0250639181401,12.3994366582283,
133.485636610226)) ;
#148721=CARTESIAN_POINT('Ctrl Pts',(-11.9330778249773,12.5839727611718,
133.250184991413)) ;
#148722=CARTESIAN_POINT('Ctrl Pts',(-11.8605383338059,12.8264919442356,
133.071221263827)) ;
#148723=CARTESIAN_POINT('Ctrl Pts',(-11.8105329668041,13.1141227557289,
132.958401040611)) ;
#148724=CARTESIAN_POINT('Ctrl Pts',(-11.7948211693083,13.3194869799383,
132.934542691027)) ;
#148725=CARTESIAN_POINT('Ctrl Pts',(-11.7914080085508,13.4222384087837,
132.935592717388)) ;
#148726=CARTESIAN_POINT('Ctrl Pts',(-33.372552283912,13.1368456608817,127.94074177726)) ;
#148727=CARTESIAN_POINT('Ctrl Pts',(-33.3717780316138,13.1302434100695,
127.939210950719)) ;
#148728=CARTESIAN_POINT('Ctrl Pts',(-33.3591440063766,13.0249711622575,
127.91398623386)) ;
#148729=CARTESIAN_POINT('Ctrl Pts',(-33.3246270598641,12.8263018173041,
127.836128436635)) ;
#148730=CARTESIAN_POINT('Ctrl Pts',(-33.2518258931156,12.5833995397257,
127.656480341887)) ;
#148731=CARTESIAN_POINT('Ctrl Pts',(-33.1602821282434,12.3996267675037,
127.42216387292)) ;
#148732=CARTESIAN_POINT('Ctrl Pts',(-33.0552813371174,12.2890731746127,
127.148703526175)) ;
#148733=CARTESIAN_POINT('Ctrl Pts',(-32.9453207624895,12.2602312933653,
126.860410133392)) ;
#148734=CARTESIAN_POINT('Ctrl Pts',(-32.8354844413288,12.3144254327404,
126.5727765393)) ;
#148735=CARTESIAN_POINT('Ctrl Pts',(-32.7343044732474,12.4480642485612,
126.310296325994)) ;
#148736=CARTESIAN_POINT('Ctrl Pts',(-32.647713423827,12.6516399128533,126.090485649053)) ;
#148737=CARTESIAN_POINT('Ctrl Pts',(-32.5814045317866,12.9104451953934,
125.929904053096)) ;
#148738=CARTESIAN_POINT('Ctrl Pts',(-32.539361864737,13.2058491339696,125.840200965284)) ;
#148739=CARTESIAN_POINT('Ctrl Pts',(-32.5237679482684,13.5166184158111,
125.827737740167)) ;
#148740=CARTESIAN_POINT('Ctrl Pts',(-32.5352548048312,13.822409942281,125.89458343385)) ;
#148741=CARTESIAN_POINT('Ctrl Pts',(-32.5718813221576,14.0967864271645,
126.034540409285)) ;
#148742=CARTESIAN_POINT('Ctrl Pts',(-32.6305856565637,14.3244562376795,
126.239159768777)) ;
#148743=CARTESIAN_POINT('Ctrl Pts',(-32.7063816647152,14.4874741588536,
126.493693734194)) ;
#148744=CARTESIAN_POINT('Ctrl Pts',(-32.7933567848837,14.5744204782189,
126.78098226786)) ;
#148745=CARTESIAN_POINT('Ctrl Pts',(-32.8840723683445,14.5784621865543,
127.079105132271)) ;
#148746=CARTESIAN_POINT('Ctrl Pts',(-32.9714000447983,14.5000470189108,
127.367281428271)) ;
#148747=CARTESIAN_POINT('Ctrl Pts',(-33.0485978146599,14.3445727913024,
127.625899065993)) ;
#148748=CARTESIAN_POINT('Ctrl Pts',(-33.1094227295156,14.1228339214572,
127.836735242549)) ;
#148749=CARTESIAN_POINT('Ctrl Pts',(-33.1486346997481,13.850151796375,127.9845077735)) ;
#148750=CARTESIAN_POINT('Ctrl Pts',(-33.1625834468356,13.5490424798657,
128.058234479633)) ;
#148751=CARTESIAN_POINT('Ctrl Pts',(-33.1498770654012,13.2374718016147,
128.054257906591)) ;
#148752=CARTESIAN_POINT('Ctrl Pts',(-33.110281108,12.9386845516003,127.971796151102)) ;
#148753=CARTESIAN_POINT('Ctrl Pts',(-33.0464969729853,12.6761377912153,
127.818477928809)) ;
#148754=CARTESIAN_POINT('Ctrl Pts',(-32.9616310346417,12.4657587239521,
127.603760965913)) ;
#148755=CARTESIAN_POINT('Ctrl Pts',(-32.8617323746109,12.3246285907277,
127.344999609685)) ;
#148756=CARTESIAN_POINT('Ctrl Pts',(-32.7524169820034,12.2619062274696,
127.058889535839)) ;
#148757=CARTESIAN_POINT('Ctrl Pts',(-32.6419963192406,12.2824388238971,
126.769324981895)) ;
#148758=CARTESIAN_POINT('Ctrl Pts',(-32.5362628789588,12.3848777352211,
126.493663129602)) ;
#148759=CARTESIAN_POINT('Ctrl Pts',(-32.4431445614343,12.5614991526439,
126.254730121884)) ;
#148760=CARTESIAN_POINT('Ctrl Pts',(-32.3680539595633,12.7995867932639,
126.068470241934)) ;
#148761=CARTESIAN_POINT('Ctrl Pts',(-32.3155888176679,13.0840299785093,
125.948484575688)) ;
#148762=CARTESIAN_POINT('Ctrl Pts',(-32.2893312633254,13.3899587126068,
125.904739149321)) ;
#148763=CARTESIAN_POINT('Ctrl Pts',(-32.2897584792436,13.6996411315525,
125.939101557284)) ;
#148764=CARTESIAN_POINT('Ctrl Pts',(-32.3165996493069,13.9903747332587,
126.050727800221)) ;
#148765=CARTESIAN_POINT('Ctrl Pts',(-32.3669241137826,14.2393240400609,
126.230826853994)) ;
#148766=CARTESIAN_POINT('Ctrl Pts',(-32.4363513245266,14.4298400308443,
126.46669969067)) ;
#148767=CARTESIAN_POINT('Ctrl Pts',(-32.519430880019,14.5487685214643,126.742513227334)) ;
#148768=CARTESIAN_POINT('Ctrl Pts',(-32.6096330962241,14.5869290459119,
127.039223094392)) ;
#148769=CARTESIAN_POINT('Ctrl Pts',(-32.6990799621577,14.5417666883846,
127.333562773258)) ;
#148770=CARTESIAN_POINT('Ctrl Pts',(-32.7814232479936,14.4163781247343,
127.607278938856)) ;
#148771=CARTESIAN_POINT('Ctrl Pts',(-32.8496169733658,14.2194053349132,
127.839665758422)) ;
#148772=CARTESIAN_POINT('Ctrl Pts',(-32.8979064624203,13.9666437223108,
128.013748817654)) ;
#148773=CARTESIAN_POINT('Ctrl Pts',(-32.9225596490422,13.6737230615468,
128.118947651821)) ;
#148774=CARTESIAN_POINT('Ctrl Pts',(-32.9207144430641,13.3629183562335,
128.146716806087)) ;
#148775=CARTESIAN_POINT('Ctrl Pts',(-32.8919279335873,13.0570541926124,
128.095721621593)) ;
#148776=CARTESIAN_POINT('Ctrl Pts',(-32.8376033356132,12.7772474882028,
127.970123458047)) ;
#148777=CARTESIAN_POINT('Ctrl Pts',(-32.7603558327083,12.5427680986525,
127.777727930602)) ;
#148778=CARTESIAN_POINT('Ctrl Pts',(-32.6662279784257,12.3730788782687,
127.53571899559)) ;
#148779=CARTESIAN_POINT('Ctrl Pts',(-32.5599217010986,12.2773830666973,
127.258340083159)) ;
#148780=CARTESIAN_POINT('Ctrl Pts',(-32.4489850033344,12.2641121652248,
126.967384354349)) ;
#148781=CARTESIAN_POINT('Ctrl Pts',(-32.3405436242218,12.3337583003129,
126.683712432675)) ;
#148782=CARTESIAN_POINT('Ctrl Pts',(-32.2416220298584,12.481316017211,126.42783978584)) ;
#148783=CARTESIAN_POINT('Ctrl Pts',(-32.1584105156519,12.6966779051232,
126.217918468821)) ;
#148784=CARTESIAN_POINT('Ctrl Pts',(-32.0964113311334,12.96405838434,126.069941333546)) ;
#148785=CARTESIAN_POINT('Ctrl Pts',(-32.0592942459553,13.2633620040759,
125.994551630201)) ;
#148786=CARTESIAN_POINT('Ctrl Pts',(-32.0487513263688,13.5752566966047,
125.996917495549)) ;
#148787=CARTESIAN_POINT('Ctrl Pts',(-32.0651787613996,13.8766501658651,
126.078125527416)) ;
#148788=CARTESIAN_POINT('Ctrl Pts',(-32.106237139948,14.1438625345399,126.231076917147)) ;
#148789=CARTESIAN_POINT('Ctrl Pts',(-32.1688151496798,14.3611557729943,
126.447120106865)) ;
#148790=CARTESIAN_POINT('Ctrl Pts',(-32.2472987630035,14.5102070639316,
126.709529597132)) ;
#148791=CARTESIAN_POINT('Ctrl Pts',(-32.3349170372181,14.5813677790431,
126.99845205783)) ;
#148792=CARTESIAN_POINT('Ctrl Pts',(-32.4257587129059,14.5701315167375,
127.297011355326)) ;
#148793=CARTESIAN_POINT('Ctrl Pts',(-32.5121114944259,14.4759919392145,
127.582506664814)) ;
#148794=CARTESIAN_POINT('Ctrl Pts',(-32.586577018117,14.3066893243029,127.833144617972)) ;
#148795=CARTESIAN_POINT('Ctrl Pts',(-32.6433606397653,14.075187939402,128.032015916789)) ;
#148796=CARTESIAN_POINT('Ctrl Pts',(-32.6780690407698,13.7962287438528,
128.166528915326)) ;
#148797=CARTESIAN_POINT('Ctrl Pts',(-32.6872064373839,13.4897393556908,
128.226418122972)) ;
#148798=CARTESIAN_POINT('Ctrl Pts',(-32.6691192160608,13.1781057377786,
128.206822501505)) ;
#148799=CARTESIAN_POINT('Ctrl Pts',(-32.6251388666684,12.8871395007703,
128.11122499469)) ;
#148800=CARTESIAN_POINT('Ctrl Pts',(-32.5567420099813,12.6313543298591,
127.944663176923)) ;
#148801=CARTESIAN_POINT('Ctrl Pts',(-32.468480326082,12.4333423964865,127.720004921838)) ;
#148802=CARTESIAN_POINT('Ctrl Pts',(-32.3667523701111,12.3067788295905,
127.45578803769)) ;
#148803=CARTESIAN_POINT('Ctrl Pts',(-32.2563735289916,12.2592790110699,
127.166620834658)) ;
#148804=CARTESIAN_POINT('Ctrl Pts',(-32.1460193447871,12.2958890741667,
126.877373493955)) ;
#148805=CARTESIAN_POINT('Ctrl Pts',(-32.0427219858457,12.412515964046,126.608629772059)) ;
#148806=CARTESIAN_POINT('Ctrl Pts',(-31.9523858329491,12.6017795231482,
126.377868646038)) ;
#148807=CARTESIAN_POINT('Ctrl Pts',(-31.8811024103402,12.8508820416093,
126.20286039856)) ;
#148808=CARTESIAN_POINT('Ctrl Pts',(-31.8336722130978,13.1389626246921,
126.097293690777)) ;
#148809=CARTESIAN_POINT('Ctrl Pts',(-31.8121351013455,13.4502019068506,
126.067683040548)) ;
#148810=CARTESIAN_POINT('Ctrl Pts',(-31.8178503511759,13.7571545047615,
126.117429724884)) ;
#148811=CARTESIAN_POINT('Ctrl Pts',(-31.8491017041277,14.0399279502617,
126.241716326633)) ;
#148812=CARTESIAN_POINT('Ctrl Pts',(-31.9036445538269,14.2804627240583,
126.43430783686)) ;
#148813=CARTESIAN_POINT('Ctrl Pts',(-31.976030827149,14.4580430249791,126.678783103797)) ;
#148814=CARTESIAN_POINT('Ctrl Pts',(-32.0610740513668,14.5623041717052,
126.960389503841)) ;
#148815=CARTESIAN_POINT('Ctrl Pts',(-32.1514066726644,14.5848738329504,
127.257341934247)) ;
#148816=CARTESIAN_POINT('Ctrl Pts',(-32.2406996744394,14.5236285487513,
127.551504825239)) ;
#148817=CARTESIAN_POINT('Ctrl Pts',(-32.3203563629849,14.3842859128116,
127.81718848941)) ;
#148818=CARTESIAN_POINT('Ctrl Pts',(-32.3852114437279,14.1760037258481,
128.039769410632)) ;
#148819=CARTESIAN_POINT('Ctrl Pts',(-32.4295530229322,13.9123646323485,
128.202565138207)) ;
#148820=CARTESIAN_POINT('Ctrl Pts',(-32.4491140406027,13.6155080091082,
128.292745839514)) ;
#148821=CARTESIAN_POINT('Ctrl Pts',(-32.442267685353,13.3048787604148,128.305795361212)) ;
#148822=CARTESIAN_POINT('Ctrl Pts',(-32.4084189396864,13.0013159560589,
128.240117209961)) ;
#148823=CARTESIAN_POINT('Ctrl Pts',(-32.3495230158094,12.7290185702227,
128.101151404377)) ;
#148824=CARTESIAN_POINT('Ctrl Pts',(-32.2688647109356,12.5059453720444,
127.898672028067)) ;
#148825=CARTESIAN_POINT('Ctrl Pts',(-32.171709171051,12.348935712054,127.647947097826)) ;
#148826=CARTESIAN_POINT('Ctrl Pts',(-32.0642724896307,12.2685725815048,
127.367166374823)) ;
#148827=CARTESIAN_POINT('Ctrl Pts',(-31.9528808938988,12.2709800121234,
127.074994579475)) ;
#148828=CARTESIAN_POINT('Ctrl Pts',(-31.8458710839946,12.3558596886437,
126.795453239474)) ;
#148829=CARTESIAN_POINT('Ctrl Pts',(-31.7493426472634,12.5173148322773,
126.546620338384)) ;
#148830=CARTESIAN_POINT('Ctrl Pts',(-31.669870845794,12.7436532410187,126.347587050169)) ;
#148831=CARTESIAN_POINT('Ctrl Pts',(-31.6123394354576,13.0184389835147,
126.212627252227)) ;
#148832=CARTESIAN_POINT('Ctrl Pts',(-31.5800749292973,13.3224258162056,
126.151504283828)) ;
#148833=CARTESIAN_POINT('Ctrl Pts',(-31.5747290724803,13.6337495707095,
126.169029469326)) ;
#148834=CARTESIAN_POINT('Ctrl Pts',(-31.5959652324382,13.9298381021214,
126.264195066353)) ;
#148835=CARTESIAN_POINT('Ctrl Pts',(-31.6414442989228,14.1894305566765,
126.430148429791)) ;
#148836=CARTESIAN_POINT('Ctrl Pts',(-31.7073577282004,14.394475711673,126.655854752782)) ;
#148837=CARTESIAN_POINT('Ctrl Pts',(-31.787889015417,14.5294751286176,126.924154341006)) ;
#148838=CARTESIAN_POINT('Ctrl Pts',(-31.8769652278811,14.5857784674847,
127.217493619742)) ;
#148839=CARTESIAN_POINT('Ctrl Pts',(-31.967547767219,14.5584758053027,127.515317123615)) ;
#148840=CARTESIAN_POINT('Ctrl Pts',(-32.0518753014039,14.4499269628754,
127.794753752466)) ;
#148841=CARTESIAN_POINT('Ctrl Pts',(-32.1235837510951,14.2678362538152,
128.037358324424)) ;
#148842=CARTESIAN_POINT('Ctrl Pts',(-32.1767041734191,14.025181469635,128.225662324627)) ;
#148843=CARTESIAN_POINT('Ctrl Pts',(-32.2067108970508,13.7395989406437,
128.346424348598)) ;
#148844=CARTESIAN_POINT('Ctrl Pts',(-32.2107486585136,13.4312396287892,
128.391339089257)) ;
#148845=CARTESIAN_POINT('Ctrl Pts',(-32.187850141749,13.1225497292761,128.357535369758)) ;
#148846=CARTESIAN_POINT('Ctrl Pts',(-32.1387034319013,12.8344723647331,
128.247162948321)) ;
#148847=CARTESIAN_POINT('Ctrl Pts',(-32.0663825406077,12.5894057804916,
128.068995833289)) ;
#148848=CARTESIAN_POINT('Ctrl Pts',(-31.9751968195314,12.40386696018,127.835743163197)) ;
#148849=CARTESIAN_POINT('Ctrl Pts',(-31.8710345103169,12.2913271454925,
127.564562587712)) ;
#148850=CARTESIAN_POINT('Ctrl Pts',(-31.7602866795664,12.2598830910962,
127.274231377558)) ;
#148851=CARTESIAN_POINT('Ctrl Pts',(-31.650876260428,12.3117248665292,126.987672720107)) ;
#148852=CARTESIAN_POINT('Ctrl Pts',(-31.5491888340202,12.4432581620118,
126.723765797051)) ;
#148853=CARTESIAN_POINT('Ctrl Pts',(-31.4622339713139,12.6447767866554,
126.502841897175)) ;
#148854=CARTESIAN_POINT('Ctrl Pts',(-31.3952636966444,12.9020426127521,
126.340316351523)) ;
#148855=CARTESIAN_POINT('Ctrl Pts',(-31.3524307764882,13.1969219794908,
126.248333436724)) ;
#148856=CARTESIAN_POINT('Ctrl Pts',(-31.3360597331942,13.5073632860462,
126.233579460567)) ;
#148857=CARTESIAN_POINT('Ctrl Pts',(-31.3467467970684,13.813502723387,126.298071632455)) ;
#148858=CARTESIAN_POINT('Ctrl Pts',(-31.3826080772341,14.089063380816,126.435785315651)) ;
#148859=CARTESIAN_POINT('Ctrl Pts',(-31.4410196431954,14.319268429037,126.639693220211)) ;
#148860=CARTESIAN_POINT('Ctrl Pts',(-31.5161372632697,14.4835637196257,
126.892114231068)) ;
#148861=CARTESIAN_POINT('Ctrl Pts',(-31.6028715211698,14.5730187968723,
127.178702983459)) ;
#148862=CARTESIAN_POINT('Ctrl Pts',(-31.6935959532657,14.5795967994517,
127.47685559871)) ;
#148863=CARTESIAN_POINT('Ctrl Pts',(-31.7812976545653,14.5032854437543,
127.766198609052)) ;
#148864=CARTESIAN_POINT('Ctrl Pts',(-31.8588077042813,14.350115255618,128.025685725528)) ;
#148865=CARTESIAN_POINT('Ctrl Pts',(-31.9203271776916,14.1289953523701,
128.238682003332)) ;
#148866=CARTESIAN_POINT('Ctrl Pts',(-31.9599005577063,13.8600885343661,
128.38719829855)) ;
#148867=CARTESIAN_POINT('Ctrl Pts',(-31.9748262172758,13.5571077993043,
128.464060699988)) ;
#148868=CARTESIAN_POINT('Ctrl Pts',(-31.962757597202,13.2461442417419,128.46187610043)) ;
#148869=CARTESIAN_POINT('Ctrl Pts',(-31.9241515733642,12.9474785821981,
128.382201956869)) ;
#148870=CARTESIAN_POINT('Ctrl Pts',(-31.8604665395994,12.6818051231589,
128.229429013214)) ;
#148871=CARTESIAN_POINT('Ctrl Pts',(-31.7767215134204,12.4713262557242,
128.017732941446)) ;
#148872=CARTESIAN_POINT('Ctrl Pts',(-31.6766990193786,12.3273775591191,
127.758780001682)) ;
#148873=CARTESIAN_POINT('Ctrl Pts',(-31.5681563819875,12.2625380497534,
127.474731473525)) ;
#148874=CARTESIAN_POINT('Ctrl Pts',(-31.456705348187,12.2810707437097,127.182462188082)) ;
#148875=CARTESIAN_POINT('Ctrl Pts',(-31.3518550564754,12.3803128917833,
126.909020385735)) ;
#148876=CARTESIAN_POINT('Ctrl Pts',(-31.257702619694,12.5556238817755,126.66726187908)) ;
#148877=CARTESIAN_POINT('Ctrl Pts',(-31.1822947771,12.7914916788268,126.479962924463)) ;
#148878=CARTESIAN_POINT('Ctrl Pts',(-31.128989212263,13.075040960321,126.357555646944)) ;
#148879=CARTESIAN_POINT('Ctrl Pts',(-31.1019281701604,13.3808908357546,
126.311493897852)) ;
#148880=CARTESIAN_POINT('Ctrl Pts',(-31.101598677276,13.6908804801079,126.343656174616)) ;
#148881=CARTESIAN_POINT('Ctrl Pts',(-31.1276137979724,13.9819858711707,
126.452802987788)) ;
#148882=CARTESIAN_POINT('Ctrl Pts',(-31.1774498129048,14.2331023132834,
126.631574159292)) ;
#148883=CARTESIAN_POINT('Ctrl Pts',(-31.2463221547252,14.4253737396298,
126.865787908676)) ;
#148884=CARTESIAN_POINT('Ctrl Pts',(-31.3296291551697,14.54690254864,127.142464376561)) ;
#148885=CARTESIAN_POINT('Ctrl Pts',(-31.4191291908472,14.5868798000434,
127.43689176411)) ;
#148886=CARTESIAN_POINT('Ctrl Pts',(-31.5088033883795,14.5442430109602,
127.731941184325)) ;
#148887=CARTESIAN_POINT('Ctrl Pts',(-31.5913579378226,14.4211466700167,
128.006234530102)) ;
#148888=CARTESIAN_POINT('Ctrl Pts',(-31.6600527357246,14.2262607777735,
128.24007434236)) ;
#148889=CARTESIAN_POINT('Ctrl Pts',(-31.7090806186089,13.9744157685803,
128.41637832251)) ;
#148890=CARTESIAN_POINT('Ctrl Pts',(-31.7343968963979,13.6824770382547,
128.523494114923)) ;
#148891=CARTESIAN_POINT('Ctrl Pts',(-31.733427314249,13.3726811668738,128.553735367064)) ;
#148892=CARTESIAN_POINT('Ctrl Pts',(-31.7051969519129,13.06445534207,128.504576440852)) ;
#148893=CARTESIAN_POINT('Ctrl Pts',(-31.6517486616812,12.7851438246932,
128.381371124061)) ;
#148894=CARTESIAN_POINT('Ctrl Pts',(-31.5753581104184,12.5493640778092,
128.191406816883)) ;
#148895=CARTESIAN_POINT('Ctrl Pts',(-31.4814357009972,12.3769707838731,
127.950088842735)) ;
#148896=CARTESIAN_POINT('Ctrl Pts',(-31.3750785325616,12.2789143225366,
127.672647100852)) ;
#148897=CARTESIAN_POINT('Ctrl Pts',(-31.2645011786584,12.2633331212568,
127.382644142174)) ;
#148898=CARTESIAN_POINT('Ctrl Pts',(-31.1556392002351,12.3306602276622,
127.097816362084)) ;
#148899=CARTESIAN_POINT('Ctrl Pts',(-31.0562518667152,12.4766202323596,
126.840633530145)) ;
#148900=CARTESIAN_POINT('Ctrl Pts',(-30.972938158,12.6891735601127,126.630245983775)) ;
#148901=CARTESIAN_POINT('Ctrl Pts',(-30.9101457934406,12.9552554154068,
126.479968848149)) ;
#148902=CARTESIAN_POINT('Ctrl Pts',(-30.8721764023773,13.2547269193452,
126.402177144233)) ;
#148903=CARTESIAN_POINT('Ctrl Pts',(-30.8609235836592,13.5662745338838,
126.402436753715)) ;
#148904=CARTESIAN_POINT('Ctrl Pts',(-30.8764476985309,13.8673045434185,
126.480887327569)) ;
#148905=CARTESIAN_POINT('Ctrl Pts',(-30.9169530211909,14.1368395947381,
126.632353008074)) ;
#148906=CARTESIAN_POINT('Ctrl Pts',(-30.9787492522739,14.355047357882,126.845986583721)) ;
#148907=CARTESIAN_POINT('Ctrl Pts',(-31.0567851807192,14.5066809215218,
127.107093173731)) ;
#148908=CARTESIAN_POINT('Ctrl Pts',(-31.1446588781563,14.5805549818753,
127.396924345416)) ;
#148909=CARTESIAN_POINT('Ctrl Pts',(-31.2352728616708,14.5715434476004,
127.69472820504)) ;
#148910=CARTESIAN_POINT('Ctrl Pts',(-31.3215614046395,14.4804615024267,
127.979908754942)) ;
#148911=CARTESIAN_POINT('Ctrl Pts',(-31.3967763756955,14.3129345410317,
128.232850337699)) ;
#148912=CARTESIAN_POINT('Ctrl Pts',(-31.4542633909924,14.0824720621631,
128.433850809568)) ;
#148913=CARTESIAN_POINT('Ctrl Pts',(-31.489623472081,13.8045960831527,128.570261385745)) ;
#148914=CARTESIAN_POINT('Ctrl Pts',(-31.4995214449114,13.4994873044745,
128.632276592149)) ;
#148915=CARTESIAN_POINT('Ctrl Pts',(-31.4823318161701,13.1877259359498,
128.615295704579)) ;
#148916=CARTESIAN_POINT('Ctrl Pts',(-31.4389383199175,12.8947282234829,
128.521543366635)) ;
#148917=CARTESIAN_POINT('Ctrl Pts',(-31.3710227559662,12.6375710763399,
128.35641831796)) ;
#148918=CARTESIAN_POINT('Ctrl Pts',(-31.2837896130209,12.438646888205,128.134577930559)) ;
#148919=CARTESIAN_POINT('Ctrl Pts',(-31.1818199730732,12.3091461051662,
127.869843437161)) ;
#148920=CARTESIAN_POINT('Ctrl Pts',(-31.0721930263466,12.2596124817515,
127.582678546268)) ;
#148921=CARTESIAN_POINT('Ctrl Pts',(-30.9614915352443,12.2934287573512,
127.292491909052)) ;
#148922=CARTESIAN_POINT('Ctrl Pts',(-30.8574567264293,12.4085128318244,
127.021738717277)) ;
#148923=CARTESIAN_POINT('Ctrl Pts',(-30.7669612991102,12.5956557318582,
126.790429502215)) ;
#148924=CARTESIAN_POINT('Ctrl Pts',(-30.6952746289736,12.8419007286425,
126.614087904973)) ;
#148925=CARTESIAN_POINT('Ctrl Pts',(-30.646823062796,13.131017500255,126.505762609354)) ;
#148926=CARTESIAN_POINT('Ctrl Pts',(-30.6246568272436,13.4394174344068,
126.47403583793)) ;
#148927=CARTESIAN_POINT('Ctrl Pts',(-30.6294887388324,13.7489280786131,
126.521433227491)) ;
#148928=CARTESIAN_POINT('Ctrl Pts',(-30.6601827171697,14.0326636171821,
126.644108290625)) ;
#148929=CARTESIAN_POINT('Ctrl Pts',(-30.7138555910178,14.2739040584896,
126.834025044744)) ;
#148930=CARTESIAN_POINT('Ctrl Pts',(-30.7861586740712,14.4542738931404,
127.078423495766)) ;
#148931=CARTESIAN_POINT('Ctrl Pts',(-30.8705668756073,14.5602989567159,
127.358020430857)) ;
#148932=CARTESIAN_POINT('Ctrl Pts',(-30.9611627968773,14.5853165181453,
127.655868520581)) ;
#148933=CARTESIAN_POINT('Ctrl Pts',(-31.050038446453,14.5269567294315,127.948592774541)) ;
#148934=CARTESIAN_POINT('Ctrl Pts',(-31.1306389772583,14.3891798235028,
128.217257244013)) ;
#148935=CARTESIAN_POINT('Ctrl Pts',(-31.1959979491023,14.1817903606507,
128.44137499461)) ;
#148936=CARTESIAN_POINT('Ctrl Pts',(-31.2406347364941,13.9219442821041,
128.60472994041)) ;
#148937=CARTESIAN_POINT('Ctrl Pts',(-31.2611632325786,13.6244334028394,
128.697907886607)) ;
#148938=CARTESIAN_POINT('Ctrl Pts',(-31.2550704721298,13.313830933939,128.713157746917)) ;
#148939=CARTESIAN_POINT('Ctrl Pts',(-31.2218492806563,13.0089908308966,
128.649399781927)) ;
#148940=CARTESIAN_POINT('Ctrl Pts',(-31.1638471119269,12.7367006174924,
128.512907453242)) ;
#148941=CARTESIAN_POINT('Ctrl Pts',(-31.0837932668277,12.511790352846,128.312199836649)) ;
#148942=CARTESIAN_POINT('Ctrl Pts',(-30.9870335192191,12.3525056557872,
128.062637893671)) ;
#148943=CARTESIAN_POINT('Ctrl Pts',(-30.8793393489368,12.2695603711095,
127.781244876956)) ;
#148944=CARTESIAN_POINT('Ctrl Pts',(-30.7681133580193,12.2698997293224,
127.489506388524)) ;
#148945=CARTESIAN_POINT('Ctrl Pts',(-30.6611822400165,12.3521639545542,
127.21010491514)) ;
#148946=CARTESIAN_POINT('Ctrl Pts',(-30.5641504847242,12.5116414320552,
126.959834218351)) ;
#148947=CARTESIAN_POINT('Ctrl Pts',(-30.4841799844132,12.7360068046191,
126.759304891877)) ;
#148948=CARTESIAN_POINT('Ctrl Pts',(-30.4258743728948,13.0100794462922,
126.622138522883)) ;
#148949=CARTESIAN_POINT('Ctrl Pts',(-30.3928856489435,13.3126251519116,
126.558801239046)) ;
#148950=CARTESIAN_POINT('Ctrl Pts',(-30.3867270276499,13.6254713838339,
126.574107468755)) ;
#148951=CARTESIAN_POINT('Ctrl Pts',(-30.4071673743065,13.9212363983898,
126.666825972568)) ;
#148952=CARTESIAN_POINT('Ctrl Pts',(-30.4520657346943,14.182693359551,126.831154475535)) ;
#148953=CARTESIAN_POINT('Ctrl Pts',(-30.5172045915089,14.388968587839,127.054480565499)) ;
#148954=CARTESIAN_POINT('Ctrl Pts',(-30.5978949912035,14.5271449828327,
127.323459118803)) ;
#148955=CARTESIAN_POINT('Ctrl Pts',(-30.6869252863348,14.5852339313446,
127.616686057635)) ;
#148956=CARTESIAN_POINT('Ctrl Pts',(-30.7769736137098,14.5605427839008,
127.912730055109)) ;
#148957=CARTESIAN_POINT('Ctrl Pts',(-30.8618338634156,14.4541441821425,
128.193820416888)) ;
#148958=CARTESIAN_POINT('Ctrl Pts',(-30.933942967095,14.2740963581792,128.437570738178)) ;
#148959=CARTESIAN_POINT('Ctrl Pts',(-30.9878091811295,14.0323113149494,
128.628141355214)) ;
#148960=CARTESIAN_POINT('Ctrl Pts',(-31.0184130329351,13.7476340244825,
128.750639914861)) ;
#148961=CARTESIAN_POINT('Ctrl Pts',(-31.0232549340075,13.4408490996929,
128.797771945858)) ;
#148962=CARTESIAN_POINT('Ctrl Pts',(-31.0010012554192,13.1304291597349,
128.766011349424)) ;
#148963=CARTESIAN_POINT('Ctrl Pts',(-30.9527573293382,12.8426172775068,
128.658135893252)) ;
#148964=CARTESIAN_POINT('Ctrl Pts',(-30.8807389453885,12.5951022403137,
128.480994628538)) ;
#148965=CARTESIAN_POINT('Ctrl Pts',(-30.7904651788176,12.4086451366238,
128.250233623956)) ;
#148966=CARTESIAN_POINT('Ctrl Pts',(-30.6863228080809,12.2933533554013,
127.9792074839)) ;
#148967=CARTESIAN_POINT('Ctrl Pts',(-30.5756850359936,12.2596356648428,
127.689183859545)) ;
#148968=CARTESIAN_POINT('Ctrl Pts',(-30.466203016368,12.3091205496962,127.402403834731)) ;
#148969=CARTESIAN_POINT('Ctrl Pts',(-30.3643703623581,12.4379929184033,
127.138001306152)) ;
#148970=CARTESIAN_POINT('Ctrl Pts',(-30.2764808806105,12.6386444733354,
126.914510251683)) ;
#148971=CARTESIAN_POINT('Ctrl Pts',(-30.2090793318311,12.8942394600066,
126.750661369868)) ;
#148972=CARTESIAN_POINT('Ctrl Pts',(-30.1655515186205,13.1876523061434,
126.6565785761)) ;
#148973=CARTESIAN_POINT('Ctrl Pts',(-30.1483782750824,13.4984174202856,
126.639535142431)) ;
#148974=CARTESIAN_POINT('Ctrl Pts',(-30.1582136153607,13.804322851742,126.701452487564)) ;
#148975=CARTESIAN_POINT('Ctrl Pts',(-30.1935881730914,14.0825043451859,
126.837930713879)) ;
#148976=CARTESIAN_POINT('Ctrl Pts',(-30.2513065925607,14.3134150870924,
127.039706314653)) ;
#148977=CARTESIAN_POINT('Ctrl Pts',(-30.3260116279673,14.4799819682822,
127.290938064371)) ;
#148978=CARTESIAN_POINT('Ctrl Pts',(-30.4128554732831,14.5717628794977,
127.577963905631)) ;
#148979=CARTESIAN_POINT('Ctrl Pts',(-30.5031073153007,14.5804902548306,
127.874570300572)) ;
#148980=CARTESIAN_POINT('Ctrl Pts',(-30.5909549614635,14.5068426765183,
128.16431731435)) ;
#148981=CARTESIAN_POINT('Ctrl Pts',(-30.6689392721254,14.3556216409034,
128.425228448955)) ;
#148982=CARTESIAN_POINT('Ctrl Pts',(-30.7309826796393,14.1365917034713,
128.639714474064)) ;
#148983=CARTESIAN_POINT('Ctrl Pts',(-30.7713121688787,13.8680781333687,
128.790537435745)) ;
#148984=CARTESIAN_POINT('Ctrl Pts',(-30.7869976676125,13.5671870152877,
128.869457137254)) ;
#148985=CARTESIAN_POINT('Ctrl Pts',(-30.7756199855816,13.253754715573,128.869553597425)) ;
#148986=CARTESIAN_POINT('Ctrl Pts',(-30.7378428697437,12.9561226298826,
128.792121574417)) ;
#148987=CARTESIAN_POINT('Ctrl Pts',(-30.6750924058368,12.689577131159,128.6420045891)) ;
#148988=CARTESIAN_POINT('Ctrl Pts',(-30.5916276957833,12.4765149553713,
128.431238476743)) ;
#148989=CARTESIAN_POINT('Ctrl Pts',(-30.4919348522374,12.330399344862,128.173255254871)) ;
#148990=CARTESIAN_POINT('Ctrl Pts',(-30.3834739315927,12.2633426723701,
127.889471684178)) ;
#148991=CARTESIAN_POINT('Ctrl Pts',(-30.2725618689719,12.2791039533646,
127.598598845165)) ;
#148992=CARTESIAN_POINT('Ctrl Pts',(-30.1667739512017,12.3764766971553,
127.322629115757)) ;
#148993=CARTESIAN_POINT('Ctrl Pts',(-30.0722613215076,12.5500288330121,
127.079808436229)) ;
#148994=CARTESIAN_POINT('Ctrl Pts',(-29.9964223473625,12.7839577704924,
126.891194707482)) ;
#148995=CARTESIAN_POINT('Ctrl Pts',(-29.942454441113,13.0658040445484,126.766783601565)) ;
#148996=CARTESIAN_POINT('Ctrl Pts',(-29.9144858273214,13.3726170007347,
126.718219451376)) ;
#148997=CARTESIAN_POINT('Ctrl Pts',(-29.9135066816094,13.6826397065971,
126.748467644402)) ;
#148998=CARTESIAN_POINT('Ctrl Pts',(-29.93864177303,13.973415999198,126.854904439915)) ;
#148999=CARTESIAN_POINT('Ctrl Pts',(-29.9879875205848,14.2269288255441,
127.032360766386)) ;
#149000=CARTESIAN_POINT('Ctrl Pts',(-30.0562982578127,14.4205112234245,
127.264872894418)) ;
#149001=CARTESIAN_POINT('Ctrl Pts',(-30.1388423960146,14.5441065980074,
127.539162805067)) ;
#149002=CARTESIAN_POINT('Ctrl Pts',(-30.2288796774429,14.5870792667271,
127.835398320618)) ;
#149003=CARTESIAN_POINT('Ctrl Pts',(-30.318752130409,14.5462510446376,128.131069708792)) ;
#149004=CARTESIAN_POINT('Ctrl Pts',(-30.4011990424657,14.4261089740706,
128.404876189564)) ;
#149005=CARTESIAN_POINT('Ctrl Pts',(-30.4707707769806,14.2320089324099,
128.641468375281)) ;
#149006=CARTESIAN_POINT('Ctrl Pts',(-30.5201915042362,13.9821035017428,
128.818820320772)) ;
#149007=CARTESIAN_POINT('Ctrl Pts',(-30.5462282037767,13.6914861208152,
128.927995546701)) ;
#149008=CARTESIAN_POINT('Ctrl Pts',(-30.5460671305447,13.3820427303129,
128.96058514073)) ;
#149009=CARTESIAN_POINT('Ctrl Pts',(-30.5186186649558,13.0731825073203,
128.913731663666)) ;
#149010=CARTESIAN_POINT('Ctrl Pts',(-30.4658657649698,12.792789184468,128.792563884169)) ;
#149011=CARTESIAN_POINT('Ctrl Pts',(-30.390062659985,12.5553087421356,128.604324240762)) ;
#149012=CARTESIAN_POINT('Ctrl Pts',(-30.2964051343669,12.3807971817362,
128.363831596065)) ;
#149013=CARTESIAN_POINT('Ctrl Pts',(-30.1906919248692,12.2807361570638,
128.088147478697)) ;
#149014=CARTESIAN_POINT('Ctrl Pts',(-30.0798079005075,12.2625961451368,
127.797356146879)) ;
#149015=CARTESIAN_POINT('Ctrl Pts',(-29.970954505239,12.32755343176,127.512498551753)) ;
#149016=CARTESIAN_POINT('Ctrl Pts',(-29.8712078270959,12.4713199441997,
127.254267669833)) ;
#149017=CARTESIAN_POINT('Ctrl Pts',(-29.7873334259334,12.6818353121991,
127.042222843029)) ;
#149018=CARTESIAN_POINT('Ctrl Pts',(-29.7235176767161,12.9488694906299,
126.889210528772)) ;
#149019=CARTESIAN_POINT('Ctrl Pts',(-29.6852261685552,13.2449963341531,
126.810169235645)) ;
#149020=CARTESIAN_POINT('Ctrl Pts',(-29.6730505875199,13.5577145851588,
126.807868872823)) ;
#149021=CARTESIAN_POINT('Ctrl Pts',(-29.6878754711503,13.8591378593898,
126.884253177317)) ;
#149022=CARTESIAN_POINT('Ctrl Pts',(-29.7277642234698,14.130166831006,127.033958962988)) ;
#149023=CARTESIAN_POINT('Ctrl Pts',(-29.7890265231427,14.349825857909,127.246014723046)) ;
#149024=CARTESIAN_POINT('Ctrl Pts',(-29.8665533617496,14.5033075139511,
127.505580619346)) ;
#149025=CARTESIAN_POINT('Ctrl Pts',(-29.9542811977828,14.5795880781192,
127.795003544742)) ;
#149026=CARTESIAN_POINT('Ctrl Pts',(-30.0449500375347,14.5729975365321,
128.092978630465)) ;
#149027=CARTESIAN_POINT('Ctrl Pts',(-30.1317041723412,14.4837968841282,
128.379616319117)) ;
#149028=CARTESIAN_POINT('Ctrl Pts',(-30.2071928803997,14.3181446441766,
128.633325545973)) ;
#149029=CARTESIAN_POINT('Ctrl Pts',(-30.2650803133091,14.0900337543834,
128.83539277785)) ;
#149030=CARTESIAN_POINT('Ctrl Pts',(-30.3012106539237,13.8125788202494,
128.974133301393)) ;
#149031=CARTESIAN_POINT('Ctrl Pts',(-30.3117972843206,13.5087144247666,
129.038074958722)) ;
#149032=CARTESIAN_POINT('Ctrl Pts',(-30.2954912808033,13.1970642860529,
129.02364480025)) ;
#149033=CARTESIAN_POINT('Ctrl Pts',(-30.2526709527815,12.9023259165876,
128.931677028235)) ;
#149034=CARTESIAN_POINT('Ctrl Pts',(-30.1856053589782,12.6446851896536,
128.768924943894)) ;
#149035=CARTESIAN_POINT('Ctrl Pts',(-30.0988846407419,12.4436426987833,
128.548597777783)) ;
#149036=CARTESIAN_POINT('Ctrl Pts',(-29.9971156856899,12.311800617446,128.284491079494)) ;
#149037=CARTESIAN_POINT('Ctrl Pts',(-29.8875872119017,12.2597626710197,
127.997619613751)) ;
#149038=CARTESIAN_POINT('Ctrl Pts',(-29.7764046490522,12.2917039117493,
127.706157620277)) ;
#149039=CARTESIAN_POINT('Ctrl Pts',(-29.6728942100867,12.4035190207528,
127.436666928702)) ;
#149040=CARTESIAN_POINT('Ctrl Pts',(-29.5811635921256,12.5902948819765,
127.202036427248)) ;
#149041=CARTESIAN_POINT('Ctrl Pts',(-29.5093504589281,12.8337324593119,
127.02511882226)) ;
#149042=CARTESIAN_POINT('Ctrl Pts',(-29.459889065768,13.1235886512336,126.914040981108)) ;
#149043=CARTESIAN_POINT('Ctrl Pts',(-29.4372132851433,13.4302519465087,
126.880664182196)) ;
#149044=CARTESIAN_POINT('Ctrl Pts',(-29.4410746743041,13.7390104769504,
126.925099881042)) ;
#149045=CARTESIAN_POINT('Ctrl Pts',(-29.4713124307665,14.026006220093,127.046710522163)) ;
#149046=CARTESIAN_POINT('Ctrl Pts',(-29.5241600420331,14.267226887447,127.23403016745)) ;
#149047=CARTESIAN_POINT('Ctrl Pts',(-29.5958998341777,14.4498458774909,
127.476774523752)) ;
#149048=CARTESIAN_POINT('Ctrl Pts',(-29.6804543579856,14.5586319222976,
127.75695530447)) ;
#149049=CARTESIAN_POINT('Ctrl Pts',(-29.7710143154337,14.5856242109288,
128.054706589964)) ;
#149050=CARTESIAN_POINT('Ctrl Pts',(-29.8596478809037,14.5299078426425,
128.346578696437)) ;
#149051=CARTESIAN_POINT('Ctrl Pts',(-29.940797824085,14.3940108170827,128.616933746993)) ;
#149052=CARTESIAN_POINT('Ctrl Pts',(-30.0065313921842,14.1888421373124,
128.842072173602)) ;
#149053=CARTESIAN_POINT('Ctrl Pts',(-30.0518836645061,13.9299825539778,
129.007565480482)) ;
#149054=CARTESIAN_POINT('Ctrl Pts',(-30.0731422301956,13.6339609889882,
129.102792375169)) ;
#149055=CARTESIAN_POINT('Ctrl Pts',(-30.0678240733041,13.322716019869,129.120388848256)) ;
#149056=CARTESIAN_POINT('Ctrl Pts',(-30.0355611101008,13.0187245278142,
129.059274077997)) ;
#149057=CARTESIAN_POINT('Ctrl Pts',(-29.9782043992279,12.7442185255371,
128.924769323151)) ;
#149058=CARTESIAN_POINT('Ctrl Pts',(-29.8982556126516,12.5167189734132,
128.724530848476)) ;
#149059=CARTESIAN_POINT('Ctrl Pts',(-29.8023192584172,12.3563386644065,
128.477216795645)) ;
#149060=CARTESIAN_POINT('Ctrl Pts',(-29.6950698376708,12.2709228506509,
128.197061735731)) ;
#149061=CARTESIAN_POINT('Ctrl Pts',(-29.5837196202969,12.268610094108,127.904997982331)) ;
#149062=CARTESIAN_POINT('Ctrl Pts',(-29.4763327572683,12.3485945923255,
127.624335641344)) ;
#149063=CARTESIAN_POINT('Ctrl Pts',(-29.3786180682244,12.5068355789937,
127.372187573838)) ;
#149064=CARTESIAN_POINT('Ctrl Pts',(-29.2985863374153,12.7283300538896,
127.171287513075)) ;
#149065=CARTESIAN_POINT('Ctrl Pts',(-29.2394412133029,13.0013549210284,
127.031702565481)) ;
#149066=CARTESIAN_POINT('Ctrl Pts',(-29.2056837300174,13.3039530597295,
126.96618289312)) ;
#149067=CARTESIAN_POINT('Ctrl Pts',(-29.1987066729557,13.615850743561,126.978983927502)) ;
#149068=CARTESIAN_POINT('Ctrl Pts',(-29.2185194823492,13.9138454553417,
127.070043003934)) ;
#149069=CARTESIAN_POINT('Ctrl Pts',(-29.2625769744912,14.1752851805425,
127.231751072296)) ;
#149070=CARTESIAN_POINT('Ctrl Pts',(-29.3272880904875,14.3839668392215,
127.45390258644)) ;
#149071=CARTESIAN_POINT('Ctrl Pts',(-29.4075505220235,14.5240578226957,
127.721592281445)) ;
#149072=CARTESIAN_POINT('Ctrl Pts',(-29.4963462070103,14.584818929902,128.014106992847)) ;
#149073=CARTESIAN_POINT('Ctrl Pts',(-29.587047691809,14.5621167472896,128.312281230879)) ;
#149074=CARTESIAN_POINT('Ctrl Pts',(-29.6716157083653,14.4583966602146,
128.592308831358)) ;
#149075=CARTESIAN_POINT('Ctrl Pts',(-29.7442665614833,14.2803904178195,
128.837668999258)) ;
#149076=CARTESIAN_POINT('Ctrl Pts',(-29.7986307677681,14.0406559765549,
129.02962703218)) ;
#149077=CARTESIAN_POINT('Ctrl Pts',(-29.8301070762697,13.7571590399429,
129.154671220007)) ;
#149078=CARTESIAN_POINT('Ctrl Pts',(-29.8356379413796,13.4483332736025,
129.204074994619)) ;
#149079=CARTESIAN_POINT('Ctrl Pts',(-29.8143943312686,13.1406103992417,
129.174937518758)) ;
#149080=CARTESIAN_POINT('Ctrl Pts',(-29.7664779024948,12.8492377170497,
129.068326740931)) ;
#149081=CARTESIAN_POINT('Ctrl Pts',(-29.695477480617,12.6021186018862,128.893930092439)) ;
#149082=CARTESIAN_POINT('Ctrl Pts',(-29.6056095162878,12.4130744412516,
128.664414490585)) ;
#149083=CARTESIAN_POINT('Ctrl Pts',(-29.5013486547958,12.2953575367152,
128.393159695613)) ;
#149084=CARTESIAN_POINT('Ctrl Pts',(-29.3912652273664,12.2595400052722,
128.104616314454)) ;
#149085=CARTESIAN_POINT('Ctrl Pts',(-29.2815644215268,12.3063152816415,
127.81721837263)) ;
#149086=CARTESIAN_POINT('Ctrl Pts',(-29.1788437256449,12.4341408158502,
127.550424574528)) ;
#149087=CARTESIAN_POINT('Ctrl Pts',(-29.0911599373369,12.6316134537437,
127.327283665833)) ;
#149088=CARTESIAN_POINT('Ctrl Pts',(-29.0229070295168,12.8861349922411,
127.161015018853)) ;
#149089=CARTESIAN_POINT('Ctrl Pts',(-28.97860409195,13.1792138645797,127.064713176007)) ;
#149090=CARTESIAN_POINT('Ctrl Pts',(-28.960680378975,13.4905686905893,127.045557913132)) ;
#149091=CARTESIAN_POINT('Ctrl Pts',(-28.9698588717169,13.7964603430473,
127.105511528331)) ;
#149092=CARTESIAN_POINT('Ctrl Pts',(-29.0043770379677,14.0743847640953,
127.239335900994)) ;
#149093=CARTESIAN_POINT('Ctrl Pts',(-29.0613333209739,14.3070162131528,
127.438846969311)) ;
#149094=CARTESIAN_POINT('Ctrl Pts',(-29.1360898555168,14.4764518119822,
127.690429115817)) ;
#149095=CARTESIAN_POINT('Ctrl Pts',(-29.2219415160562,14.5698501625241,
127.974264672901)) ;
#149096=CARTESIAN_POINT('Ctrl Pts',(-29.3126334826048,14.5816111326668,
128.272334008304)) ;
#149097=CARTESIAN_POINT('Ctrl Pts',(-29.400926685228,14.5098992068035,128.563479690303)) ;
#149098=CARTESIAN_POINT('Ctrl Pts',(-29.4793116651,14.3604030985763,128.825592204278)) ;
#149099=CARTESIAN_POINT('Ctrl Pts',(-29.541687497227,14.1435657734104,129.04096069706)) ;
#149100=CARTESIAN_POINT('Ctrl Pts',(-29.5827585769447,13.8762647134096,
129.193957278894)) ;
#149101=CARTESIAN_POINT('Ctrl Pts',(-29.5990886189644,13.5746435358358,
129.274900295363)) ;
#149102=CARTESIAN_POINT('Ctrl Pts',(-29.5886877794002,13.2647987939523,
129.27746114699)) ;
#149103=CARTESIAN_POINT('Ctrl Pts',(-29.5514689178778,12.9638357563477,
129.201951033959)) ;
#149104=CARTESIAN_POINT('Ctrl Pts',(-29.489458499903,12.6967407948571,129.053914570688)) ;
#149105=CARTESIAN_POINT('Ctrl Pts',(-29.4063560646129,12.481516798795,128.844280719317)) ;
#149106=CARTESIAN_POINT('Ctrl Pts',(-29.3073900325767,12.3337893926253,
128.588297373864)) ;
#149107=CARTESIAN_POINT('Ctrl Pts',(-29.1988456086286,12.264079799943,128.304354062159)) ;
#149108=CARTESIAN_POINT('Ctrl Pts',(-29.0880318599508,12.2774691330631,
128.013725536534)) ;
#149109=CARTESIAN_POINT('Ctrl Pts',(-28.9819973355058,12.3724670081561,
127.737037424083)) ;
#149110=CARTESIAN_POINT('Ctrl Pts',(-28.8870857299463,12.5437673872502,
127.493027576055)) ;
#149111=CARTESIAN_POINT('Ctrl Pts',(-28.8105213920732,12.7765746367498,
127.302360710588)) ;
#149112=CARTESIAN_POINT('Ctrl Pts',(-28.7559878003064,13.056442650052,127.176189804149)) ;
#149113=CARTESIAN_POINT('Ctrl Pts',(-28.7271624657516,13.3632373960093,
127.125177982557)) ;
#149114=CARTESIAN_POINT('Ctrl Pts',(-28.7252862623066,13.6730054777402,
127.152742684901)) ;
#149115=CARTESIAN_POINT('Ctrl Pts',(-28.7500212628402,13.9671153090071,
127.258316722838)) ;
#149116=CARTESIAN_POINT('Ctrl Pts',(-28.7982268980631,14.2192390976399,
127.432074162142)) ;
#149117=CARTESIAN_POINT('Ctrl Pts',(-28.8665165492583,14.4164802278466,
127.664792796035)) ;
#149118=CARTESIAN_POINT('Ctrl Pts',(-28.9485994104117,14.5415580379271,
127.937643046099)) ;
#149119=CARTESIAN_POINT('Ctrl Pts',(-29.0382249365808,14.5869148385537,
128.232577398888)) ;
#149120=CARTESIAN_POINT('Ctrl Pts',(-29.1281597523479,14.5490099524811,
128.528401805914)) ;
#149121=CARTESIAN_POINT('Ctrl Pts',(-29.2114841346123,14.4299835675068,
128.805020302905)) ;
#149122=CARTESIAN_POINT('Ctrl Pts',(-29.2809121923004,14.2395160245118,
129.040888123246)) ;
#149123=CARTESIAN_POINT('Ctrl Pts',(-29.331316063822,13.9900850970595,129.221281104942)) ;
#149124=CARTESIAN_POINT('Ctrl Pts',(-29.3580576799696,13.7002631215164,
129.332511895375)) ;
#149125=CARTESIAN_POINT('Ctrl Pts',(-29.3586251855949,13.3906063614652,
129.367283951049)) ;
#149126=CARTESIAN_POINT('Ctrl Pts',(-29.332111341756,13.0826197728353,129.323015853458)) ;
#149127=CARTESIAN_POINT('Ctrl Pts',(-29.2798112779405,12.799748141124,129.203343741946)) ;
#149128=CARTESIAN_POINT('Ctrl Pts',(-29.2047720620516,12.5614903219102,
129.017238791305)) ;
#149129=CARTESIAN_POINT('Ctrl Pts',(-29.1114211901215,12.3846250484045,
128.777697539592)) ;
#149130=CARTESIAN_POINT('Ctrl Pts',(-29.0059135943882,12.2824688023076,
128.502620720195)) ;
#149131=CARTESIAN_POINT('Ctrl Pts',(-28.8953832435428,12.2619556296945,
128.212772441659)) ;
#149132=CARTESIAN_POINT('Ctrl Pts',(-28.7862638141337,12.3244284918516,
127.927167021378)) ;
#149133=CARTESIAN_POINT('Ctrl Pts',(-28.6859244781036,12.4664339674621,
127.667281194282)) ;
#149134=CARTESIAN_POINT('Ctrl Pts',(-28.601649102341,12.6753486557463,127.454052709534)) ;
#149135=CARTESIAN_POINT('Ctrl Pts',(-28.5375143918303,12.9390313518122,
127.299872509753)) ;
#149136=CARTESIAN_POINT('Ctrl Pts',(-28.4980517300494,13.2369182053758,
127.217692199479)) ;
#149137=CARTESIAN_POINT('Ctrl Pts',(-28.4852684345572,13.5497742859679,
127.213631750286)) ;
#149138=CARTESIAN_POINT('Ctrl Pts',(-28.4993005500257,13.8506093508767,
127.28757579924)) ;
#149139=CARTESIAN_POINT('Ctrl Pts',(-28.5384951621769,14.1229208970494,
127.435261606474)) ;
#149140=CARTESIAN_POINT('Ctrl Pts',(-28.599114960893,14.3440340084818,127.645398935015)) ;
#149141=CARTESIAN_POINT('Ctrl Pts',(-28.6763470623928,14.5000650086301,
127.904155603546)) ;
#149142=CARTESIAN_POINT('Ctrl Pts',(-28.7642922709141,14.5786444496306,
128.194360198328)) ;
#149143=CARTESIAN_POINT('Ctrl Pts',(-28.8544048477181,14.5743811791395,
128.490498687061)) ;
#149144=CARTESIAN_POINT('Ctrl Pts',(-28.9416453449683,14.4873599141627,
128.778661127787)) ;
#149145=CARTESIAN_POINT('Ctrl Pts',(-29.0173714867235,14.3240887387416,
129.032983567367)) ;
#149146=CARTESIAN_POINT('Ctrl Pts',(-29.0759121873307,14.0972553768965,
129.237016152545)) ;
#149147=CARTESIAN_POINT('Ctrl Pts',(-29.1126883189575,13.8219068186535,
129.377531219329)) ;
#149148=CARTESIAN_POINT('Ctrl Pts',(-29.1241085948694,13.5160257304535,
129.444183524273)) ;
#149149=CARTESIAN_POINT('Ctrl Pts',(-29.1084287640549,13.2050738330625,
129.431492819495)) ;
#149150=CARTESIAN_POINT('Ctrl Pts',(-29.0664893049883,12.9106474660782,
129.341984766231)) ;
#149151=CARTESIAN_POINT('Ctrl Pts',(-29.000224510898,12.6518068845878,129.181529079168)) ;
#149152=CARTESIAN_POINT('Ctrl Pts',(-28.9136374703434,12.4481718764226,
128.961732310351)) ;
#149153=CARTESIAN_POINT('Ctrl Pts',(-28.8123624754787,12.314346622866,128.699007111475)) ;
#149154=CARTESIAN_POINT('Ctrl Pts',(-28.7023901141071,12.2602411291599,
128.4110156196)) ;
#149155=CARTESIAN_POINT('Ctrl Pts',(-28.5926670744185,12.289044210784,128.123343501971)) ;
#149156=CARTESIAN_POINT('Ctrl Pts',(-28.4876267780401,12.3996398985986,
127.84978474962)) ;
#149157=CARTESIAN_POINT('Ctrl Pts',(-28.3962438763497,12.5827969028938,
127.61585743653)) ;
#149158=CARTESIAN_POINT('Ctrl Pts',(-28.3231203552759,12.8269629878668,
127.435435519098)) ;
#149159=CARTESIAN_POINT('Ctrl Pts',(-28.2734596418954,13.1127056220744,
127.323400536975)) ;
#149160=CARTESIAN_POINT('Ctrl Pts',(-28.2496308502148,13.4217118821407,
127.286956931971)) ;
#149161=CARTESIAN_POINT('Ctrl Pts',(-28.2528361924696,13.73042511485,127.329433354869)) ;
#149162=CARTESIAN_POINT('Ctrl Pts',(-28.2823066708455,14.0183443112805,
127.448796933238)) ;
#149163=CARTESIAN_POINT('Ctrl Pts',(-28.3346958598102,14.2615011985034,
127.634845761707)) ;
#149164=CARTESIAN_POINT('Ctrl Pts',(-28.4058819950025,14.4455241600489,
127.875911043545)) ;
#149165=CARTESIAN_POINT('Ctrl Pts',(-28.4898905661539,14.5564730484766,
128.154399957566)) ;
#149166=CARTESIAN_POINT('Ctrl Pts',(-28.5807055884456,14.5860332576142,
128.453018836069)) ;
#149167=CARTESIAN_POINT('Ctrl Pts',(-28.6693097598626,14.5327319969804,
128.744739341118)) ;
#149168=CARTESIAN_POINT('Ctrl Pts',(-28.7508832134965,14.3988255377981,
129.016374996236)) ;
#149169=CARTESIAN_POINT('Ctrl Pts',(-28.8168463104849,14.1966329987979,
129.242018320441)) ;
#149170=CARTESIAN_POINT('Ctrl Pts',(-28.8631468967079,13.9381995065902,
129.410426459371)) ;
#149171=CARTESIAN_POINT('Ctrl Pts',(-28.8851222804496,13.64215083048,129.50782242196)) ;
#149172=CARTESIAN_POINT('Ctrl Pts',(-28.8805504060926,13.3319748624789,
129.527502418803)) ;
#149173=CARTESIAN_POINT('Ctrl Pts',(-28.8491918684474,13.0275242268779,
129.469008498518)) ;
#149174=CARTESIAN_POINT('Ctrl Pts',(-28.7919506539434,12.7499513876655,
129.335103926236)) ;
#149175=CARTESIAN_POINT('Ctrl Pts',(-28.7132681692753,12.5230806555812,
129.138248537529)) ;
#149176=CARTESIAN_POINT('Ctrl Pts',(-28.6172910431696,12.3595163887299,
128.89099290087)) ;
#149177=CARTESIAN_POINT('Ctrl Pts',(-28.5099858369398,12.2720601229367,
128.610740548863)) ;
#149178=CARTESIAN_POINT('Ctrl Pts',(-28.3988746086419,12.2676665272562,
128.319307904433)) ;
#149179=CARTESIAN_POINT('Ctrl Pts',(-28.2916704296753,12.3451447883363,
128.039067626911)) ;
#149180=CARTESIAN_POINT('Ctrl Pts',(-28.1938030804671,12.5004781878849,
127.786370689149)) ;
#149181=CARTESIAN_POINT('Ctrl Pts',(-28.1127625486316,12.7212076725333,
127.582685380892)) ;
#149182=CARTESIAN_POINT('Ctrl Pts',(-28.0529273651762,12.9936144334216,
127.44113357359)) ;
#149183=CARTESIAN_POINT('Ctrl Pts',(-28.0185364565288,13.2947836175078,
127.373668817087)) ;
#149184=CARTESIAN_POINT('Ctrl Pts',(-28.0107408413296,13.6064067051063,
127.384044252762)) ;
#149185=CARTESIAN_POINT('Ctrl Pts',(-28.0297193147551,13.9050216556666,
127.472646955327)) ;
#149186=CARTESIAN_POINT('Ctrl Pts',(-28.073239487346,14.1686336001984,127.632890974336)) ;
#149187=CARTESIAN_POINT('Ctrl Pts',(-28.1374216336648,14.378818223522,127.853475232984)) ;
#149188=CARTESIAN_POINT('Ctrl Pts',(-28.2171034635145,14.520866250274,128.119384876184)) ;
#149189=CARTESIAN_POINT('Ctrl Pts',(-28.3058570218466,14.5841619926364,
128.411824363996)) ;
#149190=CARTESIAN_POINT('Ctrl Pts',(-28.3963167152646,14.5641966334699,
128.709179860555)) ;
#149191=CARTESIAN_POINT('Ctrl Pts',(-28.4815558486508,14.4625802261662,
128.991316551239)) ;
#149192=CARTESIAN_POINT('Ctrl Pts',(-28.5547405617564,14.2860055470816,
129.238296594858)) ;
#149193=CARTESIAN_POINT('Ctrl Pts',(-28.6095231775212,14.0484512040757,
129.431382925857)) ;
#149194=CARTESIAN_POINT('Ctrl Pts',(-28.6417291928216,13.7663469877686,
129.558524603165)) ;
#149195=CARTESIAN_POINT('Ctrl Pts',(-28.6481036317158,13.4574608016115,
129.610440627955)) ;
#149196=CARTESIAN_POINT('Ctrl Pts',(-28.6275137977541,13.1488899436826,
129.583281486172)) ;
#149197=CARTESIAN_POINT('Ctrl Pts',(-28.5806601514756,12.8583365068185,
129.47957329379)) ;
#149198=CARTESIAN_POINT('Ctrl Pts',(-28.5101080825143,12.6085157636358,
129.306619716631)) ;
#149199=CARTESIAN_POINT('Ctrl Pts',(-28.4204678433571,12.4173946881525,
129.077837978652)) ;
#149200=CARTESIAN_POINT('Ctrl Pts',(-28.3170957380088,12.2980452511377,
128.808995646945)) ;
#149201=CARTESIAN_POINT('Ctrl Pts',(-28.2070141547135,12.2592457783441,
128.520489824639)) ;
#149202=CARTESIAN_POINT('Ctrl Pts',(-28.0966798508768,12.3040208599772,
128.231400572317)) ;
#149203=CARTESIAN_POINT('Ctrl Pts',(-27.9943480589568,12.42869393012,127.965511512337)) ;
#149204=CARTESIAN_POINT('Ctrl Pts',(-27.9058058272702,12.6243589904513,
127.739953405032)) ;
#149205=CARTESIAN_POINT('Ctrl Pts',(-27.8366054021169,12.8789083134422,
127.571086073474)) ;
#149206=CARTESIAN_POINT('Ctrl Pts',(-27.7917969297281,13.1702260749438,
127.473192849682)) ;
#149207=CARTESIAN_POINT('Ctrl Pts',(-27.7730507275345,13.4805036565043,
127.451546760695)) ;
#149208=CARTESIAN_POINT('Ctrl Pts',(-27.7813694599879,13.7876510907378,
127.509064273961)) ;
#149209=CARTESIAN_POINT('Ctrl Pts',(-27.8154365035927,14.0678452038592,
127.641730149674)) ;
#149210=CARTESIAN_POINT('Ctrl Pts',(-27.8715485760057,14.3007432153336,
127.838599286977)) ;
#149211=CARTESIAN_POINT('Ctrl Pts',(-27.9459217672765,14.4725786028925,
128.089102623514)) ;
#149212=CARTESIAN_POINT('Ctrl Pts',(-28.0315487597573,14.5682598705244,
128.372281879499)) ;
#149213=CARTESIAN_POINT('Ctrl Pts',(-28.1221926549195,14.582415300085,128.670208784852)) ;
#149214=CARTESIAN_POINT('Ctrl Pts',(-28.2105289219673,14.5133615021942,
128.961420781404)) ;
#149215=CARTESIAN_POINT('Ctrl Pts',(-28.2894313960368,14.3656856001402,
129.225113968176)) ;
#149216=CARTESIAN_POINT('Ctrl Pts',(-28.3521146601827,14.1519224163712,
129.441208760275)) ;
#149217=CARTESIAN_POINT('Ctrl Pts',(-28.3942042091648,13.8839966757843,
129.597426788259)) ;
#149218=CARTESIAN_POINT('Ctrl Pts',(-28.411183496847,13.5839687082689,129.680149626296)) ;
#149219=CARTESIAN_POINT('Ctrl Pts',(-28.4015693530436,13.2736212101871,
129.685068948691)) ;
#149220=CARTESIAN_POINT('Ctrl Pts',(-28.3652283835743,12.972761740788,129.612034453461)) ;
#149221=CARTESIAN_POINT('Ctrl Pts',(-28.3037016460954,12.7034621724925,
129.465528552906)) ;
#149222=CARTESIAN_POINT('Ctrl Pts',(-28.2211593027135,12.4867212726039,
129.257507750308)) ;
#149223=CARTESIAN_POINT('Ctrl Pts',(-28.1224616177338,12.33686375234,129.00233956032)) ;
#149224=CARTESIAN_POINT('Ctrl Pts',(-28.0144538218038,12.2650347020363,
128.719854075902)) ;
#149225=CARTESIAN_POINT('Ctrl Pts',(-27.903322484762,12.2758062427332,128.428381261578)) ;
#149226=CARTESIAN_POINT('Ctrl Pts',(-27.7966709347457,12.3692806824326,
128.150022376286)) ;
#149227=CARTESIAN_POINT('Ctrl Pts',(-27.7018440324355,12.5378928700438,
127.90609386885)) ;
#149228=CARTESIAN_POINT('Ctrl Pts',(-27.6245512268183,12.7694276671961,
127.71335608596)) ;
#149229=CARTESIAN_POINT('Ctrl Pts',(-27.5693299508102,13.0484835222186,
127.585194618187)) ;
#149230=CARTESIAN_POINT('Ctrl Pts',(-27.5397791508547,13.3553251323831,
127.532112766213)) ;
#149231=CARTESIAN_POINT('Ctrl Pts',(-27.5372330226569,13.6640555528138,
127.557595480549)) ;
#149232=CARTESIAN_POINT('Ctrl Pts',(-27.5609754676578,13.9577070020221,
127.660108078298)) ;
#149233=CARTESIAN_POINT('Ctrl Pts',(-27.6087555543691,14.2128779574234,
127.832817362159)) ;
#149234=CARTESIAN_POINT('Ctrl Pts',(-27.6765781719764,14.4117544090383,
128.06416116346)) ;
#149235=CARTESIAN_POINT('Ctrl Pts',(-27.7582934482354,14.5391282978367,
128.335923995923)) ;
#149236=CARTESIAN_POINT('Ctrl Pts',(-27.8482168316244,14.5867879388137,
128.631877918567)) ;
#149237=CARTESIAN_POINT('Ctrl Pts',(-27.9378092608112,14.5512051558335,
128.926543960514)) ;
#149238=CARTESIAN_POINT('Ctrl Pts',(-28.0215701238513,14.4343419868163,
129.204490622999)) ;
#149239=CARTESIAN_POINT('Ctrl Pts',(-28.0914436828456,14.2455278890041,
129.441668406184)) ;
#149240=CARTESIAN_POINT('Ctrl Pts',(-28.14235674795,13.9981929113896,129.623467068814)) ;
#149241=CARTESIAN_POINT('Ctrl Pts',(-28.1698989580778,13.7085066713852,
129.737123007789)) ;
#149242=CARTESIAN_POINT('Ctrl Pts',(-28.1711628301339,13.399579397686,129.773878387293)) ;
#149243=CARTESIAN_POINT('Ctrl Pts',(-28.1455841160295,13.0919774800644,
129.732252462512)) ;
#149244=CARTESIAN_POINT('Ctrl Pts',(-28.093714453794,12.8067303941414,129.614004992358)) ;
#149245=CARTESIAN_POINT('Ctrl Pts',(-28.019645857162,12.5682009002538,129.430560739033)) ;
#149246=CARTESIAN_POINT('Ctrl Pts',(-27.9266142891176,12.3888212381261,
129.192018455593)) ;
#149247=CARTESIAN_POINT('Ctrl Pts',(-27.821510585854,12.2844119567793,128.918075924403)) ;
#149248=CARTESIAN_POINT('Ctrl Pts',(-27.7106897292081,12.2613333921228,
128.62748362164)) ;
#149249=CARTESIAN_POINT('Ctrl Pts',(-27.6015516143989,12.3215794364131,
128.341786595649)) ;
#149250=CARTESIAN_POINT('Ctrl Pts',(-27.5011797769738,12.460691871722,128.081688658565)) ;
#149251=CARTESIAN_POINT('Ctrl Pts',(-27.4159829565428,12.6684213350559,
127.865897041431)) ;
#149252=CARTESIAN_POINT('Ctrl Pts',(-27.3510487739651,12.9319194586172,
127.709496777072)) ;
#149253=CARTESIAN_POINT('Ctrl Pts',(-27.3111098739424,13.227908152673,127.625786027641)) ;
#149254=CARTESIAN_POINT('Ctrl Pts',(-27.2974612593413,13.5392232276546,
127.619043390422)) ;
#149255=CARTESIAN_POINT('Ctrl Pts',(-27.3107067357766,13.842168223521,127.690850798586)) ;
#149256=CARTESIAN_POINT('Ctrl Pts',(-27.3492738204767,14.115831938889,127.836726726766)) ;
#149257=CARTESIAN_POINT('Ctrl Pts',(-27.4094876845083,14.3390092448437,
128.045746045153)) ;
#149258=CARTESIAN_POINT('Ctrl Pts',(-27.4862037303775,14.4964745213525,
128.302922976793)) ;
#149259=CARTESIAN_POINT('Ctrl Pts',(-27.5734126890435,14.5773715613601,
128.590785930487)) ;
#149260=CARTESIAN_POINT('Ctrl Pts',(-27.6642277201677,14.5757025452078,
128.889231125655)) ;
#149261=CARTESIAN_POINT('Ctrl Pts',(-27.7514325880381,14.4908671565799,
129.177203535286)) ;
#149262=CARTESIAN_POINT('Ctrl Pts',(-27.8273172084641,14.3305923822081,
129.431861219863)) ;
#149263=CARTESIAN_POINT('Ctrl Pts',(-27.8867448350719,14.104809150226,129.638607059385)) ;
#149264=CARTESIAN_POINT('Ctrl Pts',(-27.924232723082,13.8293692517449,129.781327493485)) ;
#149265=CARTESIAN_POINT('Ctrl Pts',(-27.9363393689926,13.5265764588792,
129.849706205578)) ;
#149266=CARTESIAN_POINT('Ctrl Pts',(-27.9215766706455,13.2147295864641,
129.839779247584)) ;
#149267=CARTESIAN_POINT('Ctrl Pts',(-27.8803348251946,12.9189025959915,
129.752369876601)) ;
#149268=CARTESIAN_POINT('Ctrl Pts',(-27.8144585897609,12.6580300058624,
129.593157007656)) ;
#149269=CARTESIAN_POINT('Ctrl Pts',(-27.7287463868753,12.4534346092271,
129.375772364678)) ;
#149270=CARTESIAN_POINT('Ctrl Pts',(-27.6275620489468,12.3171076875182,
129.113399636911)) ;
#149271=CARTESIAN_POINT('Ctrl Pts',(-27.518308419636,12.2606844041001,128.827331139409)) ;
#149272=CARTESIAN_POINT('Ctrl Pts',(-27.4077125727585,12.28708894542,128.537351097586)) ;
#149273=CARTESIAN_POINT('Ctrl Pts',(-27.3024709202027,12.3957982979784,
128.26319136607)) ;
#149274=CARTESIAN_POINT('Ctrl Pts',(-27.2108581166926,12.5767256931705,
128.02852604486)) ;
#149275=CARTESIAN_POINT('Ctrl Pts',(-27.1372315199395,12.8186993090181,
127.846557861036)) ;
#149276=CARTESIAN_POINT('Ctrl Pts',(-27.0866060204049,13.1050418122632,
127.73188330392)) ;
#149277=CARTESIAN_POINT('Ctrl Pts',(-27.062162804843,13.4130762774239,127.693567342574)) ;
#149278=CARTESIAN_POINT('Ctrl Pts',(-27.0646120500407,13.7214651922854,
127.733776018884)) ;
#149279=CARTESIAN_POINT('Ctrl Pts',(-27.0931056884195,14.0093161803211,
127.850144303508)) ;
#149280=CARTESIAN_POINT('Ctrl Pts',(-27.1453032721948,14.2560736745197,
128.035916176362)) ;
#149281=CARTESIAN_POINT('Ctrl Pts',(-27.2158872721112,14.4412184324741,
128.275118516804)) ;
#149282=CARTESIAN_POINT('Ctrl Pts',(-27.2996010171685,14.5543182486296,
128.552747603182)) ;
#149283=CARTESIAN_POINT('Ctrl Pts',(-27.3899118087328,14.5864671226158,
128.84973273768)) ;
#149284=CARTESIAN_POINT('Ctrl Pts',(-27.4792618290635,14.5351930483474,
129.14386643155)) ;
#149285=CARTESIAN_POINT('Ctrl Pts',(-27.560663470632,14.4042256836979,129.414791679736)) ;
#149286=CARTESIAN_POINT('Ctrl Pts',(-27.6274454081149,14.2033620376663,
129.642954413426)) ;
#149287=CARTESIAN_POINT('Ctrl Pts',(-27.6743631483564,13.9460943554148,
129.81317254965)) ;
#149288=CARTESIAN_POINT('Ctrl Pts',(-27.697059062296,13.6510940707038,129.912646290026)) ;
#149289=CARTESIAN_POINT('Ctrl Pts',(-27.6932988178505,13.340963323575,129.934704831616)) ;
#149290=CARTESIAN_POINT('Ctrl Pts',(-27.6625764453814,13.0355469770442,
129.878128940385)) ;
#149291=CARTESIAN_POINT('Ctrl Pts',(-27.6064258233987,12.7584810816834,
129.747205231254)) ;
#149292=CARTESIAN_POINT('Ctrl Pts',(-27.5280729952501,12.5287899159639,
129.551452346458)) ;
#149293=CARTESIAN_POINT('Ctrl Pts',(-27.4324998329583,12.3633457442531,
129.305367372387)) ;
#149294=CARTESIAN_POINT('Ctrl Pts',(-27.3258016217117,12.2737023514909,
129.026778387411)) ;
#149295=CARTESIAN_POINT('Ctrl Pts',(-27.21466759507,12.2663504443872,128.73528774347)) ;
#149296=CARTESIAN_POINT('Ctrl Pts',(-27.1066093889239,12.3420800967331,
128.452760176601)) ;
#149297=CARTESIAN_POINT('Ctrl Pts',(-27.0088321504467,12.4946575605773,
128.200166185438)) ;
#149298=CARTESIAN_POINT('Ctrl Pts',(-26.9269407651993,12.7142648856192,
127.994104420372)) ;
#149299=CARTESIAN_POINT('Ctrl Pts',(-26.8665124531143,12.9853993961476,
127.850796596108)) ;
#149300=CARTESIAN_POINT('Ctrl Pts',(-26.8313430052465,13.2860373557687,
127.781066453358)) ;
#149301=CARTESIAN_POINT('Ctrl Pts',(-26.8227999641649,13.5985521220417,
127.789346344921)) ;
#149302=CARTESIAN_POINT('Ctrl Pts',(-26.8411427705591,13.8975127829307,
127.876068717954)) ;
#149303=CARTESIAN_POINT('Ctrl Pts',(-26.8838031630307,14.1612605834451,
128.033657379763)) ;
#149304=CARTESIAN_POINT('Ctrl Pts',(-26.9476004607464,14.3739607965711,
128.253212935099)) ;
#149305=CARTESIAN_POINT('Ctrl Pts',(-27.0272151946275,14.5182946770733,
128.519024634964)) ;
#149306=CARTESIAN_POINT('Ctrl Pts',(-27.1156612052403,14.5834512789115,
128.810503268048)) ;
#149307=CARTESIAN_POINT('Ctrl Pts',(-27.2058710054321,14.5659482327596,
129.107021227185)) ;
#149308=CARTESIAN_POINT('Ctrl Pts',(-27.2913403326924,14.4667698012676,
129.389820244375)) ;
#149309=CARTESIAN_POINT('Ctrl Pts',(-27.365037513102,14.2923286042259,129.638305562232)) ;
#149310=CARTESIAN_POINT('Ctrl Pts',(-27.4206675378827,14.0548140829524,
129.834057411563)) ;
#149311=CARTESIAN_POINT('Ctrl Pts',(-27.4532942174668,13.7751054623822,
129.962249175486)) ;
#149312=CARTESIAN_POINT('Ctrl Pts',(-27.4605705712052,13.4671707180117,
130.016748758532)) ;
#149313=CARTESIAN_POINT('Ctrl Pts',(-27.4405768382025,13.1566326950211,
129.99151897037)) ;
#149314=CARTESIAN_POINT('Ctrl Pts',(-27.3947125191724,12.867030876862,129.890495120701)) ;
#149315=CARTESIAN_POINT('Ctrl Pts',(-27.3246005780535,12.6146257470566,
129.718955677147)) ;
#149316=CARTESIAN_POINT('Ctrl Pts',(-27.2352104972191,12.4216271704312,
129.490959132207)) ;
#149317=CARTESIAN_POINT('Ctrl Pts',(-27.1326277544319,12.300493633533,129.224268899247)) ;
#149318=CARTESIAN_POINT('Ctrl Pts',(-27.0220193247481,12.2591976943658,
128.934414356228)) ;
#149319=CARTESIAN_POINT('Ctrl Pts',(-26.9123324711744,12.3014766472521,
128.646990110332)) ;
#149320=CARTESIAN_POINT('Ctrl Pts',(-26.8094227622297,12.4236752420719,
128.379476345014)) ;
#149321=CARTESIAN_POINT('Ctrl Pts',(-26.7198695890128,12.619137551761,128.151191815619)) ;
#149322=CARTESIAN_POINT('Ctrl Pts',(-26.6505624975948,12.8707902283033,
127.981794105051)) ;
#149323=CARTESIAN_POINT('Ctrl Pts',(-26.6049003931584,13.1617413070734,
127.881471015381)) ;
#149324=CARTESIAN_POINT('Ctrl Pts',(-26.5854473892697,13.4713352459494,
127.857705276412)) ;
#149325=CARTESIAN_POINT('Ctrl Pts',(-26.5929490593232,13.778502178637,127.912793617474)) ;
#149326=CARTESIAN_POINT('Ctrl Pts',(-26.6261889122264,14.0596468984735,
128.043011359952)) ;
#149327=CARTESIAN_POINT('Ctrl Pts',(-26.6819953534812,14.2953142204187,
128.239156752771)) ;
#149328=CARTESIAN_POINT('Ctrl Pts',(-26.7559539371804,14.4689647045759,
128.488434863537)) ;
#149329=CARTESIAN_POINT('Ctrl Pts',(-26.8416162758305,14.5668407202151,
128.771816073632)) ;
#149330=CARTESIAN_POINT('Ctrl Pts',(-26.9317772171447,14.5831863672356,
129.06816269229)) ;
#149331=CARTESIAN_POINT('Ctrl Pts',(-27.0206452753331,14.5160479467046,
129.361074683035)) ;
#149332=CARTESIAN_POINT('Ctrl Pts',(-27.0994865478493,14.371057406114,129.624417159767)) ;
#149333=CARTESIAN_POINT('Ctrl Pts',(-27.1628566341757,14.1586832935138,
129.842590444057)) ;
#149334=CARTESIAN_POINT('Ctrl Pts',(-27.2054989868208,13.8924169027706,
130.000362090636)) ;
#149335=CARTESIAN_POINT('Ctrl Pts',(-27.223288580354,13.5934591668299,130.085415073904)) ;
#149336=CARTESIAN_POINT('Ctrl Pts',(-27.2144128625738,13.2817950572783,
130.092631458139)) ;
#149337=CARTESIAN_POINT('Ctrl Pts',(-27.1787460156679,12.9807521840059,
130.021531190684)) ;
#149338=CARTESIAN_POINT('Ctrl Pts',(-27.1182536558926,12.7114089548823,
129.877887175819)) ;
#149339=CARTESIAN_POINT('Ctrl Pts',(-27.0359874106081,12.4920356351317,
129.670798191775)) ;
#149340=CARTESIAN_POINT('Ctrl Pts',(-26.9379376281562,12.3404092688171,
129.417431448621)) ;
#149341=CARTESIAN_POINT('Ctrl Pts',(-26.829743084675,12.2658594334509,129.134518780991)) ;
#149342=CARTESIAN_POINT('Ctrl Pts',(-26.7187403880943,12.2744067631739,
128.843375453836)) ;
#149343=CARTESIAN_POINT('Ctrl Pts',(-26.6121463544767,12.3651073313828,
128.565090827221)) ;
#149344=CARTESIAN_POINT('Ctrl Pts',(-26.5167176009969,12.5316552187529,
128.319448476852)) ;
#149345=CARTESIAN_POINT('Ctrl Pts',(-26.4386322226201,12.7621960771077,
128.124482385513)) ;
#149346=CARTESIAN_POINT('Ctrl Pts',(-26.3828261298418,13.0400248542652,
127.994587296118)) ;
#149347=CARTESIAN_POINT('Ctrl Pts',(-26.3525190565265,13.3449924415224,
127.939149409341)) ;
#149348=CARTESIAN_POINT('Ctrl Pts',(-26.3491468760843,13.6560823827408,
127.962454240853)) ;
#149349=CARTESIAN_POINT('Ctrl Pts',(-26.372164679168,13.9495229886617,128.062741811689)) ;
#149350=CARTESIAN_POINT('Ctrl Pts',(-26.4192453975585,14.2060601785511,
128.233401209434)) ;
#149351=CARTESIAN_POINT('Ctrl Pts',(-26.4865387051378,14.406853356067,128.463190725204)) ;
#149352=CARTESIAN_POINT('Ctrl Pts',(-26.568036262976,14.5364834433348,128.734360307803)) ;
#149353=CARTESIAN_POINT('Ctrl Pts',(-26.6574616375403,14.5865952299809,
129.028720457278)) ;
#149354=CARTESIAN_POINT('Ctrl Pts',(-26.7476261509057,14.5532896957255,
129.325240815001)) ;
#149355=CARTESIAN_POINT('Ctrl Pts',(-26.831290016583,14.4391769984152,129.602746393984)) ;
#149356=CARTESIAN_POINT('Ctrl Pts',(-26.9018234679493,14.2521193913653,
129.841924000037)) ;
#149357=CARTESIAN_POINT('Ctrl Pts',(-26.953372839476,14.0064609984077,130.025559364404)) ;
#149358=CARTESIAN_POINT('Ctrl Pts',(-26.9817302296853,13.7162751815943,
130.14175646995)) ;
#149359=CARTESIAN_POINT('Ctrl Pts',(-26.9837110537891,13.4088590373153,
130.18046815682)) ;
#149360=CARTESIAN_POINT('Ctrl Pts',(-26.9588874732449,13.1005339058846,
130.141091745965)) ;
#149361=CARTESIAN_POINT('Ctrl Pts',(-26.907970796887,12.8153801533597,130.025495563498)) ;
#149362=CARTESIAN_POINT('Ctrl Pts',(-26.8343613372862,12.5742829537778,
129.843499520031)) ;
#149363=CARTESIAN_POINT('Ctrl Pts',(-26.7412853262,12.392420790546,129.604979348717)) ;
#149364=CARTESIAN_POINT('Ctrl Pts',(-26.6369717859904,12.2864008615048,
129.333172629999)) ;
#149365=CARTESIAN_POINT('Ctrl Pts',(-26.5258572296115,12.2608494064564,
129.041832035797)) ;
#149366=CARTESIAN_POINT('Ctrl Pts',(-26.4170347717267,12.3186106427626,
128.756917900028)) ;
#149367=CARTESIAN_POINT('Ctrl Pts',(-26.3160996326238,12.4554522853447,
128.495226419321)) ;
#149368=CARTESIAN_POINT('Ctrl Pts',(-26.2301003884934,12.6626734835884,
128.277242969498)) ;
#149369=CARTESIAN_POINT('Ctrl Pts',(-26.1651571607187,12.9221025323028,
128.120471859074)) ;
#149370=CARTESIAN_POINT('Ctrl Pts',(-26.1240596389376,13.2188657935947,
128.033566809399)) ;
#149371=CARTESIAN_POINT('Ctrl Pts',(-26.1097033403075,13.5309968714097,
128.024847539681)) ;
#149372=CARTESIAN_POINT('Ctrl Pts',(-26.1221635460237,13.833390940375,128.094243989074)) ;
#149373=CARTESIAN_POINT('Ctrl Pts',(-26.1599919314982,14.1082731705155,
128.237962010862)) ;
#149374=CARTESIAN_POINT('Ctrl Pts',(-26.2196288030865,14.3332733281916,
128.445300705723)) ;
#149375=CARTESIAN_POINT('Ctrl Pts',(-26.2961210056048,14.4930898845826,
128.701897547713)) ;
#149376=CARTESIAN_POINT('Ctrl Pts',(-26.3830264974971,14.5762694584335,
128.988831295629)) ;
#149377=CARTESIAN_POINT('Ctrl Pts',(-26.4741788643102,14.5766426622739,
129.288393030434)) ;
#149378=CARTESIAN_POINT('Ctrl Pts',(-26.5608022072879,14.4950562230295,
129.57435464937)) ;
#149379=CARTESIAN_POINT('Ctrl Pts',(-26.6377807342573,14.3357813404639,
129.832489798271)) ;
#149380=CARTESIAN_POINT('Ctrl Pts',(-26.6975264006213,14.1117727148765,
130.040093620744)) ;
#149381=CARTESIAN_POINT('Ctrl Pts',(-26.7356954570761,13.8385113362907,
130.184699682537)) ;
#149382=CARTESIAN_POINT('Ctrl Pts',(-26.7485655418517,13.5338963360909,
130.255564378225)) ;
#149383=CARTESIAN_POINT('Ctrl Pts',(-26.7346407265886,13.2242576561067,
130.247831508955)) ;
#149384=CARTESIAN_POINT('Ctrl Pts',(-26.6939418479399,12.9262819739174,
130.162178455022)) ;
#149385=CARTESIAN_POINT('Ctrl Pts',(-26.6291144483335,12.6654698991639,
130.005833635842)) ;
#149386=CARTESIAN_POINT('Ctrl Pts',(-26.5431047888369,12.4574146452965,
129.787885297242)) ;
#149387=CARTESIAN_POINT('Ctrl Pts',(-26.443309400981,12.3205165730399,129.529210198504)) ;
#149388=CARTESIAN_POINT('Ctrl Pts',(-26.3336075645494,12.2610390486759,
129.242027806129)) ;
#149389=CARTESIAN_POINT('Ctrl Pts',(-26.2233061878199,12.2851065048332,
128.952795655811)) ;
#149390=CARTESIAN_POINT('Ctrl Pts',(-26.1176723705432,12.3913707363663,
128.677523801392)) ;
#149391=CARTESIAN_POINT('Ctrl Pts',(-26.025506878235,12.5705078611999,128.441274776628)) ;
#149392=CARTESIAN_POINT('Ctrl Pts',(-25.9512744951246,12.8110530748773,
128.257547459859)) ;
#149393=CARTESIAN_POINT('Ctrl Pts',(-25.8999845865538,13.0958080893831,
128.140865241115)) ;
#149394=CARTESIAN_POINT('Ctrl Pts',(-25.8746957774511,13.4043791335754,
128.100179674998)) ;
#149395=CARTESIAN_POINT('Ctrl Pts',(-25.8763352309333,13.7127503625776,
128.137978637021)) ;
#149396=CARTESIAN_POINT('Ctrl Pts',(-25.9044463776869,14.003146544252,128.253450200463)) ;
#149397=CARTESIAN_POINT('Ctrl Pts',(-25.9553220324677,14.2480984913921,
128.434908631351)) ;
#149398=CARTESIAN_POINT('Ctrl Pts',(-26.0258527600041,14.4370589151547,
128.67421395397)) ;
#149399=CARTESIAN_POINT('Ctrl Pts',(-26.1092792616536,14.5521322459825,
128.950981738852)) ;
#149400=CARTESIAN_POINT('Ctrl Pts',(-26.199596367935,14.5867077629414,129.248023960277)) ;
#149401=CARTESIAN_POINT('Ctrl Pts',(-26.2889097076484,14.5378478997284,
129.541988386777)) ;
#149402=CARTESIAN_POINT('Ctrl Pts',(-26.3706225884636,14.4092030440239,
129.813815833598)) ;
#149403=CARTESIAN_POINT('Ctrl Pts',(-26.4379731393695,14.2102655467961,
130.043646526883)) ;
#149404=CARTESIAN_POINT('Ctrl Pts',(-26.4856636420017,13.9531165249686,
130.216267974669)) ;
#149405=CARTESIAN_POINT('Ctrl Pts',(-26.5089520228723,13.6605445823028,
130.31728180732)) ;
#149406=CARTESIAN_POINT('Ctrl Pts',(-26.505983006858,13.3493860420966,130.341784421963)) ;
#149407=CARTESIAN_POINT('Ctrl Pts',(-26.4760795773027,13.0444136066678,
130.287498366656)) ;
#149408=CARTESIAN_POINT('Ctrl Pts',(-26.4205900967314,12.7658509592001,
130.158551123139)) ;
#149409=CARTESIAN_POINT('Ctrl Pts',(-26.3428502090789,12.5346699181632,
129.964569939688)) ;
#149410=CARTESIAN_POINT('Ctrl Pts',(-26.2475525447978,12.3668713397562,
129.719341661414)) ;
#149411=CARTESIAN_POINT('Ctrl Pts',(-26.1408738407262,12.2750736667704,
129.440865631469)) ;
#149412=CARTESIAN_POINT('Ctrl Pts',(-26.0303295842009,12.2654123740739,
129.150928666223)) ;
#149413=CARTESIAN_POINT('Ctrl Pts',(-25.9220058556232,12.338500075334,128.867642928314)) ;
#149414=CARTESIAN_POINT('Ctrl Pts',(-25.823580121359,12.4893940348924,128.613242211606)) ;
#149415=CARTESIAN_POINT('Ctrl Pts',(-25.7412693678322,12.7071834548376,
128.405922936625)) ;
#149416=CARTESIAN_POINT('Ctrl Pts',(-25.6802965616572,12.9760085814995,
128.26090587194)) ;
#149417=CARTESIAN_POINT('Ctrl Pts',(-25.6441923860615,13.2771670277102,
128.188575058199)) ;
#149418=CARTESIAN_POINT('Ctrl Pts',(-25.6348985777501,13.5885362669385,
128.194535927645)) ;
#149419=CARTESIAN_POINT('Ctrl Pts',(-25.6523328897567,13.8883473983697,
128.278609254777)) ;
#149420=CARTESIAN_POINT('Ctrl Pts',(-25.6945375325596,14.1546796544185,
128.435029104442)) ;
#149421=CARTESIAN_POINT('Ctrl Pts',(-25.7576722938783,14.3683944607912,
128.652558927551)) ;
#149422=CARTESIAN_POINT('Ctrl Pts',(-25.8365524919284,14.5146640106003,
128.916097753154)) ;
#149423=CARTESIAN_POINT('Ctrl Pts',(-25.9251110929857,14.5827891509108,
129.208019589231)) ;
#149424=CARTESIAN_POINT('Ctrl Pts',(-26.015573321456,14.5676066114005,129.505349333004)) ;
#149425=CARTESIAN_POINT('Ctrl Pts',(-26.1012556109092,14.4706131467255,
129.788764317248)) ;
#149426=CARTESIAN_POINT('Ctrl Pts',(-26.1751826362596,14.2987449409649,
130.037825229019)) ;
#149427=CARTESIAN_POINT('Ctrl Pts',(-26.231476999422,14.063095845739,130.235510412299)) ;
#149428=CARTESIAN_POINT('Ctrl Pts',(-26.2649721046301,13.783320877813,130.36636990385)) ;
#149429=CARTESIAN_POINT('Ctrl Pts',(-26.2729003428569,13.4754883561184,
130.422804556592)) ;
#149430=CARTESIAN_POINT('Ctrl Pts',(-26.2538588179999,13.1664273020677,
130.400169807561)) ;
#149431=CARTESIAN_POINT('Ctrl Pts',(-26.2084817055547,12.8743475374644,
130.30075703385)) ;
#149432=CARTESIAN_POINT('Ctrl Pts',(-26.1393771918487,12.6220180754337,
130.131968605388)) ;
#149433=CARTESIAN_POINT('Ctrl Pts',(-26.0504026601184,12.4263341505379,
129.905252967717)) ;
#149434=CARTESIAN_POINT('Ctrl Pts',(-25.947535881916,12.3026056588691,129.637908781085)) ;
#149435=CARTESIAN_POINT('Ctrl Pts',(-25.8376937080852,12.2593725245785,
129.350094272485)) ;
#149436=CARTESIAN_POINT('Ctrl Pts',(-25.7277681341655,12.2987734031186,
129.062003328986)) ;
#149437=CARTESIAN_POINT('Ctrl Pts',(-25.6238087024035,12.4202091784099,
128.791687112019)) ;
#149438=CARTESIAN_POINT('Ctrl Pts',(-25.5347909469648,12.6117736557302,
128.564597278483)) ;
#149439=CARTESIAN_POINT('Ctrl Pts',(-25.4644647312364,12.8626551517495,
128.392353071568)) ;
#149440=CARTESIAN_POINT('Ctrl Pts',(-25.4181059842558,13.1527448205317,
128.289985266207)) ;
#149441=CARTESIAN_POINT('Ctrl Pts',(-25.3978265921149,13.4624297632054,
128.26384262381)) ;
#149442=CARTESIAN_POINT('Ctrl Pts',(-25.4046046149136,13.7701810558333,
128.316837011734)) ;
#149443=CARTESIAN_POINT('Ctrl Pts',(-25.4370679406513,14.0517728078933,
128.444718605914)) ;
#149444=CARTESIAN_POINT('Ctrl Pts',(-25.4922811148997,14.2892526496134,
128.639150351661)) ;
#149445=CARTESIAN_POINT('Ctrl Pts',(-25.5658191040767,14.4648239971076,
128.887203395093)) ;
#149446=CARTESIAN_POINT('Ctrl Pts',(-25.6509413981458,14.5650402955601,
129.168902206863)) ;
#149447=CARTESIAN_POINT('Ctrl Pts',(-25.7416323438765,14.5837489624633,
129.467013900429)) ;
#149448=CARTESIAN_POINT('Ctrl Pts',(-25.8298583850632,14.5197168158782,
129.75773720294)) ;
#149449=CARTESIAN_POINT('Ctrl Pts',(-25.9096537578399,14.3763315271282,
130.024093124728)) ;
#149450=CARTESIAN_POINT('Ctrl Pts',(-25.973514050232,14.1656646034779,130.243682507277)) ;
#149451=CARTESIAN_POINT('Ctrl Pts',(-26.0168945296712,13.8999129369224,
130.403701320786)) ;
#149452=CARTESIAN_POINT('Ctrl Pts',(-26.0353238984872,13.6028236441132,
130.490484775464)) ;
#149453=CARTESIAN_POINT('Ctrl Pts',(-26.0272964629209,13.291184662554,130.500185473863)) ;
#149454=CARTESIAN_POINT('Ctrl Pts',(-25.9924298041082,12.9894031508225,
130.431429463874)) ;
#149455=CARTESIAN_POINT('Ctrl Pts',(-25.9323345518416,12.7177660513116,
130.289085423949)) ;
#149456=CARTESIAN_POINT('Ctrl Pts',(-25.8506637020188,12.4972590440602,
130.083685272878)) ;
#149457=CARTESIAN_POINT('Ctrl Pts',(-25.7532768706347,12.3438957808923,
129.832165172526)) ;
#149458=CARTESIAN_POINT('Ctrl Pts',(-25.6451767858764,12.2668705331881,
129.549560973497)) ;
#149459=CARTESIAN_POINT('Ctrl Pts',(-25.5342771990314,12.2729077976525,
129.258679649349)) ;
#149460=CARTESIAN_POINT('Ctrl Pts',(-25.4272944138605,12.3614501040313,
128.979314451413)) ;
#149461=CARTESIAN_POINT('Ctrl Pts',(-25.3316928534878,12.5253314471916,
128.733068601897)) ;
#149462=CARTESIAN_POINT('Ctrl Pts',(-25.2526702517292,12.7552769702176,
128.535519977571)) ;
#149463=CARTESIAN_POINT('Ctrl Pts',(-25.1963868103433,13.0310568986237,
128.404108114085)) ;
#149464=CARTESIAN_POINT('Ctrl Pts',(-25.1652356923081,13.3361216893249,
128.346276085526)) ;
#149465=CARTESIAN_POINT('Ctrl Pts',(-25.1610447906198,13.6463104400421,
128.367071713508)) ;
#149466=CARTESIAN_POINT('Ctrl Pts',(-25.1834279122032,13.9424873380838,
128.465719369502)) ;
#149467=CARTESIAN_POINT('Ctrl Pts',(-25.2300651046473,14.2002008792275,
128.63510490389)) ;
#149468=CARTESIAN_POINT('Ctrl Pts',(-25.2964021821312,14.4015262359145,
128.861882102586)) ;
#149469=CARTESIAN_POINT('Ctrl Pts',(-25.377774803287,14.5339054889456,129.132784185914)) ;
#149470=CARTESIAN_POINT('Ctrl Pts',(-25.4670176153515,14.5863178639959,
129.426586569099)) ;
#149471=CARTESIAN_POINT('Ctrl Pts',(-25.5575016604959,14.5553221796482,
129.724127530759)) ;
#149472=CARTESIAN_POINT('Ctrl Pts',(-25.6413823541268,14.4431215079252,
130.002261657312)) ;
#149473=CARTESIAN_POINT('Ctrl Pts',(-25.7121297022502,14.2589451950462,
130.241921219066)) ;
#149474=CARTESIAN_POINT('Ctrl Pts',(-25.7645376943468,14.0132050908334,
130.428265572224)) ;
#149475=CARTESIAN_POINT('Ctrl Pts',(-25.7934072860426,13.7264814717307,
130.545664324976)) ;
#149476=CARTESIAN_POINT('Ctrl Pts',(-25.7962481463893,13.4166671207193,
130.587186681068)) ;
#149477=CARTESIAN_POINT('Ctrl Pts',(-25.7721344714061,13.1090562113246,
130.549771064034)) ;
#149478=CARTESIAN_POINT('Ctrl Pts',(-25.721972342848,12.8228936758021,130.436381366975)) ;
#149479=CARTESIAN_POINT('Ctrl Pts',(-25.648887215864,12.5803482632518,130.255929141698)) ;
#149480=CARTESIAN_POINT('Ctrl Pts',(-25.5567250208858,12.3971382948885,
130.019928622796)) ;
#149481=CARTESIAN_POINT('Ctrl Pts',(-25.4521561710051,12.2881794831016,
129.747548587076)) ;
#149482=CARTESIAN_POINT('Ctrl Pts',(-25.341278028209,12.260444772771,129.45684395212)) ;
#149483=CARTESIAN_POINT('Ctrl Pts',(-25.2320854545694,12.3158800352752,
129.170914587755)) ;
#149484=CARTESIAN_POINT('Ctrl Pts',(-25.1307342445682,12.4512315889953,
128.908061261342)) ;
#149485=CARTESIAN_POINT('Ctrl Pts',(-25.0449098942256,12.6546809056087,
128.690298448963)) ;
#149486=CARTESIAN_POINT('Ctrl Pts',(-24.9787438302227,12.9147730695688,
128.53022636553)) ;
#149487=CARTESIAN_POINT('Ctrl Pts',(-24.9371546931072,13.2095558762223,
128.441731585585)) ;
#149488=CARTESIAN_POINT('Ctrl Pts',(-24.9219358688328,13.5223873446286,
128.430586778961)) ;
#149489=CARTESIAN_POINT('Ctrl Pts',(-24.9336416813406,13.8250174171808,
128.497741444582)) ;
#149490=CARTESIAN_POINT('Ctrl Pts',(-24.9709882879253,14.1019894892023,
128.640183490629)) ;
#149491=CARTESIAN_POINT('Ctrl Pts',(-25.0298178161762,14.3273312033298,
128.844994185111)) ;
#149492=CARTESIAN_POINT('Ctrl Pts',(-25.10580372417,14.4893435077641,129.10009070675)) ;
#149493=CARTESIAN_POINT('Ctrl Pts',(-25.1925946679685,14.5749599942803,
129.386728128292)) ;
#149494=CARTESIAN_POINT('Ctrl Pts',(-25.2836420775207,14.5779281388509,
129.685942527895)) ;
#149495=CARTESIAN_POINT('Ctrl Pts',(-25.3707009485329,14.498336569716,129.973274291318)) ;
#149496=CARTESIAN_POINT('Ctrl Pts',(-25.4477523301807,14.3420896850988,
130.231459883249)) ;
#149497=CARTESIAN_POINT('Ctrl Pts',(-25.5085283667888,14.1180212398974,
130.442336334764)) ;
#149498=CARTESIAN_POINT('Ctrl Pts',(-25.5470625789099,13.8471809568527,
130.587829774937)) ;
#149499=CARTESIAN_POINT('Ctrl Pts',(-25.5607996567635,13.5439414016218,
130.66115301931)) ;
#149500=CARTESIAN_POINT('Ctrl Pts',(-25.5476548595395,13.2331635587154,
130.655809870217)) ;
#149501=CARTESIAN_POINT('Ctrl Pts',(-25.5076848410153,12.9343809245396,
130.5722927305)) ;
#149502=CARTESIAN_POINT('Ctrl Pts',(-25.4434208273164,12.6721978750302,
130.417619951137)) ;
#149503=CARTESIAN_POINT('Ctrl Pts',(-25.3584430705461,12.4632419957696,
130.202508041582)) ;
#149504=CARTESIAN_POINT('Ctrl Pts',(-25.25839433447,12.3231158873288,129.943303971723)) ;
#149505=CARTESIAN_POINT('Ctrl Pts',(-25.1488417963276,12.2616017925994,
129.656547762908)) ;
#149506=CARTESIAN_POINT('Ctrl Pts',(-25.038684912235,12.2833201710628,129.367682393325)) ;
#149507=CARTESIAN_POINT('Ctrl Pts',(-24.9329793112531,12.3868877150975,
129.092131865543)) ;
#149508=CARTESIAN_POINT('Ctrl Pts',(-24.8399384850518,12.5648231149356,
128.853474687072)) ;
#149509=CARTESIAN_POINT('Ctrl Pts',(-24.7652402822907,12.8039601972563,
128.668370041775)) ;
#149510=CARTESIAN_POINT('Ctrl Pts',(-24.7134183488315,13.0864728883471,
128.549995424853)) ;
#149511=CARTESIAN_POINT('Ctrl Pts',(-24.6872157946094,13.395723837035,128.506754165196)) ;
#149512=CARTESIAN_POINT('Ctrl Pts',(-24.6881919566604,13.7038340403903,
128.542568479247)) ;
#149513=CARTESIAN_POINT('Ctrl Pts',(-24.715198213589,13.9936201443638,128.654601982)) ;
#149514=CARTESIAN_POINT('Ctrl Pts',(-24.766143048851,14.2431366577781,128.836696575373)) ;
#149515=CARTESIAN_POINT('Ctrl Pts',(-24.8355233115694,14.4318623943572,
129.072286946739)) ;
#149516=CARTESIAN_POINT('Ctrl Pts',(-24.9191764312831,14.5502397442867,
129.349948983629)) ;
#149517=CARTESIAN_POINT('Ctrl Pts',(-25.009185749029,14.5868194741509,129.645997652474)) ;
#149518=CARTESIAN_POINT('Ctrl Pts',(-25.0987232119014,14.5403267808585,
129.940661741851)) ;
#149519=CARTESIAN_POINT('Ctrl Pts',(-25.1807290894155,14.4138414992085,
130.213331551178)) ;
#149520=CARTESIAN_POINT('Ctrl Pts',(-25.2485825472388,14.2163547115684,
130.444669381933)) ;
#149521=CARTESIAN_POINT('Ctrl Pts',(-25.2966444415633,13.9624648084783,
130.618145353059)) ;
#149522=CARTESIAN_POINT('Ctrl Pts',(-25.3208833248344,13.6693367941651,
130.722106531436)) ;
#149523=CARTESIAN_POINT('Ctrl Pts',(-25.3186739748594,13.3586798877786,
130.748788087223)) ;
#149524=CARTESIAN_POINT('Ctrl Pts',(-25.2895027866024,13.0526930051948,
130.696702454147)) ;
#149525=CARTESIAN_POINT('Ctrl Pts',(-25.2346977316742,12.7731728607976,
130.569743521304)) ;
#149526=CARTESIAN_POINT('Ctrl Pts',(-25.1575260769634,12.5404162495143,
130.37742441001)) ;
#149527=CARTESIAN_POINT('Ctrl Pts',(-25.0627516347693,12.3707608334166,
130.133688280252)) ;
#149528=CARTESIAN_POINT('Ctrl Pts',(-24.9563296046017,12.2766729754023,
129.855958777249)) ;
#149529=CARTESIAN_POINT('Ctrl Pts',(-24.8458555258651,12.2643218379507,
129.566208802592)) ;
#149530=CARTESIAN_POINT('Ctrl Pts',(-24.7365680360254,12.3360206173623,
129.280361704469)) ;
#149531=CARTESIAN_POINT('Ctrl Pts',(-24.6387085221223,12.4836396452835,
129.02730656166)) ;
#149532=CARTESIAN_POINT('Ctrl Pts',(-24.5554652249711,12.7003318361734,
128.817398714957)) ;
#149533=CARTESIAN_POINT('Ctrl Pts',(-24.4939102279339,12.9678916740203,
128.67065729352)) ;
#149534=CARTESIAN_POINT('Ctrl Pts',(-24.4570242893103,13.2687868226262,
128.596084011808)) ;
#149535=CARTESIAN_POINT('Ctrl Pts',(-24.4470222252909,13.5800033962545,
128.599957819028)) ;
#149536=CARTESIAN_POINT('Ctrl Pts',(-24.4636781049398,13.8799728738773,
128.681703631968)) ;
#149537=CARTESIAN_POINT('Ctrl Pts',(-24.5052266831448,14.1476993247652,
128.836224797639)) ;
#149538=CARTESIAN_POINT('Ctrl Pts',(-24.5678445404094,14.3632524005006,
129.052255584623)) ;
#149539=CARTESIAN_POINT('Ctrl Pts',(-24.6466140551618,14.5119335521308,
129.315568097717)) ;
#149540=CARTESIAN_POINT('Ctrl Pts',(-24.7349394738753,14.5819602078055,
129.606776733132)) ;
#149541=CARTESIAN_POINT('Ctrl Pts',(-24.8251551713637,14.5692454474693,
129.903283329894)) ;
#149542=CARTESIAN_POINT('Ctrl Pts',(-24.9112782216652,14.4742855004693,
130.188065709167)) ;
#149543=CARTESIAN_POINT('Ctrl Pts',(-24.9854145282877,14.3047439678629,
130.437652687695)) ;
#149544=CARTESIAN_POINT('Ctrl Pts',(-25.0423106791957,14.0710831645145,
130.63706527833)) ;
#149545=CARTESIAN_POINT('Ctrl Pts',(-25.0765997942413,13.7914036967699,
130.770354473467)) ;
#149546=CARTESIAN_POINT('Ctrl Pts',(-25.0852494656584,13.4850123615767,
130.828786595683)) ;
#149547=CARTESIAN_POINT('Ctrl Pts',(-25.0670539308989,13.1755844342699,
130.808639517333)) ;
#149548=CARTESIAN_POINT('Ctrl Pts',(-25.0223515514235,12.8823157939158,
130.71123929387)) ;
#149549=CARTESIAN_POINT('Ctrl Pts',(-24.953889165623,12.6284363118315,130.544332688521)) ;
#149550=CARTESIAN_POINT('Ctrl Pts',(-24.8649952863517,12.430459524885,130.31798174757)) ;
#149551=CARTESIAN_POINT('Ctrl Pts',(-24.7632620671208,12.3053999545834,
130.053682988785)) ;
#149552=CARTESIAN_POINT('Ctrl Pts',(-24.6526433526302,12.259348439198,129.763874618342)) ;
#149553=CARTESIAN_POINT('Ctrl Pts',(-24.543147783903,12.2965483927982,129.476879582069)) ;
#149554=CARTESIAN_POINT('Ctrl Pts',(-24.4388189231228,12.4156949329505,
129.205508703888)) ;
#149555=CARTESIAN_POINT('Ctrl Pts',(-24.3494211561216,12.6050470822163,
128.97725948019)) ;
#149556=CARTESIAN_POINT('Ctrl Pts',(-24.2782871788887,12.8553420961893,
128.802763975287)) ;
#149557=CARTESIAN_POINT('Ctrl Pts',(-24.2314133234197,13.1429454488516,
128.698707201268)) ;
#149558=CARTESIAN_POINT('Ctrl Pts',(-24.2101989369583,13.454391681807,128.670054503265)) ;
#149559=CARTESIAN_POINT('Ctrl Pts',(-24.2162621143245,13.7614619706277,
128.720842820947)) ;
#149560=CARTESIAN_POINT('Ctrl Pts',(-24.2480829792965,14.0447127899292,
128.846925564753)) ;
#149561=CARTESIAN_POINT('Ctrl Pts',(-24.3026006806666,14.2828872647388,
129.039230695789)) ;
#149562=CARTESIAN_POINT('Ctrl Pts',(-24.3753681458238,14.4603132079677,
129.284922796906)) ;
#149563=CARTESIAN_POINT('Ctrl Pts',(-24.4609023941818,14.5634617296136,
129.568084681882)) ;
#149564=CARTESIAN_POINT('Ctrl Pts',(-24.5508494400508,14.5844329944993,
129.863760728172)) ;
#149565=CARTESIAN_POINT('Ctrl Pts',(-24.639839531071,14.5225343745256,130.156946138094)) ;
#149566=CARTESIAN_POINT('Ctrl Pts',(-24.7197008453795,14.3815448921276,
130.423379851621)) ;
#149567=CARTESIAN_POINT('Ctrl Pts',(-24.7841346291663,14.1725755942996,
130.644670202512)) ;
#149568=CARTESIAN_POINT('Ctrl Pts',(-24.8280424045697,13.9093042080622,
130.806088923475)) ;
#149569=CARTESIAN_POINT('Ctrl Pts',(-24.8474183136767,13.6121560169538,
130.89573531851)) ;
#149570=CARTESIAN_POINT('Ctrl Pts',(-24.8400459886506,13.2990172973707,
130.907513124008)) ;
#149571=CARTESIAN_POINT('Ctrl Pts',(-24.8060258678097,12.9981567008458,
130.841072315911)) ;
#149572=CARTESIAN_POINT('Ctrl Pts',(-24.7468166542393,12.7257034100229,
130.701255434815)) ;
#149573=CARTESIAN_POINT('Ctrl Pts',(-24.6656622236315,12.503075938083,130.497401491787)) ;
#149574=CARTESIAN_POINT('Ctrl Pts',(-24.5684692840645,12.3471530516957,
130.246518289706)) ;
#149575=CARTESIAN_POINT('Ctrl Pts',(-24.4601592445073,12.2678408813101,
129.963418414353)) ;
#149576=CARTESIAN_POINT('Ctrl Pts',(-24.3498913902178,12.2715868988579,
129.674190683696)) ;
#149577=CARTESIAN_POINT('Ctrl Pts',(-24.2425522782409,12.3575775425478,
129.39381841984)) ;
#149578=CARTESIAN_POINT('Ctrl Pts',(-24.1463896718838,12.519859116392,129.145996967163)) ;
#149579=CARTESIAN_POINT('Ctrl Pts',(-24.0670162200056,12.7472699624983,
128.947309088182)) ;
#149580=CARTESIAN_POINT('Ctrl Pts',(-24.0097627776868,13.0233713370029,
128.813237370851)) ;
#149581=CARTESIAN_POINT('Ctrl Pts',(-23.9780360421946,13.3264774087469,
128.753559775016)) ;
#149582=CARTESIAN_POINT('Ctrl Pts',(-23.972984735808,13.6374828083211,128.771916902171)) ;
#149583=CARTESIAN_POINT('Ctrl Pts',(-23.9946301893743,13.9340521911672,
128.868370985109)) ;
#149584=CARTESIAN_POINT('Ctrl Pts',(-24.0404917441425,14.193123894667,129.035463808342)) ;
#149585=CARTESIAN_POINT('Ctrl Pts',(-24.1068147894344,14.3974304405376,
129.262422211174)) ;
#149586=CARTESIAN_POINT('Ctrl Pts',(-24.1873859593662,14.5309245304013,
129.530773973435)) ;
#149587=CARTESIAN_POINT('Ctrl Pts',(-24.2765414629164,14.5859814529116,
129.824348558805)) ;
#149588=CARTESIAN_POINT('Ctrl Pts',(-24.3669136839927,14.5574777921035,
130.12149550496)) ;
#149589=CARTESIAN_POINT('Ctrl Pts',(-24.4511409095846,14.4480150679812,
130.400638885907)) ;
#149590=CARTESIAN_POINT('Ctrl Pts',(-24.5228192659594,14.2640747016683,
130.643277300762)) ;
#149591=CARTESIAN_POINT('Ctrl Pts',(-24.5753535527293,14.0222278748094,
130.829662909355)) ;
#149592=CARTESIAN_POINT('Ctrl Pts',(-24.6052393635017,13.7339092268223,
130.950338760758)) ;
#149593=CARTESIAN_POINT('Ctrl Pts',(-24.6087423113482,13.4264443315917,
130.993564327821)) ;
#149594=CARTESIAN_POINT('Ctrl Pts',(-24.5854552385146,13.117933729061,130.958630105936)) ;
#149595=CARTESIAN_POINT('Ctrl Pts',(-24.5360542246663,12.8308236543942,
130.847449580538)) ;
#149596=CARTESIAN_POINT('Ctrl Pts',(-24.4632259609744,12.5859821244952,
130.667884994936)) ;
#149597=CARTESIAN_POINT('Ctrl Pts',(-24.3721859047241,12.4020104693658,
130.434925127817)) ;
#149598=CARTESIAN_POINT('Ctrl Pts',(-24.2672388487678,12.2899875702474,
130.161658393472)) ;
#149599=CARTESIAN_POINT('Ctrl Pts',(-24.1570061952322,12.2601247777389,
129.872660322031)) ;
#149600=CARTESIAN_POINT('Ctrl Pts',(-24.0474842604457,12.3130228920766,
129.585829133635)) ;
#149601=CARTESIAN_POINT('Ctrl Pts',(-23.9459955773779,12.4457555265159,
129.322497926636)) ;
#149602=CARTESIAN_POINT('Ctrl Pts',(-23.8593193186365,12.6478748445304,
129.102358913556)) ;
#149603=CARTESIAN_POINT('Ctrl Pts',(-23.7923711383799,12.90742344953,128.940087473062)) ;
#149604=CARTESIAN_POINT('Ctrl Pts',(-23.7501513912619,13.2015878623563,
128.849756858677)) ;
#149605=CARTESIAN_POINT('Ctrl Pts',(-23.7341995328484,13.513246132059,128.83635605202)) ;
#149606=CARTESIAN_POINT('Ctrl Pts',(-23.7452242106922,13.8170403560637,
128.901601785867)) ;
#149607=CARTESIAN_POINT('Ctrl Pts',(-23.7815365397005,14.0930903285622,
129.040762499699)) ;
#149608=CARTESIAN_POINT('Ctrl Pts',(-23.8399631313571,14.3215764376153,
129.244564779432)) ;
#149609=CARTESIAN_POINT('Ctrl Pts',(-23.9158125493605,14.4860163871687,
129.499361949974)) ;
#149610=CARTESIAN_POINT('Ctrl Pts',(-24.0024884712054,14.5737421831593,
129.785693667344)) ;
#149611=CARTESIAN_POINT('Ctrl Pts',(-24.0932764888338,14.5789283519424,
130.084061847356)) ;
#149612=CARTESIAN_POINT('Ctrl Pts',(-24.1805810257139,14.5018180781457,
130.372118460608)) ;
#149613=CARTESIAN_POINT('Ctrl Pts',(-24.2582426096159,14.3465572138388,
130.632227060123)) ;
#149614=CARTESIAN_POINT('Ctrl Pts',(-24.318922055871,14.1268975859946,130.842432120294)) ;
#149615=CARTESIAN_POINT('Ctrl Pts',(-24.3585878491517,13.8551173333083,
130.991522309819)) ;
#149616=CARTESIAN_POINT('Ctrl Pts',(-24.3729811727422,13.5530514979448,
131.066681273596)) ;
#149617=CARTESIAN_POINT('Ctrl Pts',(-24.3605810853974,13.2415865700778,
131.063587579124)) ;
#149618=CARTESIAN_POINT('Ctrl Pts',(-24.3215051289014,12.9431698181064,
130.982558898571)) ;
#149619=CARTESIAN_POINT('Ctrl Pts',(-24.2577823597366,12.6789857022783,
130.82955143097)) ;
#149620=CARTESIAN_POINT('Ctrl Pts',(-24.1734213941347,12.4685394355876,
130.616198443188)) ;
#149621=CARTESIAN_POINT('Ctrl Pts',(-24.073742301987,12.3261975065515,130.358076220312)) ;
#149622=CARTESIAN_POINT('Ctrl Pts',(-23.964425817923,12.2622045944374,130.07198593286)) ;
#149623=CARTESIAN_POINT('Ctrl Pts',(-23.85400734296,12.2815898104216,129.782422227761)) ;
#149624=CARTESIAN_POINT('Ctrl Pts',(-23.7483648318689,12.3824517320663,
129.506948722711)) ;
#149625=CARTESIAN_POINT('Ctrl Pts',(-23.6547176816251,12.5585396445524,
129.266575329298)) ;
#149626=CARTESIAN_POINT('Ctrl Pts',(-23.5794496136605,12.7954954473237,
129.079743076793)) ;
#149627=CARTESIAN_POINT('Ctrl Pts',(-23.5265530513227,13.0796939722615,
128.958534945504)) ;
#149628=CARTESIAN_POINT('Ctrl Pts',(-23.4998982470055,13.3852304092896,
128.913605172704)) ;
#149629=CARTESIAN_POINT('Ctrl Pts',(-23.4999888970711,13.6960444391784,
128.947097240951)) ;
#149630=CARTESIAN_POINT('Ctrl Pts',(-23.5263685356686,13.9858667251667,
129.057221274521)) ;
#149631=CARTESIAN_POINT('Ctrl Pts',(-23.5763701013332,14.2358877354541,
129.236412760875)) ;
#149632=CARTESIAN_POINT('Ctrl Pts',(-23.6455558699911,14.427599936546,129.471589612086)) ;
#149633=CARTESIAN_POINT('Ctrl Pts',(-23.7290651686037,14.5480862875162,
129.748875677401)) ;
#149634=CARTESIAN_POINT('Ctrl Pts',(-23.8186690168967,14.5868446714445,
130.043626720831)) ;
#149635=CARTESIAN_POINT('Ctrl Pts',(-23.9082230495936,14.543035766912,130.338299611746)) ;
#149636=CARTESIAN_POINT('Ctrl Pts',(-23.9906596269093,14.4187440233768,
130.61226747632)) ;
#149637=CARTESIAN_POINT('Ctrl Pts',(-24.0590906655054,14.2230681699305,
130.845316199776)) ;
#149638=CARTESIAN_POINT('Ctrl Pts',(-24.1078676594404,13.9697197802327,
131.020979313656)) ;
#149639=CARTESIAN_POINT('Ctrl Pts',(-24.1327346146683,13.678752384422,131.126622427397)) ;
#149640=CARTESIAN_POINT('Ctrl Pts',(-24.1313280770406,13.3668523493994,
131.155805587828)) ;
#149641=CARTESIAN_POINT('Ctrl Pts',(-24.1028121227854,13.0606725524935,
131.10561289289)) ;
#149642=CARTESIAN_POINT('Ctrl Pts',(-24.0489129518643,12.7810811870564,
130.981183215495)) ;
#149643=CARTESIAN_POINT('Ctrl Pts',(-23.9723802111595,12.5467078049701,
130.790724008006)) ;
#149644=CARTESIAN_POINT('Ctrl Pts',(-23.878243975613,12.3750360916392,130.548796694559)) ;
#149645=CARTESIAN_POINT('Ctrl Pts',(-23.7714355652821,12.2779852659618,
130.270134963112)) ;
#149646=CARTESIAN_POINT('Ctrl Pts',(-23.6611435021707,12.2637459415924,
129.980872210853)) ;
#149647=CARTESIAN_POINT('Ctrl Pts',(-23.5523935290098,12.3321871278704,
129.696367849268)) ;
#149648=CARTESIAN_POINT('Ctrl Pts',(-23.4532846730256,12.4786899197398,
129.439942969293)) ;
#149649=CARTESIAN_POINT('Ctrl Pts',(-23.369577036012,12.6941597985184,129.228694490344)) ;
#149650=CARTESIAN_POINT('Ctrl Pts',(-23.3076081758044,12.95948963943,129.0806195286)) ;
#149651=CARTESIAN_POINT('Ctrl Pts',(-23.2699369429155,13.2597800757016,
129.003760027813)) ;
#149652=CARTESIAN_POINT('Ctrl Pts',(-23.259151387003,13.570593176475,129.005303519991)) ;
#149653=CARTESIAN_POINT('Ctrl Pts',(-23.2750101957861,13.8717553022586,
129.084772659304)) ;
#149654=CARTESIAN_POINT('Ctrl Pts',(-23.3161725222393,14.1416795276356,
129.238312148315)) ;
#149655=CARTESIAN_POINT('Ctrl Pts',(-23.3778830225391,14.3575207602719,
129.451480700559)) ;
#149656=CARTESIAN_POINT('Ctrl Pts',(-23.456487612726,14.5088742129947,129.714415384989)) ;
#149657=CARTESIAN_POINT('Ctrl Pts',(-23.5444425261219,14.5810485747374,
130.004461283364)) ;
#149658=CARTESIAN_POINT('Ctrl Pts',(-23.6348221144792,14.5707018423974,
130.301503634973)) ;
#149659=CARTESIAN_POINT('Ctrl Pts',(-23.720929050143,14.4785663086567,130.58612695697)) ;
#149660=CARTESIAN_POINT('Ctrl Pts',(-23.796091874448,14.3096046901172,130.838988013443)) ;
#149661=CARTESIAN_POINT('Ctrl Pts',(-23.8532786750127,14.0777450848623,
131.039159906717)) ;
#149662=CARTESIAN_POINT('Ctrl Pts',(-23.8881290823669,13.8001342656759,
131.173975253073)) ;
#149663=CARTESIAN_POINT('Ctrl Pts',(-23.8976235031685,13.4946153798022,
131.234832161425)) ;
#149664=CARTESIAN_POINT('Ctrl Pts',(-23.8801038719591,13.1837407483122,
131.216799463619)) ;
#149665=CARTESIAN_POINT('Ctrl Pts',(-23.8362104970674,12.8901082923596,
131.121701071398)) ;
#149666=CARTESIAN_POINT('Ctrl Pts',(-23.7678922757388,12.6339161097821,
130.955392278708)) ;
#149667=CARTESIAN_POINT('Ctrl Pts',(-23.6807913010125,12.43659258656,130.733805167857)) ;
#149668=CARTESIAN_POINT('Ctrl Pts',(-23.5782209974731,12.3075969650438,
130.467461898583)) ;
#149669=CARTESIAN_POINT('Ctrl Pts',(-23.4687021830052,12.25954136932,130.18055487232)) ;
#149670=CARTESIAN_POINT('Ctrl Pts',(-23.3580959689389,12.2945981234014,
129.890635929431)) ;
#149671=CARTESIAN_POINT('Ctrl Pts',(-23.2545594842742,12.4101972587338,
129.621216465596)) ;
#149672=CARTESIAN_POINT('Ctrl Pts',(-23.1639430593023,12.5987159490307,
129.38966556076)) ;
#149673=CARTESIAN_POINT('Ctrl Pts',(-23.0924891951647,12.8461743758197,
129.214054201236)) ;
#149674=CARTESIAN_POINT('Ctrl Pts',(-23.044410224878,13.135926237231,129.1068328996)) ;
#149675=CARTESIAN_POINT('Ctrl Pts',(-23.0226954450076,13.4447581443412,
129.076453559591)) ;
#149676=CARTESIAN_POINT('Ctrl Pts',(-23.0279406480016,13.7530929006016,
129.124954375836)) ;
#149677=CARTESIAN_POINT('Ctrl Pts',(-23.0589188674744,14.0362080227333,
129.248437506434)) ;
#149678=CARTESIAN_POINT('Ctrl Pts',(-23.1129427190555,14.2769559751065,
129.43941471817)) ;
#149679=CARTESIAN_POINT('Ctrl Pts',(-23.1854563521041,14.4563581668246,
129.684422602972)) ;
#149680=CARTESIAN_POINT('Ctrl Pts',(-23.2701501049664,14.5613193380967,
129.964912349614)) ;
#149681=CARTESIAN_POINT('Ctrl Pts',(-23.3606421210985,14.5851466782009,
130.262402055223)) ;
#149682=CARTESIAN_POINT('Ctrl Pts',(-23.4498301224202,14.5250094575114,
130.556196196659)) ;
#149683=CARTESIAN_POINT('Ctrl Pts',(-23.5296219906433,14.3871119607425,
130.822238990892)) ;
#149684=CARTESIAN_POINT('Ctrl Pts',(-23.594925658701,14.1786614290351,131.046268453031)) ;
#149685=CARTESIAN_POINT('Ctrl Pts',(-23.6392653935183,13.9181922877867,
131.208752582989)) ;
#149686=CARTESIAN_POINT('Ctrl Pts',(-23.659486219196,13.6189924395308,131.301176945121)) ;
#149687=CARTESIAN_POINT('Ctrl Pts',(-23.6528706435111,13.3089362850498,
131.314836717611)) ;
#149688=CARTESIAN_POINT('Ctrl Pts',(-23.6195413006821,13.0058326835249,
131.250594746638)) ;
#149689=CARTESIAN_POINT('Ctrl Pts',(-23.5607526391566,12.7318653591864,
131.112071177331)) ;
#149690=CARTESIAN_POINT('Ctrl Pts',(-23.4802503319466,12.5082427552374,
130.910055459354)) ;
#149691=CARTESIAN_POINT('Ctrl Pts',(-23.3837706397875,12.3508733005898,
130.661144170979)) ;
#149692=CARTESIAN_POINT('Ctrl Pts',(-23.2760281567671,12.269103663372,130.379599385189)) ;
#149693=CARTESIAN_POINT('Ctrl Pts',(-23.1652080396249,12.2702137118359,
130.088920070481)) ;
#149694=CARTESIAN_POINT('Ctrl Pts',(-23.0575184300557,12.3542929443511,
129.807572897361)) ;
#149695=CARTESIAN_POINT('Ctrl Pts',(-22.9612440374846,12.5141175803543,
129.559330205376)) ;
#149696=CARTESIAN_POINT('Ctrl Pts',(-22.8813580521407,12.7395233280602,
129.359110706345)) ;
#149697=CARTESIAN_POINT('Ctrl Pts',(-22.8233745273822,13.0142278391015,
129.222887167103)) ;
#149698=CARTESIAN_POINT('Ctrl Pts',(-22.7907608487807,13.3177661715459,
129.160724179542)) ;
#149699=CARTESIAN_POINT('Ctrl Pts',(-22.7849933023356,13.6286636556953,
129.176966985141)) ;
#149700=CARTESIAN_POINT('Ctrl Pts',(-22.8057875541623,13.925291797829,129.270850522391)) ;
#149701=CARTESIAN_POINT('Ctrl Pts',(-22.8510343106894,14.1860949206715,
129.436195197481)) ;
#149702=CARTESIAN_POINT('Ctrl Pts',(-22.9165695111379,14.3917323897328,
129.6607396938)) ;
#149703=CARTESIAN_POINT('Ctrl Pts',(-22.9971196771895,14.5282787292637,
129.929178676751)) ;
#149704=CARTESIAN_POINT('Ctrl Pts',(-23.0863190684493,14.5855538686264,
130.222941810588)) ;
#149705=CARTESIAN_POINT('Ctrl Pts',(-23.1764960201686,14.5594424276329,
130.519424297724)) ;
#149706=CARTESIAN_POINT('Ctrl Pts',(-23.260922733227,14.4525338463175,130.799116406476)) ;
#149707=CARTESIAN_POINT('Ctrl Pts',(-23.3332076886336,14.2704302035547,
131.043574251826)) ;
#149708=CARTESIAN_POINT('Ctrl Pts',(-23.3863890212945,14.0294404893197,
131.23192060155)) ;
#149709=CARTESIAN_POINT('Ctrl Pts',(-23.4168682308191,13.7439522566763,
131.354120127472)) ;
#149710=CARTESIAN_POINT('Ctrl Pts',(-23.4212510479879,13.4354033012877,
131.400078141052)) ;
#149711=CARTESIAN_POINT('Ctrl Pts',(-23.3987589168995,13.1268757860435,
131.367427280398)) ;
#149712=CARTESIAN_POINT('Ctrl Pts',(-23.3498917515074,12.8380942311381,
131.257906778931)) ;
#149713=CARTESIAN_POINT('Ctrl Pts',(-23.2781287469993,12.593020734814,131.081261436538)) ;
#149714=CARTESIAN_POINT('Ctrl Pts',(-23.1869981180015,12.406038864334,130.848244567597)) ;
#149715=CARTESIAN_POINT('Ctrl Pts',(-23.0832130154599,12.2925312393263,
130.578091002702)) ;
#149716=CARTESIAN_POINT('Ctrl Pts',(-22.9721460034913,12.2597001756507,
130.286938563817)) ;
#149717=CARTESIAN_POINT('Ctrl Pts',(-22.8627372801265,12.3104428480306,
130.000362594001)) ;
#149718=CARTESIAN_POINT('Ctrl Pts',(-22.7608153842907,12.4411375343228,
129.735804833059)) ;
#149719=CARTESIAN_POINT('Ctrl Pts',(-22.6738551041291,12.6410412260459,
129.514759298238)) ;
#149720=CARTESIAN_POINT('Ctrl Pts',(-22.6062140340479,12.8990709412412,
129.350458683346)) ;
#149721=CARTESIAN_POINT('Ctrl Pts',(-22.563180860829,13.1932158422951,129.257833604546)) ;
#149722=CARTESIAN_POINT('Ctrl Pts',(-22.5465084812916,13.5039483153196,
129.242243533921)) ;
#149723=CARTESIAN_POINT('Ctrl Pts',(-22.5567390519965,13.8084629331276,
129.305193170766)) ;
#149724=CARTESIAN_POINT('Ctrl Pts',(-22.5923567807548,14.0856214522983,
129.442322762653)) ;
#149725=CARTESIAN_POINT('Ctrl Pts',(-22.6502043847312,14.3156973723363,
129.644432208859)) ;
#149726=CARTESIAN_POINT('Ctrl Pts',(-22.7254796481943,14.4820692516826,
129.897492489586)) ;
#149727=CARTESIAN_POINT('Ctrl Pts',(-22.8120983348714,14.5722583226928,
130.183725983055)) ;
#149728=CARTESIAN_POINT('Ctrl Pts',(-22.9024146711451,14.5801737014987,
130.480544456833)) ;
#149729=CARTESIAN_POINT('Ctrl Pts',(-22.9905600558702,14.5050114292979,
130.771303640142)) ;
#149730=CARTESIAN_POINT('Ctrl Pts',(-23.0683259692311,14.3522166044366,
131.031600216903)) ;
#149731=CARTESIAN_POINT('Ctrl Pts',(-23.1296712033648,14.1339604328417,
131.243810544313)) ;
#149732=CARTESIAN_POINT('Ctrl Pts',(-23.1699417301646,13.8641114718027,
131.394578383652)) ;
#149733=CARTESIAN_POINT('Ctrl Pts',(-23.1851714520848,13.5616227135085,
131.472298291736)) ;
#149734=CARTESIAN_POINT('Ctrl Pts',(-23.1735168490952,13.2502936297686,
131.47135922614)) ;
#149735=CARTESIAN_POINT('Ctrl Pts',(-23.1351157903928,12.9509784394827,
131.392333342699)) ;
#149736=CARTESIAN_POINT('Ctrl Pts',(-23.0722677645441,12.6863950306147,
131.241771426111)) ;
#149737=CARTESIAN_POINT('Ctrl Pts',(-22.9882746146552,12.4734607184327,
131.029576395243)) ;
#149738=CARTESIAN_POINT('Ctrl Pts',(-22.8884966331246,12.3287824290801,
130.771297011611)) ;
#149739=CARTESIAN_POINT('Ctrl Pts',(-22.7798708475332,12.2629634188969,
130.487058336271)) ;
#149740=CARTESIAN_POINT('Ctrl Pts',(-22.6692239157049,12.2798963089147,
130.196884376816)) ;
#149741=CARTESIAN_POINT('Ctrl Pts',(-22.5632797991812,12.3786943596861,
129.920548149089)) ;
#149742=CARTESIAN_POINT('Ctrl Pts',(-22.4691047373813,12.5532636786749,
129.678681828688)) ;
#149743=CARTESIAN_POINT('Ctrl Pts',(-22.3936121882583,12.7879391419199,
129.491068858609)) ;
#149744=CARTESIAN_POINT('Ctrl Pts',(-22.3401335624516,13.0695370930121,
129.367998395707)) ;
#149745=CARTESIAN_POINT('Ctrl Pts',(-22.3124627686297,13.3764286772832,
129.32029580838)) ;
#149746=CARTESIAN_POINT('Ctrl Pts',(-22.3118479090046,13.6873693589622,
129.351715741832)) ;
#149747=CARTESIAN_POINT('Ctrl Pts',(-22.3374491968515,13.9780097335569,
129.459554831409)) ;
#149748=CARTESIAN_POINT('Ctrl Pts',(-22.3870967384103,14.2303816852456,
129.637852506658)) ;
#149749=CARTESIAN_POINT('Ctrl Pts',(-22.4556103846514,14.4229832269157,
129.870941575462)) ;
#149750=CARTESIAN_POINT('Ctrl Pts',(-22.5386005193327,14.5456071990929,
130.146637869672)) ;
#149751=CARTESIAN_POINT('Ctrl Pts',(-22.6282642571968,14.5869244372619,
130.441623746508)) ;
#149752=CARTESIAN_POINT('Ctrl Pts',(-22.7179879086847,14.545413997822,130.736814107986)) ;
#149753=CARTESIAN_POINT('Ctrl Pts',(-22.8007463302778,14.4231615321001,
131.011735541558)) ;
#149754=CARTESIAN_POINT('Ctrl Pts',(-22.8694507154982,14.2299646068936,
131.245482052944)) ;
#149755=CARTESIAN_POINT('Ctrl Pts',(-22.918951836608,13.9782380541428,131.423258260038)) ;
#149756=CARTESIAN_POINT('Ctrl Pts',(-22.9445965328865,13.6869897055948,
131.531296852322)) ;
#149757=CARTESIAN_POINT('Ctrl Pts',(-22.943990289379,13.3772462796711,131.562611149052)) ;
#149758=CARTESIAN_POINT('Ctrl Pts',(-22.9163803749009,13.0701027009942,
131.515113736096)) ;
#149759=CARTESIAN_POINT('Ctrl Pts',(-22.8629756360469,12.7883758458207,
131.392255641816)) ;
#149760=CARTESIAN_POINT('Ctrl Pts',(-22.7870243908306,12.5524788761833,
131.203489638896)) ;
#149761=CARTESIAN_POINT('Ctrl Pts',(-22.693119134411,12.3787206471269,130.962295345711)) ;
#149762=CARTESIAN_POINT('Ctrl Pts',(-22.5872002079186,12.2799428632339,
130.686031470634)) ;
#149763=CARTESIAN_POINT('Ctrl Pts',(-22.4767054930379,12.262781436098,130.396251358911)) ;
#149764=CARTESIAN_POINT('Ctrl Pts',(-22.3671975211959,12.3295043869385,
130.109715154456)) ;
#149765=CARTESIAN_POINT('Ctrl Pts',(-22.2682597339845,12.473510372606,129.853632818829)) ;
#149766=CARTESIAN_POINT('Ctrl Pts',(-22.1842913044772,12.6859034724392,
129.641472948318)) ;
#149767=CARTESIAN_POINT('Ctrl Pts',(-22.1212728778799,12.9511126916242,
129.490491975582)) ;
#149768=CARTESIAN_POINT('Ctrl Pts',(-22.0828450680906,13.2510040815984,
129.411445954069)) ;
#149769=CARTESIAN_POINT('Ctrl Pts',(-22.0712938830656,13.5624346911567,
129.410820581416)) ;
#149770=CARTESIAN_POINT('Ctrl Pts',(-22.0864657444321,13.863434989198,129.488210788799)) ;
#149771=CARTESIAN_POINT('Ctrl Pts',(-22.126593878773,14.1332612598468,129.638538262364)) ;
#149772=CARTESIAN_POINT('Ctrl Pts',(-22.1881835845486,14.3526408923895,
129.851608596392)) ;
#149773=CARTESIAN_POINT('Ctrl Pts',(-22.2662698967249,14.5054039149979,
130.112943305636)) ;
#149774=CARTESIAN_POINT('Ctrl Pts',(-22.3536617688702,14.5799567514586,
130.401216699648)) ;
#149775=CARTESIAN_POINT('Ctrl Pts',(-22.4444166235303,14.5723714395277,
130.699477612996)) ;
#149776=CARTESIAN_POINT('Ctrl Pts',(-22.5310362051364,14.4818104958985,
130.985724648343)) ;
#149777=CARTESIAN_POINT('Ctrl Pts',(-22.6060015969075,14.3163443663444,
131.237730292278)) ;
#149778=CARTESIAN_POINT('Ctrl Pts',(-22.6640340596901,14.0859121454152,
131.440457148936)) ;
#149779=CARTESIAN_POINT('Ctrl Pts',(-22.6996929687443,13.8088759018265,
131.577695110842)) ;
#149780=CARTESIAN_POINT('Ctrl Pts',(-22.7099178996743,13.5028416968273,
131.640793767491)) ;
#149781=CARTESIAN_POINT('Ctrl Pts',(-22.6932495161997,13.1931031843273,
131.625104283202)) ;
#149782=CARTESIAN_POINT('Ctrl Pts',(-22.6499855145804,12.89795929161,131.531932093916)) ;
#149783=CARTESIAN_POINT('Ctrl Pts',(-22.5827221854466,12.6415807135438,
131.368528308909)) ;
#149784=CARTESIAN_POINT('Ctrl Pts',(-22.4955321587869,12.4408172344946,
131.146922824915)) ;
#149785=CARTESIAN_POINT('Ctrl Pts',(-22.393252860788,12.3100401659206,130.881416910317)) ;
#149786=CARTESIAN_POINT('Ctrl Pts',(-22.2840884304056,12.2598615754433,
130.595478670003)) ;
#149787=CARTESIAN_POINT('Ctrl Pts',(-22.1736356223127,12.2922205414055,
130.305931435607)) ;
#149788=CARTESIAN_POINT('Ctrl Pts',(-22.0692646768025,12.4062484922091,
130.034252292892)) ;
#149789=CARTESIAN_POINT('Ctrl Pts',(-21.9784401265655,12.5927140655513,
129.802018991146)) ;
#149790=CARTESIAN_POINT('Ctrl Pts',(-21.9065444640982,12.8381489007341,
129.62504663551)) ;
#149791=CARTESIAN_POINT('Ctrl Pts',(-21.857754981397,13.1260095421298,129.515650593897)) ;
#149792=CARTESIAN_POINT('Ctrl Pts',(-21.8351198417726,13.4367097246031,
129.482816396722)) ;
#149793=CARTESIAN_POINT('Ctrl Pts',(-21.8396215028571,13.7438376703634,
129.528974842274)) ;
#149794=CARTESIAN_POINT('Ctrl Pts',(-21.8699032060914,14.0287736404421,
129.650514879023)) ;
#149795=CARTESIAN_POINT('Ctrl Pts',(-21.9233871407245,14.270962157525,129.839919077007)) ;
#149796=CARTESIAN_POINT('Ctrl Pts',(-21.9953096059553,14.4520607782582,
130.083142298059)) ;
#149797=CARTESIAN_POINT('Ctrl Pts',(-22.0798724098477,14.5594794315335,
130.363302132946)) ;
#149798=CARTESIAN_POINT('Ctrl Pts',(-22.170121644081,14.5855261775524,130.660019013588)) ;
#149799=CARTESIAN_POINT('Ctrl Pts',(-22.2592468971728,14.5283738977508,
130.953536397664)) ;
#149800=CARTESIAN_POINT('Ctrl Pts',(-22.3398966660071,14.391653675229,131.222308593128)) ;
#149801=CARTESIAN_POINT('Ctrl Pts',(-22.4053261752883,14.1863633924956,
131.446488605931)) ;
#149802=CARTESIAN_POINT('Ctrl Pts',(-22.4506077808692,13.9255969369485,
131.611940327664)) ;
#149803=CARTESIAN_POINT('Ctrl Pts',(-22.4714276383869,13.6292801899933,
131.705867636475)) ;
#149804=CARTESIAN_POINT('Ctrl Pts',(-22.4656985706484,13.3179690921283,
131.722267859741)) ;
#149805=CARTESIAN_POINT('Ctrl Pts',(-22.4330809865824,13.0144329999001,
131.660092690325)) ;
#149806=CARTESIAN_POINT('Ctrl Pts',(-22.3752337324937,12.7401668642732,
131.524210201602)) ;
#149807=CARTESIAN_POINT('Ctrl Pts',(-22.2953919549194,12.5144107984142,
131.324132448709)) ;
#149808=CARTESIAN_POINT('Ctrl Pts',(-22.1986907467925,12.3540785091182,
131.074781660547)) ;
#149809=CARTESIAN_POINT('Ctrl Pts',(-22.0916577558985,12.2704506972946,
130.795149181821)) ;
#149810=CARTESIAN_POINT('Ctrl Pts',(-21.9804835857871,12.2689820751512,
130.503544699241)) ;
#149811=CARTESIAN_POINT('Ctrl Pts',(-21.8726683552619,12.3508509067205,
130.221807220938)) ;
#149812=CARTESIAN_POINT('Ctrl Pts',(-21.7759646206819,12.5086054650755,
129.972319239919)) ;
#149813=CARTESIAN_POINT('Ctrl Pts',(-21.6953381788648,12.7330676157862,
129.770024556173)) ;
#149814=CARTESIAN_POINT('Ctrl Pts',(-21.6368282731019,13.0066123030749,
129.632239940653)) ;
#149815=CARTESIAN_POINT('Ctrl Pts',(-21.6035887086732,13.3082724111724,
129.568104862639)) ;
#149816=CARTESIAN_POINT('Ctrl Pts',(-21.5969642140476,13.6201711563921,
129.581939837877)) ;
#149817=CARTESIAN_POINT('Ctrl Pts',(-21.6171785071835,13.9183339563094,
129.674227224857)) ;
#149818=CARTESIAN_POINT('Ctrl Pts',(-21.6617871521888,14.1797387152336,
129.837645381447)) ;
#149819=CARTESIAN_POINT('Ctrl Pts',(-21.7265912402179,14.3864986617501,
130.059946572306)) ;
#149820=CARTESIAN_POINT('Ctrl Pts',(-21.8067464305552,14.5252641386946,
130.327221597644)) ;
#149821=CARTESIAN_POINT('Ctrl Pts',(-21.8958184713667,14.5851720998815,
130.620620927139)) ;
#149822=CARTESIAN_POINT('Ctrl Pts',(-21.9865681374424,14.561066934574,130.918966487023)) ;
#149823=CARTESIAN_POINT('Ctrl Pts',(-22.0707594233655,14.4566510125324,
131.19779203029)) ;
#149824=CARTESIAN_POINT('Ctrl Pts',(-22.1434681961939,14.2771545547794,
131.443436921697)) ;
#149825=CARTESIAN_POINT('Ctrl Pts',(-22.1975055554167,14.0362065593723,
131.634471428032)) ;
#149826=CARTESIAN_POINT('Ctrl Pts',(-22.228481100872,13.7533987365905,131.757917035488)) ;
#149827=CARTESIAN_POINT('Ctrl Pts',(-22.2337680807398,13.444128366597,131.806637674055)) ;
#149828=CARTESIAN_POINT('Ctrl Pts',(-22.2118313707014,13.1346408962195,
131.775690169026)) ;
#149829=CARTESIAN_POINT('Ctrl Pts',(-22.1641188393883,12.8470251691959,
131.66929025756)) ;
#149830=CARTESIAN_POINT('Ctrl Pts',(-22.0924166245413,12.5984937822196,
131.493091002478)) ;
#149831=CARTESIAN_POINT('Ctrl Pts',(-22.0022409153909,12.4108688263379,
131.262663941909)) ;
#149832=CARTESIAN_POINT('Ctrl Pts',(-21.898534109697,12.2946081111199,130.992821647308)) ;
#149833=CARTESIAN_POINT('Ctrl Pts',(-21.7874624784035,12.2594450542174,
130.701676041375)) ;
#149834=CARTESIAN_POINT('Ctrl Pts',(-21.6778492662529,12.3080481401079,
130.414533549498)) ;
#149835=CARTESIAN_POINT('Ctrl Pts',(-21.5759437155099,12.4360760785603,
130.149908558154)) ;
#149836=CARTESIAN_POINT('Ctrl Pts',(-21.4882912931024,12.6345257825012,
129.926914377626)) ;
#149837=CARTESIAN_POINT('Ctrl Pts',(-21.420235735472,12.8902136369556,129.761280181062)) ;
#149838=CARTESIAN_POINT('Ctrl Pts',(-21.3763386660893,13.1836914556234,
129.666160682438)) ;
#149839=CARTESIAN_POINT('Ctrl Pts',(-21.3588102921648,13.4943233171344,
129.64807578917)) ;
#149840=CARTESIAN_POINT('Ctrl Pts',(-21.3683109889988,13.800844370543,129.709055456557)) ;
#149841=CARTESIAN_POINT('Ctrl Pts',(-21.4034525605879,14.0793169381169,
129.844852216424)) ;
#149842=CARTESIAN_POINT('Ctrl Pts',(-21.4604693997575,14.3098744283553,
130.044376194059)) ;
#149843=CARTESIAN_POINT('Ctrl Pts',(-21.5356692735843,14.4788323999099,
130.297359822827)) ;
#149844=CARTESIAN_POINT('Ctrl Pts',(-21.6216446878527,14.5706779805767,
130.581543004274)) ;
#149845=CARTESIAN_POINT('Ctrl Pts',(-21.7121217703692,14.5811216751553,
130.878902955014)) ;
#149846=CARTESIAN_POINT('Ctrl Pts',(-21.8002831689519,14.5082992229446,
131.169647708702)) ;
#149847=CARTESIAN_POINT('Ctrl Pts',(-21.8783799046181,14.3580059118444,
131.43087371812)) ;
#149848=CARTESIAN_POINT('Ctrl Pts',(-21.9405361241306,14.1405258591395,
131.645593076356)) ;
#149849=CARTESIAN_POINT('Ctrl Pts',(-21.9813282753517,13.8719963111484,
131.797849655205)) ;
#149850=CARTESIAN_POINT('Ctrl Pts',(-21.9973134311112,13.5716291757303,
131.877616580862)) ;
#149851=CARTESIAN_POINT('Ctrl Pts',(-21.986445843118,13.2591264952113,131.879101856403)) ;
#149852=CARTESIAN_POINT('Ctrl Pts',(-21.9489161756331,12.9599152981085,
131.80253028907)) ;
#149853=CARTESIAN_POINT('Ctrl Pts',(-21.8865489034867,12.6930802012435,
131.653491136013)) ;
#149854=CARTESIAN_POINT('Ctrl Pts',(-21.8031604369027,12.4788238742032,
131.443016238686)) ;
#149855=CARTESIAN_POINT('Ctrl Pts',(-21.7040670699751,12.3322479611375,
131.186643032547)) ;
#149856=CARTESIAN_POINT('Ctrl Pts',(-21.5954848934324,12.2636849703181,
130.902576073362)) ;
#149857=CARTESIAN_POINT('Ctrl Pts',(-21.4844977011893,12.2782423508481,
130.611495128797)) ;
#149858=CARTESIAN_POINT('Ctrl Pts',(-21.3784236599933,12.3748788138008,
130.334754138936)) ;
#149859=CARTESIAN_POINT('Ctrl Pts',(-21.2841566381779,12.5463734301239,
130.092472417729)) ;
#149860=CARTESIAN_POINT('Ctrl Pts',(-21.2075185163092,12.7810696053441,
129.901748161502)) ;
#149861=CARTESIAN_POINT('Ctrl Pts',(-21.1535857557247,13.0608632810621,
129.777242893781)) ;
#149862=CARTESIAN_POINT('Ctrl Pts',(-21.1251082585069,13.3671882377426,
129.727176867914)) ;
#149863=CARTESIAN_POINT('Ctrl Pts',(-21.1236808485437,13.6783220595412,
129.756215090546)) ;
#149864=CARTESIAN_POINT('Ctrl Pts',(-21.1486075426851,13.9701100472944,
129.862126299147)) ;
#149865=CARTESIAN_POINT('Ctrl Pts',(-21.1973535450429,14.2230345165602,
130.037651301572)) ;
#149866=CARTESIAN_POINT('Ctrl Pts',(-21.2657341311525,14.4186168854027,
130.270535077452)) ;
#149867=CARTESIAN_POINT('Ctrl Pts',(-21.3480366756193,14.5428705868712,
130.54406387908)) ;
#149868=CARTESIAN_POINT('Ctrl Pts',(-21.4377691926866,14.5869069851008,
130.839327006419)) ;
#149869=CARTESIAN_POINT('Ctrl Pts',(-21.5275182421065,14.5480013167689,
131.134553678454)) ;
#149870=CARTESIAN_POINT('Ctrl Pts',(-21.6110497338832,14.4271740757264,
131.411928848396)) ;
#149871=CARTESIAN_POINT('Ctrl Pts',(-21.6799255328032,14.2362638789622,
131.646058353633)) ;
#149872=CARTESIAN_POINT('Ctrl Pts',(-21.7300456232936,13.9863048422078,
131.825612120033)) ;
#149873=CARTESIAN_POINT('Ctrl Pts',(-21.7564143680409,13.6957298315302,
131.935786982782)) ;
#149874=CARTESIAN_POINT('Ctrl Pts',(-21.7566600694498,13.3866515918627,
131.969541292452)) ;
#149875=CARTESIAN_POINT('Ctrl Pts',(-21.729544783517,13.0771469983457,131.923709750482)) ;
#149876=CARTESIAN_POINT('Ctrl Pts',(-21.6771516178043,12.7963921312271,
131.803576103484)) ;
#149877=CARTESIAN_POINT('Ctrl Pts',(-21.601485043082,12.5578779663261,131.615788388401)) ;
#149878=CARTESIAN_POINT('Ctrl Pts',(-21.5083743731948,12.3830735911952,
131.376772518408)) ;
#149879=CARTESIAN_POINT('Ctrl Pts',(-21.4027033277101,12.2815115328469,
131.101246209364)) ;
#149880=CARTESIAN_POINT('Ctrl Pts',(-21.2914566395192,12.2623682351307,
130.809508334023)) ;
#149881=CARTESIAN_POINT('Ctrl Pts',(-21.183156911401,12.3259183972767,130.526081481035)) ;
#149882=CARTESIAN_POINT('Ctrl Pts',(-21.0831383092239,12.4680808771893,
130.267052456152)) ;
#149883=CARTESIAN_POINT('Ctrl Pts',(-20.9984926472638,12.6795622431896,
130.052999466313)) ;
#149884=CARTESIAN_POINT('Ctrl Pts',(-20.9350511107532,12.942589382418,129.900666960476)) ;
#149885=CARTESIAN_POINT('Ctrl Pts',(-20.8958233184202,13.2417281941733,
129.819283617023)) ;
#149886=CARTESIAN_POINT('Ctrl Pts',(-20.8834458948203,13.5531901597367,
129.816249612058)) ;
#149887=CARTESIAN_POINT('Ctrl Pts',(-20.8979142935974,13.8554127215433,
129.891658607767)) ;
#149888=CARTESIAN_POINT('Ctrl Pts',(-20.9373087909547,14.1261607802399,
130.039800242733)) ;
#149889=CARTESIAN_POINT('Ctrl Pts',(-20.9986572396186,14.3478084011447,
130.252296892612)) ;
#149890=CARTESIAN_POINT('Ctrl Pts',(-21.0756161881204,14.5013886239399,
130.510026273036)) ;
#149891=CARTESIAN_POINT('Ctrl Pts',(-21.1635267894519,14.5792262889595,
130.800096886863)) ;
#149892=CARTESIAN_POINT('Ctrl Pts',(-21.2541062230571,14.5735423486693,
131.097774254365)) ;
#149893=CARTESIAN_POINT('Ctrl Pts',(-21.3407174693846,14.4859392632534,
131.383892695644)) ;
#149894=CARTESIAN_POINT('Ctrl Pts',(-21.4166169572043,14.3210240501096,
131.638882857702)) ;
#149895=CARTESIAN_POINT('Ctrl Pts',(-21.4747584664031,14.0938130208259,
131.841674679454)) ;
#149896=CARTESIAN_POINT('Ctrl Pts',(-21.5112781420335,13.8165580564643,
131.981597335147)) ;
#149897=CARTESIAN_POINT('Ctrl Pts',(-21.5222480980289,13.5127265390552,
132.046676530408)) ;
#149898=CARTESIAN_POINT('Ctrl Pts',(-21.5061347629943,13.2000972464797,
132.032913742005)) ;
#149899=CARTESIAN_POINT('Ctrl Pts',(-21.4640156292753,12.9073427660881,
131.942726153517)) ;
#149900=CARTESIAN_POINT('Ctrl Pts',(-21.397117735376,12.6479572947944,131.780585336987)) ;
#149901=CARTESIAN_POINT('Ctrl Pts',(-21.3106813900893,12.4461100602533,
131.561069221284)) ;
#149902=CARTESIAN_POINT('Ctrl Pts',(-21.2086821275541,12.3127706355445,
131.296414857345)) ;
#149903=CARTESIAN_POINT('Ctrl Pts',(-21.0995344791146,12.2601401093184,
131.010556487313)) ;
#149904=CARTESIAN_POINT('Ctrl Pts',(-20.9889798404996,12.2901733170219,
130.720722307534)) ;
#149905=CARTESIAN_POINT('Ctrl Pts',(-20.8845090238334,12.4015832972313,
130.448684666842)) ;
#149906=CARTESIAN_POINT('Ctrl Pts',(-20.7929548516875,12.5866483743453,
130.214420543969)) ;
#149907=CARTESIAN_POINT('Ctrl Pts',(-20.720494862863,12.8302723297284,130.035755542928)) ;
#149908=CARTESIAN_POINT('Ctrl Pts',(-20.6708320754766,13.1192440323379,
129.924028986074)) ;
#149909=CARTESIAN_POINT('Ctrl Pts',(-20.6477168971474,13.4254781979924,
129.889340729932)) ;
#149910=CARTESIAN_POINT('Ctrl Pts',(-20.6512834404018,13.735359683146,129.933026055129)) ;
#149911=CARTESIAN_POINT('Ctrl Pts',(-20.6809119562705,14.0210481955409,
130.052635771819)) ;
#149912=CARTESIAN_POINT('Ctrl Pts',(-20.7338408988299,14.2649914593589,
130.240457331941)) ;
#149913=CARTESIAN_POINT('Ctrl Pts',(-20.8051898847713,14.4476746883627,
130.481943155495)) ;
#149914=CARTESIAN_POINT('Ctrl Pts',(-20.8894411703123,14.5574099930499,
130.761185950254)) ;
#149915=CARTESIAN_POINT('Ctrl Pts',(-20.9796503552771,14.5860647522522,
131.057792726659)) ;
#149916=CARTESIAN_POINT('Ctrl Pts',(-21.0692814846415,14.5307819491484,
131.352933777741)) ;
#149917=CARTESIAN_POINT('Ctrl Pts',(-21.1498107519784,14.3969445600344,
131.621163297151)) ;
#149918=CARTESIAN_POINT('Ctrl Pts',(-21.2160230444839,14.1927449819674,
131.847762712336)) ;
#149919=CARTESIAN_POINT('Ctrl Pts',(-21.2617909617919,13.9340125126876,
132.014532566798)) ;
#149920=CARTESIAN_POINT('Ctrl Pts',(-21.2834169760681,13.6381122428634,
132.110859969198)) ;
#149921=CARTESIAN_POINT('Ctrl Pts',(-21.2784641686458,13.3270743882958,
132.129508993966)) ;
#149922=CARTESIAN_POINT('Ctrl Pts',(-21.2465760701754,13.022510775008,132.069516737505)) ;
#149923=CARTESIAN_POINT('Ctrl Pts',(-21.1892311552638,12.7468021187138,
131.935157683102)) ;
#149924=CARTESIAN_POINT('Ctrl Pts',(-21.1103505322267,12.5205888533643,
131.737718520491)) ;
#149925=CARTESIAN_POINT('Ctrl Pts',(-21.0140654020534,12.3578210122937,
131.489600695312)) ;
#149926=CARTESIAN_POINT('Ctrl Pts',(-20.9069519089274,12.2716455027741,
131.209820749627)) ;
#149927=CARTESIAN_POINT('Ctrl Pts',(-20.7959007646827,12.2679542835663,
130.91854323311)) ;
#149928=CARTESIAN_POINT('Ctrl Pts',(-20.6882404753147,12.3469221374096,
130.637139748733)) ;
#149929=CARTESIAN_POINT('Ctrl Pts',(-20.590745173864,12.5030897490068,130.385469307244)) ;
#149930=CARTESIAN_POINT('Ctrl Pts',(-20.5098618731191,12.7250181142628,
130.182298437456)) ;
#149931=CARTESIAN_POINT('Ctrl Pts',(-20.4505145686487,12.997182712002,130.042072465219)) ;
#149932=CARTESIAN_POINT('Ctrl Pts',(-20.4163461458151,13.2997827331154,
129.97538649999)) ;
#149933=CARTESIAN_POINT('Ctrl Pts',(-20.4090290392878,13.6108909290664,
129.98710788454)) ;
#149934=CARTESIAN_POINT('Ctrl Pts',(-20.4282921071053,13.9087322628313,
130.076489390265)) ;
#149935=CARTESIAN_POINT('Ctrl Pts',(-20.4722899184275,14.1725575472539,
130.238237437672)) ;
#149936=CARTESIAN_POINT('Ctrl Pts',(-20.5367340681886,14.3815587405522,
130.4595615294)) ;
#149937=CARTESIAN_POINT('Ctrl Pts',(-20.6165397161228,14.5223295633007,
130.725809297898)) ;
#149938=CARTESIAN_POINT('Ctrl Pts',(-20.7051933027261,14.5844939623778,
131.017890368957)) ;
#149939=CARTESIAN_POINT('Ctrl Pts',(-20.7959857696704,14.5631534424975,
131.316353588216)) ;
#149940=CARTESIAN_POINT('Ctrl Pts',(-20.8807942840004,14.4606751322893,
131.597113045962)) ;
#149941=CARTESIAN_POINT('Ctrl Pts',(-20.9539376095154,14.2826954398612,
131.844058123702)) ;
#149942=CARTESIAN_POINT('Ctrl Pts',(-21.0083263347871,14.0447463788915,
132.03593245135)) ;
#149943=CARTESIAN_POINT('Ctrl Pts',(-21.040197088768,13.7613771395104,132.162181015758)) ;
#149944=CARTESIAN_POINT('Ctrl Pts',(-21.0461960024793,13.4542323467487,
132.212789454969)) ;
#149945=CARTESIAN_POINT('Ctrl Pts',(-21.0251622314024,13.1437994705374,
132.184546651193)) ;
#149946=CARTESIAN_POINT('Ctrl Pts',(-20.977827703154,12.8538469195634,132.079426774606)) ;
#149947=CARTESIAN_POINT('Ctrl Pts',(-20.907128727735,12.6054873461084,131.905959845305)) ;
#149948=CARTESIAN_POINT('Ctrl Pts',(-20.8174409553095,12.4153273171675,
131.676988843587)) ;
#149949=CARTESIAN_POINT('Ctrl Pts',(-20.713143280337,12.2964112453651,131.405684529226)) ;
#149950=CARTESIAN_POINT('Ctrl Pts',(-20.6033763157009,12.2594155907016,
131.117980797481)) ;
#149951=CARTESIAN_POINT('Ctrl Pts',(-20.4932077646269,12.3053349417689,
130.829346648373)) ;
#149952=CARTESIAN_POINT('Ctrl Pts',(-20.3910080733494,12.4312258982637,
130.563852755589)) ;
#149953=CARTESIAN_POINT('Ctrl Pts',(-20.3027473879503,12.627959699626,130.339118872896)) ;
#149954=CARTESIAN_POINT('Ctrl Pts',(-20.2340446900552,12.8824932642082,
130.171614220239)) ;
#149955=CARTESIAN_POINT('Ctrl Pts',(-20.1895024515561,13.1745455141317,
130.074542304732)) ;
#149956=CARTESIAN_POINT('Ctrl Pts',(-20.1711377465811,13.4851755332174,
130.05403371038)) ;
#149957=CARTESIAN_POINT('Ctrl Pts',(-20.1799007530891,13.7921378916297,
130.112861990177)) ;
#149958=CARTESIAN_POINT('Ctrl Pts',(-20.2141338523858,14.0710147358115,
130.245900077458)) ;
#149959=CARTESIAN_POINT('Ctrl Pts',(-20.2709644008969,14.3045451630866,
130.445096643664)) ;
#149960=CARTESIAN_POINT('Ctrl Pts',(-20.3450269541787,14.4740865668841,
130.694444672256)) ;
#149961=CARTESIAN_POINT('Ctrl Pts',(-20.4312885839604,14.5693022255178,
130.979690231724)) ;
#149962=CARTESIAN_POINT('Ctrl Pts',(-20.5217224177781,14.5820126404232,
131.276907919029)) ;
#149963=CARTESIAN_POINT('Ctrl Pts',(-20.6102794068549,14.511227148385,131.56889920101)) ;
#149964=CARTESIAN_POINT('Ctrl Pts',(-20.6884126712052,14.3635592095882,
131.830093439836)) ;
#149965=CARTESIAN_POINT('Ctrl Pts',(-20.751162116013,14.1479540457657,132.046552023884)) ;
#149966=CARTESIAN_POINT('Ctrl Pts',(-20.7926884527049,13.8806548150988,
132.200960049177)) ;
#149967=CARTESIAN_POINT('Ctrl Pts',(-20.8094672658813,13.5796274976099,
132.283185376369)) ;
#149968=CARTESIAN_POINT('Ctrl Pts',(-20.7992847698798,13.2675903207149,
132.286621512042)) ;
#149969=CARTESIAN_POINT('Ctrl Pts',(-20.7626296984893,12.9685393954342,
132.212514858308)) ;
#149970=CARTESIAN_POINT('Ctrl Pts',(-20.7008934220108,12.7001828412868,
132.065351539406)) ;
#149971=CARTESIAN_POINT('Ctrl Pts',(-20.6181564504024,12.484351447388,131.856740622627)) ;
#149972=CARTESIAN_POINT('Ctrl Pts',(-20.5192778681803,12.3354378229303,
131.60104993334)) ;
#149973=CARTESIAN_POINT('Ctrl Pts',(-20.4111933713258,12.2645466644513,
131.318338142685)) ;
#149974=CARTESIAN_POINT('Ctrl Pts',(-20.2996662166456,12.2767400310682,
131.025835168853)) ;
#149975=CARTESIAN_POINT('Ctrl Pts',(-20.1937352114642,12.3708038596253,
130.749389711576)) ;
#149976=CARTESIAN_POINT('Ctrl Pts',(-20.0988429416229,12.5405713719576,
130.505353011285)) ;
#149977=CARTESIAN_POINT('Ctrl Pts',(-20.021843202684,12.7727635932404,130.31345487307)) ;
#149978=CARTESIAN_POINT('Ctrl Pts',(-19.9668156943562,13.0532481868504,
130.185965715989)) ;
#149979=CARTESIAN_POINT('Ctrl Pts',(-19.9377532447316,13.3594503322591,
130.134212682871)) ;
#149980=CARTESIAN_POINT('Ctrl Pts',(-19.9355477333015,13.6687250263673,
130.16075894901)) ;
#149981=CARTESIAN_POINT('Ctrl Pts',(-19.9597474888427,13.9622483916866,
130.26464405238)) ;
#149982=CARTESIAN_POINT('Ctrl Pts',(-20.0078395553135,14.216383713817,130.438234282855)) ;
#149983=CARTESIAN_POINT('Ctrl Pts',(-20.0759089225194,14.4143549366633,
130.670296074007)) ;
#149984=CARTESIAN_POINT('Ctrl Pts',(-20.157927076402,14.5404303817965,130.942989232008)) ;
#149985=CARTESIAN_POINT('Ctrl Pts',(-20.2471634575349,14.5868747918771,
131.236660122781)) ;
#149986=CARTESIAN_POINT('Ctrl Pts',(-20.3375200447807,14.5499212465235,
131.533862304864)) ;
#149987=CARTESIAN_POINT('Ctrl Pts',(-20.4206467735753,14.4324626280189,
131.809760427588)) ;
#149988=CARTESIAN_POINT('Ctrl Pts',(-20.4906530935794,14.2419356925952,
132.04749075942)) ;
#149989=CARTESIAN_POINT('Ctrl Pts',(-20.5411214430323,13.9939564781135,
132.227948854795)) ;
#149990=CARTESIAN_POINT('Ctrl Pts',(-20.5682544096884,13.704318184283,132.340358463569)) ;
#149991=CARTESIAN_POINT('Ctrl Pts',(-20.5692014180171,13.3953698080797,
132.376173579921)) ;
#149992=CARTESIAN_POINT('Ctrl Pts',(-20.543054261984,13.0868084154143,132.333020355237)) ;
#149993=CARTESIAN_POINT('Ctrl Pts',(-20.4911384960752,12.8035341969557,
132.214453828355)) ;
#149994=CARTESIAN_POINT('Ctrl Pts',(-20.4161441436802,12.5639567807414,
132.028575184502)) ;
#149995=CARTESIAN_POINT('Ctrl Pts',(-20.323298875788,12.3867441637874,131.790400600433)) ;
#149996=CARTESIAN_POINT('Ctrl Pts',(-20.2176703488979,12.2832559851663,
131.515052106227)) ;
#149997=CARTESIAN_POINT('Ctrl Pts',(-20.1074375512045,12.2616345605918,
131.225985798419)) ;
#149998=CARTESIAN_POINT('Ctrl Pts',(-19.9980972507774,12.3231638536054,
130.939790413276)) ;
#149999=CARTESIAN_POINT('Ctrl Pts',(-19.8981987414102,12.4627499394219,
130.680958618524)) ;
#150000=CARTESIAN_POINT('Ctrl Pts',(-19.8127745396768,12.6729052718455,
130.464725436601)) ;
#150001=CARTESIAN_POINT('Ctrl Pts',(-19.7487491589229,12.9344259227914,
130.310649365382)) ;
#150002=CARTESIAN_POINT('Ctrl Pts',(-19.7086902319659,13.2340773776093,
130.226969486189)) ;
#150003=CARTESIAN_POINT('Ctrl Pts',(-19.6956791745323,13.5439037579597,
130.221914932001)) ;
#150004=CARTESIAN_POINT('Ctrl Pts',(-19.7092885690522,13.8465580418888,
130.294793249448)) ;
#150005=CARTESIAN_POINT('Ctrl Pts',(-19.7480403292005,14.1188038713519,
130.441095578693)) ;
#150006=CARTESIAN_POINT('Ctrl Pts',(-19.8087237127228,14.3420290100945,
130.651608670912)) ;
#150007=CARTESIAN_POINT('Ctrl Pts',(-19.8855246325867,14.4980359942342,
130.908974260646)) ;
#150008=CARTESIAN_POINT('Ctrl Pts',(-19.9728075519884,14.5780642273586,
131.197048865793)) ;
#150009=CARTESIAN_POINT('Ctrl Pts',(-20.0641053332561,14.5747644826435,
131.497087362298)) ;
#150010=CARTESIAN_POINT('Ctrl Pts',(-20.1504360631443,14.4895501610045,
131.78220700389)) ;
#150011=CARTESIAN_POINT('Ctrl Pts',(-20.2266398469847,14.3274512492284,
132.038011928508)) ;
#150012=CARTESIAN_POINT('Ctrl Pts',(-20.2855836739268,14.1012132638127,
132.24325861374)) ;
#150013=CARTESIAN_POINT('Ctrl Pts',(-20.322802771727,13.8249845460598,132.38523118764)) ;
#150014=CARTESIAN_POINT('Ctrl Pts',(-20.3344826698602,13.5214322498008,
132.452410552018)) ;
#150015=CARTESIAN_POINT('Ctrl Pts',(-20.3193210016494,13.2103012906498,
132.441249802482)) ;
#150016=CARTESIAN_POINT('Ctrl Pts',(-20.2777434342537,12.9148532229271,
132.35285539736)) ;
#150017=CARTESIAN_POINT('Ctrl Pts',(-20.2114185666706,12.6543478093024,
132.19237858542)) ;
#150018=CARTESIAN_POINT('Ctrl Pts',(-20.1256275275734,12.4511189000955,
131.974692258579)) ;
#150019=CARTESIAN_POINT('Ctrl Pts',(-20.0242015823174,12.3156705580683,
131.711643730949)) ;
#150020=CARTESIAN_POINT('Ctrl Pts',(-19.9146972236327,12.2603783302423,
131.424892243311)) ;
#150021=CARTESIAN_POINT('Ctrl Pts',(-19.804137467759,12.2883877203707,131.13502656788)) ;
#150022=CARTESIAN_POINT('Ctrl Pts',(-19.699816800067,12.396958249081,130.86328933831)) ;
#150023=CARTESIAN_POINT('Ctrl Pts',(-19.6074508319546,12.5805839633338,
130.626767342191)) ;
#150024=CARTESIAN_POINT('Ctrl Pts',(-19.534586073173,12.8225431186843,130.446872902408)) ;
#150025=CARTESIAN_POINT('Ctrl Pts',(-19.48430105852,13.1085293603561,130.333118269165)) ;
#150026=CARTESIAN_POINT('Ctrl Pts',(-19.4601499587593,13.4184312880114,
130.29583788212)) ;
#150027=CARTESIAN_POINT('Ctrl Pts',(-19.4629889713343,13.725396861632,130.337043757937)) ;
#150028=CARTESIAN_POINT('Ctrl Pts',(-19.4919997843254,14.0140710256624,
130.455081243063)) ;
#150029=CARTESIAN_POINT('Ctrl Pts',(-19.5442604752578,14.2586953044857,
130.640856243093)) ;
#150030=CARTESIAN_POINT('Ctrl Pts',(-19.6152214709248,14.4435712314573,
130.881253585167)) ;
#150031=CARTESIAN_POINT('Ctrl Pts',(-19.6991862638108,14.5554638006899,
131.159645901593)) ;
#150032=CARTESIAN_POINT('Ctrl Pts',(-19.7894150942462,14.5862678502932,
131.45634808166)) ;
#150033=CARTESIAN_POINT('Ctrl Pts',(-19.8785826985735,14.5339455436029,
131.749904644687)) ;
#150034=CARTESIAN_POINT('Ctrl Pts',(-19.9598958275185,14.4019055973539,
132.020594708233)) ;
#150035=CARTESIAN_POINT('Ctrl Pts',(-20.0265337164306,14.1996929983724,
132.248397159288)) ;
#150036=CARTESIAN_POINT('Ctrl Pts',(-20.0730460777264,13.9418840737313,
132.417403083246)) ;
#150037=CARTESIAN_POINT('Ctrl Pts',(-20.0953762004544,13.6467946760401,
132.515776294982)) ;
#150038=CARTESIAN_POINT('Ctrl Pts',(-20.0911858048577,13.3358858786889,
132.536654639505)) ;
#150039=CARTESIAN_POINT('Ctrl Pts',(-20.0600962019105,13.0311284856173,
132.47895867768)) ;
#150040=CARTESIAN_POINT('Ctrl Pts',(-20.0034577116224,12.7543596486341,
132.346659990378)) ;
#150041=CARTESIAN_POINT('Ctrl Pts',(-19.9252445945777,12.5263865010007,
132.151152771168)) ;
#150042=CARTESIAN_POINT('Ctrl Pts',(-19.8285737015795,12.3607018495905,
131.902162071254)) ;
#150043=CARTESIAN_POINT('Ctrl Pts',(-19.7226384575838,12.2732420345152,
131.625515596499)) ;
#150044=CARTESIAN_POINT('Ctrl Pts',(-19.6111674213246,12.2668291057712,
131.333147098468)) ;
#150045=CARTESIAN_POINT('Ctrl Pts',(-19.5033876747326,12.3436151679642,
131.051371024019)) ;
#150046=CARTESIAN_POINT('Ctrl Pts',(-19.40539646053,12.4979166687538,130.79829315841)) ;
#150047=CARTESIAN_POINT('Ctrl Pts',(-19.3240491831095,12.7181779713464,
130.593748829707)) ;
#150048=CARTESIAN_POINT('Ctrl Pts',(-19.2641202298485,12.9887183065796,
130.451770199842)) ;
#150049=CARTESIAN_POINT('Ctrl Pts',(-19.2291670799778,13.2908825887428,
130.382809693789)) ;
#150050=CARTESIAN_POINT('Ctrl Pts',(-19.2210624747814,13.6021682784688,
130.392241564163)) ;
#150051=CARTESIAN_POINT('Ctrl Pts',(-19.2396860598708,13.9015372403182,
130.47985199514)) ;
#150052=CARTESIAN_POINT('Ctrl Pts',(-19.2830862718829,14.1661756912177,
130.639822284067)) ;
#150053=CARTESIAN_POINT('Ctrl Pts',(-19.3468000223966,14.3763136257562,
130.858909722296)) ;
#150054=CARTESIAN_POINT('Ctrl Pts',(-19.4264441058091,14.5195378836765,
131.124765334975)) ;
#150055=CARTESIAN_POINT('Ctrl Pts',(-19.5147201923918,14.5837467686513,
131.415658330279)) ;
#150056=CARTESIAN_POINT('Ctrl Pts',(-19.6054851848399,14.5651055728363,
131.714010716355)) ;
#150057=CARTESIAN_POINT('Ctrl Pts',(-19.6908231045242,14.4645029027952,
131.996426898387)) ;
#150058=CARTESIAN_POINT('Ctrl Pts',(-19.7641560074583,14.2890440216263,
132.243815754987)) ;
#150059=CARTESIAN_POINT('Ctrl Pts',(-19.8192252487056,14.0526945141533,
132.437694359878)) ;
#150060=CARTESIAN_POINT('Ctrl Pts',(-19.8518415513689,13.769986617102,132.566162345859)) ;
#150061=CARTESIAN_POINT('Ctrl Pts',(-19.8586489010726,13.4631529516268,
132.619138437853)) ;
#150062=CARTESIAN_POINT('Ctrl Pts',(-19.8381858668256,13.1513621108982,
132.592691996163)) ;
#150063=CARTESIAN_POINT('Ctrl Pts',(-19.7919813808844,12.8627668355385,
132.490607274321)) ;
#150064=CARTESIAN_POINT('Ctrl Pts',(-19.7213546290731,12.6109028724027,
132.317625946872)) ;
#150065=CARTESIAN_POINT('Ctrl Pts',(-19.6324894396037,12.420019305974,132.090897675296)) ;
#150066=CARTESIAN_POINT('Ctrl Pts',(-19.5284529577394,12.2986947230639,
131.820380912839)) ;
#150067=CARTESIAN_POINT('Ctrl Pts',(-19.4189287181224,12.259272392657,131.5333369683)) ;
#150068=CARTESIAN_POINT('Ctrl Pts',(-19.3083138956178,12.3030853474754,
131.243507528801)) ;
#150069=CARTESIAN_POINT('Ctrl Pts',(-19.2063363439977,12.4259705757025,
130.978478363128)) ;
#150070=CARTESIAN_POINT('Ctrl Pts',(-19.1169914034161,12.6220549882292,
130.750798394588)) ;
#150071=CARTESIAN_POINT('Ctrl Pts',(-19.0479500852708,12.8744669108447,
130.582186724412)) ;
#150072=CARTESIAN_POINT('Ctrl Pts',(-19.0025666487703,13.1663405634683,
130.482735394788)) ;
#150073=CARTESIAN_POINT('Ctrl Pts',(-18.9835597805517,13.4758788255352,
130.460255917191)) ;
#150074=CARTESIAN_POINT('Ctrl Pts',(-18.9913631683965,13.7823952267848,
130.516170859479)) ;
#150075=CARTESIAN_POINT('Ctrl Pts',(-19.0251922780675,14.0644181271455,
130.648288433154)) ;
#150076=CARTESIAN_POINT('Ctrl Pts',(-19.0810022453044,14.2977470624668,
130.844241092897)) ;
#150077=CARTESIAN_POINT('Ctrl Pts',(-19.1550953089256,14.470619356869,131.093908367077)) ;
#150078=CARTESIAN_POINT('Ctrl Pts',(-19.2408649444371,14.5675954870708,
131.37760184104)) ;
#150079=CARTESIAN_POINT('Ctrl Pts',(-19.331312849513,14.5827756114501,131.674886283311)) ;
#150080=CARTESIAN_POINT('Ctrl Pts',(-19.4196868659102,14.5148009028155,
131.966202591199)) ;
#150081=CARTESIAN_POINT('Ctrl Pts',(-19.4984938247197,14.369224395635,132.229462715935)) ;
#150082=CARTESIAN_POINT('Ctrl Pts',(-19.5620352226328,14.1540995770501,
132.448398160212)) ;
#150083=CARTESIAN_POINT('Ctrl Pts',(-19.6039630489008,13.8891947674814,
132.60382128396)) ;
#150084=CARTESIAN_POINT('Ctrl Pts',(-19.6215605930756,13.5894850421774,
132.688377146492)) ;
#150085=CARTESIAN_POINT('Ctrl Pts',(-19.612225543082,13.2771023843451,132.694326506547)) ;
#150086=CARTESIAN_POINT('Ctrl Pts',(-19.576287627729,12.9767130862842,132.622385343517)) ;
#150087=CARTESIAN_POINT('Ctrl Pts',(-19.514916360472,12.7063603271624,132.476405969442)) ;
#150088=CARTESIAN_POINT('Ctrl Pts',(-19.4331680822589,12.4901610418877,
132.270491422667)) ;
#150089=CARTESIAN_POINT('Ctrl Pts',(-19.3346192424875,12.3386882869186,
132.015797856231)) ;
#150090=CARTESIAN_POINT('Ctrl Pts',(-19.2264990527328,12.2654833410071,
131.73304515697)) ;
#150091=CARTESIAN_POINT('Ctrl Pts',(-19.1153149338654,12.2750423619251,
131.44142995182)) ;
#150092=CARTESIAN_POINT('Ctrl Pts',(-19.0086090943406,12.3673308735559,
131.162894773645)) ;
#150093=CARTESIAN_POINT('Ctrl Pts',(-18.9137735051228,12.5343468737747,
130.9188596151)) ;
#150094=CARTESIAN_POINT('Ctrl Pts',(-18.8359718102372,12.7652870390172,
130.724693720235)) ;
#150095=CARTESIAN_POINT('Ctrl Pts',(-18.7803364844381,13.0444118412715,
130.5953903177)) ;
#150096=CARTESIAN_POINT('Ctrl Pts',(-18.7504170703459,13.3498616588083,
130.541106996476)) ;
#150097=CARTESIAN_POINT('Ctrl Pts',(-18.7474986385281,13.6613614501294,
130.565792830486)) ;
#150098=CARTESIAN_POINT('Ctrl Pts',(-18.770895305451,13.9537821761938,130.667122829529)) ;
#150099=CARTESIAN_POINT('Ctrl Pts',(-18.8183173068615,14.2096141280325,
130.838782877024)) ;
#150100=CARTESIAN_POINT('Ctrl Pts',(-18.8857427274339,14.4090573125523,
131.06889618268)) ;
#150101=CARTESIAN_POINT('Ctrl Pts',(-18.9673787677367,14.5378227703646,
131.340470029779)) ;
#150102=CARTESIAN_POINT('Ctrl Pts',(-19.0571958207579,14.586641023904,131.636096348978)) ;
#150103=CARTESIAN_POINT('Ctrl Pts',(-19.1467790983166,14.5524956993372,
131.930711805515)) ;
#150104=CARTESIAN_POINT('Ctrl Pts',(-19.2309617987245,14.4363359778134,
132.210003154507)) ;
#150105=CARTESIAN_POINT('Ctrl Pts',(-19.300918514833,14.2487612489542,132.447357659532)) ;
#150106=CARTESIAN_POINT('Ctrl Pts',(-19.3521712301763,14.001996361713,132.630173766833)) ;
#150107=CARTESIAN_POINT('Ctrl Pts',(-19.3800605103585,13.7133413728872,
132.744778521747)) ;
#150108=CARTESIAN_POINT('Ctrl Pts',(-19.3817028074299,13.4034231145874,
132.782762033844)) ;
#150109=CARTESIAN_POINT('Ctrl Pts',(-19.3565445968679,13.096615616376,132.742260368403)) ;
#150110=CARTESIAN_POINT('Ctrl Pts',(-19.3050439571965,12.8104956483767,
132.625124675271)) ;
#150111=CARTESIAN_POINT('Ctrl Pts',(-19.2310094888665,12.5707042667784,
132.441871024858)) ;
#150112=CARTESIAN_POINT('Ctrl Pts',(-19.1385073184765,12.391019395432,132.204759045366)) ;
#150113=CARTESIAN_POINT('Ctrl Pts',(-19.0333885201903,12.2853288824572,
131.930823316902)) ;
#150114=CARTESIAN_POINT('Ctrl Pts',(-18.9228482359354,12.2609818492728,
131.640971207791)) ;
#150115=CARTESIAN_POINT('Ctrl Pts',(-18.8130720194284,12.320475723284,131.353587807363)) ;
#150116=CARTESIAN_POINT('Ctrl Pts',(-18.7128689247104,12.4582515201719,
131.093872581941)) ;
#150117=CARTESIAN_POINT('Ctrl Pts',(-18.6272057293813,12.6658997536836,
130.876826622372)) ;
#150118=CARTESIAN_POINT('Ctrl Pts',(-18.5624249500162,12.9268094738204,
130.720624674853)) ;
#150119=CARTESIAN_POINT('Ctrl Pts',(-18.5218696438751,13.2233760165972,
130.635234806146)) ;
#150120=CARTESIAN_POINT('Ctrl Pts',(-18.5078382142161,13.5346575170046,
130.62736814531)) ;
#150121=CARTESIAN_POINT('Ctrl Pts',(-18.5207859995942,13.8387959699086,
130.698413100486)) ;
#150122=CARTESIAN_POINT('Ctrl Pts',(-18.5589704650504,14.1123016431052,
130.843088517918)) ;
#150123=CARTESIAN_POINT('Ctrl Pts',(-18.6189702798864,14.3364686131329,
131.051516258642)) ;
#150124=CARTESIAN_POINT('Ctrl Pts',(-18.6953756786293,14.4947707498965,
131.307733622343)) ;
#150125=CARTESIAN_POINT('Ctrl Pts',(-18.7828513417895,14.5769227712613,
131.596511728995)) ;
#150126=CARTESIAN_POINT('Ctrl Pts',(-18.8731056944461,14.5762675707607,
131.893112870536)) ;
#150127=CARTESIAN_POINT('Ctrl Pts',(-18.9604254053233,14.493055502163,132.181412688869)) ;
#150128=CARTESIAN_POINT('Ctrl Pts',(-19.0368313978755,14.3331651665745,
132.437726971307)) ;
#150129=CARTESIAN_POINT('Ctrl Pts',(-19.096452344443,14.1081177718604,132.645025662247)) ;
#150130=CARTESIAN_POINT('Ctrl Pts',(-19.1342305945688,13.8340180428126,
132.788508335971)) ;
#150131=CARTESIAN_POINT('Ctrl Pts',(-19.1467439432002,13.5302900584997,
132.858206622598)) ;
#150132=CARTESIAN_POINT('Ctrl Pts',(-19.1323635330917,13.2194243094674,
132.849285246013)) ;
#150133=CARTESIAN_POINT('Ctrl Pts',(-19.0915547199997,12.9232189359804,
132.763138594267)) ;
#150134=CARTESIAN_POINT('Ctrl Pts',(-19.0259667523677,12.6614613466154,
132.604790806233)) ;
#150135=CARTESIAN_POINT('Ctrl Pts',(-18.9405194772865,12.4560560790089,
132.38817454474)) ;
#150136=CARTESIAN_POINT('Ctrl Pts',(-18.8397676633806,12.3187614770299,
132.12698805268)) ;
#150137=CARTESIAN_POINT('Ctrl Pts',(-18.7302531161927,12.2608758941321,
131.840261818826)) ;
#150138=CARTESIAN_POINT('Ctrl Pts',(-18.6197960101115,12.2860567415008,
131.550633129398)) ;
#150139=CARTESIAN_POINT('Ctrl Pts',(-18.5143020976164,12.3936760642326,
131.275774302405)) ;
#150140=CARTESIAN_POINT('Ctrl Pts',(-18.4225005529432,12.5734426987992,
131.040533763975)) ;
#150141=CARTESIAN_POINT('Ctrl Pts',(-18.3483666747467,12.8155556665824,
130.857196460178)) ;
#150142=CARTESIAN_POINT('Ctrl Pts',(-18.2976375855543,13.1001458874772,
130.742065616185)) ;
#150143=CARTESIAN_POINT('Ctrl Pts',(-18.2727174764149,13.4082451870112,
130.70239118206)) ;
#150144=CARTESIAN_POINT('Ctrl Pts',(-18.2747208829564,13.7170001852575,
130.741310681003)) ;
#150145=CARTESIAN_POINT('Ctrl Pts',(-18.3031428718883,14.0068803460707,
130.857672223853)) ;
#150146=CARTESIAN_POINT('Ctrl Pts',(-18.3546279874812,14.2520830316222,
131.041068421816)) ;
#150147=CARTESIAN_POINT('Ctrl Pts',(-18.4249893528057,14.4388654813696,
131.279674482647)) ;
#150148=CARTESIAN_POINT('Ctrl Pts',(-18.5087523962848,14.5532758693692,
131.557517303815)) ;
#150149=CARTESIAN_POINT('Ctrl Pts',(-18.5989724091081,14.5866372914021,
131.854217352645)) ;
#150150=CARTESIAN_POINT('Ctrl Pts',(-18.688512540162,14.536325428207,132.148960312918)) ;
#150151=CARTESIAN_POINT('Ctrl Pts',(-18.7697882731236,14.4070821895425,
132.419388304922)) ;
#150152=CARTESIAN_POINT('Ctrl Pts',(-18.837264340709,14.2058492618622,132.649795674961)) ;
#150153=CARTESIAN_POINT('Ctrl Pts',(-18.8842859072995,13.9493210754263,
132.820267948791)) ;
#150154=CARTESIAN_POINT('Ctrl Pts',(-18.9072831227603,13.6560817466226,
132.920472843849)) ;
#150155=CARTESIAN_POINT('Ctrl Pts',(-18.9039153111855,13.3454214916358,
132.943747640608)) ;
#150156=CARTESIAN_POINT('Ctrl Pts',(-18.8737437347605,13.0405959101595,
132.888677922555)) ;
#150157=CARTESIAN_POINT('Ctrl Pts',(-18.8174933706068,12.7610204461784,
132.757709543441)) ;
#150158=CARTESIAN_POINT('Ctrl Pts',(-18.7398455096899,12.5320805798767,
132.56380909295)) ;
#150159=CARTESIAN_POINT('Ctrl Pts',(-18.6443213273581,12.3651154017827,
132.317940745462)) ;
#150160=CARTESIAN_POINT('Ctrl Pts',(-18.5377336770975,12.2743250187668,
132.039668340086)) ;
#150161=CARTESIAN_POINT('Ctrl Pts',(-18.426213086566,12.2660445050815,131.747170907628)) ;
#150162=CARTESIAN_POINT('Ctrl Pts',(-18.318662949734,12.3402670873944,131.465941046569)) ;
#150163=CARTESIAN_POINT('Ctrl Pts',(-18.2202545547588,12.4924310818324,
131.211652318231)) ;
#150164=CARTESIAN_POINT('Ctrl Pts',(-18.1384496981742,12.7106680082788,
131.0057297513)) ;
#150165=CARTESIAN_POINT('Ctrl Pts',(-18.0776794875304,12.9803448576749,
130.861345367367)) ;
#150166=CARTESIAN_POINT('Ctrl Pts',(-18.0419366209274,13.2833169308344,
130.790224557314)) ;
#150167=CARTESIAN_POINT('Ctrl Pts',(-18.0331437091799,13.5926826730587,
130.797434096829)) ;
#150168=CARTESIAN_POINT('Ctrl Pts',(-18.0510291214455,13.8936496800992,
130.882992090183)) ;
#150169=CARTESIAN_POINT('Ctrl Pts',(-18.0936826181807,14.1589429573028,
131.040700633816)) ;
#150170=CARTESIAN_POINT('Ctrl Pts',(-18.1569645287966,14.371150690962,131.258583540615)) ;
#150171=CARTESIAN_POINT('Ctrl Pts',(-18.2359601650018,14.5162610236172,
131.522432886244)) ;
#150172=CARTESIAN_POINT('Ctrl Pts',(-18.324804161584,14.5833063391636,131.815260245813)) ;
#150173=CARTESIAN_POINT('Ctrl Pts',(-18.4153699590213,14.5665129861826,
132.1129409694)) ;
#150174=CARTESIAN_POINT('Ctrl Pts',(-18.5006408256147,14.4685224536154,
132.39504774045)) ;
#150175=CARTESIAN_POINT('Ctrl Pts',(-18.5743747429956,14.2954966749806,
132.643565116707)) ;
#150176=CARTESIAN_POINT('Ctrl Pts',(-18.6302405909945,14.0596947072176,
132.839910707945)) ;
#150177=CARTESIAN_POINT('Ctrl Pts',(-18.6635175583225,13.7784556667528,
132.970247185244)) ;
#150178=CARTESIAN_POINT('Ctrl Pts',(-18.6709408038792,13.4704205936671,
133.025199141352)) ;
#150179=CARTESIAN_POINT('Ctrl Pts',(-18.6516378389852,13.1626907214352,
133.001667851695)) ;
#150180=CARTESIAN_POINT('Ctrl Pts',(-18.6057075222045,12.8697533437124,
132.900784883066)) ;
#150181=CARTESIAN_POINT('Ctrl Pts',(-18.5363453302047,12.618666846953,132.731185914356)) ;
#150182=CARTESIAN_POINT('Ctrl Pts',(-18.4471574026767,12.424057056317,132.503835420592)) ;
#150183=CARTESIAN_POINT('Ctrl Pts',(-18.3445263647179,12.301712900972,132.237061004765)) ;
#150184=CARTESIAN_POINT('Ctrl Pts',(-18.234308555707,12.2592124432014,131.948249300947)) ;
#150185=CARTESIAN_POINT('Ctrl Pts',(-18.1241338500386,12.300200425655,131.659524177675)) ;
#150186=CARTESIAN_POINT('Ctrl Pts',(-18.0207803153287,12.4222100084694,
131.390831333215)) ;
#150187=CARTESIAN_POINT('Ctrl Pts',(-17.9317044908737,12.6151763749812,
131.163672662444)) ;
#150188=CARTESIAN_POINT('Ctrl Pts',(-17.8617861726409,12.8667635353633,
130.99260106119)) ;
#150189=CARTESIAN_POINT('Ctrl Pts',(-17.8158506667333,13.1566082723263,
130.891398967559)) ;
#150190=CARTESIAN_POINT('Ctrl Pts',(-17.7958948224345,13.4669634672463,
130.866262027044)) ;
#150191=CARTESIAN_POINT('Ctrl Pts',(-17.8030608695675,13.7743605227785,
130.920372423503)) ;
#150192=CARTESIAN_POINT('Ctrl Pts',(-17.8359001119113,14.0556835016132,
131.049381504432)) ;
#150193=CARTESIAN_POINT('Ctrl Pts',(-17.8914209618374,14.2923698001693,
131.244711234281)) ;
#150194=CARTESIAN_POINT('Ctrl Pts',(-17.9652475904261,14.4669397818909,
131.493630765107)) ;
#150195=CARTESIAN_POINT('Ctrl Pts',(-18.050276614613,14.5658236939165,131.77497266956)) ;
#150196=CARTESIAN_POINT('Ctrl Pts',(-18.1412026892029,14.5834030857371,
132.073851921233)) ;
#150197=CARTESIAN_POINT('Ctrl Pts',(-18.2292576150982,14.5182209911816,
132.364039623745)) ;
#150198=CARTESIAN_POINT('Ctrl Pts',(-18.309103978395,14.3732473260144,132.630645865943)) ;
#150199=CARTESIAN_POINT('Ctrl Pts',(-18.3725034947101,14.1617341890797,
132.848838139851)) ;
#150200=CARTESIAN_POINT('Ctrl Pts',(-18.4154172019829,13.8968740490593,
133.007322174194)) ;
#150201=CARTESIAN_POINT('Ctrl Pts',(-18.4336530523727,13.5970562228853,
133.093807465727)) ;
#150202=CARTESIAN_POINT('Ctrl Pts',(-18.4250129097242,13.2853499830191,
133.101720033997)) ;
#150203=CARTESIAN_POINT('Ctrl Pts',(-18.3899205655734,12.9854215224893,
133.032137337284)) ;
#150204=CARTESIAN_POINT('Ctrl Pts',(-18.3295227235463,12.7145027585382,
132.888898701989)) ;
#150205=CARTESIAN_POINT('Ctrl Pts',(-18.2479735328657,12.4953423449653,
132.683727463283)) ;
#150206=CARTESIAN_POINT('Ctrl Pts',(-18.1496105042201,12.3417858317011,
132.429625686426)) ;
#150207=CARTESIAN_POINT('Ctrl Pts',(-18.0419827382182,12.2665368316973,
132.148216804111)) ;
#150208=CARTESIAN_POINT('Ctrl Pts',(-17.9308988626219,12.2735361419267,
131.856860060952)) ;
#150209=CARTESIAN_POINT('Ctrl Pts',(-17.8239987755081,12.363229877568,131.577738375418)) ;
#150210=CARTESIAN_POINT('Ctrl Pts',(-17.7284277907829,12.5286846808382,
131.331660535556)) ;
#150211=CARTESIAN_POINT('Ctrl Pts',(-17.650146576631,12.7579693374739,131.13607184284)) ;
#150212=CARTESIAN_POINT('Ctrl Pts',(-17.5939037235543,13.0352201558529,
131.00490973182)) ;
#150213=CARTESIAN_POINT('Ctrl Pts',(-17.5631487906681,13.3405827861553,
130.948233479656)) ;
#150214=CARTESIAN_POINT('Ctrl Pts',(-17.5593786927079,13.6512270836361,
130.970318968351)) ;
#150215=CARTESIAN_POINT('Ctrl Pts',(-17.5820478450478,13.9458586294117,
131.069672284471)) ;
#150216=CARTESIAN_POINT('Ctrl Pts',(-17.6289872140888,14.2033946145398,
131.239982776778)) ;
#150217=CARTESIAN_POINT('Ctrl Pts',(-17.6957349745663,14.4040390929878,
131.468022433177)) ;
#150218=CARTESIAN_POINT('Ctrl Pts',(-17.7769298692206,14.5350227299355,
131.738273550231)) ;
#150219=CARTESIAN_POINT('Ctrl Pts',(-17.8667505697732,14.5864958770583,
132.033957919984)) ;
#150220=CARTESIAN_POINT('Ctrl Pts',(-17.9565884461338,14.5544169288515,
132.329387676471)) ;
#150221=CARTESIAN_POINT('Ctrl Pts',(-18.0405609017563,14.4414134411267,
132.607855045807)) ;
#150222=CARTESIAN_POINT('Ctrl Pts',(-18.1113732977568,14.2551029687745,
132.84787133366)) ;
#150223=CARTESIAN_POINT('Ctrl Pts',(-18.16319522583,14.0100365363148,133.032311388359)) ;
#150224=CARTESIAN_POINT('Ctrl Pts',(-18.191835749466,13.7214335689568,133.149211235179)) ;
#150225=CARTESIAN_POINT('Ctrl Pts',(-18.1943014025765,13.4135493064467,
133.189407327766)) ;
#150226=CARTESIAN_POINT('Ctrl Pts',(-18.1697502158279,13.1045553590735,
133.150886523563)) ;
#150227=CARTESIAN_POINT('Ctrl Pts',(-18.1194362562685,12.8197359183053,
133.036936233067)) ;
#150228=CARTESIAN_POINT('Ctrl Pts',(-18.045466735335,12.5762135336046,132.854155324105)) ;
#150229=CARTESIAN_POINT('Ctrl Pts',(-17.9535452105021,12.3952020079458,
132.618664061262)) ;
#150230=CARTESIAN_POINT('Ctrl Pts',(-17.8485836535312,12.2871509240411,
132.345226650551)) ;
#150231=CARTESIAN_POINT('Ctrl Pts',(-17.7383571681942,12.260566124011,132.056214410167)) ;
#150232=CARTESIAN_POINT('Ctrl Pts',(-17.6284396914457,12.3174695873532,
131.768413290461)) ;
#150233=CARTESIAN_POINT('Ctrl Pts',(-17.5276588111919,12.453509519007,131.5070919687)) ;
#150234=CARTESIAN_POINT('Ctrl Pts',(-17.441706070518,12.6588730452131,131.289115738783)) ;
#150235=CARTESIAN_POINT('Ctrl Pts',(-17.376196852656,12.918573180631,131.13080952964)) ;
#150236=CARTESIAN_POINT('Ctrl Pts',(-17.3348968149211,13.2144046243544,
131.043242092145)) ;
#150237=CARTESIAN_POINT('Ctrl Pts',(-17.3200920505239,13.5255440796009,
131.033114858903)) ;
#150238=CARTESIAN_POINT('Ctrl Pts',(-17.3321967590095,13.829753908523,131.101637331332)) ;
#150239=CARTESIAN_POINT('Ctrl Pts',(-17.3697701983736,14.1049217078337,
131.244596755897)) ;
#150240=CARTESIAN_POINT('Ctrl Pts',(-17.4288267699135,14.3298723137222,
131.450097233909)) ;
#150241=CARTESIAN_POINT('Ctrl Pts',(-17.5053580167981,14.4915527560892,
131.706928465452)) ;
#150242=CARTESIAN_POINT('Ctrl Pts',(-17.592352901495,14.5755974314799,131.994185295194)) ;
#150243=CARTESIAN_POINT('Ctrl Pts',(-17.6827508417145,14.5774288452973,
132.291266219485)) ;
#150244=CARTESIAN_POINT('Ctrl Pts',(-17.7700634635431,14.4968431861705,
132.579456392972)) ;
#150245=CARTESIAN_POINT('Ctrl Pts',(-17.8471469337488,14.338559634622,132.837867370615)) ;
#150246=CARTESIAN_POINT('Ctrl Pts',(-17.9072657239944,14.1152211662258,
133.046597266871)) ;
#150247=CARTESIAN_POINT('Ctrl Pts',(-17.9457240149027,13.8419815633955,
133.192097761732)) ;
#150248=CARTESIAN_POINT('Ctrl Pts',(-17.9589569606329,13.5398086158385,
133.263788376459)) ;
#150249=CARTESIAN_POINT('Ctrl Pts',(-17.9453990657103,13.2280436814142,
133.257353253558)) ;
#150250=CARTESIAN_POINT('Ctrl Pts',(-17.905043823452,12.9300591800615,133.172663322675)) ;
#150251=CARTESIAN_POINT('Ctrl Pts',(-17.8403773368806,12.6684085006953,
133.016841323401)) ;
#150252=CARTESIAN_POINT('Ctrl Pts',(-17.7553253291571,12.4608091979395,
132.801436870079)) ;
#150253=CARTESIAN_POINT('Ctrl Pts',(-17.6548315660994,12.3214093724075,
132.541022558559)) ;
#150254=CARTESIAN_POINT('Ctrl Pts',(-17.545287414388,12.2613303026755,132.25425908364)) ;
#150255=CARTESIAN_POINT('Ctrl Pts',(-17.4352053399009,12.2843254889888,
131.965601011091)) ;
#150256=CARTESIAN_POINT('Ctrl Pts',(-17.3299104259236,12.3887269550652,
131.691161540009)) ;
#150257=CARTESIAN_POINT('Ctrl Pts',(-17.237062784242,12.5673627247375,131.453060235114)) ;
#150258=CARTESIAN_POINT('Ctrl Pts',(-17.1624022535704,12.8080166646894,
131.268173285497)) ;
#150259=CARTESIAN_POINT('Ctrl Pts',(-17.1109366121169,13.0914774239872,
131.150879601895)) ;
#150260=CARTESIAN_POINT('Ctrl Pts',(-17.085215035143,13.4005589621793,131.109004255832)) ;
#150261=CARTESIAN_POINT('Ctrl Pts',(-17.0865508110795,13.7083911586178,
131.14584909413)) ;
#150262=CARTESIAN_POINT('Ctrl Pts',(-17.1141226769015,13.9985991401632,
131.259654047056)) ;
#150263=CARTESIAN_POINT('Ctrl Pts',(-17.1650584656608,14.2457812582848,
131.441505397051)) ;
#150264=CARTESIAN_POINT('Ctrl Pts',(-17.2350111236326,14.4345734163401,
131.678939485648)) ;
#150265=CARTESIAN_POINT('Ctrl Pts',(-17.3185332049843,14.5511370874347,
131.956091770258)) ;
#150266=CARTESIAN_POINT('Ctrl Pts',(-17.4083874998686,14.5867802184263,
132.251622731321)) ;
#150267=CARTESIAN_POINT('Ctrl Pts',(-17.4980680409966,14.5391948509929,
132.546773593608)) ;
#150268=CARTESIAN_POINT('Ctrl Pts',(-17.5799467374303,14.4115345503253,
132.819086492873)) ;
#150269=CARTESIAN_POINT('Ctrl Pts',(-17.6475128932711,14.2134356096031,
133.049550301058)) ;
#150270=CARTESIAN_POINT('Ctrl Pts',(-17.6953912867036,13.9582378109792,
133.22257409294)) ;
#150271=CARTESIAN_POINT('Ctrl Pts',(-17.7192157998652,13.6646543280563,
133.32532295919)) ;
#150272=CARTESIAN_POINT('Ctrl Pts',(-17.7166085475005,13.3541837462344,
133.350814052753)) ;
#150273=CARTESIAN_POINT('Ctrl Pts',(-17.6870730407865,13.0484270052538,
133.297660731118)) ;
#150274=CARTESIAN_POINT('Ctrl Pts',(-17.6318650358643,12.7694396720145,
133.169536797612)) ;
#150275=CARTESIAN_POINT('Ctrl Pts',(-17.5547367408699,12.5380418317107,
132.977228775516)) ;
#150276=CARTESIAN_POINT('Ctrl Pts',(-17.4590541050436,12.3683286468607,
132.73108001436)) ;
#150277=CARTESIAN_POINT('Ctrl Pts',(-17.3531735443108,12.276042045724,132.454716010959)) ;
#150278=CARTESIAN_POINT('Ctrl Pts',(-17.2421870088341,12.2649171865401,
132.163629145715)) ;
#150279=CARTESIAN_POINT('Ctrl Pts',(-17.1339083209122,12.3368690244089,
131.8804310438)) ;
#150280=CARTESIAN_POINT('Ctrl Pts',(-17.035054500192,12.4871141807711,131.624864749109)) ;
#150281=CARTESIAN_POINT('Ctrl Pts',(-16.9525609483888,12.7041604883304,
131.41699806149)) ;
#150282=CARTESIAN_POINT('Ctrl Pts',(-16.8913487827029,12.9721741232452,
131.271250432799)) ;
#150283=CARTESIAN_POINT('Ctrl Pts',(-16.8549145668053,13.2726901834042,
131.197919141356)) ;
#150284=CARTESIAN_POINT('Ctrl Pts',(-16.8452026953237,13.5844633646991,
131.202698812117)) ;
#150285=CARTESIAN_POINT('Ctrl Pts',(-16.8624065683868,13.8852369971297,
131.286179901398)) ;
#150286=CARTESIAN_POINT('Ctrl Pts',(-16.9041286488751,14.1508959663415,
131.441039820401)) ;
#150287=CARTESIAN_POINT('Ctrl Pts',(-16.9670321127304,14.3659569774688,
131.657939494814)) ;
#150288=CARTESIAN_POINT('Ctrl Pts',(-17.0460179767883,14.5133844128615,
131.92188643313)) ;
#150289=CARTESIAN_POINT('Ctrl Pts',(-17.1339465963916,14.5822824831324,
132.21176107558)) ;
#150290=CARTESIAN_POINT('Ctrl Pts',(-17.2247754522715,14.5684017849453,
132.510294823667)) ;
#150291=CARTESIAN_POINT('Ctrl Pts',(-17.3104806432216,14.4726240674175,
132.793731139819)) ;
#150292=CARTESIAN_POINT('Ctrl Pts',(-17.3848392552526,14.3009018680156,
133.044181149527)) ;
#150293=CARTESIAN_POINT('Ctrl Pts',(-17.4410593342651,14.06766624957,133.241418037696)) ;
#150294=CARTESIAN_POINT('Ctrl Pts',(-17.4751195477601,13.7867923876229,
133.374130221132)) ;
#150295=CARTESIAN_POINT('Ctrl Pts',(-17.4833469392014,13.4808116155242,
133.431254688991)) ;
#150296=CARTESIAN_POINT('Ctrl Pts',(-17.464747462014,13.170617767173,133.41002024296)) ;
#150297=CARTESIAN_POINT('Ctrl Pts',(-17.4194321247648,12.8770484299103,
133.310921042257)) ;
#150298=CARTESIAN_POINT('Ctrl Pts',(-17.3508127869087,12.6251910653491,
133.143425682724)) ;
#150299=CARTESIAN_POINT('Ctrl Pts',(-17.2623582572588,12.4289584805404,
132.918141206375)) ;
#150300=CARTESIAN_POINT('Ctrl Pts',(-17.159481434093,12.3038002389648,132.650826788061)) ;
#150301=CARTESIAN_POINT('Ctrl Pts',(-17.049593615255,12.2593442697271,132.36290466408)) ;
#150302=CARTESIAN_POINT('Ctrl Pts',(-16.9395766193849,12.297889877657,132.07456986564)) ;
#150303=CARTESIAN_POINT('Ctrl Pts',(-16.8361631294826,12.4169444300621,
131.80560272998)) ;
#150304=CARTESIAN_POINT('Ctrl Pts',(-16.7459877628339,12.6093773199724,
131.575465763003)) ;
#150305=CARTESIAN_POINT('Ctrl Pts',(-16.6758357276199,12.858373409298,131.403541123782)) ;
#150306=CARTESIAN_POINT('Ctrl Pts',(-16.6289825241189,13.1480449631144,
131.299749807383)) ;
#150307=CARTESIAN_POINT('Ctrl Pts',(-16.6083146433778,13.4582417774946,
131.272537046797)) ;
#150308=CARTESIAN_POINT('Ctrl Pts',(-16.6146793730458,13.7655078893865,
131.324248877105)) ;
#150309=CARTESIAN_POINT('Ctrl Pts',(-16.6468582865308,14.0483169401814,
131.451381588369)) ;
#150310=CARTESIAN_POINT('Ctrl Pts',(-16.7017047560325,14.2859989758831,
131.644677680424)) ;
#150311=CARTESIAN_POINT('Ctrl Pts',(-16.7748115336735,14.4624790270523,
131.891400883999)) ;
#150312=CARTESIAN_POINT('Ctrl Pts',(-16.8601571097669,14.5642183790962,
132.173890767713)) ;
#150313=CARTESIAN_POINT('Ctrl Pts',(-16.9504675640042,14.5841609537885,
132.470754565741)) ;
#150314=CARTESIAN_POINT('Ctrl Pts',(-17.0392368807652,14.5209707585958,
132.763245331408)) ;
#150315=CARTESIAN_POINT('Ctrl Pts',(-17.1188682502455,14.3791779816594,
133.02897653721)) ;
#150316=CARTESIAN_POINT('Ctrl Pts',(-17.1831683138652,14.1688152035408,
133.249950274552)) ;
#150317=CARTESIAN_POINT('Ctrl Pts',(-17.2266852823441,13.905195794164,133.410184160549)) ;
#150318=CARTESIAN_POINT('Ctrl Pts',(-17.2456647537425,13.6071501662918,
133.49873274648)) ;
#150319=CARTESIAN_POINT('Ctrl Pts',(-17.2379795146638,13.2953844839231,
133.509443223532)) ;
#150320=CARTESIAN_POINT('Ctrl Pts',(-17.2033907892679,12.9930170511922,
133.441539336307)) ;
#150321=CARTESIAN_POINT('Ctrl Pts',(-17.1439345398936,12.7222274559466,
133.300891034768)) ;
#150322=CARTESIAN_POINT('Ctrl Pts',(-17.0627161251801,12.5005441594065,
133.096795193658)) ;
#150323=CARTESIAN_POINT('Ctrl Pts',(-16.9647728460759,12.3451353729422,
132.843896282304)) ;
#150324=CARTESIAN_POINT('Ctrl Pts',(-16.8573151177925,12.2674914409628,
132.562993056805)) ;
#150325=CARTESIAN_POINT('Ctrl Pts',(-16.745916203242,12.2722652498167,132.270803885411)) ;
#150326=CARTESIAN_POINT('Ctrl Pts',(-16.6389119181345,12.3599738059354,
131.99135443123)) ;
#150327=CARTESIAN_POINT('Ctrl Pts',(-16.5433418169087,12.5226377882888,
131.745135458993)) ;
#150328=CARTESIAN_POINT('Ctrl Pts',(-16.4642169436847,12.7508221881861,
131.547177756897)) ;
#150329=CARTESIAN_POINT('Ctrl Pts',(-16.4072037644663,13.0279564689842,
131.413863382206)) ;
#150330=CARTESIAN_POINT('Ctrl Pts',(-16.375865594437,13.3323086828982,131.355420914037)) ;
#150331=CARTESIAN_POINT('Ctrl Pts',(-16.3713312480991,13.6420773453948,
131.375166298422)) ;
#150332=CARTESIAN_POINT('Ctrl Pts',(-16.393213710967,13.9374077798728,131.472211358002)) ;
#150333=CARTESIAN_POINT('Ctrl Pts',(-16.4394591109491,14.1965319026708,
131.640502803954)) ;
#150334=CARTESIAN_POINT('Ctrl Pts',(-16.506134908146,14.3999725565714,131.868522260138)) ;
#150335=CARTESIAN_POINT('Ctrl Pts',(-16.5866083664928,14.5320840030957,
132.136487051069)) ;
#150336=CARTESIAN_POINT('Ctrl Pts',(-16.6761358475962,14.5862914480512,
132.43126381356)) ;
#150337=CARTESIAN_POINT('Ctrl Pts',(-16.766552339434,14.5562373226541,132.728571335906)) ;
#150338=CARTESIAN_POINT('Ctrl Pts',(-16.850279782507,14.4460760144195,133.006119112852)) ;
#150339=CARTESIAN_POINT('Ctrl Pts',(-16.9218856051312,14.2613118721967,
133.248574536486)) ;
#150340=CARTESIAN_POINT('Ctrl Pts',(-16.9743127705121,14.0168342944474,
133.434863473203)) ;
#150341=CARTESIAN_POINT('Ctrl Pts',(-17.003524928258,13.7314084897265,133.553180813754)) ;
#150342=CARTESIAN_POINT('Ctrl Pts',(-17.0068016806013,13.421392773908,133.596014845283)) ;
#150343=CARTESIAN_POINT('Ctrl Pts',(-16.9830906971717,13.1138964793829,
133.559748732295)) ;
#150344=CARTESIAN_POINT('Ctrl Pts',(-16.9334554372867,12.8273574977414,
133.447863646689)) ;
#150345=CARTESIAN_POINT('Ctrl Pts',(-16.8600151228304,12.5821904329902,
133.26664901627)) ;
#150346=CARTESIAN_POINT('Ctrl Pts',(-16.7684365133115,12.3992406705926,
133.032190342738)) ;
#150347=CARTESIAN_POINT('Ctrl Pts',(-16.6641078345942,12.289263542394,132.76048675717)) ;
#150348=CARTESIAN_POINT('Ctrl Pts',(-16.553718708184,12.260188272694,132.47107268329)) ;
#150349=CARTESIAN_POINT('Ctrl Pts',(-16.4440558695573,12.3144490228481,
132.183892674013)) ;
#150350=CARTESIAN_POINT('Ctrl Pts',(-16.3428146204697,12.4481500069378,
131.921255741908)) ;
#150351=CARTESIAN_POINT('Ctrl Pts',(-16.2562794181923,12.6515764939739,
131.701583750563)) ;
#150352=CARTESIAN_POINT('Ctrl Pts',(-16.1897800646174,12.9112089841373,
131.540547278658)) ;
#150353=CARTESIAN_POINT('Ctrl Pts',(-16.1478371964019,13.2069679929226,
131.451160112557)) ;
#150354=CARTESIAN_POINT('Ctrl Pts',(-16.1323491810072,13.5165269909875,
131.438878337385)) ;
#150355=CARTESIAN_POINT('Ctrl Pts',(-16.143795189693,13.8224960289794,131.505620155425)) ;
#150356=CARTESIAN_POINT('Ctrl Pts',(-16.1805498235764,14.0973149318537,
131.646016489691)) ;
#150357=CARTESIAN_POINT('Ctrl Pts',(-16.23913426865,14.3244517336708,131.850209657004)) ;
#150358=CARTESIAN_POINT('Ctrl Pts',(-16.3151462424385,14.4877799140032,
132.105462744924)) ;
#150359=CARTESIAN_POINT('Ctrl Pts',(-16.401805129707,14.5742904717488,132.391701051472)) ;
#150360=CARTESIAN_POINT('Ctrl Pts',(-16.492585860518,14.5785355539825,132.690040136978)) ;
#150361=CARTESIAN_POINT('Ctrl Pts',(-16.5799680048269,14.4999983626793,
132.978398341277)) ;
#150362=CARTESIAN_POINT('Ctrl Pts',(-16.6571136565244,14.3447574910545,
133.236831164026)) ;
#150363=CARTESIAN_POINT('Ctrl Pts',(-16.7180463250183,14.1223925047645,
133.448063876043)) ;
#150364=CARTESIAN_POINT('Ctrl Pts',(-16.7571048654271,13.8510687474612,
133.595226610732)) ;
#150365=CARTESIAN_POINT('Ctrl Pts',(-16.7711828604265,13.5484337104113,
133.66950419217)) ;
#150366=CARTESIAN_POINT('Ctrl Pts',(-16.758359396265,13.237024252248,133.66516822926)) ;
#150367=CARTESIAN_POINT('Ctrl Pts',(-16.7189312234401,12.9391312355254,
133.583092750207)) ;
#150368=CARTESIAN_POINT('Ctrl Pts',(-16.6549202670634,12.6756661013292,
133.429230049725)) ;
#150369=CARTESIAN_POINT('Ctrl Pts',(-16.5701642224514,12.465702834837,133.214777187573)) ;
#150370=CARTESIAN_POINT('Ctrl Pts',(-16.4700761526249,12.3244745737951,
132.955522794711)) ;
#150371=CARTESIAN_POINT('Ctrl Pts',(-16.3611846564961,12.261923279364,132.670519137022)) ;
#150372=CARTESIAN_POINT('Ctrl Pts',(-16.2502670389918,12.2825882232678,
132.379655456716)) ;
#150373=CARTESIAN_POINT('Ctrl Pts',(-16.1450742603988,12.3846500947886,
132.105406192287)) ;
#150374=CARTESIAN_POINT('Ctrl Pts',(-16.0517868994275,12.5611186866008,
131.866013505962)) ;
#150375=CARTESIAN_POINT('Ctrl Pts',(-15.9765085489102,12.8001288642586,
131.679313704519)) ;
#150376=CARTESIAN_POINT('Ctrl Pts',(-15.9242993403601,13.0829558196603,
131.559890650521)) ;
#150377=CARTESIAN_POINT('Ctrl Pts',(-15.8978264794063,13.3903655314665,
131.51568156666)) ;
#150378=CARTESIAN_POINT('Ctrl Pts',(-15.8983687766488,13.7001366120665,
131.550391855689)) ;
#150379=CARTESIAN_POINT('Ctrl Pts',(-15.9250955464469,13.9898881855453,
131.661569200131)) ;
#150380=CARTESIAN_POINT('Ctrl Pts',(-15.9754500848428,14.2391934633215,
131.841798893272)) ;
#150381=CARTESIAN_POINT('Ctrl Pts',(-16.0448273016722,14.4298567311308,
132.077514083438)) ;
#150382=CARTESIAN_POINT('Ctrl Pts',(-16.1285516719131,14.549247146468,132.355452702111)) ;
#150383=CARTESIAN_POINT('Ctrl Pts',(-16.2180137706109,14.5868020953667,
132.649720204288)) ;
#150384=CARTESIAN_POINT('Ctrl Pts',(-16.3077295677544,14.5417975168182,
132.944943445594)) ;
#150385=CARTESIAN_POINT('Ctrl Pts',(-16.3899638321532,14.4162088309709,
133.218316186842)) ;
#150386=CARTESIAN_POINT('Ctrl Pts',(-16.4579840959181,14.2204083444341,
133.45005782146)) ;
#150387=CARTESIAN_POINT('Ctrl Pts',(-16.5067331774277,13.9647701488693,
133.625846053146)) ;
#150388=CARTESIAN_POINT('Ctrl Pts',(-16.5310706681232,13.6739289079279,
133.72986283775)) ;
#150389=CARTESIAN_POINT('Ctrl Pts',(-16.5292510761197,13.3623285568061,
133.757801584865)) ;
#150390=CARTESIAN_POINT('Ctrl Pts',(-16.500529680411,13.0574725166072,133.706883722544)) ;
#150391=CARTESIAN_POINT('Ctrl Pts',(-16.4461335867092,12.7770677802999,
133.581145035692)) ;
#150392=CARTESIAN_POINT('Ctrl Pts',(-16.3689064255398,12.5427865648713,
133.388787147722)) ;
#150393=CARTESIAN_POINT('Ctrl Pts',(-16.274842442146,12.3731888767337,133.14694664983)) ;
#150394=CARTESIAN_POINT('Ctrl Pts',(-16.1686014384922,12.2773794535172,
132.869740353412)) ;
#150395=CARTESIAN_POINT('Ctrl Pts',(-16.0573374850372,12.2641879567031,
132.577928332093)) ;
#150396=CARTESIAN_POINT('Ctrl Pts',(-15.9492700825767,12.3335960199066,
132.295231932845)) ;
#150397=CARTESIAN_POINT('Ctrl Pts',(-15.850023314516,12.481561593043,132.038517373115)) ;
#150398=CARTESIAN_POINT('Ctrl Pts',(-15.7669381618391,12.6968286383091,
131.82892749163)) ;
#150399=CARTESIAN_POINT('Ctrl Pts',(-15.7049421360384,12.9642189214816,
131.680963788946)) ;
#150400=CARTESIAN_POINT('Ctrl Pts',(-15.6677820428019,13.2637553890215,
131.605469326867)) ;
#150401=CARTESIAN_POINT('Ctrl Pts',(-15.6573682454385,13.576692280422,131.608329578821)) ;
#150402=CARTESIAN_POINT('Ctrl Pts',(-15.6736161246103,13.8753721133811,
131.688705955498)) ;
#150403=CARTESIAN_POINT('Ctrl Pts',(-15.7149268964637,14.1446744627024,
131.842646209192)) ;
#150404=CARTESIAN_POINT('Ctrl Pts',(-15.7772771295284,14.36064855191,132.057858656137)) ;
#150405=CARTESIAN_POINT('Ctrl Pts',(-15.8555887750143,14.5100785493016,
132.319731780122)) ;
#150406=CARTESIAN_POINT('Ctrl Pts',(-15.9440283856208,14.5815775750292,
132.611354939558)) ;
#150407=CARTESIAN_POINT('Ctrl Pts',(-16.0342190695844,14.5700420013307,
132.907770831432)) ;
#150408=CARTESIAN_POINT('Ctrl Pts',(-16.1205674523234,14.4761038026697,
133.193256248184)) ;
#150409=CARTESIAN_POINT('Ctrl Pts',(-16.1949655569345,14.307434697937,133.443625750521)) ;
#150410=CARTESIAN_POINT('Ctrl Pts',(-16.2522128289874,14.0735726732338,
133.644168593153)) ;
#150411=CARTESIAN_POINT('Ctrl Pts',(-16.286567085948,13.7966475167134,133.777379895401)) ;
#150412=CARTESIAN_POINT('Ctrl Pts',(-16.2957241267505,13.4894705902725,
133.83741554962)) ;
#150413=CARTESIAN_POINT('Ctrl Pts',(-16.277915731801,13.1800818840159,133.818379729644)) ;
#150414=CARTESIAN_POINT('Ctrl Pts',(-16.233382384928,12.8853356480997,133.721598421941)) ;
#150415=CARTESIAN_POINT('Ctrl Pts',(-16.1653339151511,12.6318026190054,
133.555801564048)) ;
#150416=CARTESIAN_POINT('Ctrl Pts',(-16.0773393373828,12.4337108597235,
133.331871256496)) ;
#150417=CARTESIAN_POINT('Ctrl Pts',(-15.9749977446359,12.3064394733644,
133.066053638971)) ;
#150418=CARTESIAN_POINT('Ctrl Pts',(-15.8649060852758,12.2594672530152,
132.777636639602)) ;
#150419=CARTESIAN_POINT('Ctrl Pts',(-15.7549091018377,12.2954707768407,
132.489316203072)) ;
#150420=CARTESIAN_POINT('Ctrl Pts',(-15.6506039958486,12.4135506766909,
132.21796505975)) ;
#150421=CARTESIAN_POINT('Ctrl Pts',(-15.5611531746748,12.6014761735562,
131.989492941064)) ;
#150422=CARTESIAN_POINT('Ctrl Pts',(-15.4896861055833,12.8505488639341,
131.813985346776)) ;
#150423=CARTESIAN_POINT('Ctrl Pts',(-15.4422008192573,13.1393106596108,
131.708325362233)) ;
#150424=CARTESIAN_POINT('Ctrl Pts',(-15.4207351710859,13.4495612540633,
131.678820753104)) ;
#150425=CARTESIAN_POINT('Ctrl Pts',(-15.426337100979,13.7566530786408,131.728242130976)) ;
#150426=CARTESIAN_POINT('Ctrl Pts',(-15.4577656885259,14.0404143241467,
131.853175929721)) ;
#150427=CARTESIAN_POINT('Ctrl Pts',(-15.5119856948056,14.2798567692648,
132.044648848123)) ;
#150428=CARTESIAN_POINT('Ctrl Pts',(-15.5850085796815,14.458860759646,132.291272848204)) ;
#150429=CARTESIAN_POINT('Ctrl Pts',(-15.6696256144766,14.5622468001176,
132.57144381166)) ;
#150430=CARTESIAN_POINT('Ctrl Pts',(-15.7602275007173,14.5847589339645,
132.869291645903)) ;
#150431=CARTESIAN_POINT('Ctrl Pts',(-15.8488837215895,14.5239999698819,
133.161349516975)) ;
#150432=CARTESIAN_POINT('Ctrl Pts',(-15.9289853890852,14.3842926564904,
133.428499684631)) ;
#150433=CARTESIAN_POINT('Ctrl Pts',(-15.9937731842162,14.1758059968765,
133.650879354936)) ;
#150434=CARTESIAN_POINT('Ctrl Pts',(-16.0380364943461,13.9130885413349,
133.813345394859)) ;
#150435=CARTESIAN_POINT('Ctrl Pts',(-16.0576964829059,13.615158117942,133.903937919873)) ;
#150436=CARTESIAN_POINT('Ctrl Pts',(-16.050810517652,13.3050555466183,133.916814091063)) ;
#150437=CARTESIAN_POINT('Ctrl Pts',(-16.0170723190309,13.0018872896554,
133.85141230611)) ;
#150438=CARTESIAN_POINT('Ctrl Pts',(-15.9581350119924,12.7291798994599,
133.71236767288)) ;
#150439=CARTESIAN_POINT('Ctrl Pts',(-15.8775156954164,12.5061727549264,
133.50998953017)) ;
#150440=CARTESIAN_POINT('Ctrl Pts',(-15.7803572447695,12.3489726739453,
133.259264679238)) ;
#150441=CARTESIAN_POINT('Ctrl Pts',(-15.6726919794867,12.2685650260664,
132.977885098156)) ;
#150442=CARTESIAN_POINT('Ctrl Pts',(-15.5617033607869,12.2709027283838,
132.686768675325)) ;
#150443=CARTESIAN_POINT('Ctrl Pts',(-15.4544229833051,12.3558099877511,
132.406517587879)) ;
#150444=CARTESIAN_POINT('Ctrl Pts',(-15.3579664336319,12.5172181290402,
132.157871619068)) ;
#150445=CARTESIAN_POINT('Ctrl Pts',(-15.2785412794525,12.7432704544133,
131.958946428183)) ;
#150446=CARTESIAN_POINT('Ctrl Pts',(-15.220940870672,13.0180146572784,131.823789499591)) ;
#150447=CARTESIAN_POINT('Ctrl Pts',(-15.1886061274104,13.3228198676384,
131.762550075545)) ;
#150448=CARTESIAN_POINT('Ctrl Pts',(-15.1832971970252,13.6334361388998,
131.780107071404)) ;
#150449=CARTESIAN_POINT('Ctrl Pts',(-15.2044737072776,13.9294162640336,
131.875083706159)) ;
#150450=CARTESIAN_POINT('Ctrl Pts',(-15.2499149788137,14.1891569843553,
132.040930237774)) ;
#150451=CARTESIAN_POINT('Ctrl Pts',(-15.3159882637482,14.3946401780078,
132.267182223925)) ;
#150452=CARTESIAN_POINT('Ctrl Pts',(-15.3964422708231,14.529556883976,132.535221020513)) ;
#150453=CARTESIAN_POINT('Ctrl Pts',(-15.4859266051064,14.5858061305694,
132.829902483417)) ;
#150454=CARTESIAN_POINT('Ctrl Pts',(-15.575921095585,14.5585141813688,133.125790617441)) ;
#150455=CARTESIAN_POINT('Ctrl Pts',(-15.660393004627,14.4500372288901,133.405700992678)) ;
#150456=CARTESIAN_POINT('Ctrl Pts',(-15.7320322458967,14.2682020295539,
133.648062095577)) ;
#150457=CARTESIAN_POINT('Ctrl Pts',(-15.7853081761487,14.0250734212292,
133.836897476779)) ;
#150458=CARTESIAN_POINT('Ctrl Pts',(-15.8153071073788,13.7389393527222,
133.957688978132)) ;
#150459=CARTESIAN_POINT('Ctrl Pts',(-15.8192713850197,13.4311036991076,
134.002333051418)) ;
#150460=CARTESIAN_POINT('Ctrl Pts',(-15.7964833343467,13.1229020252546,
133.968793735116)) ;
#150461=CARTESIAN_POINT('Ctrl Pts',(-15.7470151225786,12.8333723826346,
133.857660705835)) ;
#150462=CARTESIAN_POINT('Ctrl Pts',(-15.6749499819258,12.5895126808553,
133.680093919526)) ;
#150463=CARTESIAN_POINT('Ctrl Pts',(-15.5835820228647,12.4035405044014,
133.44638124524)) ;
#150464=CARTESIAN_POINT('Ctrl Pts',(-15.4795359363878,12.2914040543739,
133.175493546379)) ;
#150465=CARTESIAN_POINT('Ctrl Pts',(-15.3691067042144,12.2598122660064,
132.885999507054)) ;
#150466=CARTESIAN_POINT('Ctrl Pts',(-15.2592491515748,12.3118570092467,
132.598270697777)) ;
#150467=CARTESIAN_POINT('Ctrl Pts',(-15.1578846173847,12.4430958477667,
132.335205909277)) ;
#150468=CARTESIAN_POINT('Ctrl Pts',(-15.0707569923601,12.6447072106669,
132.113822737163)) ;
#150469=CARTESIAN_POINT('Ctrl Pts',(-15.0036348239267,12.9030426443817,
131.950970459127)) ;
#150470=CARTESIAN_POINT('Ctrl Pts',(-14.9609666584116,13.1970328357363,
131.859359722779)) ;
#150471=CARTESIAN_POINT('Ctrl Pts',(-14.9446463507845,13.508431210418,131.844863395647)) ;
#150472=CARTESIAN_POINT('Ctrl Pts',(-14.955182994799,13.8121186853756,131.908635532583)) ;
#150473=CARTESIAN_POINT('Ctrl Pts',(-14.9913474493756,14.0900961116511,
132.047534065062)) ;
#150474=CARTESIAN_POINT('Ctrl Pts',(-15.0493834153807,14.3187298480659,
132.250109058127)) ;
#150475=CARTESIAN_POINT('Ctrl Pts',(-15.1252001144207,14.4844226501879,
132.504882601538)) ;
#150476=CARTESIAN_POINT('Ctrl Pts',(-15.2112957458124,14.5727758610145,
132.789337009017)) ;
#150477=CARTESIAN_POINT('Ctrl Pts',(-15.3020656236423,14.5796460652876,
133.087650648783)) ;
#150478=CARTESIAN_POINT('Ctrl Pts',(-15.3896841845459,14.5035866280562,
133.3767061857)) ;
#150479=CARTESIAN_POINT('Ctrl Pts',(-15.4675294606947,14.3497064261521,
133.637322714956)) ;
#150480=CARTESIAN_POINT('Ctrl Pts',(-15.5288442157173,14.1291331402223,
133.849621128442)) ;
#150481=CARTESIAN_POINT('Ctrl Pts',(-15.5684922654212,13.8597728320795,
133.998415963195)) ;
#150482=CARTESIAN_POINT('Ctrl Pts',(-15.58336190046,13.5574625507345,134.075038663256)) ;
#150483=CARTESIAN_POINT('Ctrl Pts',(-15.5713632930057,13.2463367213565,
134.073073116115)) ;
#150484=CARTESIAN_POINT('Ctrl Pts',(-15.5326175841816,12.9472974934633,
133.993046368162)) ;
#150485=CARTESIAN_POINT('Ctrl Pts',(-15.4695006632167,12.6832079210241,
133.841696695539)) ;
#150486=CARTESIAN_POINT('Ctrl Pts',(-15.38489066345,12.4704983369195,133.62782581185)) ;
#150487=CARTESIAN_POINT('Ctrl Pts',(-15.2855041099453,12.3276823761117,
133.370498419458)) ;
#150488=CARTESIAN_POINT('Ctrl Pts',(-15.1765599844448,12.2625925296001,
133.085412552406)) ;
#150489=CARTESIAN_POINT('Ctrl Pts',(-15.0659710389737,12.2806191987991,
132.795391506155)) ;
#150490=CARTESIAN_POINT('Ctrl Pts',(-14.959826977886,12.3809214254249,132.518577452134)) ;
#150491=CARTESIAN_POINT('Ctrl Pts',(-14.8661523667106,12.5560400663307,
132.278075298556)) ;
#150492=CARTESIAN_POINT('Ctrl Pts',(-14.7907697004394,12.7918900929914,
132.090851846458)) ;
#150493=CARTESIAN_POINT('Ctrl Pts',(-14.7376403432757,13.0744209302394,
131.968838267981)) ;
#150494=CARTESIAN_POINT('Ctrl Pts',(-14.7104300876091,13.3812416408414,
131.922450614359)) ;
#150495=CARTESIAN_POINT('Ctrl Pts',(-14.7101971910909,13.6920796910028,
131.954983498533)) ;
#150496=CARTESIAN_POINT('Ctrl Pts',(-14.7363062855789,13.9824941646698,
132.064351689695)) ;
#150497=CARTESIAN_POINT('Ctrl Pts',(-14.7857702497481,14.2323227439513,
132.24183650497)) ;
#150498=CARTESIAN_POINT('Ctrl Pts',(-14.8551154475838,14.4258243504284,
132.477660321935)) ;
#150499=CARTESIAN_POINT('Ctrl Pts',(-14.937793900891,14.5465247241855,132.752243575491)) ;
#150500=CARTESIAN_POINT('Ctrl Pts',(-15.0279945492941,14.5869806831231,
133.048986776495)) ;
#150501=CARTESIAN_POINT('Ctrl Pts',(-15.1173109934759,14.5442058467449,
133.342856019278)) ;
#150502=CARTESIAN_POINT('Ctrl Pts',(-15.2000430741247,14.4209679616749,
133.617739309619)) ;
#150503=CARTESIAN_POINT('Ctrl Pts',(-15.2687315291286,14.2257906653135,
133.851574766913)) ;
#150504=CARTESIAN_POINT('Ctrl Pts',(-15.3176437052182,13.9741287874761,
134.027505853864)) ;
#150505=CARTESIAN_POINT('Ctrl Pts',(-15.3429679172076,13.6829512743861,
134.134561979873)) ;
#150506=CARTESIAN_POINT('Ctrl Pts',(-15.3419099139476,13.3714665722058,
134.164728515353)) ;
#150507=CARTESIAN_POINT('Ctrl Pts',(-15.3138886729906,13.0656059038766,
134.115919871799)) ;
#150508=CARTESIAN_POINT('Ctrl Pts',(-15.2603010980268,12.7850335054103,
133.992449867698)) ;
#150509=CARTESIAN_POINT('Ctrl Pts',(-15.1840570554085,12.54966734435,133.802845091161)) ;
#150510=CARTESIAN_POINT('Ctrl Pts',(-15.0897673247278,12.3766688899815,
133.560585713602)) ;
#150511=CARTESIAN_POINT('Ctrl Pts',(-14.9837573750352,12.2789529397111,
133.284042602105)) ;
#150512=CARTESIAN_POINT('Ctrl Pts',(-14.8727227918643,12.2634413447035,
132.992846291171)) ;
#150513=CARTESIAN_POINT('Ctrl Pts',(-14.7644615600363,12.3304156583785,
132.709585444456)) ;
#150514=CARTESIAN_POINT('Ctrl Pts',(-14.6645328719311,12.477034323666,132.450999584505)) ;
#150515=CARTESIAN_POINT('Ctrl Pts',(-14.5813805381505,12.6896429302191,
132.241046767438)) ;
#150516=CARTESIAN_POINT('Ctrl Pts',(-14.5186828849514,12.9554490393123,
132.091011360375)) ;
#150517=CARTESIAN_POINT('Ctrl Pts',(-14.4807212473634,13.2546654169279,
132.013213880204)) ;
#150518=CARTESIAN_POINT('Ctrl Pts',(-14.4694798018736,13.5672373629207,
132.013615571884)) ;
#150519=CARTESIAN_POINT('Ctrl Pts',(-14.4850511399121,13.867352650113,132.092113461199)) ;
#150520=CARTESIAN_POINT('Ctrl Pts',(-14.5254309896077,14.1367234867938,
132.243171857793)) ;
#150521=CARTESIAN_POINT('Ctrl Pts',(-14.5877190733466,14.3561275745404,
132.458465397783)) ;
#150522=CARTESIAN_POINT('Ctrl Pts',(-14.665301266002,14.5065131149989,132.718028260505)) ;
#150523=CARTESIAN_POINT('Ctrl Pts',(-14.7533173483588,14.5806176797064,
133.008340016427)) ;
#150524=CARTESIAN_POINT('Ctrl Pts',(-14.8438421700134,14.5715967155624,
133.305843094671)) ;
#150525=CARTESIAN_POINT('Ctrl Pts',(-14.9304491532105,14.4799161202559,
133.592090673458)) ;
#150526=CARTESIAN_POINT('Ctrl Pts',(-15.0052826955154,14.3130126833991,
133.843758445213)) ;
#150527=CARTESIAN_POINT('Ctrl Pts',(-15.0628752850329,14.0821692542283,
134.045132020763)) ;
#150528=CARTESIAN_POINT('Ctrl Pts',(-15.0982104834664,13.8046646113754,
134.181420036656)) ;
#150529=CARTESIAN_POINT('Ctrl Pts',(-15.1080300159495,13.4979411637468,
134.243381047743)) ;
#150530=CARTESIAN_POINT('Ctrl Pts',(-15.0909992445679,13.1889484555023,
134.226561548948)) ;
#150531=CARTESIAN_POINT('Ctrl Pts',(-15.0473604790679,12.8939178939325,
134.132324580271)) ;
#150532=CARTESIAN_POINT('Ctrl Pts',(-14.9796563895563,12.6378239616322,
133.967682652965)) ;
#150533=CARTESIAN_POINT('Ctrl Pts',(-14.8921232379636,12.4382802323548,
133.745083826517)) ;
#150534=CARTESIAN_POINT('Ctrl Pts',(-14.7905512472213,12.3092349725469,
133.481375904344)) ;
#150535=CARTESIAN_POINT('Ctrl Pts',(-14.6802035483952,12.2595575244022,
133.192325666085)) ;
#150536=CARTESIAN_POINT('Ctrl Pts',(-14.5703130707885,12.2934341290355,
132.904265169207)) ;
#150537=CARTESIAN_POINT('Ctrl Pts',(-14.4662452413034,12.4080333821748,
132.63341243339)) ;
#150538=CARTESIAN_POINT('Ctrl Pts',(-14.3752794576045,12.5960960444092,
132.400890382292)) ;
#150539=CARTESIAN_POINT('Ctrl Pts',(-14.3036377782328,12.8430835986194,
132.224736503118)) ;
#150540=CARTESIAN_POINT('Ctrl Pts',(-14.2554826671856,13.1299282695534,
132.117020119139)) ;
#150541=CARTESIAN_POINT('Ctrl Pts',(-14.2331496418005,13.4413370794651,
132.085134325359)) ;
#150542=CARTESIAN_POINT('Ctrl Pts',(-14.2380431690014,13.7480777708716,
132.132410606473)) ;
#150543=CARTESIAN_POINT('Ctrl Pts',(-14.2687349931395,14.0327532731281,
132.255184675896)) ;
#150544=CARTESIAN_POINT('Ctrl Pts',(-14.3223115413622,14.2736050674125,
132.444755998041)) ;
#150545=CARTESIAN_POINT('Ctrl Pts',(-14.3949353266048,14.4547314005176,
132.690239889969)) ;
#150546=CARTESIAN_POINT('Ctrl Pts',(-14.4791730889678,14.560267557326,132.969257871009)) ;
#150547=CARTESIAN_POINT('Ctrl Pts',(-14.5697810156274,14.5853381835963,
133.267148625969)) ;
#150548=CARTESIAN_POINT('Ctrl Pts',(-14.6586815272113,14.5268296207526,
133.559956030392)) ;
#150549=CARTESIAN_POINT('Ctrl Pts',(-14.7390790372614,14.3893358191871,
133.827950281821)) ;
#150550=CARTESIAN_POINT('Ctrl Pts',(-14.8044047562451,14.1825587760216,
134.051913962829)) ;
#150551=CARTESIAN_POINT('Ctrl Pts',(-14.8492884325481,13.9213689273391,
134.216162794773)) ;
#150552=CARTESIAN_POINT('Ctrl Pts',(-14.8696886675527,13.624244891243,134.308912651173)) ;
#150553=CARTESIAN_POINT('Ctrl Pts',(-14.8636799148611,13.3143405109537,
134.32433386635)) ;
#150554=CARTESIAN_POINT('Ctrl Pts',(-14.8303143719492,13.0084391813705,
134.260274614731)) ;
#150555=CARTESIAN_POINT('Ctrl Pts',(-14.7725318389689,12.7371910069822,
134.124294910933)) ;
#150556=CARTESIAN_POINT('Ctrl Pts',(-14.6922271432579,12.5114338941523,
133.92297148257)) ;
#150557=CARTESIAN_POINT('Ctrl Pts',(-14.5954862728848,12.3524150089363,
133.673442871905)) ;
#150558=CARTESIAN_POINT('Ctrl Pts',(-14.4878943565415,12.2696328223672,
133.392318829169)) ;
#150559=CARTESIAN_POINT('Ctrl Pts',(-14.3769613848032,12.2697667116298,
133.101346904939)) ;
#150560=CARTESIAN_POINT('Ctrl Pts',(-14.2696468649251,12.3522196481958,
132.820942570017)) ;
#150561=CARTESIAN_POINT('Ctrl Pts',(-14.1727339204591,12.5116176555494,
132.57098120525)) ;
#150562=CARTESIAN_POINT('Ctrl Pts',(-14.0927105287885,12.7360826079941,
132.370319381871)) ;
#150563=CARTESIAN_POINT('Ctrl Pts',(-14.0342994277323,13.0105745884039,
132.232891230406)) ;
#150564=CARTESIAN_POINT('Ctrl Pts',(-14.0013588827428,13.3146277352433,
132.16985008646)) ;
#150565=CARTESIAN_POINT('Ctrl Pts',(-13.9952825294897,13.6243830684314,
132.185062273086)) ;
#150566=CARTESIAN_POINT('Ctrl Pts',(-14.0157755566262,13.9217977302755,
132.278122090516)) ;
#150567=CARTESIAN_POINT('Ctrl Pts',(-14.0604892593674,14.182101761474,132.441757903395)) ;
#150568=CARTESIAN_POINT('Ctrl Pts',(-14.1259274137499,14.38941229378,132.6661239332)) ;
#150569=CARTESIAN_POINT('Ctrl Pts',(-14.2063159513169,14.5268848124279,
132.93408166804)) ;
#150570=CARTESIAN_POINT('Ctrl Pts',(-14.2953666004889,14.5852561632452,
133.227386196288)) ;
#150571=CARTESIAN_POINT('Ctrl Pts',(-14.385474115087,14.5605921487245,133.523620813497)) ;
#150572=CARTESIAN_POINT('Ctrl Pts',(-14.4703177026304,14.4542388685168,
133.804658441133)) ;
#150573=CARTESIAN_POINT('Ctrl Pts',(-14.5424565250029,14.2743936484204,
134.048484935615)) ;
#150574=CARTESIAN_POINT('Ctrl Pts',(-14.5964352897309,14.0316377347413,
134.239502626191)) ;
#150575=CARTESIAN_POINT('Ctrl Pts',(-14.6269461364899,13.748755621538,134.361523364928)) ;
#150576=CARTESIAN_POINT('Ctrl Pts',(-14.6317385626997,13.4387761369995,
134.408862066181)) ;
#150577=CARTESIAN_POINT('Ctrl Pts',(-14.6097163065701,13.1317846538023,
134.377396710751)) ;
#150578=CARTESIAN_POINT('Ctrl Pts',(-14.5609664968543,12.8410201849047,
134.268397592025)) ;
#150579=CARTESIAN_POINT('Ctrl Pts',(-14.4896923945512,12.5963885979045,
134.093052311552)) ;
#150580=CARTESIAN_POINT('Ctrl Pts',(-14.3989961430771,12.4083250169264,
133.861260268425)) ;
#150581=CARTESIAN_POINT('Ctrl Pts',(-14.2945354469835,12.2932606250205,
133.589381296788)) ;
#150582=CARTESIAN_POINT('Ctrl Pts',(-14.1847109735173,12.2596773195356,
133.301492991178)) ;
#150583=CARTESIAN_POINT('Ctrl Pts',(-14.0747870087407,12.3089369784701,
133.013549726303)) ;
#150584=CARTESIAN_POINT('Ctrl Pts',(-13.9726728971743,12.4384178929668,
132.748422319335)) ;
#150585=CARTESIAN_POINT('Ctrl Pts',(-13.8849973180957,12.6389284156292,
132.525500717228)) ;
#150586=CARTESIAN_POINT('Ctrl Pts',(-13.8177319116897,12.8936368315776,
132.361950917148)) ;
#150587=CARTESIAN_POINT('Ctrl Pts',(-13.7739215665659,13.189035253119,132.267264094376)) ;
#150588=CARTESIAN_POINT('Ctrl Pts',(-13.7569639775647,13.4997523048697,
132.250839898931)) ;
#150589=CARTESIAN_POINT('Ctrl Pts',(-13.7667722639485,13.80398082463,132.312499872932)) ;
#150590=CARTESIAN_POINT('Ctrl Pts',(-13.802078194261,14.0820720991441,132.448762814885)) ;
#150591=CARTESIAN_POINT('Ctrl Pts',(-13.8596807492491,14.3130040222785,
132.650167238859)) ;
#150592=CARTESIAN_POINT('Ctrl Pts',(-13.9347033118994,14.4800544799105,
132.902461711407)) ;
#150593=CARTESIAN_POINT('Ctrl Pts',(-14.0207960816125,14.5714591728311,
133.187010624179)) ;
#150594=CARTESIAN_POINT('Ctrl Pts',(-14.1119985592697,14.5804983969621,
133.486750014196)) ;
#150595=CARTESIAN_POINT('Ctrl Pts',(-14.1993670996661,14.5069052814483,
133.774917777498)) ;
#150596=CARTESIAN_POINT('Ctrl Pts',(-14.2774944784524,14.3557030567126,
134.036297112957)) ;
#150597=CARTESIAN_POINT('Ctrl Pts',(-14.3394840095035,14.1367620675431,
134.250604362259)) ;
#150598=CARTESIAN_POINT('Ctrl Pts',(-14.3799392246789,13.868069475113,134.40182762202)) ;
#150599=CARTESIAN_POINT('Ctrl Pts',(-14.3955136344173,13.5652243934133,
134.480626813103)) ;
#150600=CARTESIAN_POINT('Ctrl Pts',(-14.3843153384494,13.2558697743365,
134.480807322357)) ;
#150601=CARTESIAN_POINT('Ctrl Pts',(-14.3463859800688,12.9557647499979,
134.403199207339)) ;
#150602=CARTESIAN_POINT('Ctrl Pts',(-14.2837682658718,12.6900042913403,
134.253371208713)) ;
#150603=CARTESIAN_POINT('Ctrl Pts',(-14.2000145590644,12.4761056036643,
134.041887452853)) ;
#150604=CARTESIAN_POINT('Ctrl Pts',(-14.1004715127018,12.3304586966932,
133.784276677697)) ;
#150605=CARTESIAN_POINT('Ctrl Pts',(-13.9922126022772,12.2634381679405,
133.501028466864)) ;
#150606=CARTESIAN_POINT('Ctrl Pts',(-13.8813369849944,12.2788783439155,
133.210244944469)) ;
#150607=CARTESIAN_POINT('Ctrl Pts',(-13.775078356608,12.3768659519767,132.933057558503)) ;
#150608=CARTESIAN_POINT('Ctrl Pts',(-13.6809728489137,12.5495629773897,
132.691269773362)) ;
#150609=CARTESIAN_POINT('Ctrl Pts',(-13.6045565383643,12.7855771010426,
132.501248970332)) ;
#150610=CARTESIAN_POINT('Ctrl Pts',(-13.551130995295,13.0654344689711,132.378161083515)) ;
#150611=CARTESIAN_POINT('Ctrl Pts',(-13.5230559798106,13.3720088898766,
132.329274492978)) ;
#150612=CARTESIAN_POINT('Ctrl Pts',(-13.5220367594244,13.6824356605847,
132.359442967812)) ;
#150613=CARTESIAN_POINT('Ctrl Pts',(-13.5472597305976,13.9739144612511,
132.466219512344)) ;
#150614=CARTESIAN_POINT('Ctrl Pts',(-13.5965669447147,14.2268633656514,
132.643505517909)) ;
#150615=CARTESIAN_POINT('Ctrl Pts',(-13.6647515661538,14.4204385538483,
132.875611430777)) ;
#150616=CARTESIAN_POINT('Ctrl Pts',(-13.7478512385664,14.5445800995036,
133.151733148704)) ;
#150617=CARTESIAN_POINT('Ctrl Pts',(-13.837360442129,14.5868220519023,133.446227338674)) ;
#150618=CARTESIAN_POINT('Ctrl Pts',(-13.9269497874624,14.5468039096368,
133.740953745142)) ;
#150619=CARTESIAN_POINT('Ctrl Pts',(-14.010258873857,14.4251034045477,134.017640108798)) ;
#150620=CARTESIAN_POINT('Ctrl Pts',(-14.0791078279441,14.2325286601305,
134.251805282762)) ;
#150621=CARTESIAN_POINT('Ctrl Pts',(-14.1287834744318,13.9823226220566,
134.429987882651)) ;
#150622=CARTESIAN_POINT('Ctrl Pts',(-14.1548696941534,13.6900857926319,
134.539472968083)) ;
#150623=CARTESIAN_POINT('Ctrl Pts',(-14.154524247537,13.3811330388435,134.571470330088)) ;
#150624=CARTESIAN_POINT('Ctrl Pts',(-14.1273161252456,13.0742212515847,
134.525104298596)) ;
#150625=CARTESIAN_POINT('Ctrl Pts',(-14.0743300860021,12.7922256350364,
134.403436831635)) ;
#150626=CARTESIAN_POINT('Ctrl Pts',(-13.9984404651805,12.5548594605115,
134.21494790383)) ;
#150627=CARTESIAN_POINT('Ctrl Pts',(-13.9046425023917,12.3804086732527,
133.97408020415)) ;
#150628=CARTESIAN_POINT('Ctrl Pts',(-13.7993773640674,12.2809059933595,
133.699560773721)) ;
#150629=CARTESIAN_POINT('Ctrl Pts',(-13.6885089045968,12.2624888444475,
133.408811622449)) ;
#150630=CARTESIAN_POINT('Ctrl Pts',(-13.5794505161669,12.3276776788202,
133.123422025871)) ;
#150631=CARTESIAN_POINT('Ctrl Pts',(-13.4800072576751,12.4707928531316,
132.865962382066)) ;
#150632=CARTESIAN_POINT('Ctrl Pts',(-13.3957567744659,12.6823313434113,
132.652978802577)) ;
#150633=CARTESIAN_POINT('Ctrl Pts',(-13.3322501543121,12.9478030946643,
132.500677270835)) ;
#150634=CARTESIAN_POINT('Ctrl Pts',(-13.29359415217,13.2466922642525,132.420882288356)) ;
#150635=CARTESIAN_POINT('Ctrl Pts',(-13.2816622838855,13.5583771774669,
132.419178441367)) ;
#150636=CARTESIAN_POINT('Ctrl Pts',(-13.2964274275055,13.8592555730131,
132.495328464001)) ;
#150637=CARTESIAN_POINT('Ctrl Pts',(-13.3364443297289,14.130642447192,132.645467030027)) ;
#150638=CARTESIAN_POINT('Ctrl Pts',(-13.397423996239,14.3493759206944,132.856549116759)) ;
#150639=CARTESIAN_POINT('Ctrl Pts',(-13.4752202752693,14.5035317147663,
133.117028484369)) ;
#150640=CARTESIAN_POINT('Ctrl Pts',(-13.5628805610133,14.5795844939409,
133.406219517999)) ;
#150641=CARTESIAN_POINT('Ctrl Pts',(-13.6536045252838,14.5729335746648,
133.704378305314)) ;
#150642=CARTESIAN_POINT('Ctrl Pts',(-13.7401299984418,14.4838965301244,
133.990264440643)) ;
#150643=CARTESIAN_POINT('Ctrl Pts',(-13.8155852912765,14.3187458157033,
134.243832703353)) ;
#150644=CARTESIAN_POINT('Ctrl Pts',(-13.8736731440813,14.089767661644,134.446610185744)) ;
#150645=CARTESIAN_POINT('Ctrl Pts',(-13.9097250084666,13.8134083502436,
134.584993791328)) ;
#150646=CARTESIAN_POINT('Ctrl Pts',(-13.9203543833699,13.507393703558,134.649296910112)) ;
#150647=CARTESIAN_POINT('Ctrl Pts',(-13.9040592972145,13.1976577760434,
134.634692382924)) ;
#150648=CARTESIAN_POINT('Ctrl Pts',(-13.8613296465157,12.9027230155048,
134.543003893407)) ;
#150649=CARTESIAN_POINT('Ctrl Pts',(-13.794207561342,12.6448108807206,134.380117189179)) ;
#150650=CARTESIAN_POINT('Ctrl Pts',(-13.7074007923663,12.4434495892378,
134.159577368362)) ;
#150651=CARTESIAN_POINT('Ctrl Pts',(-13.6051896084249,12.3113759849424,
133.894308207864)) ;
#150652=CARTESIAN_POINT('Ctrl Pts',(-13.4961596498729,12.2599503304548,
133.608739116444)) ;
#150653=CARTESIAN_POINT('Ctrl Pts',(-13.38530707921,12.2913693198197,133.318136196378)) ;
#150654=CARTESIAN_POINT('Ctrl Pts',(-13.2812750961412,12.4038516007803,
133.047296028386)) ;
#150655=CARTESIAN_POINT('Ctrl Pts',(-13.1901071149032,12.589262648139,132.814084987751)) ;
#150656=CARTESIAN_POINT('Ctrl Pts',(-13.1177680098582,12.834296673012,132.635864585431)) ;
#150657=CARTESIAN_POINT('Ctrl Pts',(-13.0686062567482,13.122430570677,132.525456230108)) ;
#150658=CARTESIAN_POINT('Ctrl Pts',(-13.0457037121026,13.4307504343076,
132.491602073184)) ;
#150659=CARTESIAN_POINT('Ctrl Pts',(-13.0497041032677,13.7394115379672,
132.53643828218)) ;
#150660=CARTESIAN_POINT('Ctrl Pts',(-13.0797168042505,14.0250582462743,
132.657224771886)) ;
#150661=CARTESIAN_POINT('Ctrl Pts',(-13.1327979298348,14.267685746029,132.845402925329)) ;
#150662=CARTESIAN_POINT('Ctrl Pts',(-13.2046359566746,14.4501343666904,
133.088446513753)) ;
#150663=CARTESIAN_POINT('Ctrl Pts',(-13.2890293737238,14.5585281597601,
133.368092017486)) ;
#150664=CARTESIAN_POINT('Ctrl Pts',(-13.3793248440442,14.5857500281756,
133.664973177061)) ;
#150665=CARTESIAN_POINT('Ctrl Pts',(-13.4685173888611,14.5296138402308,
133.958689264273)) ;
#150666=CARTESIAN_POINT('Ctrl Pts',(-13.5492449744867,14.3940563949584,
134.227654399362)) ;
#150667=CARTESIAN_POINT('Ctrl Pts',(-13.6149101345716,14.1896706789709,
134.452519557024)) ;
#150668=CARTESIAN_POINT('Ctrl Pts',(-13.6605349934702,13.9296796265153,
134.618962908852)) ;
#150669=CARTESIAN_POINT('Ctrl Pts',(-13.6817176477053,13.632561455883,134.714074782053)) ;
#150670=CARTESIAN_POINT('Ctrl Pts',(-13.6763653200233,13.3229080728124,
134.731401281699)) ;
#150671=CARTESIAN_POINT('Ctrl Pts',(-13.6441156519113,13.0185267768755,
134.670365678224)) ;
#150672=CARTESIAN_POINT('Ctrl Pts',(-13.5866122080201,12.7436674784671,
134.535483497722)) ;
#150673=CARTESIAN_POINT('Ctrl Pts',(-13.5066983561414,12.516497959597,134.335317034424)) ;
#150674=CARTESIAN_POINT('Ctrl Pts',(-13.4107184546331,12.3560840678509,
134.08788704279)) ;
#150675=CARTESIAN_POINT('Ctrl Pts',(-13.3033206756955,12.2708854944156,
133.807337914075)) ;
#150676=CARTESIAN_POINT('Ctrl Pts',(-13.1925318588269,12.2685611985324,
133.51674558693)) ;
#150677=CARTESIAN_POINT('Ctrl Pts',(-13.0848159423213,12.3486009329829,
133.235220443721)) ;
#150678=CARTESIAN_POINT('Ctrl Pts',(-12.9871465907751,12.5069430119851,
132.983196082065)) ;
#150679=CARTESIAN_POINT('Ctrl Pts',(-12.9070956244391,12.7284058667927,
132.782242099243)) ;
#150680=CARTESIAN_POINT('Ctrl Pts',(-12.8477873224849,13.0024844630991,
132.642296947381)) ;
#150681=CARTESIAN_POINT('Ctrl Pts',(-12.8141762094062,13.3053155340302,
132.57721650409)) ;
#150682=CARTESIAN_POINT('Ctrl Pts',(-12.8073152976066,13.6156286046676,
132.590193775333)) ;
#150683=CARTESIAN_POINT('Ctrl Pts',(-12.8269279491894,13.9128849150777,
132.680569802002)) ;
#150684=CARTESIAN_POINT('Ctrl Pts',(-12.8713684246668,14.1766184698676,
132.843682795941)) ;
#150685=CARTESIAN_POINT('Ctrl Pts',(-12.9362504869269,14.3847398233907,
133.066334572889)) ;
#150686=CARTESIAN_POINT('Ctrl Pts',(-13.0160033501416,14.523836080727,133.332321804548)) ;
#150687=CARTESIAN_POINT('Ctrl Pts',(-13.1047838223045,14.5847742986496,
133.624794125344)) ;
#150688=CARTESIAN_POINT('Ctrl Pts',(-13.1953163380789,14.5623309512569,
133.922410172408)) ;
#150689=CARTESIAN_POINT('Ctrl Pts',(-13.2802958590821,14.4584178345544,
134.203783409206)) ;
#150690=CARTESIAN_POINT('Ctrl Pts',(-13.3531293445272,14.2791868966926,
134.449815883522)) ;
#150691=CARTESIAN_POINT('Ctrl Pts',(-13.4070402409324,14.0415187300811,
134.640161537634)) ;
#150692=CARTESIAN_POINT('Ctrl Pts',(-13.4387033407001,13.7564325475948,
134.765949365673)) ;
#150693=CARTESIAN_POINT('Ctrl Pts',(-13.4442407332801,13.4495648633329,
134.815151727329)) ;
#150694=CARTESIAN_POINT('Ctrl Pts',(-13.4228103575776,13.139416785511,134.785739085568)) ;
#150695=CARTESIAN_POINT('Ctrl Pts',(-13.3753386049812,12.8508801252525,
134.680098633708)) ;
#150696=CARTESIAN_POINT('Ctrl Pts',(-13.3041873758787,12.6022770135179,
134.505413740681)) ;
#150697=CARTESIAN_POINT('Ctrl Pts',(-13.21398842626,12.4127865766784,134.275031656731)) ;
#150698=CARTESIAN_POINT('Ctrl Pts',(-13.1098628114342,12.2953916616204,
134.004125903995)) ;
#150699=CARTESIAN_POINT('Ctrl Pts',(-12.9998843833805,12.2594835085984,
133.715856211852)) ;
#150700=CARTESIAN_POINT('Ctrl Pts',(-12.890063684845,12.3065006883116,133.428152917967)) ;
#150701=CARTESIAN_POINT('Ctrl Pts',(-12.7878923147766,12.4331949818184,
133.162761248478)) ;
#150702=CARTESIAN_POINT('Ctrl Pts',(-12.6993847702854,12.6325250875222,
132.937531738056)) ;
#150703=CARTESIAN_POINT('Ctrl Pts',(-12.6316222787159,12.8854153645511,
132.77246408779)) ;
#150704=CARTESIAN_POINT('Ctrl Pts',(-12.5870341048101,13.1803566291491,
132.67554844166)) ;
#150705=CARTESIAN_POINT('Ctrl Pts',(-12.5693200633778,13.4893560631302,
132.65674883301)) ;
#150706=CARTESIAN_POINT('Ctrl Pts',(-12.5782837478994,13.7954469993451,
132.716086060484)) ;
#150707=CARTESIAN_POINT('Ctrl Pts',(-12.6130490170968,14.0751704523599,
132.850844642907)) ;
#150708=CARTESIAN_POINT('Ctrl Pts',(-12.6699292025348,14.3069079863902,
133.050042271564)) ;
#150709=CARTESIAN_POINT('Ctrl Pts',(-12.7444274445508,14.4762412630358,
133.300783850622)) ;
#150710=CARTESIAN_POINT('Ctrl Pts',(-12.8310022377509,14.5702449515651,
133.587003668086)) ;
#150711=CARTESIAN_POINT('Ctrl Pts',(-12.9213296926271,14.5813885782014,
133.883870771373)) ;
#150712=CARTESIAN_POINT('Ctrl Pts',(-13.0093623207136,14.5100797260329,
134.174156031041)) ;
#150713=CARTESIAN_POINT('Ctrl Pts',(-13.0879614538735,14.3602445926638,
134.436979157099)) ;
#150714=CARTESIAN_POINT('Ctrl Pts',(-13.1502927048958,14.1432533152037,
134.652217619341)) ;
#150715=CARTESIAN_POINT('Ctrl Pts',(-13.1912501163863,13.8766591291424,
134.804796321906)) ;
#150716=CARTESIAN_POINT('Ctrl Pts',(-13.2076514124531,13.5754713250829,
134.885908155711)) ;
#150717=CARTESIAN_POINT('Ctrl Pts',(-13.1972577477252,13.2645670010663,
134.888600930151)) ;
#150718=CARTESIAN_POINT('Ctrl Pts',(-13.1599327354177,12.9634278823174,
134.812807254142)) ;
#150719=CARTESIAN_POINT('Ctrl Pts',(-13.0981398878319,12.6972349900806,
134.665294225835)) ;
#150720=CARTESIAN_POINT('Ctrl Pts',(-13.0150465902604,12.481723120017,134.455705324013)) ;
#150721=CARTESIAN_POINT('Ctrl Pts',(-12.9159624724356,12.3338052298827,
134.199416140809)) ;
#150722=CARTESIAN_POINT('Ctrl Pts',(-12.8075320102091,12.2641456097446,
133.915772384435)) ;
#150723=CARTESIAN_POINT('Ctrl Pts',(-12.6966987609025,12.277353556164,133.625090634121)) ;
#150724=CARTESIAN_POINT('Ctrl Pts',(-12.5904476511584,12.3726334343567,
133.347841250545)) ;
#150725=CARTESIAN_POINT('Ctrl Pts',(-12.4957672976613,12.5434757962,133.104422029015)) ;
#150726=CARTESIAN_POINT('Ctrl Pts',(-12.4189551559165,12.7769497154647,
132.913132493819)) ;
#150727=CARTESIAN_POINT('Ctrl Pts',(-12.3644955449637,13.0568799295701,
132.787172403634)) ;
#150728=CARTESIAN_POINT('Ctrl Pts',(-12.3356835525213,13.3636449055978,
132.73619324156)) ;
#150729=CARTESIAN_POINT('Ctrl Pts',(-12.3339186693949,13.6733774156544,
132.764089446736)) ;
#150730=CARTESIAN_POINT('Ctrl Pts',(-12.3583243925336,13.965438068356,132.86844444326)) ;
#150731=CARTESIAN_POINT('Ctrl Pts',(-12.4070227423529,14.2203012587836,
133.043999653821)) ;
#150732=CARTESIAN_POINT('Ctrl Pts',(-12.4749034404365,14.4159470406951,
133.275286549984)) ;
#150733=CARTESIAN_POINT('Ctrl Pts',(-12.5571654799498,14.5416943667992,
133.54875796597)) ;
#150734=CARTESIAN_POINT('Ctrl Pts',(-12.6469182873543,14.5869018903293,
133.844101856402)) ;
#150735=CARTESIAN_POINT('Ctrl Pts',(-12.7367367973124,14.5489491297832,
134.139548585729)) ;
#150736=CARTESIAN_POINT('Ctrl Pts',(-12.8200676024084,14.4300240433963,
134.416180797309)) ;
#150737=CARTESIAN_POINT('Ctrl Pts',(-12.8896854587349,14.2387296175427,
134.652716325118)) ;
#150738=CARTESIAN_POINT('Ctrl Pts',(-12.9398689479383,13.9899469029636,
134.832358869625)) ;
#150739=CARTESIAN_POINT('Ctrl Pts',(-12.9666061416785,13.7002922437487,
134.943563277021)) ;
#150740=CARTESIAN_POINT('Ctrl Pts',(-12.9672119408705,13.3909003280038,
134.978416886849)) ;
#150741=CARTESIAN_POINT('Ctrl Pts',(-12.9405858686605,13.0819914624154,
134.933923958189)) ;
#150742=CARTESIAN_POINT('Ctrl Pts',(-12.8884188883953,12.8000707590593,
134.814533654396)) ;
#150743=CARTESIAN_POINT('Ctrl Pts',(-12.8134045786365,12.5616135129792,
134.62851387434)) ;
#150744=CARTESIAN_POINT('Ctrl Pts',(-12.719888608477,12.3844499171478,134.38854536565)) ;
#150745=CARTESIAN_POINT('Ctrl Pts',(-12.6143404917224,12.2824628358376,
134.113358649894)) ;
#150746=CARTESIAN_POINT('Ctrl Pts',(-12.5041008453743,12.2618989558539,
133.824270652504)) ;
#150747=CARTESIAN_POINT('Ctrl Pts',(-12.3947436272254,12.3245801207235,
133.53804913358)) ;
#150748=CARTESIAN_POINT('Ctrl Pts',(-12.2949373759615,12.4655889395947,
133.279529105452)) ;
#150749=CARTESIAN_POINT('Ctrl Pts',(-12.2101743985447,12.6753257670411,
133.065046394778)) ;
#150750=CARTESIAN_POINT('Ctrl Pts',(-12.1460605408991,12.9389694466535,
132.910911474602)) ;
#150751=CARTESIAN_POINT('Ctrl Pts',(-12.1065857640139,13.2377440459955,
132.828793571842)) ;
#150752=CARTESIAN_POINT('Ctrl Pts',(-12.0938230998767,13.5478076708615,
132.824490961141)) ;
#150753=CARTESIAN_POINT('Ctrl Pts',(-12.1078810488391,13.8515134131997,
132.898821311669)) ;
#150754=CARTESIAN_POINT('Ctrl Pts',(-12.1471350028197,14.1231096251736,
133.046614309383)) ;
#150755=CARTESIAN_POINT('Ctrl Pts',(-12.20764101,14.3439545931311,133.256373038123)) ;
#150756=CARTESIAN_POINT('Ctrl Pts',(-12.2848385159864,14.4998916589537,
133.515014296344)) ;
#150757=CARTESIAN_POINT('Ctrl Pts',(-12.3725989192797,14.5786386310749,
133.804615404426)) ;
#150758=CARTESIAN_POINT('Ctrl Pts',(-12.4632852821564,14.5742675213239,
134.102641221154)) ;
#150759=CARTESIAN_POINT('Ctrl Pts',(-12.550091515244,14.4873447468798,134.389378773216)) ;
#150760=CARTESIAN_POINT('Ctrl Pts',(-12.6257089828659,14.3247914484279,
134.643310986823)) ;
#150761=CARTESIAN_POINT('Ctrl Pts',(-12.6845766874469,14.0970302958978,
134.848450091851)) ;
#150762=CARTESIAN_POINT('Ctrl Pts',(-12.7213449167932,13.8204924579681,
134.989058109086)) ;
#150763=CARTESIAN_POINT('Ctrl Pts',(-12.7326160006419,13.5164550314446,
135.055069728641)) ;
#150764=CARTESIAN_POINT('Ctrl Pts',(-12.7170978355958,13.2060700526839,
135.042791920806)) ;
#150765=CARTESIAN_POINT('Ctrl Pts',(-12.6750312631745,12.9102233152311,
134.953058802789)) ;
#150766=CARTESIAN_POINT('Ctrl Pts',(-12.6083863873251,12.6507291998818,
134.791615396846)) ;
#150767=CARTESIAN_POINT('Ctrl Pts',(-12.5223567020033,12.448558591514,134.573220681831)) ;
#150768=CARTESIAN_POINT('Ctrl Pts',(-12.4210378931773,12.3145373927892,
134.310396455084)) ;
#150769=CARTESIAN_POINT('Ctrl Pts',(-12.3115104666657,12.2601564003865,
134.023569123454)) ;
#150770=CARTESIAN_POINT('Ctrl Pts',(-12.200619808401,12.2893926143671,133.732844409505)) ;
#150771=CARTESIAN_POINT('Ctrl Pts',(-12.0963310670659,12.399436637318,133.461240632214)) ;
#150772=CARTESIAN_POINT('Ctrl Pts',(-12.0043449575091,12.5839727968354,
133.225788965511)) ;
#150773=CARTESIAN_POINT('Ctrl Pts',(-11.9318054869342,12.8264918557582,
133.046825298092)) ;
#150774=CARTESIAN_POINT('Ctrl Pts',(-11.88180009377,13.1141229255637,132.934004998449)) ;
#150775=CARTESIAN_POINT('Ctrl Pts',(-11.8660883176702,13.3194868174309,
132.910146711368)) ;
#150776=CARTESIAN_POINT('Ctrl Pts',(-11.862675149115,13.4222383333956,132.91119671495)) ;
#150777=CARTESIAN_POINT('Ctrl Pts',(-33.3489959095147,13.1551399285885,
127.871927411069)) ;
#150778=CARTESIAN_POINT('Ctrl Pts',(-33.3482570091173,13.1489709609094,
127.870499856875)) ;
#150779=CARTESIAN_POINT('Ctrl Pts',(-33.3362031847492,13.0505878441039,
127.846970056077)) ;
#150780=CARTESIAN_POINT('Ctrl Pts',(-33.303456104594,12.8648900473044,127.774282508598)) ;
#150781=CARTESIAN_POINT('Ctrl Pts',(-33.2347176391245,12.6378996894465,
127.606502631126)) ;
#150782=CARTESIAN_POINT('Ctrl Pts',(-33.1484631699894,12.4661938442505,
127.38763758675)) ;
#150783=CARTESIAN_POINT('Ctrl Pts',(-33.0496339239794,12.3629468779938,
127.132205946451)) ;
#150784=CARTESIAN_POINT('Ctrl Pts',(-32.9461836982222,12.3360866578135,
126.862930995212)) ;
#150785=CARTESIAN_POINT('Ctrl Pts',(-32.8428524780797,12.3868467815327,
126.594300512203)) ;
#150786=CARTESIAN_POINT('Ctrl Pts',(-32.7476240151848,12.5118616193735,
126.34920621096)) ;
#150787=CARTESIAN_POINT('Ctrl Pts',(-32.6660393235339,12.7022376314793,
126.14402042184)) ;
#150788=CARTESIAN_POINT('Ctrl Pts',(-32.6034202579729,12.9442211340136,
125.994217779495)) ;
#150789=CARTESIAN_POINT('Ctrl Pts',(-32.5634889320909,13.2203922331636,
125.91068247448)) ;
#150790=CARTESIAN_POINT('Ctrl Pts',(-32.5482836171183,13.5109001041669,
125.899354456419)) ;
#150791=CARTESIAN_POINT('Ctrl Pts',(-32.5583885908025,13.7967277450532,
125.962163306551)) ;
#150792=CARTESIAN_POINT('Ctrl Pts',(-32.5919970185865,14.0531634695327,
126.093303648423)) ;
#150793=CARTESIAN_POINT('Ctrl Pts',(-32.6462352627175,14.2659161102292,
126.2848763833)) ;
#150794=CARTESIAN_POINT('Ctrl Pts',(-32.7164440425069,14.4182155312585,
126.52308858485)) ;
#150795=CARTESIAN_POINT('Ctrl Pts',(-32.7970929244734,14.4993926065239,
126.791896512519)) ;
#150796=CARTESIAN_POINT('Ctrl Pts',(-32.8812312900771,14.5030674016304,
127.070805593369)) ;
#150797=CARTESIAN_POINT('Ctrl Pts',(-32.9621947752627,14.4296658181567,
127.340390412531)) ;
#150798=CARTESIAN_POINT('Ctrl Pts',(-33.0336799536047,14.2842405620309,
127.582320067705)) ;
#150799=CARTESIAN_POINT('Ctrl Pts',(-33.0898518257578,14.0768885755418,
127.779563482544)) ;
#150800=CARTESIAN_POINT('Ctrl Pts',(-33.1258131095785,13.821937566696,127.917839903426)) ;
#150801=CARTESIAN_POINT('Ctrl Pts',(-33.1381603359796,13.5404397832619,
127.986888146398)) ;
#150802=CARTESIAN_POINT('Ctrl Pts',(-33.1255862370588,13.2491903771815,
127.98329800545)) ;
#150803=CARTESIAN_POINT('Ctrl Pts',(-33.0878760919221,12.9699188880577,
127.906345203758)) ;
#150804=CARTESIAN_POINT('Ctrl Pts',(-33.0275630545352,12.7245502986717,
127.763166970814)) ;
#150805=CARTESIAN_POINT('Ctrl Pts',(-32.9475449968705,12.5279694687298,
127.562611942766)) ;
#150806=CARTESIAN_POINT('Ctrl Pts',(-32.853484832887,12.3961377043517,127.320906369453)) ;
#150807=CARTESIAN_POINT('Ctrl Pts',(-32.7506275244767,12.3376103677892,
127.053662058531)) ;
#150808=CARTESIAN_POINT('Ctrl Pts',(-32.6467508382538,12.3569098529355,
126.783214181605)) ;
#150809=CARTESIAN_POINT('Ctrl Pts',(-32.5472606088073,12.452769019898,126.525790390631)) ;
#150810=CARTESIAN_POINT('Ctrl Pts',(-32.4595735399336,12.6179593573441,
126.30272348908)) ;
#150811=CARTESIAN_POINT('Ctrl Pts',(-32.388745121808,12.8405880377693,126.12891456918)) ;
#150812=CARTESIAN_POINT('Ctrl Pts',(-32.3390681420419,13.1065246421439,
126.017073858121)) ;
#150813=CARTESIAN_POINT('Ctrl Pts',(-32.313898204756,13.3925179674891,125.976505647384)) ;
#150814=CARTESIAN_POINT('Ctrl Pts',(-32.3136699242009,13.6819916651313,
126.008953177836)) ;
#150815=CARTESIAN_POINT('Ctrl Pts',(-32.3381285657715,13.9537242418059,
126.113619428421)) ;
#150816=CARTESIAN_POINT('Ctrl Pts',(-32.384536696511,14.1863734291659,126.28227784121)) ;
#150817=CARTESIAN_POINT('Ctrl Pts',(-32.4487957222161,14.3643807985693,
126.503053049914)) ;
#150818=CARTESIAN_POINT('Ctrl Pts',(-32.5258074280907,14.4754559850244,
126.761140801679)) ;
#150819=CARTESIAN_POINT('Ctrl Pts',(-32.6094667487868,14.5110246739577,
127.038737149779)) ;
#150820=CARTESIAN_POINT('Ctrl Pts',(-32.6924145513944,14.4687063588107,
127.314091355005)) ;
#150821=CARTESIAN_POINT('Ctrl Pts',(-32.7687110106265,14.3514018815055,
127.570143149353)) ;
#150822=CARTESIAN_POINT('Ctrl Pts',(-32.8317732094795,14.1671964752596,
127.787539429963)) ;
#150823=CARTESIAN_POINT('Ctrl Pts',(-32.8762267217076,13.9308608041133,
127.950416591701)) ;
#150824=CARTESIAN_POINT('Ctrl Pts',(-32.8985780094168,13.6570089999716,
128.048890973466)) ;
#150825=CARTESIAN_POINT('Ctrl Pts',(-32.896157678737,13.3664659574419,128.074980037028)) ;
#150826=CARTESIAN_POINT('Ctrl Pts',(-32.8685548522265,13.0805681472547,
128.027442701697)) ;
#150827=CARTESIAN_POINT('Ctrl Pts',(-32.8170821736547,12.8190539470386,
127.91017574478)) ;
#150828=CARTESIAN_POINT('Ctrl Pts',(-32.7441829163896,12.5999338423892,
127.73048258649)) ;
#150829=CARTESIAN_POINT('Ctrl Pts',(-32.6555170250936,12.4413957528131,
127.504429482033)) ;
#150830=CARTESIAN_POINT('Ctrl Pts',(-32.5554705400289,12.3520378265489,
127.245337069314)) ;
#150831=CARTESIAN_POINT('Ctrl Pts',(-32.4511053019089,12.339734386482,126.973578302647)) ;
#150832=CARTESIAN_POINT('Ctrl Pts',(-32.3490815539954,12.4049383167358,
126.708653969777)) ;
#150833=CARTESIAN_POINT('Ctrl Pts',(-32.2559652828001,12.5429634979505,
126.469740198936)) ;
#150834=CARTESIAN_POINT('Ctrl Pts',(-32.1775406776191,12.7443553986761,
126.273802702315)) ;
#150835=CARTESIAN_POINT('Ctrl Pts',(-32.1189511785612,12.9943521537239,
126.135786155147)) ;
#150836=CARTESIAN_POINT('Ctrl Pts',(-32.0836266547703,13.2741647768729,
126.065632995122)) ;
#150837=CARTESIAN_POINT('Ctrl Pts',(-32.0731422430725,13.565720269456,126.068169777388)) ;
#150838=CARTESIAN_POINT('Ctrl Pts',(-32.0878672761987,13.8474315556546,
126.144404645481)) ;
#150839=CARTESIAN_POINT('Ctrl Pts',(-32.1256175280986,14.0971649669908,
126.287692127083)) ;
#150840=CARTESIAN_POINT('Ctrl Pts',(-32.1834742057281,14.3002122843455,
126.489943063825)) ;
#150841=CARTESIAN_POINT('Ctrl Pts',(-32.2561937622249,14.4394509674979,
126.73551422792)) ;
#150842=CARTESIAN_POINT('Ctrl Pts',(-32.3374471159419,14.5058688200503,
127.005843081603)) ;
#150843=CARTESIAN_POINT('Ctrl Pts',(-32.4217002826958,14.4952594831202,
127.285155611484)) ;
#150844=CARTESIAN_POINT('Ctrl Pts',(-32.5017471426193,14.4071576912799,
127.552229665334)) ;
#150845=CARTESIAN_POINT('Ctrl Pts',(-32.5706761898774,14.2488070341169,
127.786694114575)) ;
#150846=CARTESIAN_POINT('Ctrl Pts',(-32.6230717724866,14.032332595662,127.972746797191)) ;
#150847=CARTESIAN_POINT('Ctrl Pts',(-32.6548239115267,13.7715185673777,
128.098623777025)) ;
#150848=CARTESIAN_POINT('Ctrl Pts',(-32.6626680714647,13.4849968555095,
128.154735100321)) ;
#150849=CARTESIAN_POINT('Ctrl Pts',(-32.6450616243189,13.1936954317484,
128.136543946875)) ;
#150850=CARTESIAN_POINT('Ctrl Pts',(-32.6032602463952,12.9217410981826,
128.047311789015)) ;
#150851=CARTESIAN_POINT('Ctrl Pts',(-32.5386314820962,12.6826993167214,
127.891757560495)) ;
#150852=CARTESIAN_POINT('Ctrl Pts',(-32.4554412889622,12.4976839220085,
127.681914464153)) ;
#150853=CARTESIAN_POINT('Ctrl Pts',(-32.3596753952525,12.3794711428103,
127.435114332308)) ;
#150854=CARTESIAN_POINT('Ctrl Pts',(-32.2558253838943,12.3351744196322,
127.165019558565)) ;
#150855=CARTESIAN_POINT('Ctrl Pts',(-32.1520107530796,12.3695012763354,
126.894875973638)) ;
#150856=CARTESIAN_POINT('Ctrl Pts',(-32.0548036090535,12.4786183736045,
126.643923371603)) ;
#150857=CARTESIAN_POINT('Ctrl Pts',(-31.9697179472944,12.6556201701116,
126.428500311369)) ;
#150858=CARTESIAN_POINT('Ctrl Pts',(-31.9024466959007,12.8885376957079,
126.26521267139)) ;
#150859=CARTESIAN_POINT('Ctrl Pts',(-31.8574815700017,13.1578672277872,
126.166847085394)) ;
#150860=CARTESIAN_POINT('Ctrl Pts',(-31.8367167778053,13.4488181058444,
126.139492583638)) ;
#150861=CARTESIAN_POINT('Ctrl Pts',(-31.8414313820349,13.7357351250712,
126.186316118843)) ;
#150862=CARTESIAN_POINT('Ctrl Pts',(-31.8700151821842,14.0000244154435,
126.30281009704)) ;
#150863=CARTESIAN_POINT('Ctrl Pts',(-31.9203616130848,14.2248063693443,
126.483142763909)) ;
#150864=CARTESIAN_POINT('Ctrl Pts',(-31.9873859775564,14.3907221531774,
126.711954484493)) ;
#150865=CARTESIAN_POINT('Ctrl Pts',(-32.0662309963865,14.4880878052934,
126.975454295977)) ;
#150866=CARTESIAN_POINT('Ctrl Pts',(-32.1500140049146,14.5090844515927,
127.253273584441)) ;
#150867=CARTESIAN_POINT('Ctrl Pts',(-32.2328114906108,14.4517331277302,
127.528461364111)) ;
#150868=CARTESIAN_POINT('Ctrl Pts',(-32.306599429151,14.3213873494252,127.777000865602)) ;
#150869=CARTESIAN_POINT('Ctrl Pts',(-32.3665410586647,14.1266126254878,
127.985228303146)) ;
#150870=CARTESIAN_POINT('Ctrl Pts',(-32.4072983071001,13.8801113803002,
128.137553257528)) ;
#150871=CARTESIAN_POINT('Ctrl Pts',(-32.4248919159062,13.6025840232108,
128.221986639911)) ;
#150872=CARTESIAN_POINT('Ctrl Pts',(-32.4177985341224,13.3122088978665,
128.234314532032)) ;
#150873=CARTESIAN_POINT('Ctrl Pts',(-32.3854612722872,13.0284665595888,
128.173051822567)) ;
#150874=CARTESIAN_POINT('Ctrl Pts',(-32.3297158719588,12.7739765033465,
128.043289524966)) ;
#150875=CARTESIAN_POINT('Ctrl Pts',(-32.2536312710535,12.5655228915478,
127.854171141032)) ;
#150876=CARTESIAN_POINT('Ctrl Pts',(-32.1621333883639,12.4188418488155,
127.619973715704)) ;
#150877=CARTESIAN_POINT('Ctrl Pts',(-32.0610335191924,12.3438198182334,
127.357704488195)) ;
#150878=CARTESIAN_POINT('Ctrl Pts',(-31.9562422849269,12.3461749880073,
127.084814084959)) ;
#150879=CARTESIAN_POINT('Ctrl Pts',(-31.8555595514267,12.4256199459212,
126.823755799531)) ;
#150880=CARTESIAN_POINT('Ctrl Pts',(-31.7646812381954,12.5766359900473,
126.591428395529)) ;
#150881=CARTESIAN_POINT('Ctrl Pts',(-31.6897549709183,12.7882864475543,
126.405673808487)) ;
#150882=CARTESIAN_POINT('Ctrl Pts',(-31.6353440859288,13.0452019382586,
126.279829886042)) ;
#150883=CARTESIAN_POINT('Ctrl Pts',(-31.6045551307125,13.3293877258915,
126.223017390213)) ;
#150884=CARTESIAN_POINT('Ctrl Pts',(-31.598929994185,13.6204035856812,126.239726726341)) ;
#150885=CARTESIAN_POINT('Ctrl Pts',(-31.6181519561243,13.8971496153171,
126.329008321255)) ;
#150886=CARTESIAN_POINT('Ctrl Pts',(-31.660032440097,14.1397539052331,126.4844492787)) ;
#150887=CARTESIAN_POINT('Ctrl Pts',(-31.7210074180807,14.3313464702874,
126.695729086547)) ;
#150888=CARTESIAN_POINT('Ctrl Pts',(-31.7956413070931,14.4574458616527,
126.94680082343)) ;
#150889=CARTESIAN_POINT('Ctrl Pts',(-31.8782525153513,14.5099723944026,
127.221254124399)) ;
#150890=CARTESIAN_POINT('Ctrl Pts',(-31.9622607746967,14.4843439695083,
127.499872427198)) ;
#150891=CARTESIAN_POINT('Ctrl Pts',(-32.0404152099778,14.3827749410654,
127.761275810437)) ;
#150892=CARTESIAN_POINT('Ctrl Pts',(-32.1067647607671,14.2124739950545,
127.988225629159)) ;
#150893=CARTESIAN_POINT('Ctrl Pts',(-32.1557319181306,13.9855789386979,
128.164396849995)) ;
#150894=CARTESIAN_POINT('Ctrl Pts',(-32.1830886305706,13.7185805864342,
128.27741749427)) ;
#150895=CARTESIAN_POINT('Ctrl Pts',(-32.1861674536437,13.4303185636673,
128.319530923703)) ;
#150896=CARTESIAN_POINT('Ctrl Pts',(-32.164067606359,13.1417758325219,128.288060327875)) ;
#150897=CARTESIAN_POINT('Ctrl Pts',(-32.1174319130124,12.8725286043858,
128.185023246156)) ;
#150898=CARTESIAN_POINT('Ctrl Pts',(-32.0491401802662,12.6435096258014,
128.018626363072)) ;
#150899=CARTESIAN_POINT('Ctrl Pts',(-31.9632199754991,12.4701546223289,
127.800755651149)) ;
#150900=CARTESIAN_POINT('Ctrl Pts',(-31.8651776863348,12.3650501876111,
127.547453264018)) ;
#150901=CARTESIAN_POINT('Ctrl Pts',(-31.7609862185599,12.3357586674927,
127.276274914652)) ;
#150902=CARTESIAN_POINT('Ctrl Pts',(-31.6580563102104,12.3843195509594,
127.008647533804)) ;
#150903=CARTESIAN_POINT('Ctrl Pts',(-31.5623522569141,12.5073666683789,
126.762219617398)) ;
#150904=CARTESIAN_POINT('Ctrl Pts',(-31.4804283317136,12.6958200369819,
126.55599240923)) ;
#150905=CARTESIAN_POINT('Ctrl Pts',(-31.4171911262104,12.9363649293222,
126.404372140452)) ;
#150906=CARTESIAN_POINT('Ctrl Pts',(-31.3765204454803,13.212046231595,126.318705695641)) ;
#150907=CARTESIAN_POINT('Ctrl Pts',(-31.3605890149829,13.5022481067603,
126.305235943963)) ;
#150908=CARTESIAN_POINT('Ctrl Pts',(-31.3699466511949,13.7884016128943,
126.365844507772)) ;
#150909=CARTESIAN_POINT('Ctrl Pts',(-31.402839929772,14.045945075732,126.494887877481)) ;
#150910=CARTESIAN_POINT('Ctrl Pts',(-31.456801839307,14.2610680704969,126.685797164984)) ;
#150911=CARTESIAN_POINT('Ctrl Pts',(-31.5263791105061,14.4145624165552,
126.922033359285)) ;
#150912=CARTESIAN_POINT('Ctrl Pts',(-31.6068029650713,14.4980852125695,
127.190187763467)) ;
#150913=CARTESIAN_POINT('Ctrl Pts',(-31.6909497784616,14.5041312739862,
127.469125424148)) ;
#150914=CARTESIAN_POINT('Ctrl Pts',(-31.7722616933248,14.4326962339747,
127.739802187408)) ;
#150915=CARTESIAN_POINT('Ctrl Pts',(-31.8440399327869,14.289424830309,127.982545178335)) ;
#150916=CARTESIAN_POINT('Ctrl Pts',(-31.9008586342929,14.0826507854277,
128.181809264848)) ;
#150917=CARTESIAN_POINT('Ctrl Pts',(-31.9371644477761,13.8312291814697,
128.320780138694)) ;
#150918=CARTESIAN_POINT('Ctrl Pts',(-31.9504192122518,13.5479805821752,
128.392761416066)) ;
#150919=CARTESIAN_POINT('Ctrl Pts',(-31.9384428607775,13.2572981016289,
128.390846357411)) ;
#150920=CARTESIAN_POINT('Ctrl Pts',(-31.9016603090654,12.9781391944844,
128.316499055668)) ;
#150921=CARTESIAN_POINT('Ctrl Pts',(-31.8414344653115,12.7298471383749,
128.173831316095)) ;
#150922=CARTESIAN_POINT('Ctrl Pts',(-31.7624693619783,12.5331718510569,
127.976098656417)) ;
#150923=CARTESIAN_POINT('Ctrl Pts',(-31.6682896816273,12.3987050488903,
127.734214112554)) ;
#150924=CARTESIAN_POINT('Ctrl Pts',(-31.5661584069127,12.3381977133859,
127.468894861423)) ;
#150925=CARTESIAN_POINT('Ctrl Pts',(-31.4613121151811,12.3556285786372,
127.195919765139)) ;
#150926=CARTESIAN_POINT('Ctrl Pts',(-31.3626542471411,12.448498640132,126.940567661376)) ;
#150927=CARTESIAN_POINT('Ctrl Pts',(-31.2739963638957,12.6124651727369,
126.714860191145)) ;
#150928=CARTESIAN_POINT('Ctrl Pts',(-31.2028733579617,12.8330193864531,
126.540078371683)) ;
#150929=CARTESIAN_POINT('Ctrl Pts',(-31.1524099899045,13.0981216515098,
126.425973898796)) ;
#150930=CARTESIAN_POINT('Ctrl Pts',(-31.1264884036244,13.3840423616995,
126.383240800023)) ;
#150931=CARTESIAN_POINT('Ctrl Pts',(-31.1255526905879,13.6738043197191,
126.413632148392)) ;
#150932=CARTESIAN_POINT('Ctrl Pts',(-31.1492407119047,13.9458856450603,
126.515980892251)) ;
#150933=CARTESIAN_POINT('Ctrl Pts',(-31.1951906788803,14.1805609741337,
126.683399895541)) ;
#150934=CARTESIAN_POINT('Ctrl Pts',(-31.2589322113538,14.3602096703021,
126.902625201214)) ;
#150935=CARTESIAN_POINT('Ctrl Pts',(-31.336152907064,14.4737146563849,127.161521971997)) ;
#150936=CARTESIAN_POINT('Ctrl Pts',(-31.4191607366893,14.510981736058,127.436983917868)) ;
#150937=CARTESIAN_POINT('Ctrl Pts',(-31.5023202222332,14.4710234538019,
127.713002150618)) ;
#150938=CARTESIAN_POINT('Ctrl Pts',(-31.5788150531214,14.3558611755068,
127.9695934644)) ;
#150939=CARTESIAN_POINT('Ctrl Pts',(-31.6423459010436,14.1736059642118,
128.188348020273)) ;
#150940=CARTESIAN_POINT('Ctrl Pts',(-31.6874883180192,13.9381264816024,
128.353301532308)) ;
#150941=CARTESIAN_POINT('Ctrl Pts',(-31.7104598612239,13.665192099168,128.453567738071)) ;
#150942=CARTESIAN_POINT('Ctrl Pts',(-31.7088598170554,13.3755914984187,
128.481967244671)) ;
#150943=CARTESIAN_POINT('Ctrl Pts',(-31.6817723867748,13.0874857506397,
128.436147123456)) ;
#150944=CARTESIAN_POINT('Ctrl Pts',(-31.6311222896079,12.8264337657975,
128.32111606456)) ;
#150945=CARTESIAN_POINT('Ctrl Pts',(-31.5590254861687,12.6060974389448,
128.143694924089)) ;
#150946=CARTESIAN_POINT('Ctrl Pts',(-31.4705496041744,12.4450313389733,
127.91828768914)) ;
#150947=CARTESIAN_POINT('Ctrl Pts',(-31.3704536339561,12.3534666197661,
127.659136554107)) ;
#150948=CARTESIAN_POINT('Ctrl Pts',(-31.2664260741019,12.3390029903486,
127.388267266672)) ;
#150949=CARTESIAN_POINT('Ctrl Pts',(-31.1640074542676,12.4020392430349,
127.122262231831)) ;
#150950=CARTESIAN_POINT('Ctrl Pts',(-31.0704546098695,12.5385711173323,
126.882123477286)) ;
#150951=CARTESIAN_POINT('Ctrl Pts',(-30.9919375233747,12.737337324062,126.685748126109)) ;
#150952=CARTESIAN_POINT('Ctrl Pts',(-30.9326059877163,12.9861206892308,
126.545580982005)) ;
#150953=CARTESIAN_POINT('Ctrl Pts',(-30.8964828802307,13.2660910782566,
126.473182758033)) ;
#150954=CARTESIAN_POINT('Ctrl Pts',(-30.8853353619794,13.5573227840952,
126.473749977841)) ;
#150955=CARTESIAN_POINT('Ctrl Pts',(-30.8992181639316,13.8386952169897,
126.547405844888)) ;
#150956=CARTESIAN_POINT('Ctrl Pts',(-30.9364490028324,14.0906007554108,
126.689305896974)) ;
#150957=CARTESIAN_POINT('Ctrl Pts',(-30.993577379338,14.2945039762926,126.889303441531)) ;
#150958=CARTESIAN_POINT('Ctrl Pts',(-31.0658785833472,14.4361574187858,
127.133657392973)) ;
#150959=CARTESIAN_POINT('Ctrl Pts',(-31.1473678175875,14.5051117570611,
127.404837868273)) ;
#150960=CARTESIAN_POINT('Ctrl Pts',(-31.2314101845586,14.496582620466,127.68344430737)) ;
#150961=CARTESIAN_POINT('Ctrl Pts',(-31.3113999047549,14.4113394819302,
127.950224339128)) ;
#150962=CARTESIAN_POINT('Ctrl Pts',(-31.3810275644355,14.2546479447355,
128.186843915728)) ;
#150963=CARTESIAN_POINT('Ctrl Pts',(-31.434079388976,14.039143877786,128.374888028828)) ;
#150964=CARTESIAN_POINT('Ctrl Pts',(-31.4664410188237,13.7793416572316,
128.502539340318)) ;
#150965=CARTESIAN_POINT('Ctrl Pts',(-31.4749982660917,13.4941095874199,
128.560637934817)) ;
#150966=CARTESIAN_POINT('Ctrl Pts',(-31.4582310109701,13.2026874966814,
128.544890911873)) ;
#150967=CARTESIAN_POINT('Ctrl Pts',(-31.4169753439866,12.928833346161,128.457383735722)) ;
#150968=CARTESIAN_POINT('Ctrl Pts',(-31.3527956487623,12.6885083712283,
128.303172142516)) ;
#150969=CARTESIAN_POINT('Ctrl Pts',(-31.2705703901443,12.5026390795781,
128.0959611027)) ;
#150970=CARTESIAN_POINT('Ctrl Pts',(-31.1745744230575,12.3816810236162,
127.848677279268)) ;
#150971=CARTESIAN_POINT('Ctrl Pts',(-31.0714307037018,12.3354826595071,
127.580451601079)) ;
#150972=CARTESIAN_POINT('Ctrl Pts',(-30.9672895160686,12.3671988660942,
127.309429336125)) ;
#150973=CARTESIAN_POINT('Ctrl Pts',(-30.8693900237751,12.4748749581507,
127.056599017908)) ;
#150974=CARTESIAN_POINT('Ctrl Pts',(-30.7841568236753,12.6498955190515,
126.840662152846)) ;
#150975=CARTESIAN_POINT('Ctrl Pts',(-30.7165115975955,12.8801431332148,
126.67612667683)) ;
#150976=CARTESIAN_POINT('Ctrl Pts',(-30.6705876552176,13.1504415297617,
126.575185235204)) ;
#150977=CARTESIAN_POINT('Ctrl Pts',(-30.6492401911973,13.438739202615,126.545850310757)) ;
#150978=CARTESIAN_POINT('Ctrl Pts',(-30.6531248486497,13.7280473502378,
126.590480521703)) ;
#150979=CARTESIAN_POINT('Ctrl Pts',(-30.6811874381857,13.9932362064335,
126.705468605857)) ;
#150980=CARTESIAN_POINT('Ctrl Pts',(-30.7307233901376,14.2186783745982,
126.88330032276)) ;
#150981=CARTESIAN_POINT('Ctrl Pts',(-30.7976668939673,14.3872014330787,
127.112042032862)) ;
#150982=CARTESIAN_POINT('Ctrl Pts',(-30.8759215226086,14.486216521528,127.373662762679)) ;
#150983=CARTESIAN_POINT('Ctrl Pts',(-30.9599483085192,14.5095010567365,
127.652320679818)) ;
#150984=CARTESIAN_POINT('Ctrl Pts',(-31.0423602583126,14.4548476689191,
127.926162766265)) ;
#150985=CARTESIAN_POINT('Ctrl Pts',(-31.1170261636548,14.3259646517619,
128.177490633467)) ;
#150986=CARTESIAN_POINT('Ctrl Pts',(-31.1774376241067,14.1320240566172,
128.38715540167)) ;
#150987=CARTESIAN_POINT('Ctrl Pts',(-31.2184772814882,13.8890687487633,
128.540002184362)) ;
#150988=CARTESIAN_POINT('Ctrl Pts',(-31.2369718788586,13.6109288487181,
128.62723857725)) ;
#150989=CARTESIAN_POINT('Ctrl Pts',(-31.2305830637653,13.3205780973656,
128.64162358396)) ;
#150990=CARTESIAN_POINT('Ctrl Pts',(-31.1988306507602,13.0356410236252,
128.582156307125)) ;
#150991=CARTESIAN_POINT('Ctrl Pts',(-31.1439236012217,12.7811568557338,
128.454705635715)) ;
#150992=CARTESIAN_POINT('Ctrl Pts',(-31.0684038299569,12.5709851276515,
128.267243241426)) ;
#150993=CARTESIAN_POINT('Ctrl Pts',(-30.9772756205,12.4221766619671,128.03413250274)) ;
#150994=CARTESIAN_POINT('Ctrl Pts',(-30.8759319496152,12.3447406812541,
127.771290965256)) ;
#150995=CARTESIAN_POINT('Ctrl Pts',(-30.7712963261735,12.3451621602759,
127.498804673837)) ;
#150996=CARTESIAN_POINT('Ctrl Pts',(-30.6706886680026,12.4221617733591,
127.237875690043)) ;
#150997=CARTESIAN_POINT('Ctrl Pts',(-30.5793389036692,12.5713293574021,
127.00420358355)) ;
#150998=CARTESIAN_POINT('Ctrl Pts',(-30.5039469378259,12.7811357471148,
126.817049360709)) ;
#150999=CARTESIAN_POINT('Ctrl Pts',(-30.4488110435835,13.037385413305,126.689142569762)) ;
#151000=CARTESIAN_POINT('Ctrl Pts',(-30.4173468141487,13.3202247802994,
126.630258735514)) ;
#151001=CARTESIAN_POINT('Ctrl Pts',(-30.4109588954888,13.6126649497902,
126.644895127432)) ;
#151002=CARTESIAN_POINT('Ctrl Pts',(-30.4294392941911,13.889109539137,126.731888107809)) ;
#151003=CARTESIAN_POINT('Ctrl Pts',(-30.47077570761,14.1334576219234,126.885811226843)) ;
#151004=CARTESIAN_POINT('Ctrl Pts',(-30.53102912446,14.3262010857029,127.094865661672)) ;
#151005=CARTESIAN_POINT('Ctrl Pts',(-30.6058078949067,14.4552702241494,
127.346574791049)) ;
#151006=CARTESIAN_POINT('Ctrl Pts',(-30.6883760016807,14.5094659873619,
127.620923977953)) ;
#151007=CARTESIAN_POINT('Ctrl Pts',(-30.7718896570381,14.48627928254,127.897878479629)) ;
#151008=CARTESIAN_POINT('Ctrl Pts',(-30.8505404170833,14.3867194330965,
128.16082928885)) ;
#151009=CARTESIAN_POINT('Ctrl Pts',(-30.9172652518935,14.2183273389604,
128.388850744567)) ;
#151010=CARTESIAN_POINT('Ctrl Pts',(-30.966927867041,13.9922441011096,128.567141543632)) ;
#151011=CARTESIAN_POINT('Ctrl Pts',(-30.9948429554227,13.7260908863955,
128.681785518138)) ;
#151012=CARTESIAN_POINT('Ctrl Pts',(-30.9986761317404,13.4392990683917,
128.725970798859)) ;
#151013=CARTESIAN_POINT('Ctrl Pts',(-30.9771754995003,13.1491383926391,
128.696410048975)) ;
#151014=CARTESIAN_POINT('Ctrl Pts',(-30.9313862314932,12.880138144259,128.595705294773)) ;
#151015=CARTESIAN_POINT('Ctrl Pts',(-30.8633741700187,12.6488312040692,
128.430267551873)) ;
#151016=CARTESIAN_POINT('Ctrl Pts',(-30.7783096718615,12.4746173052797,
128.214724190605)) ;
#151017=CARTESIAN_POINT('Ctrl Pts',(-30.6802839201009,12.3669410581914,
127.961566303494)) ;
#151018=CARTESIAN_POINT('Ctrl Pts',(-30.5761954681339,12.3355244467329,
127.690674965918)) ;
#151019=CARTESIAN_POINT('Ctrl Pts',(-30.4731987242308,12.3818824637266,
127.42284013735)) ;
#151020=CARTESIAN_POINT('Ctrl Pts',(-30.3773601675738,12.502442440452,127.175947943775)) ;
#151021=CARTESIAN_POINT('Ctrl Pts',(-30.2945593439143,12.6900860359651,
126.967322197996)) ;
#151022=CARTESIAN_POINT('Ctrl Pts',(-30.2309201264915,12.9290693621117,
126.814464075625)) ;
#151023=CARTESIAN_POINT('Ctrl Pts',(-30.1896011311781,13.2033802627449,
126.726833819823)) ;
#151024=CARTESIAN_POINT('Ctrl Pts',(-30.1729187517655,13.493885424346,126.711224329232)) ;
#151025=CARTESIAN_POINT('Ctrl Pts',(-30.1814818466642,13.7798208359641,
126.769425110779)) ;
#151026=CARTESIAN_POINT('Ctrl Pts',(-30.2139166442141,14.0398147256928,
126.897315524147)) ;
#151027=CARTESIAN_POINT('Ctrl Pts',(-30.2672327260932,14.2555980954836,
127.086230738633)) ;
#151028=CARTESIAN_POINT('Ctrl Pts',(-30.3364241626342,14.4112165057251,
127.321355815591)) ;
#151029=CARTESIAN_POINT('Ctrl Pts',(-30.4169483545396,14.4969135755094,
127.589920286704)) ;
#151030=CARTESIAN_POINT('Ctrl Pts',(-30.5006568417281,14.5049696810031,
127.867411820872)) ;
#151031=CARTESIAN_POINT('Ctrl Pts',(-30.5821059141925,14.4360249735447,
128.13846691764)) ;
#151032=CARTESIAN_POINT('Ctrl Pts',(-30.6543269887437,14.2945754362065,
128.382542123477)) ;
#151033=CARTESIAN_POINT('Ctrl Pts',(-30.7116365732865,14.0897548858671,
128.583199406406)) ;
#151034=CARTESIAN_POINT('Ctrl Pts',(-30.7486474004249,13.8387001375239,
128.724327683098)) ;
#151035=CARTESIAN_POINT('Ctrl Pts',(-30.7626160375506,13.5574044598577,
128.79823198023)) ;
#151036=CARTESIAN_POINT('Ctrl Pts',(-30.751280169492,13.2644130009093,128.798450590054)) ;
#151037=CARTESIAN_POINT('Ctrl Pts',(-30.7152762753897,12.9862195730077,
128.726198614227)) ;
#151038=CARTESIAN_POINT('Ctrl Pts',(-30.6559255495121,12.7371111819008,
128.586013158079)) ;
#151039=CARTESIAN_POINT('Ctrl Pts',(-30.5772199975952,12.5380203242925,
128.389149798631)) ;
#151040=CARTESIAN_POINT('Ctrl Pts',(-30.4833480932253,12.4015272632005,
128.148171071429)) ;
#151041=CARTESIAN_POINT('Ctrl Pts',(-30.3812924082162,12.3389470103484,
127.883098879055)) ;
#151042=CARTESIAN_POINT('Ctrl Pts',(-30.2769531606877,12.3537864997403,
127.611426962061)) ;
#151043=CARTESIAN_POINT('Ctrl Pts',(-30.1774142848297,12.4449099176858,
127.353712328041)) ;
#151044=CARTESIAN_POINT('Ctrl Pts',(-30.0884196313121,12.6072327563546,
127.127011108624)) ;
#151045=CARTESIAN_POINT('Ctrl Pts',(-30.0168944583603,12.8259751420657,
126.950999128042)) ;
#151046=CARTESIAN_POINT('Ctrl Pts',(-29.9658131020968,13.0894865209779,
126.835020394129)) ;
#151047=CARTESIAN_POINT('Ctrl Pts',(-29.9390402950618,13.3763086244584,
126.789949510195)) ;
#151048=CARTESIAN_POINT('Ctrl Pts',(-29.9374976893148,13.666102426872,126.818551688385)) ;
#151049=CARTESIAN_POINT('Ctrl Pts',(-29.9603659689101,13.9378774393092,
126.918366530385)) ;
#151050=CARTESIAN_POINT('Ctrl Pts',(-30.0058557147277,14.174793298913,127.084558461599)) ;
#151051=CARTESIAN_POINT('Ctrl Pts',(-30.0690738202602,14.355667987911,127.302193672896)) ;
#151052=CARTESIAN_POINT('Ctrl Pts',(-30.1455851444044,14.4711053294092,
127.558860146817)) ;
#151053=CARTESIAN_POINT('Ctrl Pts',(-30.2290907276294,14.511170979715,127.836014853784)) ;
#151054=CARTESIAN_POINT('Ctrl Pts',(-30.3124346958538,14.4729025341711,
128.112614820692)) ;
#151055=CARTESIAN_POINT('Ctrl Pts',(-30.3888326028229,14.3605014183323,
128.368750566373)) ;
#151056=CARTESIAN_POINT('Ctrl Pts',(-30.4531791538599,14.1789799497678,
128.590078616567)) ;
#151057=CARTESIAN_POINT('Ctrl Pts',(-30.4986908853725,13.9453130755044,
128.756011357139)) ;
#151058=CARTESIAN_POINT('Ctrl Pts',(-30.5223367702664,13.673613297581,128.858202384461)) ;
#151059=CARTESIAN_POINT('Ctrl Pts',(-30.5214927257582,13.3843416477693,
128.888796839614)) ;
#151060=CARTESIAN_POINT('Ctrl Pts',(-30.4951356796959,13.0956424787648,
128.845131685907)) ;
#151061=CARTESIAN_POINT('Ctrl Pts',(-30.4451353943437,12.8335787485534,
128.73200501772)) ;
#151062=CARTESIAN_POINT('Ctrl Pts',(-30.3735874311193,12.6116522531053,
128.556195762552)) ;
#151063=CARTESIAN_POINT('Ctrl Pts',(-30.2853579635812,12.4486058050818,
128.33155990322)) ;
#151064=CARTESIAN_POINT('Ctrl Pts',(-30.1858663129506,12.3551665981467,
128.074050595748)) ;
#151065=CARTESIAN_POINT('Ctrl Pts',(-30.0815496988783,12.3383111368361,
127.802444396815)) ;
#151066=CARTESIAN_POINT('Ctrl Pts',(-29.9791399961725,12.3991318667188,
127.536410522558)) ;
#151067=CARTESIAN_POINT('Ctrl Pts',(-29.885250975789,12.5336133546432,127.2952913997)) ;
#151068=CARTESIAN_POINT('Ctrl Pts',(-29.8062098846917,12.7304747525644,
127.097365942919)) ;
#151069=CARTESIAN_POINT('Ctrl Pts',(-29.7459166115697,12.9801493565206,
126.954643707808)) ;
#151070=CARTESIAN_POINT('Ctrl Pts',(-29.7094981424688,13.2569930870622,
126.881074054437)) ;
#151071=CARTESIAN_POINT('Ctrl Pts',(-29.697485321225,13.5493201067258,126.879249155707)) ;
#151072=CARTESIAN_POINT('Ctrl Pts',(-29.7107148915496,13.8310609228274,
126.950973130347)) ;
#151073=CARTESIAN_POINT('Ctrl Pts',(-29.7473686079901,14.0843638099265,
127.091228525209)) ;
#151074=CARTESIAN_POINT('Ctrl Pts',(-29.8039983073089,14.2896244491401,
127.289751241016)) ;
#151075=CARTESIAN_POINT('Ctrl Pts',(-29.8758248177242,14.4330063116879,
127.5326649792)) ;
#151076=CARTESIAN_POINT('Ctrl Pts',(-29.9571776043441,14.5042107415309,
127.803464708327)) ;
#151077=CARTESIAN_POINT('Ctrl Pts',(-30.0412713276901,14.4979449999679,
128.082232149485)) ;
#151078=CARTESIAN_POINT('Ctrl Pts',(-30.121694639328,14.4144601779744,128.350375838408)) ;
#151079=CARTESIAN_POINT('Ctrl Pts',(-30.1915790917938,14.2595209902124,
128.587713560571)) ;
#151080=CARTESIAN_POINT('Ctrl Pts',(-30.2450076010872,14.046214919979,128.776755103724)) ;
#151081=CARTESIAN_POINT('Ctrl Pts',(-30.2780878046331,13.7868053449528,
128.906585374679)) ;
#151082=CARTESIAN_POINT('Ctrl Pts',(-30.2872906950602,13.5027357390144,
128.966484763682)) ;
#151083=CARTESIAN_POINT('Ctrl Pts',(-30.2713500951273,13.2114164567146,
128.953122045362)) ;
#151084=CARTESIAN_POINT('Ctrl Pts',(-30.230627814723,12.9359342983456,128.86728322249)) ;
#151085=CARTESIAN_POINT('Ctrl Pts',(-30.1672447422047,12.6951562018299,
128.715288751686)) ;
#151086=CARTESIAN_POINT('Ctrl Pts',(-30.0854978465419,12.5073061272103,
128.509491429827)) ;
#151087=CARTESIAN_POINT('Ctrl Pts',(-29.9896882822811,12.3841592686752,
128.262793679839)) ;
#151088=CARTESIAN_POINT('Ctrl Pts',(-29.8866361087517,12.3356200239572,
127.994841190901)) ;
#151089=CARTESIAN_POINT('Ctrl Pts',(-29.7820423738734,12.3655842279676,
127.722626897302)) ;
#151090=CARTESIAN_POINT('Ctrl Pts',(-29.6846378874882,12.4702048591763,
127.470973299483)) ;
#151091=CARTESIAN_POINT('Ctrl Pts',(-29.5982444318826,12.6448837976238,
127.251934053335)) ;
#151092=CARTESIAN_POINT('Ctrl Pts',(-29.530484788473,12.872508423284,127.086857758343)) ;
#151093=CARTESIAN_POINT('Ctrl Pts',(-29.4836133061575,13.1434988331289,
126.983345728084)) ;
#151094=CARTESIAN_POINT('Ctrl Pts',(-29.4617927517553,13.4301737780494,
126.952467269919)) ;
#151095=CARTESIAN_POINT('Ctrl Pts',(-29.4647728375027,13.7187795914099,
126.994328449619)) ;
#151096=CARTESIAN_POINT('Ctrl Pts',(-29.4924039666026,13.9870154433738,
127.108324446431)) ;
#151097=CARTESIAN_POINT('Ctrl Pts',(-29.5411722729436,14.2124398345738,
127.283727368873)) ;
#151098=CARTESIAN_POINT('Ctrl Pts',(-29.6075895922723,14.3830654461858,
127.510923381855)) ;
#151099=CARTESIAN_POINT('Ctrl Pts',(-29.6859780654117,14.4846609541733,
127.773091506423)) ;
#151100=CARTESIAN_POINT('Ctrl Pts',(-29.7699711987632,14.5097913616969,
128.051659371141)) ;
#151101=CARTESIAN_POINT('Ctrl Pts',(-29.8521599614632,14.4576093080194,
128.324704513275)) ;
#151102=CARTESIAN_POINT('Ctrl Pts',(-29.9273378651692,14.3304831317374,
128.57761366537)) ;
#151103=CARTESIAN_POINT('Ctrl Pts',(-29.9881011678196,14.1386183822934,
128.788232639006)) ;
#151104=CARTESIAN_POINT('Ctrl Pts',(-30.0298088081978,13.8965846856625,
128.943079017119)) ;
#151105=CARTESIAN_POINT('Ctrl Pts',(-30.048987740085,13.6198365630073,129.032230754272)) ;
#151106=CARTESIAN_POINT('Ctrl Pts',(-30.0433213484704,13.3288844737818,
129.048809941996)) ;
#151107=CARTESIAN_POINT('Ctrl Pts',(-30.0124680035273,13.0447399832046,
128.991813037362)) ;
#151108=CARTESIAN_POINT('Ctrl Pts',(-29.958162147996,12.7881836368688,128.866220633411)) ;
#151109=CARTESIAN_POINT('Ctrl Pts',(-29.8827371039613,12.5755910115287,
128.67919720058)) ;
#151110=CARTESIAN_POINT('Ctrl Pts',(-29.7923817501949,12.4257574465567,
128.448186718166)) ;
#151111=CARTESIAN_POINT('Ctrl Pts',(-29.6914548654442,12.3460112405744,
128.186501449005)) ;
#151112=CARTESIAN_POINT('Ctrl Pts',(-29.5867020660159,12.3439532504127,
127.913710488866)) ;
#151113=CARTESIAN_POINT('Ctrl Pts',(-29.485666657119,12.4188218900739,127.651602416161)) ;
#151114=CARTESIAN_POINT('Ctrl Pts',(-29.3936759004092,12.5668341062151,
127.416175460721)) ;
#151115=CARTESIAN_POINT('Ctrl Pts',(-29.3182301931701,12.7739565310488,
127.2286723812)) ;
#151116=CARTESIAN_POINT('Ctrl Pts',(-29.2623086088496,13.0292275295923,
127.098504241357)) ;
#151117=CARTESIAN_POINT('Ctrl Pts',(-29.2301243830033,13.3121167714202,
127.037580467898)) ;
#151118=CARTESIAN_POINT('Ctrl Pts',(-29.2229734795966,13.6036711588795,
127.049873651472)) ;
#151119=CARTESIAN_POINT('Ctrl Pts',(-29.2408639834952,13.8822010088686,
127.135317168003)) ;
#151120=CARTESIAN_POINT('Ctrl Pts',(-29.2814175857852,14.126534024312,127.286789452504)) ;
#151121=CARTESIAN_POINT('Ctrl Pts',(-29.341269933413,14.3215277156221,127.494747226261)) ;
#151122=CARTESIAN_POINT('Ctrl Pts',(-29.4156496701704,14.4523872469144,
127.745252022521)) ;
#151123=CARTESIAN_POINT('Ctrl Pts',(-29.4979993749135,14.509081269933,128.018936330148)) ;
#151124=CARTESIAN_POINT('Ctrl Pts',(-29.5821194390776,14.4877530584647,
128.297884507417)) ;
#151125=CARTESIAN_POINT('Ctrl Pts',(-29.6605015766084,14.3906972492053,
128.559841528178)) ;
#151126=CARTESIAN_POINT('Ctrl Pts',(-29.7277325620602,14.2242127265294,
128.789368837068)) ;
#151127=CARTESIAN_POINT('Ctrl Pts',(-29.7778622908604,14.0000453961231,
128.968956847515)) ;
#151128=CARTESIAN_POINT('Ctrl Pts',(-29.8065930602879,13.7349941187306,
129.085980593616)) ;
#151129=CARTESIAN_POINT('Ctrl Pts',(-29.8110647581583,13.4462938086935,
129.132290262238)) ;
#151130=CARTESIAN_POINT('Ctrl Pts',(-29.7905149481192,13.1586524064852,
129.105179558969)) ;
#151131=CARTESIAN_POINT('Ctrl Pts',(-29.7450251194424,12.8863235925418,
129.005657518442)) ;
#151132=CARTESIAN_POINT('Ctrl Pts',(-29.6779688870286,12.6553854575325,
128.842782884932)) ;
#151133=CARTESIAN_POINT('Ctrl Pts',(-29.5932822353585,12.4787538591612,
128.628403260321)) ;
#151134=CARTESIAN_POINT('Ctrl Pts',(-29.4951432611704,12.3688114822916,
128.375032108495)) ;
#151135=CARTESIAN_POINT('Ctrl Pts',(-29.3915755638739,12.3354319136936,
128.105522888968)) ;
#151136=CARTESIAN_POINT('Ctrl Pts',(-29.2883737439491,12.3792576310417,
127.83711019449)) ;
#151137=CARTESIAN_POINT('Ctrl Pts',(-29.1917010872287,12.4988398999205,
127.587984309591)) ;
#151138=CARTESIAN_POINT('Ctrl Pts',(-29.1090972687786,12.6835118512005,
127.379683329034)) ;
#151139=CARTESIAN_POINT('Ctrl Pts',(-29.0446608613966,12.9214923912795,
127.224563683631)) ;
#151140=CARTESIAN_POINT('Ctrl Pts',(-29.0026163941945,13.1954916424955,
127.134859426664)) ;
#151141=CARTESIAN_POINT('Ctrl Pts',(-28.985230945197,13.4865485670219,127.117276574287)) ;
#151142=CARTESIAN_POINT('Ctrl Pts',(-28.9931808891691,13.772471589557,127.173641275195)) ;
#151143=CARTESIAN_POINT('Ctrl Pts',(-29.0248180797672,14.0322259092952,
127.299049560001)) ;
#151144=CARTESIAN_POINT('Ctrl Pts',(-29.0774225647813,14.2496185339524,
127.485847881482)) ;
#151145=CARTESIAN_POINT('Ctrl Pts',(-29.1466584272716,14.4079186586772,
127.721302692546)) ;
#151146=CARTESIAN_POINT('Ctrl Pts',(-29.2262609733389,14.495128940057,127.986882942297)) ;
#151147=CARTESIAN_POINT('Ctrl Pts',(-29.310377688868,14.5060206783235,128.265744239721)) ;
#151148=CARTESIAN_POINT('Ctrl Pts',(-29.3922415681972,14.4388851972431,
128.538108177024)) ;
#151149=CARTESIAN_POINT('Ctrl Pts',(-29.4648367940965,14.2990479598781,
128.783307296558)) ;
#151150=CARTESIAN_POINT('Ctrl Pts',(-29.5224591681686,14.096277092635,128.984789687897)) ;
#151151=CARTESIAN_POINT('Ctrl Pts',(-29.5601633246064,13.8463552274942,
129.12795060112)) ;
#151152=CARTESIAN_POINT('Ctrl Pts',(-29.5747316968106,13.5643762793268,
129.203747316631)) ;
#151153=CARTESIAN_POINT('Ctrl Pts',(-29.5643172687888,13.2747380866486,
129.206268472805)) ;
#151154=CARTESIAN_POINT('Ctrl Pts',(-29.5288291438255,12.9934296976024,
129.135814296567)) ;
#151155=CARTESIAN_POINT('Ctrl Pts',(-29.470171863856,12.7438068041656,128.99757323151)) ;
#151156=CARTESIAN_POINT('Ctrl Pts',(-29.391803285665,12.5426943442427,128.801768222048)) ;
#151157=CARTESIAN_POINT('Ctrl Pts',(-29.2986131391391,12.4046936236787,
128.56265775762)) ;
#151158=CARTESIAN_POINT('Ctrl Pts',(-29.1964773761958,12.3396331759052,
128.297435830634)) ;
#151159=CARTESIAN_POINT('Ctrl Pts',(-29.092230590555,12.3522550875064,128.025991131613)) ;
#151160=CARTESIAN_POINT('Ctrl Pts',(-28.9924608185787,12.441158614988,127.767604009206)) ;
#151161=CARTESIAN_POINT('Ctrl Pts',(-28.9030933450802,12.6013769713038,
127.539790029494)) ;
#151162=CARTESIAN_POINT('Ctrl Pts',(-28.8308886096015,12.819071640269,127.361858709555)) ;
#151163=CARTESIAN_POINT('Ctrl Pts',(-28.779280341327,13.0807346140254,127.244233442709)) ;
#151164=CARTESIAN_POINT('Ctrl Pts',(-28.7517055757331,13.3675408612144,
127.196874862189)) ;
#151165=CARTESIAN_POINT('Ctrl Pts',(-28.7493257047856,13.6570979280699,
127.222968219409)) ;
#151166=CARTESIAN_POINT('Ctrl Pts',(-28.7718142821641,13.9319893911641,
127.321979864566)) ;
#151167=CARTESIAN_POINT('Ctrl Pts',(-28.8162456944187,14.1676085258846,
127.484711805867)) ;
#151168=CARTESIAN_POINT('Ctrl Pts',(-28.8794392120634,14.3519029604138,
127.702543293248)) ;
#151169=CARTESIAN_POINT('Ctrl Pts',(-28.955521536148,14.4687263868581,127.957864396171)) ;
#151170=CARTESIAN_POINT('Ctrl Pts',(-29.0386446837284,14.5110206744739,
128.233803590714)) ;
#151171=CARTESIAN_POINT('Ctrl Pts',(-29.1220480184099,14.4754839101951,
128.510547823415)) ;
#151172=CARTESIAN_POINT('Ctrl Pts',(-29.1992609632459,14.3641243881349,
128.769313204063)) ;
#151173=CARTESIAN_POINT('Ctrl Pts',(-29.2634796257756,14.1859981150162,
128.989963010774)) ;
#151174=CARTESIAN_POINT('Ctrl Pts',(-29.309906743687,13.9527739629267,129.158738849017)) ;
#151175=CARTESIAN_POINT('Ctrl Pts',(-29.3342115703911,13.6818171869407,
129.262851136394)) ;
#151176=CARTESIAN_POINT('Ctrl Pts',(-29.3340473631818,13.3923456599437,
129.295485666288)) ;
#151177=CARTESIAN_POINT('Ctrl Pts',(-29.3085669103323,13.1044625348289,
129.254236375475)) ;
#151178=CARTESIAN_POINT('Ctrl Pts',(-29.258986211392,12.8400820200563,129.142508243958)) ;
#151179=CARTESIAN_POINT('Ctrl Pts',(-29.1881542029012,12.6174283224968,
128.968693652698)) ;
#151180=CARTESIAN_POINT('Ctrl Pts',(-29.1002100971169,12.4521814963559,
128.744946986999)) ;
#151181=CARTESIAN_POINT('Ctrl Pts',(-29.0009103649547,12.3567835155047,
128.48800496993)) ;
#151182=CARTESIAN_POINT('Ctrl Pts',(-28.896925987083,12.3377092271658,128.21727920025)) ;
#151183=CARTESIAN_POINT('Ctrl Pts',(-28.7942667965697,12.3962076032604,
127.950545837014)) ;
#151184=CARTESIAN_POINT('Ctrl Pts',(-28.6998220504126,12.5290432373042,
127.70787965737)) ;
#151185=CARTESIAN_POINT('Ctrl Pts',(-28.6204061898145,12.7244085230837,
127.508847094626)) ;
#151186=CARTESIAN_POINT('Ctrl Pts',(-28.559819094265,12.9709500550387,127.365030411237)) ;
#151187=CARTESIAN_POINT('Ctrl Pts',(-28.5223002592329,13.2494402817627,
127.288528530129)) ;
#151188=CARTESIAN_POINT('Ctrl Pts',(-28.5097189788881,13.5418967084717,
127.285058220228)) ;
#151189=CARTESIAN_POINT('Ctrl Pts',(-28.5222097719137,13.8230883914708,
127.354499660829)) ;
#151190=CARTESIAN_POINT('Ctrl Pts',(-28.5582144837367,14.0775910910953,
127.492866930045)) ;
#151191=CARTESIAN_POINT('Ctrl Pts',(-28.6142444612186,14.2842118886259,
127.689596183375)) ;
#151192=CARTESIAN_POINT('Ctrl Pts',(-28.6857946550641,14.4299775435325,
127.931754504999)) ;
#151193=CARTESIAN_POINT('Ctrl Pts',(-28.7673480084958,14.503331032243,128.203286809695)) ;
#151194=CARTESIAN_POINT('Ctrl Pts',(-28.8509261449003,14.4992417837061,
128.480336479146)) ;
#151195=CARTESIAN_POINT('Ctrl Pts',(-28.9318023648984,14.4177939822546,
128.749907191947)) ;
#151196=CARTESIAN_POINT('Ctrl Pts',(-29.001910688641,14.2650806147523,128.987818507409)) ;
#151197=CARTESIAN_POINT('Ctrl Pts',(-29.0559489688668,14.0529681509037,
129.178698338362)) ;
#151198=CARTESIAN_POINT('Ctrl Pts',(-29.0896354038435,13.7955270319932,
129.310187588582)) ;
#151199=CARTESIAN_POINT('Ctrl Pts',(-29.099611948193,13.5095709535078,129.372622374006)) ;
#151200=CARTESIAN_POINT('Ctrl Pts',(-29.0842585907111,13.2189036520177,
129.360885383851)) ;
#151201=CARTESIAN_POINT('Ctrl Pts',(-29.0443620584725,12.9437120966298,
129.277345257376)) ;
#151202=CARTESIAN_POINT('Ctrl Pts',(-28.9817282559493,12.7018113312773,
129.127496651977)) ;
#151203=CARTESIAN_POINT('Ctrl Pts',(-28.900103185758,12.5115374792667,128.922195104015)) ;
#151204=CARTESIAN_POINT('Ctrl Pts',(-28.8047562754635,12.3865362509785,
128.676787399727)) ;
#151205=CARTESIAN_POINT('Ctrl Pts',(-28.7012853562746,12.3360647683775,
128.40778833087)) ;
#151206=CARTESIAN_POINT('Ctrl Pts',(-28.5980648305844,12.3630945002041,
128.139111767235)) ;
#151207=CARTESIAN_POINT('Ctrl Pts',(-28.4992221941751,12.4665769548229,
127.883658010127)) ;
#151208=CARTESIAN_POINT('Ctrl Pts',(-28.4131594840602,12.637873730405,127.665272376222)) ;
#151209=CARTESIAN_POINT('Ctrl Pts',(-28.3441687124707,12.8661806742055,
127.496923307267)) ;
#151210=CARTESIAN_POINT('Ctrl Pts',(-28.2971179753842,13.1333277515124,
127.392512752519)) ;
#151211=CARTESIAN_POINT('Ctrl Pts',(-28.2742141661044,13.4221934836715,
127.358771264461)) ;
#151212=CARTESIAN_POINT('Ctrl Pts',(-28.2765820238562,13.7107571318464,
127.398801174816)) ;
#151213=CARTESIAN_POINT('Ctrl Pts',(-28.3034962448371,13.9798563780996,
127.510697252844)) ;
#151214=CARTESIAN_POINT('Ctrl Pts',(-28.3518348917567,14.2070905580459,
127.684913382421)) ;
#151215=CARTESIAN_POINT('Ctrl Pts',(-28.417736051092,14.3790287482914,127.910539859451)) ;
#151216=CARTESIAN_POINT('Ctrl Pts',(-28.4956163030634,14.4826462514907,
128.171126340958)) ;
#151217=CARTESIAN_POINT('Ctrl Pts',(-28.5798455524846,14.5101765749395,
128.450506444325)) ;
#151218=CARTESIAN_POINT('Ctrl Pts',(-28.66200834704,14.4602521093363,128.723409993032)) ;
#151219=CARTESIAN_POINT('Ctrl Pts',(-28.7375813833395,14.3349863303821,
128.977516850491)) ;
#151220=CARTESIAN_POINT('Ctrl Pts',(-28.7985628235098,14.1459036519263,
129.188607444567)) ;
#151221=CARTESIAN_POINT('Ctrl Pts',(-28.8411540818564,13.9042674567381,
129.346179660859)) ;
#151222=CARTESIAN_POINT('Ctrl Pts',(-28.8610016097192,13.6274934121279,
129.437359596521)) ;
#151223=CARTESIAN_POINT('Ctrl Pts',(-28.8560349310886,13.3375401227482,
129.455886266098)) ;
#151224=CARTESIAN_POINT('Ctrl Pts',(-28.8260275084833,13.0529656397982,
129.401339308127)) ;
#151225=CARTESIAN_POINT('Ctrl Pts',(-28.7718240751871,12.793542004979,129.276308893705)) ;
#151226=CARTESIAN_POINT('Ctrl Pts',(-28.69758931411,12.5815361452067,129.09244647551)) ;
#151227=CARTESIAN_POINT('Ctrl Pts',(-28.607191982818,12.4287258471182,128.861490887195)) ;
#151228=CARTESIAN_POINT('Ctrl Pts',(-28.5062114306704,12.3470719994747,
128.599714513405)) ;
#151229=CARTESIAN_POINT('Ctrl Pts',(-28.4016831964791,12.3430683223392,
128.327512526391)) ;
#151230=CARTESIAN_POINT('Ctrl Pts',(-28.3008205475048,12.4155936091128,
128.065797526111)) ;
#151231=CARTESIAN_POINT('Ctrl Pts',(-28.2086887982306,12.5608875783812,
127.829855784513)) ;
#151232=CARTESIAN_POINT('Ctrl Pts',(-28.1322966051425,12.7672957855937,
127.639749496506)) ;
#151233=CARTESIAN_POINT('Ctrl Pts',(-28.0757288054588,13.0219896288371,
127.507742576733)) ;
#151234=CARTESIAN_POINT('Ctrl Pts',(-28.0429540969002,13.3035436342973,
127.44499916588)) ;
#151235=CARTESIAN_POINT('Ctrl Pts',(-28.0350385580784,13.5948422510341,
127.455024273178)) ;
#151236=CARTESIAN_POINT('Ctrl Pts',(-28.0521494910461,13.8739529691167,
127.538171398898)) ;
#151237=CARTESIAN_POINT('Ctrl Pts',(-28.0921989061459,14.1203174233417,
127.688276422386)) ;
#151238=CARTESIAN_POINT('Ctrl Pts',(-28.151557364416,14.3167168643634,127.894769419474)) ;
#151239=CARTESIAN_POINT('Ctrl Pts',(-28.2253962663715,14.4494066861711,
128.14361033343)) ;
#151240=CARTESIAN_POINT('Ctrl Pts',(-28.3077059790347,14.5084702688582,
128.41722565312)) ;
#151241=CARTESIAN_POINT('Ctrl Pts',(-28.3916026412673,14.489700746972,128.695408809309)) ;
#151242=CARTESIAN_POINT('Ctrl Pts',(-28.4706094716546,14.3946106074975,
128.959339303664)) ;
#151243=CARTESIAN_POINT('Ctrl Pts',(-28.5383385063881,14.2294635345246,
129.190381875795)) ;
#151244=CARTESIAN_POINT('Ctrl Pts',(-28.5888615094772,14.0073333887475,
129.371024757805)) ;
#151245=CARTESIAN_POINT('Ctrl Pts',(-28.6182752167583,13.7435828448799,
129.490009369002)) ;
#151246=CARTESIAN_POINT('Ctrl Pts',(-28.6235344183767,13.454824745877,129.538667492509)) ;
#151247=CARTESIAN_POINT('Ctrl Pts',(-28.6035941708859,13.1663898496403,
129.513405963783)) ;
#151248=CARTESIAN_POINT('Ctrl Pts',(-28.5591016772346,12.8948251888563,
129.416595319443)) ;
#151249=CARTESIAN_POINT('Ctrl Pts',(-28.4924613979654,12.6613614393991,
129.255069109059)) ;
#151250=CARTESIAN_POINT('Ctrl Pts',(-28.4079858158223,12.4827884864443,
129.041374692839)) ;
#151251=CARTESIAN_POINT('Ctrl Pts',(-28.3106810095428,12.3713198999723,
128.790256537741)) ;
#151252=CARTESIAN_POINT('Ctrl Pts',(-28.2071142233906,12.3351536539427,
128.520782151597)) ;
#151253=CARTESIAN_POINT('Ctrl Pts',(-28.1033170651269,12.3771106003778,
128.250789621036)) ;
#151254=CARTESIAN_POINT('Ctrl Pts',(-28.0070122936131,12.493746042562,128.002507073001)) ;
#151255=CARTESIAN_POINT('Ctrl Pts',(-27.9236042223444,12.6767291405437,
127.791947198724)) ;
#151256=CARTESIAN_POINT('Ctrl Pts',(-27.8582788554542,12.9147362953278,
127.634399931538)) ;
#151257=CARTESIAN_POINT('Ctrl Pts',(-27.8157639814054,13.1870897175325,
127.543206911709)) ;
#151258=CARTESIAN_POINT('Ctrl Pts',(-27.7976113632335,13.4771402294594,
127.523294837643)) ;
#151259=CARTESIAN_POINT('Ctrl Pts',(-27.8047562191335,13.7642376991577,
127.577383148529)) ;
#151260=CARTESIAN_POINT('Ctrl Pts',(-27.8359687279842,14.0261140050281,
127.701710177171)) ;
#151261=CARTESIAN_POINT('Ctrl Pts',(-27.8877875139809,14.2437566095146,
127.886037495367)) ;
#151262=CARTESIAN_POINT('Ctrl Pts',(-27.9566643830394,14.4043004510961,
128.12048462873)) ;
#151263=CARTESIAN_POINT('Ctrl Pts',(-28.0360570915207,14.4936451763547,
128.385451901082)) ;
#151264=CARTESIAN_POINT('Ctrl Pts',(-28.120129115805,14.5067755223083,128.664180642723)) ;
#151265=CARTESIAN_POINT('Ctrl Pts',(-28.2020346856407,14.4421251633059,
128.936606880987)) ;
#151266=CARTESIAN_POINT('Ctrl Pts',(-28.2751125216823,14.3039891726026,
129.183284767789)) ;
#151267=CARTESIAN_POINT('Ctrl Pts',(-28.3330260630189,14.1040922169467,
129.385445944809)) ;
#151268=CARTESIAN_POINT('Ctrl Pts',(-28.3716774412633,13.8535852347893,
129.531620171577)) ;
#151269=CARTESIAN_POINT('Ctrl Pts',(-28.3868553207156,13.5730952435811,
129.609080622274)) ;
#151270=CARTESIAN_POINT('Ctrl Pts',(-28.3771751540194,13.2829861782011,
129.613807074417)) ;
#151271=CARTESIAN_POINT('Ctrl Pts',(-28.3425095932928,13.0017737284941,
129.545666888846)) ;
#151272=CARTESIAN_POINT('Ctrl Pts',(-28.284301937165,12.7500890797144,129.408856898039)) ;
#151273=CARTESIAN_POINT('Ctrl Pts',(-28.2064572920802,12.5475577998432,
129.214559307957)) ;
#151274=CARTESIAN_POINT('Ctrl Pts',(-28.1135171544018,12.4075652478031,
128.976210428243)) ;
#151275=CARTESIAN_POINT('Ctrl Pts',(-28.0118850220544,12.3405227377109,
128.712349934362)) ;
#151276=CARTESIAN_POINT('Ctrl Pts',(-27.9073393263242,12.3506975715296,
128.440115510787)) ;
#151277=CARTESIAN_POINT('Ctrl Pts',(-27.8069898708441,12.438177489278,128.180166701549)) ;
#151278=CARTESIAN_POINT('Ctrl Pts',(-27.7177045614419,12.5958827964123,
127.952426644854)) ;
#151279=CARTESIAN_POINT('Ctrl Pts',(-27.6448174995369,12.8123887822574,
127.772559198421)) ;
#151280=CARTESIAN_POINT('Ctrl Pts',(-27.5925658802496,13.0732934241726,
127.653072879261)) ;
#151281=CARTESIAN_POINT('Ctrl Pts',(-27.5643119574423,13.3601444544887,
127.603779546763)) ;
#151282=CARTESIAN_POINT('Ctrl Pts',(-27.5613082454556,13.6487324697402,
127.627925538602)) ;
#151283=CARTESIAN_POINT('Ctrl Pts',(-27.5828722691528,13.9231969052117,
127.724074394844)) ;
#151284=CARTESIAN_POINT('Ctrl Pts',(-27.6269024064909,14.1616648845749,
127.885829090303)) ;
#151285=CARTESIAN_POINT('Ctrl Pts',(-27.6896598747405,14.3474885130478,
128.102376258084)) ;
#151286=CARTESIAN_POINT('Ctrl Pts',(-27.7653992680876,14.4664584587802,
128.356681964705)) ;
#151287=CARTESIAN_POINT('Ctrl Pts',(-27.8487981620875,14.5109046603937,
128.633576137683)) ;
#151288=CARTESIAN_POINT('Ctrl Pts',(-27.9318850392023,14.477538406395,128.909237750788)) ;
#151289=CARTESIAN_POINT('Ctrl Pts',(-28.0095052256554,14.3681997132881,
129.169245881706)) ;
#151290=CARTESIAN_POINT('Ctrl Pts',(-28.0741401659524,14.19161807787,129.391120281656)) ;
#151291=CARTESIAN_POINT('Ctrl Pts',(-28.1210449004513,13.9603524956053,
129.561209556167)) ;
#151292=CARTESIAN_POINT('Ctrl Pts',(-28.1460961632202,13.6895220911817,
129.667588782595)) ;
#151293=CARTESIAN_POINT('Ctrl Pts',(-28.1465838645101,13.4007319641459,
129.702076763037)) ;
#151294=CARTESIAN_POINT('Ctrl Pts',(-28.1219792750298,13.1132078283894,
129.663296512428)) ;
#151295=CARTESIAN_POINT('Ctrl Pts',(-28.072797303837,12.8466068578935,129.552900494661)) ;
#151296=CARTESIAN_POINT('Ctrl Pts',(-28.0028760663637,12.6236984730367,
129.381571768306)) ;
#151297=CARTESIAN_POINT('Ctrl Pts',(-27.9152289217031,12.4561011970055,
129.15875880179)) ;
#151298=CARTESIAN_POINT('Ctrl Pts',(-27.8163074914158,12.3585968124196,
128.902876316079)) ;
#151299=CARTESIAN_POINT('Ctrl Pts',(-27.7120492591559,12.3371246735504,
128.631455165304)) ;
#151300=CARTESIAN_POINT('Ctrl Pts',(-27.6093731664381,12.3935413485491,
128.364635405542)) ;
#151301=CARTESIAN_POINT('Ctrl Pts',(-27.5149001295544,12.5236723848828,
128.121769416389)) ;
#151302=CARTESIAN_POINT('Ctrl Pts',(-27.4346201824783,12.7179304240541,
127.920341279588)) ;
#151303=CARTESIAN_POINT('Ctrl Pts',(-27.3732833708595,12.9643000603806,
127.774449881944)) ;
#151304=CARTESIAN_POINT('Ctrl Pts',(-27.3353218805088,13.2410161239663,
127.696515666237)) ;
#151305=CARTESIAN_POINT('Ctrl Pts',(-27.3219345106549,13.5320326358814,
127.690536193544)) ;
#151306=CARTESIAN_POINT('Ctrl Pts',(-27.3336868555628,13.8151976332958,
127.757981771659)) ;
#151307=CARTESIAN_POINT('Ctrl Pts',(-27.3691045396702,14.070965110173,127.894657472177)) ;
#151308=CARTESIAN_POINT('Ctrl Pts',(-27.4247538548607,14.2795161854134,
128.090342542637)) ;
#151309=CARTESIAN_POINT('Ctrl Pts',(-27.495823154164,14.4266233568165,128.331023842141)) ;
#151310=CARTESIAN_POINT('Ctrl Pts',(-27.5766922115291,14.5021444966585,
128.600366276399)) ;
#151311=CARTESIAN_POINT('Ctrl Pts',(-27.6609223179021,14.5004799279669,
128.8795751742)) ;
#151312=CARTESIAN_POINT('Ctrl Pts',(-27.7417671934519,14.4210758361391,
129.14896837329)) ;
#151313=CARTESIAN_POINT('Ctrl Pts',(-27.8120265768946,14.2711637356508,
129.38719326095)) ;
#151314=CARTESIAN_POINT('Ctrl Pts',(-27.866891762874,14.0600320259714,129.580611011308)) ;
#151315=CARTESIAN_POINT('Ctrl Pts',(-27.9012411174026,13.8025046463563,
129.714162963611)) ;
#151316=CARTESIAN_POINT('Ctrl Pts',(-27.9118652501947,13.5194350300881,
129.778210865001)) ;
#151317=CARTESIAN_POINT('Ctrl Pts',(-27.8973675127668,13.227929848522,129.769057927685)) ;
#151318=CARTESIAN_POINT('Ctrl Pts',(-27.8581217638387,12.9514279979351,
129.687479679852)) ;
#151319=CARTESIAN_POINT('Ctrl Pts',(-27.7958487933346,12.7076270254922,
129.538792895781)) ;
#151320=CARTESIAN_POINT('Ctrl Pts',(-27.7150442368328,12.5164543914562,
129.335744778992)) ;
#151321=CARTESIAN_POINT('Ctrl Pts',(-27.6197799723084,12.3891143889345,
129.090666143106)) ;
#151322=CARTESIAN_POINT('Ctrl Pts',(-27.5169840616899,12.3364756158918,
128.823462340777)) ;
#151323=CARTESIAN_POINT('Ctrl Pts',(-27.4129425204162,12.3612642231578,
128.552629149903)) ;
#151324=CARTESIAN_POINT('Ctrl Pts',(-27.3139116309648,12.4629838840005,
128.296612691349)) ;
#151325=CARTESIAN_POINT('Ctrl Pts',(-27.2276350555539,12.6321971699934,
128.077535896234)) ;
#151326=CARTESIAN_POINT('Ctrl Pts',(-27.1581753164316,12.8584558798932,
127.907740199772)) ;
#151327=CARTESIAN_POINT('Ctrl Pts',(-27.1102193532803,13.1261648647243,
127.800864060768)) ;
#151328=CARTESIAN_POINT('Ctrl Pts',(-27.0867427780488,13.4141234552309,
127.765371910168)) ;
#151329=CARTESIAN_POINT('Ctrl Pts',(-27.088405263082,13.7023852342343,127.803282253112)) ;
#151330=CARTESIAN_POINT('Ctrl Pts',(-27.1144094066955,13.9714212012371,
127.912378068659)) ;
#151331=CARTESIAN_POINT('Ctrl Pts',(-27.1625636190418,14.202020081249,128.086338189894)) ;
#151332=CARTESIAN_POINT('Ctrl Pts',(-27.2279041571622,14.3750071736422,
128.310222999053)) ;
#151333=CARTESIAN_POINT('Ctrl Pts',(-27.3055089641359,14.4806351346196,
128.570006270221)) ;
#151334=CARTESIAN_POINT('Ctrl Pts',(-27.3892702869014,14.5105855297535,
128.847858683373)) ;
#151335=CARTESIAN_POINT('Ctrl Pts',(-27.4721256647169,14.4625550657111,
129.123019817885)) ;
#151336=CARTESIAN_POINT('Ctrl Pts',(-27.5475424958297,14.3400369417443,
129.376461860258)) ;
#151337=CARTESIAN_POINT('Ctrl Pts',(-27.6092868870231,14.1521957535254,
129.589908595948)) ;
#151338=CARTESIAN_POINT('Ctrl Pts',(-27.6524549950664,13.9116489154345,
129.749173070005)) ;
#151339=CARTESIAN_POINT('Ctrl Pts',(-27.6729767158619,13.6358544266559,
129.842295420114)) ;
#151340=CARTESIAN_POINT('Ctrl Pts',(-27.6687686357343,13.3459427675745,
129.863045715734)) ;
#151341=CARTESIAN_POINT('Ctrl Pts',(-27.6393546558192,13.0604649745041,
129.810291983176)) ;
#151342=CARTESIAN_POINT('Ctrl Pts',(-27.5861749748563,12.8015143832803,
129.688047174148)) ;
#151343=CARTESIAN_POINT('Ctrl Pts',(-27.5122453552566,12.586871423154,129.505215644939)) ;
#151344=CARTESIAN_POINT('Ctrl Pts',(-27.4222257102063,12.4323032180318,
129.275353955494)) ;
#151345=CARTESIAN_POINT('Ctrl Pts',(-27.321814640165,12.348604012381,129.015131363742)) ;
#151346=CARTESIAN_POINT('Ctrl Pts',(-27.2172646277251,12.3418345254331,
128.742874357153)) ;
#151347=CARTESIAN_POINT('Ctrl Pts',(-27.1155991989799,12.4127257697425,
128.479021774659)) ;
#151348=CARTESIAN_POINT('Ctrl Pts',(-27.0235546029965,12.5554430365515,
128.24317434018)) ;
#151349=CARTESIAN_POINT('Ctrl Pts',(-26.946364611968,12.7608029240068,128.050846584327)) ;
#151350=CARTESIAN_POINT('Ctrl Pts',(-26.8892425932522,13.0143079229722,
127.917197312737)) ;
#151351=CARTESIAN_POINT('Ctrl Pts',(-26.8557397574038,13.2953661026702,
127.852335782128)) ;
#151352=CARTESIAN_POINT('Ctrl Pts',(-26.8471237684322,13.587499191953,127.86040257377)) ;
#151353=CARTESIAN_POINT('Ctrl Pts',(-26.8636409106043,13.8669338626205,
127.941791701437)) ;
#151354=CARTESIAN_POINT('Ctrl Pts',(-26.9028894020443,14.1134263503453,
128.089413302891)) ;
#151355=CARTESIAN_POINT('Ctrl Pts',(-26.9618864660315,14.3121780897716,
128.294946112899)) ;
#151356=CARTESIAN_POINT('Ctrl Pts',(-27.0356609756341,14.4470050265316,
128.543696981495)) ;
#151357=CARTESIAN_POINT('Ctrl Pts',(-27.1176846698481,14.5078086325279,
128.816414339099)) ;
#151358=CARTESIAN_POINT('Ctrl Pts',(-27.2013501944063,14.4913412737729,
129.093814747738)) ;
#151359=CARTESIAN_POINT('Ctrl Pts',(-27.2805727554514,14.3985299043882,
129.358365317732)) ;
#151360=CARTESIAN_POINT('Ctrl Pts',(-27.3487809879748,14.2353764928408,
129.590815975098)) ;
#151361=CARTESIAN_POINT('Ctrl Pts',(-27.4000923756535,14.0132824388172,
129.773951949604)) ;
#151362=CARTESIAN_POINT('Ctrl Pts',(-27.4299031588905,13.751770584179,129.893917739675)) ;
#151363=CARTESIAN_POINT('Ctrl Pts',(-27.4360065328396,13.4639004603942,
129.944990740374)) ;
#151364=CARTESIAN_POINT('Ctrl Pts',(-27.4166194504997,13.1736259559936,
129.921533138526)) ;
#151365=CARTESIAN_POINT('Ctrl Pts',(-27.3730557967721,12.9029494351804,
129.827230137503)) ;
#151366=CARTESIAN_POINT('Ctrl Pts',(-27.3068239081708,12.6670694829694,
129.667025348139)) ;
#151367=CARTESIAN_POINT('Ctrl Pts',(-27.2225807375648,12.4867414535482,
129.454064281963)) ;
#151368=CARTESIAN_POINT('Ctrl Pts',(-27.1260163205075,12.3736046950475,
129.204955161642)) ;
#151369=CARTESIAN_POINT('Ctrl Pts',(-27.0219531940928,12.3351061359291,
128.934221171249)) ;
#151370=CARTESIAN_POINT('Ctrl Pts',(-26.9187654991147,12.3747297412366,
128.665782677207)) ;
#151371=CARTESIAN_POINT('Ctrl Pts',(-26.8219192185406,12.4890530273647,
128.415981781108)) ;
#151372=CARTESIAN_POINT('Ctrl Pts',(-26.7375618368722,12.6718473822343,
128.20287552548)) ;
#151373=CARTESIAN_POINT('Ctrl Pts',(-26.6721408995713,12.9071471042355,
128.044830293244)) ;
#151374=CARTESIAN_POINT('Ctrl Pts',(-26.6288268693924,13.1791583633753,
127.951366546025)) ;
#151375=CARTESIAN_POINT('Ctrl Pts',(-26.6100146219695,13.4685703303894,
127.929472625113)) ;
#151376=CARTESIAN_POINT('Ctrl Pts',(-26.6163965606096,13.7556865610863,
127.981289936006)) ;
#151377=CARTESIAN_POINT('Ctrl Pts',(-26.6468365176563,14.0184520779736,
128.103328446011)) ;
#151378=CARTESIAN_POINT('Ctrl Pts',(-26.6983664732469,14.2386835545227,
128.286981099105)) ;
#151379=CARTESIAN_POINT('Ctrl Pts',(-26.7668561678463,14.4009245247973,
128.520283146029)) ;
#151380=CARTESIAN_POINT('Ctrl Pts',(-26.8462801396179,14.4923209079493,
128.785440445302)) ;
#151381=CARTESIAN_POINT('Ctrl Pts',(-26.9299042318789,14.5074993821674,
129.062691208225)) ;
#151382=CARTESIAN_POINT('Ctrl Pts',(-27.0123042045344,14.4446391320812,
129.336708219525)) ;
#151383=CARTESIAN_POINT('Ctrl Pts',(-27.0853285109314,14.309013886893,129.583057807955)) ;
#151384=CARTESIAN_POINT('Ctrl Pts',(-27.1438828659143,14.1104149351794,
129.787163074108)) ;
#151385=CARTESIAN_POINT('Ctrl Pts',(-27.1830524640317,13.8614588559076,
129.934789891105)) ;
#151386=CARTESIAN_POINT('Ctrl Pts',(-27.1989887778394,13.5819687002437,
130.014428956727)) ;
#151387=CARTESIAN_POINT('Ctrl Pts',(-27.1899960665713,13.2906279013141,
130.021303572167)) ;
#151388=CARTESIAN_POINT('Ctrl Pts',(-27.1559614540415,13.009243305788,129.95497149067)) ;
#151389=CARTESIAN_POINT('Ctrl Pts',(-27.0987240639522,12.7575168112921,
129.820836098485)) ;
#151390=CARTESIAN_POINT('Ctrl Pts',(-27.0211347642334,12.5525240138587,
129.627409702748)) ;
#151391=CARTESIAN_POINT('Ctrl Pts',(-26.9288019853003,12.4108770336832,
129.390743830787)) ;
#151392=CARTESIAN_POINT('Ctrl Pts',(-26.8269925769389,12.3412909140522,
129.126483822534)) ;
#151393=CARTESIAN_POINT('Ctrl Pts',(-26.7225678003105,12.3493861735078,
128.854556329981)) ;
#151394=CARTESIAN_POINT('Ctrl Pts',(-26.6222736426069,12.4342727909203,
128.594675298208)) ;
#151395=CARTESIAN_POINT('Ctrl Pts',(-26.5324245140866,12.5900489009072,
128.365332500197)) ;
#151396=CARTESIAN_POINT('Ctrl Pts',(-26.4587946173494,12.8056265995217,
128.183382042886)) ;
#151397=CARTESIAN_POINT('Ctrl Pts',(-26.4059966216722,13.0653848746049,
128.062274396553)) ;
#151398=CARTESIAN_POINT('Ctrl Pts',(-26.3770384247468,13.3504851063388,
128.01077693268)) ;
#151399=CARTESIAN_POINT('Ctrl Pts',(-26.3732580768289,13.6412798147236,
128.032889399786)) ;
#151400=CARTESIAN_POINT('Ctrl Pts',(-26.3941468859038,13.915548156852,128.126957619226)) ;
#151401=CARTESIAN_POINT('Ctrl Pts',(-26.4375236270793,14.1552942040558,
128.286796725341)) ;
#151402=CARTESIAN_POINT('Ctrl Pts',(-26.499786802166,14.3429101935435,128.501891901076)) ;
#151403=CARTESIAN_POINT('Ctrl Pts',(-26.5753221744753,14.4639893047867,
128.755644371512)) ;
#151404=CARTESIAN_POINT('Ctrl Pts',(-26.658258796401,14.5107279953385,129.031049167775)) ;
#151405=CARTESIAN_POINT('Ctrl Pts',(-26.7418770326506,14.4794893752074,
129.308446128137)) ;
#151406=CARTESIAN_POINT('Ctrl Pts',(-26.819410154467,14.3727211578977,129.56804219168)) ;
#151407=CARTESIAN_POINT('Ctrl Pts',(-26.884660652684,14.1977799584113,129.791786901947)) ;
#151408=CARTESIAN_POINT('Ctrl Pts',(-26.9321606344241,13.9680803032242,
129.963592933574)) ;
#151409=CARTESIAN_POINT('Ctrl Pts',(-26.9579703404882,13.6967826933105,
130.072347583536)) ;
#151410=CARTESIAN_POINT('Ctrl Pts',(-26.9591310030642,13.4094043760888,
130.108663362794)) ;
#151411=CARTESIAN_POINT('Ctrl Pts',(-26.935231210856,13.1212039321583,130.071985580596)) ;
#151412=CARTESIAN_POINT('Ctrl Pts',(-26.8869426549206,12.8546896237207,
129.964066829109)) ;
#151413=CARTESIAN_POINT('Ctrl Pts',(-26.8174482093006,12.6293810356165,
129.794091823838)) ;
#151414=CARTESIAN_POINT('Ctrl Pts',(-26.7297563031988,12.4594635396626,
129.571300039305)) ;
#151415=CARTESIAN_POINT('Ctrl Pts',(-26.6315768169788,12.3604529302704,
129.317412505758)) ;
#151416=CARTESIAN_POINT('Ctrl Pts',(-26.527041677516,12.3366695079855,129.045292118923)) ;
#151417=CARTESIAN_POINT('Ctrl Pts',(-26.4246632418904,12.3907630606801,
128.779202667163)) ;
#151418=CARTESIAN_POINT('Ctrl Pts',(-26.3296624090555,12.5187717527639,
128.534846855937)) ;
#151419=CARTESIAN_POINT('Ctrl Pts',(-26.2486292653153,12.7125553045139,
128.331370691531)) ;
#151420=CARTESIAN_POINT('Ctrl Pts',(-26.187290463919,12.9551208485313,128.185129058602)) ;
#151421=CARTESIAN_POINT('Ctrl Pts',(-26.1482420973643,13.2325620060974,
128.104210130242)) ;
#151422=CARTESIAN_POINT('Ctrl Pts',(-26.1341913899476,13.5243419796884,
128.096383572714)) ;
#151423=CARTESIAN_POINT('Ctrl Pts',(-26.1452118388481,13.8069926528057,
128.161574113629)) ;
#151424=CARTESIAN_POINT('Ctrl Pts',(-26.1799390075941,14.0639000199269,
128.296232665471)) ;
#151425=CARTESIAN_POINT('Ctrl Pts',(-26.2350489546991,14.2741558930926,
128.490347023028)) ;
#151426=CARTESIAN_POINT('Ctrl Pts',(-26.3059077450582,14.4234615625839,
128.730487186166)) ;
#151427=CARTESIAN_POINT('Ctrl Pts',(-26.386494169588,14.5011170686614,128.998961276038)) ;
#151428=CARTESIAN_POINT('Ctrl Pts',(-26.4710372754606,14.5013614779113,
129.279215621043)) ;
#151429=CARTESIAN_POINT('Ctrl Pts',(-26.5513450363698,14.4249956630962,
129.546727763435)) ;
#151430=CARTESIAN_POINT('Ctrl Pts',(-26.6226216620681,14.2760171565871,
129.788206158856)) ;
#151431=CARTESIAN_POINT('Ctrl Pts',(-26.6777858163634,14.0665442400002,
129.982426179449)) ;
#151432=CARTESIAN_POINT('Ctrl Pts',(-26.7127743428566,13.8110528410318,
130.117741076645)) ;
#151433=CARTESIAN_POINT('Ctrl Pts',(-26.7241069347589,13.5262786463887,
130.184114351317)) ;
#151434=CARTESIAN_POINT('Ctrl Pts',(-26.7103978253846,13.2368369901033,
130.177011615775)) ;
#151435=CARTESIAN_POINT('Ctrl Pts',(-26.6716560461567,12.9583255903659,
130.097075764209)) ;
#151436=CARTESIAN_POINT('Ctrl Pts',(-26.6103674672222,12.7145800096232,
129.95106877123)) ;
#151437=CARTESIAN_POINT('Ctrl Pts',(-26.5292783226885,12.5201730384604,
129.747494551372)) ;
#151438=CARTESIAN_POINT('Ctrl Pts',(-26.4353195353877,12.392297716127,129.505869698294)) ;
#151439=CARTESIAN_POINT('Ctrl Pts',(-26.3321003131888,12.3368042043637,
129.23762472755)) ;
#151440=CARTESIAN_POINT('Ctrl Pts',(-26.2283359448761,12.3594079574846,
128.967488898529)) ;
#151441=CARTESIAN_POINT('Ctrl Pts',(-26.1289374320057,12.4588426243277,
128.710432008687)) ;
#151442=CARTESIAN_POINT('Ctrl Pts',(-26.0421433826271,12.6263832935465,
128.489874381818)) ;
#151443=CARTESIAN_POINT('Ctrl Pts',(-25.9721170036289,12.8513078071139,
128.318433909601)) ;
#151444=CARTESIAN_POINT('Ctrl Pts',(-25.9235411833855,13.1175341941134,
128.209680256936)) ;
#151445=CARTESIAN_POINT('Ctrl Pts',(-25.8992723616796,13.4059954970849,
128.171974342421)) ;
#151446=CARTESIAN_POINT('Ctrl Pts',(-25.9001789667653,13.6942419645787,
128.207632461566)) ;
#151447=CARTESIAN_POINT('Ctrl Pts',(-25.9258216003677,13.9656571359195,
128.31589284879)) ;
#151448=CARTESIAN_POINT('Ctrl Pts',(-25.9727492712161,14.1945698215837,
128.485818180082)) ;
#151449=CARTESIAN_POINT('Ctrl Pts',(-26.0380351219601,14.3711224528334,
128.709801837872)) ;
#151450=CARTESIAN_POINT('Ctrl Pts',(-26.115372034482,14.4785950091488,128.968780330961)) ;
#151451=CARTESIAN_POINT('Ctrl Pts',(-26.1991386228248,14.5108133112394,
129.246686766249)) ;
#151452=CARTESIAN_POINT('Ctrl Pts',(-26.281961118953,14.4650394200622,129.521689731091)) ;
#151453=CARTESIAN_POINT('Ctrl Pts',(-26.3576691539897,14.3446919400874,
129.775975443665)) ;
#151454=CARTESIAN_POINT('Ctrl Pts',(-26.4199450377268,14.1586507898245,
129.990981699106)) ;
#151455=CARTESIAN_POINT('Ctrl Pts',(-26.4638325348643,13.9182142591253,
130.152493567261)) ;
#151456=CARTESIAN_POINT('Ctrl Pts',(-26.4849121372087,13.6446894301756,
130.247054976681)) ;
#151457=CARTESIAN_POINT('Ctrl Pts',(-26.4814409395297,13.3538163555555,
130.270090586414)) ;
#151458=CARTESIAN_POINT('Ctrl Pts',(-26.4527946492839,13.0687529323482,
130.219476965581)) ;
#151459=CARTESIAN_POINT('Ctrl Pts',(-26.4002320096581,12.8084025711039,
130.099079794229)) ;
#151460=CARTESIAN_POINT('Ctrl Pts',(-26.3268756685072,12.5923662507696,
129.91790410308)) ;
#151461=CARTESIAN_POINT('Ctrl Pts',(-26.2371123368209,12.4355966936421,
129.688843066008)) ;
#151462=CARTESIAN_POINT('Ctrl Pts',(-26.1367181878628,12.3498834173245,
129.42872587461)) ;
#151463=CARTESIAN_POINT('Ctrl Pts',(-26.032722719753,12.3409542808635,129.157919642926)) ;
#151464=CARTESIAN_POINT('Ctrl Pts',(-25.9308084387583,12.4093757248112,
128.893357587352)) ;
#151465=CARTESIAN_POINT('Ctrl Pts',(-25.838155620905,12.5505196315372,128.655821078007)) ;
#151466=CARTESIAN_POINT('Ctrl Pts',(-25.7605740007468,12.7541803006072,
128.462316845571)) ;
#151467=CARTESIAN_POINT('Ctrl Pts',(-25.7029450253967,13.0055267425044,
128.327067990315)) ;
#151468=CARTESIAN_POINT('Ctrl Pts',(-25.6685657347824,13.2870724884799,
128.259776019344)) ;
#151469=CARTESIAN_POINT('Ctrl Pts',(-25.6592502061655,13.5781354317469,
128.265673438089)) ;
#151470=CARTESIAN_POINT('Ctrl Pts',(-25.6749179654199,13.8583662507443,
128.344586199981)) ;
#151471=CARTESIAN_POINT('Ctrl Pts',(-25.7137374162889,14.1072755060793,
128.491117013587)) ;
#151472=CARTESIAN_POINT('Ctrl Pts',(-25.7721169966564,14.3069765889331,
128.694755702354)) ;
#151473=CARTESIAN_POINT('Ctrl Pts',(-25.845207577047,14.443614067786,128.941381531894)) ;
#151474=CARTESIAN_POINT('Ctrl Pts',(-25.9273346325596,14.5071928082345,
129.214515131727)) ;
#151475=CARTESIAN_POINT('Ctrl Pts',(-26.011234962119,14.4928945220509,129.492675842775)) ;
#151476=CARTESIAN_POINT('Ctrl Pts',(-26.0906570279007,14.4021254936154,
129.757803067043)) ;
#151477=CARTESIAN_POINT('Ctrl Pts',(-26.159082383682,14.2413770477371,129.990792154917)) ;
#151478=CARTESIAN_POINT('Ctrl Pts',(-26.2110152100895,14.0210258594474,
130.175736142196)) ;
#151479=CARTESIAN_POINT('Ctrl Pts',(-26.241635177827,13.7594508415378,130.298196601018)) ;
#151480=CARTESIAN_POINT('Ctrl Pts',(-26.2483473113095,13.4716753030503,
130.351078692086)) ;
#151481=CARTESIAN_POINT('Ctrl Pts',(-26.2298541426232,13.18278007244,130.330045835803)) ;
#151482=CARTESIAN_POINT('Ctrl Pts',(-26.1867418068547,12.9097866347109,
130.237249070666)) ;
#151483=CARTESIAN_POINT('Ctrl Pts',(-26.1214552754847,12.6739761120234,
130.079613973061)) ;
#151484=CARTESIAN_POINT('Ctrl Pts',(-26.037598712626,12.4911376353209,129.867849268882)) ;
#151485=CARTESIAN_POINT('Ctrl Pts',(-25.9407649580424,12.3755758788311,
129.618129131331)) ;
#151486=CARTESIAN_POINT('Ctrl Pts',(-25.8374214950217,12.3352662329562,
129.34929906656)) ;
#151487=CARTESIAN_POINT('Ctrl Pts',(-25.7340098362028,12.3722006143293,
129.0802369826)) ;
#151488=CARTESIAN_POINT('Ctrl Pts',(-25.6361773432197,12.4858118722087,
128.827819165484)) ;
#151489=CARTESIAN_POINT('Ctrl Pts',(-25.5523274084712,12.6649628027199,
128.615825895545)) ;
#151490=CARTESIAN_POINT('Ctrl Pts',(-25.4859513870995,12.8995424291904,
128.455121245363)) ;
#151491=CARTESIAN_POINT('Ctrl Pts',(-25.4419863750333,13.1707489990253,
128.359746169264)) ;
#151492=CARTESIAN_POINT('Ctrl Pts',(-25.4224009992562,13.4602465419289,
128.335630931104)) ;
#151493=CARTESIAN_POINT('Ctrl Pts',(-25.4281061795563,13.7479094104328,
128.385491263721)) ;
#151494=CARTESIAN_POINT('Ctrl Pts',(-25.4578216450762,14.0110933638022,
128.505345635233)) ;
#151495=CARTESIAN_POINT('Ctrl Pts',(-25.5087967768197,14.2330195298938,
128.687396943834)) ;
#151496=CARTESIAN_POINT('Ctrl Pts',(-25.5768933622651,14.397056415232,128.919554215411)) ;
#151497=CARTESIAN_POINT('Ctrl Pts',(-25.6558147544988,14.4906410938832,
129.183138561615)) ;
#151498=CARTESIAN_POINT('Ctrl Pts',(-25.7399301950195,14.5080280130628,
129.462041474598)) ;
#151499=CARTESIAN_POINT('Ctrl Pts',(-25.8217364878674,14.4480725424633,
129.734011003358)) ;
#151500=CARTESIAN_POINT('Ctrl Pts',(-25.8956483813608,14.3139470607326,
129.983179734343)) ;
#151501=CARTESIAN_POINT('Ctrl Pts',(-25.9546615112484,14.1169437524237,
130.188609280051)) ;
#151502=CARTESIAN_POINT('Ctrl Pts',(-25.994519421204,13.8684682048696,130.338337741358)) ;
#151503=CARTESIAN_POINT('Ctrl Pts',(-26.0110568377318,13.5907243651,130.419594305655)) ;
#151504=CARTESIAN_POINT('Ctrl Pts',(-26.0028570943019,13.2994062522709,
130.428791647391)) ;
#151505=CARTESIAN_POINT('Ctrl Pts',(-25.9695704025357,13.0173302811176,
130.364651136717)) ;
#151506=CARTESIAN_POINT('Ctrl Pts',(-25.9127012517306,12.7634586998748,
130.23173138777)) ;
#151507=CARTESIAN_POINT('Ctrl Pts',(-25.8356694959319,12.5574053612187,
130.039883250671)) ;
#151508=CARTESIAN_POINT('Ctrl Pts',(-25.7439581375389,12.4141338116398,
129.804942699892)) ;
#151509=CARTESIAN_POINT('Ctrl Pts',(-25.6422361078924,12.342233208706,129.540970477651)) ;
#151510=CARTESIAN_POINT('Ctrl Pts',(-25.5379082160016,12.3479816385131,
129.269286803224)) ;
#151511=CARTESIAN_POINT('Ctrl Pts',(-25.4372492426153,12.4308508598937,
129.00839512309)) ;
#151512=CARTESIAN_POINT('Ctrl Pts',(-25.3472402005208,12.5841342714032,
128.778486490676)) ;
#151513=CARTESIAN_POINT('Ctrl Pts',(-25.272730898508,12.7991564308112,128.594122402279)) ;
#151514=CARTESIAN_POINT('Ctrl Pts',(-25.2194888387276,13.0569999610756,
128.471595214616)) ;
#151515=CARTESIAN_POINT('Ctrl Pts',(-25.1897401476562,13.3421921034464,
128.417860044275)) ;
#151516=CARTESIAN_POINT('Ctrl Pts',(-25.1851966857885,13.6321454574867,
128.437625751363)) ;
#151517=CARTESIAN_POINT('Ctrl Pts',(-25.2054882351433,13.9089725412032,
128.530163374861)) ;
#151518=CARTESIAN_POINT('Ctrl Pts',(-25.2484501051326,14.1498188340954,
128.688812325716)) ;
#151519=CARTESIAN_POINT('Ctrl Pts',(-25.3098239459612,14.3379335225619,
128.901090604678)) ;
#151520=CARTESIAN_POINT('Ctrl Pts',(-25.3852409841119,14.4615825769609,
129.154594863581)) ;
#151521=CARTESIAN_POINT('Ctrl Pts',(-25.4680078103566,14.5104718339952,
129.429479188798)) ;
#151522=CARTESIAN_POINT('Ctrl Pts',(-25.5519233175472,14.4813917081873,
129.707831723369)) ;
#151523=CARTESIAN_POINT('Ctrl Pts',(-25.6296594879759,14.3764101476522,
129.968016081421)) ;
#151524=CARTESIAN_POINT('Ctrl Pts',(-25.6951131634194,14.2041613001764,
130.192211432841)) ;
#151525=CARTESIAN_POINT('Ctrl Pts',(-25.7434116042681,13.9743839791119,
130.36655070585)) ;
#151526=CARTESIAN_POINT('Ctrl Pts',(-25.7697062526325,13.7063210401926,
130.476427371815)) ;
#151527=CARTESIAN_POINT('Ctrl Pts',(-25.7716643333024,13.416701167449,130.515370896243)) ;
#151528=CARTESIAN_POINT('Ctrl Pts',(-25.7484303453548,13.1291677758352,
130.480525076402)) ;
#151529=CARTESIAN_POINT('Ctrl Pts',(-25.7008468729498,12.86171027905,130.374668312212)) ;
#151530=CARTESIAN_POINT('Ctrl Pts',(-25.6318421414092,12.6350478480017,
130.206135995294)) ;
#151531=CARTESIAN_POINT('Ctrl Pts',(-25.5450073178082,12.4638699665219,
129.985698129429)) ;
#151532=CARTESIAN_POINT('Ctrl Pts',(-25.4465855133018,12.3621126869917,
129.731275230113)) ;
#151533=CARTESIAN_POINT('Ctrl Pts',(-25.3422723144961,12.336288293437,129.459748523319)) ;
#151534=CARTESIAN_POINT('Ctrl Pts',(-25.2395464146887,12.3882079133966,
129.192710014154)) ;
#151535=CARTESIAN_POINT('Ctrl Pts',(-25.1441554739243,12.5148240028862,
128.947268201873)) ;
#151536=CARTESIAN_POINT('Ctrl Pts',(-25.0632912716036,12.7050812653244,
128.743995286524)) ;
#151537=CARTESIAN_POINT('Ctrl Pts',(-25.0008040035337,12.9482677220772,
128.594669933562)) ;
#151538=CARTESIAN_POINT('Ctrl Pts',(-24.9612989083473,13.2238578222556,
128.512263188183)) ;
#151539=CARTESIAN_POINT('Ctrl Pts',(-24.9464400414306,13.5162932448957,
128.502169911524)) ;
#151540=CARTESIAN_POINT('Ctrl Pts',(-24.9567559801261,13.799165239793,128.565264390033)) ;
#151541=CARTESIAN_POINT('Ctrl Pts',(-24.9910303138475,14.0580267764743,
128.698731518742)) ;
#151542=CARTESIAN_POINT('Ctrl Pts',(-25.0453888541943,14.2686028129511,
128.890481281382)) ;
#151543=CARTESIAN_POINT('Ctrl Pts',(-25.1157749327763,14.4199618502008,
129.129219228183)) ;
#151544=CARTESIAN_POINT('Ctrl Pts',(-25.1962537469819,14.4998958219189,
129.397417258709)) ;
#151545=CARTESIAN_POINT('Ctrl Pts',(-25.2806998076144,14.5025664794371,
129.677347381576)) ;
#151546=CARTESIAN_POINT('Ctrl Pts',(-25.3614130293349,14.4280652825415,
129.946141834169)) ;
#151547=CARTESIAN_POINT('Ctrl Pts',(-25.4327613411336,14.2819177513075,
130.187667258866)) ;
#151548=CARTESIAN_POINT('Ctrl Pts',(-25.4888836010397,14.0723877227319,
130.384948804485)) ;
#151549=CARTESIAN_POINT('Ctrl Pts',(-25.524217369076,13.8191595273478,130.52109290564)) ;
#151550=CARTESIAN_POINT('Ctrl Pts',(-25.5363621720147,13.5356702848312,
130.589764696207)) ;
#151551=CARTESIAN_POINT('Ctrl Pts',(-25.5233799731752,13.2451626614465,
130.584896539849)) ;
#151552=CARTESIAN_POINT('Ctrl Pts',(-25.4853193673611,12.9658959397094,
130.506957297054)) ;
#151553=CARTESIAN_POINT('Ctrl Pts',(-25.4245567948317,12.720867949973,130.362513148524)) ;
#151554=CARTESIAN_POINT('Ctrl Pts',(-25.3444357384131,12.5256178596935,
130.161588938401)) ;
#151555=CARTESIAN_POINT('Ctrl Pts',(-25.2502354927177,12.3947249390078,
129.91946984754)) ;
#151556=CARTESIAN_POINT('Ctrl Pts',(-25.1471557384846,12.3373274128747,
129.651622343389)) ;
#151557=CARTESIAN_POINT('Ctrl Pts',(-25.04352722843,12.3577351376061,129.3818280718)) ;
#151558=CARTESIAN_POINT('Ctrl Pts',(-24.9440625937448,12.4546492514378,
129.124509048456)) ;
#151559=CARTESIAN_POINT('Ctrl Pts',(-24.8564471604785,12.6210676591383,
128.901700870073)) ;
#151560=CARTESIAN_POINT('Ctrl Pts',(-24.7859855036776,12.8446766854148,
128.728972290107)) ;
#151561=CARTESIAN_POINT('Ctrl Pts',(-24.7369148940067,13.108808163257,128.618635013836)) ;
#151562=CARTESIAN_POINT('Ctrl Pts',(-24.7117898455147,13.3979062620311,
128.578541432007)) ;
#151563=CARTESIAN_POINT('Ctrl Pts',(-24.7120774707783,13.6859097607706,
128.612344349061)) ;
#151564=CARTESIAN_POINT('Ctrl Pts',(-24.7366917620368,13.9567565280856,
128.717390290963)) ;
#151565=CARTESIAN_POINT('Ctrl Pts',(-24.7836759760245,14.1899349125241,
128.887914867791)) ;
#151566=CARTESIAN_POINT('Ctrl Pts',(-24.8478937377255,14.3662692626876,
129.10842421568)) ;
#151567=CARTESIAN_POINT('Ctrl Pts',(-24.9254379812952,14.4768289979695,
129.368240618362)) ;
#151568=CARTESIAN_POINT('Ctrl Pts',(-25.0089189154175,14.5109207090365,
129.645218161262)) ;
#151569=CARTESIAN_POINT('Ctrl Pts',(-25.0919501200887,14.4673589954117,
129.920875758852)) ;
#151570=CARTESIAN_POINT('Ctrl Pts',(-25.1679324131496,14.3490298117359,
130.175949093355)) ;
#151571=CARTESIAN_POINT('Ctrl Pts',(-25.2306776791176,14.1643442573792,
130.392364551844)) ;
#151572=CARTESIAN_POINT('Ctrl Pts',(-25.2749172208417,13.9269540764464,
130.554674425406)) ;
#151573=CARTESIAN_POINT('Ctrl Pts',(-25.296881801977,13.6529087066834,130.651991768824)) ;
#151574=CARTESIAN_POINT('Ctrl Pts',(-25.294121582554,13.3625040426011,130.677064089887)) ;
#151575=CARTESIAN_POINT('Ctrl Pts',(-25.2661584777254,13.0764917625792,
130.628507586136)) ;
#151576=CARTESIAN_POINT('Ctrl Pts',(-25.2142358128611,12.8152457852602,
130.509968872735)) ;
#151577=CARTESIAN_POINT('Ctrl Pts',(-25.1414105163864,12.5977360848388,
130.330346617025)) ;
#151578=CARTESIAN_POINT('Ctrl Pts',(-25.0521369052221,12.4392301767845,
130.102679861577)) ;
#151579=CARTESIAN_POINT('Ctrl Pts',(-24.9519825847367,12.3513755992719,
129.843259987167)) ;
#151580=CARTESIAN_POINT('Ctrl Pts',(-24.8480528333298,12.3399316332142,
129.572627714051)) ;
#151581=CARTESIAN_POINT('Ctrl Pts',(-24.7452323261505,12.4070554351268,
129.305672373312)) ;
#151582=CARTESIAN_POINT('Ctrl Pts',(-24.653114699296,12.5451369869361,129.069390792946)) ;
#151583=CARTESIAN_POINT('Ctrl Pts',(-24.574658401759,12.7477726868892,128.873467031278)) ;
#151584=CARTESIAN_POINT('Ctrl Pts',(-24.516485448288,12.9979367372735,128.736605448719)) ;
#151585=CARTESIAN_POINT('Ctrl Pts',(-24.4813744014041,13.2792370978739,
128.667217092649)) ;
#151586=CARTESIAN_POINT('Ctrl Pts',(-24.4713970354524,13.5701580555343,
128.671163049425)) ;
#151587=CARTESIAN_POINT('Ctrl Pts',(-24.4863380916386,13.8505377724051,
128.747899411962)) ;
#151588=CARTESIAN_POINT('Ctrl Pts',(-24.5245439679385,14.1007512372239,
128.892655666103)) ;
#151589=CARTESIAN_POINT('Ctrl Pts',(-24.5824402788279,14.3021715583994,
129.094893574169)) ;
#151590=CARTESIAN_POINT('Ctrl Pts',(-24.6554257346924,14.4410638226486,
129.341309329826)) ;
#151591=CARTESIAN_POINT('Ctrl Pts',(-24.7373356695316,14.506420576945,129.613776649341)) ;
#151592=CARTESIAN_POINT('Ctrl Pts',(-24.8210078848283,14.4944296739133,
129.89116801343)) ;
#151593=CARTESIAN_POINT('Ctrl Pts',(-24.9008406879447,14.4055611915821,
130.157574926146)) ;
#151594=CARTESIAN_POINT('Ctrl Pts',(-24.9694636925505,14.2469875620131,
130.391056099313)) ;
#151595=CARTESIAN_POINT('Ctrl Pts',(-25.0219599711088,14.0284942715184,
130.577615505577)) ;
#151596=CARTESIAN_POINT('Ctrl Pts',(-25.053320022464,13.7670074742828,130.70234813533)) ;
#151597=CARTESIAN_POINT('Ctrl Pts',(-25.0607089051815,13.4805781215048,
130.757097162265)) ;
#151598=CARTESIAN_POINT('Ctrl Pts',(-25.0430061476845,13.1913388058783,
130.73838961606)) ;
#151599=CARTESIAN_POINT('Ctrl Pts',(-25.0005234997867,12.9172330933754,
130.647473812606)) ;
#151600=CARTESIAN_POINT('Ctrl Pts',(-24.9358367964898,12.6799728703758,
130.491596969194)) ;
#151601=CARTESIAN_POINT('Ctrl Pts',(-24.8520526958292,12.4949910418975,
130.280173035867)) ;
#151602=CARTESIAN_POINT('Ctrl Pts',(-24.756283433586,12.3781840447206,130.033296564361)) ;
#151603=CARTESIAN_POINT('Ctrl Pts',(-24.6522083130104,12.3352411023339,
129.762603753164)) ;
#151604=CARTESIAN_POINT('Ctrl Pts',(-24.5492013359519,12.3701183957634,
129.494563600041)) ;
#151605=CARTESIAN_POINT('Ctrl Pts',(-24.4510228781676,12.4815908370187,
129.241159666924)) ;
#151606=CARTESIAN_POINT('Ctrl Pts',(-24.3668186999168,12.6586744463426,
129.02808228214)) ;
#151607=CARTESIAN_POINT('Ctrl Pts',(-24.2996856218142,12.8927064505131,
128.86527445598)) ;
#151608=CARTESIAN_POINT('Ctrl Pts',(-24.2552426505653,13.1615895986342,
128.768318934161)) ;
#151609=CARTESIAN_POINT('Ctrl Pts',(-24.2347791741716,13.4527337961883,
128.741859841865)) ;
#151610=CARTESIAN_POINT('Ctrl Pts',(-24.2398184692911,13.7397606263225,
128.789657130047)) ;
#151611=CARTESIAN_POINT('Ctrl Pts',(-24.2689320023009,14.0044956878458,
128.907831044878)) ;
#151612=CARTESIAN_POINT('Ctrl Pts',(-24.3192589693072,14.2270717047825,
129.087893938316)) ;
#151613=CARTESIAN_POINT('Ctrl Pts',(-24.386637598686,14.3928428531141,129.31784383242)) ;
#151614=CARTESIAN_POINT('Ctrl Pts',(-24.4659391407555,14.4891679896536,
129.582798342604)) ;
#151615=CARTESIAN_POINT('Ctrl Pts',(-24.5493645856168,14.5086708936273,
129.859423076708)) ;
#151616=CARTESIAN_POINT('Ctrl Pts',(-24.6318807172738,14.4507091204102,
130.133696348165)) ;
#151617=CARTESIAN_POINT('Ctrl Pts',(-24.7058567597393,14.318823465338,130.382937634357)) ;
#151618=CARTESIAN_POINT('Ctrl Pts',(-24.7654056750014,14.1234067424229,
130.589957999186)) ;
#151619=CARTESIAN_POINT('Ctrl Pts',(-24.8057595992627,13.8772496577341,
130.740994985991)) ;
#151620=CARTESIAN_POINT('Ctrl Pts',(-24.8231799857801,13.5994498547175,
130.82492878504)) ;
#151621=CARTESIAN_POINT('Ctrl Pts',(-24.8155893045152,13.3067289539218,
130.836068714423)) ;
#151622=CARTESIAN_POINT('Ctrl Pts',(-24.7830973206933,13.025513208076,130.774091996489)) ;
#151623=CARTESIAN_POINT('Ctrl Pts',(-24.7270577046474,12.7708776887036,
130.643534343482)) ;
#151624=CARTESIAN_POINT('Ctrl Pts',(-24.6505077984341,12.5628412979246,
130.453131427416)) ;
#151625=CARTESIAN_POINT('Ctrl Pts',(-24.5589760348122,12.4171764122364,
130.218786009453)) ;
#151626=CARTESIAN_POINT('Ctrl Pts',(-24.4570551071365,12.3431378359771,
129.954350410602)) ;
#151627=CARTESIAN_POINT('Ctrl Pts',(-24.3533214115063,12.3467434972734,
129.684210676246)) ;
#151628=CARTESIAN_POINT('Ctrl Pts',(-24.2523283182393,12.4272274658185,
129.422376802438)) ;
#151629=CARTESIAN_POINT('Ctrl Pts',(-24.1617932807192,12.5790158149027,
129.190994958755)) ;
#151630=CARTESIAN_POINT('Ctrl Pts',(-24.0869579392724,12.7916687829571,
129.005564094205)) ;
#151631=CARTESIAN_POINT('Ctrl Pts',(-24.0328055760906,13.0498138992039,
128.8805514449)) ;
#151632=CARTESIAN_POINT('Ctrl Pts',(-24.002521804032,13.3331756720239,128.825089124936)) ;
#151633=CARTESIAN_POINT('Ctrl Pts',(-23.9971725769105,13.6238935345468,
128.842575947387)) ;
#151634=CARTESIAN_POINT('Ctrl Pts',(-24.0167753636582,13.9010885274901,
128.933062863381)) ;
#151635=CARTESIAN_POINT('Ctrl Pts',(-24.0590128945408,14.1432054793993,
129.089568959686)) ;
#151636=CARTESIAN_POINT('Ctrl Pts',(-24.1203695555296,14.3341070280144,
129.302019247719)) ;
#151637=CARTESIAN_POINT('Ctrl Pts',(-24.1950418049019,14.4587991787124,
129.553138711427)) ;
#151638=CARTESIAN_POINT('Ctrl Pts',(-24.2777268658875,14.5101605081857,
129.827811432152)) ;
#151639=CARTESIAN_POINT('Ctrl Pts',(-24.3615395865942,14.4834097576633,
130.105796352381)) ;
#151640=CARTESIAN_POINT('Ctrl Pts',(-24.4396001237497,14.380986704451,130.366925214371)) ;
#151641=CARTESIAN_POINT('Ctrl Pts',(-24.5059188478657,14.2089571607828,
130.593906733665)) ;
#151642=CARTESIAN_POINT('Ctrl Pts',(-24.5543423873352,13.9828180453883,
130.768283768123)) ;
#151643=CARTESIAN_POINT('Ctrl Pts',(-24.5815804292821,13.7132629209954,
130.881224790375)) ;
#151644=CARTESIAN_POINT('Ctrl Pts',(-24.5841620980753,13.42583764063,130.921759059005)) ;
#151645=CARTESIAN_POINT('Ctrl Pts',(-24.5616991302751,13.1374631065902,
130.889232264708)) ;
#151646=CARTESIAN_POINT('Ctrl Pts',(-24.5148271925072,12.8691197006536,
130.785439835784)) ;
#151647=CARTESIAN_POINT('Ctrl Pts',(-24.4460595852779,12.6403113443668,
130.617737495797)) ;
#151648=CARTESIAN_POINT('Ctrl Pts',(-24.3602783070861,12.468420702256,130.400139902644)) ;
#151649=CARTESIAN_POINT('Ctrl Pts',(-24.2614984282295,12.3638000217504,
130.144889114756)) ;
#151650=CARTESIAN_POINT('Ctrl Pts',(-24.1577920148866,12.3359859144704,
129.874955907544)) ;
#151651=CARTESIAN_POINT('Ctrl Pts',(-24.054756872384,12.3855342690204,129.607074345636)) ;
#151652=CARTESIAN_POINT('Ctrl Pts',(-23.9592387590454,12.5097023136888,
129.361184743235)) ;
#151653=CARTESIAN_POINT('Ctrl Pts',(-23.8775758716564,12.6987169895182,
129.155691106511)) ;
#151654=CARTESIAN_POINT('Ctrl Pts',(-23.8143557456443,12.9413958856346,
129.004310292951)) ;
#151655=CARTESIAN_POINT('Ctrl Pts',(-23.7742609530853,13.2164083911014,
128.920187229679)) ;
#151656=CARTESIAN_POINT('Ctrl Pts',(-23.7587189631835,13.5077476116907,
128.907983756604)) ;
#151657=CARTESIAN_POINT('Ctrl Pts',(-23.7683966260473,13.7917084995172,
128.969294505237)) ;
#151658=CARTESIAN_POINT('Ctrl Pts',(-23.8017090745378,14.0497089633418,
129.099691778832)) ;
#151659=CARTESIAN_POINT('Ctrl Pts',(-23.855687851068,14.2632250030891,129.290500820459)) ;
#151660=CARTESIAN_POINT('Ctrl Pts',(-23.9259445764529,14.4168537708596,
129.528960264585)) ;
#151661=CARTESIAN_POINT('Ctrl Pts',(-24.0063154571533,14.4987598986465,
129.796873298139)) ;
#151662=CARTESIAN_POINT('Ctrl Pts',(-24.0905209887515,14.5035045718472,
130.07601230486)) ;
#151663=CARTESIAN_POINT('Ctrl Pts',(-24.1714640122117,14.4313229997249,
130.345485263966)) ;
#151664=CARTESIAN_POINT('Ctrl Pts',(-24.243380136318,14.286096674379,130.588809864043)) ;
#151665=CARTESIAN_POINT('Ctrl Pts',(-24.2994203289572,14.0806888556304,
130.785462444038)) ;
#151666=CARTESIAN_POINT('Ctrl Pts',(-24.3358061636431,13.8265805447723,
130.924971011733)) ;
#151667=CARTESIAN_POINT('Ctrl Pts',(-24.3485662665821,13.5441879409374,
130.995358908411)) ;
#151668=CARTESIAN_POINT('Ctrl Pts',(-24.3362787692544,13.2530370689606,
130.992594119063)) ;
#151669=CARTESIAN_POINT('Ctrl Pts',(-24.2990565233592,12.9741114175935,
130.916980614884)) ;
#151670=CARTESIAN_POINT('Ctrl Pts',(-24.2387980421576,12.7272119216586,
130.774093243821)) ;
#151671=CARTESIAN_POINT('Ctrl Pts',(-24.1592542721153,12.5305677659782,
130.57481255156)) ;
#151672=CARTESIAN_POINT('Ctrl Pts',(-24.0653992661587,12.3976028767503,
130.333704016612)) ;
#151673=CARTESIAN_POINT('Ctrl Pts',(-23.9625403093089,12.3378877564715,
130.06647786499)) ;
#151674=CARTESIAN_POINT('Ctrl Pts',(-23.8586656317476,12.3561146457162,
129.796030313594)) ;
#151675=CARTESIAN_POINT('Ctrl Pts',(-23.7592617382335,12.4504996091204,
129.538781451731)) ;
#151676=CARTESIAN_POINT('Ctrl Pts',(-23.6710781493093,12.6151918179393,
129.314368558311)) ;
#151677=CARTESIAN_POINT('Ctrl Pts',(-23.6000847768971,12.8367627956422,
129.140023816127)) ;
#151678=CARTESIAN_POINT('Ctrl Pts',(-23.5500037307086,13.102471284239,129.027040548326)) ;
#151679=CARTESIAN_POINT('Ctrl Pts',(-23.5244629176484,13.388098474674,128.985365037134)) ;
#151680=CARTESIAN_POINT('Ctrl Pts',(-23.5239179211507,13.6786302634614,
129.017000214703)) ;
#151681=CARTESIAN_POINT('Ctrl Pts',(-23.5479482075075,13.9495118019851,
129.120261172471)) ;
#151682=CARTESIAN_POINT('Ctrl Pts',(-23.5940539896427,14.1831630717315,
129.28807205042)) ;
#151683=CARTESIAN_POINT('Ctrl Pts',(-23.658087369295,14.3622887251467,129.508197418047)) ;
#151684=CARTESIAN_POINT('Ctrl Pts',(-23.7354964858561,14.4748192529362,
129.767663246934)) ;
#151685=CARTESIAN_POINT('Ctrl Pts',(-23.8186008712506,14.5109473630978,
130.043427649505)) ;
#151686=CARTESIAN_POINT('Ctrl Pts',(-23.9016485189198,14.46989386631,130.319093678178)) ;
#151687=CARTESIAN_POINT('Ctrl Pts',(-23.9780326629865,14.3536144736526,
130.57538079303)) ;
#151688=CARTESIAN_POINT('Ctrl Pts',(-24.041317392537,14.17062113719,130.793395793898)) ;
#151689=CARTESIAN_POINT('Ctrl Pts',(-24.0862233608817,13.933736573907,130.957750623604)) ;
#151690=CARTESIAN_POINT('Ctrl Pts',(-24.1087782693582,13.6617104442443,
131.056639640472)) ;
#151691=CARTESIAN_POINT('Ctrl Pts',(-24.1067652069901,13.3701432171844,
131.084050982405)) ;
#151692=CARTESIAN_POINT('Ctrl Pts',(-24.0794150200347,13.0839501475181,
131.037263800254)) ;
#151693=CARTESIAN_POINT('Ctrl Pts',(-24.0283415442683,12.8226369063403,
130.921088721576)) ;
#151694=CARTESIAN_POINT('Ctrl Pts',(-23.9561135287856,12.6036153158418,
130.74320474868)) ;
#151695=CARTESIAN_POINT('Ctrl Pts',(-23.8674374985634,12.4432239429731,
130.517228131168)) ;
#151696=CARTESIAN_POINT('Ctrl Pts',(-23.7669177824065,12.3525997513282,
130.256937329486)) ;
#151697=CARTESIAN_POINT('Ctrl Pts',(-23.6631589097691,12.3393903655815,
129.986759745082)) ;
#151698=CARTESIAN_POINT('Ctrl Pts',(-23.5608451726887,12.403468098602,129.721057322036)) ;
#151699=CARTESIAN_POINT('Ctrl Pts',(-23.4675538333872,12.5405072085783,
129.481626938511)) ;
#151700=CARTESIAN_POINT('Ctrl Pts',(-23.388662980097,12.7420005519616,129.284449551793)) ;
#151701=CARTESIAN_POINT('Ctrl Pts',(-23.3301053404809,12.9900801149227,
129.146339662681)) ;
#151702=CARTESIAN_POINT('Ctrl Pts',(-23.2942598700259,13.2708158721555,
129.07481369419)) ;
#151703=CARTESIAN_POINT('Ctrl Pts',(-23.2835507653219,13.5613604134334,
129.07658052044)) ;
#151704=CARTESIAN_POINT('Ctrl Pts',(-23.2977457009926,13.8428560081929,
129.151189048699)) ;
#151705=CARTESIAN_POINT('Ctrl Pts',(-23.3355877732922,14.0951246502648,
129.295029201952)) ;
#151706=CARTESIAN_POINT('Ctrl Pts',(-23.392640021767,14.2968154125605,129.494589775277)) ;
#151707=CARTESIAN_POINT('Ctrl Pts',(-23.4654695271126,14.4382062812648,
129.740653917803)) ;
#151708=CARTESIAN_POINT('Ctrl Pts',(-23.5470349400498,14.5055713938207,
130.012034404642)) ;
#151709=CARTESIAN_POINT('Ctrl Pts',(-23.6308595315768,14.4957941932041,
130.289927886282)) ;
#151710=CARTESIAN_POINT('Ctrl Pts',(-23.7106798599952,14.4095662340998,
130.556186374908)) ;
#151711=CARTESIAN_POINT('Ctrl Pts',(-23.7802571461447,14.2515335127425,
130.792730605287)) ;
#151712=CARTESIAN_POINT('Ctrl Pts',(-23.8330271584667,14.0347236874785,
130.979999898394)) ;
#151713=CARTESIAN_POINT('Ctrl Pts',(-23.8649144470802,13.7751700114088,
131.106159195577)) ;
#151714=CARTESIAN_POINT('Ctrl Pts',(-23.8730939748177,13.489555102194,131.163174955555)) ;
#151715=CARTESIAN_POINT('Ctrl Pts',(-23.8560200827014,13.1989624545804,
131.146444379055)) ;
#151716=CARTESIAN_POINT('Ctrl Pts',(-23.8142948031392,12.9245155762064,
131.057679563774)) ;
#151717=CARTESIAN_POINT('Ctrl Pts',(-23.7497390288408,12.6850932088169,
130.90236186876)) ;
#151718=CARTESIAN_POINT('Ctrl Pts',(-23.6676401734867,12.5007200500438,
130.695387264516)) ;
#151719=CARTESIAN_POINT('Ctrl Pts',(-23.5710799792398,12.3802348015134,
130.446601105623)) ;
#151720=CARTESIAN_POINT('Ctrl Pts',(-23.4680387193144,12.3354177830535,
130.178616720221)) ;
#151721=CARTESIAN_POINT('Ctrl Pts',(-23.3639870057212,12.3682931650198,
129.907845197495)) ;
#151722=CARTESIAN_POINT('Ctrl Pts',(-23.2665557781875,12.4764500222757,
129.656260795804)) ;
#151723=CARTESIAN_POINT('Ctrl Pts',(-23.1812074615382,12.6527561756398,
129.440099421206)) ;
#151724=CARTESIAN_POINT('Ctrl Pts',(-23.1137789148354,12.8841372675975,
129.276247072773)) ;
#151725=CARTESIAN_POINT('Ctrl Pts',(-23.0682028417558,13.1550291136418,
129.176337392218)) ;
#151726=CARTESIAN_POINT('Ctrl Pts',(-23.0472767378411,13.4437302360126,
129.148261982065)) ;
#151727=CARTESIAN_POINT('Ctrl Pts',(-23.0515496084932,13.7319393007276,
129.193922359653)) ;
#151728=CARTESIAN_POINT('Ctrl Pts',(-23.079878251099,13.9965481623833,129.309665379139)) ;
#151729=CARTESIAN_POINT('Ctrl Pts',(-23.129741526764,14.2215298170475,129.488488454029)) ;
#151730=CARTESIAN_POINT('Ctrl Pts',(-23.1968818888558,14.3891483272759,
129.717799600751)) ;
#151731=CARTESIAN_POINT('Ctrl Pts',(-23.2754021964238,14.4871687024338,
129.980255089599)) ;
#151732=CARTESIAN_POINT('Ctrl Pts',(-23.3593328759968,14.5093408079897,
130.258577404978)) ;
#151733=CARTESIAN_POINT('Ctrl Pts',(-23.4420335332337,14.4530254583256,
130.533420307647)) ;
#151734=CARTESIAN_POINT('Ctrl Pts',(-23.5159486858221,14.3240305585518,
130.782295669503)) ;
#151735=CARTESIAN_POINT('Ctrl Pts',(-23.5763068870408,14.1290979717854,
130.991878121919)) ;
#151736=CARTESIAN_POINT('Ctrl Pts',(-23.617068843589,13.8855604155571,131.143910620301)) ;
#151737=CARTESIAN_POINT('Ctrl Pts',(-23.6352727286933,13.6058416707122,
131.230442968303)) ;
#151738=CARTESIAN_POINT('Ctrl Pts',(-23.6283964341607,13.3160021377259,
131.243341112372)) ;
#151739=CARTESIAN_POINT('Ctrl Pts',(-23.5965464340223,13.0326886676077,
131.183420690455)) ;
#151740=CARTESIAN_POINT('Ctrl Pts',(-23.5408985622457,12.7766372190837,
131.054072194123)) ;
#151741=CARTESIAN_POINT('Ctrl Pts',(-23.4649595861684,12.5676698161814,
130.865387166735)) ;
#151742=CARTESIAN_POINT('Ctrl Pts',(-23.3740967453034,12.4206517790888,
130.632884178497)) ;
#151743=CARTESIAN_POINT('Ctrl Pts',(-23.2727082372118,12.3443150505119,
130.369901024895)) ;
#151744=CARTESIAN_POINT('Ctrl Pts',(-23.1684546893583,12.3454567433165,
130.098404386445)) ;
#151745=CARTESIAN_POINT('Ctrl Pts',(-23.0671327036379,12.4241540146565,
129.835658717647)) ;
#151746=CARTESIAN_POINT('Ctrl Pts',(-22.9764947583752,12.5736454649868,
129.60388157098)) ;
#151747=CARTESIAN_POINT('Ctrl Pts',(-22.9011806814661,12.7844244258342,
129.417017819213)) ;
#151748=CARTESIAN_POINT('Ctrl Pts',(-22.8463459628872,13.041264478038,129.289992771218)) ;
#151749=CARTESIAN_POINT('Ctrl Pts',(-22.815230919969,13.3250313838274,129.232207692813)) ;
#151750=CARTESIAN_POINT('Ctrl Pts',(-22.8092125202162,13.6156492492809,
129.247717690027)) ;
#151751=CARTESIAN_POINT('Ctrl Pts',(-22.8280212526032,13.8929002803611,
129.335801002832)) ;
#151752=CARTESIAN_POINT('Ctrl Pts',(-22.8696833153775,14.1366366428793,
129.490673844657)) ;
#151753=CARTESIAN_POINT('Ctrl Pts',(-22.9303059421642,14.3287833833703,
129.70086742119)) ;
#151754=CARTESIAN_POINT('Ctrl Pts',(-23.0049559964505,14.4563288342089,
129.952070625789)) ;
#151755=CARTESIAN_POINT('Ctrl Pts',(-23.0876811988293,14.5097636463918,
130.226920951019)) ;
#151756=CARTESIAN_POINT('Ctrl Pts',(-23.171313625943,14.4852491819093,130.504285160366)) ;
#151757=CARTESIAN_POINT('Ctrl Pts',(-23.2495616828516,14.385213180382,130.765927789329)) ;
#151758=CARTESIAN_POINT('Ctrl Pts',(-23.3164467304666,14.2148994362801,
130.994611083723)) ;
#151759=CARTESIAN_POINT('Ctrl Pts',(-23.3654737459425,13.9895605141043,
131.170821580244)) ;
#151760=CARTESIAN_POINT('Ctrl Pts',(-23.3932709418014,13.7226496289756,
131.285186238845)) ;
#151761=CARTESIAN_POINT('Ctrl Pts',(-23.3966715321499,13.4342098859693,
131.328274909581)) ;
#151762=CARTESIAN_POINT('Ctrl Pts',(-23.3749521692447,13.1458182759752,
131.297881508113)) ;
#151763=CARTESIAN_POINT('Ctrl Pts',(-23.3285769346008,12.8759127132536,
131.195640591877)) ;
#151764=CARTESIAN_POINT('Ctrl Pts',(-23.2608087751802,12.6468868556867,
131.030665242811)) ;
#151765=CARTESIAN_POINT('Ctrl Pts',(-23.1749384545703,12.4721832296684,
130.81301511834)) ;
#151766=CARTESIAN_POINT('Ctrl Pts',(-23.0772501521557,12.3661739274481,
130.560671910315)) ;
#151767=CARTESIAN_POINT('Ctrl Pts',(-22.972758046801,12.3355863385396,130.288726503058)) ;
#151768=CARTESIAN_POINT('Ctrl Pts',(-22.8698300820149,12.3831198658751,
130.021082533712)) ;
#151769=CARTESIAN_POINT('Ctrl Pts',(-22.7739061268904,12.5053833023315,
129.774046335208)) ;
#151770=CARTESIAN_POINT('Ctrl Pts',(-22.6919791045737,12.6923270702948,
129.567704270438)) ;
#151771=CARTESIAN_POINT('Ctrl Pts',(-22.6281112723494,12.9335865705139,
129.414426275698)) ;
#151772=CARTESIAN_POINT('Ctrl Pts',(-22.5872544610613,13.2085814539572,
129.328158922446)) ;
#151773=CARTESIAN_POINT('Ctrl Pts',(-22.5710404902249,13.4990557588074,
129.313907984072)) ;
#151774=CARTESIAN_POINT('Ctrl Pts',(-22.5799753665134,13.7836907462661,
129.373072556554)) ;
#151775=CARTESIAN_POINT('Ctrl Pts',(-22.612638583778,14.0427281414566,129.501571243045)) ;
#151776=CARTESIAN_POINT('Ctrl Pts',(-22.6660762367978,14.2577309750281,
129.69079806233)) ;
#151777=CARTESIAN_POINT('Ctrl Pts',(-22.7357975374954,14.4131664617501,
129.927633756715)) ;
#151778=CARTESIAN_POINT('Ctrl Pts',(-22.8161137666784,14.4973755702956,
130.195456113862)) ;
#151779=CARTESIAN_POINT('Ctrl Pts',(-22.8998820017925,14.5046724130054,
130.47314586159)) ;
#151780=CARTESIAN_POINT('Ctrl Pts',(-22.9816064513032,14.4343111747756,
130.745147804022)) ;
#151781=CARTESIAN_POINT('Ctrl Pts',(-23.0536227051492,14.2913904033354,
130.98864811284)) ;
#151782=CARTESIAN_POINT('Ctrl Pts',(-23.1102843211941,14.0872940403586,
131.187176359758)) ;
#151783=CARTESIAN_POINT('Ctrl Pts',(-23.1472375329922,13.8349907742835,
131.328253449348)) ;
#151784=CARTESIAN_POINT('Ctrl Pts',(-23.1607772342592,13.5522018199285,
131.401036362566)) ;
#151785=CARTESIAN_POINT('Ctrl Pts',(-23.1491871925298,13.2611771320633,
131.400285897439)) ;
#151786=CARTESIAN_POINT('Ctrl Pts',(-23.1125952006362,12.9814107201437,
131.326544774095)) ;
#151787=CARTESIAN_POINT('Ctrl Pts',(-23.0531566614903,12.7341369610279,
131.185942865115)) ;
#151788=CARTESIAN_POINT('Ctrl Pts',(-22.9739547949964,12.535166216503,130.98774443351)) ;
#151789=CARTESIAN_POINT('Ctrl Pts',(-22.8800044204222,12.4000170891871,
130.746489022896)) ;
#151790=CARTESIAN_POINT('Ctrl Pts',(-22.7777942394703,12.3385941106561,
130.480992016477)) ;
#151791=CARTESIAN_POINT('Ctrl Pts',(-22.6737045237347,12.3545286685026,
130.209973410253)) ;
#151792=CARTESIAN_POINT('Ctrl Pts',(-22.574018025731,12.4469846430608,129.951917332464)) ;
#151793=CARTESIAN_POINT('Ctrl Pts',(-22.4853397321754,12.6102579412087,
129.726108518223)) ;
#151794=CARTESIAN_POINT('Ctrl Pts',(-22.4141387274598,12.8296977311719,
129.551032278381)) ;
#151795=CARTESIAN_POINT('Ctrl Pts',(-22.3635165048781,13.0929763552362,
129.436306120848)) ;
#151796=CARTESIAN_POINT('Ctrl Pts',(-22.3370222640428,13.3798715107165,
129.392040554444)) ;
#151797=CARTESIAN_POINT('Ctrl Pts',(-22.3358180956749,13.6705227535771,
129.421738962196)) ;
#151798=CARTESIAN_POINT('Ctrl Pts',(-22.359121262081,13.9421700423004,129.522864634634)) ;
#151799=CARTESIAN_POINT('Ctrl Pts',(-22.4048936915904,14.1780191011813,
129.689842088352)) ;
#151800=CARTESIAN_POINT('Ctrl Pts',(-22.4683015911897,14.3579768124892,
129.908015928199)) ;
#151801=CARTESIAN_POINT('Ctrl Pts',(-22.5452274463354,14.4725057553617,
130.165996866725)) ;
#151802=CARTESIAN_POINT('Ctrl Pts',(-22.6283868280108,14.5110248787396,
130.441981808158)) ;
#151803=CARTESIAN_POINT('Ctrl Pts',(-22.7115926468901,14.4721191969269,
130.718131866034)) ;
#151804=CARTESIAN_POINT('Ctrl Pts',(-22.7882774144574,14.3577454336847,
130.975310558445)) ;
#151805=CARTESIAN_POINT('Ctrl Pts',(-22.8518198048839,14.1770688666527,
131.193977525084)) ;
#151806=CARTESIAN_POINT('Ctrl Pts',(-22.8974027115045,13.9416997327419,
131.360307596844)) ;
#151807=CARTESIAN_POINT('Ctrl Pts',(-22.9206820190988,13.6694104353782,
131.461436266431)) ;
#151808=CARTESIAN_POINT('Ctrl Pts',(-22.9194213574652,13.3798585935035,
131.490838835533)) ;
#151809=CARTESIAN_POINT('Ctrl Pts',(-22.8929170330155,13.0927640382574,
131.446571141722)) ;
#151810=CARTESIAN_POINT('Ctrl Pts',(-22.8423030043868,12.8294542733058,
131.331865445954)) ;
#151811=CARTESIAN_POINT('Ctrl Pts',(-22.7706185679307,12.6090080043084,
131.155563913664)) ;
#151812=CARTESIAN_POINT('Ctrl Pts',(-22.6821571255679,12.4466659582347,
130.930272433196)) ;
#151813=CARTESIAN_POINT('Ctrl Pts',(-22.5824728331909,12.3544265354386,
130.672221564255)) ;
#151814=CARTESIAN_POINT('Ctrl Pts',(-22.478522759517,12.338485550426,130.401560070963)) ;
#151815=CARTESIAN_POINT('Ctrl Pts',(-22.3754966015088,12.4009576070215,
130.133958949611)) ;
#151816=CARTESIAN_POINT('Ctrl Pts',(-22.2823680889779,12.5356622675021,
129.894847033385)) ;
#151817=CARTESIAN_POINT('Ctrl Pts',(-22.2032360996956,12.7342792931547,
129.696815676907)) ;
#151818=CARTESIAN_POINT('Ctrl Pts',(-22.1436939987442,12.9822470405306,
129.555989965758)) ;
#151819=CARTESIAN_POINT('Ctrl Pts',(-22.1071406671597,13.2626104241267,
129.482419788097)) ;
#151820=CARTESIAN_POINT('Ctrl Pts',(-22.0957144593787,13.5537330357078,
129.482159506806)) ;
#151821=CARTESIAN_POINT('Ctrl Pts',(-22.1092685563454,13.8350780443648,
129.554823798795)) ;
#151822=CARTESIAN_POINT('Ctrl Pts',(-22.1461475103679,14.0872562376869,
129.695659561939)) ;
#151823=CARTESIAN_POINT('Ctrl Pts',(-22.2030821358645,14.2922552735091,
129.895131181954)) ;
#151824=CARTESIAN_POINT('Ctrl Pts',(-22.2754289643042,14.4349645919609,
130.139699349458)) ;
#151825=CARTESIAN_POINT('Ctrl Pts',(-22.3564708008619,14.5045540577175,
130.40942261917)) ;
#151826=CARTESIAN_POINT('Ctrl Pts',(-22.4406441329642,14.4973581396257,
130.688457173911)) ;
#151827=CARTESIAN_POINT('Ctrl Pts',(-22.5209414268602,14.4126016842873,
130.956235143864)) ;
#151828=CARTESIAN_POINT('Ctrl Pts',(-22.5903401138937,14.2578370889756,
131.191978979017)) ;
#151829=CARTESIAN_POINT('Ctrl Pts',(-22.643899231601,14.0423606370671,131.381638018117)) ;
#151830=CARTESIAN_POINT('Ctrl Pts',(-22.676541227732,13.7833430848993,131.510062783894)) ;
#151831=CARTESIAN_POINT('Ctrl Pts',(-22.6854014712124,13.4972454461382,
131.569174829683)) ;
#151832=CARTESIAN_POINT('Ctrl Pts',(-22.6691263169549,13.2077137971034,
131.554634071507)) ;
#151833=CARTESIAN_POINT('Ctrl Pts',(-22.6279874269016,12.9318531124,131.467669892297)) ;
#151834=CARTESIAN_POINT('Ctrl Pts',(-22.5644211603477,12.6922552108513,
131.31506619976)) ;
#151835=CARTESIAN_POINT('Ctrl Pts',(-22.4822337913331,12.504666487009,131.108074794862)) ;
#151836=CARTESIAN_POINT('Ctrl Pts',(-22.3859455591042,12.3825157199122,
130.860070359518)) ;
#151837=CARTESIAN_POINT('Ctrl Pts',(-22.283236535859,12.3357140444497,130.592990061673)) ;
#151838=CARTESIAN_POINT('Ctrl Pts',(-22.1793293005588,12.3660679541908,
130.322564167356)) ;
#151839=CARTESIAN_POINT('Ctrl Pts',(-22.0811143599576,12.4727573812884,
130.068868334442)) ;
#151840=CARTESIAN_POINT('Ctrl Pts',(-21.995572717209,12.6471452986828,129.852067795218)) ;
#151841=CARTESIAN_POINT('Ctrl Pts',(-21.9277324469771,12.8766362181276,
129.686942307119)) ;
#151842=CARTESIAN_POINT('Ctrl Pts',(-21.88149427899,13.1457609561308,129.584999326918)) ;
#151843=CARTESIAN_POINT('Ctrl Pts',(-21.8597035864534,13.436208516762,129.554631981768)) ;
#151844=CARTESIAN_POINT('Ctrl Pts',(-21.8632848179525,13.7232902020091,
129.598101610311)) ;
#151845=CARTESIAN_POINT('Ctrl Pts',(-21.8909607988816,13.9896012284326,
129.712029646671)) ;
#151846=CARTESIAN_POINT('Ctrl Pts',(-21.9403194385609,14.2159296230216,
129.889382772798)) ;
#151847=CARTESIAN_POINT('Ctrl Pts',(-22.0069084874016,14.3851342144556,
130.117025681466)) ;
#151848=CARTESIAN_POINT('Ctrl Pts',(-22.0853055168022,14.4854516976048,
130.379173666988)) ;
#151849=CARTESIAN_POINT('Ctrl Pts',(-22.1690106808166,14.5096986607512,
130.656773596937)) ;
#151850=CARTESIAN_POINT('Ctrl Pts',(-22.2516547688815,14.4561737731647,
130.931357792915)) ;
#151851=CARTESIAN_POINT('Ctrl Pts',(-22.3263675110369,14.3282785458503,
131.182786371531)) ;
#151852=CARTESIAN_POINT('Ctrl Pts',(-22.3868479785871,14.1363003864466,
131.392508931439)) ;
#151853=CARTESIAN_POINT('Ctrl Pts',(-22.4284860760948,13.8924839857025,
131.547317007501)) ;
#151854=CARTESIAN_POINT('Ctrl Pts',(-22.44725520974,13.6154602436594,131.6352536123)) ;
#151855=CARTESIAN_POINT('Ctrl Pts',(-22.4412045671012,13.3244466531158,
131.650714430567)) ;
#151856=CARTESIAN_POINT('Ctrl Pts',(-22.4100202102661,13.0407282159145,
131.592726094803)) ;
#151857=CARTESIAN_POINT('Ctrl Pts',(-22.3552546417009,12.7843965627726,
131.465846020052)) ;
#151858=CARTESIAN_POINT('Ctrl Pts',(-22.2799328403175,12.5734338880589,
131.27897230653)) ;
#151859=CARTESIAN_POINT('Ctrl Pts',(-22.1888584470267,12.4236459559127,
131.046058924602)) ;
#151860=CARTESIAN_POINT('Ctrl Pts',(-22.0881362776665,12.3455712635568,
130.784862015627)) ;
#151861=CARTESIAN_POINT('Ctrl Pts',(-21.9835492566618,12.3443023671055,
130.512500328341)) ;
#151862=CARTESIAN_POINT('Ctrl Pts',(-21.8821100407858,12.420933178294,130.249388866071)) ;
#151863=CARTESIAN_POINT('Ctrl Pts',(-21.7910702729597,12.5684896870098,
130.016446821888)) ;
#151864=CARTESIAN_POINT('Ctrl Pts',(-21.7150620477299,12.7783872300958,
129.827643163685)) ;
#151865=CARTESIAN_POINT('Ctrl Pts',(-21.6597355302853,13.0341435528073,
129.699158062916)) ;
#151866=CARTESIAN_POINT('Ctrl Pts',(-21.6280379920894,13.3161552682329,
129.639527649233)) ;
#151867=CARTESIAN_POINT('Ctrl Pts',(-21.6212166338096,13.6077102167408,
129.65278753406)) ;
#151868=CARTESIAN_POINT('Ctrl Pts',(-21.6394813968357,13.8863966863271,
129.739379830896)) ;
#151869=CARTESIAN_POINT('Ctrl Pts',(-21.6805482499846,14.1306963082603,
129.892451481926)) ;
#151870=CARTESIAN_POINT('Ctrl Pts',(-21.7404897132441,14.3238933046915,
130.100547666824)) ;
#151871=CARTESIAN_POINT('Ctrl Pts',(-21.8147710462659,14.4535137780173,
130.350663609957)) ;
#151872=CARTESIAN_POINT('Ctrl Pts',(-21.8973774190617,14.5094099168095,
130.625175022534)) ;
#151873=CARTESIAN_POINT('Ctrl Pts',(-21.9815416990517,14.4867701673882,
130.904282937535)) ;
#151874=CARTESIAN_POINT('Ctrl Pts',(-22.0595736035611,14.3890643828725,
131.165115307558)) ;
#151875=CARTESIAN_POINT('Ctrl Pts',(-22.1268562117523,14.2211869107964,
131.394908944864)) ;
#151876=CARTESIAN_POINT('Ctrl Pts',(-22.1766796342833,13.9958858020985,
131.573633433779)) ;
#151877=CARTESIAN_POINT('Ctrl Pts',(-22.2049451389284,13.7314793548645,
131.689162299244)) ;
#151878=CARTESIAN_POINT('Ctrl Pts',(-22.2091882562906,13.4423639400344,
131.734833540967)) ;
#151879=CARTESIAN_POINT('Ctrl Pts',(-22.187986226038,13.1530743203904,131.706032228928)) ;
#151880=CARTESIAN_POINT('Ctrl Pts',(-22.1426951060036,12.8842566111771,
131.60670589681)) ;
#151881=CARTESIAN_POINT('Ctrl Pts',(-22.0749780240027,12.6519995362001,
131.442148263088)) ;
#151882=CARTESIAN_POINT('Ctrl Pts',(-21.9900041425516,12.4766942436469,
131.226917109559)) ;
#151883=CARTESIAN_POINT('Ctrl Pts',(-21.8923871793902,12.3681120678918,
130.974864846892)) ;
#151884=CARTESIAN_POINT('Ctrl Pts',(-21.787890239755,12.3353450096833,130.70292564467)) ;
#151885=CARTESIAN_POINT('Ctrl Pts',(-21.6847703934588,12.3808789292608,
130.434751982444)) ;
#151886=CARTESIAN_POINT('Ctrl Pts',(-21.5888638247786,12.5006496739186,
130.187651595634)) ;
#151887=CARTESIAN_POINT('Ctrl Pts',(-21.5062882918341,12.6862348924807,
129.979488344586)) ;
#151888=CARTESIAN_POINT('Ctrl Pts',(-21.4420352783819,12.9253055289241,
129.824962379676)) ;
#151889=CARTESIAN_POINT('Ctrl Pts',(-21.4003702869002,13.1996774467986,
129.7363633676)) ;
#151890=CARTESIAN_POINT('Ctrl Pts',(-21.3833560025974,13.4900583198245,
129.719780265193)) ;
#151891=CARTESIAN_POINT('Ctrl Pts',(-21.3916055296796,13.7765694769724,
129.777104936438)) ;
#151892=CARTESIAN_POINT('Ctrl Pts',(-21.4238225675142,14.036835662277,129.904358363752)) ;
#151893=CARTESIAN_POINT('Ctrl Pts',(-21.4764867420294,14.2522894974628,
130.091167062838)) ;
#151894=CARTESIAN_POINT('Ctrl Pts',(-21.5461349346789,14.410142650821,130.327932770345)) ;
#151895=CARTESIAN_POINT('Ctrl Pts',(-21.6258533196047,14.4959011359271,
130.593837523055)) ;
#151896=CARTESIAN_POINT('Ctrl Pts',(-21.7097706486653,14.5055615596735,
130.872034708298)) ;
#151897=CARTESIAN_POINT('Ctrl Pts',(-21.7915115159255,14.4373879166647,
131.144023400965)) ;
#151898=CARTESIAN_POINT('Ctrl Pts',(-21.8638380594977,14.2968056087925,
131.388393161352)) ;
#151899=CARTESIAN_POINT('Ctrl Pts',(-21.9212551892473,14.0934340145334,
131.589268391717)) ;
#151900=CARTESIAN_POINT('Ctrl Pts',(-21.9586969314941,13.8423638114029,
131.731737544598)) ;
#151901=CARTESIAN_POINT('Ctrl Pts',(-21.9729463381941,13.5615577206812,
131.806433890657)) ;
#151902=CARTESIAN_POINT('Ctrl Pts',(-21.9620894874447,13.2694348944804,
131.807950532534)) ;
#151903=CARTESIAN_POINT('Ctrl Pts',(-21.9263140164209,12.9897647818979,
131.73650343455)) ;
#151904=CARTESIAN_POINT('Ctrl Pts',(-21.8673223314263,12.7403852471457,
131.597325259585)) ;
#151905=CARTESIAN_POINT('Ctrl Pts',(-21.7886865523693,12.5401778472151,
131.400734212814)) ;
#151906=CARTESIAN_POINT('Ctrl Pts',(-21.6953778525397,12.4032538731495,
131.161259541037)) ;
#151907=CARTESIAN_POINT('Ctrl Pts',(-21.5932072064287,12.3392654765734,
130.895922348931)) ;
#151908=CARTESIAN_POINT('Ctrl Pts',(-21.4887973419696,12.3529795705707,
130.624055509138)) ;
#151909=CARTESIAN_POINT('Ctrl Pts',(-21.3889895957889,12.44341496887,130.365620015526)) ;
#151910=CARTESIAN_POINT('Ctrl Pts',(-21.3002278613015,12.6038142404483,
130.13942068693)) ;
#151911=CARTESIAN_POINT('Ctrl Pts',(-21.2279512253468,12.8232746698558,
129.96143747852)) ;
#151912=CARTESIAN_POINT('Ctrl Pts',(-21.1769064226059,13.0848674095602,
129.845368695489)) ;
#151913=CARTESIAN_POINT('Ctrl Pts',(-21.149658170467,13.3712340427374,129.798893618011)) ;
#151914=CARTESIAN_POINT('Ctrl Pts',(-21.1476946959762,13.6620670155129,
129.826365855313)) ;
#151915=CARTESIAN_POINT('Ctrl Pts',(-21.1703666330339,13.9347879219274,
129.92569032549)) ;
#151916=CARTESIAN_POINT('Ctrl Pts',(-21.2152993770454,14.1711547034761,
130.090075797328)) ;
#151917=CARTESIAN_POINT('Ctrl Pts',(-21.2785796529392,14.3538985958079,
130.308060225528)) ;
#151918=CARTESIAN_POINT('Ctrl Pts',(-21.3548663994536,14.4699515410886,
130.564015298951)) ;
#151919=CARTESIAN_POINT('Ctrl Pts',(-21.4380889896721,14.511011729743,130.840261217569)) ;
#151920=CARTESIAN_POINT('Ctrl Pts',(-21.5213196238039,14.4745400421894,
131.116445883889)) ;
#151921=CARTESIAN_POINT('Ctrl Pts',(-21.5987228795245,14.3614974996119,
131.37591886424)) ;
#151922=CARTESIAN_POINT('Ctrl Pts',(-21.6624280158677,14.1829580277845,
131.594943503888)) ;
#151923=CARTESIAN_POINT('Ctrl Pts',(-21.7085901232024,13.9492404929465,
131.762934960253)) ;
#151924=CARTESIAN_POINT('Ctrl Pts',(-21.7325457579653,13.6775800982586,
131.866060493852)) ;
#151925=CARTESIAN_POINT('Ctrl Pts',(-21.7320824211323,13.3886494635436,
131.897743516193)) ;
#151926=CARTESIAN_POINT('Ctrl Pts',(-21.7060357693068,13.0993478015478,
131.855033735375)) ;
#151927=CARTESIAN_POINT('Ctrl Pts',(-21.6563720516456,12.8369458310676,
131.74287352401)) ;
#151928=CARTESIAN_POINT('Ctrl Pts',(-21.5849505607058,12.6140529768099,
131.567486815159)) ;
#151929=CARTESIAN_POINT('Ctrl Pts',(-21.4972346922135,12.4507323341902,
131.344230579028)) ;
#151930=CARTESIAN_POINT('Ctrl Pts',(-21.3977816403119,12.3558899306528,
131.086868664739)) ;
#151931=CARTESIAN_POINT('Ctrl Pts',(-21.2931236526698,12.3380969081111,
130.814378116707)) ;
#151932=CARTESIAN_POINT('Ctrl Pts',(-21.1912351475806,12.3976016694818,
130.549680132567)) ;
#151933=CARTESIAN_POINT('Ctrl Pts',(-21.0970918464179,12.530583824708,130.307814407326)) ;
#151934=CARTESIAN_POINT('Ctrl Pts',(-21.0173249384038,12.7283490506027,
130.108013541003)) ;
#151935=CARTESIAN_POINT('Ctrl Pts',(-20.9573893511929,12.9742771227128,
129.965922835233)) ;
#151936=CARTESIAN_POINT('Ctrl Pts',(-20.9200880297606,13.2539376227601,
129.890167219948)) ;
#151937=CARTESIAN_POINT('Ctrl Pts',(-20.907889243952,13.5450903335013,129.887655062896)) ;
#151938=CARTESIAN_POINT('Ctrl Pts',(-20.920784302057,13.8275787514848,129.958467916581)) ;
#151939=CARTESIAN_POINT('Ctrl Pts',(-20.9569782930972,14.080619519853,130.097260030665)) ;
#151940=CARTESIAN_POINT('Ctrl Pts',(-21.0136849887986,14.2877392133105,
130.296196899106)) ;
#151941=CARTESIAN_POINT('Ctrl Pts',(-21.0849841102122,14.431213841156,130.537392435781)) ;
#151942=CARTESIAN_POINT('Ctrl Pts',(-21.1665056814218,14.5038738166411,
130.808799012005)) ;
#151943=CARTESIAN_POINT('Ctrl Pts',(-21.2505166479721,14.4984557576167,
131.087288159437)) ;
#151944=CARTESIAN_POINT('Ctrl Pts',(-21.3308085825838,14.4164646825051,
131.354946228948)) ;
#151945=CARTESIAN_POINT('Ctrl Pts',(-21.4010755566249,14.2622140461571,
131.593482336718)) ;
#151946=CARTESIAN_POINT('Ctrl Pts',(-21.4547420541191,14.0497489487789,
131.7832014722)) ;
#151947=CARTESIAN_POINT('Ctrl Pts',(-21.4881853748102,13.7905258352839,
131.91413728601)) ;
#151948=CARTESIAN_POINT('Ctrl Pts',(-21.4977462696728,13.506486494377,131.975100243164)) ;
#151949=CARTESIAN_POINT('Ctrl Pts',(-21.4819835887124,13.2142515667239,
131.96236180773)) ;
#151950=CARTESIAN_POINT('Ctrl Pts',(-21.4419223606185,12.9406232851689,
131.878185903014)) ;
#151951=CARTESIAN_POINT('Ctrl Pts',(-21.3786934156362,12.6982138740687,
131.726763051586)) ;
#151952=CARTESIAN_POINT('Ctrl Pts',(-21.2972126241658,12.5096112048297,
131.521723412285)) ;
#151953=CARTESIAN_POINT('Ctrl Pts',(-21.2011850848722,12.3850648620669,
131.274514023005)) ;
#151954=CARTESIAN_POINT('Ctrl Pts',(-21.0984907761846,12.3359713268051,
131.007507556083)) ;
#151955=CARTESIAN_POINT('Ctrl Pts',(-20.9944877940312,12.3641515700291,
130.736812488399)) ;
#151956=CARTESIAN_POINT('Ctrl Pts',(-20.8961804382662,12.4683944776065,
130.482779938443)) ;
#151957=CARTESIAN_POINT('Ctrl Pts',(-20.8099546373725,12.6414744910879,
130.264081389746)) ;
#151958=CARTESIAN_POINT('Ctrl Pts',(-20.7415876002801,12.8692739707259,
130.097372977444)) ;
#151959=CARTESIAN_POINT('Ctrl Pts',(-20.6945289877427,13.1394382839076,
129.993253900407)) ;
#151960=CARTESIAN_POINT('Ctrl Pts',(-20.672298328365,13.4257125423889,129.961149556797)) ;
#151961=CARTESIAN_POINT('Ctrl Pts',(-20.6750007501078,13.7153678926771,
130.002310555712)) ;
#151962=CARTESIAN_POINT('Ctrl Pts',(-20.7020667565521,13.9823826092166,
130.114434508231)) ;
#151963=CARTESIAN_POINT('Ctrl Pts',(-20.7509060316579,14.210351268189,130.290309073817)) ;
#151964=CARTESIAN_POINT('Ctrl Pts',(-20.8169604036749,14.3810373513132,
130.516327937223)) ;
#151965=CARTESIAN_POINT('Ctrl Pts',(-20.8950665489886,14.4835203874639,
130.777619160747)) ;
#151966=CARTESIAN_POINT('Ctrl Pts',(-20.9787343216663,14.5102051470099,
131.055116750985)) ;
#151967=CARTESIAN_POINT('Ctrl Pts',(-21.0618484768981,14.4584272467564,
131.331220006128)) ;
#151968=CARTESIAN_POINT('Ctrl Pts',(-21.1364526301434,14.3332271538461,
131.582140708526)) ;
#151969=CARTESIAN_POINT('Ctrl Pts',(-21.1976622623504,14.1422679027751,
131.794126036847)) ;
#151970=CARTESIAN_POINT('Ctrl Pts',(-21.23975721544,13.9003526545792,131.950166196499)) ;
#151971=CARTESIAN_POINT('Ctrl Pts',(-21.2592791168289,13.6237176044633,
132.040346931511)) ;
#151972=CARTESIAN_POINT('Ctrl Pts',(-21.2539545891703,13.3329588361478,
132.057910063551)) ;
#151973=CARTESIAN_POINT('Ctrl Pts',(-21.2234510913761,13.0482791472687,
132.00196258976)) ;
#151974=CARTESIAN_POINT('Ctrl Pts',(-21.1691539099102,12.7905984211716,
131.876506766355)) ;
#151975=CARTESIAN_POINT('Ctrl Pts',(-21.0947340593749,12.5792074314873,
131.692098693563)) ;
#151976=CARTESIAN_POINT('Ctrl Pts',(-21.0040480835755,12.4271420328258,
131.460337471105)) ;
#151977=CARTESIAN_POINT('Ctrl Pts',(-20.9032486407606,12.3466854620337,
131.199002527252)) ;
#151978=CARTESIAN_POINT('Ctrl Pts',(-20.7987770579087,12.3433384451733,
130.926945640301)) ;
#151979=CARTESIAN_POINT('Ctrl Pts',(-20.6974847568586,12.417256873973,130.664144724903)) ;
#151980=CARTESIAN_POINT('Ctrl Pts',(-20.6057021506296,12.5633304568432,
130.429162568903)) ;
#151981=CARTESIAN_POINT('Ctrl Pts',(-20.5294560018403,12.7708593905581,
130.239538039818)) ;
#151982=CARTESIAN_POINT('Ctrl Pts',(-20.4733463103174,13.025326349885,130.108769986711)) ;
#151983=CARTESIAN_POINT('Ctrl Pts',(-20.4407772110818,13.3082178025067,
130.046756066484)) ;
#151984=CARTESIAN_POINT('Ctrl Pts',(-20.4333100328866,13.5990344955289,
130.058039052296)) ;
#151985=CARTESIAN_POINT('Ctrl Pts',(-20.4506880067864,13.8774216043795,
130.141913702905)) ;
#151986=CARTESIAN_POINT('Ctrl Pts',(-20.4911818153333,14.1239848990119,
130.293425636597)) ;
#151987=CARTESIAN_POINT('Ctrl Pts',(-20.5507855806424,14.3192776170792,
130.500609692184)) ;
#151988=CARTESIAN_POINT('Ctrl Pts',(-20.6247405377758,14.4507732360595,
130.749766053951)) ;
#151989=CARTESIAN_POINT('Ctrl Pts',(-20.7069579624013,14.5087792678555,
131.023045402965)) ;
#151990=CARTESIAN_POINT('Ctrl Pts',(-20.7911628034135,14.4887238336712,
131.302264434157)) ;
#151991=CARTESIAN_POINT('Ctrl Pts',(-20.8697693366433,14.3928285084541,
131.564906273796)) ;
#151992=CARTESIAN_POINT('Ctrl Pts',(-20.9374577677181,14.2263682040696,
131.795916170133)) ;
#151993=CARTESIAN_POINT('Ctrl Pts',(-20.9876137387477,14.0038696460673,
131.975425509327)) ;
#151994=CARTESIAN_POINT('Ctrl Pts',(-21.0167121922335,13.7389372008462,
132.093575454873)) ;
#151995=CARTESIAN_POINT('Ctrl Pts',(-21.021624803058,13.4518073715824,132.141010517718)) ;
#151996=CARTESIAN_POINT('Ctrl Pts',(-21.001265184062,13.1616327439453,132.114737089628)) ;
#151997=CARTESIAN_POINT('Ctrl Pts',(-20.9563235153239,12.8906304372966,
132.016607385205)) ;
#151998=CARTESIAN_POINT('Ctrl Pts',(-20.8895478488704,12.6585325321797,
131.854601473478)) ;
#151999=CARTESIAN_POINT('Ctrl Pts',(-20.8050290649649,12.4808578746759,
131.640730446969)) ;
#152000=CARTESIAN_POINT('Ctrl Pts',(-20.706854482996,12.369794968941,131.387313297938)) ;
#152001=CARTESIAN_POINT('Ctrl Pts',(-20.6035841518815,12.3353140243209,
131.118587941619)) ;
#152002=CARTESIAN_POINT('Ctrl Pts',(-20.4999425243112,12.3783402005982,
130.849020652898)) ;
#152003=CARTESIAN_POINT('Ctrl Pts',(-20.4037610912831,12.4961137906607,
130.601107675479)) ;
#152004=CARTESIAN_POINT('Ctrl Pts',(-20.3206161817449,12.6800956082709,
130.391318319672)) ;
#152005=CARTESIAN_POINT('Ctrl Pts',(-20.2557578107062,12.9180877152906,
130.235043956869)) ;
#152006=CARTESIAN_POINT('Ctrl Pts',(-20.2134909793572,13.1911275173993,
130.144619104063)) ;
#152007=CARTESIAN_POINT('Ctrl Pts',(-20.1956945315034,13.4815072415882,
130.125770538085)) ;
#152008=CARTESIAN_POINT('Ctrl Pts',(-20.2032544219231,13.7684314308885,
130.181084199128)) ;
#152009=CARTESIAN_POINT('Ctrl Pts',(-20.2346242895992,14.029076308477,130.305758033525)) ;
#152010=CARTESIAN_POINT('Ctrl Pts',(-20.2871102678795,14.2473093926041,
130.492262967075)) ;
#152011=CARTESIAN_POINT('Ctrl Pts',(-20.3557014691764,14.4057091519906,
130.725627737145)) ;
#152012=CARTESIAN_POINT('Ctrl Pts',(-20.4356832288713,14.4946178708306,
130.992528144001)) ;
#152013=CARTESIAN_POINT('Ctrl Pts',(-20.5195606513706,14.5063975208026,
131.270592829057)) ;
#152014=CARTESIAN_POINT('Ctrl Pts',(-20.601669735203,14.4401278585609,131.543748083559)) ;
#152015=CARTESIAN_POINT('Ctrl Pts',(-20.6740334559909,14.3020001323071,
131.788087967881)) ;
#152016=CARTESIAN_POINT('Ctrl Pts',(-20.7320052756849,14.100380875427,131.990589852135)) ;
#152017=CARTESIAN_POINT('Ctrl Pts',(-20.7701334334659,13.8504602239821,
132.135070902885)) ;
#152018=CARTESIAN_POINT('Ctrl Pts',(-20.7851220054825,13.5690360496352,
132.212066464694)) ;
#152019=CARTESIAN_POINT('Ctrl Pts',(-20.7749067351906,13.277347744237,132.215406858043)) ;
#152020=CARTESIAN_POINT('Ctrl Pts',(-20.739950771466,12.9978265767653,132.146263744771)) ;
#152021=CARTESIAN_POINT('Ctrl Pts',(-20.6815482067024,12.747023860199,132.008839074771)) ;
#152022=CARTESIAN_POINT('Ctrl Pts',(-20.6035221230103,12.5453431667421,
131.813989900865)) ;
#152023=CARTESIAN_POINT('Ctrl Pts',(-20.5104128505178,12.4062333259034,
131.575152883014)) ;
#152024=CARTESIAN_POINT('Ctrl Pts',(-20.4087091658857,12.3400677949455,
131.311081123435)) ;
#152025=CARTESIAN_POINT('Ctrl Pts',(-20.303791085454,12.3515722965719,131.037884994155)) ;
#152026=CARTESIAN_POINT('Ctrl Pts',(-20.2041191745575,12.4396025465946,
130.779723997866)) ;
#152027=CARTESIAN_POINT('Ctrl Pts',(-20.1147712529316,12.5983879462257,
130.551883797315)) ;
#152028=CARTESIAN_POINT('Ctrl Pts',(-20.0421585923302,12.8155081778463,
130.372801469089)) ;
#152029=CARTESIAN_POINT('Ctrl Pts',(-19.9900861703505,13.0777480891852,
130.253944896754)) ;
#152030=CARTESIAN_POINT('Ctrl Pts',(-19.9622906553043,13.3640007134148,
130.205892912972)) ;
#152031=CARTESIAN_POINT('Ctrl Pts',(-19.9596040305283,13.6530970190172,
130.231033720601)) ;
#152032=CARTESIAN_POINT('Ctrl Pts',(-19.9815947583038,13.9274410550996,
130.328465672942)) ;
#152033=CARTESIAN_POINT('Ctrl Pts',(-20.0259169621657,14.1649405448642,
130.491043143204)) ;
#152034=CARTESIAN_POINT('Ctrl Pts',(-20.0889049637749,14.3499176915205,
130.708260928926)) ;
#152035=CARTESIAN_POINT('Ctrl Pts',(-20.1649263048442,14.4676736740884,
130.963435819328)) ;
#152036=CARTESIAN_POINT('Ctrl Pts',(-20.247688472556,14.5109849198275,131.238193829716)) ;
#152037=CARTESIAN_POINT('Ctrl Pts',(-20.331483197017,14.4763368011369,131.516227084564)) ;
#152038=CARTESIAN_POINT('Ctrl Pts',(-20.4085145537121,14.3664425274482,
131.774319022009)) ;
#152039=CARTESIAN_POINT('Ctrl Pts',(-20.4732700628347,14.1882602546085,
131.996710354005)) ;
#152040=CARTESIAN_POINT('Ctrl Pts',(-20.5197600667737,13.9563928712726,
132.165546655575)) ;
#152041=CARTESIAN_POINT('Ctrl Pts',(-20.544429934519,13.6856075071528,132.270760904427)) ;
#152042=CARTESIAN_POINT('Ctrl Pts',(-20.5446218153691,13.3967978155194,
132.304370094684)) ;
#152043=CARTESIAN_POINT('Ctrl Pts',(-20.5194831662747,13.1083772147109,
132.264162983921)) ;
#152044=CARTESIAN_POINT('Ctrl Pts',(-20.4702619913672,12.8436201216384,
132.15346806604)) ;
#152045=CARTESIAN_POINT('Ctrl Pts',(-20.3994698940617,12.6197329650473,
131.979865314557)) ;
#152046=CARTESIAN_POINT('Ctrl Pts',(-20.3120006020497,12.4541610182818,
131.75739537006)) ;
#152047=CARTESIAN_POINT('Ctrl Pts',(-20.2125860830344,12.3575181073951,
131.500199627294)) ;
#152048=CARTESIAN_POINT('Ctrl Pts',(-20.1088815096965,12.337407534574,131.230203979974)) ;
#152049=CARTESIAN_POINT('Ctrl Pts',(-20.0060146641454,12.3950240477661,
130.962919259217)) ;
#152050=CARTESIAN_POINT('Ctrl Pts',(-19.9119864658295,12.5255974682326,
130.721236187127)) ;
#152051=CARTESIAN_POINT('Ctrl Pts',(-19.8314897395286,12.7221236513144,
130.519397456966)) ;
#152052=CARTESIAN_POINT('Ctrl Pts',(-19.7710089279874,12.966643820031,130.375676004731)) ;
#152053=CARTESIAN_POINT('Ctrl Pts',(-19.732928013481,13.2467842966359,130.297774420096)) ;
#152054=CARTESIAN_POINT('Ctrl Pts',(-19.7201400299444,13.5364084867458,
130.293371523372)) ;
#152055=CARTESIAN_POINT('Ctrl Pts',(-19.7322324408918,13.819301352246,130.361818332685)) ;
#152056=CARTESIAN_POINT('Ctrl Pts',(-19.7678249009645,14.0737430594077,
130.498891515294)) ;
#152057=CARTESIAN_POINT('Ctrl Pts',(-19.8239107737393,14.2823383256047,
130.695974069195)) ;
#152058=CARTESIAN_POINT('Ctrl Pts',(-19.8950604586474,14.4280819786068,
130.936830915041)) ;
#152059=CARTESIAN_POINT('Ctrl Pts',(-19.9759986631136,14.5027907188546,
131.20637093887)) ;
#152060=CARTESIAN_POINT('Ctrl Pts',(-20.0606762821136,14.4996009182714,
131.487070199978)) ;
#152061=CARTESIAN_POINT('Ctrl Pts',(-20.1407098011001,14.4198435135005,
131.753794032065)) ;
#152062=CARTESIAN_POINT('Ctrl Pts',(-20.2112630859601,14.2682255575811,
131.993092362855)) ;
#152063=CARTESIAN_POINT('Ctrl Pts',(-20.2656775957736,14.0566692320112,
132.185107721384)) ;
#152064=CARTESIAN_POINT('Ctrl Pts',(-20.2997748055791,13.7984046917339,
132.317960439349)) ;
#152065=CARTESIAN_POINT('Ctrl Pts',(-20.3099989318143,13.5146255183712,
132.38088711118)) ;
#152066=CARTESIAN_POINT('Ctrl Pts',(-20.2951296394703,13.22379017507,132.370580468596)) ;
#152067=CARTESIAN_POINT('Ctrl Pts',(-20.2555701663945,12.9476430099182,
132.288081447981)) ;
#152068=CARTESIAN_POINT('Ctrl Pts',(-20.1928769291611,12.7041858709694,
132.138213583783)) ;
#152069=CARTESIAN_POINT('Ctrl Pts',(-20.1120002752265,12.5142908380612,
131.934883468866)) ;
#152070=CARTESIAN_POINT('Ctrl Pts',(-20.0165096996154,12.3877724329813,
131.689173717466)) ;
#152071=CARTESIAN_POINT('Ctrl Pts',(-19.913478604829,12.3361912043238,131.421332336646)) ;
#152072=CARTESIAN_POINT('Ctrl Pts',(-19.8094708653727,12.3624798224069,
131.150606824843)) ;
#152073=CARTESIAN_POINT('Ctrl Pts',(-19.7113062006748,12.4640688022784,
130.896852899496)) ;
#152074=CARTESIAN_POINT('Ctrl Pts',(-19.6243191332476,12.6358046245907,
130.676044087363)) ;
#152075=CARTESIAN_POINT('Ctrl Pts',(-19.5555745074161,12.862048858162,130.508185639822)) ;
#152076=CARTESIAN_POINT('Ctrl Pts',(-19.5079382213539,13.1294243703739,
130.402168639634)) ;
#152077=CARTESIAN_POINT('Ctrl Pts',(-19.4847311841948,13.419127554444,130.367646107838)) ;
#152078=CARTESIAN_POINT('Ctrl Pts',(-19.486760537507,13.7060585256719,130.406486755971)) ;
#152079=CARTESIAN_POINT('Ctrl Pts',(-19.5132448910941,13.9758635071568,
130.517143788552)) ;
#152080=CARTESIAN_POINT('Ctrl Pts',(-19.561461527867,14.2044690811379,130.691105042514)) ;
#152081=CARTESIAN_POINT('Ctrl Pts',(-19.6271525262166,14.3772046466544,
130.916107336043)) ;
#152082=CARTESIAN_POINT('Ctrl Pts',(-19.7049913038784,14.4817041640368,
131.17660395042)) ;
#152083=CARTESIAN_POINT('Ctrl Pts',(-19.7886768197028,14.5103977605507,
131.454191387136)) ;
#152084=CARTESIAN_POINT('Ctrl Pts',(-19.8713625246764,14.461387716176,131.728812616932)) ;
#152085=CARTESIAN_POINT('Ctrl Pts',(-19.9466960883751,14.3378670523305,
131.982034797292)) ;
#152086=CARTESIAN_POINT('Ctrl Pts',(-20.0083045176645,14.1487649480966,
132.195144873615)) ;
#152087=CARTESIAN_POINT('Ctrl Pts',(-20.0510942154457,13.9077124472436,
132.35327591803)) ;
#152088=CARTESIAN_POINT('Ctrl Pts',(-20.0712746305926,13.6318349091011,
132.445369268278)) ;
#152089=CARTESIAN_POINT('Ctrl Pts',(-20.0666628175852,13.3411961915081,
132.465016541542)) ;
#152090=CARTESIAN_POINT('Ctrl Pts',(-20.0369065317575,13.0563347009616,
132.411215549619)) ;
#152091=CARTESIAN_POINT('Ctrl Pts',(-19.9832697572704,12.7976622253545,
132.287685663652)) ;
#152092=CARTESIAN_POINT('Ctrl Pts',(-19.909474160919,12.584625305209,132.105083184337)) ;
#152093=CARTESIAN_POINT('Ctrl Pts',(-19.8184221729735,12.429833286881,131.872506784025)) ;
#152094=CARTESIAN_POINT('Ctrl Pts',(-19.7187303437125,12.3481748757021,
131.614098966012)) ;
#152095=CARTESIAN_POINT('Ctrl Pts',(-19.6138632113487,12.3422836205948,
131.341022208364)) ;
#152096=CARTESIAN_POINT('Ctrl Pts',(-19.5124594677726,12.414162317258,131.077872115915)) ;
#152097=CARTESIAN_POINT('Ctrl Pts',(-19.420212188348,12.55849168118,130.841573794732)) ;
#152098=CARTESIAN_POINT('Ctrl Pts',(-19.3435324232807,12.7644624942609,
130.65066449742)) ;
#152099=CARTESIAN_POINT('Ctrl Pts',(-19.2868798087134,13.0174115077838,
130.518256914751)) ;
#152100=CARTESIAN_POINT('Ctrl Pts',(-19.2535766304538,13.2998964348547,
130.454116409847)) ;
#152101=CARTESIAN_POINT('Ctrl Pts',(-19.2453729976278,13.5908799629275,
130.463258994527)) ;
#152102=CARTESIAN_POINT('Ctrl Pts',(-19.2621513468008,13.8706960081611,
130.545479006086)) ;
#152103=CARTESIAN_POINT('Ctrl Pts',(-19.3020872042403,14.1180202656557,
130.695329004107)) ;
#152104=CARTESIAN_POINT('Ctrl Pts',(-19.3610103361281,14.3143765894564,
130.900421785235)) ;
#152105=CARTESIAN_POINT('Ctrl Pts',(-19.434812974818,14.4481660809184,131.149213001408)) ;
#152106=CARTESIAN_POINT('Ctrl Pts',(-19.5166794707772,14.5080838606745,
131.421381896559)) ;
#152107=CARTESIAN_POINT('Ctrl Pts',(-19.6008596180551,14.4905518531177,
131.700498217892)) ;
#152108=CARTESIAN_POINT('Ctrl Pts',(-19.679959110775,14.3964092296967,131.964690313878)) ;
#152109=CARTESIAN_POINT('Ctrl Pts',(-19.7478273039877,14.232304987228,132.196115316038)) ;
#152110=CARTESIAN_POINT('Ctrl Pts',(-19.7986192880396,14.0113006854444,
132.37749892765)) ;
#152111=CARTESIAN_POINT('Ctrl Pts',(-19.8284139029138,13.7469853282518,
132.497724021509)) ;
#152112=CARTESIAN_POINT('Ctrl Pts',(-19.8340820683678,13.4601451324146,
132.547372256783)) ;
#152113=CARTESIAN_POINT('Ctrl Pts',(-19.8142531422841,13.1687003200991,
132.522778212001)) ;
#152114=CARTESIAN_POINT('Ctrl Pts',(-19.7703730343976,12.8989650919222,
132.427483609972)) ;
#152115=CARTESIAN_POINT('Ctrl Pts',(-19.7036589079187,12.6635916504989,
132.265932090456)) ;
#152116=CARTESIAN_POINT('Ctrl Pts',(-19.6199118535932,12.485239800862,132.054155238019)) ;
#152117=CARTESIAN_POINT('Ctrl Pts',(-19.5219805853211,12.3719259500599,
131.801473410491)) ;
#152118=CARTESIAN_POINT('Ctrl Pts',(-19.4189379680128,12.3351771032852,
131.53336398971)) ;
#152119=CARTESIAN_POINT('Ctrl Pts',(-19.3148770024859,12.3762351050997,
131.26268009039)) ;
#152120=CARTESIAN_POINT('Ctrl Pts',(-19.2189066435572,12.4911992435135,
131.01519951472)) ;
#152121=CARTESIAN_POINT('Ctrl Pts',(-19.1347439547889,12.6745749260732,
130.802658266804)) ;
#152122=CARTESIAN_POINT('Ctrl Pts',(-19.0695712650756,12.9105841176317,
130.64534787781)) ;
#152123=CARTESIAN_POINT('Ctrl Pts',(-19.026516615279,13.1834575472762,130.552699546602)) ;
#152124=CARTESIAN_POINT('Ctrl Pts',(-19.0081217007437,13.4728172007292,
130.532007746554)) ;
#152125=CARTESIAN_POINT('Ctrl Pts',(-19.0147866964172,13.7593252111675,
130.584597145698)) ;
#152126=CARTESIAN_POINT('Ctrl Pts',(-19.0457740324292,14.0229111380707,
130.708413150787)) ;
#152127=CARTESIAN_POINT('Ctrl Pts',(-19.0973111190571,14.2409568530166,
130.891883602161)) ;
#152128=CARTESIAN_POINT('Ctrl Pts',(-19.165926552844,14.4024702596202,131.125549278518)) ;
#152129=CARTESIAN_POINT('Ctrl Pts',(-19.2454507888212,14.4930252918819,
131.390998297428)) ;
#152130=CARTESIAN_POINT('Ctrl Pts',(-19.3293410740711,14.5071138077779,
131.669126207063)) ;
#152131=CARTESIAN_POINT('Ctrl Pts',(-19.4112821511384,14.4434722304718,
131.941650206842)) ;
#152132=CARTESIAN_POINT('Ctrl Pts',(-19.4842739640058,14.3072991508372,
132.187922760495)) ;
#152133=CARTESIAN_POINT('Ctrl Pts',(-19.5429829781195,14.1061281755834,
132.392741540416)) ;
#152134=CARTESIAN_POINT('Ctrl Pts',(-19.5814898983426,13.8584458365122,
132.538171297678)) ;
#152135=CARTESIAN_POINT('Ctrl Pts',(-19.5972452937213,13.5782527615593,
132.617345758941)) ;
#152136=CARTESIAN_POINT('Ctrl Pts',(-19.587821553024,13.2862405830432,132.623036030091)) ;
#152137=CARTESIAN_POINT('Ctrl Pts',(-19.5535345414538,13.0054673407222,
132.55591759128)) ;
#152138=CARTESIAN_POINT('Ctrl Pts',(-19.4954706738399,12.7527978446706,
132.419600001604)) ;
#152139=CARTESIAN_POINT('Ctrl Pts',(-19.4183727349997,12.5507722085017,
132.227270319449)) ;
#152140=CARTESIAN_POINT('Ctrl Pts',(-19.3255707730553,12.4092693590586,
131.989364894937)) ;
#152141=CARTESIAN_POINT('Ctrl Pts',(-19.2238321783356,12.3409406073707,
131.725254513543)) ;
#152142=CARTESIAN_POINT('Ctrl Pts',(-19.119236753858,12.3499819194409,131.452886617979)) ;
#152143=CARTESIAN_POINT('Ctrl Pts',(-19.0188367516298,12.4363532158425,
131.192772449436)) ;
#152144=CARTESIAN_POINT('Ctrl Pts',(-18.9295447538629,12.5925663631045,
130.964931579883)) ;
#152145=CARTESIAN_POINT('Ctrl Pts',(-18.85618070133,12.8085170384963,130.783729205798)) ;
#152146=CARTESIAN_POINT('Ctrl Pts',(-18.8035406576781,13.0694866152918,
130.663175810496)) ;
#152147=CARTESIAN_POINT('Ctrl Pts',(-18.774944483164,13.3550371201656,130.612758020313)) ;
#152148=CARTESIAN_POINT('Ctrl Pts',(-18.7715872372659,13.6462143005165,
130.636161963138)) ;
#152149=CARTESIAN_POINT('Ctrl Pts',(-18.7928313609646,13.9195287631536,
130.73120381732)) ;
#152150=CARTESIAN_POINT('Ctrl Pts',(-18.8365269344384,14.1586150899391,
130.891977988719)) ;
#152151=CARTESIAN_POINT('Ctrl Pts',(-18.8989146423201,14.3449689837057,
131.10737481057)) ;
#152152=CARTESIAN_POINT('Ctrl Pts',(-18.9745793166611,14.465239738532,131.36150472704)) ;
#152153=CARTESIAN_POINT('Ctrl Pts',(-19.0578793507872,14.5107689866746,
131.638093119859)) ;
#152154=CARTESIAN_POINT('Ctrl Pts',(-19.1409583613005,14.4787461978325,
131.913707901465)) ;
#152155=CARTESIAN_POINT('Ctrl Pts',(-19.2189706552468,14.3700644324197,
132.17497387013)) ;
#152156=CARTESIAN_POINT('Ctrl Pts',(-19.2836848317943,14.1946408166751,
132.397013538057)) ;
#152157=CARTESIAN_POINT('Ctrl Pts',(-19.3309065027156,13.963907732595,132.568053904224)) ;
#152158=CARTESIAN_POINT('Ctrl Pts',(-19.3562835215805,13.6940409321305,
132.675319682935)) ;
#152159=CARTESIAN_POINT('Ctrl Pts',(-19.3571223286895,13.4043243937501,
132.710955989412)) ;
#152160=CARTESIAN_POINT('Ctrl Pts',(-19.3329129352278,13.1175424358185,
132.673226068229)) ;
#152161=CARTESIAN_POINT('Ctrl Pts',(-19.284075134649,12.8501254079525,132.563869228407)) ;
#152162=CARTESIAN_POINT('Ctrl Pts',(-19.2141838640519,12.6260375389968,
132.392718948333)) ;
#152163=CARTESIAN_POINT('Ctrl Pts',(-19.1270338823226,12.4581545252769,
132.171242119684)) ;
#152164=CARTESIAN_POINT('Ctrl Pts',(-19.0280972219191,12.3594525497003,
131.915366042047)) ;
#152165=CARTESIAN_POINT('Ctrl Pts',(-18.9241027514417,12.3367944069397,
131.644635976731)) ;
#152166=CARTESIAN_POINT('Ctrl Pts',(-18.8208265565642,12.3925085409291,
131.376240849143)) ;
#152167=CARTESIAN_POINT('Ctrl Pts',(-18.7265133411892,12.5213898755188,
131.133731510503)) ;
#152168=CARTESIAN_POINT('Ctrl Pts',(-18.6457952560714,12.7155724021421,
130.931131518529)) ;
#152169=CARTESIAN_POINT('Ctrl Pts',(-18.5846065804363,12.9595220676015,
130.785423050799)) ;
#152170=CARTESIAN_POINT('Ctrl Pts',(-18.546066469657,13.2367788940881,130.70592009773)) ;
#152171=CARTESIAN_POINT('Ctrl Pts',(-18.5323213213029,13.5277643625836,
130.698889739784)) ;
#152172=CARTESIAN_POINT('Ctrl Pts',(-18.543793348028,13.8120453761231,130.765623615628)) ;
#152173=CARTESIAN_POINT('Ctrl Pts',(-18.5788549474306,14.0676654739834,
130.901176319765)) ;
#152174=CARTESIAN_POINT('Ctrl Pts',(-18.6343035780449,14.2771419928287,
131.096308854122)) ;
#152175=CARTESIAN_POINT('Ctrl Pts',(-18.7050835708224,14.425031880978,131.336092927187)) ;
#152176=CARTESIAN_POINT('Ctrl Pts',(-18.7861994089251,14.5017260060049,
131.60629231186)) ;
#152177=CARTESIAN_POINT('Ctrl Pts',(-18.8699095303306,14.5010099059246,
131.883776032442)) ;
#152178=CARTESIAN_POINT('Ctrl Pts',(-18.950862117856,14.4231233705973,132.153475808602)) ;
#152179=CARTESIAN_POINT('Ctrl Pts',(-19.0216063325537,14.2735700722065,
132.393250548626)) ;
#152180=CARTESIAN_POINT('Ctrl Pts',(-19.0766525736922,14.0631260843178,
132.587185321685)) ;
#152181=CARTESIAN_POINT('Ctrl Pts',(-19.1112752517511,13.8068513237717,
132.721449739404)) ;
#152182=CARTESIAN_POINT('Ctrl Pts',(-19.1222768851844,13.5229068768556,
132.786731908381)) ;
#152183=CARTESIAN_POINT('Ctrl Pts',(-19.1081388609896,13.2323185296325,
132.778518604924)) ;
#152184=CARTESIAN_POINT('Ctrl Pts',(-19.0692979350921,12.955462422634,132.698120669452)) ;
#152185=CARTESIAN_POINT('Ctrl Pts',(-19.0072938758856,12.7108337306576,
132.550242420851)) ;
#152186=CARTESIAN_POINT('Ctrl Pts',(-18.9267369862212,12.5189036902296,
132.347912261719)) ;
#152187=CARTESIAN_POINT('Ctrl Pts',(-18.8318784493428,12.3906586207823,
132.103941582259)) ;
#152188=CARTESIAN_POINT('Ctrl Pts',(-18.7288363533557,12.3366531336248,
131.836123081131)) ;
#152189=CARTESIAN_POINT('Ctrl Pts',(-18.624925410328,12.360297772879,131.565617456112)) ;
#152190=CARTESIAN_POINT('Ctrl Pts',(-18.5256578035359,12.4609988515391,
131.308947306111)) ;
#152191=CARTESIAN_POINT('Ctrl Pts',(-18.4392051331275,12.6291274638668,
131.089332236554)) ;
#152192=CARTESIAN_POINT('Ctrl Pts',(-18.3692689876453,12.8555169755094,
130.918257614385)) ;
#152193=CARTESIAN_POINT('Ctrl Pts',(-18.3212190683975,13.1215885522129,
130.810953330662)) ;
#152194=CARTESIAN_POINT('Ctrl Pts',(-18.2972960902934,13.4096083938423,
130.774191778671)) ;
#152195=CARTESIAN_POINT('Ctrl Pts',(-18.2985416991129,13.698212942693,130.810897551179)) ;
#152196=CARTESIAN_POINT('Ctrl Pts',(-18.3244750392328,13.9691452295141,
130.91998909622)) ;
#152197=CARTESIAN_POINT('Ctrl Pts',(-18.3719691340465,14.1982918407705,
131.091726472608)) ;
#152198=CARTESIAN_POINT('Ctrl Pts',(-18.437100638801,14.3728095621698,131.315054734931)) ;
#152199=CARTESIAN_POINT('Ctrl Pts',(-18.5147502122421,14.479662285758,131.575038501861)) ;
#152200=CARTESIAN_POINT('Ctrl Pts',(-18.5984271700058,14.5107460879228,
131.852624565577)) ;
#152201=CARTESIAN_POINT('Ctrl Pts',(-18.6814592251425,14.4636147982726,
132.128355723987)) ;
#152202=CARTESIAN_POINT('Ctrl Pts',(-18.7567611079911,14.3427084720644,
132.38133252825)) ;
#152203=CARTESIAN_POINT('Ctrl Pts',(-18.8191499212685,14.1545214106307,
132.596878690056)) ;
#152204=CARTESIAN_POINT('Ctrl Pts',(-18.8624161383915,13.914665784431,132.756380600079)) ;
#152205=CARTESIAN_POINT('Ctrl Pts',(-18.8832226690577,13.6405172708492,
132.850185928448)) ;
#152206=CARTESIAN_POINT('Ctrl Pts',(-18.879379985006,13.3501102818962,132.872073497633)) ;
#152207=CARTESIAN_POINT('Ctrl Pts',(-18.8504830366193,13.0651843315454,
132.820727303234)) ;
#152208=CARTESIAN_POINT('Ctrl Pts',(-18.7972049191449,12.80388772374,132.698441638351)) ;
#152209=CARTESIAN_POINT('Ctrl Pts',(-18.723938579695,12.5899465270377,132.517340764542)) ;
#152210=CARTESIAN_POINT('Ctrl Pts',(-18.6339631078438,12.4339563210189,
132.28768165985)) ;
#152211=CARTESIAN_POINT('Ctrl Pts',(-18.533655418016,12.3491846989202,132.027754670765)) ;
#152212=CARTESIAN_POINT('Ctrl Pts',(-18.4287414629348,12.3415474281895,
131.754556958259)) ;
#152213=CARTESIAN_POINT('Ctrl Pts',(-18.3275546121177,12.4110292201394,
131.491915929484)) ;
#152214=CARTESIAN_POINT('Ctrl Pts',(-18.2349169164515,12.5533605448057,
131.254484931781)) ;
#152215=CARTESIAN_POINT('Ctrl Pts',(-18.1578099509812,12.7574391512257,
131.062286140571)) ;
#152216=CARTESIAN_POINT('Ctrl Pts',(-18.1003696787992,13.0095817126533,
130.92762938283)) ;
#152217=CARTESIAN_POINT('Ctrl Pts',(-18.0663253206741,13.2928226801242,
130.861470362866)) ;
#152218=CARTESIAN_POINT('Ctrl Pts',(-18.0574821752941,13.5820119966617,
130.868533156755)) ;
#152219=CARTESIAN_POINT('Ctrl Pts',(-18.0735684910089,13.8633229249982,
130.948835515899)) ;
#152220=CARTESIAN_POINT('Ctrl Pts',(-18.1128079244624,14.1112602779132,
131.096570682687)) ;
#152221=CARTESIAN_POINT('Ctrl Pts',(-18.1713264366975,14.3095521754014,
131.300538449874)) ;
#152222=CARTESIAN_POINT('Ctrl Pts',(-18.2445253330056,14.4451057235358,
131.547453993518)) ;
#152223=CARTESIAN_POINT('Ctrl Pts',(-18.3269176211252,14.5076745769451,
131.821434215678)) ;
#152224=CARTESIAN_POINT('Ctrl Pts',(-18.4109135921778,14.4918702514085,
132.09992274832)) ;
#152225=CARTESIAN_POINT('Ctrl Pts',(-18.4899530140776,14.4001695900989,
132.363825830347)) ;
#152226=CARTESIAN_POINT('Ctrl Pts',(-18.5581972721776,14.238339270588,132.596306467926)) ;
#152227=CARTESIAN_POINT('Ctrl Pts',(-18.6097312244741,14.0178457541506,
132.77999745246)) ;
#152228=CARTESIAN_POINT('Ctrl Pts',(-18.6401448193709,13.7549024704848,
132.901969265826)) ;
#152229=CARTESIAN_POINT('Ctrl Pts',(-18.6463850313128,13.4669383655623,
132.953465269722)) ;
#152230=CARTESIAN_POINT('Ctrl Pts',(-18.6276503009215,13.1792878389568,
132.931593942622)) ;
#152231=CARTESIAN_POINT('Ctrl Pts',(-18.5840179153444,12.9054935275296,
132.837423835677)) ;
#152232=CARTESIAN_POINT('Ctrl Pts',(-18.5184918875895,12.6708451835732,
132.679031311941)) ;
#152233=CARTESIAN_POINT('Ctrl Pts',(-18.4344363065144,12.4890109361581,
132.466673752346)) ;
#152234=CARTESIAN_POINT('Ctrl Pts',(-18.3378254602386,12.3747427440592,
132.217485900113)) ;
#152235=CARTESIAN_POINT('Ctrl Pts',(-18.2341291109171,12.335118127865,131.947725095572)) ;
#152236=CARTESIAN_POINT('Ctrl Pts',(-18.1304829793124,12.3735357257966,
131.678071654494)) ;
#152237=CARTESIAN_POINT('Ctrl Pts',(-18.0332195672274,12.4876827050984,
131.427169660191)) ;
#152238=CARTESIAN_POINT('Ctrl Pts',(-17.9493134502573,12.668143871092,131.215113064817)) ;
#152239=CARTESIAN_POINT('Ctrl Pts',(-17.8833190355393,12.9033827829949,
131.055504217813)) ;
#152240=CARTESIAN_POINT('Ctrl Pts',(-17.8397509602161,13.1743601664502,
130.961218011576)) ;
#152241=CARTESIAN_POINT('Ctrl Pts',(-17.8204668396867,13.4644840041335,
130.938043352746)) ;
#152242=CARTESIAN_POINT('Ctrl Pts',(-17.8265350254978,13.7518155739233,
130.988946607329)) ;
#152243=CARTESIAN_POINT('Ctrl Pts',(-17.8566012791567,14.0147480425275,
131.109855058721)) ;
#152244=CARTESIAN_POINT('Ctrl Pts',(-17.90786398017,14.2359322469135,131.292745615315)) ;
#152245=CARTESIAN_POINT('Ctrl Pts',(-17.9762298617494,14.3990328419962,
131.525712867481)) ;
#152246=CARTESIAN_POINT('Ctrl Pts',(-18.055065638864,14.4913721211862,131.788962667964)) ;
#152247=CARTESIAN_POINT('Ctrl Pts',(-18.1393991985355,14.5077030613306,
132.068583449212)) ;
#152248=CARTESIAN_POINT('Ctrl Pts',(-18.2210461373333,14.4466726935246,
132.340051735665)) ;
#152249=CARTESIAN_POINT('Ctrl Pts',(-18.2950035387414,14.3110620977678,
132.589454770925)) ;
#152250=CARTESIAN_POINT('Ctrl Pts',(-18.3535868279914,14.1132680684101,
132.793577578567)) ;
#152251=CARTESIAN_POINT('Ctrl Pts',(-18.393011856418,13.8656264960883,132.941870264204)) ;
#152252=CARTESIAN_POINT('Ctrl Pts',(-18.4093627200831,13.5853317318957,
133.022849013586)) ;
#152253=CARTESIAN_POINT('Ctrl Pts',(-18.4005900814448,13.2939513094312,
133.030374526169)) ;
#152254=CARTESIAN_POINT('Ctrl Pts',(-18.3670959101891,13.0136081090702,
132.965460512865)) ;
#152255=CARTESIAN_POINT('Ctrl Pts',(-18.3099441323283,12.7604084565328,
132.831704484875)) ;
#152256=CARTESIAN_POINT('Ctrl Pts',(-18.2330287799136,12.5556140537718,
132.640069906698)) ;
#152257=CARTESIAN_POINT('Ctrl Pts',(-18.1403993250708,12.412162783817,132.402717407191)) ;
#152258=CARTESIAN_POINT('Ctrl Pts',(-18.039122761627,12.3419224833159,132.139862058296)) ;
#152259=CARTESIAN_POINT('Ctrl Pts',(-17.9346214328855,12.3485705631489,
131.867734666129)) ;
#152260=CARTESIAN_POINT('Ctrl Pts',(-17.8340398826189,12.4325162173742,
131.60707108893)) ;
#152261=CARTESIAN_POINT('Ctrl Pts',(-17.7440580525167,12.5872706018155,
131.377320640071)) ;
#152262=CARTESIAN_POINT('Ctrl Pts',(-17.6702459325862,12.8016741765326,
131.1947873473)) ;
#152263=CARTESIAN_POINT('Ctrl Pts',(-17.6170393754709,13.0608926757193,
131.072495055625)) ;
#152264=CARTESIAN_POINT('Ctrl Pts',(-17.5876611427528,13.3463627388947,
131.019840506949)) ;
#152265=CARTESIAN_POINT('Ctrl Pts',(-17.5835099051843,13.6367413735624,
131.040812586735)) ;
#152266=CARTESIAN_POINT('Ctrl Pts',(-17.6040712549613,13.912123441329,131.134008457263)) ;
#152267=CARTESIAN_POINT('Ctrl Pts',(-17.6473147092117,14.1528033236638,
131.293522210415)) ;
#152268=CARTESIAN_POINT('Ctrl Pts',(-17.7090710684674,14.3402810134416,
131.506980670982)) ;
#152269=CARTESIAN_POINT('Ctrl Pts',(-17.784324421975,14.4626257099404,131.759874983544)) ;
#152270=CARTESIAN_POINT('Ctrl Pts',(-17.8676273435361,14.5106364099982,
132.036519206507)) ;
#152271=CARTESIAN_POINT('Ctrl Pts',(-17.9509431998974,14.4805445966973,
132.31289642704)) ;
#152272=CARTESIAN_POINT('Ctrl Pts',(-18.0287637016259,14.3748126779467,
132.57339232087)) ;
#152273=CARTESIAN_POINT('Ctrl Pts',(-18.0942745357637,14.2005693776624,
132.797921352006)) ;
#152274=CARTESIAN_POINT('Ctrl Pts',(-18.1420291731984,13.9714224956824,
132.970479780879)) ;
#152275=CARTESIAN_POINT('Ctrl Pts',(-18.1681061343277,13.7016038456452,
133.07989078727)) ;
#152276=CARTESIAN_POINT('Ctrl Pts',(-18.1697184694213,13.4137877720204,
133.117594113432)) ;
#152277=CARTESIAN_POINT('Ctrl Pts',(-18.1460719924332,13.1249621059971,
133.081716204354)) ;
#152278=CARTESIAN_POINT('Ctrl Pts',(-18.098349112227,12.858759801946,132.975335138158)) ;
#152279=CARTESIAN_POINT('Ctrl Pts',(-18.0285125557916,12.6311849064932,
132.804627705542)) ;
#152280=CARTESIAN_POINT('Ctrl Pts',(-17.9419067380147,12.4620614418067,
132.584665021202)) ;
#152281=CARTESIAN_POINT('Ctrl Pts',(-17.8431161137062,12.3611529243014,
132.329254527925)) ;
#152282=CARTESIAN_POINT('Ctrl Pts',(-17.7394163400758,12.336402737043,132.059308529178)) ;
#152283=CARTESIAN_POINT('Ctrl Pts',(-17.636008023939,12.3896954767389,131.790522379684)) ;
#152284=CARTESIAN_POINT('Ctrl Pts',(-17.5411529235148,12.5169545730866,
131.54651181945)) ;
#152285=CARTESIAN_POINT('Ctrl Pts',(-17.4601656512396,12.7090014500136,
131.343041028757)) ;
#152286=CARTESIAN_POINT('Ctrl Pts',(-17.3982954159609,12.9518209129291,
131.195365244849)) ;
#152287=CARTESIAN_POINT('Ctrl Pts',(-17.3590590475251,13.2283911259786,
131.113826328101)) ;
#152288=CARTESIAN_POINT('Ctrl Pts',(-17.3445909288019,13.5192444476926,
131.104682525303)) ;
#152289=CARTESIAN_POINT('Ctrl Pts',(-17.3552759397806,13.8035929406365,
131.169057687742)) ;
#152290=CARTESIAN_POINT('Ctrl Pts',(-17.3897650651813,14.0607675161601,
131.30300701978)) ;
#152291=CARTESIAN_POINT('Ctrl Pts',(-17.4443353177419,14.2709776513911,
131.49540177985)) ;
#152292=CARTESIAN_POINT('Ctrl Pts',(-17.5152284115638,14.4220258151157,
131.735762483094)) ;
#152293=CARTESIAN_POINT('Ctrl Pts',(-17.5958972727999,14.5004899933202,
132.004539334194)) ;
#152294=CARTESIAN_POINT('Ctrl Pts',(-17.6797407048686,14.5020985766214,
132.282472815977)) ;
#152295=CARTESIAN_POINT('Ctrl Pts',(-17.7606887259789,14.426667623352,132.552070316538)) ;
#152296=CARTESIAN_POINT('Ctrl Pts',(-17.8320641853255,14.2786158189735,
132.79380669298)) ;
#152297=CARTESIAN_POINT('Ctrl Pts',(-17.8875765378756,14.0697690186074,
132.989079973035)) ;
#152298=CARTESIAN_POINT('Ctrl Pts',(-17.922834488677,13.8142976320865,133.125231432651)) ;
#152299=CARTESIAN_POINT('Ctrl Pts',(-17.9345112522901,13.5318062075926,
133.19237603013)) ;
#152300=CARTESIAN_POINT('Ctrl Pts',(-17.9211404368569,13.2403761874523,
133.186487415733)) ;
#152301=CARTESIAN_POINT('Ctrl Pts',(-17.8827207165006,12.9618561593774,
133.107451653599)) ;
#152302=CARTESIAN_POINT('Ctrl Pts',(-17.821581417852,12.7173263730279,132.96193349821)) ;
#152303=CARTESIAN_POINT('Ctrl Pts',(-17.7413926221805,12.5233446886838,
132.760735766704)) ;
#152304=CARTESIAN_POINT('Ctrl Pts',(-17.6467746618759,12.3931312315505,
132.517486220828)) ;
#152305=CARTESIAN_POINT('Ctrl Pts',(-17.5437035922363,12.337075246258,132.249632321582)) ;
#152306=CARTESIAN_POINT('Ctrl Pts',(-17.4401454160532,12.3586764449227,
131.98003227223)) ;
#152307=CARTESIAN_POINT('Ctrl Pts',(-17.3410665934673,12.4563696314589,
131.723751639427)) ;
#152308=CARTESIAN_POINT('Ctrl Pts',(-17.2536320179894,12.6234424170359,
131.50146332499)) ;
#152309=CARTESIAN_POINT('Ctrl Pts',(-17.1832036195686,12.8484690314232,
131.32893954711)) ;
#152310=CARTESIAN_POINT('Ctrl Pts',(-17.1344653483001,13.1134860607375,
131.219613229379)) ;
#152311=CARTESIAN_POINT('Ctrl Pts',(-17.1097906021278,13.402425050447,131.180795951585)) ;
#152312=CARTESIAN_POINT('Ctrl Pts',(-17.1104146704051,13.6901681944769,
131.215561704661)) ;
#152313=CARTESIAN_POINT('Ctrl Pts',(-17.1355551568111,13.9614083380647,
131.322263958797)) ;
#152314=CARTESIAN_POINT('Ctrl Pts',(-17.1825349214449,14.1924050674132,
131.492558721692)) ;
#152315=CARTESIAN_POINT('Ctrl Pts',(-17.247284144374,14.3688010159201,131.714792207733)) ;
#152316=CARTESIAN_POINT('Ctrl Pts',(-17.3247083783915,14.4776662097744,
131.974131076165)) ;
#152317=CARTESIAN_POINT('Ctrl Pts',(-17.4080456851403,14.5108828480259,
132.250624200494)) ;
#152318=CARTESIAN_POINT('Ctrl Pts',(-17.4912091781135,14.4662997711349,
132.526737050679)) ;
#152319=CARTESIAN_POINT('Ctrl Pts',(-17.5670722488366,14.3468724358185,
132.781476724685)) ;
#152320=CARTESIAN_POINT('Ctrl Pts',(-17.6295496572066,14.161614932188,132.997074962764)) ;
#152321=CARTESIAN_POINT('Ctrl Pts',(-17.6736158962945,13.9230022753498,
133.158962448849)) ;
#152322=CARTESIAN_POINT('Ctrl Pts',(-17.6951931588153,13.6485314062169,
133.25514650467)) ;
#152323=CARTESIAN_POINT('Ctrl Pts',(-17.6920615738823,13.3583011743042,
133.279105884718)) ;
#152324=CARTESIAN_POINT('Ctrl Pts',(-17.6637579865309,13.072504270402,133.229551323447)) ;
#152325=CARTESIAN_POINT('Ctrl Pts',(-17.6114584214845,12.8117566735177,
133.109923707737)) ;
#152326=CARTESIAN_POINT('Ctrl Pts',(-17.5386760935971,12.5955171582893,
132.930311398659)) ;
#152327=CARTESIAN_POINT('Ctrl Pts',(-17.4485485923782,12.4369580568928,
132.700390646819)) ;
#152328=CARTESIAN_POINT('Ctrl Pts',(-17.3489049682672,12.3507869630092,
132.442246375848)) ;
#152329=CARTESIAN_POINT('Ctrl Pts',(-17.2444930320388,12.3404899643528,
132.170365644373)) ;
#152330=CARTESIAN_POINT('Ctrl Pts',(-17.1426216271441,12.4078494476239,
131.905884901552)) ;
#152331=CARTESIAN_POINT('Ctrl Pts',(-17.0495668256941,12.5483871977687,
131.667259067528)) ;
#152332=CARTESIAN_POINT('Ctrl Pts',(-16.971814498006,12.7513533086917,131.473242742698)) ;
#152333=CARTESIAN_POINT('Ctrl Pts',(-16.9139622836365,13.001941318222,131.337310415625)) ;
#152334=CARTESIAN_POINT('Ctrl Pts',(-16.8792750897038,13.2828868274063,
131.269082634896)) ;
#152335=CARTESIAN_POINT('Ctrl Pts',(-16.8695679518648,13.5743278631276,
131.273876133887)) ;
#152336=CARTESIAN_POINT('Ctrl Pts',(-16.8850187674673,13.8554587804339,
131.352236081223)) ;
#152337=CARTESIAN_POINT('Ctrl Pts',(-16.9233899892215,14.103739100914,131.497307260457)) ;
#152338=CARTESIAN_POINT('Ctrl Pts',(-16.9815525794946,14.3046990175591,
131.70035759611)) ;
#152339=CARTESIAN_POINT('Ctrl Pts',(-17.0547401043487,14.4424188711516,
131.947366060444)) ;
#152340=CARTESIAN_POINT('Ctrl Pts',(-17.1362824190426,14.5067209234145,
132.218584626412)) ;
#152341=CARTESIAN_POINT('Ctrl Pts',(-17.2205230150152,14.4936392684735,
132.497872334383)) ;
#152342=CARTESIAN_POINT('Ctrl Pts',(-17.2999675507863,14.404006740505,132.76301963)) ;
#152343=CARTESIAN_POINT('Ctrl Pts',(-17.3687938432936,14.2433942656814,
132.99730827925)) ;
#152344=CARTESIAN_POINT('Ctrl Pts',(-17.4206621252372,14.0252993056693,
133.181832423558)) ;
#152345=CARTESIAN_POINT('Ctrl Pts',(-17.4518062177166,13.7626963119846,
133.306025850587)) ;
#152346=CARTESIAN_POINT('Ctrl Pts',(-17.4588018749284,13.4766513624265,
133.3595520989)) ;
#152347=CARTESIAN_POINT('Ctrl Pts',(-17.4407196010973,13.1866966293381,
133.339828540076)) ;
#152348=CARTESIAN_POINT('Ctrl Pts',(-17.3976621744542,12.9123106961637,
133.247325290375)) ;
#152349=CARTESIAN_POINT('Ctrl Pts',(-17.3328316521718,12.6769408805555,
133.090898057899)) ;
#152350=CARTESIAN_POINT('Ctrl Pts',(-17.2494627622651,12.4935889535621,
132.880470073151)) ;
#152351=CARTESIAN_POINT('Ctrl Pts',(-17.152618226233,12.3766908568814,132.630777552473)) ;
#152352=CARTESIAN_POINT('Ctrl Pts',(-17.049231423334,12.3352383862452,132.361846606225)) ;
#152353=CARTESIAN_POINT('Ctrl Pts',(-16.9457336891591,12.3713736006973,
132.092556286143)) ;
#152354=CARTESIAN_POINT('Ctrl Pts',(-16.8484161060952,12.4827590293817,
131.841396897906)) ;
#152355=CARTESIAN_POINT('Ctrl Pts',(-16.7634777794498,12.6627224306716,
131.626558702344)) ;
#152356=CARTESIAN_POINT('Ctrl Pts',(-16.6972681323854,12.8955397849013,
131.466150815898)) ;
#152357=CARTESIAN_POINT('Ctrl Pts',(-16.652840547036,13.1663558963296,131.369445368094)) ;
#152358=CARTESIAN_POINT('Ctrl Pts',(-16.6328908225603,13.4563321062043,
131.344330530745)) ;
#152359=CARTESIAN_POINT('Ctrl Pts',(-16.6382111416064,13.74354179735,131.392991362756)) ;
#152360=CARTESIAN_POINT('Ctrl Pts',(-16.6676592322395,14.007863745204,131.512146621969)) ;
#152361=CARTESIAN_POINT('Ctrl Pts',(-16.7182928746253,14.2299792391956,
131.693135937676)) ;
#152362=CARTESIAN_POINT('Ctrl Pts',(-16.7859878307255,14.3948659481182,
131.924049786769)) ;
#152363=CARTESIAN_POINT('Ctrl Pts',(-16.8651153132331,14.4898740802148,
132.188374983265)) ;
#152364=CARTESIAN_POINT('Ctrl Pts',(-16.9488778829896,14.5084149248409,
132.466110688147)) ;
#152365=CARTESIAN_POINT('Ctrl Pts',(-17.0311885247318,14.4492459338564,
132.739733964955)) ;
#152366=CARTESIAN_POINT('Ctrl Pts',(-17.104950151554,14.316609488643,132.988318108268)) ;
#152367=CARTESIAN_POINT('Ctrl Pts',(-17.1643724443007,14.1198900556279,
133.195042593654)) ;
#152368=CARTESIAN_POINT('Ctrl Pts',(-17.2043618345605,13.8734079349303,
133.344971495627)) ;
#152369=CARTESIAN_POINT('Ctrl Pts',(-17.2214102827416,13.5947694158123,
133.42787905469)) ;
#152370=CARTESIAN_POINT('Ctrl Pts',(-17.2135302438731,13.3033325180628,
133.438020470237)) ;
#152371=CARTESIAN_POINT('Ctrl Pts',(-17.1805025277542,13.0207084742087,
133.374676701685)) ;
#152372=CARTESIAN_POINT('Ctrl Pts',(-17.124234300538,12.767628690545,133.243341451459)) ;
#152373=CARTESIAN_POINT('Ctrl Pts',(-17.0476257592213,12.5604751539345,
133.052712263167)) ;
#152374=CARTESIAN_POINT('Ctrl Pts',(-16.9553890051503,12.4152916729436,
132.816483612565)) ;
#152375=CARTESIAN_POINT('Ctrl Pts',(-16.8542709676215,12.3428120631862,
132.554100291461)) ;
#152376=CARTESIAN_POINT('Ctrl Pts',(-16.7494730831066,12.3473797413046,
132.281194465277)) ;
#152377=CARTESIAN_POINT('Ctrl Pts',(-16.6487943422117,12.4294695368143,
132.020223589768)) ;
#152378=CARTESIAN_POINT('Ctrl Pts',(-16.5588158738871,12.5816148375682,
131.790339248201)) ;
#152379=CARTESIAN_POINT('Ctrl Pts',(-16.4842129576639,12.7949907280796,
131.605591372129)) ;
#152380=CARTESIAN_POINT('Ctrl Pts',(-16.4302842435271,13.054101177031,131.481287531456)) ;
#152381=CARTESIAN_POINT('Ctrl Pts',(-16.4003618883851,13.3386274126212,
131.426981031138)) ;
#152382=CARTESIAN_POINT('Ctrl Pts',(-16.3954982522069,13.6281884734652,
131.445764473398)) ;
#152383=CARTESIAN_POINT('Ctrl Pts',(-16.4153244875857,13.9042249218154,
131.536802751734)) ;
#152384=CARTESIAN_POINT('Ctrl Pts',(-16.4579192874622,14.1463903457502,
131.694429834647)) ;
#152385=CARTESIAN_POINT('Ctrl Pts',(-16.519604946235,14.3364819716926,131.907871784003)) ;
#152386=CARTESIAN_POINT('Ctrl Pts',(-16.5941877045133,14.4598817702337,
132.158628290576)) ;
#152387=CARTESIAN_POINT('Ctrl Pts',(-16.6772180078865,14.5104486170863,
132.434425087988)) ;
#152388=CARTESIAN_POINT('Ctrl Pts',(-16.7610712369098,14.4822486369166,
132.712559593312)) ;
#152389=CARTESIAN_POINT('Ctrl Pts',(-16.8386672352436,14.3791733041028,
132.97219580738)) ;
#152390=CARTESIAN_POINT('Ctrl Pts',(-16.9049174530084,14.2063740303146,
133.199006100538)) ;
#152391=CARTESIAN_POINT('Ctrl Pts',(-16.9532362150924,13.9777765864427,
133.373293310572)) ;
#152392=CARTESIAN_POINT('Ctrl Pts',(-16.9798528341138,13.7109259499415,
133.484028399788)) ;
#152393=CARTESIAN_POINT('Ctrl Pts',(-16.9822174695309,13.4211174151953,
133.524197897855)) ;
#152394=CARTESIAN_POINT('Ctrl Pts',(-16.9593603734184,13.1336909339448,
133.490426214311)) ;
#152395=CARTESIAN_POINT('Ctrl Pts',(-16.9122699848515,12.8658812639418,
133.385975367206)) ;
#152396=CARTESIAN_POINT('Ctrl Pts',(-16.8429275372481,12.6367690190525,
133.216731683706)) ;
#152397=CARTESIAN_POINT('Ctrl Pts',(-16.7566414738858,12.4658337897599,
132.997733929609)) ;
#152398=CARTESIAN_POINT('Ctrl Pts',(-16.6584445847538,12.3631245211514,
132.743942914283)) ;
#152399=CARTESIAN_POINT('Ctrl Pts',(-16.5545911413088,12.3360466241608,
132.473621289443)) ;
#152400=CARTESIAN_POINT('Ctrl Pts',(-16.4514231221753,12.3868688002356,
132.205414356226)) ;
#152401=CARTESIAN_POINT('Ctrl Pts',(-16.3561369237034,12.5119418325269,
131.960173693308)) ;
#152402=CARTESIAN_POINT('Ctrl Pts',(-16.2746048987367,12.7021783709845,
131.755117298832)) ;
#152403=CARTESIAN_POINT('Ctrl Pts',(-16.2118058427217,12.9449353770794,
131.604890369302)) ;
#152404=CARTESIAN_POINT('Ctrl Pts',(-16.1719673653937,13.2214383784226,
131.521650682401)) ;
#152405=CARTESIAN_POINT('Ctrl Pts',(-16.1568634879724,13.5108147708277,
131.510491075186)) ;
#152406=CARTESIAN_POINT('Ctrl Pts',(-16.1669300007681,13.7968084175674,
131.573203022695)) ;
#152407=CARTESIAN_POINT('Ctrl Pts',(-16.2006569741179,14.0536576083437,
131.704754764011)) ;
#152408=CARTESIAN_POINT('Ctrl Pts',(-16.254784608073,14.2659120564335,131.895928413579)) ;
#152409=CARTESIAN_POINT('Ctrl Pts',(-16.3251935914364,14.4185012516542,
132.134813692496)) ;
#152410=CARTESIAN_POINT('Ctrl Pts',(-16.4055493007845,14.4992712221482,
132.402638758212)) ;
#152411=CARTESIAN_POINT('Ctrl Pts',(-16.4897480826034,14.5031360116066,
132.681750239267)) ;
#152412=CARTESIAN_POINT('Ctrl Pts',(-16.5707620204115,14.4296202074177,
132.951505237183)) ;
#152413=CARTESIAN_POINT('Ctrl Pts',(-16.6421991335516,14.2844131247839,
133.193261917155)) ;
#152414=CARTESIAN_POINT('Ctrl Pts',(-16.6984700341114,14.0764755685082,
133.390876378768)) ;
#152415=CARTESIAN_POINT('Ctrl Pts',(-16.7342912161991,13.8227947339683,
133.528581938243)) ;
#152416=CARTESIAN_POINT('Ctrl Pts',(-16.7467556388197,13.5398702989391,
133.59814585037)) ;
#152417=CARTESIAN_POINT('Ctrl Pts',(-16.7340724183047,13.2487717783427,
133.594219576124)) ;
#152418=CARTESIAN_POINT('Ctrl Pts',(-16.6965212883533,12.9703362151756,
133.517627433161)) ;
#152419=CARTESIAN_POINT('Ctrl Pts',(-16.6359937287517,12.7241092781338,
133.373940651091)) ;
#152420=CARTESIAN_POINT('Ctrl Pts',(-16.5560795871543,12.5279171433205,
133.173632261453)) ;
#152421=CARTESIAN_POINT('Ctrl Pts',(-16.4618411443677,12.3959938665945,
132.931466168076)) ;
#152422=CARTESIAN_POINT('Ctrl Pts',(-16.3593827732272,12.3376260980812,
132.665255360874)) ;
#152423=CARTESIAN_POINT('Ctrl Pts',(-16.2550385035652,12.3570497794023,
132.393594158916)) ;
#152424=CARTESIAN_POINT('Ctrl Pts',(-16.1560569930776,12.4525559733436,
132.137489642659)) ;
#152425=CARTESIAN_POINT('Ctrl Pts',(-16.0682112092327,12.6176036105847,
131.9139932347)) ;
#152426=CARTESIAN_POINT('Ctrl Pts',(-15.9972052369213,12.8410947019102,
131.739774174027)) ;
#152427=CARTESIAN_POINT('Ctrl Pts',(-15.9477710009751,13.1055203518464,
131.628457545108)) ;
#152428=CARTESIAN_POINT('Ctrl Pts',(-15.9223966595682,13.3928980327512,
131.587457525944)) ;
#152429=CARTESIAN_POINT('Ctrl Pts',(-15.9222756880834,13.6824543649216,
131.620230232659)) ;
#152430=CARTESIAN_POINT('Ctrl Pts',(-15.9466295677973,13.9532692757644,
131.724475741057)) ;
#152431=CARTESIAN_POINT('Ctrl Pts',(-15.9930649492766,14.1862511235797,
131.893256545959)) ;
#152432=CARTESIAN_POINT('Ctrl Pts',(-16.0572774469947,14.3643962082537,
132.113884233036)) ;
#152433=CARTESIAN_POINT('Ctrl Pts',(-16.1348869305229,14.4759024807437,
132.373959659061)) ;
#152434=CARTESIAN_POINT('Ctrl Pts',(-16.2178601983213,14.5109062464403,
132.649271579231)) ;
#152435=CARTESIAN_POINT('Ctrl Pts',(-16.3010573982548,14.4687351628052,
132.925452283273)) ;
#152436=CARTESIAN_POINT('Ctrl Pts',(-16.3772524895357,14.351243796897,133.18118301111)) ;
#152437=CARTESIAN_POINT('Ctrl Pts',(-16.4401554780105,14.1681343550178,
133.397975738382)) ;
#152438=CARTESIAN_POINT('Ctrl Pts',(-16.4850310227968,13.9291093552066,
133.562448350169)) ;
#152439=CARTESIAN_POINT('Ctrl Pts',(-16.5070926720565,13.6572015399983,
133.659816803159)) ;
#152440=CARTESIAN_POINT('Ctrl Pts',(-16.5046943032788,13.3659146668707,
133.686064790888)) ;
#152441=CARTESIAN_POINT('Ctrl Pts',(-16.4771547092974,13.0809591455927,
133.638599282157)) ;
#152442=CARTESIAN_POINT('Ctrl Pts',(-16.4256137570119,12.8188859308948,
133.521201214271)) ;
#152443=CARTESIAN_POINT('Ctrl Pts',(-16.3527339561376,12.5999510440463,
133.341543109138)) ;
#152444=CARTESIAN_POINT('Ctrl Pts',(-16.2641281336111,12.4414984825018,
133.115647334815)) ;
#152445=CARTESIAN_POINT('Ctrl Pts',(-16.1641430091743,12.3520343108791,
132.85671610708)) ;
#152446=CARTESIAN_POINT('Ctrl Pts',(-16.0594698293865,12.3398054622105,
132.584157469235)) ;
#152447=CARTESIAN_POINT('Ctrl Pts',(-15.9577980199829,12.4047865271677,
132.320144279598)) ;
#152448=CARTESIAN_POINT('Ctrl Pts',(-15.8643756324851,12.5431933869583,
132.080444267518)) ;
#152449=CARTESIAN_POINT('Ctrl Pts',(-15.7860699178347,12.7444965603529,
131.884816381687)) ;
#152450=CARTESIAN_POINT('Ctrl Pts',(-15.7274833077799,12.9945025224571,
131.746812479205)) ;
#152451=CARTESIAN_POINT('Ctrl Pts',(-15.6921182047523,13.2745329094811,
131.676561655677)) ;
#152452=CARTESIAN_POINT('Ctrl Pts',(-15.6817523163213,13.5670626370277,
131.679561862218)) ;
#152453=CARTESIAN_POINT('Ctrl Pts',(-15.6963153264075,13.8462370772247,
131.755016293096)) ;
#152454=CARTESIAN_POINT('Ctrl Pts',(-15.7342967830937,14.0979241250953,
131.899230741437)) ;
#152455=CARTESIAN_POINT('Ctrl Pts',(-15.7919436686276,14.2997383418867,
132.100703473067)) ;
#152456=CARTESIAN_POINT('Ctrl Pts',(-15.8645031781154,14.4393312193764,
132.345773094754)) ;
#152457=CARTESIAN_POINT('Ctrl Pts',(-15.9465184391645,14.5060643569228,
132.618629039297)) ;
#152458=CARTESIAN_POINT('Ctrl Pts',(-16.0301677623958,14.4951758782706,
132.895935895831)) ;
#152459=CARTESIAN_POINT('Ctrl Pts',(-16.1102104627669,14.4072623281432,
133.163000755797)) ;
#152460=CARTESIAN_POINT('Ctrl Pts',(-16.1790779676799,14.2495039694875,
133.397213921694)) ;
#152461=CARTESIAN_POINT('Ctrl Pts',(-16.2319003919638,14.0308221258824,
133.584830620202)) ;
#152462=CARTESIAN_POINT('Ctrl Pts',(-16.2633270017823,13.7719100664948,
133.709489495124)) ;
#152463=CARTESIAN_POINT('Ctrl Pts',(-16.2711876727272,13.4847456450531,
133.765738112161)) ;
#152464=CARTESIAN_POINT('Ctrl Pts',(-16.253847194686,13.1955425031336,133.748069200693)) ;
#152465=CARTESIAN_POINT('Ctrl Pts',(-16.2115198754741,12.9200552968874,
133.65773228028)) ;
#152466=CARTESIAN_POINT('Ctrl Pts',(-16.147222084084,12.6831184385928,133.502892140705)) ;
#152467=CARTESIAN_POINT('Ctrl Pts',(-16.064282599147,12.4980281206389,133.293729089209)) ;
#152468=CARTESIAN_POINT('Ctrl Pts',(-15.9679392810076,12.3791543430107,
133.045434009803)) ;
#152469=CARTESIAN_POINT('Ctrl Pts',(-15.8643595558364,12.3353503717386,
132.776040083288)) ;
#152470=CARTESIAN_POINT('Ctrl Pts',(-15.7608810145636,12.3691099621928,
132.506761731086)) ;
#152471=CARTESIAN_POINT('Ctrl Pts',(-15.6627255542582,12.4795856785055,
132.253375320536)) ;
#152472=CARTESIAN_POINT('Ctrl Pts',(-15.5784730291827,12.6553361009926,
132.040088792181)) ;
#152473=CARTESIAN_POINT('Ctrl Pts',(-15.5110293575352,12.8882259217544,
131.876334600156)) ;
#152474=CARTESIAN_POINT('Ctrl Pts',(-15.4660114239873,13.1581921393272,
131.777882402057)) ;
#152475=CARTESIAN_POINT('Ctrl Pts',(-15.4453153424862,13.4482190387101,
131.750625899504)) ;
#152476=CARTESIAN_POINT('Ctrl Pts',(-15.4499239120655,13.7352663202425,
131.797145410483)) ;
#152477=CARTESIAN_POINT('Ctrl Pts',(-15.4786708796544,14.0004787425337,
131.914245491789)) ;
#152478=CARTESIAN_POINT('Ctrl Pts',(-15.528718936817,14.2242401467777,132.093531049238)) ;
#152479=CARTESIAN_POINT('Ctrl Pts',(-15.5963327554751,14.391486003047,132.324353743837)) ;
#152480=CARTESIAN_POINT('Ctrl Pts',(-15.6747831211035,14.4880341837757,
132.586510244365)) ;
#152481=CARTESIAN_POINT('Ctrl Pts',(-15.7588156763009,14.5089767222778,
132.865167334381)) ;
#152482=CARTESIAN_POINT('Ctrl Pts',(-15.8410228376495,14.4520807364783,
133.138385805997)) ;
#152483=CARTESIAN_POINT('Ctrl Pts',(-15.9152233944989,14.3213934969356,
133.388297276998)) ;
#152484=CARTESIAN_POINT('Ctrl Pts',(-15.9751021978438,14.126427628205,133.596336490836)) ;
#152485=CARTESIAN_POINT('Ctrl Pts',(-16.0157883783172,13.8807880817665,
133.748352793927)) ;
#152486=CARTESIAN_POINT('Ctrl Pts',(-16.0334719367804,13.6022566506269,
133.833171646611)) ;
#152487=CARTESIAN_POINT('Ctrl Pts',(-16.0263427101219,13.3123739575692,
133.845337187169)) ;
#152488=CARTESIAN_POINT('Ctrl Pts',(-15.9941097511416,13.0290004002489,
133.784332603085)) ;
#152489=CARTESIAN_POINT('Ctrl Pts',(-15.9383247563886,12.7741270713226,
133.65449670321)) ;
#152490=CARTESIAN_POINT('Ctrl Pts',(-15.8622768484471,12.5657352250487,
133.465472847607)) ;
#152491=CARTESIAN_POINT('Ctrl Pts',(-15.7707760397584,12.4188762117679,
133.231275457079)) ;
#152492=CARTESIAN_POINT('Ctrl Pts',(-15.6694610724198,12.3438128452305,
132.968446766761)) ;
#152493=CARTESIAN_POINT('Ctrl Pts',(-15.5650490222749,12.3461025205116,
132.696542230689)) ;
#152494=CARTESIAN_POINT('Ctrl Pts',(-15.4641117267899,12.4255735874937,
132.43482095437)) ;
#152495=CARTESIAN_POINT('Ctrl Pts',(-15.3733010936375,12.5765456735502,
132.202668192957)) ;
#152496=CARTESIAN_POINT('Ctrl Pts',(-15.2984189865204,12.7879286592572,
132.017014437685)) ;
#152497=CARTESIAN_POINT('Ctrl Pts',(-15.243943520018,13.0448054046113,131.89098628761)) ;
#152498=CARTESIAN_POINT('Ctrl Pts',(-15.2130872375626,13.329756321322,131.834065836623)) ;
#152499=CARTESIAN_POINT('Ctrl Pts',(-15.207498078425,13.6201107178654,131.850804210703)) ;
#152500=CARTESIAN_POINT('Ctrl Pts',(-15.226664565684,13.8967554382586,131.93990903969)) ;
#152501=CARTESIAN_POINT('Ctrl Pts',(-15.2685096670752,14.1394983367384,
132.095250212473)) ;
#152502=CARTESIAN_POINT('Ctrl Pts',(-15.3296325471033,14.3315001569242,
132.307040763849)) ;
#152503=CARTESIAN_POINT('Ctrl Pts',(-15.4041948784221,14.4575222943013,
132.557868425866)) ;
#152504=CARTESIAN_POINT('Ctrl Pts',(-15.4871845489021,14.5099977938908,
132.833577267545)) ;
#152505=CARTESIAN_POINT('Ctrl Pts',(-15.5706474715052,14.4843800867397,
133.110384973781)) ;
#152506=CARTESIAN_POINT('Ctrl Pts',(-15.6489358172198,14.3828781461486,
133.372231534079)) ;
#152507=CARTESIAN_POINT('Ctrl Pts',(-15.7152215321923,14.212816168216,133.598953578525)) ;
#152508=CARTESIAN_POINT('Ctrl Pts',(-15.7643324415315,13.9854781681749,
133.775621838138)) ;
#152509=CARTESIAN_POINT('Ctrl Pts',(-15.7916807767753,13.7179644909653,
133.888670251454)) ;
#152510=CARTESIAN_POINT('Ctrl Pts',(-15.7946921387686,13.4301920376034,
133.930530607513)) ;
#152511=CARTESIAN_POINT('Ctrl Pts',(-15.7726967990617,13.1421055633853,
133.899307008492)) ;
#152512=CARTESIAN_POINT('Ctrl Pts',(-15.725756949418,12.87150128464,133.795559990037)) ;
#152513=CARTESIAN_POINT('Ctrl Pts',(-15.6577073073503,12.6436097991943,
133.629723531333)) ;
#152514=CARTESIAN_POINT('Ctrl Pts',(-15.5716152896333,12.4698498437503,
133.411423269474)) ;
#152515=CARTESIAN_POINT('Ctrl Pts',(-15.4736825799438,12.3651221856613,
133.158394352247)) ;
#152516=CARTESIAN_POINT('Ctrl Pts',(-15.3697907387214,12.335692224637,132.887997751447)) ;
#152517=CARTESIAN_POINT('Ctrl Pts',(-15.2664401785828,12.3844432071478,
132.619277578795)) ;
#152518=CARTESIAN_POINT('Ctrl Pts',(-15.1710399074463,12.5072147901112,
132.373635971455)) ;
#152519=CARTESIAN_POINT('Ctrl Pts',(-15.0889535850671,12.6957550150873,
132.166979770339)) ;
#152520=CARTESIAN_POINT('Ctrl Pts',(-15.0255721551039,12.9372999479051,
132.01505517321)) ;
#152521=CARTESIAN_POINT('Ctrl Pts',(-14.9850575690906,13.2121499543988,
131.929735608954)) ;
#152522=CARTESIAN_POINT('Ctrl Pts',(-14.9691714974783,13.5032465104466,
131.91650779929)) ;
#152523=CARTESIAN_POINT('Ctrl Pts',(-14.9783938577685,13.7871080328991,
131.976440567623)) ;
#152524=CARTESIAN_POINT('Ctrl Pts',(-15.0115648784408,14.0469104745439,
132.106594492085)) ;
#152525=CARTESIAN_POINT('Ctrl Pts',(-15.0651801887707,14.2605649124229,
132.296255586953)) ;
#152526=CARTESIAN_POINT('Ctrl Pts',(-15.1354050179275,14.4153649488043,
132.534693807358)) ;
#152527=CARTESIAN_POINT('Ctrl Pts',(-15.2152370606947,14.4978582783663,
132.800850624746)) ;
#152528=CARTESIAN_POINT('Ctrl Pts',(-15.2994258322498,14.5041773990225,
133.079939121836)) ;
#152529=CARTESIAN_POINT('Ctrl Pts',(-15.3806609287712,14.4329779197685,
133.350346880059)) ;
#152530=CARTESIAN_POINT('Ctrl Pts',(-15.4527495072584,14.2890422314917,
133.594146581102)) ;
#152531=CARTESIAN_POINT('Ctrl Pts',(-15.5093788401438,14.082779433517,133.79275764401)) ;
#152532=CARTESIAN_POINT('Ctrl Pts',(-15.545753191267,13.8309337098099,133.931989144067)) ;
#152533=CARTESIAN_POINT('Ctrl Pts',(-15.5589571408963,13.5483120187831,
134.003745938923)) ;
#152534=CARTESIAN_POINT('Ctrl Pts',(-15.5470459162325,13.2574777531019,
134.002035659956)) ;
#152535=CARTESIAN_POINT('Ctrl Pts',(-15.510131605999,12.9779697529959,133.92735890912)) ;
#152536=CARTESIAN_POINT('Ctrl Pts',(-15.4504417667573,12.7311580251373,
133.786020643798)) ;
#152537=CARTESIAN_POINT('Ctrl Pts',(-15.3706607271275,12.5323980592304,
133.586256423076)) ;
#152538=CARTESIAN_POINT('Ctrl Pts',(-15.2770803375685,12.3989897288854,
133.345890363007)) ;
#152539=CARTESIAN_POINT('Ctrl Pts',(-15.1745710010167,12.3382487603058,
133.079602207309)) ;
#152540=CARTESIAN_POINT('Ctrl Pts',(-15.0705359722807,12.3552058083452,
132.808726876001)) ;
#152541=CARTESIAN_POINT('Ctrl Pts',(-14.9706606470321,12.4490680703867,
132.550225448555)) ;
#152542=CARTESIAN_POINT('Ctrl Pts',(-14.8824522342596,12.612854304799,132.325691498574)) ;
#152543=CARTESIAN_POINT('Ctrl Pts',(-14.8113527265263,12.8333918295054,
132.150980279395)) ;
#152544=CARTESIAN_POINT('Ctrl Pts',(-14.7610563805274,13.0975419155814,
132.037242671929)) ;
#152545=CARTESIAN_POINT('Ctrl Pts',(-14.7349932181902,13.3843701567211,
131.99420597981)) ;
#152546=CARTESIAN_POINT('Ctrl Pts',(-14.7341460984049,13.6749248626015,
132.024944556395)) ;
#152547=CARTESIAN_POINT('Ctrl Pts',(-14.7579228982456,13.9463602578246,
132.127499501483)) ;
#152548=CARTESIAN_POINT('Ctrl Pts',(-14.8035289837161,14.1798324379302,
132.293714438332)) ;
#152549=CARTESIAN_POINT('Ctrl Pts',(-14.8677079251816,14.3606302769089,
132.514446261517)) ;
#152550=CARTESIAN_POINT('Ctrl Pts',(-14.9443462637881,14.4733618864566,
132.771384751192)) ;
#152551=CARTESIAN_POINT('Ctrl Pts',(-15.0280034573494,14.5110756600993,
133.049012799316)) ;
#152552=CARTESIAN_POINT('Ctrl Pts',(-15.1108313580727,14.4709889009811,
133.323927299789)) ;
#152553=CARTESIAN_POINT('Ctrl Pts',(-15.1874906865422,14.3556941984043,
133.581070483478)) ;
#152554=CARTESIAN_POINT('Ctrl Pts',(-15.2510153385486,14.1731666486328,
133.79982111375)) ;
#152555=CARTESIAN_POINT('Ctrl Pts',(-15.2960503606692,13.9378584167298,
133.964426013949)) ;
#152556=CARTESIAN_POINT('Ctrl Pts',(-15.3190310826371,13.6656355311939,
134.064636189014)) ;
#152557=CARTESIAN_POINT('Ctrl Pts',(-15.3173445451022,13.3744563081115,
134.092966610367)) ;
#152558=CARTESIAN_POINT('Ctrl Pts',(-15.2904580609234,13.0885611803192,
134.047472889722)) ;
#152559=CARTESIAN_POINT('Ctrl Pts',(-15.2396747814133,12.8263306498725,
133.932194970172)) ;
#152560=CARTESIAN_POINT('Ctrl Pts',(-15.1677163389787,12.6063807769631,
133.755109558956)) ;
#152561=CARTESIAN_POINT('Ctrl Pts',(-15.0788943634793,12.4447492933123,
133.528822932428)) ;
#152562=CARTESIAN_POINT('Ctrl Pts',(-14.9791253222199,12.3535025882306,
133.270511156007)) ;
#152563=CARTESIAN_POINT('Ctrl Pts',(-14.8746674650902,12.3391045054194,
132.998527191728)) ;
#152564=CARTESIAN_POINT('Ctrl Pts',(-14.7728141849366,12.4018104241151,
132.733985657383)) ;
#152565=CARTESIAN_POINT('Ctrl Pts',(-14.6787517401919,12.5389586489687,
132.49253663729)) ;
#152566=CARTESIAN_POINT('Ctrl Pts',(-14.6003862698118,12.7377764458565,
132.296567507347)) ;
#152567=CARTESIAN_POINT('Ctrl Pts',(-14.5411439660413,12.9863019722805,
132.156626084833)) ;
#152568=CARTESIAN_POINT('Ctrl Pts',(-14.5050286674343,13.2660338630659,
132.084222246459)) ;
#152569=CARTESIAN_POINT('Ctrl Pts',(-14.4938897468974,13.5582232268191,
132.08492344046)) ;
#152570=CARTESIAN_POINT('Ctrl Pts',(-14.507818431321,13.8387404070693,132.158622706454)) ;
#152571=CARTESIAN_POINT('Ctrl Pts',(-14.5449327754259,14.0904925183414,
132.300141702221)) ;
#152572=CARTESIAN_POINT('Ctrl Pts',(-14.6025167026814,14.2955136011611,
132.501693163721)) ;
#152573=CARTESIAN_POINT('Ctrl Pts',(-14.6743979140284,14.4360006812449,
132.744601960421)) ;
#152574=CARTESIAN_POINT('Ctrl Pts',(-14.7560190059001,14.5051702931602,
133.016232266989)) ;
#152575=CARTESIAN_POINT('Ctrl Pts',(-14.8399788108669,14.4966323764384,
133.29455720462)) ;
#152576=CARTESIAN_POINT('Ctrl Pts',(-14.92026343514,14.4108291399258,133.562335509995)) ;
#152577=CARTESIAN_POINT('Ctrl Pts',(-14.9895377292265,14.2547209501546,
133.797763255438)) ;
#152578=CARTESIAN_POINT('Ctrl Pts',(-15.0426869064103,14.0388606089928,
133.986156454842)) ;
#152579=CARTESIAN_POINT('Ctrl Pts',(-15.0750262925721,13.779405578044,134.113692915164)) ;
#152580=CARTESIAN_POINT('Ctrl Pts',(-15.0835065338818,13.4926641580088,
134.171741504609)) ;
#152581=CARTESIAN_POINT('Ctrl Pts',(-15.0668941196817,13.2038302112353,
134.156144137311)) ;
#152582=CARTESIAN_POINT('Ctrl Pts',(-15.0254043328273,12.9280759931688,
134.068184900734)) ;
#152583=CARTESIAN_POINT('Ctrl Pts',(-14.9614251335503,12.6887447492448,
133.914424357805)) ;
#152584=CARTESIAN_POINT('Ctrl Pts',(-14.8789170489459,12.5022966343227,
133.706505074034)) ;
#152585=CARTESIAN_POINT('Ctrl Pts',(-14.7832955283864,12.381763978882,133.460180040676)) ;
#152586=CARTESIAN_POINT('Ctrl Pts',(-14.6794737714671,12.3354318114705,
133.190193795545)) ;
#152587=CARTESIAN_POINT('Ctrl Pts',(-14.5760954726489,12.3672035513488,
132.921157086038)) ;
#152588=CARTESIAN_POINT('Ctrl Pts',(-14.4781651153176,12.474426481286,132.668233520948)) ;
#152589=CARTESIAN_POINT('Ctrl Pts',(-14.3924892268079,12.6503068829769,
132.451164645272)) ;
#152590=CARTESIAN_POINT('Ctrl Pts',(-14.3248849840194,12.8812481424524,
132.28680518042)) ;
#152591=CARTESIAN_POINT('Ctrl Pts',(-14.2792429233544,13.1494231082653,
132.186430077652)) ;
#152592=CARTESIAN_POINT('Ctrl Pts',(-14.2577333010081,13.4405328283774,
132.156949660664)) ;
#152593=CARTESIAN_POINT('Ctrl Pts',(-14.2616812486159,13.7272524095848,
132.201463654968)) ;
#152594=CARTESIAN_POINT('Ctrl Pts',(-14.2897398061011,13.9933197786215,
132.316545259697)) ;
#152595=CARTESIAN_POINT('Ctrl Pts',(-14.3391869583318,14.2183989061991,
132.494053529779)) ;
#152596=CARTESIAN_POINT('Ctrl Pts',(-14.4064273444875,14.3876287517767,
132.723811096672)) ;
#152597=CARTESIAN_POINT('Ctrl Pts',(-14.4845242454382,14.4861870970875,
132.984890006035)) ;
#152598=CARTESIAN_POINT('Ctrl Pts',(-14.5685621236943,14.5095212297327,
133.263587921165)) ;
#152599=CARTESIAN_POINT('Ctrl Pts',(-14.6509971062007,14.4547287275128,
133.537507814222)) ;
#152600=CARTESIAN_POINT('Ctrl Pts',(-14.7254748058222,14.3261105544631,
133.788208742009)) ;
#152601=CARTESIAN_POINT('Ctrl Pts',(-14.7858563786915,14.1327425032557,
133.997729271496)) ;
#152602=CARTESIAN_POINT('Ctrl Pts',(-14.8271232484926,13.8885306001009,
134.151412460096)) ;
#152603=CARTESIAN_POINT('Ctrl Pts',(-14.8454990345243,13.6107524410049,
134.23824836838)) ;
#152604=CARTESIAN_POINT('Ctrl Pts',(-14.8391902936134,13.3210542583331,
134.252793238962)) ;
#152605=CARTESIAN_POINT('Ctrl Pts',(-14.8073003870615,13.0351251235983,
134.193044709195)) ;
#152606=CARTESIAN_POINT('Ctrl Pts',(-14.7526013452373,12.7816150209491,
134.066072694138)) ;
#152607=CARTESIAN_POINT('Ctrl Pts',(-14.6768446022253,12.5706518061014,
133.878035031889)) ;
#152608=CARTESIAN_POINT('Ctrl Pts',(-14.5857344899984,12.422091900903,133.644955346922)) ;
#152609=CARTESIAN_POINT('Ctrl Pts',(-14.4844870236026,12.3448083833829,
133.382365111388)) ;
#152610=CARTESIAN_POINT('Ctrl Pts',(-14.3801271179856,12.3450375607664,
133.110594842367)) ;
#152611=CARTESIAN_POINT('Ctrl Pts',(-14.2791586916205,12.4222140372622,
132.848729115977)) ;
#152612=CARTESIAN_POINT('Ctrl Pts',(-14.1879207671711,12.5713072693593,
132.615345977553)) ;
#152613=CARTESIAN_POINT('Ctrl Pts',(-14.1124789413141,12.7812068465324,
132.428068113172)) ;
#152614=CARTESIAN_POINT('Ctrl Pts',(-14.0572435650617,13.0378486801572,
132.299917089332)) ;
#152615=CARTESIAN_POINT('Ctrl Pts',(-14.0258214639467,13.3220972424203,
132.241311719484)) ;
#152616=CARTESIAN_POINT('Ctrl Pts',(-14.0195168117333,13.6116477161832,
132.255856984885)) ;
#152617=CARTESIAN_POINT('Ctrl Pts',(-14.0380429091883,13.8896343949454,
132.343170883447)) ;
#152618=CARTESIAN_POINT('Ctrl Pts',(-14.0792096341859,14.1329048293709,
132.496445041414)) ;
#152619=CARTESIAN_POINT('Ctrl Pts',(-14.139739650008,14.3266157424045,132.706473107546)) ;
#152620=CARTESIAN_POINT('Ctrl Pts',(-14.2142389199618,14.4550271923226,
132.957226742653)) ;
#152621=CARTESIAN_POINT('Ctrl Pts',(-14.2968257149156,14.5094869156272,
133.231648652557)) ;
#152622=CARTESIAN_POINT('Ctrl Pts',(-14.3803943332945,14.4863255111229,
133.508781433968)) ;
#152623=CARTESIAN_POINT('Ctrl Pts',(-14.4590295914748,14.3868080890416,
133.771682898577)) ;
#152624=CARTESIAN_POINT('Ctrl Pts',(-14.5257824357843,14.2186053771164,
133.999775534479)) ;
#152625=CARTESIAN_POINT('Ctrl Pts',(-14.5755477699378,13.9916146831158,
134.17848468615)) ;
#152626=CARTESIAN_POINT('Ctrl Pts',(-14.6033802697407,13.727139474133,134.292681268961)) ;
#152627=CARTESIAN_POINT('Ctrl Pts',(-14.6071598535866,13.437362164295,134.337061191346)) ;
#152628=CARTESIAN_POINT('Ctrl Pts',(-14.5858835306319,13.1504054531947,
134.307774902983)) ;
#152629=CARTESIAN_POINT('Ctrl Pts',(-14.5396141567361,12.8786465021209,
134.206021789804)) ;
#152630=CARTESIAN_POINT('Ctrl Pts',(-14.4723055377556,12.6500332814425,
134.042260729231)) ;
#152631=CARTESIAN_POINT('Ctrl Pts',(-14.386841995621,12.4743183897028,133.825754806519)) ;
#152632=CARTESIAN_POINT('Ctrl Pts',(-14.2885171909372,12.3668547922141,
133.571800387653)) ;
#152633=CARTESIAN_POINT('Ctrl Pts',(-14.1851936733311,12.335562941567,133.302903084124)) ;
#152634=CARTESIAN_POINT('Ctrl Pts',(-14.0817812802112,12.3817108072099,
133.033981832815)) ;
#152635=CARTESIAN_POINT('Ctrl Pts',(-13.9856777323266,12.502839824897,132.78641286331)) ;
#152636=CARTESIAN_POINT('Ctrl Pts',(-13.9030779122353,12.690351441453,132.578318888232)) ;
#152637=CARTESIAN_POINT('Ctrl Pts',(-13.8395678233593,12.9285059391321,
132.425739358382)) ;
#152638=CARTESIAN_POINT('Ctrl Pts',(-13.7979805061536,13.2046731907038,
132.337546584743)) ;
#152639=CARTESIAN_POINT('Ctrl Pts',(-13.7814999331058,13.4951333113011,
132.322515878226)) ;
#152640=CARTESIAN_POINT('Ctrl Pts',(-13.7900411291653,13.779501210584,132.380474347949)) ;
#152641=CARTESIAN_POINT('Ctrl Pts',(-13.8224120698119,14.0394108332529,
132.508163412887)) ;
#152642=CARTESIAN_POINT('Ctrl Pts',(-13.8756204987681,14.2552141196343,
132.696731438701)) ;
#152643=CARTESIAN_POINT('Ctrl Pts',(-13.9451061652378,14.4112842226695,
132.932851180889)) ;
#152644=CARTESIAN_POINT('Ctrl Pts',(-14.0249337755901,14.49663037618,133.199097915004)) ;
#152645=CARTESIAN_POINT('Ctrl Pts',(-14.1095239733355,14.5049768783044,
133.479521095915)) ;
#152646=CARTESIAN_POINT('Ctrl Pts',(-14.190528704622,14.4360835729073,133.749098498737)) ;
#152647=CARTESIAN_POINT('Ctrl Pts',(-14.262882528703,14.2946513922982,133.993611762097)) ;
#152648=CARTESIAN_POINT('Ctrl Pts',(-14.320142163076,14.0899140100411,134.194101738961)) ;
#152649=CARTESIAN_POINT('Ctrl Pts',(-14.3572698390389,13.8386917046902,
134.335604381356)) ;
#152650=CARTESIAN_POINT('Ctrl Pts',(-14.3711303129086,13.5555692125345,
134.40939671493)) ;
#152651=CARTESIAN_POINT('Ctrl Pts',(-14.3599713476779,13.2663901180779,
134.409692119641)) ;
#152652=CARTESIAN_POINT('Ctrl Pts',(-14.3238194723227,12.9858847333076,
134.337276500168)) ;
#152653=CARTESIAN_POINT('Ctrl Pts',(-14.2645948958419,12.7375102459871,
134.197360749458)) ;
#152654=CARTESIAN_POINT('Ctrl Pts',(-14.1856165305326,12.5376376287816,
133.99982702238)) ;
#152655=CARTESIAN_POINT('Ctrl Pts',(-14.0918860241884,12.4015826977934,
133.759196205742)) ;
#152656=CARTESIAN_POINT('Ctrl Pts',(-13.9900202965247,12.3390360902595,
133.494624163606)) ;
#152657=CARTESIAN_POINT('Ctrl Pts',(-13.885715431319,12.353575403094,133.223035536617)) ;
#152658=CARTESIAN_POINT('Ctrl Pts',(-13.7857334521546,12.445274073871,132.964183894283)) ;
#152659=CARTESIAN_POINT('Ctrl Pts',(-13.6971224342536,12.6067971683827,
132.738446959323)) ;
#152660=CARTESIAN_POINT('Ctrl Pts',(-13.6250522220287,12.8274892534517,
132.561122252927)) ;
#152661=CARTESIAN_POINT('Ctrl Pts',(-13.5744828714336,13.0891408927057,
132.446378055787)) ;
#152662=CARTESIAN_POINT('Ctrl Pts',(-13.547610803124,13.375740122579,132.401005590542)) ;
#152663=CARTESIAN_POINT('Ctrl Pts',(-13.5460300274622,13.6659116032671,
132.429533614848)) ;
#152664=CARTESIAN_POINT('Ctrl Pts',(-13.5689788396593,13.9383430672958,
132.529666742918)) ;
#152665=CARTESIAN_POINT('Ctrl Pts',(-13.6144336268274,14.1747318786697,
132.695698796106)) ;
#152666=CARTESIAN_POINT('Ctrl Pts',(-13.6775346028895,14.3556000224366,
132.912954043635)) ;
#152667=CARTESIAN_POINT('Ctrl Pts',(-13.7545609195232,14.4715471852787,
133.171333891809)) ;
#152668=CARTESIAN_POINT('Ctrl Pts',(-13.8375768659038,14.5109306884899,
133.446859569505)) ;
#152669=CARTESIAN_POINT('Ctrl Pts',(-13.9206587334674,14.4734197510009,
133.722575921601)) ;
#152670=CARTESIAN_POINT('Ctrl Pts',(-13.9978549774587,14.3595613312843,
133.981405064546)) ;
#152671=CARTESIAN_POINT('Ctrl Pts',(-14.0615326101247,14.179466171533,134.200463448237)) ;
#152672=CARTESIAN_POINT('Ctrl Pts',(-14.1072808462681,13.9455181185487,
134.367173049305)) ;
#152673=CARTESIAN_POINT('Ctrl Pts',(-14.1309695714097,13.6723045745694,
134.469654422256)) ;
#152674=CARTESIAN_POINT('Ctrl Pts',(-14.1299543421008,13.3834915874396,
134.49969517271)) ;
#152675=CARTESIAN_POINT('Ctrl Pts',(-14.103826459953,13.0966134068724,134.456484806691)) ;
#152676=CARTESIAN_POINT('Ctrl Pts',(-14.0536044519402,12.8330521051259,
134.342891801889)) ;
#152677=CARTESIAN_POINT('Ctrl Pts',(-13.9819755458689,12.6112324338377,
134.166849542491)) ;
#152678=CARTESIAN_POINT('Ctrl Pts',(-13.8936140788126,12.4482429025448,
133.941863276773)) ;
#152679=CARTESIAN_POINT('Ctrl Pts',(-13.7945442209898,12.3553252392396,
133.68544189025)) ;
#152680=CARTESIAN_POINT('Ctrl Pts',(-13.6902421881023,12.3382107107946,
133.413874998198)) ;
#152681=CARTESIAN_POINT('Ctrl Pts',(-13.5876395250276,12.3992481458877,
133.147344273434)) ;
#152682=CARTESIAN_POINT('Ctrl Pts',(-13.4940363967205,12.5331204758664,
132.906945186053)) ;
#152683=CARTESIAN_POINT('Ctrl Pts',(-13.4146406339235,12.7309387918669,
132.708143521826)) ;
#152684=CARTESIAN_POINT('Ctrl Pts',(-13.3546400489765,12.9791524410526,
132.566084041094)) ;
#152685=CARTESIAN_POINT('Ctrl Pts',(-13.3178749195276,13.2585790598106,
132.491812795079)) ;
#152686=CARTESIAN_POINT('Ctrl Pts',(-13.3060921658157,13.5499397896395,
132.490544550928)) ;
#152687=CARTESIAN_POINT('Ctrl Pts',(-13.319267039209,13.8311712407388,132.562048975874)) ;
#152688=CARTESIAN_POINT('Ctrl Pts',(-13.3560394645477,14.0848085651835,
132.702709571436)) ;
#152689=CARTESIAN_POINT('Ctrl Pts',(-13.4124077844404,14.2892041446737,
132.900320701676)) ;
#152690=CARTESIAN_POINT('Ctrl Pts',(-13.4844837717321,14.4332159069687,
133.144089592404)) ;
#152691=CARTESIAN_POINT('Ctrl Pts',(-13.5657740695195,14.5042073782218,
133.414672215616)) ;
#152692=CARTESIAN_POINT('Ctrl Pts',(-13.6499188668072,14.4978850554144,
133.693611525571)) ;
#152693=CARTESIAN_POINT('Ctrl Pts',(-13.7301300690243,14.4145534025925,
133.96105201458)) ;
#152694=CARTESIAN_POINT('Ctrl Pts',(-13.7999841881705,14.2600830965558,
134.198257775645)) ;
#152695=CARTESIAN_POINT('Ctrl Pts',(-13.8535974701144,14.0459659620245,
134.387963859614)) ;
#152696=CARTESIAN_POINT('Ctrl Pts',(-13.8866069561238,13.7875807752627,
134.517459877776)) ;
#152697=CARTESIAN_POINT('Ctrl Pts',(-13.8958448391708,13.5015008973902,
134.577698082975)) ;
#152698=CARTESIAN_POINT('Ctrl Pts',(-13.8799187621032,13.2119712102584,
134.564171528529)) ;
#152699=CARTESIAN_POINT('Ctrl Pts',(-13.8392809382772,12.9363053782512,
134.478593815727)) ;
#152700=CARTESIAN_POINT('Ctrl Pts',(-13.7758444278724,12.6952736602129,
134.326473645072)) ;
#152701=CARTESIAN_POINT('Ctrl Pts',(-13.6940162958856,12.507125678723,134.120477732686)) ;
#152702=CARTESIAN_POINT('Ctrl Pts',(-13.5977907900013,12.3837628513247,
133.872694312529)) ;
#152703=CARTESIAN_POINT('Ctrl Pts',(-13.4952077550757,12.3357954087756,
133.605958381013)) ;
#152704=CARTESIAN_POINT('Ctrl Pts',(-13.3909244959306,12.3652711251859,
133.33454614811)) ;
#152705=CARTESIAN_POINT('Ctrl Pts',(-13.2930291637441,12.4705156806676,
133.081632751708)) ;
#152706=CARTESIAN_POINT('Ctrl Pts',(-13.2071658759881,12.6439184973371,
132.863918116231)) ;
#152707=CARTESIAN_POINT('Ctrl Pts',(-13.1389101581012,12.8730354055636,
132.697626362)) ;
#152708=CARTESIAN_POINT('Ctrl Pts',(-13.0923226075365,13.1424159445997,
132.594737929481)) ;
#152709=CARTESIAN_POINT('Ctrl Pts',(-13.0702865542668,13.4306391754528,
132.563415021775)) ;
#152710=CARTESIAN_POINT('Ctrl Pts',(-13.0733966131089,13.7191539441457,
132.605650335791)) ;
#152711=CARTESIAN_POINT('Ctrl Pts',(-13.1008205861734,13.9861293896989,
132.718874470187)) ;
#152712=CARTESIAN_POINT('Ctrl Pts',(-13.1498037441585,14.2128684001206,
132.89508138218)) ;
#152713=CARTESIAN_POINT('Ctrl Pts',(-13.2163126321001,14.3833347965248,
133.122557153896)) ;
#152714=CARTESIAN_POINT('Ctrl Pts',(-13.2945517934649,14.4845639099252,
133.384224457738)) ;
#152715=CARTESIAN_POINT('Ctrl Pts',(-13.3782996834148,14.5099092471542,
133.66197841254)) ;
#152716=CARTESIAN_POINT('Ctrl Pts',(-13.4610067103196,14.4573341215463,
133.936748595732)) ;
#152717=CARTESIAN_POINT('Ctrl Pts',(-13.535792979438,14.3305258270945,134.188357582262)) ;
#152718=CARTESIAN_POINT('Ctrl Pts',(-13.5964938791261,14.1393930806654,
134.398720829303)) ;
#152719=CARTESIAN_POINT('Ctrl Pts',(-13.6384531516596,13.8963012865058,
134.554456038958)) ;
#152720=CARTESIAN_POINT('Ctrl Pts',(-13.6575588644819,13.618527952916,134.64350061979)) ;
#152721=CARTESIAN_POINT('Ctrl Pts',(-13.6518640795297,13.3290638567204,
134.659826711564)) ;
#152722=CARTESIAN_POINT('Ctrl Pts',(-13.6210222993908,13.0445549081066,
134.602903919085)) ;
#152723=CARTESIAN_POINT('Ctrl Pts',(-13.5665781809899,12.7876683953407,
134.476958833009)) ;
#152724=CARTESIAN_POINT('Ctrl Pts',(-13.4911864112069,12.5753843248543,
134.290002560966)) ;
#152725=CARTESIAN_POINT('Ctrl Pts',(-13.4007901006825,12.4255194566962,
134.05888370733)) ;
#152726=CARTESIAN_POINT('Ctrl Pts',(-13.2997237377735,12.3459765628223,
133.796830310285)) ;
#152727=CARTESIAN_POINT('Ctrl Pts',(-13.1954991747945,12.3439073333341,
133.52541389548)) ;
#152728=CARTESIAN_POINT('Ctrl Pts',(-13.0941541677024,12.4188279963137,
133.262499854551)) ;
#152729=CARTESIAN_POINT('Ctrl Pts',(-13.002205997662,12.5669347456838,133.027188569075)) ;
#152730=CARTESIAN_POINT('Ctrl Pts',(-12.9267422753913,12.7740276750078,
132.839635132885)) ;
#152731=CARTESIAN_POINT('Ctrl Pts',(-12.8706659445136,13.0302839963835,
132.709131418789)) ;
#152732=CARTESIAN_POINT('Ctrl Pts',(-12.8386183811773,13.3133908418281,
132.648618515674)) ;
#152733=CARTESIAN_POINT('Ctrl Pts',(-12.8315791622469,13.603463644202,132.661074904967)) ;
#152734=CARTESIAN_POINT('Ctrl Pts',(-12.8492844367411,13.8813033828735,
132.745878981524)) ;
#152735=CARTESIAN_POINT('Ctrl Pts',(-12.8901906349179,14.1277803353935,
132.898667421918)) ;
#152736=CARTESIAN_POINT('Ctrl Pts',(-12.9502027043241,14.3222499491186,
133.107092668811)) ;
#152737=CARTESIAN_POINT('Ctrl Pts',(-13.0241102247799,14.4521801137134,
133.356004116762)) ;
#152738=CARTESIAN_POINT('Ctrl Pts',(-13.1064456796044,14.5090397013049,
133.629648846685)) ;
#152739=CARTESIAN_POINT('Ctrl Pts',(-13.1904091031337,14.4879536383768,
133.908074847443)) ;
#152740=CARTESIAN_POINT('Ctrl Pts',(-13.2691730073198,14.3907169193799,
134.171290632638)) ;
#152741=CARTESIAN_POINT('Ctrl Pts',(-13.3365717682159,14.2230874926912,
134.401446847104)) ;
#152742=CARTESIAN_POINT('Ctrl Pts',(-13.3862837725614,14.0008521290395,
134.579526433076)) ;
#152743=CARTESIAN_POINT('Ctrl Pts',(-13.4151850077251,13.7343152663338,
134.697246128251)) ;
#152744=CARTESIAN_POINT('Ctrl Pts',(-13.4196674461843,13.4474451530714,
134.74336669151)) ;
#152745=CARTESIAN_POINT('Ctrl Pts',(-13.3989374427175,13.1575373599845,
134.716000021385)) ;
#152746=CARTESIAN_POINT('Ctrl Pts',(-13.3538701206744,12.8878586186382,
134.617383543723)) ;
#152747=CARTESIAN_POINT('Ctrl Pts',(-13.2866697814604,12.6555337160297,
134.454240239388)) ;
#152748=CARTESIAN_POINT('Ctrl Pts',(-13.2016717965965,12.4784852863875,
134.239051541609)) ;
#152749=CARTESIAN_POINT('Ctrl Pts',(-13.103660140851,12.3688435126028,133.986006271584)) ;
#152750=CARTESIAN_POINT('Ctrl Pts',(-13.0001912147535,12.335379050582,133.716752546929)) ;
#152751=CARTESIAN_POINT('Ctrl Pts',(-12.8968764365744,12.3794309050292,
133.448054757706)) ;
#152752=CARTESIAN_POINT('Ctrl Pts',(-12.8007211226384,12.4979553005814,
133.200237570607)) ;
#152753=CARTESIAN_POINT('Ctrl Pts',(-12.7173411751848,12.6843641512771,
132.989987119788)) ;
#152754=CARTESIAN_POINT('Ctrl Pts',(-12.6533675978781,12.9208195190715,
132.835987884663)) ;
#152755=CARTESIAN_POINT('Ctrl Pts',(-12.6110523141971,13.1965599156971,
132.745711948575)) ;
#152756=CARTESIAN_POINT('Ctrl Pts',(-12.5938677361115,13.4854150034454,
132.728459041513)) ;
#152757=CARTESIAN_POINT('Ctrl Pts',(-12.6016166796287,13.7715245103546,
132.784247690811)) ;
#152758=CARTESIAN_POINT('Ctrl Pts',(-12.6334808333027,14.0329603333754,
132.910531351478)) ;
#152759=CARTESIAN_POINT('Ctrl Pts',(-12.6860159227242,14.2495174070446,
133.097035811552)) ;
#152760=CARTESIAN_POINT('Ctrl Pts',(-12.7550120282424,14.4077221355952,
133.331704202413)) ;
#152761=CARTESIAN_POINT('Ctrl Pts',(-12.8352852858367,14.4954974794661,
133.599515576589)) ;
#152762=CARTESIAN_POINT('Ctrl Pts',(-12.9190639071468,14.5058124227374,
133.877251814252)) ;
#152763=CARTESIAN_POINT('Ctrl Pts',(-13.0006861903333,14.4390540160987,
134.148810770118)) ;
#152764=CARTESIAN_POINT('Ctrl Pts',(-13.0734798970183,14.2988995016989,
134.394674718231)) ;
#152765=CARTESIAN_POINT('Ctrl Pts',(-13.1310605574008,14.0959846822767,
134.59603545551)) ;
#152766=CARTESIAN_POINT('Ctrl Pts',(-13.1686602075177,13.8467238077785,
134.738805253809)) ;
#152767=CARTESIAN_POINT('Ctrl Pts',(-13.1832960063071,13.5651499595772,
134.814759605636)) ;
#152768=CARTESIAN_POINT('Ctrl Pts',(-13.1728859358929,13.2745210705863,
134.817404454761)) ;
#152769=CARTESIAN_POINT('Ctrl Pts',(-13.1372979957402,12.9930481847516,
134.746685223495)) ;
#152770=CARTESIAN_POINT('Ctrl Pts',(-13.0788464460579,12.7442685275202,
134.608933005347)) ;
#152771=CARTESIAN_POINT('Ctrl Pts',(-13.0004860021476,12.5428869624623,
134.413170014133)) ;
#152772=CARTESIAN_POINT('Ctrl Pts',(-12.9071846487547,12.4047083280592,
134.173773807101)) ;
#152773=CARTESIAN_POINT('Ctrl Pts',(-12.8051561028839,12.3396945526809,
133.90883173255)) ;
#152774=CARTESIAN_POINT('Ctrl Pts',(-12.7008909970313,12.3521469576885,
133.637337257152)) ;
#152775=CARTESIAN_POINT('Ctrl Pts',(-12.6009173642389,12.441314353945,133.378426035197)) ;
#152776=CARTESIAN_POINT('Ctrl Pts',(-12.5117677396135,12.6011043288198,
133.151163527727)) ;
#152777=CARTESIAN_POINT('Ctrl Pts',(-12.4393294114449,12.8194224397463,
132.97265105268)) ;
#152778=CARTESIAN_POINT('Ctrl Pts',(-12.387790426931,13.0811434342732,132.85522288076)) ;
#152779=CARTESIAN_POINT('Ctrl Pts',(-12.360228261411,13.3679217852881,132.807894792067)) ;
#152780=CARTESIAN_POINT('Ctrl Pts',(-12.3579523050129,13.6574454003315,
132.834298017918)) ;
#152781=CARTESIAN_POINT('Ctrl Pts',(-12.3801380175334,13.9304218890574,
132.932167779584)) ;
#152782=CARTESIAN_POINT('Ctrl Pts',(-12.4250230602689,14.1686008595605,
133.096583317216)) ;
#152783=CARTESIAN_POINT('Ctrl Pts',(-12.4878388913045,14.3514046814191,
133.313074404504)) ;
#152784=CARTESIAN_POINT('Ctrl Pts',(-12.5640867721586,14.4688537010489,
133.568976881112)) ;
#152785=CARTESIAN_POINT('Ctrl Pts',(-12.6473280614042,14.5110084065472,
133.845298914204)) ;
#152786=CARTESIAN_POINT('Ctrl Pts',(-12.7306234368668,14.4754271659884,
134.121689851781)) ;
#152787=CARTESIAN_POINT('Ctrl Pts',(-12.8078424891508,14.3641624802179,
134.38046802569)) ;
#152788=CARTESIAN_POINT('Ctrl Pts',(-12.8722362238059,14.1852632695012,
134.601742519835)) ;
#152789=CARTESIAN_POINT('Ctrl Pts',(-12.9184596429682,13.9526451401233,
134.769816657982)) ;
#152790=CARTESIAN_POINT('Ctrl Pts',(-12.9427606566985,13.6818447118076,
134.873904342633)) ;
#152791=CARTESIAN_POINT('Ctrl Pts',(-12.9426329031674,13.3926206452482,
134.906615051885)) ;
#152792=CARTESIAN_POINT('Ctrl Pts',(-12.9170454040847,13.1038754923078,
134.865156068369)) ;
#152793=CARTESIAN_POINT('Ctrl Pts',(-12.8675913433402,12.8403836297391,
134.753690916011)) ;
#152794=CARTESIAN_POINT('Ctrl Pts',(-12.7967823441445,12.6175434576375,
134.579955954179)) ;
#152795=CARTESIAN_POINT('Ctrl Pts',(-12.70868276548,12.4520178789147,134.355810149669)) ;
#152796=CARTESIAN_POINT('Ctrl Pts',(-12.6093449823904,12.3567780608222,
134.098765452035)) ;
#152797=CARTESIAN_POINT('Ctrl Pts',(-12.5056341234011,12.3376561109864,
133.828749759816)) ;
#152798=CARTESIAN_POINT('Ctrl Pts',(-12.402751079868,12.3963494804203,133.561441007829)) ;
#152799=CARTESIAN_POINT('Ctrl Pts',(-12.3088084112223,12.5282529228556,
133.320050046839)) ;
#152800=CARTESIAN_POINT('Ctrl Pts',(-12.2289334019483,12.7243873042916,
133.119846376778)) ;
#152801=CARTESIAN_POINT('Ctrl Pts',(-12.1683661165357,12.9708923918956,
132.976071926915)) ;
#152802=CARTESIAN_POINT('Ctrl Pts',(-12.1308341182304,13.2502126197918,
132.899629391339)) ;
#152803=CARTESIAN_POINT('Ctrl Pts',(-12.1182778756421,13.5400583828972,
132.895929792219)) ;
#152804=CARTESIAN_POINT('Ctrl Pts',(-12.1307869570981,13.8239338286533,
132.965735493257)) ;
#152805=CARTESIAN_POINT('Ctrl Pts',(-12.1668484142908,14.0777676729547,
133.104202368024)) ;
#152806=CARTESIAN_POINT('Ctrl Pts',(-12.222772912384,14.2841378500946,133.300577303525)) ;
#152807=CARTESIAN_POINT('Ctrl Pts',(-12.2942910489215,14.429815657766,133.542627629611)) ;
#152808=CARTESIAN_POINT('Ctrl Pts',(-12.3756729115768,14.5033259168077,
133.813595342621)) ;
#152809=CARTESIAN_POINT('Ctrl Pts',(-12.4597832810724,14.499135115111,134.092410952893)) ;
#152810=CARTESIAN_POINT('Ctrl Pts',(-12.5402566051309,14.4177798325381,
134.360648411857)) ;
#152811=CARTESIAN_POINT('Ctrl Pts',(-12.6102648440973,14.2657377102023,
134.59819459311)) ;
#152812=CARTESIAN_POINT('Ctrl Pts',(-12.6646057115603,14.0527574173429,
134.790109616224)) ;
#152813=CARTESIAN_POINT('Ctrl Pts',(-12.6982822917971,13.7942044324148,
134.921686113269)) ;
#152814=CARTESIAN_POINT('Ctrl Pts',(-12.7081236290535,13.509972220369,134.983521067054)) ;
#152815=CARTESIAN_POINT('Ctrl Pts',(-12.6929226435767,13.219834764377,134.972169824304)) ;
#152816=CARTESIAN_POINT('Ctrl Pts',(-12.6529041959642,12.9433154987134,
134.888419817773)) ;
#152817=CARTESIAN_POINT('Ctrl Pts',(-12.5899125810331,12.7008042356819,
134.737648548155)) ;
#152818=CARTESIAN_POINT('Ctrl Pts',(-12.5088132067507,12.5118988342583,
134.533656568728)) ;
#152819=CARTESIAN_POINT('Ctrl Pts',(-12.4134247671775,12.3867144480253,
134.288156510762)) ;
#152820=CARTESIAN_POINT('Ctrl Pts',(-12.3103723850424,12.3359851161897,
134.020244487105)) ;
#152821=CARTESIAN_POINT('Ctrl Pts',(-12.2060535029749,12.3634203970633,
133.748717660543)) ;
#152822=CARTESIAN_POINT('Ctrl Pts',(-12.1079177935451,12.4663876358086,
133.495088507556)) ;
#152823=CARTESIAN_POINT('Ctrl Pts',(-12.0212873996097,12.6389701182042,
133.275282296474)) ;
#152824=CARTESIAN_POINT('Ctrl Pts',(-11.9528459850857,12.8657474577828,
133.108290126159)) ;
#152825=CARTESIAN_POINT('Ctrl Pts',(-11.9054705654115,13.1346343436699,
133.003152675926)) ;
#152826=CARTESIAN_POINT('Ctrl Pts',(-11.8903642795437,13.3266512177486,
132.98106317886)) ;
#152827=CARTESIAN_POINT('Ctrl Pts',(-11.8869647971046,13.4226801736581,
132.982153164817)) ;
#152828=CARTESIAN_POINT('',(-33.3489959095147,13.1551399285885,127.871927411069)) ;
#152829=CARTESIAN_POINT('',(-22.6320187065114,12.9778651918053,131.474336592418)) ;
#152830=CARTESIAN_POINT('Ctrl Pts',(-33.3489959095147,13.1551399285885,
127.871927411069)) ;
#152831=CARTESIAN_POINT('Ctrl Pts',(-33.3482570091173,13.1489709609094,
127.870499856875)) ;
#152832=CARTESIAN_POINT('Ctrl Pts',(-33.3362031847492,13.0505878441039,
127.846970056077)) ;
#152833=CARTESIAN_POINT('Ctrl Pts',(-33.303456104594,12.8648900473044,127.774282508598)) ;
#152834=CARTESIAN_POINT('Ctrl Pts',(-33.2347176391245,12.6378996894465,
127.606502631126)) ;
#152835=CARTESIAN_POINT('Ctrl Pts',(-33.1484631699894,12.4661938442505,
127.38763758675)) ;
#152836=CARTESIAN_POINT('Ctrl Pts',(-33.0496339239794,12.3629468779938,
127.132205946451)) ;
#152837=CARTESIAN_POINT('Ctrl Pts',(-32.9461836982222,12.3360866578135,
126.862930995212)) ;
#152838=CARTESIAN_POINT('Ctrl Pts',(-32.8428524780797,12.3868467815327,
126.594300512203)) ;
#152839=CARTESIAN_POINT('Ctrl Pts',(-32.7476240151848,12.5118616193735,
126.34920621096)) ;
#152840=CARTESIAN_POINT('Ctrl Pts',(-32.6660393235339,12.7022376314793,
126.14402042184)) ;
#152841=CARTESIAN_POINT('Ctrl Pts',(-32.6034202579729,12.9442211340136,
125.994217779495)) ;
#152842=CARTESIAN_POINT('Ctrl Pts',(-32.5634889320909,13.2203922331636,
125.91068247448)) ;
#152843=CARTESIAN_POINT('Ctrl Pts',(-32.5482836171183,13.5109001041669,
125.899354456419)) ;
#152844=CARTESIAN_POINT('Ctrl Pts',(-32.5583885908025,13.7967277450532,
125.962163306551)) ;
#152845=CARTESIAN_POINT('Ctrl Pts',(-32.5919970185865,14.0531634695327,
126.093303648423)) ;
#152846=CARTESIAN_POINT('Ctrl Pts',(-32.6462352627175,14.2659161102292,
126.2848763833)) ;
#152847=CARTESIAN_POINT('Ctrl Pts',(-32.7164440425069,14.4182155312585,
126.52308858485)) ;
#152848=CARTESIAN_POINT('Ctrl Pts',(-32.7970929244734,14.4993926065239,
126.791896512519)) ;
#152849=CARTESIAN_POINT('Ctrl Pts',(-32.8812312900771,14.5030674016304,
127.070805593369)) ;
#152850=CARTESIAN_POINT('Ctrl Pts',(-32.9621947752627,14.4296658181567,
127.340390412531)) ;
#152851=CARTESIAN_POINT('Ctrl Pts',(-33.0336799536047,14.2842405620309,
127.582320067705)) ;
#152852=CARTESIAN_POINT('Ctrl Pts',(-33.0898518257578,14.0768885755418,
127.779563482544)) ;
#152853=CARTESIAN_POINT('Ctrl Pts',(-33.1258131095785,13.821937566696,127.917839903426)) ;
#152854=CARTESIAN_POINT('Ctrl Pts',(-33.1381603359796,13.5404397832619,
127.986888146398)) ;
#152855=CARTESIAN_POINT('Ctrl Pts',(-33.1255862370588,13.2491903771815,
127.98329800545)) ;
#152856=CARTESIAN_POINT('Ctrl Pts',(-33.0878760919221,12.9699188880577,
127.906345203758)) ;
#152857=CARTESIAN_POINT('Ctrl Pts',(-33.0275630545352,12.7245502986717,
127.763166970814)) ;
#152858=CARTESIAN_POINT('Ctrl Pts',(-32.9475449968705,12.5279694687298,
127.562611942766)) ;
#152859=CARTESIAN_POINT('Ctrl Pts',(-32.853484832887,12.3961377043517,127.320906369453)) ;
#152860=CARTESIAN_POINT('Ctrl Pts',(-32.7506275244767,12.3376103677892,
127.053662058531)) ;
#152861=CARTESIAN_POINT('Ctrl Pts',(-32.6467508382538,12.3569098529355,
126.783214181605)) ;
#152862=CARTESIAN_POINT('Ctrl Pts',(-32.5472606088073,12.452769019898,126.525790390631)) ;
#152863=CARTESIAN_POINT('Ctrl Pts',(-32.4595735399336,12.6179593573441,
126.30272348908)) ;
#152864=CARTESIAN_POINT('Ctrl Pts',(-32.388745121808,12.8405880377693,126.12891456918)) ;
#152865=CARTESIAN_POINT('Ctrl Pts',(-32.3390681420419,13.1065246421439,
126.017073858121)) ;
#152866=CARTESIAN_POINT('Ctrl Pts',(-32.313898204756,13.3925179674891,125.976505647384)) ;
#152867=CARTESIAN_POINT('Ctrl Pts',(-32.3136699242009,13.6819916651313,
126.008953177836)) ;
#152868=CARTESIAN_POINT('Ctrl Pts',(-32.3381285657715,13.9537242418059,
126.113619428421)) ;
#152869=CARTESIAN_POINT('Ctrl Pts',(-32.384536696511,14.1863734291659,126.28227784121)) ;
#152870=CARTESIAN_POINT('Ctrl Pts',(-32.4487957222161,14.3643807985693,
126.503053049914)) ;
#152871=CARTESIAN_POINT('Ctrl Pts',(-32.5258074280907,14.4754559850244,
126.761140801679)) ;
#152872=CARTESIAN_POINT('Ctrl Pts',(-32.6094667487868,14.5110246739577,
127.038737149779)) ;
#152873=CARTESIAN_POINT('Ctrl Pts',(-32.6924145513944,14.4687063588107,
127.314091355005)) ;
#152874=CARTESIAN_POINT('Ctrl Pts',(-32.7687110106265,14.3514018815055,
127.570143149353)) ;
#152875=CARTESIAN_POINT('Ctrl Pts',(-32.8317732094795,14.1671964752596,
127.787539429963)) ;
#152876=CARTESIAN_POINT('Ctrl Pts',(-32.8762267217076,13.9308608041133,
127.950416591701)) ;
#152877=CARTESIAN_POINT('Ctrl Pts',(-32.8985780094168,13.6570089999716,
128.048890973466)) ;
#152878=CARTESIAN_POINT('Ctrl Pts',(-32.896157678737,13.3664659574419,128.074980037028)) ;
#152879=CARTESIAN_POINT('Ctrl Pts',(-32.8685548522265,13.0805681472547,
128.027442701697)) ;
#152880=CARTESIAN_POINT('Ctrl Pts',(-32.8170821736547,12.8190539470386,
127.91017574478)) ;
#152881=CARTESIAN_POINT('Ctrl Pts',(-32.7441829163896,12.5999338423892,
127.73048258649)) ;
#152882=CARTESIAN_POINT('Ctrl Pts',(-32.6555170250936,12.4413957528131,
127.504429482033)) ;
#152883=CARTESIAN_POINT('Ctrl Pts',(-32.5554705400289,12.3520378265489,
127.245337069314)) ;
#152884=CARTESIAN_POINT('Ctrl Pts',(-32.4511053019089,12.339734386482,126.973578302647)) ;
#152885=CARTESIAN_POINT('Ctrl Pts',(-32.3490815539954,12.4049383167358,
126.708653969777)) ;
#152886=CARTESIAN_POINT('Ctrl Pts',(-32.2559652828001,12.5429634979505,
126.469740198936)) ;
#152887=CARTESIAN_POINT('Ctrl Pts',(-32.1775406776191,12.7443553986761,
126.273802702315)) ;
#152888=CARTESIAN_POINT('Ctrl Pts',(-32.1189511785612,12.9943521537239,
126.135786155147)) ;
#152889=CARTESIAN_POINT('Ctrl Pts',(-32.0836266547703,13.2741647768729,
126.065632995122)) ;
#152890=CARTESIAN_POINT('Ctrl Pts',(-32.0731422430725,13.565720269456,126.068169777388)) ;
#152891=CARTESIAN_POINT('Ctrl Pts',(-32.0878672761987,13.8474315556546,
126.144404645481)) ;
#152892=CARTESIAN_POINT('Ctrl Pts',(-32.1256175280986,14.0971649669908,
126.287692127083)) ;
#152893=CARTESIAN_POINT('Ctrl Pts',(-32.1834742057281,14.3002122843455,
126.489943063825)) ;
#152894=CARTESIAN_POINT('Ctrl Pts',(-32.2561937622249,14.4394509674979,
126.73551422792)) ;
#152895=CARTESIAN_POINT('Ctrl Pts',(-32.3374471159419,14.5058688200503,
127.005843081603)) ;
#152896=CARTESIAN_POINT('Ctrl Pts',(-32.4217002826958,14.4952594831202,
127.285155611484)) ;
#152897=CARTESIAN_POINT('Ctrl Pts',(-32.5017471426193,14.4071576912799,
127.552229665334)) ;
#152898=CARTESIAN_POINT('Ctrl Pts',(-32.5706761898774,14.2488070341169,
127.786694114575)) ;
#152899=CARTESIAN_POINT('Ctrl Pts',(-32.6230717724866,14.032332595662,127.972746797191)) ;
#152900=CARTESIAN_POINT('Ctrl Pts',(-32.6548239115267,13.7715185673777,
128.098623777025)) ;
#152901=CARTESIAN_POINT('Ctrl Pts',(-32.6626680714647,13.4849968555095,
128.154735100321)) ;
#152902=CARTESIAN_POINT('Ctrl Pts',(-32.6450616243189,13.1936954317484,
128.136543946875)) ;
#152903=CARTESIAN_POINT('Ctrl Pts',(-32.6032602463952,12.9217410981826,
128.047311789015)) ;
#152904=CARTESIAN_POINT('Ctrl Pts',(-32.5386314820962,12.6826993167214,
127.891757560495)) ;
#152905=CARTESIAN_POINT('Ctrl Pts',(-32.4554412889622,12.4976839220085,
127.681914464153)) ;
#152906=CARTESIAN_POINT('Ctrl Pts',(-32.3596753952525,12.3794711428103,
127.435114332308)) ;
#152907=CARTESIAN_POINT('Ctrl Pts',(-32.2558253838943,12.3351744196322,
127.165019558565)) ;
#152908=CARTESIAN_POINT('Ctrl Pts',(-32.1520107530796,12.3695012763354,
126.894875973638)) ;
#152909=CARTESIAN_POINT('Ctrl Pts',(-32.0548036090535,12.4786183736045,
126.643923371603)) ;
#152910=CARTESIAN_POINT('Ctrl Pts',(-31.9697179472944,12.6556201701116,
126.428500311369)) ;
#152911=CARTESIAN_POINT('Ctrl Pts',(-31.9024466959007,12.8885376957079,
126.26521267139)) ;
#152912=CARTESIAN_POINT('Ctrl Pts',(-31.8574815700017,13.1578672277872,
126.166847085394)) ;
#152913=CARTESIAN_POINT('Ctrl Pts',(-31.8367167778053,13.4488181058444,
126.139492583638)) ;
#152914=CARTESIAN_POINT('Ctrl Pts',(-31.8414313820349,13.7357351250712,
126.186316118843)) ;
#152915=CARTESIAN_POINT('Ctrl Pts',(-31.8700151821842,14.0000244154435,
126.30281009704)) ;
#152916=CARTESIAN_POINT('Ctrl Pts',(-31.9203616130848,14.2248063693443,
126.483142763909)) ;
#152917=CARTESIAN_POINT('Ctrl Pts',(-31.9873859775564,14.3907221531774,
126.711954484493)) ;
#152918=CARTESIAN_POINT('Ctrl Pts',(-32.0662309963865,14.4880878052934,
126.975454295977)) ;
#152919=CARTESIAN_POINT('Ctrl Pts',(-32.1500140049146,14.5090844515927,
127.253273584441)) ;
#152920=CARTESIAN_POINT('Ctrl Pts',(-32.2328114906108,14.4517331277302,
127.528461364111)) ;
#152921=CARTESIAN_POINT('Ctrl Pts',(-32.306599429151,14.3213873494252,127.777000865602)) ;
#152922=CARTESIAN_POINT('Ctrl Pts',(-32.3665410586647,14.1266126254878,
127.985228303146)) ;
#152923=CARTESIAN_POINT('Ctrl Pts',(-32.4072983071001,13.8801113803002,
128.137553257528)) ;
#152924=CARTESIAN_POINT('Ctrl Pts',(-32.4248919159062,13.6025840232108,
128.221986639911)) ;
#152925=CARTESIAN_POINT('Ctrl Pts',(-32.4177985341224,13.3122088978665,
128.234314532032)) ;
#152926=CARTESIAN_POINT('Ctrl Pts',(-32.3854612722872,13.0284665595888,
128.173051822567)) ;
#152927=CARTESIAN_POINT('Ctrl Pts',(-32.3297158719588,12.7739765033465,
128.043289524966)) ;
#152928=CARTESIAN_POINT('Ctrl Pts',(-32.2536312710535,12.5655228915478,
127.854171141032)) ;
#152929=CARTESIAN_POINT('Ctrl Pts',(-32.1621333883639,12.4188418488155,
127.619973715704)) ;
#152930=CARTESIAN_POINT('Ctrl Pts',(-32.0610335191924,12.3438198182334,
127.357704488195)) ;
#152931=CARTESIAN_POINT('Ctrl Pts',(-31.9562422849269,12.3461749880073,
127.084814084959)) ;
#152932=CARTESIAN_POINT('Ctrl Pts',(-31.8555595514267,12.4256199459212,
126.823755799531)) ;
#152933=CARTESIAN_POINT('Ctrl Pts',(-31.7646812381954,12.5766359900473,
126.591428395529)) ;
#152934=CARTESIAN_POINT('Ctrl Pts',(-31.6897549709183,12.7882864475543,
126.405673808487)) ;
#152935=CARTESIAN_POINT('Ctrl Pts',(-31.6353440859288,13.0452019382586,
126.279829886042)) ;
#152936=CARTESIAN_POINT('Ctrl Pts',(-31.6045551307125,13.3293877258915,
126.223017390213)) ;
#152937=CARTESIAN_POINT('Ctrl Pts',(-31.598929994185,13.6204035856812,126.239726726341)) ;
#152938=CARTESIAN_POINT('Ctrl Pts',(-31.6181519561243,13.8971496153171,
126.329008321255)) ;
#152939=CARTESIAN_POINT('Ctrl Pts',(-31.660032440097,14.1397539052331,126.4844492787)) ;
#152940=CARTESIAN_POINT('Ctrl Pts',(-31.7210074180807,14.3313464702874,
126.695729086547)) ;
#152941=CARTESIAN_POINT('Ctrl Pts',(-31.7956413070931,14.4574458616527,
126.94680082343)) ;
#152942=CARTESIAN_POINT('Ctrl Pts',(-31.8782525153513,14.5099723944026,
127.221254124399)) ;
#152943=CARTESIAN_POINT('Ctrl Pts',(-31.9622607746967,14.4843439695083,
127.499872427198)) ;
#152944=CARTESIAN_POINT('Ctrl Pts',(-32.0404152099778,14.3827749410654,
127.761275810437)) ;
#152945=CARTESIAN_POINT('Ctrl Pts',(-32.1067647607671,14.2124739950545,
127.988225629159)) ;
#152946=CARTESIAN_POINT('Ctrl Pts',(-32.1557319181306,13.9855789386979,
128.164396849995)) ;
#152947=CARTESIAN_POINT('Ctrl Pts',(-32.1830886305706,13.7185805864342,
128.27741749427)) ;
#152948=CARTESIAN_POINT('Ctrl Pts',(-32.1861674536437,13.4303185636673,
128.319530923703)) ;
#152949=CARTESIAN_POINT('Ctrl Pts',(-32.164067606359,13.1417758325219,128.288060327875)) ;
#152950=CARTESIAN_POINT('Ctrl Pts',(-32.1174319130124,12.8725286043858,
128.185023246156)) ;
#152951=CARTESIAN_POINT('Ctrl Pts',(-32.0491401802662,12.6435096258014,
128.018626363072)) ;
#152952=CARTESIAN_POINT('Ctrl Pts',(-31.9632199754991,12.4701546223289,
127.800755651149)) ;
#152953=CARTESIAN_POINT('Ctrl Pts',(-31.8651776863348,12.3650501876111,
127.547453264018)) ;
#152954=CARTESIAN_POINT('Ctrl Pts',(-31.7609862185599,12.3357586674927,
127.276274914652)) ;
#152955=CARTESIAN_POINT('Ctrl Pts',(-31.6580563102104,12.3843195509594,
127.008647533804)) ;
#152956=CARTESIAN_POINT('Ctrl Pts',(-31.5623522569141,12.5073666683789,
126.762219617398)) ;
#152957=CARTESIAN_POINT('Ctrl Pts',(-31.4804283317136,12.6958200369819,
126.55599240923)) ;
#152958=CARTESIAN_POINT('Ctrl Pts',(-31.4171911262104,12.9363649293222,
126.404372140452)) ;
#152959=CARTESIAN_POINT('Ctrl Pts',(-31.3765204454803,13.212046231595,126.318705695641)) ;
#152960=CARTESIAN_POINT('Ctrl Pts',(-31.3605890149829,13.5022481067603,
126.305235943963)) ;
#152961=CARTESIAN_POINT('Ctrl Pts',(-31.3699466511949,13.7884016128943,
126.365844507772)) ;
#152962=CARTESIAN_POINT('Ctrl Pts',(-31.402839929772,14.045945075732,126.494887877481)) ;
#152963=CARTESIAN_POINT('Ctrl Pts',(-31.456801839307,14.2610680704969,126.685797164984)) ;
#152964=CARTESIAN_POINT('Ctrl Pts',(-31.5263791105061,14.4145624165552,
126.922033359285)) ;
#152965=CARTESIAN_POINT('Ctrl Pts',(-31.6068029650713,14.4980852125695,
127.190187763467)) ;
#152966=CARTESIAN_POINT('Ctrl Pts',(-31.6909497784616,14.5041312739862,
127.469125424148)) ;
#152967=CARTESIAN_POINT('Ctrl Pts',(-31.7722616933248,14.4326962339747,
127.739802187408)) ;
#152968=CARTESIAN_POINT('Ctrl Pts',(-31.8440399327869,14.289424830309,127.982545178335)) ;
#152969=CARTESIAN_POINT('Ctrl Pts',(-31.9008586342929,14.0826507854277,
128.181809264848)) ;
#152970=CARTESIAN_POINT('Ctrl Pts',(-31.9371644477761,13.8312291814697,
128.320780138694)) ;
#152971=CARTESIAN_POINT('Ctrl Pts',(-31.9504192122518,13.5479805821752,
128.392761416066)) ;
#152972=CARTESIAN_POINT('Ctrl Pts',(-31.9384428607775,13.2572981016289,
128.390846357411)) ;
#152973=CARTESIAN_POINT('Ctrl Pts',(-31.9016603090654,12.9781391944844,
128.316499055668)) ;
#152974=CARTESIAN_POINT('Ctrl Pts',(-31.8414344653115,12.7298471383749,
128.173831316095)) ;
#152975=CARTESIAN_POINT('Ctrl Pts',(-31.7624693619783,12.5331718510569,
127.976098656417)) ;
#152976=CARTESIAN_POINT('Ctrl Pts',(-31.6682896816273,12.3987050488903,
127.734214112554)) ;
#152977=CARTESIAN_POINT('Ctrl Pts',(-31.5661584069127,12.3381977133859,
127.468894861423)) ;
#152978=CARTESIAN_POINT('Ctrl Pts',(-31.4613121151811,12.3556285786372,
127.195919765139)) ;
#152979=CARTESIAN_POINT('Ctrl Pts',(-31.3626542471411,12.448498640132,126.940567661376)) ;
#152980=CARTESIAN_POINT('Ctrl Pts',(-31.2739963638957,12.6124651727369,
126.714860191145)) ;
#152981=CARTESIAN_POINT('Ctrl Pts',(-31.2028733579617,12.8330193864531,
126.540078371683)) ;
#152982=CARTESIAN_POINT('Ctrl Pts',(-31.1524099899045,13.0981216515098,
126.425973898796)) ;
#152983=CARTESIAN_POINT('Ctrl Pts',(-31.1264884036244,13.3840423616995,
126.383240800023)) ;
#152984=CARTESIAN_POINT('Ctrl Pts',(-31.1255526905879,13.6738043197191,
126.413632148392)) ;
#152985=CARTESIAN_POINT('Ctrl Pts',(-31.1492407119047,13.9458856450603,
126.515980892251)) ;
#152986=CARTESIAN_POINT('Ctrl Pts',(-31.1951906788803,14.1805609741337,
126.683399895541)) ;
#152987=CARTESIAN_POINT('Ctrl Pts',(-31.2589322113538,14.3602096703021,
126.902625201214)) ;
#152988=CARTESIAN_POINT('Ctrl Pts',(-31.336152907064,14.4737146563849,127.161521971997)) ;
#152989=CARTESIAN_POINT('Ctrl Pts',(-31.4191607366893,14.510981736058,127.436983917868)) ;
#152990=CARTESIAN_POINT('Ctrl Pts',(-31.5023202222332,14.4710234538019,
127.713002150618)) ;
#152991=CARTESIAN_POINT('Ctrl Pts',(-31.5788150531214,14.3558611755068,
127.9695934644)) ;
#152992=CARTESIAN_POINT('Ctrl Pts',(-31.6423459010436,14.1736059642118,
128.188348020273)) ;
#152993=CARTESIAN_POINT('Ctrl Pts',(-31.6874883180192,13.9381264816024,
128.353301532308)) ;
#152994=CARTESIAN_POINT('Ctrl Pts',(-31.7104598612239,13.665192099168,128.453567738071)) ;
#152995=CARTESIAN_POINT('Ctrl Pts',(-31.7088598170554,13.3755914984187,
128.481967244671)) ;
#152996=CARTESIAN_POINT('Ctrl Pts',(-31.6817723867748,13.0874857506397,
128.436147123456)) ;
#152997=CARTESIAN_POINT('Ctrl Pts',(-31.6311222896079,12.8264337657975,
128.32111606456)) ;
#152998=CARTESIAN_POINT('Ctrl Pts',(-31.5590254861687,12.6060974389448,
128.143694924089)) ;
#152999=CARTESIAN_POINT('Ctrl Pts',(-31.4705496041744,12.4450313389733,
127.91828768914)) ;
#153000=CARTESIAN_POINT('Ctrl Pts',(-31.3704536339561,12.3534666197661,
127.659136554107)) ;
#153001=CARTESIAN_POINT('Ctrl Pts',(-31.2664260741019,12.3390029903486,
127.388267266672)) ;
#153002=CARTESIAN_POINT('Ctrl Pts',(-31.1640074542676,12.4020392430349,
127.122262231831)) ;
#153003=CARTESIAN_POINT('Ctrl Pts',(-31.0704546098695,12.5385711173323,
126.882123477286)) ;
#153004=CARTESIAN_POINT('Ctrl Pts',(-30.9919375233747,12.737337324062,126.685748126109)) ;
#153005=CARTESIAN_POINT('Ctrl Pts',(-30.9326059877163,12.9861206892308,
126.545580982005)) ;
#153006=CARTESIAN_POINT('Ctrl Pts',(-30.8964828802307,13.2660910782566,
126.473182758033)) ;
#153007=CARTESIAN_POINT('Ctrl Pts',(-30.8853353619794,13.5573227840952,
126.473749977841)) ;
#153008=CARTESIAN_POINT('Ctrl Pts',(-30.8992181639316,13.8386952169897,
126.547405844888)) ;
#153009=CARTESIAN_POINT('Ctrl Pts',(-30.9364490028324,14.0906007554108,
126.689305896974)) ;
#153010=CARTESIAN_POINT('Ctrl Pts',(-30.993577379338,14.2945039762926,126.889303441531)) ;
#153011=CARTESIAN_POINT('Ctrl Pts',(-31.0658785833472,14.4361574187858,
127.133657392973)) ;
#153012=CARTESIAN_POINT('Ctrl Pts',(-31.1473678175875,14.5051117570611,
127.404837868273)) ;
#153013=CARTESIAN_POINT('Ctrl Pts',(-31.2314101845586,14.496582620466,127.68344430737)) ;
#153014=CARTESIAN_POINT('Ctrl Pts',(-31.3113999047549,14.4113394819302,
127.950224339128)) ;
#153015=CARTESIAN_POINT('Ctrl Pts',(-31.3810275644355,14.2546479447355,
128.186843915728)) ;
#153016=CARTESIAN_POINT('Ctrl Pts',(-31.434079388976,14.039143877786,128.374888028828)) ;
#153017=CARTESIAN_POINT('Ctrl Pts',(-31.4664410188237,13.7793416572316,
128.502539340318)) ;
#153018=CARTESIAN_POINT('Ctrl Pts',(-31.4749982660917,13.4941095874199,
128.560637934817)) ;
#153019=CARTESIAN_POINT('Ctrl Pts',(-31.4582310109701,13.2026874966814,
128.544890911873)) ;
#153020=CARTESIAN_POINT('Ctrl Pts',(-31.4169753439866,12.928833346161,128.457383735722)) ;
#153021=CARTESIAN_POINT('Ctrl Pts',(-31.3527956487623,12.6885083712283,
128.303172142516)) ;
#153022=CARTESIAN_POINT('Ctrl Pts',(-31.2705703901443,12.5026390795781,
128.0959611027)) ;
#153023=CARTESIAN_POINT('Ctrl Pts',(-31.1745744230575,12.3816810236162,
127.848677279268)) ;
#153024=CARTESIAN_POINT('Ctrl Pts',(-31.0714307037018,12.3354826595071,
127.580451601079)) ;
#153025=CARTESIAN_POINT('Ctrl Pts',(-30.9672895160686,12.3671988660942,
127.309429336125)) ;
#153026=CARTESIAN_POINT('Ctrl Pts',(-30.8693900237751,12.4748749581507,
127.056599017908)) ;
#153027=CARTESIAN_POINT('Ctrl Pts',(-30.7841568236753,12.6498955190515,
126.840662152846)) ;
#153028=CARTESIAN_POINT('Ctrl Pts',(-30.7165115975955,12.8801431332148,
126.67612667683)) ;
#153029=CARTESIAN_POINT('Ctrl Pts',(-30.6705876552176,13.1504415297617,
126.575185235204)) ;
#153030=CARTESIAN_POINT('Ctrl Pts',(-30.6492401911973,13.438739202615,126.545850310757)) ;
#153031=CARTESIAN_POINT('Ctrl Pts',(-30.6531248486497,13.7280473502378,
126.590480521703)) ;
#153032=CARTESIAN_POINT('Ctrl Pts',(-30.6811874381857,13.9932362064335,
126.705468605857)) ;
#153033=CARTESIAN_POINT('Ctrl Pts',(-30.7307233901376,14.2186783745982,
126.88330032276)) ;
#153034=CARTESIAN_POINT('Ctrl Pts',(-30.7976668939673,14.3872014330787,
127.112042032862)) ;
#153035=CARTESIAN_POINT('Ctrl Pts',(-30.8759215226086,14.486216521528,127.373662762679)) ;
#153036=CARTESIAN_POINT('Ctrl Pts',(-30.9599483085192,14.5095010567365,
127.652320679818)) ;
#153037=CARTESIAN_POINT('Ctrl Pts',(-31.0423602583126,14.4548476689191,
127.926162766265)) ;
#153038=CARTESIAN_POINT('Ctrl Pts',(-31.1170261636548,14.3259646517619,
128.177490633467)) ;
#153039=CARTESIAN_POINT('Ctrl Pts',(-31.1774376241067,14.1320240566172,
128.38715540167)) ;
#153040=CARTESIAN_POINT('Ctrl Pts',(-31.2184772814882,13.8890687487633,
128.540002184362)) ;
#153041=CARTESIAN_POINT('Ctrl Pts',(-31.2369718788586,13.6109288487181,
128.62723857725)) ;
#153042=CARTESIAN_POINT('Ctrl Pts',(-31.2305830637653,13.3205780973656,
128.64162358396)) ;
#153043=CARTESIAN_POINT('Ctrl Pts',(-31.1988306507602,13.0356410236252,
128.582156307125)) ;
#153044=CARTESIAN_POINT('Ctrl Pts',(-31.1439236012217,12.7811568557338,
128.454705635715)) ;
#153045=CARTESIAN_POINT('Ctrl Pts',(-31.0684038299569,12.5709851276515,
128.267243241426)) ;
#153046=CARTESIAN_POINT('Ctrl Pts',(-30.9772756205,12.4221766619671,128.03413250274)) ;
#153047=CARTESIAN_POINT('Ctrl Pts',(-30.8759319496152,12.3447406812541,
127.771290965256)) ;
#153048=CARTESIAN_POINT('Ctrl Pts',(-30.7712963261735,12.3451621602759,
127.498804673837)) ;
#153049=CARTESIAN_POINT('Ctrl Pts',(-30.6706886680026,12.4221617733591,
127.237875690043)) ;
#153050=CARTESIAN_POINT('Ctrl Pts',(-30.5793389036692,12.5713293574021,
127.00420358355)) ;
#153051=CARTESIAN_POINT('Ctrl Pts',(-30.5039469378259,12.7811357471148,
126.817049360709)) ;
#153052=CARTESIAN_POINT('Ctrl Pts',(-30.4488110435835,13.037385413305,126.689142569762)) ;
#153053=CARTESIAN_POINT('Ctrl Pts',(-30.4173468141487,13.3202247802994,
126.630258735514)) ;
#153054=CARTESIAN_POINT('Ctrl Pts',(-30.4109588954888,13.6126649497902,
126.644895127432)) ;
#153055=CARTESIAN_POINT('Ctrl Pts',(-30.4294392941911,13.889109539137,126.731888107809)) ;
#153056=CARTESIAN_POINT('Ctrl Pts',(-30.47077570761,14.1334576219234,126.885811226843)) ;
#153057=CARTESIAN_POINT('Ctrl Pts',(-30.53102912446,14.3262010857029,127.094865661672)) ;
#153058=CARTESIAN_POINT('Ctrl Pts',(-30.6058078949067,14.4552702241494,
127.346574791049)) ;
#153059=CARTESIAN_POINT('Ctrl Pts',(-30.6883760016807,14.5094659873619,
127.620923977953)) ;
#153060=CARTESIAN_POINT('Ctrl Pts',(-30.7718896570381,14.48627928254,127.897878479629)) ;
#153061=CARTESIAN_POINT('Ctrl Pts',(-30.8505404170833,14.3867194330965,
128.16082928885)) ;
#153062=CARTESIAN_POINT('Ctrl Pts',(-30.9172652518935,14.2183273389604,
128.388850744567)) ;
#153063=CARTESIAN_POINT('Ctrl Pts',(-30.966927867041,13.9922441011096,128.567141543632)) ;
#153064=CARTESIAN_POINT('Ctrl Pts',(-30.9948429554227,13.7260908863955,
128.681785518138)) ;
#153065=CARTESIAN_POINT('Ctrl Pts',(-30.9986761317404,13.4392990683917,
128.725970798859)) ;
#153066=CARTESIAN_POINT('Ctrl Pts',(-30.9771754995003,13.1491383926391,
128.696410048975)) ;
#153067=CARTESIAN_POINT('Ctrl Pts',(-30.9313862314932,12.880138144259,128.595705294773)) ;
#153068=CARTESIAN_POINT('Ctrl Pts',(-30.8633741700187,12.6488312040692,
128.430267551873)) ;
#153069=CARTESIAN_POINT('Ctrl Pts',(-30.7783096718615,12.4746173052797,
128.214724190605)) ;
#153070=CARTESIAN_POINT('Ctrl Pts',(-30.6802839201009,12.3669410581914,
127.961566303494)) ;
#153071=CARTESIAN_POINT('Ctrl Pts',(-30.5761954681339,12.3355244467329,
127.690674965918)) ;
#153072=CARTESIAN_POINT('Ctrl Pts',(-30.4731987242308,12.3818824637266,
127.42284013735)) ;
#153073=CARTESIAN_POINT('Ctrl Pts',(-30.3773601675738,12.502442440452,127.175947943775)) ;
#153074=CARTESIAN_POINT('Ctrl Pts',(-30.2945593439143,12.6900860359651,
126.967322197996)) ;
#153075=CARTESIAN_POINT('Ctrl Pts',(-30.2309201264915,12.9290693621117,
126.814464075625)) ;
#153076=CARTESIAN_POINT('Ctrl Pts',(-30.1896011311781,13.2033802627449,
126.726833819823)) ;
#153077=CARTESIAN_POINT('Ctrl Pts',(-30.1729187517655,13.493885424346,126.711224329232)) ;
#153078=CARTESIAN_POINT('Ctrl Pts',(-30.1814818466642,13.7798208359641,
126.769425110779)) ;
#153079=CARTESIAN_POINT('Ctrl Pts',(-30.2139166442141,14.0398147256928,
126.897315524147)) ;
#153080=CARTESIAN_POINT('Ctrl Pts',(-30.2672327260932,14.2555980954836,
127.086230738633)) ;
#153081=CARTESIAN_POINT('Ctrl Pts',(-30.3364241626342,14.4112165057251,
127.321355815591)) ;
#153082=CARTESIAN_POINT('Ctrl Pts',(-30.4169483545396,14.4969135755094,
127.589920286704)) ;
#153083=CARTESIAN_POINT('Ctrl Pts',(-30.5006568417281,14.5049696810031,
127.867411820872)) ;
#153084=CARTESIAN_POINT('Ctrl Pts',(-30.5821059141925,14.4360249735447,
128.13846691764)) ;
#153085=CARTESIAN_POINT('Ctrl Pts',(-30.6543269887437,14.2945754362065,
128.382542123477)) ;
#153086=CARTESIAN_POINT('Ctrl Pts',(-30.7116365732865,14.0897548858671,
128.583199406406)) ;
#153087=CARTESIAN_POINT('Ctrl Pts',(-30.7486474004249,13.8387001375239,
128.724327683098)) ;
#153088=CARTESIAN_POINT('Ctrl Pts',(-30.7626160375506,13.5574044598577,
128.79823198023)) ;
#153089=CARTESIAN_POINT('Ctrl Pts',(-30.751280169492,13.2644130009093,128.798450590054)) ;
#153090=CARTESIAN_POINT('Ctrl Pts',(-30.7152762753897,12.9862195730077,
128.726198614227)) ;
#153091=CARTESIAN_POINT('Ctrl Pts',(-30.6559255495121,12.7371111819008,
128.586013158079)) ;
#153092=CARTESIAN_POINT('Ctrl Pts',(-30.5772199975952,12.5380203242925,
128.389149798631)) ;
#153093=CARTESIAN_POINT('Ctrl Pts',(-30.4833480932253,12.4015272632005,
128.148171071429)) ;
#153094=CARTESIAN_POINT('Ctrl Pts',(-30.3812924082162,12.3389470103484,
127.883098879055)) ;
#153095=CARTESIAN_POINT('Ctrl Pts',(-30.2769531606877,12.3537864997403,
127.611426962061)) ;
#153096=CARTESIAN_POINT('Ctrl Pts',(-30.1774142848297,12.4449099176858,
127.353712328041)) ;
#153097=CARTESIAN_POINT('Ctrl Pts',(-30.0884196313121,12.6072327563546,
127.127011108624)) ;
#153098=CARTESIAN_POINT('Ctrl Pts',(-30.0168944583603,12.8259751420657,
126.950999128042)) ;
#153099=CARTESIAN_POINT('Ctrl Pts',(-29.9658131020968,13.0894865209779,
126.835020394129)) ;
#153100=CARTESIAN_POINT('Ctrl Pts',(-29.9390402950618,13.3763086244584,
126.789949510195)) ;
#153101=CARTESIAN_POINT('Ctrl Pts',(-29.9374976893148,13.666102426872,126.818551688385)) ;
#153102=CARTESIAN_POINT('Ctrl Pts',(-29.9603659689101,13.9378774393092,
126.918366530385)) ;
#153103=CARTESIAN_POINT('Ctrl Pts',(-30.0058557147277,14.174793298913,127.084558461599)) ;
#153104=CARTESIAN_POINT('Ctrl Pts',(-30.0690738202602,14.355667987911,127.302193672896)) ;
#153105=CARTESIAN_POINT('Ctrl Pts',(-30.1455851444044,14.4711053294092,
127.558860146817)) ;
#153106=CARTESIAN_POINT('Ctrl Pts',(-30.2290907276294,14.511170979715,127.836014853784)) ;
#153107=CARTESIAN_POINT('Ctrl Pts',(-30.3124346958538,14.4729025341711,
128.112614820692)) ;
#153108=CARTESIAN_POINT('Ctrl Pts',(-30.3888326028229,14.3605014183323,
128.368750566373)) ;
#153109=CARTESIAN_POINT('Ctrl Pts',(-30.4531791538599,14.1789799497678,
128.590078616567)) ;
#153110=CARTESIAN_POINT('Ctrl Pts',(-30.4986908853725,13.9453130755044,
128.756011357139)) ;
#153111=CARTESIAN_POINT('Ctrl Pts',(-30.5223367702664,13.673613297581,128.858202384461)) ;
#153112=CARTESIAN_POINT('Ctrl Pts',(-30.5214927257582,13.3843416477693,
128.888796839614)) ;
#153113=CARTESIAN_POINT('Ctrl Pts',(-30.4951356796959,13.0956424787648,
128.845131685907)) ;
#153114=CARTESIAN_POINT('Ctrl Pts',(-30.4451353943437,12.8335787485534,
128.73200501772)) ;
#153115=CARTESIAN_POINT('Ctrl Pts',(-30.3735874311193,12.6116522531053,
128.556195762552)) ;
#153116=CARTESIAN_POINT('Ctrl Pts',(-30.2853579635812,12.4486058050818,
128.33155990322)) ;
#153117=CARTESIAN_POINT('Ctrl Pts',(-30.1858663129506,12.3551665981467,
128.074050595748)) ;
#153118=CARTESIAN_POINT('Ctrl Pts',(-30.0815496988783,12.3383111368361,
127.802444396815)) ;
#153119=CARTESIAN_POINT('Ctrl Pts',(-29.9791399961725,12.3991318667188,
127.536410522558)) ;
#153120=CARTESIAN_POINT('Ctrl Pts',(-29.885250975789,12.5336133546432,127.2952913997)) ;
#153121=CARTESIAN_POINT('Ctrl Pts',(-29.8062098846917,12.7304747525644,
127.097365942919)) ;
#153122=CARTESIAN_POINT('Ctrl Pts',(-29.7459166115697,12.9801493565206,
126.954643707808)) ;
#153123=CARTESIAN_POINT('Ctrl Pts',(-29.7094981424688,13.2569930870622,
126.881074054437)) ;
#153124=CARTESIAN_POINT('Ctrl Pts',(-29.697485321225,13.5493201067258,126.879249155707)) ;
#153125=CARTESIAN_POINT('Ctrl Pts',(-29.7107148915496,13.8310609228274,
126.950973130347)) ;
#153126=CARTESIAN_POINT('Ctrl Pts',(-29.7473686079901,14.0843638099265,
127.091228525209)) ;
#153127=CARTESIAN_POINT('Ctrl Pts',(-29.8039983073089,14.2896244491401,
127.289751241016)) ;
#153128=CARTESIAN_POINT('Ctrl Pts',(-29.8758248177242,14.4330063116879,
127.5326649792)) ;
#153129=CARTESIAN_POINT('Ctrl Pts',(-29.9571776043441,14.5042107415309,
127.803464708327)) ;
#153130=CARTESIAN_POINT('Ctrl Pts',(-30.0412713276901,14.4979449999679,
128.082232149485)) ;
#153131=CARTESIAN_POINT('Ctrl Pts',(-30.121694639328,14.4144601779744,128.350375838408)) ;
#153132=CARTESIAN_POINT('Ctrl Pts',(-30.1915790917938,14.2595209902124,
128.587713560571)) ;
#153133=CARTESIAN_POINT('Ctrl Pts',(-30.2450076010872,14.046214919979,128.776755103724)) ;
#153134=CARTESIAN_POINT('Ctrl Pts',(-30.2780878046331,13.7868053449528,
128.906585374679)) ;
#153135=CARTESIAN_POINT('Ctrl Pts',(-30.2872906950602,13.5027357390144,
128.966484763682)) ;
#153136=CARTESIAN_POINT('Ctrl Pts',(-30.2713500951273,13.2114164567146,
128.953122045362)) ;
#153137=CARTESIAN_POINT('Ctrl Pts',(-30.230627814723,12.9359342983456,128.86728322249)) ;
#153138=CARTESIAN_POINT('Ctrl Pts',(-30.1672447422047,12.6951562018299,
128.715288751686)) ;
#153139=CARTESIAN_POINT('Ctrl Pts',(-30.0854978465419,12.5073061272103,
128.509491429827)) ;
#153140=CARTESIAN_POINT('Ctrl Pts',(-29.9896882822811,12.3841592686752,
128.262793679839)) ;
#153141=CARTESIAN_POINT('Ctrl Pts',(-29.8866361087517,12.3356200239572,
127.994841190901)) ;
#153142=CARTESIAN_POINT('Ctrl Pts',(-29.7820423738734,12.3655842279676,
127.722626897302)) ;
#153143=CARTESIAN_POINT('Ctrl Pts',(-29.6846378874882,12.4702048591763,
127.470973299483)) ;
#153144=CARTESIAN_POINT('Ctrl Pts',(-29.5982444318826,12.6448837976238,
127.251934053335)) ;
#153145=CARTESIAN_POINT('Ctrl Pts',(-29.530484788473,12.872508423284,127.086857758343)) ;
#153146=CARTESIAN_POINT('Ctrl Pts',(-29.4836133061575,13.1434988331289,
126.983345728084)) ;
#153147=CARTESIAN_POINT('Ctrl Pts',(-29.4617927517553,13.4301737780494,
126.952467269919)) ;
#153148=CARTESIAN_POINT('Ctrl Pts',(-29.4647728375027,13.7187795914099,
126.994328449619)) ;
#153149=CARTESIAN_POINT('Ctrl Pts',(-29.4924039666026,13.9870154433738,
127.108324446431)) ;
#153150=CARTESIAN_POINT('Ctrl Pts',(-29.5411722729436,14.2124398345738,
127.283727368873)) ;
#153151=CARTESIAN_POINT('Ctrl Pts',(-29.6075895922723,14.3830654461858,
127.510923381855)) ;
#153152=CARTESIAN_POINT('Ctrl Pts',(-29.6859780654117,14.4846609541733,
127.773091506423)) ;
#153153=CARTESIAN_POINT('Ctrl Pts',(-29.7699711987632,14.5097913616969,
128.051659371141)) ;
#153154=CARTESIAN_POINT('Ctrl Pts',(-29.8521599614632,14.4576093080194,
128.324704513275)) ;
#153155=CARTESIAN_POINT('Ctrl Pts',(-29.9273378651692,14.3304831317374,
128.57761366537)) ;
#153156=CARTESIAN_POINT('Ctrl Pts',(-29.9881011678196,14.1386183822934,
128.788232639006)) ;
#153157=CARTESIAN_POINT('Ctrl Pts',(-30.0298088081978,13.8965846856625,
128.943079017119)) ;
#153158=CARTESIAN_POINT('Ctrl Pts',(-30.048987740085,13.6198365630073,129.032230754272)) ;
#153159=CARTESIAN_POINT('Ctrl Pts',(-30.0433213484704,13.3288844737818,
129.048809941996)) ;
#153160=CARTESIAN_POINT('Ctrl Pts',(-30.0124680035273,13.0447399832046,
128.991813037362)) ;
#153161=CARTESIAN_POINT('Ctrl Pts',(-29.958162147996,12.7881836368688,128.866220633411)) ;
#153162=CARTESIAN_POINT('Ctrl Pts',(-29.8827371039613,12.5755910115287,
128.67919720058)) ;
#153163=CARTESIAN_POINT('Ctrl Pts',(-29.7923817501949,12.4257574465567,
128.448186718166)) ;
#153164=CARTESIAN_POINT('Ctrl Pts',(-29.6914548654442,12.3460112405744,
128.186501449005)) ;
#153165=CARTESIAN_POINT('Ctrl Pts',(-29.5867020660159,12.3439532504127,
127.913710488866)) ;
#153166=CARTESIAN_POINT('Ctrl Pts',(-29.485666657119,12.4188218900739,127.651602416161)) ;
#153167=CARTESIAN_POINT('Ctrl Pts',(-29.3936759004092,12.5668341062151,
127.416175460721)) ;
#153168=CARTESIAN_POINT('Ctrl Pts',(-29.3182301931701,12.7739565310488,
127.2286723812)) ;
#153169=CARTESIAN_POINT('Ctrl Pts',(-29.2623086088496,13.0292275295923,
127.098504241357)) ;
#153170=CARTESIAN_POINT('Ctrl Pts',(-29.2301243830033,13.3121167714202,
127.037580467898)) ;
#153171=CARTESIAN_POINT('Ctrl Pts',(-29.2229734795966,13.6036711588795,
127.049873651472)) ;
#153172=CARTESIAN_POINT('Ctrl Pts',(-29.2408639834952,13.8822010088686,
127.135317168003)) ;
#153173=CARTESIAN_POINT('Ctrl Pts',(-29.2814175857852,14.126534024312,127.286789452504)) ;
#153174=CARTESIAN_POINT('Ctrl Pts',(-29.341269933413,14.3215277156221,127.494747226261)) ;
#153175=CARTESIAN_POINT('Ctrl Pts',(-29.4156496701704,14.4523872469144,
127.745252022521)) ;
#153176=CARTESIAN_POINT('Ctrl Pts',(-29.4979993749135,14.509081269933,128.018936330148)) ;
#153177=CARTESIAN_POINT('Ctrl Pts',(-29.5821194390776,14.4877530584647,
128.297884507417)) ;
#153178=CARTESIAN_POINT('Ctrl Pts',(-29.6605015766084,14.3906972492053,
128.559841528178)) ;
#153179=CARTESIAN_POINT('Ctrl Pts',(-29.7277325620602,14.2242127265294,
128.789368837068)) ;
#153180=CARTESIAN_POINT('Ctrl Pts',(-29.7778622908604,14.0000453961231,
128.968956847515)) ;
#153181=CARTESIAN_POINT('Ctrl Pts',(-29.8065930602879,13.7349941187306,
129.085980593616)) ;
#153182=CARTESIAN_POINT('Ctrl Pts',(-29.8110647581583,13.4462938086935,
129.132290262238)) ;
#153183=CARTESIAN_POINT('Ctrl Pts',(-29.7905149481192,13.1586524064852,
129.105179558969)) ;
#153184=CARTESIAN_POINT('Ctrl Pts',(-29.7450251194424,12.8863235925418,
129.005657518442)) ;
#153185=CARTESIAN_POINT('Ctrl Pts',(-29.6779688870286,12.6553854575325,
128.842782884932)) ;
#153186=CARTESIAN_POINT('Ctrl Pts',(-29.5932822353585,12.4787538591612,
128.628403260321)) ;
#153187=CARTESIAN_POINT('Ctrl Pts',(-29.4951432611704,12.3688114822916,
128.375032108495)) ;
#153188=CARTESIAN_POINT('Ctrl Pts',(-29.3915755638739,12.3354319136936,
128.105522888968)) ;
#153189=CARTESIAN_POINT('Ctrl Pts',(-29.2883737439491,12.3792576310417,
127.83711019449)) ;
#153190=CARTESIAN_POINT('Ctrl Pts',(-29.1917010872287,12.4988398999205,
127.587984309591)) ;
#153191=CARTESIAN_POINT('Ctrl Pts',(-29.1090972687786,12.6835118512005,
127.379683329034)) ;
#153192=CARTESIAN_POINT('Ctrl Pts',(-29.0446608613966,12.9214923912795,
127.224563683631)) ;
#153193=CARTESIAN_POINT('Ctrl Pts',(-29.0026163941945,13.1954916424955,
127.134859426664)) ;
#153194=CARTESIAN_POINT('Ctrl Pts',(-28.985230945197,13.4865485670219,127.117276574287)) ;
#153195=CARTESIAN_POINT('Ctrl Pts',(-28.9931808891691,13.772471589557,127.173641275195)) ;
#153196=CARTESIAN_POINT('Ctrl Pts',(-29.0248180797672,14.0322259092952,
127.299049560001)) ;
#153197=CARTESIAN_POINT('Ctrl Pts',(-29.0774225647813,14.2496185339524,
127.485847881482)) ;
#153198=CARTESIAN_POINT('Ctrl Pts',(-29.1466584272716,14.4079186586772,
127.721302692546)) ;
#153199=CARTESIAN_POINT('Ctrl Pts',(-29.2262609733389,14.495128940057,127.986882942297)) ;
#153200=CARTESIAN_POINT('Ctrl Pts',(-29.310377688868,14.5060206783235,128.265744239721)) ;
#153201=CARTESIAN_POINT('Ctrl Pts',(-29.3922415681972,14.4388851972431,
128.538108177024)) ;
#153202=CARTESIAN_POINT('Ctrl Pts',(-29.4648367940965,14.2990479598781,
128.783307296558)) ;
#153203=CARTESIAN_POINT('Ctrl Pts',(-29.5224591681686,14.096277092635,128.984789687897)) ;
#153204=CARTESIAN_POINT('Ctrl Pts',(-29.5601633246064,13.8463552274942,
129.12795060112)) ;
#153205=CARTESIAN_POINT('Ctrl Pts',(-29.5747316968106,13.5643762793268,
129.203747316631)) ;
#153206=CARTESIAN_POINT('Ctrl Pts',(-29.5643172687888,13.2747380866486,
129.206268472805)) ;
#153207=CARTESIAN_POINT('Ctrl Pts',(-29.5288291438255,12.9934296976024,
129.135814296567)) ;
#153208=CARTESIAN_POINT('Ctrl Pts',(-29.470171863856,12.7438068041656,128.99757323151)) ;
#153209=CARTESIAN_POINT('Ctrl Pts',(-29.391803285665,12.5426943442427,128.801768222048)) ;
#153210=CARTESIAN_POINT('Ctrl Pts',(-29.2986131391391,12.4046936236787,
128.56265775762)) ;
#153211=CARTESIAN_POINT('Ctrl Pts',(-29.1964773761958,12.3396331759052,
128.297435830634)) ;
#153212=CARTESIAN_POINT('Ctrl Pts',(-29.092230590555,12.3522550875064,128.025991131613)) ;
#153213=CARTESIAN_POINT('Ctrl Pts',(-28.9924608185787,12.441158614988,127.767604009206)) ;
#153214=CARTESIAN_POINT('Ctrl Pts',(-28.9030933450802,12.6013769713038,
127.539790029494)) ;
#153215=CARTESIAN_POINT('Ctrl Pts',(-28.8308886096015,12.819071640269,127.361858709555)) ;
#153216=CARTESIAN_POINT('Ctrl Pts',(-28.779280341327,13.0807346140254,127.244233442709)) ;
#153217=CARTESIAN_POINT('Ctrl Pts',(-28.7517055757331,13.3675408612144,
127.196874862189)) ;
#153218=CARTESIAN_POINT('Ctrl Pts',(-28.7493257047856,13.6570979280699,
127.222968219409)) ;
#153219=CARTESIAN_POINT('Ctrl Pts',(-28.7718142821641,13.9319893911641,
127.321979864566)) ;
#153220=CARTESIAN_POINT('Ctrl Pts',(-28.8162456944187,14.1676085258846,
127.484711805867)) ;
#153221=CARTESIAN_POINT('Ctrl Pts',(-28.8794392120634,14.3519029604138,
127.702543293248)) ;
#153222=CARTESIAN_POINT('Ctrl Pts',(-28.955521536148,14.4687263868581,127.957864396171)) ;
#153223=CARTESIAN_POINT('Ctrl Pts',(-29.0386446837284,14.5110206744739,
128.233803590714)) ;
#153224=CARTESIAN_POINT('Ctrl Pts',(-29.1220480184099,14.4754839101951,
128.510547823415)) ;
#153225=CARTESIAN_POINT('Ctrl Pts',(-29.1992609632459,14.3641243881349,
128.769313204063)) ;
#153226=CARTESIAN_POINT('Ctrl Pts',(-29.2634796257756,14.1859981150162,
128.989963010774)) ;
#153227=CARTESIAN_POINT('Ctrl Pts',(-29.309906743687,13.9527739629267,129.158738849017)) ;
#153228=CARTESIAN_POINT('Ctrl Pts',(-29.3342115703911,13.6818171869407,
129.262851136394)) ;
#153229=CARTESIAN_POINT('Ctrl Pts',(-29.3340473631818,13.3923456599437,
129.295485666288)) ;
#153230=CARTESIAN_POINT('Ctrl Pts',(-29.3085669103323,13.1044625348289,
129.254236375475)) ;
#153231=CARTESIAN_POINT('Ctrl Pts',(-29.258986211392,12.8400820200563,129.142508243958)) ;
#153232=CARTESIAN_POINT('Ctrl Pts',(-29.1881542029012,12.6174283224968,
128.968693652698)) ;
#153233=CARTESIAN_POINT('Ctrl Pts',(-29.1002100971169,12.4521814963559,
128.744946986999)) ;
#153234=CARTESIAN_POINT('Ctrl Pts',(-29.0009103649547,12.3567835155047,
128.48800496993)) ;
#153235=CARTESIAN_POINT('Ctrl Pts',(-28.896925987083,12.3377092271658,128.21727920025)) ;
#153236=CARTESIAN_POINT('Ctrl Pts',(-28.7942667965697,12.3962076032604,
127.950545837014)) ;
#153237=CARTESIAN_POINT('Ctrl Pts',(-28.6998220504126,12.5290432373042,
127.70787965737)) ;
#153238=CARTESIAN_POINT('Ctrl Pts',(-28.6204061898145,12.7244085230837,
127.508847094626)) ;
#153239=CARTESIAN_POINT('Ctrl Pts',(-28.559819094265,12.9709500550387,127.365030411237)) ;
#153240=CARTESIAN_POINT('Ctrl Pts',(-28.5223002592329,13.2494402817627,
127.288528530129)) ;
#153241=CARTESIAN_POINT('Ctrl Pts',(-28.5097189788881,13.5418967084717,
127.285058220228)) ;
#153242=CARTESIAN_POINT('Ctrl Pts',(-28.5222097719137,13.8230883914708,
127.354499660829)) ;
#153243=CARTESIAN_POINT('Ctrl Pts',(-28.5582144837367,14.0775910910953,
127.492866930045)) ;
#153244=CARTESIAN_POINT('Ctrl Pts',(-28.6142444612186,14.2842118886259,
127.689596183375)) ;
#153245=CARTESIAN_POINT('Ctrl Pts',(-28.6857946550641,14.4299775435325,
127.931754504999)) ;
#153246=CARTESIAN_POINT('Ctrl Pts',(-28.7673480084958,14.503331032243,128.203286809695)) ;
#153247=CARTESIAN_POINT('Ctrl Pts',(-28.8509261449003,14.4992417837061,
128.480336479146)) ;
#153248=CARTESIAN_POINT('Ctrl Pts',(-28.9318023648984,14.4177939822546,
128.749907191947)) ;
#153249=CARTESIAN_POINT('Ctrl Pts',(-29.001910688641,14.2650806147523,128.987818507409)) ;
#153250=CARTESIAN_POINT('Ctrl Pts',(-29.0559489688668,14.0529681509037,
129.178698338362)) ;
#153251=CARTESIAN_POINT('Ctrl Pts',(-29.0896354038435,13.7955270319932,
129.310187588582)) ;
#153252=CARTESIAN_POINT('Ctrl Pts',(-29.099611948193,13.5095709535078,129.372622374006)) ;
#153253=CARTESIAN_POINT('Ctrl Pts',(-29.0842585907111,13.2189036520177,
129.360885383851)) ;
#153254=CARTESIAN_POINT('Ctrl Pts',(-29.0443620584725,12.9437120966298,
129.277345257376)) ;
#153255=CARTESIAN_POINT('Ctrl Pts',(-28.9817282559493,12.7018113312773,
129.127496651977)) ;
#153256=CARTESIAN_POINT('Ctrl Pts',(-28.900103185758,12.5115374792667,128.922195104015)) ;
#153257=CARTESIAN_POINT('Ctrl Pts',(-28.8047562754635,12.3865362509785,
128.676787399727)) ;
#153258=CARTESIAN_POINT('Ctrl Pts',(-28.7012853562746,12.3360647683775,
128.40778833087)) ;
#153259=CARTESIAN_POINT('Ctrl Pts',(-28.5980648305844,12.3630945002041,
128.139111767235)) ;
#153260=CARTESIAN_POINT('Ctrl Pts',(-28.4992221941751,12.4665769548229,
127.883658010127)) ;
#153261=CARTESIAN_POINT('Ctrl Pts',(-28.4131594840602,12.637873730405,127.665272376222)) ;
#153262=CARTESIAN_POINT('Ctrl Pts',(-28.3441687124707,12.8661806742055,
127.496923307267)) ;
#153263=CARTESIAN_POINT('Ctrl Pts',(-28.2971179753842,13.1333277515124,
127.392512752519)) ;
#153264=CARTESIAN_POINT('Ctrl Pts',(-28.2742141661044,13.4221934836715,
127.358771264461)) ;
#153265=CARTESIAN_POINT('Ctrl Pts',(-28.2765820238562,13.7107571318464,
127.398801174816)) ;
#153266=CARTESIAN_POINT('Ctrl Pts',(-28.3034962448371,13.9798563780996,
127.510697252844)) ;
#153267=CARTESIAN_POINT('Ctrl Pts',(-28.3518348917567,14.2070905580459,
127.684913382421)) ;
#153268=CARTESIAN_POINT('Ctrl Pts',(-28.417736051092,14.3790287482914,127.910539859451)) ;
#153269=CARTESIAN_POINT('Ctrl Pts',(-28.4956163030634,14.4826462514907,
128.171126340958)) ;
#153270=CARTESIAN_POINT('Ctrl Pts',(-28.5798455524846,14.5101765749395,
128.450506444325)) ;
#153271=CARTESIAN_POINT('Ctrl Pts',(-28.66200834704,14.4602521093363,128.723409993032)) ;
#153272=CARTESIAN_POINT('Ctrl Pts',(-28.7375813833395,14.3349863303821,
128.977516850491)) ;
#153273=CARTESIAN_POINT('Ctrl Pts',(-28.7985628235098,14.1459036519263,
129.188607444567)) ;
#153274=CARTESIAN_POINT('Ctrl Pts',(-28.8411540818564,13.9042674567381,
129.346179660859)) ;
#153275=CARTESIAN_POINT('Ctrl Pts',(-28.8610016097192,13.6274934121279,
129.437359596521)) ;
#153276=CARTESIAN_POINT('Ctrl Pts',(-28.8560349310886,13.3375401227482,
129.455886266098)) ;
#153277=CARTESIAN_POINT('Ctrl Pts',(-28.8260275084833,13.0529656397982,
129.401339308127)) ;
#153278=CARTESIAN_POINT('Ctrl Pts',(-28.7718240751871,12.793542004979,129.276308893705)) ;
#153279=CARTESIAN_POINT('Ctrl Pts',(-28.69758931411,12.5815361452067,129.09244647551)) ;
#153280=CARTESIAN_POINT('Ctrl Pts',(-28.607191982818,12.4287258471182,128.861490887195)) ;
#153281=CARTESIAN_POINT('Ctrl Pts',(-28.5062114306704,12.3470719994747,
128.599714513405)) ;
#153282=CARTESIAN_POINT('Ctrl Pts',(-28.4016831964791,12.3430683223392,
128.327512526391)) ;
#153283=CARTESIAN_POINT('Ctrl Pts',(-28.3008205475048,12.4155936091128,
128.065797526111)) ;
#153284=CARTESIAN_POINT('Ctrl Pts',(-28.2086887982306,12.5608875783812,
127.829855784513)) ;
#153285=CARTESIAN_POINT('Ctrl Pts',(-28.1322966051425,12.7672957855937,
127.639749496506)) ;
#153286=CARTESIAN_POINT('Ctrl Pts',(-28.0757288054588,13.0219896288371,
127.507742576733)) ;
#153287=CARTESIAN_POINT('Ctrl Pts',(-28.0429540969002,13.3035436342973,
127.44499916588)) ;
#153288=CARTESIAN_POINT('Ctrl Pts',(-28.0350385580784,13.5948422510341,
127.455024273178)) ;
#153289=CARTESIAN_POINT('Ctrl Pts',(-28.0521494910461,13.8739529691167,
127.538171398898)) ;
#153290=CARTESIAN_POINT('Ctrl Pts',(-28.0921989061459,14.1203174233417,
127.688276422386)) ;
#153291=CARTESIAN_POINT('Ctrl Pts',(-28.151557364416,14.3167168643634,127.894769419474)) ;
#153292=CARTESIAN_POINT('Ctrl Pts',(-28.2253962663715,14.4494066861711,
128.14361033343)) ;
#153293=CARTESIAN_POINT('Ctrl Pts',(-28.3077059790347,14.5084702688582,
128.41722565312)) ;
#153294=CARTESIAN_POINT('Ctrl Pts',(-28.3916026412673,14.489700746972,128.695408809309)) ;
#153295=CARTESIAN_POINT('Ctrl Pts',(-28.4706094716546,14.3946106074975,
128.959339303664)) ;
#153296=CARTESIAN_POINT('Ctrl Pts',(-28.5383385063881,14.2294635345246,
129.190381875795)) ;
#153297=CARTESIAN_POINT('Ctrl Pts',(-28.5888615094772,14.0073333887475,
129.371024757805)) ;
#153298=CARTESIAN_POINT('Ctrl Pts',(-28.6182752167583,13.7435828448799,
129.490009369002)) ;
#153299=CARTESIAN_POINT('Ctrl Pts',(-28.6235344183767,13.454824745877,129.538667492509)) ;
#153300=CARTESIAN_POINT('Ctrl Pts',(-28.6035941708859,13.1663898496403,
129.513405963783)) ;
#153301=CARTESIAN_POINT('Ctrl Pts',(-28.5591016772346,12.8948251888563,
129.416595319443)) ;
#153302=CARTESIAN_POINT('Ctrl Pts',(-28.4924613979654,12.6613614393991,
129.255069109059)) ;
#153303=CARTESIAN_POINT('Ctrl Pts',(-28.4079858158223,12.4827884864443,
129.041374692839)) ;
#153304=CARTESIAN_POINT('Ctrl Pts',(-28.3106810095428,12.3713198999723,
128.790256537741)) ;
#153305=CARTESIAN_POINT('Ctrl Pts',(-28.2071142233906,12.3351536539427,
128.520782151597)) ;
#153306=CARTESIAN_POINT('Ctrl Pts',(-28.1033170651269,12.3771106003778,
128.250789621036)) ;
#153307=CARTESIAN_POINT('Ctrl Pts',(-28.0070122936131,12.493746042562,128.002507073001)) ;
#153308=CARTESIAN_POINT('Ctrl Pts',(-27.9236042223444,12.6767291405437,
127.791947198724)) ;
#153309=CARTESIAN_POINT('Ctrl Pts',(-27.8582788554542,12.9147362953278,
127.634399931538)) ;
#153310=CARTESIAN_POINT('Ctrl Pts',(-27.8157639814054,13.1870897175325,
127.543206911709)) ;
#153311=CARTESIAN_POINT('Ctrl Pts',(-27.7976113632335,13.4771402294594,
127.523294837643)) ;
#153312=CARTESIAN_POINT('Ctrl Pts',(-27.8047562191335,13.7642376991577,
127.577383148529)) ;
#153313=CARTESIAN_POINT('Ctrl Pts',(-27.8359687279842,14.0261140050281,
127.701710177171)) ;
#153314=CARTESIAN_POINT('Ctrl Pts',(-27.8877875139809,14.2437566095146,
127.886037495367)) ;
#153315=CARTESIAN_POINT('Ctrl Pts',(-27.9566643830394,14.4043004510961,
128.12048462873)) ;
#153316=CARTESIAN_POINT('Ctrl Pts',(-28.0360570915207,14.4936451763547,
128.385451901082)) ;
#153317=CARTESIAN_POINT('Ctrl Pts',(-28.120129115805,14.5067755223083,128.664180642723)) ;
#153318=CARTESIAN_POINT('Ctrl Pts',(-28.2020346856407,14.4421251633059,
128.936606880987)) ;
#153319=CARTESIAN_POINT('Ctrl Pts',(-28.2751125216823,14.3039891726026,
129.183284767789)) ;
#153320=CARTESIAN_POINT('Ctrl Pts',(-28.3330260630189,14.1040922169467,
129.385445944809)) ;
#153321=CARTESIAN_POINT('Ctrl Pts',(-28.3716774412633,13.8535852347893,
129.531620171577)) ;
#153322=CARTESIAN_POINT('Ctrl Pts',(-28.3868553207156,13.5730952435811,
129.609080622274)) ;
#153323=CARTESIAN_POINT('Ctrl Pts',(-28.3771751540194,13.2829861782011,
129.613807074417)) ;
#153324=CARTESIAN_POINT('Ctrl Pts',(-28.3425095932928,13.0017737284941,
129.545666888846)) ;
#153325=CARTESIAN_POINT('Ctrl Pts',(-28.284301937165,12.7500890797144,129.408856898039)) ;
#153326=CARTESIAN_POINT('Ctrl Pts',(-28.2064572920802,12.5475577998432,
129.214559307957)) ;
#153327=CARTESIAN_POINT('Ctrl Pts',(-28.1135171544018,12.4075652478031,
128.976210428243)) ;
#153328=CARTESIAN_POINT('Ctrl Pts',(-28.0118850220544,12.3405227377109,
128.712349934362)) ;
#153329=CARTESIAN_POINT('Ctrl Pts',(-27.9073393263242,12.3506975715296,
128.440115510787)) ;
#153330=CARTESIAN_POINT('Ctrl Pts',(-27.8069898708441,12.438177489278,128.180166701549)) ;
#153331=CARTESIAN_POINT('Ctrl Pts',(-27.7177045614419,12.5958827964123,
127.952426644854)) ;
#153332=CARTESIAN_POINT('Ctrl Pts',(-27.6448174995369,12.8123887822574,
127.772559198421)) ;
#153333=CARTESIAN_POINT('Ctrl Pts',(-27.5925658802496,13.0732934241726,
127.653072879261)) ;
#153334=CARTESIAN_POINT('Ctrl Pts',(-27.5643119574423,13.3601444544887,
127.603779546763)) ;
#153335=CARTESIAN_POINT('Ctrl Pts',(-27.5613082454556,13.6487324697402,
127.627925538602)) ;
#153336=CARTESIAN_POINT('Ctrl Pts',(-27.5828722691528,13.9231969052117,
127.724074394844)) ;
#153337=CARTESIAN_POINT('Ctrl Pts',(-27.6269024064909,14.1616648845749,
127.885829090303)) ;
#153338=CARTESIAN_POINT('Ctrl Pts',(-27.6896598747405,14.3474885130478,
128.102376258084)) ;
#153339=CARTESIAN_POINT('Ctrl Pts',(-27.7653992680876,14.4664584587802,
128.356681964705)) ;
#153340=CARTESIAN_POINT('Ctrl Pts',(-27.8487981620875,14.5109046603937,
128.633576137683)) ;
#153341=CARTESIAN_POINT('Ctrl Pts',(-27.9318850392023,14.477538406395,128.909237750788)) ;
#153342=CARTESIAN_POINT('Ctrl Pts',(-28.0095052256554,14.3681997132881,
129.169245881706)) ;
#153343=CARTESIAN_POINT('Ctrl Pts',(-28.0741401659524,14.19161807787,129.391120281656)) ;
#153344=CARTESIAN_POINT('Ctrl Pts',(-28.1210449004513,13.9603524956053,
129.561209556167)) ;
#153345=CARTESIAN_POINT('Ctrl Pts',(-28.1460961632202,13.6895220911817,
129.667588782595)) ;
#153346=CARTESIAN_POINT('Ctrl Pts',(-28.1465838645101,13.4007319641459,
129.702076763037)) ;
#153347=CARTESIAN_POINT('Ctrl Pts',(-28.1219792750298,13.1132078283894,
129.663296512428)) ;
#153348=CARTESIAN_POINT('Ctrl Pts',(-28.072797303837,12.8466068578935,129.552900494661)) ;
#153349=CARTESIAN_POINT('Ctrl Pts',(-28.0028760663637,12.6236984730367,
129.381571768306)) ;
#153350=CARTESIAN_POINT('Ctrl Pts',(-27.9152289217031,12.4561011970055,
129.15875880179)) ;
#153351=CARTESIAN_POINT('Ctrl Pts',(-27.8163074914158,12.3585968124196,
128.902876316079)) ;
#153352=CARTESIAN_POINT('Ctrl Pts',(-27.7120492591559,12.3371246735504,
128.631455165304)) ;
#153353=CARTESIAN_POINT('Ctrl Pts',(-27.6093731664381,12.3935413485491,
128.364635405542)) ;
#153354=CARTESIAN_POINT('Ctrl Pts',(-27.5149001295544,12.5236723848828,
128.121769416389)) ;
#153355=CARTESIAN_POINT('Ctrl Pts',(-27.4346201824783,12.7179304240541,
127.920341279588)) ;
#153356=CARTESIAN_POINT('Ctrl Pts',(-27.3732833708595,12.9643000603806,
127.774449881944)) ;
#153357=CARTESIAN_POINT('Ctrl Pts',(-27.3353218805088,13.2410161239663,
127.696515666237)) ;
#153358=CARTESIAN_POINT('Ctrl Pts',(-27.3219345106549,13.5320326358814,
127.690536193544)) ;
#153359=CARTESIAN_POINT('Ctrl Pts',(-27.3336868555628,13.8151976332958,
127.757981771659)) ;
#153360=CARTESIAN_POINT('Ctrl Pts',(-27.3691045396702,14.070965110173,127.894657472177)) ;
#153361=CARTESIAN_POINT('Ctrl Pts',(-27.4247538548607,14.2795161854134,
128.090342542637)) ;
#153362=CARTESIAN_POINT('Ctrl Pts',(-27.495823154164,14.4266233568165,128.331023842141)) ;
#153363=CARTESIAN_POINT('Ctrl Pts',(-27.5766922115291,14.5021444966585,
128.600366276399)) ;
#153364=CARTESIAN_POINT('Ctrl Pts',(-27.6609223179021,14.5004799279669,
128.8795751742)) ;
#153365=CARTESIAN_POINT('Ctrl Pts',(-27.7417671934519,14.4210758361391,
129.14896837329)) ;
#153366=CARTESIAN_POINT('Ctrl Pts',(-27.8120265768946,14.2711637356508,
129.38719326095)) ;
#153367=CARTESIAN_POINT('Ctrl Pts',(-27.866891762874,14.0600320259714,129.580611011308)) ;
#153368=CARTESIAN_POINT('Ctrl Pts',(-27.9012411174026,13.8025046463563,
129.714162963611)) ;
#153369=CARTESIAN_POINT('Ctrl Pts',(-27.9118652501947,13.5194350300881,
129.778210865001)) ;
#153370=CARTESIAN_POINT('Ctrl Pts',(-27.8973675127668,13.227929848522,129.769057927685)) ;
#153371=CARTESIAN_POINT('Ctrl Pts',(-27.8581217638387,12.9514279979351,
129.687479679852)) ;
#153372=CARTESIAN_POINT('Ctrl Pts',(-27.7958487933346,12.7076270254922,
129.538792895781)) ;
#153373=CARTESIAN_POINT('Ctrl Pts',(-27.7150442368328,12.5164543914562,
129.335744778992)) ;
#153374=CARTESIAN_POINT('Ctrl Pts',(-27.6197799723084,12.3891143889345,
129.090666143106)) ;
#153375=CARTESIAN_POINT('Ctrl Pts',(-27.5169840616899,12.3364756158918,
128.823462340777)) ;
#153376=CARTESIAN_POINT('Ctrl Pts',(-27.4129425204162,12.3612642231578,
128.552629149903)) ;
#153377=CARTESIAN_POINT('Ctrl Pts',(-27.3139116309648,12.4629838840005,
128.296612691349)) ;
#153378=CARTESIAN_POINT('Ctrl Pts',(-27.2276350555539,12.6321971699934,
128.077535896234)) ;
#153379=CARTESIAN_POINT('Ctrl Pts',(-27.1581753164316,12.8584558798932,
127.907740199772)) ;
#153380=CARTESIAN_POINT('Ctrl Pts',(-27.1102193532803,13.1261648647243,
127.800864060768)) ;
#153381=CARTESIAN_POINT('Ctrl Pts',(-27.0867427780488,13.4141234552309,
127.765371910168)) ;
#153382=CARTESIAN_POINT('Ctrl Pts',(-27.088405263082,13.7023852342343,127.803282253112)) ;
#153383=CARTESIAN_POINT('Ctrl Pts',(-27.1144094066955,13.9714212012371,
127.912378068659)) ;
#153384=CARTESIAN_POINT('Ctrl Pts',(-27.1625636190418,14.202020081249,128.086338189894)) ;
#153385=CARTESIAN_POINT('Ctrl Pts',(-27.2279041571622,14.3750071736422,
128.310222999053)) ;
#153386=CARTESIAN_POINT('Ctrl Pts',(-27.3055089641359,14.4806351346196,
128.570006270221)) ;
#153387=CARTESIAN_POINT('Ctrl Pts',(-27.3892702869014,14.5105855297535,
128.847858683373)) ;
#153388=CARTESIAN_POINT('Ctrl Pts',(-27.4721256647169,14.4625550657111,
129.123019817885)) ;
#153389=CARTESIAN_POINT('Ctrl Pts',(-27.5475424958297,14.3400369417443,
129.376461860258)) ;
#153390=CARTESIAN_POINT('Ctrl Pts',(-27.6092868870231,14.1521957535254,
129.589908595948)) ;
#153391=CARTESIAN_POINT('Ctrl Pts',(-27.6524549950664,13.9116489154345,
129.749173070005)) ;
#153392=CARTESIAN_POINT('Ctrl Pts',(-27.6729767158619,13.6358544266559,
129.842295420114)) ;
#153393=CARTESIAN_POINT('Ctrl Pts',(-27.6687686357343,13.3459427675745,
129.863045715734)) ;
#153394=CARTESIAN_POINT('Ctrl Pts',(-27.6393546558192,13.0604649745041,
129.810291983176)) ;
#153395=CARTESIAN_POINT('Ctrl Pts',(-27.5861749748563,12.8015143832803,
129.688047174148)) ;
#153396=CARTESIAN_POINT('Ctrl Pts',(-27.5122453552566,12.586871423154,129.505215644939)) ;
#153397=CARTESIAN_POINT('Ctrl Pts',(-27.4222257102063,12.4323032180318,
129.275353955494)) ;
#153398=CARTESIAN_POINT('Ctrl Pts',(-27.321814640165,12.348604012381,129.015131363742)) ;
#153399=CARTESIAN_POINT('Ctrl Pts',(-27.2172646277251,12.3418345254331,
128.742874357153)) ;
#153400=CARTESIAN_POINT('Ctrl Pts',(-27.1155991989799,12.4127257697425,
128.479021774659)) ;
#153401=CARTESIAN_POINT('Ctrl Pts',(-27.0235546029965,12.5554430365515,
128.24317434018)) ;
#153402=CARTESIAN_POINT('Ctrl Pts',(-26.946364611968,12.7608029240068,128.050846584327)) ;
#153403=CARTESIAN_POINT('Ctrl Pts',(-26.8892425932522,13.0143079229722,
127.917197312737)) ;
#153404=CARTESIAN_POINT('Ctrl Pts',(-26.8557397574038,13.2953661026702,
127.852335782128)) ;
#153405=CARTESIAN_POINT('Ctrl Pts',(-26.8471237684322,13.587499191953,127.86040257377)) ;
#153406=CARTESIAN_POINT('Ctrl Pts',(-26.8636409106043,13.8669338626205,
127.941791701437)) ;
#153407=CARTESIAN_POINT('Ctrl Pts',(-26.9028894020443,14.1134263503453,
128.089413302891)) ;
#153408=CARTESIAN_POINT('Ctrl Pts',(-26.9618864660315,14.3121780897716,
128.294946112899)) ;
#153409=CARTESIAN_POINT('Ctrl Pts',(-27.0356609756341,14.4470050265316,
128.543696981495)) ;
#153410=CARTESIAN_POINT('Ctrl Pts',(-27.1176846698481,14.5078086325279,
128.816414339099)) ;
#153411=CARTESIAN_POINT('Ctrl Pts',(-27.2013501944063,14.4913412737729,
129.093814747738)) ;
#153412=CARTESIAN_POINT('Ctrl Pts',(-27.2805727554514,14.3985299043882,
129.358365317732)) ;
#153413=CARTESIAN_POINT('Ctrl Pts',(-27.3487809879748,14.2353764928408,
129.590815975098)) ;
#153414=CARTESIAN_POINT('Ctrl Pts',(-27.4000923756535,14.0132824388172,
129.773951949604)) ;
#153415=CARTESIAN_POINT('Ctrl Pts',(-27.4299031588905,13.751770584179,129.893917739675)) ;
#153416=CARTESIAN_POINT('Ctrl Pts',(-27.4360065328396,13.4639004603942,
129.944990740374)) ;
#153417=CARTESIAN_POINT('Ctrl Pts',(-27.4166194504997,13.1736259559936,
129.921533138526)) ;
#153418=CARTESIAN_POINT('Ctrl Pts',(-27.3730557967721,12.9029494351804,
129.827230137503)) ;
#153419=CARTESIAN_POINT('Ctrl Pts',(-27.3068239081708,12.6670694829694,
129.667025348139)) ;
#153420=CARTESIAN_POINT('Ctrl Pts',(-27.2225807375648,12.4867414535482,
129.454064281963)) ;
#153421=CARTESIAN_POINT('Ctrl Pts',(-27.1260163205075,12.3736046950475,
129.204955161642)) ;
#153422=CARTESIAN_POINT('Ctrl Pts',(-27.0219531940928,12.3351061359291,
128.934221171249)) ;
#153423=CARTESIAN_POINT('Ctrl Pts',(-26.9187654991147,12.3747297412366,
128.665782677207)) ;
#153424=CARTESIAN_POINT('Ctrl Pts',(-26.8219192185406,12.4890530273647,
128.415981781108)) ;
#153425=CARTESIAN_POINT('Ctrl Pts',(-26.7375618368722,12.6718473822343,
128.20287552548)) ;
#153426=CARTESIAN_POINT('Ctrl Pts',(-26.6721408995713,12.9071471042355,
128.044830293244)) ;
#153427=CARTESIAN_POINT('Ctrl Pts',(-26.6288268693924,13.1791583633753,
127.951366546025)) ;
#153428=CARTESIAN_POINT('Ctrl Pts',(-26.6100146219695,13.4685703303894,
127.929472625113)) ;
#153429=CARTESIAN_POINT('Ctrl Pts',(-26.6163965606096,13.7556865610863,
127.981289936006)) ;
#153430=CARTESIAN_POINT('Ctrl Pts',(-26.6468365176563,14.0184520779736,
128.103328446011)) ;
#153431=CARTESIAN_POINT('Ctrl Pts',(-26.6983664732469,14.2386835545227,
128.286981099105)) ;
#153432=CARTESIAN_POINT('Ctrl Pts',(-26.7668561678463,14.4009245247973,
128.520283146029)) ;
#153433=CARTESIAN_POINT('Ctrl Pts',(-26.8462801396179,14.4923209079493,
128.785440445302)) ;
#153434=CARTESIAN_POINT('Ctrl Pts',(-26.9299042318789,14.5074993821674,
129.062691208225)) ;
#153435=CARTESIAN_POINT('Ctrl Pts',(-27.0123042045344,14.4446391320812,
129.336708219525)) ;
#153436=CARTESIAN_POINT('Ctrl Pts',(-27.0853285109314,14.309013886893,129.583057807955)) ;
#153437=CARTESIAN_POINT('Ctrl Pts',(-27.1438828659143,14.1104149351794,
129.787163074108)) ;
#153438=CARTESIAN_POINT('Ctrl Pts',(-27.1830524640317,13.8614588559076,
129.934789891105)) ;
#153439=CARTESIAN_POINT('Ctrl Pts',(-27.1989887778394,13.5819687002437,
130.014428956727)) ;
#153440=CARTESIAN_POINT('Ctrl Pts',(-27.1899960665713,13.2906279013141,
130.021303572167)) ;
#153441=CARTESIAN_POINT('Ctrl Pts',(-27.1559614540415,13.009243305788,129.95497149067)) ;
#153442=CARTESIAN_POINT('Ctrl Pts',(-27.0987240639522,12.7575168112921,
129.820836098485)) ;
#153443=CARTESIAN_POINT('Ctrl Pts',(-27.0211347642334,12.5525240138587,
129.627409702748)) ;
#153444=CARTESIAN_POINT('Ctrl Pts',(-26.9288019853003,12.4108770336832,
129.390743830787)) ;
#153445=CARTESIAN_POINT('Ctrl Pts',(-26.8269925769389,12.3412909140522,
129.126483822534)) ;
#153446=CARTESIAN_POINT('Ctrl Pts',(-26.7225678003105,12.3493861735078,
128.854556329981)) ;
#153447=CARTESIAN_POINT('Ctrl Pts',(-26.6222736426069,12.4342727909203,
128.594675298208)) ;
#153448=CARTESIAN_POINT('Ctrl Pts',(-26.5324245140866,12.5900489009072,
128.365332500197)) ;
#153449=CARTESIAN_POINT('Ctrl Pts',(-26.4587946173494,12.8056265995217,
128.183382042886)) ;
#153450=CARTESIAN_POINT('Ctrl Pts',(-26.4059966216722,13.0653848746049,
128.062274396553)) ;
#153451=CARTESIAN_POINT('Ctrl Pts',(-26.3770384247468,13.3504851063388,
128.01077693268)) ;
#153452=CARTESIAN_POINT('Ctrl Pts',(-26.3732580768289,13.6412798147236,
128.032889399786)) ;
#153453=CARTESIAN_POINT('Ctrl Pts',(-26.3941468859038,13.915548156852,128.126957619226)) ;
#153454=CARTESIAN_POINT('Ctrl Pts',(-26.4375236270793,14.1552942040558,
128.286796725341)) ;
#153455=CARTESIAN_POINT('Ctrl Pts',(-26.499786802166,14.3429101935435,128.501891901076)) ;
#153456=CARTESIAN_POINT('Ctrl Pts',(-26.5753221744753,14.4639893047867,
128.755644371512)) ;
#153457=CARTESIAN_POINT('Ctrl Pts',(-26.658258796401,14.5107279953385,129.031049167775)) ;
#153458=CARTESIAN_POINT('Ctrl Pts',(-26.7418770326506,14.4794893752074,
129.308446128137)) ;
#153459=CARTESIAN_POINT('Ctrl Pts',(-26.819410154467,14.3727211578977,129.56804219168)) ;
#153460=CARTESIAN_POINT('Ctrl Pts',(-26.884660652684,14.1977799584113,129.791786901947)) ;
#153461=CARTESIAN_POINT('Ctrl Pts',(-26.9321606344241,13.9680803032242,
129.963592933574)) ;
#153462=CARTESIAN_POINT('Ctrl Pts',(-26.9579703404882,13.6967826933105,
130.072347583536)) ;
#153463=CARTESIAN_POINT('Ctrl Pts',(-26.9591310030642,13.4094043760888,
130.108663362794)) ;
#153464=CARTESIAN_POINT('Ctrl Pts',(-26.935231210856,13.1212039321583,130.071985580596)) ;
#153465=CARTESIAN_POINT('Ctrl Pts',(-26.8869426549206,12.8546896237207,
129.964066829109)) ;
#153466=CARTESIAN_POINT('Ctrl Pts',(-26.8174482093006,12.6293810356165,
129.794091823838)) ;
#153467=CARTESIAN_POINT('Ctrl Pts',(-26.7297563031988,12.4594635396626,
129.571300039305)) ;
#153468=CARTESIAN_POINT('Ctrl Pts',(-26.6315768169788,12.3604529302704,
129.317412505758)) ;
#153469=CARTESIAN_POINT('Ctrl Pts',(-26.527041677516,12.3366695079855,129.045292118923)) ;
#153470=CARTESIAN_POINT('Ctrl Pts',(-26.4246632418904,12.3907630606801,
128.779202667163)) ;
#153471=CARTESIAN_POINT('Ctrl Pts',(-26.3296624090555,12.5187717527639,
128.534846855937)) ;
#153472=CARTESIAN_POINT('Ctrl Pts',(-26.2486292653153,12.7125553045139,
128.331370691531)) ;
#153473=CARTESIAN_POINT('Ctrl Pts',(-26.187290463919,12.9551208485313,128.185129058602)) ;
#153474=CARTESIAN_POINT('Ctrl Pts',(-26.1482420973643,13.2325620060974,
128.104210130242)) ;
#153475=CARTESIAN_POINT('Ctrl Pts',(-26.1341913899476,13.5243419796884,
128.096383572714)) ;
#153476=CARTESIAN_POINT('Ctrl Pts',(-26.1452118388481,13.8069926528057,
128.161574113629)) ;
#153477=CARTESIAN_POINT('Ctrl Pts',(-26.1799390075941,14.0639000199269,
128.296232665471)) ;
#153478=CARTESIAN_POINT('Ctrl Pts',(-26.2350489546991,14.2741558930926,
128.490347023028)) ;
#153479=CARTESIAN_POINT('Ctrl Pts',(-26.3059077450582,14.4234615625839,
128.730487186166)) ;
#153480=CARTESIAN_POINT('Ctrl Pts',(-26.386494169588,14.5011170686614,128.998961276038)) ;
#153481=CARTESIAN_POINT('Ctrl Pts',(-26.4710372754606,14.5013614779113,
129.279215621043)) ;
#153482=CARTESIAN_POINT('Ctrl Pts',(-26.5513450363698,14.4249956630962,
129.546727763435)) ;
#153483=CARTESIAN_POINT('Ctrl Pts',(-26.6226216620681,14.2760171565871,
129.788206158856)) ;
#153484=CARTESIAN_POINT('Ctrl Pts',(-26.6777858163634,14.0665442400002,
129.982426179449)) ;
#153485=CARTESIAN_POINT('Ctrl Pts',(-26.7127743428566,13.8110528410318,
130.117741076645)) ;
#153486=CARTESIAN_POINT('Ctrl Pts',(-26.7241069347589,13.5262786463887,
130.184114351317)) ;
#153487=CARTESIAN_POINT('Ctrl Pts',(-26.7103978253846,13.2368369901033,
130.177011615775)) ;
#153488=CARTESIAN_POINT('Ctrl Pts',(-26.6716560461567,12.9583255903659,
130.097075764209)) ;
#153489=CARTESIAN_POINT('Ctrl Pts',(-26.6103674672222,12.7145800096232,
129.95106877123)) ;
#153490=CARTESIAN_POINT('Ctrl Pts',(-26.5292783226885,12.5201730384604,
129.747494551372)) ;
#153491=CARTESIAN_POINT('Ctrl Pts',(-26.4353195353877,12.392297716127,129.505869698294)) ;
#153492=CARTESIAN_POINT('Ctrl Pts',(-26.3321003131888,12.3368042043637,
129.23762472755)) ;
#153493=CARTESIAN_POINT('Ctrl Pts',(-26.2283359448761,12.3594079574846,
128.967488898529)) ;
#153494=CARTESIAN_POINT('Ctrl Pts',(-26.1289374320057,12.4588426243277,
128.710432008687)) ;
#153495=CARTESIAN_POINT('Ctrl Pts',(-26.0421433826271,12.6263832935465,
128.489874381818)) ;
#153496=CARTESIAN_POINT('Ctrl Pts',(-25.9721170036289,12.8513078071139,
128.318433909601)) ;
#153497=CARTESIAN_POINT('Ctrl Pts',(-25.9235411833855,13.1175341941134,
128.209680256936)) ;
#153498=CARTESIAN_POINT('Ctrl Pts',(-25.8992723616796,13.4059954970849,
128.171974342421)) ;
#153499=CARTESIAN_POINT('Ctrl Pts',(-25.9001789667653,13.6942419645787,
128.207632461566)) ;
#153500=CARTESIAN_POINT('Ctrl Pts',(-25.9258216003677,13.9656571359195,
128.31589284879)) ;
#153501=CARTESIAN_POINT('Ctrl Pts',(-25.9727492712161,14.1945698215837,
128.485818180082)) ;
#153502=CARTESIAN_POINT('Ctrl Pts',(-26.0380351219601,14.3711224528334,
128.709801837872)) ;
#153503=CARTESIAN_POINT('Ctrl Pts',(-26.115372034482,14.4785950091488,128.968780330961)) ;
#153504=CARTESIAN_POINT('Ctrl Pts',(-26.1991386228248,14.5108133112394,
129.246686766249)) ;
#153505=CARTESIAN_POINT('Ctrl Pts',(-26.281961118953,14.4650394200622,129.521689731091)) ;
#153506=CARTESIAN_POINT('Ctrl Pts',(-26.3576691539897,14.3446919400874,
129.775975443665)) ;
#153507=CARTESIAN_POINT('Ctrl Pts',(-26.4199450377268,14.1586507898245,
129.990981699106)) ;
#153508=CARTESIAN_POINT('Ctrl Pts',(-26.4638325348643,13.9182142591253,
130.152493567261)) ;
#153509=CARTESIAN_POINT('Ctrl Pts',(-26.4849121372087,13.6446894301756,
130.247054976681)) ;
#153510=CARTESIAN_POINT('Ctrl Pts',(-26.4814409395297,13.3538163555555,
130.270090586414)) ;
#153511=CARTESIAN_POINT('Ctrl Pts',(-26.4527946492839,13.0687529323482,
130.219476965581)) ;
#153512=CARTESIAN_POINT('Ctrl Pts',(-26.4002320096581,12.8084025711039,
130.099079794229)) ;
#153513=CARTESIAN_POINT('Ctrl Pts',(-26.3268756685072,12.5923662507696,
129.91790410308)) ;
#153514=CARTESIAN_POINT('Ctrl Pts',(-26.2371123368209,12.4355966936421,
129.688843066008)) ;
#153515=CARTESIAN_POINT('Ctrl Pts',(-26.1367181878628,12.3498834173245,
129.42872587461)) ;
#153516=CARTESIAN_POINT('Ctrl Pts',(-26.032722719753,12.3409542808635,129.157919642926)) ;
#153517=CARTESIAN_POINT('Ctrl Pts',(-25.9308084387583,12.4093757248112,
128.893357587352)) ;
#153518=CARTESIAN_POINT('Ctrl Pts',(-25.838155620905,12.5505196315372,128.655821078007)) ;
#153519=CARTESIAN_POINT('Ctrl Pts',(-25.7605740007468,12.7541803006072,
128.462316845571)) ;
#153520=CARTESIAN_POINT('Ctrl Pts',(-25.7029450253967,13.0055267425044,
128.327067990315)) ;
#153521=CARTESIAN_POINT('Ctrl Pts',(-25.6685657347824,13.2870724884799,
128.259776019344)) ;
#153522=CARTESIAN_POINT('Ctrl Pts',(-25.6592502061655,13.5781354317469,
128.265673438089)) ;
#153523=CARTESIAN_POINT('Ctrl Pts',(-25.6749179654199,13.8583662507443,
128.344586199981)) ;
#153524=CARTESIAN_POINT('Ctrl Pts',(-25.7137374162889,14.1072755060793,
128.491117013587)) ;
#153525=CARTESIAN_POINT('Ctrl Pts',(-25.7721169966564,14.3069765889331,
128.694755702354)) ;
#153526=CARTESIAN_POINT('Ctrl Pts',(-25.845207577047,14.443614067786,128.941381531894)) ;
#153527=CARTESIAN_POINT('Ctrl Pts',(-25.9273346325596,14.5071928082345,
129.214515131727)) ;
#153528=CARTESIAN_POINT('Ctrl Pts',(-26.011234962119,14.4928945220509,129.492675842775)) ;
#153529=CARTESIAN_POINT('Ctrl Pts',(-26.0906570279007,14.4021254936154,
129.757803067043)) ;
#153530=CARTESIAN_POINT('Ctrl Pts',(-26.159082383682,14.2413770477371,129.990792154917)) ;
#153531=CARTESIAN_POINT('Ctrl Pts',(-26.2110152100895,14.0210258594474,
130.175736142196)) ;
#153532=CARTESIAN_POINT('Ctrl Pts',(-26.241635177827,13.7594508415378,130.298196601018)) ;
#153533=CARTESIAN_POINT('Ctrl Pts',(-26.2483473113095,13.4716753030503,
130.351078692086)) ;
#153534=CARTESIAN_POINT('Ctrl Pts',(-26.2298541426232,13.18278007244,130.330045835803)) ;
#153535=CARTESIAN_POINT('Ctrl Pts',(-26.1867418068547,12.9097866347109,
130.237249070666)) ;
#153536=CARTESIAN_POINT('Ctrl Pts',(-26.1214552754847,12.6739761120234,
130.079613973061)) ;
#153537=CARTESIAN_POINT('Ctrl Pts',(-26.037598712626,12.4911376353209,129.867849268882)) ;
#153538=CARTESIAN_POINT('Ctrl Pts',(-25.9407649580424,12.3755758788311,
129.618129131331)) ;
#153539=CARTESIAN_POINT('Ctrl Pts',(-25.8374214950217,12.3352662329562,
129.34929906656)) ;
#153540=CARTESIAN_POINT('Ctrl Pts',(-25.7340098362028,12.3722006143293,
129.0802369826)) ;
#153541=CARTESIAN_POINT('Ctrl Pts',(-25.6361773432197,12.4858118722087,
128.827819165484)) ;
#153542=CARTESIAN_POINT('Ctrl Pts',(-25.5523274084712,12.6649628027199,
128.615825895545)) ;
#153543=CARTESIAN_POINT('Ctrl Pts',(-25.4859513870995,12.8995424291904,
128.455121245363)) ;
#153544=CARTESIAN_POINT('Ctrl Pts',(-25.4419863750333,13.1707489990253,
128.359746169264)) ;
#153545=CARTESIAN_POINT('Ctrl Pts',(-25.4224009992562,13.4602465419289,
128.335630931104)) ;
#153546=CARTESIAN_POINT('Ctrl Pts',(-25.4281061795563,13.7479094104328,
128.385491263721)) ;
#153547=CARTESIAN_POINT('Ctrl Pts',(-25.4578216450762,14.0110933638022,
128.505345635233)) ;
#153548=CARTESIAN_POINT('Ctrl Pts',(-25.5087967768197,14.2330195298938,
128.687396943834)) ;
#153549=CARTESIAN_POINT('Ctrl Pts',(-25.5768933622651,14.397056415232,128.919554215411)) ;
#153550=CARTESIAN_POINT('Ctrl Pts',(-25.6558147544988,14.4906410938832,
129.183138561615)) ;
#153551=CARTESIAN_POINT('Ctrl Pts',(-25.7399301950195,14.5080280130628,
129.462041474598)) ;
#153552=CARTESIAN_POINT('Ctrl Pts',(-25.8217364878674,14.4480725424633,
129.734011003358)) ;
#153553=CARTESIAN_POINT('Ctrl Pts',(-25.8956483813608,14.3139470607326,
129.983179734343)) ;
#153554=CARTESIAN_POINT('Ctrl Pts',(-25.9546615112484,14.1169437524237,
130.188609280051)) ;
#153555=CARTESIAN_POINT('Ctrl Pts',(-25.994519421204,13.8684682048696,130.338337741358)) ;
#153556=CARTESIAN_POINT('Ctrl Pts',(-26.0110568377318,13.5907243651,130.419594305655)) ;
#153557=CARTESIAN_POINT('Ctrl Pts',(-26.0028570943019,13.2994062522709,
130.428791647391)) ;
#153558=CARTESIAN_POINT('Ctrl Pts',(-25.9695704025357,13.0173302811176,
130.364651136717)) ;
#153559=CARTESIAN_POINT('Ctrl Pts',(-25.9127012517306,12.7634586998748,
130.23173138777)) ;
#153560=CARTESIAN_POINT('Ctrl Pts',(-25.8356694959319,12.5574053612187,
130.039883250671)) ;
#153561=CARTESIAN_POINT('Ctrl Pts',(-25.7439581375389,12.4141338116398,
129.804942699892)) ;
#153562=CARTESIAN_POINT('Ctrl Pts',(-25.6422361078924,12.342233208706,129.540970477651)) ;
#153563=CARTESIAN_POINT('Ctrl Pts',(-25.5379082160016,12.3479816385131,
129.269286803224)) ;
#153564=CARTESIAN_POINT('Ctrl Pts',(-25.4372492426153,12.4308508598937,
129.00839512309)) ;
#153565=CARTESIAN_POINT('Ctrl Pts',(-25.3472402005208,12.5841342714032,
128.778486490676)) ;
#153566=CARTESIAN_POINT('Ctrl Pts',(-25.272730898508,12.7991564308112,128.594122402279)) ;
#153567=CARTESIAN_POINT('Ctrl Pts',(-25.2194888387276,13.0569999610756,
128.471595214616)) ;
#153568=CARTESIAN_POINT('Ctrl Pts',(-25.1897401476562,13.3421921034464,
128.417860044275)) ;
#153569=CARTESIAN_POINT('Ctrl Pts',(-25.1851966857885,13.6321454574867,
128.437625751363)) ;
#153570=CARTESIAN_POINT('Ctrl Pts',(-25.2054882351433,13.9089725412032,
128.530163374861)) ;
#153571=CARTESIAN_POINT('Ctrl Pts',(-25.2484501051326,14.1498188340954,
128.688812325716)) ;
#153572=CARTESIAN_POINT('Ctrl Pts',(-25.3098239459612,14.3379335225619,
128.901090604678)) ;
#153573=CARTESIAN_POINT('Ctrl Pts',(-25.3852409841119,14.4615825769609,
129.154594863581)) ;
#153574=CARTESIAN_POINT('Ctrl Pts',(-25.4680078103566,14.5104718339952,
129.429479188798)) ;
#153575=CARTESIAN_POINT('Ctrl Pts',(-25.5519233175472,14.4813917081873,
129.707831723369)) ;
#153576=CARTESIAN_POINT('Ctrl Pts',(-25.6296594879759,14.3764101476522,
129.968016081421)) ;
#153577=CARTESIAN_POINT('Ctrl Pts',(-25.6951131634194,14.2041613001764,
130.192211432841)) ;
#153578=CARTESIAN_POINT('Ctrl Pts',(-25.7434116042681,13.9743839791119,
130.36655070585)) ;
#153579=CARTESIAN_POINT('Ctrl Pts',(-25.7697062526325,13.7063210401926,
130.476427371815)) ;
#153580=CARTESIAN_POINT('Ctrl Pts',(-25.7716643333024,13.416701167449,130.515370896243)) ;
#153581=CARTESIAN_POINT('Ctrl Pts',(-25.7484303453548,13.1291677758352,
130.480525076402)) ;
#153582=CARTESIAN_POINT('Ctrl Pts',(-25.7008468729498,12.86171027905,130.374668312212)) ;
#153583=CARTESIAN_POINT('Ctrl Pts',(-25.6318421414092,12.6350478480017,
130.206135995294)) ;
#153584=CARTESIAN_POINT('Ctrl Pts',(-25.5450073178082,12.4638699665219,
129.985698129429)) ;
#153585=CARTESIAN_POINT('Ctrl Pts',(-25.4465855133018,12.3621126869917,
129.731275230113)) ;
#153586=CARTESIAN_POINT('Ctrl Pts',(-25.3422723144961,12.336288293437,129.459748523319)) ;
#153587=CARTESIAN_POINT('Ctrl Pts',(-25.2395464146887,12.3882079133966,
129.192710014154)) ;
#153588=CARTESIAN_POINT('Ctrl Pts',(-25.1441554739243,12.5148240028862,
128.947268201873)) ;
#153589=CARTESIAN_POINT('Ctrl Pts',(-25.0632912716036,12.7050812653244,
128.743995286524)) ;
#153590=CARTESIAN_POINT('Ctrl Pts',(-25.0008040035337,12.9482677220772,
128.594669933562)) ;
#153591=CARTESIAN_POINT('Ctrl Pts',(-24.9612989083473,13.2238578222556,
128.512263188183)) ;
#153592=CARTESIAN_POINT('Ctrl Pts',(-24.9464400414306,13.5162932448957,
128.502169911524)) ;
#153593=CARTESIAN_POINT('Ctrl Pts',(-24.9567559801261,13.799165239793,128.565264390033)) ;
#153594=CARTESIAN_POINT('Ctrl Pts',(-24.9910303138475,14.0580267764743,
128.698731518742)) ;
#153595=CARTESIAN_POINT('Ctrl Pts',(-25.0453888541943,14.2686028129511,
128.890481281382)) ;
#153596=CARTESIAN_POINT('Ctrl Pts',(-25.1157749327763,14.4199618502008,
129.129219228183)) ;
#153597=CARTESIAN_POINT('Ctrl Pts',(-25.1962537469819,14.4998958219189,
129.397417258709)) ;
#153598=CARTESIAN_POINT('Ctrl Pts',(-25.2806998076144,14.5025664794371,
129.677347381576)) ;
#153599=CARTESIAN_POINT('Ctrl Pts',(-25.3614130293349,14.4280652825415,
129.946141834169)) ;
#153600=CARTESIAN_POINT('Ctrl Pts',(-25.4327613411336,14.2819177513075,
130.187667258866)) ;
#153601=CARTESIAN_POINT('Ctrl Pts',(-25.4888836010397,14.0723877227319,
130.384948804485)) ;
#153602=CARTESIAN_POINT('Ctrl Pts',(-25.524217369076,13.8191595273478,130.52109290564)) ;
#153603=CARTESIAN_POINT('Ctrl Pts',(-25.5363621720147,13.5356702848312,
130.589764696207)) ;
#153604=CARTESIAN_POINT('Ctrl Pts',(-25.5233799731752,13.2451626614465,
130.584896539849)) ;
#153605=CARTESIAN_POINT('Ctrl Pts',(-25.4853193673611,12.9658959397094,
130.506957297054)) ;
#153606=CARTESIAN_POINT('Ctrl Pts',(-25.4245567948317,12.720867949973,130.362513148524)) ;
#153607=CARTESIAN_POINT('Ctrl Pts',(-25.3444357384131,12.5256178596935,
130.161588938401)) ;
#153608=CARTESIAN_POINT('Ctrl Pts',(-25.2502354927177,12.3947249390078,
129.91946984754)) ;
#153609=CARTESIAN_POINT('Ctrl Pts',(-25.1471557384846,12.3373274128747,
129.651622343389)) ;
#153610=CARTESIAN_POINT('Ctrl Pts',(-25.04352722843,12.3577351376061,129.3818280718)) ;
#153611=CARTESIAN_POINT('Ctrl Pts',(-24.9440625937448,12.4546492514378,
129.124509048456)) ;
#153612=CARTESIAN_POINT('Ctrl Pts',(-24.8564471604785,12.6210676591383,
128.901700870073)) ;
#153613=CARTESIAN_POINT('Ctrl Pts',(-24.7859855036776,12.8446766854148,
128.728972290107)) ;
#153614=CARTESIAN_POINT('Ctrl Pts',(-24.7369148940067,13.108808163257,128.618635013836)) ;
#153615=CARTESIAN_POINT('Ctrl Pts',(-24.7117898455147,13.3979062620311,
128.578541432007)) ;
#153616=CARTESIAN_POINT('Ctrl Pts',(-24.7120774707783,13.6859097607706,
128.612344349061)) ;
#153617=CARTESIAN_POINT('Ctrl Pts',(-24.7366917620368,13.9567565280856,
128.717390290963)) ;
#153618=CARTESIAN_POINT('Ctrl Pts',(-24.7836759760245,14.1899349125241,
128.887914867791)) ;
#153619=CARTESIAN_POINT('Ctrl Pts',(-24.8478937377255,14.3662692626876,
129.10842421568)) ;
#153620=CARTESIAN_POINT('Ctrl Pts',(-24.9254379812952,14.4768289979695,
129.368240618362)) ;
#153621=CARTESIAN_POINT('Ctrl Pts',(-25.0089189154175,14.5109207090365,
129.645218161262)) ;
#153622=CARTESIAN_POINT('Ctrl Pts',(-25.0919501200887,14.4673589954117,
129.920875758852)) ;
#153623=CARTESIAN_POINT('Ctrl Pts',(-25.1679324131496,14.3490298117359,
130.175949093355)) ;
#153624=CARTESIAN_POINT('Ctrl Pts',(-25.2306776791176,14.1643442573792,
130.392364551844)) ;
#153625=CARTESIAN_POINT('Ctrl Pts',(-25.2749172208417,13.9269540764464,
130.554674425406)) ;
#153626=CARTESIAN_POINT('Ctrl Pts',(-25.296881801977,13.6529087066834,130.651991768824)) ;
#153627=CARTESIAN_POINT('Ctrl Pts',(-25.294121582554,13.3625040426011,130.677064089887)) ;
#153628=CARTESIAN_POINT('Ctrl Pts',(-25.2661584777254,13.0764917625792,
130.628507586136)) ;
#153629=CARTESIAN_POINT('Ctrl Pts',(-25.2142358128611,12.8152457852602,
130.509968872735)) ;
#153630=CARTESIAN_POINT('Ctrl Pts',(-25.1414105163864,12.5977360848388,
130.330346617025)) ;
#153631=CARTESIAN_POINT('Ctrl Pts',(-25.0521369052221,12.4392301767845,
130.102679861577)) ;
#153632=CARTESIAN_POINT('Ctrl Pts',(-24.9519825847367,12.3513755992719,
129.843259987167)) ;
#153633=CARTESIAN_POINT('Ctrl Pts',(-24.8480528333298,12.3399316332142,
129.572627714051)) ;
#153634=CARTESIAN_POINT('Ctrl Pts',(-24.7452323261505,12.4070554351268,
129.305672373312)) ;
#153635=CARTESIAN_POINT('Ctrl Pts',(-24.653114699296,12.5451369869361,129.069390792946)) ;
#153636=CARTESIAN_POINT('Ctrl Pts',(-24.574658401759,12.7477726868892,128.873467031278)) ;
#153637=CARTESIAN_POINT('Ctrl Pts',(-24.516485448288,12.9979367372735,128.736605448719)) ;
#153638=CARTESIAN_POINT('Ctrl Pts',(-24.4813744014041,13.2792370978739,
128.667217092649)) ;
#153639=CARTESIAN_POINT('Ctrl Pts',(-24.4713970354524,13.5701580555343,
128.671163049425)) ;
#153640=CARTESIAN_POINT('Ctrl Pts',(-24.4863380916386,13.8505377724051,
128.747899411962)) ;
#153641=CARTESIAN_POINT('Ctrl Pts',(-24.5245439679385,14.1007512372239,
128.892655666103)) ;
#153642=CARTESIAN_POINT('Ctrl Pts',(-24.5824402788279,14.3021715583994,
129.094893574169)) ;
#153643=CARTESIAN_POINT('Ctrl Pts',(-24.6554257346924,14.4410638226486,
129.341309329826)) ;
#153644=CARTESIAN_POINT('Ctrl Pts',(-24.7373356695316,14.506420576945,129.613776649341)) ;
#153645=CARTESIAN_POINT('Ctrl Pts',(-24.8210078848283,14.4944296739133,
129.89116801343)) ;
#153646=CARTESIAN_POINT('Ctrl Pts',(-24.9008406879447,14.4055611915821,
130.157574926146)) ;
#153647=CARTESIAN_POINT('Ctrl Pts',(-24.9694636925505,14.2469875620131,
130.391056099313)) ;
#153648=CARTESIAN_POINT('Ctrl Pts',(-25.0219599711088,14.0284942715184,
130.577615505577)) ;
#153649=CARTESIAN_POINT('Ctrl Pts',(-25.053320022464,13.7670074742828,130.70234813533)) ;
#153650=CARTESIAN_POINT('Ctrl Pts',(-25.0607089051815,13.4805781215048,
130.757097162265)) ;
#153651=CARTESIAN_POINT('Ctrl Pts',(-25.0430061476845,13.1913388058783,
130.73838961606)) ;
#153652=CARTESIAN_POINT('Ctrl Pts',(-25.0005234997867,12.9172330933754,
130.647473812606)) ;
#153653=CARTESIAN_POINT('Ctrl Pts',(-24.9358367964898,12.6799728703758,
130.491596969194)) ;
#153654=CARTESIAN_POINT('Ctrl Pts',(-24.8520526958292,12.4949910418975,
130.280173035867)) ;
#153655=CARTESIAN_POINT('Ctrl Pts',(-24.756283433586,12.3781840447206,130.033296564361)) ;
#153656=CARTESIAN_POINT('Ctrl Pts',(-24.6522083130104,12.3352411023339,
129.762603753164)) ;
#153657=CARTESIAN_POINT('Ctrl Pts',(-24.5492013359519,12.3701183957634,
129.494563600041)) ;
#153658=CARTESIAN_POINT('Ctrl Pts',(-24.4510228781676,12.4815908370187,
129.241159666924)) ;
#153659=CARTESIAN_POINT('Ctrl Pts',(-24.3668186999168,12.6586744463426,
129.02808228214)) ;
#153660=CARTESIAN_POINT('Ctrl Pts',(-24.2996856218142,12.8927064505131,
128.86527445598)) ;
#153661=CARTESIAN_POINT('Ctrl Pts',(-24.2552426505653,13.1615895986342,
128.768318934161)) ;
#153662=CARTESIAN_POINT('Ctrl Pts',(-24.2347791741716,13.4527337961883,
128.741859841865)) ;
#153663=CARTESIAN_POINT('Ctrl Pts',(-24.2398184692911,13.7397606263225,
128.789657130047)) ;
#153664=CARTESIAN_POINT('Ctrl Pts',(-24.2689320023009,14.0044956878458,
128.907831044878)) ;
#153665=CARTESIAN_POINT('Ctrl Pts',(-24.3192589693072,14.2270717047825,
129.087893938316)) ;
#153666=CARTESIAN_POINT('Ctrl Pts',(-24.386637598686,14.3928428531141,129.31784383242)) ;
#153667=CARTESIAN_POINT('Ctrl Pts',(-24.4659391407555,14.4891679896536,
129.582798342604)) ;
#153668=CARTESIAN_POINT('Ctrl Pts',(-24.5493645856168,14.5086708936273,
129.859423076708)) ;
#153669=CARTESIAN_POINT('Ctrl Pts',(-24.6318807172738,14.4507091204102,
130.133696348165)) ;
#153670=CARTESIAN_POINT('Ctrl Pts',(-24.7058567597393,14.318823465338,130.382937634357)) ;
#153671=CARTESIAN_POINT('Ctrl Pts',(-24.7654056750014,14.1234067424229,
130.589957999186)) ;
#153672=CARTESIAN_POINT('Ctrl Pts',(-24.8057595992627,13.8772496577341,
130.740994985991)) ;
#153673=CARTESIAN_POINT('Ctrl Pts',(-24.8231799857801,13.5994498547175,
130.82492878504)) ;
#153674=CARTESIAN_POINT('Ctrl Pts',(-24.8155893045152,13.3067289539218,
130.836068714423)) ;
#153675=CARTESIAN_POINT('Ctrl Pts',(-24.7830973206933,13.025513208076,130.774091996489)) ;
#153676=CARTESIAN_POINT('Ctrl Pts',(-24.7270577046474,12.7708776887036,
130.643534343482)) ;
#153677=CARTESIAN_POINT('Ctrl Pts',(-24.6505077984341,12.5628412979246,
130.453131427416)) ;
#153678=CARTESIAN_POINT('Ctrl Pts',(-24.5589760348122,12.4171764122364,
130.218786009453)) ;
#153679=CARTESIAN_POINT('Ctrl Pts',(-24.4570551071365,12.3431378359771,
129.954350410602)) ;
#153680=CARTESIAN_POINT('Ctrl Pts',(-24.3533214115063,12.3467434972734,
129.684210676246)) ;
#153681=CARTESIAN_POINT('Ctrl Pts',(-24.2523283182393,12.4272274658185,
129.422376802438)) ;
#153682=CARTESIAN_POINT('Ctrl Pts',(-24.1617932807192,12.5790158149027,
129.190994958755)) ;
#153683=CARTESIAN_POINT('Ctrl Pts',(-24.0869579392724,12.7916687829571,
129.005564094205)) ;
#153684=CARTESIAN_POINT('Ctrl Pts',(-24.0328055760906,13.0498138992039,
128.8805514449)) ;
#153685=CARTESIAN_POINT('Ctrl Pts',(-24.002521804032,13.3331756720239,128.825089124936)) ;
#153686=CARTESIAN_POINT('Ctrl Pts',(-23.9971725769105,13.6238935345468,
128.842575947387)) ;
#153687=CARTESIAN_POINT('Ctrl Pts',(-24.0167753636582,13.9010885274901,
128.933062863381)) ;
#153688=CARTESIAN_POINT('Ctrl Pts',(-24.0590128945408,14.1432054793993,
129.089568959686)) ;
#153689=CARTESIAN_POINT('Ctrl Pts',(-24.1203695555296,14.3341070280144,
129.302019247719)) ;
#153690=CARTESIAN_POINT('Ctrl Pts',(-24.1950418049019,14.4587991787124,
129.553138711427)) ;
#153691=CARTESIAN_POINT('Ctrl Pts',(-24.2777268658875,14.5101605081857,
129.827811432152)) ;
#153692=CARTESIAN_POINT('Ctrl Pts',(-24.3615395865942,14.4834097576633,
130.105796352381)) ;
#153693=CARTESIAN_POINT('Ctrl Pts',(-24.4396001237497,14.380986704451,130.366925214371)) ;
#153694=CARTESIAN_POINT('Ctrl Pts',(-24.5059188478657,14.2089571607828,
130.593906733665)) ;
#153695=CARTESIAN_POINT('Ctrl Pts',(-24.5543423873352,13.9828180453883,
130.768283768123)) ;
#153696=CARTESIAN_POINT('Ctrl Pts',(-24.5815804292821,13.7132629209954,
130.881224790375)) ;
#153697=CARTESIAN_POINT('Ctrl Pts',(-24.5841620980753,13.42583764063,130.921759059005)) ;
#153698=CARTESIAN_POINT('Ctrl Pts',(-24.5616991302751,13.1374631065902,
130.889232264708)) ;
#153699=CARTESIAN_POINT('Ctrl Pts',(-24.5148271925072,12.8691197006536,
130.785439835784)) ;
#153700=CARTESIAN_POINT('Ctrl Pts',(-24.4460595852779,12.6403113443668,
130.617737495797)) ;
#153701=CARTESIAN_POINT('Ctrl Pts',(-24.3602783070861,12.468420702256,130.400139902644)) ;
#153702=CARTESIAN_POINT('Ctrl Pts',(-24.2614984282295,12.3638000217504,
130.144889114756)) ;
#153703=CARTESIAN_POINT('Ctrl Pts',(-24.1577920148866,12.3359859144704,
129.874955907544)) ;
#153704=CARTESIAN_POINT('Ctrl Pts',(-24.054756872384,12.3855342690204,129.607074345636)) ;
#153705=CARTESIAN_POINT('Ctrl Pts',(-23.9592387590454,12.5097023136888,
129.361184743235)) ;
#153706=CARTESIAN_POINT('Ctrl Pts',(-23.8775758716564,12.6987169895182,
129.155691106511)) ;
#153707=CARTESIAN_POINT('Ctrl Pts',(-23.8143557456443,12.9413958856346,
129.004310292951)) ;
#153708=CARTESIAN_POINT('Ctrl Pts',(-23.7742609530853,13.2164083911014,
128.920187229679)) ;
#153709=CARTESIAN_POINT('Ctrl Pts',(-23.7587189631835,13.5077476116907,
128.907983756604)) ;
#153710=CARTESIAN_POINT('Ctrl Pts',(-23.7683966260473,13.7917084995172,
128.969294505237)) ;
#153711=CARTESIAN_POINT('Ctrl Pts',(-23.8017090745378,14.0497089633418,
129.099691778832)) ;
#153712=CARTESIAN_POINT('Ctrl Pts',(-23.855687851068,14.2632250030891,129.290500820459)) ;
#153713=CARTESIAN_POINT('Ctrl Pts',(-23.9259445764529,14.4168537708596,
129.528960264585)) ;
#153714=CARTESIAN_POINT('Ctrl Pts',(-24.0063154571533,14.4987598986465,
129.796873298139)) ;
#153715=CARTESIAN_POINT('Ctrl Pts',(-24.0905209887515,14.5035045718472,
130.07601230486)) ;
#153716=CARTESIAN_POINT('Ctrl Pts',(-24.1714640122117,14.4313229997249,
130.345485263966)) ;
#153717=CARTESIAN_POINT('Ctrl Pts',(-24.243380136318,14.286096674379,130.588809864043)) ;
#153718=CARTESIAN_POINT('Ctrl Pts',(-24.2994203289572,14.0806888556304,
130.785462444038)) ;
#153719=CARTESIAN_POINT('Ctrl Pts',(-24.3358061636431,13.8265805447723,
130.924971011733)) ;
#153720=CARTESIAN_POINT('Ctrl Pts',(-24.3485662665821,13.5441879409374,
130.995358908411)) ;
#153721=CARTESIAN_POINT('Ctrl Pts',(-24.3362787692544,13.2530370689606,
130.992594119063)) ;
#153722=CARTESIAN_POINT('Ctrl Pts',(-24.2990565233592,12.9741114175935,
130.916980614884)) ;
#153723=CARTESIAN_POINT('Ctrl Pts',(-24.2387980421576,12.7272119216586,
130.774093243821)) ;
#153724=CARTESIAN_POINT('Ctrl Pts',(-24.1592542721153,12.5305677659782,
130.57481255156)) ;
#153725=CARTESIAN_POINT('Ctrl Pts',(-24.0653992661587,12.3976028767503,
130.333704016612)) ;
#153726=CARTESIAN_POINT('Ctrl Pts',(-23.9625403093089,12.3378877564715,
130.06647786499)) ;
#153727=CARTESIAN_POINT('Ctrl Pts',(-23.8586656317476,12.3561146457162,
129.796030313594)) ;
#153728=CARTESIAN_POINT('Ctrl Pts',(-23.7592617382335,12.4504996091204,
129.538781451731)) ;
#153729=CARTESIAN_POINT('Ctrl Pts',(-23.6710781493093,12.6151918179393,
129.314368558311)) ;
#153730=CARTESIAN_POINT('Ctrl Pts',(-23.6000847768971,12.8367627956422,
129.140023816127)) ;
#153731=CARTESIAN_POINT('Ctrl Pts',(-23.5500037307086,13.102471284239,129.027040548326)) ;
#153732=CARTESIAN_POINT('Ctrl Pts',(-23.5244629176484,13.388098474674,128.985365037134)) ;
#153733=CARTESIAN_POINT('Ctrl Pts',(-23.5239179211507,13.6786302634614,
129.017000214703)) ;
#153734=CARTESIAN_POINT('Ctrl Pts',(-23.5479482075075,13.9495118019851,
129.120261172471)) ;
#153735=CARTESIAN_POINT('Ctrl Pts',(-23.5940539896427,14.1831630717315,
129.28807205042)) ;
#153736=CARTESIAN_POINT('Ctrl Pts',(-23.658087369295,14.3622887251467,129.508197418047)) ;
#153737=CARTESIAN_POINT('Ctrl Pts',(-23.7354964858561,14.4748192529362,
129.767663246934)) ;
#153738=CARTESIAN_POINT('Ctrl Pts',(-23.8186008712506,14.5109473630978,
130.043427649505)) ;
#153739=CARTESIAN_POINT('Ctrl Pts',(-23.9016485189198,14.46989386631,130.319093678178)) ;
#153740=CARTESIAN_POINT('Ctrl Pts',(-23.9780326629865,14.3536144736526,
130.57538079303)) ;
#153741=CARTESIAN_POINT('Ctrl Pts',(-24.041317392537,14.17062113719,130.793395793898)) ;
#153742=CARTESIAN_POINT('Ctrl Pts',(-24.0862233608817,13.933736573907,130.957750623604)) ;
#153743=CARTESIAN_POINT('Ctrl Pts',(-24.1087782693582,13.6617104442443,
131.056639640472)) ;
#153744=CARTESIAN_POINT('Ctrl Pts',(-24.1067652069901,13.3701432171844,
131.084050982405)) ;
#153745=CARTESIAN_POINT('Ctrl Pts',(-24.0794150200347,13.0839501475181,
131.037263800254)) ;
#153746=CARTESIAN_POINT('Ctrl Pts',(-24.0283415442683,12.8226369063403,
130.921088721576)) ;
#153747=CARTESIAN_POINT('Ctrl Pts',(-23.9561135287856,12.6036153158418,
130.74320474868)) ;
#153748=CARTESIAN_POINT('Ctrl Pts',(-23.8674374985634,12.4432239429731,
130.517228131168)) ;
#153749=CARTESIAN_POINT('Ctrl Pts',(-23.7669177824065,12.3525997513282,
130.256937329486)) ;
#153750=CARTESIAN_POINT('Ctrl Pts',(-23.6631589097691,12.3393903655815,
129.986759745082)) ;
#153751=CARTESIAN_POINT('Ctrl Pts',(-23.5608451726887,12.403468098602,129.721057322036)) ;
#153752=CARTESIAN_POINT('Ctrl Pts',(-23.4675538333872,12.5405072085783,
129.481626938511)) ;
#153753=CARTESIAN_POINT('Ctrl Pts',(-23.388662980097,12.7420005519616,129.284449551793)) ;
#153754=CARTESIAN_POINT('Ctrl Pts',(-23.3301053404809,12.9900801149227,
129.146339662681)) ;
#153755=CARTESIAN_POINT('Ctrl Pts',(-23.2942598700259,13.2708158721555,
129.07481369419)) ;
#153756=CARTESIAN_POINT('Ctrl Pts',(-23.2835507653219,13.5613604134334,
129.07658052044)) ;
#153757=CARTESIAN_POINT('Ctrl Pts',(-23.2977457009926,13.8428560081929,
129.151189048699)) ;
#153758=CARTESIAN_POINT('Ctrl Pts',(-23.3355877732922,14.0951246502648,
129.295029201952)) ;
#153759=CARTESIAN_POINT('Ctrl Pts',(-23.392640021767,14.2968154125605,129.494589775277)) ;
#153760=CARTESIAN_POINT('Ctrl Pts',(-23.4654695271126,14.4382062812648,
129.740653917803)) ;
#153761=CARTESIAN_POINT('Ctrl Pts',(-23.5470349400498,14.5055713938207,
130.012034404642)) ;
#153762=CARTESIAN_POINT('Ctrl Pts',(-23.6308595315768,14.4957941932041,
130.289927886282)) ;
#153763=CARTESIAN_POINT('Ctrl Pts',(-23.7106798599952,14.4095662340998,
130.556186374908)) ;
#153764=CARTESIAN_POINT('Ctrl Pts',(-23.7802571461447,14.2515335127425,
130.792730605287)) ;
#153765=CARTESIAN_POINT('Ctrl Pts',(-23.8330271584667,14.0347236874785,
130.979999898394)) ;
#153766=CARTESIAN_POINT('Ctrl Pts',(-23.8649144470802,13.7751700114088,
131.106159195577)) ;
#153767=CARTESIAN_POINT('Ctrl Pts',(-23.8730939748177,13.489555102194,131.163174955555)) ;
#153768=CARTESIAN_POINT('Ctrl Pts',(-23.8560200827014,13.1989624545804,
131.146444379055)) ;
#153769=CARTESIAN_POINT('Ctrl Pts',(-23.8142948031392,12.9245155762064,
131.057679563774)) ;
#153770=CARTESIAN_POINT('Ctrl Pts',(-23.7497390288408,12.6850932088169,
130.90236186876)) ;
#153771=CARTESIAN_POINT('Ctrl Pts',(-23.6676401734867,12.5007200500438,
130.695387264516)) ;
#153772=CARTESIAN_POINT('Ctrl Pts',(-23.5710799792398,12.3802348015134,
130.446601105623)) ;
#153773=CARTESIAN_POINT('Ctrl Pts',(-23.4680387193144,12.3354177830535,
130.178616720221)) ;
#153774=CARTESIAN_POINT('Ctrl Pts',(-23.3639870057212,12.3682931650198,
129.907845197495)) ;
#153775=CARTESIAN_POINT('Ctrl Pts',(-23.2665557781875,12.4764500222757,
129.656260795804)) ;
#153776=CARTESIAN_POINT('Ctrl Pts',(-23.1812074615382,12.6527561756398,
129.440099421206)) ;
#153777=CARTESIAN_POINT('Ctrl Pts',(-23.1137789148354,12.8841372675975,
129.276247072773)) ;
#153778=CARTESIAN_POINT('Ctrl Pts',(-23.0682028417558,13.1550291136418,
129.176337392218)) ;
#153779=CARTESIAN_POINT('Ctrl Pts',(-23.0472767378411,13.4437302360126,
129.148261982065)) ;
#153780=CARTESIAN_POINT('Ctrl Pts',(-23.0515496084932,13.7319393007276,
129.193922359653)) ;
#153781=CARTESIAN_POINT('Ctrl Pts',(-23.079878251099,13.9965481623833,129.309665379139)) ;
#153782=CARTESIAN_POINT('Ctrl Pts',(-23.129741526764,14.2215298170475,129.488488454029)) ;
#153783=CARTESIAN_POINT('Ctrl Pts',(-23.1968818888558,14.3891483272759,
129.717799600751)) ;
#153784=CARTESIAN_POINT('Ctrl Pts',(-23.2754021964238,14.4871687024338,
129.980255089599)) ;
#153785=CARTESIAN_POINT('Ctrl Pts',(-23.3593328759968,14.5093408079897,
130.258577404978)) ;
#153786=CARTESIAN_POINT('Ctrl Pts',(-23.4420335332337,14.4530254583256,
130.533420307647)) ;
#153787=CARTESIAN_POINT('Ctrl Pts',(-23.5159486858221,14.3240305585518,
130.782295669503)) ;
#153788=CARTESIAN_POINT('Ctrl Pts',(-23.5763068870408,14.1290979717854,
130.991878121919)) ;
#153789=CARTESIAN_POINT('Ctrl Pts',(-23.617068843589,13.8855604155571,131.143910620301)) ;
#153790=CARTESIAN_POINT('Ctrl Pts',(-23.6352727286933,13.6058416707122,
131.230442968303)) ;
#153791=CARTESIAN_POINT('Ctrl Pts',(-23.6283964341607,13.3160021377259,
131.243341112372)) ;
#153792=CARTESIAN_POINT('Ctrl Pts',(-23.5965464340223,13.0326886676077,
131.183420690455)) ;
#153793=CARTESIAN_POINT('Ctrl Pts',(-23.5408985622457,12.7766372190837,
131.054072194123)) ;
#153794=CARTESIAN_POINT('Ctrl Pts',(-23.4649595861684,12.5676698161814,
130.865387166735)) ;
#153795=CARTESIAN_POINT('Ctrl Pts',(-23.3740967453034,12.4206517790888,
130.632884178497)) ;
#153796=CARTESIAN_POINT('Ctrl Pts',(-23.2727082372118,12.3443150505119,
130.369901024895)) ;
#153797=CARTESIAN_POINT('Ctrl Pts',(-23.1684546893583,12.3454567433165,
130.098404386445)) ;
#153798=CARTESIAN_POINT('Ctrl Pts',(-23.0671327036379,12.4241540146565,
129.835658717647)) ;
#153799=CARTESIAN_POINT('Ctrl Pts',(-22.9764947583752,12.5736454649868,
129.60388157098)) ;
#153800=CARTESIAN_POINT('Ctrl Pts',(-22.9011806814661,12.7844244258342,
129.417017819213)) ;
#153801=CARTESIAN_POINT('Ctrl Pts',(-22.8463459628872,13.041264478038,129.289992771218)) ;
#153802=CARTESIAN_POINT('Ctrl Pts',(-22.815230919969,13.3250313838274,129.232207692813)) ;
#153803=CARTESIAN_POINT('Ctrl Pts',(-22.8092125202162,13.6156492492809,
129.247717690027)) ;
#153804=CARTESIAN_POINT('Ctrl Pts',(-22.8280212526032,13.8929002803611,
129.335801002832)) ;
#153805=CARTESIAN_POINT('Ctrl Pts',(-22.8696833153775,14.1366366428793,
129.490673844657)) ;
#153806=CARTESIAN_POINT('Ctrl Pts',(-22.9303059421642,14.3287833833703,
129.70086742119)) ;
#153807=CARTESIAN_POINT('Ctrl Pts',(-23.0049559964505,14.4563288342089,
129.952070625789)) ;
#153808=CARTESIAN_POINT('Ctrl Pts',(-23.0876811988293,14.5097636463918,
130.226920951019)) ;
#153809=CARTESIAN_POINT('Ctrl Pts',(-23.171313625943,14.4852491819093,130.504285160366)) ;
#153810=CARTESIAN_POINT('Ctrl Pts',(-23.2495616828516,14.385213180382,130.765927789329)) ;
#153811=CARTESIAN_POINT('Ctrl Pts',(-23.3164467304666,14.2148994362801,
130.994611083723)) ;
#153812=CARTESIAN_POINT('Ctrl Pts',(-23.3654737459425,13.9895605141043,
131.170821580244)) ;
#153813=CARTESIAN_POINT('Ctrl Pts',(-23.3932709418014,13.7226496289756,
131.285186238845)) ;
#153814=CARTESIAN_POINT('Ctrl Pts',(-23.3966715321499,13.4342098859693,
131.328274909581)) ;
#153815=CARTESIAN_POINT('Ctrl Pts',(-23.3749521692447,13.1458182759752,
131.297881508113)) ;
#153816=CARTESIAN_POINT('Ctrl Pts',(-23.3285769346008,12.8759127132536,
131.195640591877)) ;
#153817=CARTESIAN_POINT('Ctrl Pts',(-23.2608087751802,12.6468868556867,
131.030665242811)) ;
#153818=CARTESIAN_POINT('Ctrl Pts',(-23.1749384545703,12.4721832296684,
130.81301511834)) ;
#153819=CARTESIAN_POINT('Ctrl Pts',(-23.0772501521557,12.3661739274481,
130.560671910315)) ;
#153820=CARTESIAN_POINT('Ctrl Pts',(-22.972758046801,12.3355863385396,130.288726503058)) ;
#153821=CARTESIAN_POINT('Ctrl Pts',(-22.8698300820149,12.3831198658751,
130.021082533712)) ;
#153822=CARTESIAN_POINT('Ctrl Pts',(-22.7739061268904,12.5053833023315,
129.774046335208)) ;
#153823=CARTESIAN_POINT('Ctrl Pts',(-22.6919791045737,12.6923270702948,
129.567704270438)) ;
#153824=CARTESIAN_POINT('Ctrl Pts',(-22.6281112723494,12.9335865705139,
129.414426275698)) ;
#153825=CARTESIAN_POINT('Ctrl Pts',(-22.5872544610613,13.2085814539572,
129.328158922446)) ;
#153826=CARTESIAN_POINT('Ctrl Pts',(-22.5710404902249,13.4990557588074,
129.313907984072)) ;
#153827=CARTESIAN_POINT('Ctrl Pts',(-22.5799753665134,13.7836907462661,
129.373072556554)) ;
#153828=CARTESIAN_POINT('Ctrl Pts',(-22.612638583778,14.0427281414566,129.501571243045)) ;
#153829=CARTESIAN_POINT('Ctrl Pts',(-22.6660762367978,14.2577309750281,
129.69079806233)) ;
#153830=CARTESIAN_POINT('Ctrl Pts',(-22.7357975374954,14.4131664617501,
129.927633756715)) ;
#153831=CARTESIAN_POINT('Ctrl Pts',(-22.8161137666784,14.4973755702956,
130.195456113862)) ;
#153832=CARTESIAN_POINT('Ctrl Pts',(-22.8998820017925,14.5046724130054,
130.47314586159)) ;
#153833=CARTESIAN_POINT('Ctrl Pts',(-22.9816064513032,14.4343111747756,
130.745147804022)) ;
#153834=CARTESIAN_POINT('Ctrl Pts',(-23.0536227051492,14.2913904033354,
130.98864811284)) ;
#153835=CARTESIAN_POINT('Ctrl Pts',(-23.1102843211941,14.0872940403586,
131.187176359758)) ;
#153836=CARTESIAN_POINT('Ctrl Pts',(-23.1472375329922,13.8349907742835,
131.328253449348)) ;
#153837=CARTESIAN_POINT('Ctrl Pts',(-23.1607772342592,13.5522018199285,
131.401036362566)) ;
#153838=CARTESIAN_POINT('Ctrl Pts',(-23.1491871925298,13.2611771320633,
131.400285897439)) ;
#153839=CARTESIAN_POINT('Ctrl Pts',(-23.1125952006362,12.9814107201437,
131.326544774095)) ;
#153840=CARTESIAN_POINT('Ctrl Pts',(-23.0531566614903,12.7341369610279,
131.185942865115)) ;
#153841=CARTESIAN_POINT('Ctrl Pts',(-22.9739547949964,12.535166216503,130.98774443351)) ;
#153842=CARTESIAN_POINT('Ctrl Pts',(-22.8800044204222,12.4000170891871,
130.746489022896)) ;
#153843=CARTESIAN_POINT('Ctrl Pts',(-22.7777942394703,12.3385941106561,
130.480992016477)) ;
#153844=CARTESIAN_POINT('Ctrl Pts',(-22.6737045237347,12.3545286685026,
130.209973410253)) ;
#153845=CARTESIAN_POINT('Ctrl Pts',(-22.574018025731,12.4469846430608,129.951917332464)) ;
#153846=CARTESIAN_POINT('Ctrl Pts',(-22.4853397321754,12.6102579412087,
129.726108518223)) ;
#153847=CARTESIAN_POINT('Ctrl Pts',(-22.4141387274598,12.8296977311719,
129.551032278381)) ;
#153848=CARTESIAN_POINT('Ctrl Pts',(-22.3635165048781,13.0929763552362,
129.436306120848)) ;
#153849=CARTESIAN_POINT('Ctrl Pts',(-22.3370222640428,13.3798715107165,
129.392040554444)) ;
#153850=CARTESIAN_POINT('Ctrl Pts',(-22.3358180956749,13.6705227535771,
129.421738962196)) ;
#153851=CARTESIAN_POINT('Ctrl Pts',(-22.359121262081,13.9421700423004,129.522864634634)) ;
#153852=CARTESIAN_POINT('Ctrl Pts',(-22.4048936915904,14.1780191011813,
129.689842088352)) ;
#153853=CARTESIAN_POINT('Ctrl Pts',(-22.4683015911897,14.3579768124892,
129.908015928199)) ;
#153854=CARTESIAN_POINT('Ctrl Pts',(-22.5452274463354,14.4725057553617,
130.165996866725)) ;
#153855=CARTESIAN_POINT('Ctrl Pts',(-22.6283868280108,14.5110248787396,
130.441981808158)) ;
#153856=CARTESIAN_POINT('Ctrl Pts',(-22.7115926468901,14.4721191969269,
130.718131866034)) ;
#153857=CARTESIAN_POINT('Ctrl Pts',(-22.7882774144574,14.3577454336847,
130.975310558445)) ;
#153858=CARTESIAN_POINT('Ctrl Pts',(-22.8518198048839,14.1770688666527,
131.193977525084)) ;
#153859=CARTESIAN_POINT('Ctrl Pts',(-22.8974027115045,13.9416997327419,
131.360307596844)) ;
#153860=CARTESIAN_POINT('Ctrl Pts',(-22.9206820190988,13.6694104353782,
131.461436266431)) ;
#153861=CARTESIAN_POINT('Ctrl Pts',(-22.9194213574652,13.3798585935035,
131.490838835533)) ;
#153862=CARTESIAN_POINT('Ctrl Pts',(-22.8929170330155,13.0927640382574,
131.446571141722)) ;
#153863=CARTESIAN_POINT('Ctrl Pts',(-22.8423030043868,12.8294542733058,
131.331865445954)) ;
#153864=CARTESIAN_POINT('Ctrl Pts',(-22.7706185679307,12.6090080043084,
131.155563913664)) ;
#153865=CARTESIAN_POINT('Ctrl Pts',(-22.6821571255679,12.4466659582347,
130.930272433196)) ;
#153866=CARTESIAN_POINT('Ctrl Pts',(-22.5824728331909,12.3544265354386,
130.672221564255)) ;
#153867=CARTESIAN_POINT('Ctrl Pts',(-22.478522759517,12.338485550426,130.401560070963)) ;
#153868=CARTESIAN_POINT('Ctrl Pts',(-22.3754966015088,12.4009576070215,
130.133958949611)) ;
#153869=CARTESIAN_POINT('Ctrl Pts',(-22.2823680889779,12.5356622675021,
129.894847033385)) ;
#153870=CARTESIAN_POINT('Ctrl Pts',(-22.2032360996956,12.7342792931547,
129.696815676907)) ;
#153871=CARTESIAN_POINT('Ctrl Pts',(-22.1436939987442,12.9822470405306,
129.555989965758)) ;
#153872=CARTESIAN_POINT('Ctrl Pts',(-22.1071406671597,13.2626104241267,
129.482419788097)) ;
#153873=CARTESIAN_POINT('Ctrl Pts',(-22.0957144593787,13.5537330357078,
129.482159506806)) ;
#153874=CARTESIAN_POINT('Ctrl Pts',(-22.1092685563454,13.8350780443648,
129.554823798795)) ;
#153875=CARTESIAN_POINT('Ctrl Pts',(-22.1461475103679,14.0872562376869,
129.695659561939)) ;
#153876=CARTESIAN_POINT('Ctrl Pts',(-22.2030821358645,14.2922552735091,
129.895131181954)) ;
#153877=CARTESIAN_POINT('Ctrl Pts',(-22.2754289643042,14.4349645919609,
130.139699349458)) ;
#153878=CARTESIAN_POINT('Ctrl Pts',(-22.3564708008619,14.5045540577175,
130.40942261917)) ;
#153879=CARTESIAN_POINT('Ctrl Pts',(-22.4406441329642,14.4973581396257,
130.688457173911)) ;
#153880=CARTESIAN_POINT('Ctrl Pts',(-22.5209414268602,14.4126016842873,
130.956235143864)) ;
#153881=CARTESIAN_POINT('Ctrl Pts',(-22.5903401138937,14.2578370889756,
131.191978979017)) ;
#153882=CARTESIAN_POINT('Ctrl Pts',(-22.643899231601,14.0423606370671,131.381638018117)) ;
#153883=CARTESIAN_POINT('Ctrl Pts',(-22.676541227732,13.7833430848993,131.510062783894)) ;
#153884=CARTESIAN_POINT('Ctrl Pts',(-22.6854014712124,13.4972454461382,
131.569174829683)) ;
#153885=CARTESIAN_POINT('Ctrl Pts',(-22.6699589229826,13.2225256872019,
131.55537794912)) ;
#153886=CARTESIAN_POINT('Ctrl Pts',(-22.6458119565126,13.0520853568101,
131.505271480944)) ;
#153887=CARTESIAN_POINT('Ctrl Pts',(-22.6320187065114,12.9778651918053,
131.474336592418)) ;
#153888=CARTESIAN_POINT('',(-33.2541723945531,13.1734341962953,127.827509047315)) ;
#153889=CARTESIAN_POINT('Origin',(-33.2777287689504,13.1551399285885,127.896323413507)) ;
#153890=CARTESIAN_POINT('',(-33.3012851433477,13.1368456608817,127.965137779698)) ;
#153891=CARTESIAN_POINT('Origin',(-33.2777287689504,13.1551399285885,127.896323413507)) ;
#153892=CARTESIAN_POINT('Origin',(-33.2777287689504,13.1551399285885,127.896323413507)) ;
#153893=CARTESIAN_POINT('Ctrl Pts',(-22.3151378258161,14.5729486667267,
130.548644386657)) ;
#153894=CARTESIAN_POINT('Ctrl Pts',(-22.329099593949,14.5730368300439,130.589430393716)) ;
#153895=CARTESIAN_POINT('Ctrl Pts',(-22.3430755637926,14.5706665958407,
130.630257665154)) ;
#153896=CARTESIAN_POINT('Ctrl Pts',(-22.3569679467077,14.5658273790944,
130.670840970083)) ;
#153897=CARTESIAN_POINT('Ctrl Pts',(-22.3627375743675,14.5638176102188,
130.687695570196)) ;
#153898=CARTESIAN_POINT('Ctrl Pts',(-22.3684933027053,14.5613818550179,
130.704509566733)) ;
#153899=CARTESIAN_POINT('Ctrl Pts',(-22.3742281245136,14.5585193175848,
130.721262489797)) ;
#153900=CARTESIAN_POINT('Ctrl Pts',(-22.4010526679328,14.5451298414636,
130.799624037403)) ;
#153901=CARTESIAN_POINT('Ctrl Pts',(-22.4274099090546,14.5224036480322,
130.876620256302)) ;
#153902=CARTESIAN_POINT('Ctrl Pts',(-22.4525800025406,14.4911112211554,
130.950148872058)) ;
#153903=CARTESIAN_POINT('Ctrl Pts',(-22.4583236353459,14.4839705162681,
130.96692756896)) ;
#153904=CARTESIAN_POINT('Ctrl Pts',(-22.4640054819444,14.4763839522856,
130.983525767063)) ;
#153905=CARTESIAN_POINT('Ctrl Pts',(-22.4696170489507,14.4683610330769,
130.999918630428)) ;
#153906=CARTESIAN_POINT('Ctrl Pts',(-22.4947273752802,14.4324605227176,
131.073272498985)) ;
#153907=CARTESIAN_POINT('Ctrl Pts',(-22.5184294421355,14.3878194900791,
131.14251292154)) ;
#153908=CARTESIAN_POINT('Ctrl Pts',(-22.54019892772,14.3354941538346,131.206106994967)) ;
#153909=CARTESIAN_POINT('Ctrl Pts',(-22.5446195882161,14.324868613512,131.219020842062)) ;
#153910=CARTESIAN_POINT('Ctrl Pts',(-22.5489605756069,14.3139263466219,
131.231701943349)) ;
#153911=CARTESIAN_POINT('Ctrl Pts',(-22.5532175237182,14.3026764237554,
131.244137608586)) ;
#153912=CARTESIAN_POINT('Ctrl Pts',(-22.5727750268273,14.2509914147576,
131.301270219829)) ;
#153913=CARTESIAN_POINT('Ctrl Pts',(-22.5905566144932,14.1928134151902,
131.353216627627)) ;
#153914=CARTESIAN_POINT('Ctrl Pts',(-22.6061216929628,14.1296950731466,
131.398685264081)) ;
#153915=CARTESIAN_POINT('Ctrl Pts',(-22.6106418870564,14.1113651201394,
131.411889634515)) ;
#153916=CARTESIAN_POINT('Ctrl Pts',(-22.6149751810526,14.0926186905486,
131.424547971201)) ;
#153917=CARTESIAN_POINT('Ctrl Pts',(-22.6191108667609,14.0734942173741,
131.43662939706)) ;
#153918=CARTESIAN_POINT('Ctrl Pts',(-22.6323692360561,14.0121841116725,
131.475360581426)) ;
#153919=CARTESIAN_POINT('Ctrl Pts',(-22.6435936004016,13.9469968841546,
131.508155446611)) ;
#153920=CARTESIAN_POINT('Ctrl Pts',(-22.652601471037,13.8791719111477,131.534467013303)) ;
#153921=CARTESIAN_POINT('Ctrl Pts',(-22.6560966798024,13.8528546548554,
131.544676353806)) ;
#153922=CARTESIAN_POINT('Ctrl Pts',(-22.659258086565,13.8261405468826,131.553909986958)) ;
#153923=CARTESIAN_POINT('Ctrl Pts',(-22.66207462569,13.799103138409,131.562137838641)) ;
#153924=CARTESIAN_POINT('Ctrl Pts',(-22.6646263132483,13.774608176419,131.569591989228)) ;
#153925=CARTESIAN_POINT('Ctrl Pts',(-22.666928934256,13.7495103406014,131.576318680967)) ;
#153926=CARTESIAN_POINT('Ctrl Pts',(-22.6689450781796,13.7240463055939,
131.582208381066)) ;
#153927=CARTESIAN_POINT('Ctrl Pts',(-22.6709623724016,13.6985677422402,
131.588101441496)) ;
#153928=CARTESIAN_POINT('Ctrl Pts',(-22.6726927838211,13.6727232379278,
131.593156345059)) ;
#153929=CARTESIAN_POINT('Ctrl Pts',(-22.6741146695638,13.646767549545,131.597309957245)) ;
#153930=CARTESIAN_POINT('Ctrl Pts',(-22.6755372042712,13.6208000146915,
131.601465465186)) ;
#153931=CARTESIAN_POINT('Ctrl Pts',(-22.6766508920783,13.5947219208586,
131.604718769158)) ;
#153932=CARTESIAN_POINT('Ctrl Pts',(-22.6774507939397,13.5687954659975,
131.607055523305)) ;
#153933=CARTESIAN_POINT('Ctrl Pts',(-22.6781594759397,13.5458256333621,
131.609125796775)) ;
#153934=CARTESIAN_POINT('Ctrl Pts',(-22.6786221002216,13.5229752443451,
131.610477364612)) ;
#153935=CARTESIAN_POINT('Ctrl Pts',(-22.6788463775648,13.5004244329661,
131.611132537728)) ;
#153936=CARTESIAN_POINT('Ctrl Pts',(-22.6790376668692,13.4811905283751,
131.611691344105)) ;
#153937=CARTESIAN_POINT('Ctrl Pts',(-22.679062679477,13.4613698797398,131.611765143739)) ;
#153938=CARTESIAN_POINT('Ctrl Pts',(-22.6788952846805,13.4412408608155,
131.611276429829)) ;
#153939=CARTESIAN_POINT('Ctrl Pts',(-22.6787281656732,13.4211450051914,
131.610788521094)) ;
#153940=CARTESIAN_POINT('Ctrl Pts',(-22.6783691766662,13.4007422200768,
131.609739715094)) ;
#153941=CARTESIAN_POINT('Ctrl Pts',(-22.6778091707993,13.3803126577526,
131.608103354377)) ;
#153942=CARTESIAN_POINT('Ctrl Pts',(-22.677257716648,13.3601950703848,131.606491982133)) ;
#153943=CARTESIAN_POINT('Ctrl Pts',(-22.6765113567921,13.3400519549882,
131.604310971553)) ;
#153944=CARTESIAN_POINT('Ctrl Pts',(-22.6755782124765,13.3201474123105,
131.601584558884)) ;
#153945=CARTESIAN_POINT('Ctrl Pts',(-22.6746233619552,13.2997798629072,
131.598794726149)) ;
#153946=CARTESIAN_POINT('Ctrl Pts',(-22.6734729150999,13.2796626021655,
131.5954338265)) ;
#153947=CARTESIAN_POINT('Ctrl Pts',(-22.6721535433962,13.2600678710267,
131.591579895431)) ;
#153948=CARTESIAN_POINT('Ctrl Pts',(-22.6708341716925,13.2404731398879,
131.587725964362)) ;
#153949=CARTESIAN_POINT('Ctrl Pts',(-22.6693459978666,13.2214012994026,
131.583379429525)) ;
#153950=CARTESIAN_POINT('Ctrl Pts',(-22.6677325901906,13.2031075416911,
131.578666241292)) ;
#153951=CARTESIAN_POINT('Ctrl Pts',(-22.6665744709625,13.1899761100796,
131.57528307038)) ;
#153952=CARTESIAN_POINT('Ctrl Pts',(-22.6652834410313,13.1764783865927,
131.571511826004)) ;
#153953=CARTESIAN_POINT('Ctrl Pts',(-22.6638758082619,13.1629676618293,
131.567399713087)) ;
#153954=CARTESIAN_POINT('Ctrl Pts',(-22.6624577740388,13.1493571019527,
131.563257214438)) ;
#153955=CARTESIAN_POINT('Ctrl Pts',(-22.6609213606832,13.1357338594017,
131.558768747133)) ;
#153956=CARTESIAN_POINT('Ctrl Pts',(-22.659299870578,13.1224444824643,131.554031896726)) ;
#153957=CARTESIAN_POINT('Ctrl Pts',(-22.6576783804728,13.109155105527,131.54929504632)) ;
#153958=CARTESIAN_POINT('Ctrl Pts',(-22.655971922004,13.096199960817,131.544310235839)) ;
#153959=CARTESIAN_POINT('Ctrl Pts',(-22.6542298620055,13.0839043074199,
131.539221220329)) ;
#153960=CARTESIAN_POINT('Ctrl Pts',(-22.6529520299329,13.0748852264018,
131.535488336708)) ;
#153961=CARTESIAN_POINT('Ctrl Pts',(-22.6515626734834,13.0655735645419,
131.531429739391)) ;
#153962=CARTESIAN_POINT('Ctrl Pts',(-22.6501095358714,13.0564196733478,
131.52718467415)) ;
#153963=CARTESIAN_POINT('Ctrl Pts',(-22.6486476168762,13.0472104647311,
131.522913955767)) ;
#153964=CARTESIAN_POINT('Ctrl Pts',(-22.6471211407257,13.0381613456492,
131.518454725706)) ;
#153965=CARTESIAN_POINT('Ctrl Pts',(-22.6455941107226,13.0297062023841,
131.513993911399)) ;
#153966=CARTESIAN_POINT('Ctrl Pts',(-22.6454270609541,13.0287812502074,
131.51350591968)) ;
#153967=CARTESIAN_POINT('Ctrl Pts',(-22.6452600191918,13.0278633792219,
131.513017949926)) ;
#153968=CARTESIAN_POINT('Ctrl Pts',(-22.645093079739,13.0269531373025,131.51253027587)) ;
#153969=CARTESIAN_POINT('Ctrl Pts',(-22.6439417998698,13.0206757524139,
131.509167084525)) ;
#153970=CARTESIAN_POINT('Ctrl Pts',(-22.6426928969163,13.0142106156177,
131.505518699242)) ;
#153971=CARTESIAN_POINT('Ctrl Pts',(-22.6414278770865,13.008138163139,131.501823231953)) ;
#153972=CARTESIAN_POINT('Ctrl Pts',(-22.6408214929086,13.0052273478162,
131.500051818699)) ;
#153973=CARTESIAN_POINT('Ctrl Pts',(-22.6402116170566,13.0024063418278,
131.498270239291)) ;
#153974=CARTESIAN_POINT('Ctrl Pts',(-22.6396083673344,12.9997366350286,
131.496507988166)) ;
#153975=CARTESIAN_POINT('Ctrl Pts',(-22.6385793197154,12.9951825418823,
131.493501869377)) ;
#153976=CARTESIAN_POINT('Ctrl Pts',(-22.6374677582898,12.9906247701674,
131.490254706053)) ;
#153977=CARTESIAN_POINT('Ctrl Pts',(-22.6364008830054,12.9868577736952,
131.487138082702)) ;
#153978=CARTESIAN_POINT('Ctrl Pts',(-22.635773853454,12.984643814723,131.485306364441)) ;
#153979=CARTESIAN_POINT('Ctrl Pts',(-22.6351266524276,12.9825760105869,
131.483415720087)) ;
#153980=CARTESIAN_POINT('Ctrl Pts',(-22.6345107978493,12.9809630503241,
131.481616646861)) ;
#153981=CARTESIAN_POINT('Ctrl Pts',(-22.6335563000255,12.9784631629888,
131.478828307635)) ;
#153982=CARTESIAN_POINT('Ctrl Pts',(-22.6326519325366,12.9769886520828,
131.47618641221)) ;
#153983=CARTESIAN_POINT('Ctrl Pts',(-22.6320187065114,12.9778651918053,
131.474336592418)) ;
#153984=CARTESIAN_POINT('Ctrl Pts',(-22.3151378869398,14.4232238463042,
130.548644361976)) ;
#153985=CARTESIAN_POINT('Ctrl Pts',(-22.2811439325193,14.4234782772113,
130.449339078899)) ;
#153986=CARTESIAN_POINT('Ctrl Pts',(-22.2474191728421,14.4076338778521,
130.350820184447)) ;
#153987=CARTESIAN_POINT('Ctrl Pts',(-22.1822291641438,14.3443721936545,
130.160383020607)) ;
#153988=CARTESIAN_POINT('Ctrl Pts',(-22.1511321866922,14.2967160993894,
130.069540569355)) ;
#153989=CARTESIAN_POINT('Ctrl Pts',(-22.0867514375386,14.1569964530343,
129.881467465523)) ;
#153990=CARTESIAN_POINT('Ctrl Pts',(-22.0558391935788,14.0563340831254,
129.79116466935)) ;
#153991=CARTESIAN_POINT('Ctrl Pts',(-22.0081129613856,13.8232128942773,
129.651743790581)) ;
#153992=CARTESIAN_POINT('Ctrl Pts',(-21.9920420955645,13.6947112909488,
129.604796564568)) ;
#153993=CARTESIAN_POINT('Ctrl Pts',(-21.9745761371278,13.4112788385579,
129.553773905501)) ;
#153994=CARTESIAN_POINT('Ctrl Pts',(-21.9770346938545,13.2936995343157,
129.560955995889)) ;
#153995=CARTESIAN_POINT('Ctrl Pts',(-21.9761622047819,13.2297469423984,
129.558407225797)) ;
#153996=CARTESIAN_POINT('Ctrl Pts',(-21.9759501313551,13.2215607234671,
129.55778770353)) ;
#153997=CARTESIAN_POINT('Ctrl Pts',(-21.9753726991377,13.2141115604543,
129.556100872128)) ;
#153998=CARTESIAN_POINT('Ctrl Pts',(-21.9751899121014,13.2123135011625,
129.555566903112)) ;
#153999=CARTESIAN_POINT('Ctrl Pts',(-21.9748392577633,13.2102931177125,
129.55454254955)) ;
#154000=CARTESIAN_POINT('Ctrl Pts',(-21.9747072455502,13.2096748296432,
129.554156907149)) ;
#154001=CARTESIAN_POINT('Ctrl Pts',(-21.9744488989635,13.2088894196123,
129.553402208811)) ;
#154002=CARTESIAN_POINT('Ctrl Pts',(-21.9743389556033,13.2086342290074,
129.553081035335)) ;
#154003=CARTESIAN_POINT('Ctrl Pts',(-21.9741045372372,13.2082979781231,
129.552396237623)) ;
#154004=CARTESIAN_POINT('Ctrl Pts',(-21.9739885035561,13.2082090859891,
129.552057272717)) ;
#154005=CARTESIAN_POINT('Ctrl Pts',(-21.973721487045,13.2081743377998,129.551277247249)) ;
#154006=CARTESIAN_POINT('Ctrl Pts',(-21.9735786216205,13.2082608228111,
129.550859899763)) ;
#154007=CARTESIAN_POINT('Ctrl Pts',(-21.9732155601285,13.2086648958773,
129.54979930164)) ;
#154008=CARTESIAN_POINT('Ctrl Pts',(-21.9730009907799,13.2091027938618,
129.549172488204)) ;
#154009=CARTESIAN_POINT('Ctrl Pts',(-21.972108851907,13.2113394407767,129.546566315876)) ;
#154010=CARTESIAN_POINT('Ctrl Pts',(-21.9714067112402,13.2145328967391,
129.544515178214)) ;
#154011=CARTESIAN_POINT('Ctrl Pts',(-21.9683523963269,13.2306316253467,
129.535592720905)) ;
#154012=CARTESIAN_POINT('Ctrl Pts',(-21.9651612110957,13.2574016528,129.526270429292)) ;
#154013=CARTESIAN_POINT('Ctrl Pts',(-21.9565989464617,13.3672753503857,
129.501257801966)) ;
#154014=CARTESIAN_POINT('Ctrl Pts',(-21.9516425801557,13.489837765544,129.486778952301)) ;
#154015=CARTESIAN_POINT('Ctrl Pts',(-21.9656761119371,13.7782522629322,
129.527774590198)) ;
#154016=CARTESIAN_POINT('Ctrl Pts',(-21.9813770244683,13.911436662301,129.57364108585)) ;
#154017=CARTESIAN_POINT('Ctrl Pts',(-22.0290989771478,14.1573235247066,
129.713049463034)) ;
#154018=CARTESIAN_POINT('Ctrl Pts',(-22.0613649266162,14.2666151380173,
129.807306789113)) ;
#154019=CARTESIAN_POINT('Ctrl Pts',(-22.1305065476335,14.4241005029476,
130.009287652021)) ;
#154020=CARTESIAN_POINT('Ctrl Pts',(-22.1651065040721,14.4793817119498,
130.110363226373)) ;
#154021=CARTESIAN_POINT('Ctrl Pts',(-22.2385031763588,14.5537967295509,
130.324774213343)) ;
#154022=CARTESIAN_POINT('Ctrl Pts',(-22.2766625743414,14.5727057162824,
130.436247852826)) ;
#154023=CARTESIAN_POINT('Ctrl Pts',(-22.315137886939,14.5729486706397,130.548644361973)) ;
#154024=CARTESIAN_POINT('Ctrl Pts',(-22.6320187065115,12.9778651918055,
131.474336592418)) ;
#154025=CARTESIAN_POINT('Ctrl Pts',(-22.6319017381682,12.9780271046061,
131.473994897119)) ;
#154026=CARTESIAN_POINT('Ctrl Pts',(-22.6318028115373,12.9782537499186,
131.473705906407)) ;
#154027=CARTESIAN_POINT('Ctrl Pts',(-22.631613822165,12.9788663176294,131.473153818736)) ;
#154028=CARTESIAN_POINT('Ctrl Pts',(-22.6315335379757,12.9792529318746,
131.4729192875)) ;
#154029=CARTESIAN_POINT('Ctrl Pts',(-22.6313068850366,12.9806654239861,
131.472257174643)) ;
#154030=CARTESIAN_POINT('Ctrl Pts',(-22.6312165058438,12.9819390751954,
131.471993153247)) ;
#154031=CARTESIAN_POINT('Ctrl Pts',(-22.6310413042841,12.9863682734726,
131.471481343404)) ;
#154032=CARTESIAN_POINT('Ctrl Pts',(-22.6311111509824,12.990696770219,131.471685383983)) ;
#154033=CARTESIAN_POINT('Ctrl Pts',(-22.6317823753756,13.0076193276447,
131.473646207003)) ;
#154034=CARTESIAN_POINT('Ctrl Pts',(-22.632964539542,13.0243616968384,131.477099619508)) ;
#154035=CARTESIAN_POINT('Ctrl Pts',(-22.6380372471069,13.0936611830537,
131.491918332697)) ;
#154036=CARTESIAN_POINT('Ctrl Pts',(-22.6433073952143,13.1624395523347,
131.507313821644)) ;
#154037=CARTESIAN_POINT('Ctrl Pts',(-22.6510369822631,13.3897587207643,
131.529893978705)) ;
#154038=CARTESIAN_POINT('Ctrl Pts',(-22.6470299561775,13.5079529376015,
131.518188401448)) ;
#154039=CARTESIAN_POINT('Ctrl Pts',(-22.6312468100604,13.7299217778491,
131.472081679835)) ;
#154040=CARTESIAN_POINT('Ctrl Pts',(-22.6154442941006,13.847789885417,131.425918373818)) ;
#154041=CARTESIAN_POINT('Ctrl Pts',(-22.568941208862,14.0688613754809,131.290070629056)) ;
#154042=CARTESIAN_POINT('Ctrl Pts',(-22.5376677274684,14.1680229125909,
131.198712563319)) ;
#154043=CARTESIAN_POINT('Ctrl Pts',(-22.4733491505273,14.3035692712769,
131.010821080874)) ;
#154044=CARTESIAN_POINT('Ctrl Pts',(-22.4429615479491,14.3485547863788,
130.922050900127)) ;
#154045=CARTESIAN_POINT('Ctrl Pts',(-22.3797662254967,14.4080651754862,
130.737440739519)) ;
#154046=CARTESIAN_POINT('Ctrl Pts',(-22.3476163144776,14.4229807584986,
130.643522392363)) ;
#154047=CARTESIAN_POINT('Ctrl Pts',(-22.3151378869399,14.4232238463042,
130.548644361976)) ;
#154048=CARTESIAN_POINT('Ctrl Pts',(-33.3489959095147,13.1551399285885,
127.871927411069)) ;
#154049=CARTESIAN_POINT('Ctrl Pts',(-33.3254395351173,13.1734341962953,
127.803113044878)) ;
#154050=CARTESIAN_POINT('Ctrl Pts',(-33.254172394553,13.1734341962953,127.827509047315)) ;
#154051=CARTESIAN_POINT('Ctrl Pts',(-33.1829052539887,13.1734341962953,
127.851905049753)) ;
#154052=CARTESIAN_POINT('Ctrl Pts',(-33.2064616283861,13.1551399285885,
127.920719415945)) ;
#154053=CARTESIAN_POINT('Ctrl Pts',(-33.2300180027834,13.1368456608817,
127.989533782136)) ;
#154054=CARTESIAN_POINT('Ctrl Pts',(-33.3012851433477,13.1368456608817,
127.965137779698)) ;
#154055=CARTESIAN_POINT('Ctrl Pts',(-33.372552283912,13.1368456608817,127.94074177726)) ;
#154056=CARTESIAN_POINT('Ctrl Pts',(-33.3489959095147,13.1551399285885,
127.871927411069)) ;
#154057=CARTESIAN_POINT('Ctrl Pts',(-33.3504264730207,13.191264605624,127.881753249117)) ;
#154058=CARTESIAN_POINT('Ctrl Pts',(-33.3264562033862,13.1991216594078,
127.810292753008)) ;
#154059=CARTESIAN_POINT('Ctrl Pts',(-33.2553374556519,13.2028260557706,
127.835126718908)) ;
#154060=CARTESIAN_POINT('Ctrl Pts',(-33.1842187079176,13.2065304521335,
127.859960684809)) ;
#154061=CARTESIAN_POINT('Ctrl Pts',(-33.2081889775521,13.1986733983497,
127.931421180918)) ;
#154062=CARTESIAN_POINT('Ctrl Pts',(-33.2321592471865,13.1908163445659,
128.002881677027)) ;
#154063=CARTESIAN_POINT('Ctrl Pts',(-33.3032779949208,13.1871119482031,
127.978047711127)) ;
#154064=CARTESIAN_POINT('Ctrl Pts',(-33.3743967426551,13.1834075518402,
127.953213745226)) ;
#154065=CARTESIAN_POINT('Ctrl Pts',(-33.3504264730207,13.191264605624,127.881753249117)) ;
#154066=CARTESIAN_POINT('Ctrl Pts',(-33.3535207816705,13.268036520819,127.884470294454)) ;
#154067=CARTESIAN_POINT('Ctrl Pts',(-33.3286589899815,13.2538025217343,
127.812609970312)) ;
#154068=CARTESIAN_POINT('Ctrl Pts',(-33.2578501843241,13.2651134066728,
127.836584356188)) ;
#154069=CARTESIAN_POINT('Ctrl Pts',(-33.1870413786667,13.2764242916113,
127.860558742064)) ;
#154070=CARTESIAN_POINT('Ctrl Pts',(-33.2119031703558,13.290658290696,127.932419066205)) ;
#154071=CARTESIAN_POINT('Ctrl Pts',(-33.2367649620448,13.3048922897807,
128.004279390347)) ;
#154072=CARTESIAN_POINT('Ctrl Pts',(-33.3075737677022,13.2935814048422,
127.980305004471)) ;
#154073=CARTESIAN_POINT('Ctrl Pts',(-33.3783825733595,13.2822705199037,
127.956330618595)) ;
#154074=CARTESIAN_POINT('Ctrl Pts',(-33.3535207816705,13.268036520819,127.884470294454)) ;
#154075=CARTESIAN_POINT('Ctrl Pts',(-33.3579140346178,13.3732912215196,
127.837501420712)) ;
#154076=CARTESIAN_POINT('Ctrl Pts',(-33.3317967099876,13.3290215614615,
127.779671185695)) ;
#154077=CARTESIAN_POINT('Ctrl Pts',(-33.2613977067381,13.3500184403787,
127.797470635037)) ;
#154078=CARTESIAN_POINT('Ctrl Pts',(-33.1909987034886,13.371015319296,127.815270084379)) ;
#154079=CARTESIAN_POINT('Ctrl Pts',(-33.2171160281188,13.4152849793541,
127.873100319396)) ;
#154080=CARTESIAN_POINT('Ctrl Pts',(-33.243233352749,13.4595546394122,127.930930554413)) ;
#154081=CARTESIAN_POINT('Ctrl Pts',(-33.3136323559985,13.4385577604949,
127.913131105071)) ;
#154082=CARTESIAN_POINT('Ctrl Pts',(-33.3840313592479,13.4175608815777,
127.895331655729)) ;
#154083=CARTESIAN_POINT('Ctrl Pts',(-33.3579140346178,13.3732912215196,
127.837501420712)) ;
#154084=CARTESIAN_POINT('Ctrl Pts',(-33.3611609335145,13.4471111688333,
127.748905537657)) ;
#154085=CARTESIAN_POINT('Ctrl Pts',(-33.3341265408441,13.3820520008154,
127.716920013205)) ;
#154086=CARTESIAN_POINT('Ctrl Pts',(-33.2639983405158,13.409026910249,127.724903336633)) ;
#154087=CARTESIAN_POINT('Ctrl Pts',(-33.1938701401876,13.4360018196825,
127.732886660062)) ;
#154088=CARTESIAN_POINT('Ctrl Pts',(-33.220904532858,13.5010609877004,127.764872184514)) ;
#154089=CARTESIAN_POINT('Ctrl Pts',(-33.2479389255284,13.5661201557183,
127.796857708966)) ;
#154090=CARTESIAN_POINT('Ctrl Pts',(-33.3180671258566,13.5391452462847,
127.788874385537)) ;
#154091=CARTESIAN_POINT('Ctrl Pts',(-33.3881953261848,13.5121703368512,
127.780891062108)) ;
#154092=CARTESIAN_POINT('Ctrl Pts',(-33.3611609335145,13.4471111688333,
127.748905537657)) ;
#154093=CARTESIAN_POINT('Ctrl Pts',(-33.3621234180406,13.4654248347116,
127.67420492204)) ;
#154094=CARTESIAN_POINT('Ctrl Pts',(-33.3348269327376,13.3954694274565,
127.663792350738)) ;
#154095=CARTESIAN_POINT('Ctrl Pts',(-33.2647501798453,13.4231551632892,
127.664144174588)) ;
#154096=CARTESIAN_POINT('Ctrl Pts',(-33.1946734269531,13.4508408991218,
127.664495998438)) ;
#154097=CARTESIAN_POINT('Ctrl Pts',(-33.2219699122561,13.5207963063769,
127.67490856974)) ;
#154098=CARTESIAN_POINT('Ctrl Pts',(-33.2492663975591,13.5907517136319,
127.685321141042)) ;
#154099=CARTESIAN_POINT('Ctrl Pts',(-33.3193431504514,13.5630659777992,
127.684969317192)) ;
#154100=CARTESIAN_POINT('Ctrl Pts',(-33.3894199033436,13.5353802419666,
127.684617493342)) ;
#154101=CARTESIAN_POINT('Ctrl Pts',(-33.3621234180406,13.4654248347116,
127.67420492204)) ;
#154102=CARTESIAN_POINT('Ctrl Pts',(-33.3622513221686,13.4658285122696,
127.63672629787)) ;
#154103=CARTESIAN_POINT('Ctrl Pts',(-33.3349255565294,13.3959427988304,
127.637093604187)) ;
#154104=CARTESIAN_POINT('Ctrl Pts',(-33.2648392434469,13.4231193515827,
127.633745568972)) ;
#154105=CARTESIAN_POINT('Ctrl Pts',(-33.1947529303645,13.4502959043349,
127.630397533756)) ;
#154106=CARTESIAN_POINT('Ctrl Pts',(-33.2220786960038,13.5201816177741,
127.63003022744)) ;
#154107=CARTESIAN_POINT('Ctrl Pts',(-33.2494044616431,13.5900673312133,
127.629662921123)) ;
#154108=CARTESIAN_POINT('Ctrl Pts',(-33.3194907747255,13.562890778461,127.633010956338)) ;
#154109=CARTESIAN_POINT('Ctrl Pts',(-33.3895770878079,13.5357142257088,
127.636358991554)) ;
#154110=CARTESIAN_POINT('Ctrl Pts',(-33.3622513221686,13.4658285122696,
127.63672629787)) ;
#154111=CARTESIAN_POINT('',(-33.3622513221686,13.4658285122696,127.63672629787)) ;
#154112=CARTESIAN_POINT('Ctrl Pts',(-33.3489959095147,13.1551399285885,
127.871927411069)) ;
#154113=CARTESIAN_POINT('Ctrl Pts',(-33.3504264730207,13.191264605624,127.881753249117)) ;
#154114=CARTESIAN_POINT('Ctrl Pts',(-33.3535207816705,13.268036520819,127.884470294454)) ;
#154115=CARTESIAN_POINT('Ctrl Pts',(-33.3579140346178,13.3732912215196,
127.837501420712)) ;
#154116=CARTESIAN_POINT('Ctrl Pts',(-33.3611609335145,13.4471111688333,
127.748905537657)) ;
#154117=CARTESIAN_POINT('Ctrl Pts',(-33.3621234180406,13.4654248347116,
127.67420492204)) ;
#154118=CARTESIAN_POINT('Ctrl Pts',(-33.3622513221686,13.4658285122696,
127.63672629787)) ;
#154119=CARTESIAN_POINT('Origin',(-33.2921650090862,13.4930050650219,127.633378262655)) ;
#154120=CARTESIAN_POINT('Ctrl Pts',(-33.3622513221686,13.4658285122696,
127.63672629787)) ;
#154121=CARTESIAN_POINT('Ctrl Pts',(-33.3349255565294,13.3959427988304,
127.637093604187)) ;
#154122=CARTESIAN_POINT('Ctrl Pts',(-33.2648392434469,13.4231193515827,
127.633745568972)) ;
#154123=CARTESIAN_POINT('Ctrl Pts',(-33.1947529303645,13.4502959043349,
127.630397533756)) ;
#154124=CARTESIAN_POINT('Ctrl Pts',(-33.2220786960038,13.5201816177741,
127.63003022744)) ;
#154125=CARTESIAN_POINT('Ctrl Pts',(-33.2494044616431,13.5900673312133,
127.629662921123)) ;
#154126=CARTESIAN_POINT('Ctrl Pts',(-33.3194907747255,13.562890778461,127.633010956338)) ;
#154127=CARTESIAN_POINT('Ctrl Pts',(-33.3895770878079,13.5357142257088,
127.636358991554)) ;
#154128=CARTESIAN_POINT('Ctrl Pts',(-33.3622513221686,13.4658285122696,
127.63672629787)) ;
#154129=CARTESIAN_POINT('Ctrl Pts',(-33.3634081045458,13.4658294080177,
127.254746417056)) ;
#154130=CARTESIAN_POINT('Ctrl Pts',(-33.3360823389065,13.3959436945786,
127.255113723373)) ;
#154131=CARTESIAN_POINT('Ctrl Pts',(-33.2659960258241,13.4231202473308,
127.251765688157)) ;
#154132=CARTESIAN_POINT('Ctrl Pts',(-33.1959097127417,13.4502968000831,
127.248417652942)) ;
#154133=CARTESIAN_POINT('Ctrl Pts',(-33.2232354783809,13.5201825135223,
127.248050346625)) ;
#154134=CARTESIAN_POINT('Ctrl Pts',(-33.2505612440202,13.5900682269615,
127.247683040309)) ;
#154135=CARTESIAN_POINT('Ctrl Pts',(-33.3206475571026,13.5628916742092,
127.251031075524)) ;
#154136=CARTESIAN_POINT('Ctrl Pts',(-33.3907338701851,13.5357151214569,
127.25437911074)) ;
#154137=CARTESIAN_POINT('Ctrl Pts',(-33.3634081045458,13.4658294080177,
127.254746417056)) ;
#154138=CARTESIAN_POINT('Ctrl Pts',(-33.364564886923,13.4658303037659,126.872766536242)) ;
#154139=CARTESIAN_POINT('Ctrl Pts',(-33.3372391212837,13.3959445903267,
126.873133842559)) ;
#154140=CARTESIAN_POINT('Ctrl Pts',(-33.2671528082013,13.423121143079,126.869785807343)) ;
#154141=CARTESIAN_POINT('Ctrl Pts',(-33.1970664951188,13.4502976958313,
126.866437772128)) ;
#154142=CARTESIAN_POINT('Ctrl Pts',(-33.2243922607581,13.5201834092705,
126.866070465811)) ;
#154143=CARTESIAN_POINT('Ctrl Pts',(-33.2517180263974,13.5900691227097,
126.865703159495)) ;
#154144=CARTESIAN_POINT('Ctrl Pts',(-33.3218043394798,13.5628925699574,
126.86905119471)) ;
#154145=CARTESIAN_POINT('Ctrl Pts',(-33.3918906525622,13.5357160172051,
126.872399229925)) ;
#154146=CARTESIAN_POINT('Ctrl Pts',(-33.364564886923,13.4658303037659,126.872766536242)) ;
#154147=CARTESIAN_POINT('Ctrl Pts',(-33.3657216693001,13.4658311995141,
126.490786655428)) ;
#154148=CARTESIAN_POINT('Ctrl Pts',(-33.3383959036609,13.3959454860749,
126.491153961744)) ;
#154149=CARTESIAN_POINT('Ctrl Pts',(-33.2683095905784,13.4231220388272,
126.487805926529)) ;
#154150=CARTESIAN_POINT('Ctrl Pts',(-33.198223277496,13.4502985915795,126.484457891314)) ;
#154151=CARTESIAN_POINT('Ctrl Pts',(-33.2255490431353,13.5201843050187,
126.484090584997)) ;
#154152=CARTESIAN_POINT('Ctrl Pts',(-33.2528748087745,13.5900700184578,
126.48372327868)) ;
#154153=CARTESIAN_POINT('Ctrl Pts',(-33.322961121857,13.5628934657056,126.487071313896)) ;
#154154=CARTESIAN_POINT('Ctrl Pts',(-33.3930474349394,13.5357169129533,
126.490419349111)) ;
#154155=CARTESIAN_POINT('Ctrl Pts',(-33.3657216693001,13.4658311995141,
126.490786655428)) ;
#154156=CARTESIAN_POINT('',(-33.3657216693001,13.4658311995141,126.490786655428)) ;
#154157=CARTESIAN_POINT('',(-33.3622513221686,13.4658285122696,127.63672629787)) ;
#154158=CARTESIAN_POINT('',(-33.2955665703368,13.4180239009611,126.488994292619)) ;
#154159=CARTESIAN_POINT('Origin',(-33.2956353562177,13.4930077522664,126.487438620212)) ;
#154160=CARTESIAN_POINT('',(-33.2957040070394,13.5679916035759,126.485882942442)) ;
#154161=CARTESIAN_POINT('Origin',(-33.2956353562177,13.4930077522664,126.487438620212)) ;
#154162=CARTESIAN_POINT('Origin',(-33.2956353562177,13.4930077522664,126.487438620212)) ;
#154163=CARTESIAN_POINT('Ctrl Pts',(-33.3657216693001,13.4658311995141,
126.490786655428)) ;
#154164=CARTESIAN_POINT('Ctrl Pts',(-33.3383959036609,13.3959454860749,
126.491153961744)) ;
#154165=CARTESIAN_POINT('Ctrl Pts',(-33.2683095905784,13.4231220388272,
126.487805926529)) ;
#154166=CARTESIAN_POINT('Ctrl Pts',(-33.198223277496,13.4502985915795,126.484457891314)) ;
#154167=CARTESIAN_POINT('Ctrl Pts',(-33.2255490431353,13.5201843050187,
126.484090584997)) ;
#154168=CARTESIAN_POINT('Ctrl Pts',(-33.2528748087745,13.5900700184578,
126.48372327868)) ;
#154169=CARTESIAN_POINT('Ctrl Pts',(-33.322961121857,13.5628934657056,126.487071313896)) ;
#154170=CARTESIAN_POINT('Ctrl Pts',(-33.3930474349394,13.5357169129533,
126.490419349111)) ;
#154171=CARTESIAN_POINT('Ctrl Pts',(-33.3657216693001,13.4658311995141,
126.490786655428)) ;
#154172=CARTESIAN_POINT('Ctrl Pts',(-33.3710709437106,13.4658311995141,
126.425157509608)) ;
#154173=CARTESIAN_POINT('Ctrl Pts',(-33.343714479123,13.3959454860749,126.422780862853)) ;
#154174=CARTESIAN_POINT('Ctrl Pts',(-33.2739832165657,13.4231220388272,
126.412393722814)) ;
#154175=CARTESIAN_POINT('Ctrl Pts',(-33.2042519540084,13.4502985915795,
126.402006582774)) ;
#154176=CARTESIAN_POINT('Ctrl Pts',(-33.2316084185959,13.5201843050187,
126.404383229528)) ;
#154177=CARTESIAN_POINT('Ctrl Pts',(-33.2589648831834,13.5900700184579,
126.406759876282)) ;
#154178=CARTESIAN_POINT('Ctrl Pts',(-33.3286961457408,13.5628934657056,
126.417147016322)) ;
#154179=CARTESIAN_POINT('Ctrl Pts',(-33.3984274082981,13.5357169129533,
126.427534156362)) ;
#154180=CARTESIAN_POINT('Ctrl Pts',(-33.3710709437106,13.4658311995141,
126.425157509608)) ;
#154181=CARTESIAN_POINT('Ctrl Pts',(-33.4026727151281,13.4658311995141,
126.292213744632)) ;
#154182=CARTESIAN_POINT('Ctrl Pts',(-33.3761162339872,13.3959454860749,
126.284199283461)) ;
#154183=CARTESIAN_POINT('Ctrl Pts',(-33.3093262459584,13.4231220388272,
126.259484856214)) ;
#154184=CARTESIAN_POINT('Ctrl Pts',(-33.2425362579296,13.4502985915795,
126.234770428968)) ;
#154185=CARTESIAN_POINT('Ctrl Pts',(-33.2690927390706,13.5201843050187,
126.242784890139)) ;
#154186=CARTESIAN_POINT('Ctrl Pts',(-33.2956492202115,13.5900700184578,
126.250799351311)) ;
#154187=CARTESIAN_POINT('Ctrl Pts',(-33.3624392082402,13.5628934657056,
126.275513778557)) ;
#154188=CARTESIAN_POINT('Ctrl Pts',(-33.429229196269,13.5357169129533,126.300228205804)) ;
#154189=CARTESIAN_POINT('Ctrl Pts',(-33.4026727151281,13.4658311995141,
126.292213744632)) ;
#154190=CARTESIAN_POINT('Ctrl Pts',(-33.5097508222684,13.4658311995141,
126.114873926673)) ;
#154191=CARTESIAN_POINT('Ctrl Pts',(-33.4869569930479,13.3959454860749,
126.099090565098)) ;
#154192=CARTESIAN_POINT('Ctrl Pts',(-33.4310376162827,13.4231220388272,
126.055050770833)) ;
#154193=CARTESIAN_POINT('Ctrl Pts',(-33.3751182395174,13.4502985915795,
126.011010976568)) ;
#154194=CARTESIAN_POINT('Ctrl Pts',(-33.3979120687378,13.5201843050187,
126.026794338144)) ;
#154195=CARTESIAN_POINT('Ctrl Pts',(-33.4207058979582,13.5900700184579,
126.042577699719)) ;
#154196=CARTESIAN_POINT('Ctrl Pts',(-33.4766252747235,13.5628934657056,
126.086617493984)) ;
#154197=CARTESIAN_POINT('Ctrl Pts',(-33.5325446514888,13.5357169129533,
126.130657288248)) ;
#154198=CARTESIAN_POINT('Ctrl Pts',(-33.5097508222684,13.4658311995141,
126.114873926673)) ;
#154199=CARTESIAN_POINT('Ctrl Pts',(-33.6669726245832,13.4658311995141,
125.979587612656)) ;
#154200=CARTESIAN_POINT('Ctrl Pts',(-33.6501853294574,13.3959454860749,
125.957588672145)) ;
#154201=CARTESIAN_POINT('Ctrl Pts',(-33.6106414771463,13.4231220388272,
125.898557790685)) ;
#154202=CARTESIAN_POINT('Ctrl Pts',(-33.5710976248353,13.4502985915795,
125.839526909225)) ;
#154203=CARTESIAN_POINT('Ctrl Pts',(-33.5878849199611,13.5201843050187,
125.861525849736)) ;
#154204=CARTESIAN_POINT('Ctrl Pts',(-33.6046722150869,13.5900700184578,
125.883524790247)) ;
#154205=CARTESIAN_POINT('Ctrl Pts',(-33.6442160673979,13.5628934657056,
125.942555671708)) ;
#154206=CARTESIAN_POINT('Ctrl Pts',(-33.683759919709,13.5357169129533,126.001586553168)) ;
#154207=CARTESIAN_POINT('Ctrl Pts',(-33.6669726245832,13.4658311995141,
125.979587612656)) ;
#154208=CARTESIAN_POINT('Ctrl Pts',(-33.8546539670386,13.4658311995141,
125.899837483417)) ;
#154209=CARTESIAN_POINT('Ctrl Pts',(-33.8453517619418,13.3959454860749,
125.873811092798)) ;
#154210=CARTESIAN_POINT('Ctrl Pts',(-33.825626690385,13.4231220388272,125.805630627847)) ;
#154211=CARTESIAN_POINT('Ctrl Pts',(-33.8059016188281,13.4502985915795,
125.737450162897)) ;
#154212=CARTESIAN_POINT('Ctrl Pts',(-33.8152038239249,13.5201843050187,
125.763476553515)) ;
#154213=CARTESIAN_POINT('Ctrl Pts',(-33.8245060290216,13.5900700184579,
125.789502944134)) ;
#154214=CARTESIAN_POINT('Ctrl Pts',(-33.8442311005785,13.5628934657056,
125.857683409085)) ;
#154215=CARTESIAN_POINT('Ctrl Pts',(-33.8639561721354,13.5357169129533,
125.925863874035)) ;
#154216=CARTESIAN_POINT('Ctrl Pts',(-33.8546539670386,13.4658311995141,
125.899837483417)) ;
#154217=CARTESIAN_POINT('Ctrl Pts',(-34.0574909713096,13.4658311995141,
125.879315368324)) ;
#154218=CARTESIAN_POINT('Ctrl Pts',(-34.056531236216,13.3959454860749,125.851661404809)) ;
#154219=CARTESIAN_POINT('Ctrl Pts',(-34.0584428323337,13.4231220388272,
125.780618176254)) ;
#154220=CARTESIAN_POINT('Ctrl Pts',(-34.0603544284514,13.4502985915795,
125.709574947699)) ;
#154221=CARTESIAN_POINT('Ctrl Pts',(-34.061314163545,13.5201843050187,125.737228911215)) ;
#154222=CARTESIAN_POINT('Ctrl Pts',(-34.0622738986387,13.5900700184579,
125.76488287473)) ;
#154223=CARTESIAN_POINT('Ctrl Pts',(-34.0603623025209,13.5628934657056,
125.835926103285)) ;
#154224=CARTESIAN_POINT('Ctrl Pts',(-34.0584507064032,13.5357169129533,
125.90696933184)) ;
#154225=CARTESIAN_POINT('Ctrl Pts',(-34.0574909713096,13.4658311995141,
125.879315368324)) ;
#154226=CARTESIAN_POINT('Ctrl Pts',(-34.2603174788621,13.4658311995141,
125.922153820006)) ;
#154227=CARTESIAN_POINT('Ctrl Pts',(-34.2679438333246,13.3959454860749,
125.895501671555)) ;
#154228=CARTESIAN_POINT('Ctrl Pts',(-34.2917008109883,13.4231220388272,
125.828374514453)) ;
#154229=CARTESIAN_POINT('Ctrl Pts',(-34.3154577886521,13.4502985915795,
125.76124735735)) ;
#154230=CARTESIAN_POINT('Ctrl Pts',(-34.3078314341896,13.5201843050187,
125.787899505801)) ;
#154231=CARTESIAN_POINT('Ctrl Pts',(-34.3002050797271,13.5900700184579,
125.814551654251)) ;
#154232=CARTESIAN_POINT('Ctrl Pts',(-34.2764481020633,13.5628934657056,
125.881678811354)) ;
#154233=CARTESIAN_POINT('Ctrl Pts',(-34.2526911243996,13.5357169129533,
125.948805968456)) ;
#154234=CARTESIAN_POINT('Ctrl Pts',(-34.2603174788621,13.4658311995141,
125.922153820006)) ;
#154235=CARTESIAN_POINT('Ctrl Pts',(-34.4394051996481,13.4658311995141,
126.026010217586)) ;
#154236=CARTESIAN_POINT('Ctrl Pts',(-34.4548670732842,13.3959454860749,
126.002982829036)) ;
#154237=CARTESIAN_POINT('Ctrl Pts',(-34.4981313355085,13.4231220388272,
125.946377991427)) ;
#154238=CARTESIAN_POINT('Ctrl Pts',(-34.5413955977328,13.4502985915795,
125.889773153818)) ;
#154239=CARTESIAN_POINT('Ctrl Pts',(-34.5259337240967,13.5201843050187,
125.912800542368)) ;
#154240=CARTESIAN_POINT('Ctrl Pts',(-34.5104718504605,13.5900700184578,
125.935827930917)) ;
#154241=CARTESIAN_POINT('Ctrl Pts',(-34.4672075882362,13.5628934657056,
125.992432768526)) ;
#154242=CARTESIAN_POINT('Ctrl Pts',(-34.423943326012,13.5357169129533,126.049037606135)) ;
#154243=CARTESIAN_POINT('Ctrl Pts',(-34.4394051996481,13.4658311995141,
126.026010217586)) ;
#154244=CARTESIAN_POINT('Ctrl Pts',(-34.5756161826405,13.4658311995141,
126.176769282622)) ;
#154245=CARTESIAN_POINT('Ctrl Pts',(-34.5973140532962,13.3959454860749,
126.159477051786)) ;
#154246=CARTESIAN_POINT('Ctrl Pts',(-34.6556528941974,13.4231220388272,
126.118553567228)) ;
#154247=CARTESIAN_POINT('Ctrl Pts',(-34.7139917350986,13.4502985915795,
126.07763008267)) ;
#154248=CARTESIAN_POINT('Ctrl Pts',(-34.6922938644429,13.5201843050187,
126.094922313507)) ;
#154249=CARTESIAN_POINT('Ctrl Pts',(-34.6705959937872,13.5900700184578,
126.112214544343)) ;
#154250=CARTESIAN_POINT('Ctrl Pts',(-34.612257152886,13.5628934657056,126.153138028901)) ;
#154251=CARTESIAN_POINT('Ctrl Pts',(-34.5539183119848,13.5357169129533,
126.194061513458)) ;
#154252=CARTESIAN_POINT('Ctrl Pts',(-34.5756161826405,13.4658311995141,
126.176769282622)) ;
#154253=CARTESIAN_POINT('Ctrl Pts',(-34.6605098387667,13.4658311995141,
126.361211761343)) ;
#154254=CARTESIAN_POINT('Ctrl Pts',(-34.6864428238696,13.3959454860749,
126.351248800186)) ;
#154255=CARTESIAN_POINT('Ctrl Pts',(-34.7544765704431,13.4231220388272,
126.329779166733)) ;
#154256=CARTESIAN_POINT('Ctrl Pts',(-34.8225103170166,13.4502985915795,
126.308309533281)) ;
#154257=CARTESIAN_POINT('Ctrl Pts',(-34.7965773319137,13.5201843050187,
126.318272494438)) ;
#154258=CARTESIAN_POINT('Ctrl Pts',(-34.7706443468108,13.5900700184578,
126.328235455595)) ;
#154259=CARTESIAN_POINT('Ctrl Pts',(-34.7026106002373,13.5628934657056,
126.349705089048)) ;
#154260=CARTESIAN_POINT('Ctrl Pts',(-34.6345768536637,13.5357169129533,
126.3711747225)) ;
#154261=CARTESIAN_POINT('Ctrl Pts',(-34.6605098387667,13.4658311995141,
126.361211761343)) ;
#154262=CARTESIAN_POINT('Ctrl Pts',(-34.6852735030978,13.4658311995141,
126.56639932233)) ;
#154263=CARTESIAN_POINT('Ctrl Pts',(-34.7130249936416,13.3959454860749,
126.564856538092)) ;
#154264=CARTESIAN_POINT('Ctrl Pts',(-34.7843881220333,13.4231220388272,
126.56525799732)) ;
#154265=CARTESIAN_POINT('Ctrl Pts',(-34.8557512504251,13.4502985915795,
126.565659456548)) ;
#154266=CARTESIAN_POINT('Ctrl Pts',(-34.8279997598812,13.5201843050187,
126.567202240786)) ;
#154267=CARTESIAN_POINT('Ctrl Pts',(-34.8002482693373,13.5900700184579,
126.568745025024)) ;
#154268=CARTESIAN_POINT('Ctrl Pts',(-34.7288851409456,13.5628934657056,
126.568343565796)) ;
#154269=CARTESIAN_POINT('Ctrl Pts',(-34.6575220125539,13.5357169129533,
126.567942106568)) ;
#154270=CARTESIAN_POINT('Ctrl Pts',(-34.6852735030978,13.4658311995141,
126.56639932233)) ;
#154271=CARTESIAN_POINT('Ctrl Pts',(-34.6444773076006,13.4658311995141,
126.769201249595)) ;
#154272=CARTESIAN_POINT('Ctrl Pts',(-34.6713161577667,13.3959454860749,
126.776230438729)) ;
#154273=CARTESIAN_POINT('Ctrl Pts',(-34.7389855153722,13.4231220388272,
126.79846338974)) ;
#154274=CARTESIAN_POINT('Ctrl Pts',(-34.8066548729777,13.4502985915795,
126.820696340751)) ;
#154275=CARTESIAN_POINT('Ctrl Pts',(-34.7798160228116,13.5201843050187,
126.813667151617)) ;
#154276=CARTESIAN_POINT('Ctrl Pts',(-34.7529771726455,13.5900700184579,
126.806637962483)) ;
#154277=CARTESIAN_POINT('Ctrl Pts',(-34.68530781504,13.5628934657056,126.784405011472)) ;
#154278=CARTESIAN_POINT('Ctrl Pts',(-34.6176384574345,13.5357169129533,
126.762172060461)) ;
#154279=CARTESIAN_POINT('Ctrl Pts',(-34.6444773076006,13.4658311995141,
126.769201249595)) ;
#154280=CARTESIAN_POINT('Ctrl Pts',(-34.5453436411495,13.4658311995141,
126.946957684585)) ;
#154281=CARTESIAN_POINT('Ctrl Pts',(-34.5687512865745,13.3959454860749,
126.961742671916)) ;
#154282=CARTESIAN_POINT('Ctrl Pts',(-34.6264015098537,13.4231220388272,
127.003319432827)) ;
#154283=CARTESIAN_POINT('Ctrl Pts',(-34.6840517331329,13.4502985915795,
127.044896193737)) ;
#154284=CARTESIAN_POINT('Ctrl Pts',(-34.6606440877079,13.5201843050187,
127.030111206405)) ;
#154285=CARTESIAN_POINT('Ctrl Pts',(-34.6372364422829,13.5900700184578,
127.015326219074)) ;
#154286=CARTESIAN_POINT('Ctrl Pts',(-34.5795862190037,13.5628934657056,
126.973749458163)) ;
#154287=CARTESIAN_POINT('Ctrl Pts',(-34.5219359957245,13.5357169129533,
126.932172697253)) ;
#154288=CARTESIAN_POINT('Ctrl Pts',(-34.5453436411495,13.4658311995141,
126.946957684585)) ;
#154289=CARTESIAN_POINT('Ctrl Pts',(-34.397695173349,13.4658311995141,127.087382113455)) ;
#154290=CARTESIAN_POINT('Ctrl Pts',(-34.4155135478261,13.3959454860749,
127.108559279803)) ;
#154291=CARTESIAN_POINT('Ctrl Pts',(-34.4578296604691,13.4231220388272,
127.16564535534)) ;
#154292=CARTESIAN_POINT('Ctrl Pts',(-34.500145773112,13.4502985915795,127.222731430876)) ;
#154293=CARTESIAN_POINT('Ctrl Pts',(-34.4823273986348,13.5201843050187,
127.201554264528)) ;
#154294=CARTESIAN_POINT('Ctrl Pts',(-34.4645090241577,13.5900700184578,
127.18037709818)) ;
#154295=CARTESIAN_POINT('Ctrl Pts',(-34.4221929115148,13.5628934657056,
127.123291022643)) ;
#154296=CARTESIAN_POINT('Ctrl Pts',(-34.3798767988718,13.5357169129533,
127.066204947107)) ;
#154297=CARTESIAN_POINT('Ctrl Pts',(-34.397695173349,13.4658311995141,127.087382113455)) ;
#154298=CARTESIAN_POINT('Ctrl Pts',(-34.2109661436266,13.4658311995141,
127.177936318607)) ;
#154299=CARTESIAN_POINT('Ctrl Pts',(-34.2213805824851,13.3959454860749,
127.203585641458)) ;
#154300=CARTESIAN_POINT('Ctrl Pts',(-34.244015597737,13.4231220388272,127.270974071339)) ;
#154301=CARTESIAN_POINT('Ctrl Pts',(-34.266650612989,13.4502985915795,127.338362501219)) ;
#154302=CARTESIAN_POINT('Ctrl Pts',(-34.2562361741305,13.5201843050187,
127.312713178368)) ;
#154303=CARTESIAN_POINT('Ctrl Pts',(-34.245821735272,13.5900700184579,127.287063855517)) ;
#154304=CARTESIAN_POINT('Ctrl Pts',(-34.2231867200201,13.5628934657056,
127.219675425636)) ;
#154305=CARTESIAN_POINT('Ctrl Pts',(-34.2005517047682,13.5357169129533,
127.152286995756)) ;
#154306=CARTESIAN_POINT('Ctrl Pts',(-34.2109661436266,13.4658311995141,
127.177936318607)) ;
#154307=CARTESIAN_POINT('Ctrl Pts',(-34.0053608811418,13.4658311995141,
127.205905827809)) ;
#154308=CARTESIAN_POINT('Ctrl Pts',(-34.0073466019005,13.3959454860749,
127.233502366642)) ;
#154309=CARTESIAN_POINT('Ctrl Pts',(-34.0080733954292,13.4231220388272,
127.304559444664)) ;
#154310=CARTESIAN_POINT('Ctrl Pts',(-34.0088001889578,13.4502985915795,
127.375616522685)) ;
#154311=CARTESIAN_POINT('Ctrl Pts',(-34.006814468199,13.5201843050187,127.348019983852)) ;
#154312=CARTESIAN_POINT('Ctrl Pts',(-34.0048287474402,13.5900700184578,
127.320423445019)) ;
#154313=CARTESIAN_POINT('Ctrl Pts',(-34.0041019539116,13.5628934657056,
127.249366366998)) ;
#154314=CARTESIAN_POINT('Ctrl Pts',(-34.003375160383,13.5357169129533,127.178309288976)) ;
#154315=CARTESIAN_POINT('Ctrl Pts',(-34.0053608811418,13.4658311995141,
127.205905827809)) ;
#154316=CARTESIAN_POINT('Ctrl Pts',(-33.8704755222901,13.4658311995141,
127.182274454702)) ;
#154317=CARTESIAN_POINT('Ctrl Pts',(-33.8667699608776,13.3959454860749,
127.209406331759)) ;
#154318=CARTESIAN_POINT('Ctrl Pts',(-33.8529850451152,13.4231220388272,
127.278378794431)) ;
#154319=CARTESIAN_POINT('Ctrl Pts',(-33.8392001293528,13.4502985915795,
127.347351257104)) ;
#154320=CARTESIAN_POINT('Ctrl Pts',(-33.8429056907652,13.5201843050187,
127.320219380047)) ;
#154321=CARTESIAN_POINT('Ctrl Pts',(-33.8466112521777,13.5900700184578,
127.29308750299)) ;
#154322=CARTESIAN_POINT('Ctrl Pts',(-33.8603961679402,13.5628934657056,
127.224115040317)) ;
#154323=CARTESIAN_POINT('Ctrl Pts',(-33.8741810837025,13.5357169129533,
127.155142577645)) ;
#154324=CARTESIAN_POINT('Ctrl Pts',(-33.8704755222901,13.4658311995141,
127.182274454702)) ;
#154325=CARTESIAN_POINT('Ctrl Pts',(-33.8079438763917,13.4658311995141,
127.161214257016)) ;
#154326=CARTESIAN_POINT('Ctrl Pts',(-33.8015609648991,13.3959454860749,
127.187711385949)) ;
#154327=CARTESIAN_POINT('Ctrl Pts',(-33.7810150851566,13.4231220388272,
127.254636339226)) ;
#154328=CARTESIAN_POINT('Ctrl Pts',(-33.760469205414,13.4502985915795,127.321561292503)) ;
#154329=CARTESIAN_POINT('Ctrl Pts',(-33.7668521169066,13.5201843050187,
127.295064163571)) ;
#154330=CARTESIAN_POINT('Ctrl Pts',(-33.7732350283992,13.5900700184578,
127.268567034639)) ;
#154331=CARTESIAN_POINT('Ctrl Pts',(-33.7937809081418,13.5628934657056,
127.201642081362)) ;
#154332=CARTESIAN_POINT('Ctrl Pts',(-33.8143267878844,13.5357169129533,
127.134717128084)) ;
#154333=CARTESIAN_POINT('Ctrl Pts',(-33.8079438763917,13.4658311995141,
127.161214257016)) ;
#154334=CARTESIAN_POINT('Ctrl Pts',(-33.3657216693001,13.4658311995141,
126.490786655428)) ;
#154335=CARTESIAN_POINT('Ctrl Pts',(-33.3710709437106,13.4658311995141,
126.425157509608)) ;
#154336=CARTESIAN_POINT('Ctrl Pts',(-33.4026727151281,13.4658311995141,
126.292213744632)) ;
#154337=CARTESIAN_POINT('Ctrl Pts',(-33.5097508222684,13.4658311995141,
126.114873926673)) ;
#154338=CARTESIAN_POINT('Ctrl Pts',(-33.6669726245832,13.4658311995141,
125.979587612656)) ;
#154339=CARTESIAN_POINT('Ctrl Pts',(-33.8546539670386,13.4658311995141,
125.899837483417)) ;
#154340=CARTESIAN_POINT('Ctrl Pts',(-34.0574909713096,13.4658311995141,
125.879315368324)) ;
#154341=CARTESIAN_POINT('Ctrl Pts',(-34.2603174788621,13.4658311995141,
125.922153820006)) ;
#154342=CARTESIAN_POINT('Ctrl Pts',(-34.4394051996481,13.4658311995141,
126.026010217586)) ;
#154343=CARTESIAN_POINT('Ctrl Pts',(-34.5756161826405,13.4658311995141,
126.176769282622)) ;
#154344=CARTESIAN_POINT('Ctrl Pts',(-34.6605098387667,13.4658311995141,
126.361211761343)) ;
#154345=CARTESIAN_POINT('Ctrl Pts',(-34.6852735030978,13.4658311995141,
126.56639932233)) ;
#154346=CARTESIAN_POINT('Ctrl Pts',(-34.6444773076006,13.4658311995141,
126.769201249595)) ;
#154347=CARTESIAN_POINT('Ctrl Pts',(-34.5453436411495,13.4658311995141,
126.946957684585)) ;
#154348=CARTESIAN_POINT('Ctrl Pts',(-34.397695173349,13.4658311995141,127.087382113455)) ;
#154349=CARTESIAN_POINT('Ctrl Pts',(-34.2109661436266,13.4658311995141,
127.177936318607)) ;
#154350=CARTESIAN_POINT('Ctrl Pts',(-34.0053608811418,13.4658311995141,
127.205905827809)) ;
#154351=CARTESIAN_POINT('Ctrl Pts',(-33.8704755222901,13.4658311995141,
127.182274454702)) ;
#154352=CARTESIAN_POINT('Ctrl Pts',(-33.8079438763917,13.4658311995141,
127.161214257016)) ;
#154353=CARTESIAN_POINT('Origin',(-21.2276309348583,13.4231221026609,127.371750482897)) ;
#154354=CARTESIAN_POINT('Origin',(-23.4026448390223,13.4231221026609,133.725538241056)) ;
#196737=UNCERTAINTY_MEASURE_WITH_UNIT(LENGTH_MEASURE(0.01),#196742,
'DISTANCE_ACCURACY_VALUE',
'Maximum model space distance between geometric entities at asserted c
onnectivities') ;
#196738=UNCERTAINTY_MEASURE_WITH_UNIT(LENGTH_MEASURE(0.01),#196742,
'DISTANCE_ACCURACY_VALUE',
'Maximum model space distance between geometric entities at asserted c
onnectivities') ;
#196740=(
GEOMETRIC_REPRESENTATION_CONTEXT(3)
GLOBAL_UNCERTAINTY_ASSIGNED_CONTEXT((#196737))
GLOBAL_UNIT_ASSIGNED_CONTEXT((#196742,#196744,#196745))
REPRESENTATION_CONTEXT('','3D')
) ;
#196741=(
GEOMETRIC_REPRESENTATION_CONTEXT(3)
GLOBAL_UNCERTAINTY_ASSIGNED_CONTEXT((#196738))
GLOBAL_UNIT_ASSIGNED_CONTEXT((#196742,#196744,#196745))
REPRESENTATION_CONTEXT('','3D')
) ;
#196742=(
LENGTH_UNIT()
NAMED_UNIT(*)
SI_UNIT(.MILLI.,.METRE.)
) ;
#196744=(
NAMED_UNIT(*)
PLANE_ANGLE_UNIT()
SI_UNIT($,.RADIAN.)
) ;
#196745=(
NAMED_UNIT(*)
SI_UNIT($,.STERADIAN.)
SOLID_ANGLE_UNIT()
) ;
#196753=PRODUCT_DEFINITION_CONTEXT('part definition',#196761,'design') ;
#196761=APPLICATION_CONTEXT(
'Core Data for Automotive Mechanical Design Process') ;
#196762=PRODUCT_CONTEXT('part definition',#196761,'mechanical') ;
#196765=PRESENTATION_STYLE_ASSIGNMENT((#196767)) ;
#196767=SURFACE_STYLE_USAGE(.BOTH.,#196769) ;
#196769=SURFACE_SIDE_STYLE('',(#196771)) ;
#196771=SURFACE_STYLE_FILL_AREA(#196773) ;
#196773=FILL_AREA_STYLE('Steel - Satin',(#196775)) ;
#196775=FILL_AREA_STYLE_COLOUR('Steel - Satin',#196777) ;
#196777=COLOUR_RGB('Steel - Satin', 0.09019608, 0.27058824, 0.51372549) ;
#197067=CARTESIAN_POINT ( '', ( 0.0, 0.0, 0.0 ) ) ;
#197068=DIRECTION ( '', ( 0.0, 0.0, 1.0 ) ) ;
#197069=DIRECTION ( '', ( 1.0, 0.0, 0.0 ) ) ;
#197070=AXIS2_PLACEMENT_3D ( '', #197067, #197068, #197069 ) ;
#197071=ADVANCED_BREP_SHAPE_REPRESENTATION ( 'Entry Return Spring', ( #350, #197070, #197081, #197394 ), #196740 ) ;
#197072=PRODUCT( 'Entry Return Spring', 'Entry Return Spring', '', ( #196762 ) ) ;
#197073=PRODUCT_DEFINITION_FORMATION ( '', '', #197072 ) ;
#197074=PRODUCT_DEFINITION( 'Entry Return Spring', 'Entry Return Spring', #197073, #196753 ) ;
#197075=PRODUCT_DEFINITION_SHAPE ( '', '', #197074 ) ;
#197076=SHAPE_DEFINITION_REPRESENTATION ( #197075, #197071 ) ;
#197078=CARTESIAN_POINT ( '', ( 0.0, 0.0, 0.0 ) ) ;
#197079=DIRECTION ( '', ( 0.0, 0.0, 1.0 ) ) ;
#197080=DIRECTION ( '', ( 1.0, 0.0, 0.0 ) ) ;
#197081=AXIS2_PLACEMENT_3D ( '', #197078, #197079, #197080 ) ;
#197391=CARTESIAN_POINT ( '', ( 0.0, 0.0, 0.0 ) ) ;
#197392=DIRECTION ( '', ( 0.0, 0.0, 1.0 ) ) ;
#197393=DIRECTION ( '', ( 1.0, 0.0, 0.0 ) ) ;
#197394=AXIS2_PLACEMENT_3D ( '', #197391, #197392, #197393 ) ;
ENDSEC;
END-ISO-10303-21;
